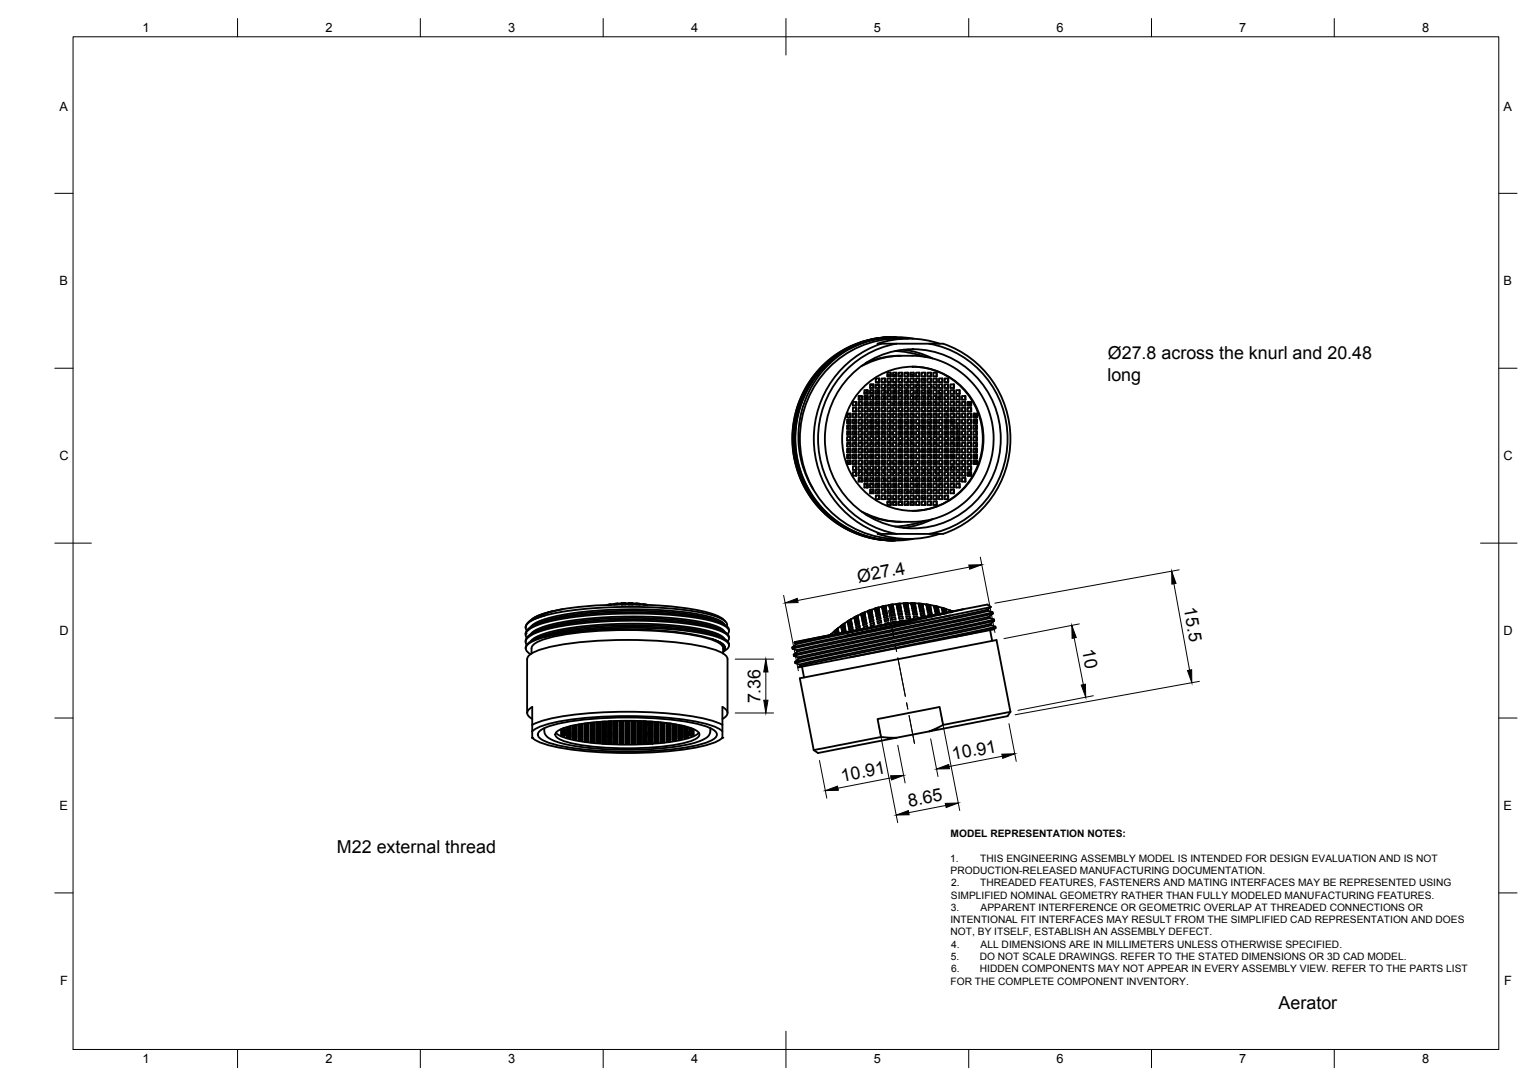
ISO-10303-21;
HEADER;
/* Generated by software containing ST-Developer
 * from STEP Tools, Inc. (www.steptools.com) 
 */

FILE_DESCRIPTION(
/* description */ ('STEP AP214'),
/* implementation_level */ '2;1');

FILE_NAME(
/* name */ 'Aerator.step',
/* time_stamp */ '2026-10-05T23:18:41-07:00',
/* author */ (''),
/* organization */ (''),
/* preprocessor_version */ 'ST-DEVELOPER v20.2',
/* originating_system */ 'Autodesk Translation Framework v15.15.0.0',
/* authorisation */ '');

FILE_SCHEMA (('AUTOMOTIVE_DESIGN { 1 0 10303 214 3 1 1 }'));
ENDSEC;

DATA;
#10=MECHANICAL_DESIGN_GEOMETRIC_PRESENTATION_REPRESENTATION('',(#110),#221662);
#71=MANIFOLD_SOLID_BREP('Body1',#79333);
#84=SHAPE_REPRESENTATION_RELATIONSHIP('SRR','None',#221719,#97);
#97=ADVANCED_BREP_SHAPE_REPRESENTATION('',(#71),#221659);
#110=STYLED_ITEM('',(#221783),#71);
#201=B_SPLINE_SURFACE_WITH_KNOTS('',3,3,((#184914,#184915,#184916,#184917,
#184918,#184919,#184920,#184921,#184922,#184923,#184924,#184925,#184926,
#184927,#184928,#184929,#184930,#184931,#184932,#184933,#184934,#184935,
#184936,#184937,#184938,#184939,#184940,#184941,#184942,#184943,#184944,
#184945,#184946,#184947,#184948),(#184949,#184950,#184951,#184952,#184953,
#184954,#184955,#184956,#184957,#184958,#184959,#184960,#184961,#184962,
#184963,#184964,#184965,#184966,#184967,#184968,#184969,#184970,#184971,
#184972,#184973,#184974,#184975,#184976,#184977,#184978,#184979,#184980,
#184981,#184982,#184983),(#184984,#184985,#184986,#184987,#184988,#184989,
#184990,#184991,#184992,#184993,#184994,#184995,#184996,#184997,#184998,
#184999,#185000,#185001,#185002,#185003,#185004,#185005,#185006,#185007,
#185008,#185009,#185010,#185011,#185012,#185013,#185014,#185015,#185016,
#185017,#185018),(#185019,#185020,#185021,#185022,#185023,#185024,#185025,
#185026,#185027,#185028,#185029,#185030,#185031,#185032,#185033,#185034,
#185035,#185036,#185037,#185038,#185039,#185040,#185041,#185042,#185043,
#185044,#185045,#185046,#185047,#185048,#185049,#185050,#185051,#185052,
#185053)),.UNSPECIFIED.,.F.,.F.,.F.,(4,4),(4,1,1,1,1,1,1,1,1,1,1,1,1,1,
1,1,1,1,1,1,1,1,1,1,1,1,1,1,1,1,1,1,4),(0.,1.),(0.,0.0312500000000065,0.0625000000000025,
0.0937500000000037,0.125000000000005,0.156250000000045,0.187500000000073,
0.218749999999969,0.249999999999997,0.281250000000024,0.312500000000052,
0.343750000000079,0.374999999999975,0.40625,0.43750000000003,0.468750000000058,
0.500000000000085,0.531249999999982,0.562500000000009,0.593750000000036,
0.625000000000064,0.656250000000091,0.687499999999988,0.718750000000015,
0.750000000000043,0.78125000000007,0.812500000000097,0.84375,0.875000000000021,
0.906250000000049,0.937500000000076,0.968750000000104,1.),.UNSPECIFIED.);
#202=B_SPLINE_SURFACE_WITH_KNOTS('',3,3,((#185513,#185514,#185515,#185516,
#185517,#185518,#185519,#185520,#185521,#185522,#185523,#185524,#185525,
#185526,#185527,#185528,#185529,#185530,#185531),(#185532,#185533,#185534,
#185535,#185536,#185537,#185538,#185539,#185540,#185541,#185542,#185543,
#185544,#185545,#185546,#185547,#185548,#185549,#185550),(#185551,#185552,
#185553,#185554,#185555,#185556,#185557,#185558,#185559,#185560,#185561,
#185562,#185563,#185564,#185565,#185566,#185567,#185568,#185569),(#185570,
#185571,#185572,#185573,#185574,#185575,#185576,#185577,#185578,#185579,
#185580,#185581,#185582,#185583,#185584,#185585,#185586,#185587,#185588)),
 .UNSPECIFIED.,.F.,.F.,.F.,(4,4),(4,1,1,1,1,1,1,1,1,1,1,1,1,1,1,1,4),(0.,
1.),(0.,0.0625000000000177,0.124999999999754,0.187499999999772,0.249999999999789,
0.312499999999525,0.374999999999543,0.437499999999561,0.499999999999297,
0.562499999999315,0.624999999999332,0.687499999999069,0.749999999999086,
0.812499999998822,0.87499999999884,0.937499999998858,1.),.UNSPECIFIED.);
#203=B_SPLINE_SURFACE_WITH_KNOTS('',3,3,((#185868,#185869,#185870,#185871,
#185872,#185873,#185874,#185875,#185876,#185877,#185878,#185879,#185880,
#185881,#185882,#185883,#185884,#185885,#185886,#185887,#185888,#185889,
#185890,#185891,#185892,#185893,#185894,#185895,#185896,#185897,#185898,
#185899,#185900,#185901,#185902),(#185903,#185904,#185905,#185906,#185907,
#185908,#185909,#185910,#185911,#185912,#185913,#185914,#185915,#185916,
#185917,#185918,#185919,#185920,#185921,#185922,#185923,#185924,#185925,
#185926,#185927,#185928,#185929,#185930,#185931,#185932,#185933,#185934,
#185935,#185936,#185937),(#185938,#185939,#185940,#185941,#185942,#185943,
#185944,#185945,#185946,#185947,#185948,#185949,#185950,#185951,#185952,
#185953,#185954,#185955,#185956,#185957,#185958,#185959,#185960,#185961,
#185962,#185963,#185964,#185965,#185966,#185967,#185968,#185969,#185970,
#185971,#185972),(#185973,#185974,#185975,#185976,#185977,#185978,#185979,
#185980,#185981,#185982,#185983,#185984,#185985,#185986,#185987,#185988,
#185989,#185990,#185991,#185992,#185993,#185994,#185995,#185996,#185997,
#185998,#185999,#186000,#186001,#186002,#186003,#186004,#186005,#186006,
#186007)),.UNSPECIFIED.,.F.,.F.,.F.,(4,4),(4,1,1,1,1,1,1,1,1,1,1,1,1,1,
1,1,1,1,1,1,1,1,1,1,1,1,1,1,1,1,1,1,4),(0.,1.),(0.,0.0312499999999954,0.0624999999999932,
0.0937499999999958,0.124999999999998,0.15625,0.187500000000028,0.218750000000055,
0.249999999999961,0.281249999999988,0.312500000000014,0.343750000000041,
0.375000000000068,0.406249999999974,0.4375,0.468750000000028,0.500000000000054,
0.531250000000081,0.562499999999987,0.593750000000014,0.625000000000041,
0.656250000000068,0.687499999999974,0.71875,0.750000000000027,0.781250000000054,
0.812500000000081,0.843749999999987,0.875000000000014,0.90625000000004,
0.937500000000067,0.968750000000094,1.),.UNSPECIFIED.);
#204=B_SPLINE_SURFACE_WITH_KNOTS('',3,3,((#186635,#186636,#186637,#186638,
#186639,#186640,#186641,#186642,#186643,#186644,#186645,#186646,#186647,
#186648,#186649,#186650,#186651,#186652,#186653,#186654,#186655,#186656,
#186657,#186658,#186659,#186660,#186661,#186662,#186663,#186664,#186665,
#186666,#186667,#186668,#186669,#186670,#186671,#186672,#186673,#186674,
#186675,#186676,#186677,#186678,#186679,#186680,#186681,#186682,#186683,
#186684,#186685,#186686,#186687,#186688,#186689,#186690,#186691,#186692,
#186693,#186694,#186695,#186696,#186697,#186698,#186699,#186700,#186701),
(#186702,#186703,#186704,#186705,#186706,#186707,#186708,#186709,#186710,
#186711,#186712,#186713,#186714,#186715,#186716,#186717,#186718,#186719,
#186720,#186721,#186722,#186723,#186724,#186725,#186726,#186727,#186728,
#186729,#186730,#186731,#186732,#186733,#186734,#186735,#186736,#186737,
#186738,#186739,#186740,#186741,#186742,#186743,#186744,#186745,#186746,
#186747,#186748,#186749,#186750,#186751,#186752,#186753,#186754,#186755,
#186756,#186757,#186758,#186759,#186760,#186761,#186762,#186763,#186764,
#186765,#186766,#186767,#186768),(#186769,#186770,#186771,#186772,#186773,
#186774,#186775,#186776,#186777,#186778,#186779,#186780,#186781,#186782,
#186783,#186784,#186785,#186786,#186787,#186788,#186789,#186790,#186791,
#186792,#186793,#186794,#186795,#186796,#186797,#186798,#186799,#186800,
#186801,#186802,#186803,#186804,#186805,#186806,#186807,#186808,#186809,
#186810,#186811,#186812,#186813,#186814,#186815,#186816,#186817,#186818,
#186819,#186820,#186821,#186822,#186823,#186824,#186825,#186826,#186827,
#186828,#186829,#186830,#186831,#186832,#186833,#186834,#186835),(#186836,
#186837,#186838,#186839,#186840,#186841,#186842,#186843,#186844,#186845,
#186846,#186847,#186848,#186849,#186850,#186851,#186852,#186853,#186854,
#186855,#186856,#186857,#186858,#186859,#186860,#186861,#186862,#186863,
#186864,#186865,#186866,#186867,#186868,#186869,#186870,#186871,#186872,
#186873,#186874,#186875,#186876,#186877,#186878,#186879,#186880,#186881,
#186882,#186883,#186884,#186885,#186886,#186887,#186888,#186889,#186890,
#186891,#186892,#186893,#186894,#186895,#186896,#186897,#186898,#186899,
#186900,#186901,#186902)),.UNSPECIFIED.,.F.,.F.,.F.,(4,4),(4,1,1,1,1,1,
1,1,1,1,1,1,1,1,1,1,1,1,1,1,1,1,1,1,1,1,1,1,1,1,1,1,1,1,1,1,1,1,1,1,1,1,
1,1,1,1,1,1,1,1,1,1,1,1,1,1,1,1,1,1,1,1,1,1,4),(0.,1.),(0.,0.0156250000000016,
0.031250000000001,0.0468750000000015,0.062500000000002,0.0781250000000025,
0.093750000000003,0.109375000000004,0.125000000000004,0.140625000000026,
0.156249999999973,0.171875000000027,0.187499999999974,0.203125000000028,
0.218749999999975,0.234375000000029,0.249999999999976,0.26562500000003,
0.281249999999977,0.296875000000031,0.312499999999978,0.328125000000032,
0.343749999999979,0.359375000000033,0.37499999999998,0.390625000000034,
0.406249999999981,0.421875000000035,0.437499999999982,0.453125000000036,
0.468749999999983,0.484375000000037,0.499999999999984,0.515625000000038,
0.531249999999985,0.546875000000039,0.562499999999986,0.57812500000004,
0.593749999999987,0.609375000000041,0.624999999999988,0.640625000000042,
0.656249999999989,0.671875000000043,0.68749999999999,0.703125000000044,
0.718749999999991,0.734375000000045,0.749999999999992,0.765625000000046,
0.78125,0.796875000000047,0.8125,0.828125000000048,0.84375,0.859374999999941,
0.875,0.890624999999943,0.90625,0.921874999999943,0.9375,0.953124999999945,
0.96875,0.984374999999945,1.),.UNSPECIFIED.);
#205=B_SPLINE_SURFACE_WITH_KNOTS('',3,3,((#186905,#186906,#186907,#186908,
#186909,#186910,#186911,#186912,#186913,#186914,#186915,#186916,#186917,
#186918,#186919,#186920,#186921,#186922,#186923),(#186924,#186925,#186926,
#186927,#186928,#186929,#186930,#186931,#186932,#186933,#186934,#186935,
#186936,#186937,#186938,#186939,#186940,#186941,#186942),(#186943,#186944,
#186945,#186946,#186947,#186948,#186949,#186950,#186951,#186952,#186953,
#186954,#186955,#186956,#186957,#186958,#186959,#186960,#186961),(#186962,
#186963,#186964,#186965,#186966,#186967,#186968,#186969,#186970,#186971,
#186972,#186973,#186974,#186975,#186976,#186977,#186978,#186979,#186980)),
 .UNSPECIFIED.,.F.,.F.,.F.,(4,4),(4,1,1,1,1,1,1,1,1,1,1,1,1,1,1,1,4),(0.,
1.),(0.,0.062499999999931,0.124999999999862,0.187500000000069,0.25,0.312499999999931,
0.374999999999862,0.437499999999793,0.499999999999724,0.562499999999931,
0.624999999999862,0.687499999999793,0.749999999999724,0.812499999999656,
0.874999999999587,0.937499999999793,1.),.UNSPECIFIED.);
#206=B_SPLINE_SURFACE_WITH_KNOTS('',3,3,((#186987,#186988,#186989,#186990,
#186991,#186992,#186993,#186994,#186995,#186996,#186997,#186998,#186999,
#187000,#187001,#187002,#187003,#187004,#187005),(#187006,#187007,#187008,
#187009,#187010,#187011,#187012,#187013,#187014,#187015,#187016,#187017,
#187018,#187019,#187020,#187021,#187022,#187023,#187024),(#187025,#187026,
#187027,#187028,#187029,#187030,#187031,#187032,#187033,#187034,#187035,
#187036,#187037,#187038,#187039,#187040,#187041,#187042,#187043),(#187044,
#187045,#187046,#187047,#187048,#187049,#187050,#187051,#187052,#187053,
#187054,#187055,#187056,#187057,#187058,#187059,#187060,#187061,#187062)),
 .UNSPECIFIED.,.F.,.F.,.F.,(4,4),(4,1,1,1,1,1,1,1,1,1,1,1,1,1,1,1,4),(0.,
1.),(0.,0.0625000000000641,0.125000000000129,0.18749999999985,0.249999999999914,
0.312499999999979,0.3749999999997,0.437499999999764,0.499999999999828,0.562499999999549,
0.624999999999614,0.687499999999335,0.749999999999399,0.812499999999464,
0.874999999999185,0.937499999999249,1.),.UNSPECIFIED.);
#319=FACE_BOUND('',#24953,.T.);
#320=FACE_BOUND('',#24954,.T.);
#321=FACE_BOUND('',#24955,.T.);
#322=FACE_BOUND('',#24959,.T.);
#323=FACE_BOUND('',#24960,.T.);
#324=FACE_BOUND('',#24961,.T.);
#325=FACE_BOUND('',#24984,.T.);
#326=FACE_BOUND('',#24986,.T.);
#327=FACE_BOUND('',#24992,.T.);
#328=FACE_BOUND('',#24994,.T.);
#329=FACE_BOUND('',#24996,.T.);
#330=FACE_BOUND('',#26056,.T.);
#331=FACE_BOUND('',#27802,.T.);
#332=FACE_BOUND('',#27804,.T.);
#333=FACE_BOUND('',#27805,.T.);
#334=FACE_BOUND('',#27806,.T.);
#335=FACE_BOUND('',#27807,.T.);
#336=FACE_BOUND('',#27808,.T.);
#337=FACE_BOUND('',#27809,.T.);
#338=FACE_BOUND('',#27810,.T.);
#339=FACE_BOUND('',#27811,.T.);
#340=FACE_BOUND('',#27812,.T.);
#341=FACE_BOUND('',#27813,.T.);
#342=FACE_BOUND('',#27814,.T.);
#343=FACE_BOUND('',#27815,.T.);
#344=FACE_BOUND('',#27816,.T.);
#345=FACE_BOUND('',#27817,.T.);
#346=FACE_BOUND('',#27818,.T.);
#347=FACE_BOUND('',#27819,.T.);
#348=FACE_BOUND('',#27820,.T.);
#349=FACE_BOUND('',#27821,.T.);
#350=FACE_BOUND('',#27822,.T.);
#351=FACE_BOUND('',#27823,.T.);
#352=FACE_BOUND('',#27824,.T.);
#353=FACE_BOUND('',#27825,.T.);
#354=FACE_BOUND('',#27826,.T.);
#355=FACE_BOUND('',#27827,.T.);
#356=FACE_BOUND('',#27828,.T.);
#357=FACE_BOUND('',#27829,.T.);
#358=FACE_BOUND('',#27830,.T.);
#359=FACE_BOUND('',#27831,.T.);
#360=FACE_BOUND('',#27832,.T.);
#361=FACE_BOUND('',#27833,.T.);
#362=FACE_BOUND('',#27834,.T.);
#363=FACE_BOUND('',#27835,.T.);
#364=FACE_BOUND('',#27836,.T.);
#365=FACE_BOUND('',#27837,.T.);
#366=FACE_BOUND('',#27838,.T.);
#367=FACE_BOUND('',#27839,.T.);
#368=FACE_BOUND('',#27840,.T.);
#369=FACE_BOUND('',#27841,.T.);
#370=FACE_BOUND('',#27842,.T.);
#371=FACE_BOUND('',#27843,.T.);
#372=FACE_BOUND('',#27844,.T.);
#373=FACE_BOUND('',#27845,.T.);
#374=FACE_BOUND('',#27846,.T.);
#375=FACE_BOUND('',#27847,.T.);
#376=FACE_BOUND('',#27848,.T.);
#377=FACE_BOUND('',#27849,.T.);
#378=FACE_BOUND('',#27850,.T.);
#379=FACE_BOUND('',#27851,.T.);
#380=FACE_BOUND('',#27852,.T.);
#381=FACE_BOUND('',#27853,.T.);
#382=FACE_BOUND('',#27854,.T.);
#383=FACE_BOUND('',#27855,.T.);
#384=FACE_BOUND('',#27856,.T.);
#385=FACE_BOUND('',#27857,.T.);
#386=FACE_BOUND('',#27858,.T.);
#387=FACE_BOUND('',#27859,.T.);
#388=FACE_BOUND('',#27860,.T.);
#389=FACE_BOUND('',#27861,.T.);
#390=FACE_BOUND('',#27862,.T.);
#391=FACE_BOUND('',#27863,.T.);
#392=FACE_BOUND('',#27864,.T.);
#393=FACE_BOUND('',#27865,.T.);
#394=FACE_BOUND('',#27866,.T.);
#395=FACE_BOUND('',#27867,.T.);
#396=FACE_BOUND('',#27868,.T.);
#397=FACE_BOUND('',#27869,.T.);
#398=FACE_BOUND('',#27870,.T.);
#399=FACE_BOUND('',#27871,.T.);
#400=FACE_BOUND('',#27872,.T.);
#401=FACE_BOUND('',#27873,.T.);
#402=FACE_BOUND('',#27874,.T.);
#403=FACE_BOUND('',#27875,.T.);
#404=FACE_BOUND('',#27876,.T.);
#405=FACE_BOUND('',#27877,.T.);
#406=FACE_BOUND('',#27878,.T.);
#407=FACE_BOUND('',#27879,.T.);
#408=FACE_BOUND('',#27880,.T.);
#409=FACE_BOUND('',#27881,.T.);
#410=FACE_BOUND('',#27882,.T.);
#411=FACE_BOUND('',#27883,.T.);
#412=FACE_BOUND('',#27884,.T.);
#413=FACE_BOUND('',#27885,.T.);
#414=FACE_BOUND('',#27886,.T.);
#415=FACE_BOUND('',#27887,.T.);
#416=FACE_BOUND('',#27888,.T.);
#417=FACE_BOUND('',#27889,.T.);
#418=FACE_BOUND('',#27890,.T.);
#419=FACE_BOUND('',#27891,.T.);
#420=FACE_BOUND('',#27892,.T.);
#421=FACE_BOUND('',#27893,.T.);
#422=FACE_BOUND('',#27894,.T.);
#423=FACE_BOUND('',#27895,.T.);
#424=FACE_BOUND('',#27896,.T.);
#425=FACE_BOUND('',#27897,.T.);
#426=FACE_BOUND('',#27898,.T.);
#427=FACE_BOUND('',#27899,.T.);
#428=FACE_BOUND('',#27900,.T.);
#429=FACE_BOUND('',#27901,.T.);
#430=FACE_BOUND('',#27902,.T.);
#431=FACE_BOUND('',#27903,.T.);
#432=FACE_BOUND('',#27904,.T.);
#433=FACE_BOUND('',#27905,.T.);
#434=FACE_BOUND('',#27906,.T.);
#435=FACE_BOUND('',#27907,.T.);
#436=FACE_BOUND('',#27908,.T.);
#437=FACE_BOUND('',#27909,.T.);
#438=FACE_BOUND('',#27910,.T.);
#439=FACE_BOUND('',#27911,.T.);
#440=FACE_BOUND('',#27912,.T.);
#441=FACE_BOUND('',#27913,.T.);
#442=FACE_BOUND('',#27914,.T.);
#443=FACE_BOUND('',#27915,.T.);
#444=FACE_BOUND('',#27916,.T.);
#445=FACE_BOUND('',#27917,.T.);
#446=FACE_BOUND('',#27918,.T.);
#447=FACE_BOUND('',#27919,.T.);
#448=FACE_BOUND('',#27920,.T.);
#449=FACE_BOUND('',#27921,.T.);
#450=FACE_BOUND('',#27922,.T.);
#451=FACE_BOUND('',#27923,.T.);
#452=FACE_BOUND('',#27924,.T.);
#453=FACE_BOUND('',#27925,.T.);
#454=FACE_BOUND('',#27926,.T.);
#455=FACE_BOUND('',#27927,.T.);
#456=FACE_BOUND('',#27928,.T.);
#457=FACE_BOUND('',#27929,.T.);
#458=FACE_BOUND('',#27930,.T.);
#459=FACE_BOUND('',#27931,.T.);
#460=FACE_BOUND('',#27932,.T.);
#461=FACE_BOUND('',#27933,.T.);
#462=FACE_BOUND('',#27934,.T.);
#463=FACE_BOUND('',#27935,.T.);
#464=FACE_BOUND('',#27936,.T.);
#465=FACE_BOUND('',#27937,.T.);
#466=FACE_BOUND('',#27938,.T.);
#467=FACE_BOUND('',#27939,.T.);
#468=FACE_BOUND('',#27940,.T.);
#469=FACE_BOUND('',#27941,.T.);
#470=FACE_BOUND('',#27942,.T.);
#471=FACE_BOUND('',#27943,.T.);
#472=FACE_BOUND('',#27944,.T.);
#473=FACE_BOUND('',#27945,.T.);
#474=FACE_BOUND('',#27946,.T.);
#475=FACE_BOUND('',#27947,.T.);
#476=FACE_BOUND('',#27948,.T.);
#477=FACE_BOUND('',#27949,.T.);
#478=FACE_BOUND('',#27950,.T.);
#479=FACE_BOUND('',#27951,.T.);
#480=FACE_BOUND('',#27952,.T.);
#481=FACE_BOUND('',#27953,.T.);
#482=FACE_BOUND('',#27954,.T.);
#483=FACE_BOUND('',#27955,.T.);
#484=FACE_BOUND('',#27956,.T.);
#485=FACE_BOUND('',#27957,.T.);
#486=FACE_BOUND('',#27958,.T.);
#487=FACE_BOUND('',#27959,.T.);
#488=FACE_BOUND('',#27960,.T.);
#489=FACE_BOUND('',#27961,.T.);
#490=FACE_BOUND('',#27962,.T.);
#491=FACE_BOUND('',#27963,.T.);
#492=FACE_BOUND('',#27964,.T.);
#493=FACE_BOUND('',#27965,.T.);
#494=FACE_BOUND('',#27966,.T.);
#495=FACE_BOUND('',#27967,.T.);
#496=FACE_BOUND('',#27968,.T.);
#497=FACE_BOUND('',#27969,.T.);
#498=FACE_BOUND('',#27970,.T.);
#499=FACE_BOUND('',#27971,.T.);
#500=FACE_BOUND('',#27972,.T.);
#501=FACE_BOUND('',#27973,.T.);
#502=FACE_BOUND('',#27974,.T.);
#503=FACE_BOUND('',#27975,.T.);
#504=FACE_BOUND('',#27976,.T.);
#505=FACE_BOUND('',#27977,.T.);
#506=FACE_BOUND('',#27978,.T.);
#507=FACE_BOUND('',#27979,.T.);
#508=FACE_BOUND('',#27980,.T.);
#509=FACE_BOUND('',#27981,.T.);
#510=FACE_BOUND('',#27982,.T.);
#511=FACE_BOUND('',#27983,.T.);
#512=FACE_BOUND('',#27984,.T.);
#513=FACE_BOUND('',#27985,.T.);
#514=FACE_BOUND('',#27986,.T.);
#515=FACE_BOUND('',#27987,.T.);
#516=FACE_BOUND('',#27988,.T.);
#517=FACE_BOUND('',#27989,.T.);
#518=FACE_BOUND('',#27990,.T.);
#519=FACE_BOUND('',#27991,.T.);
#520=FACE_BOUND('',#27992,.T.);
#521=FACE_BOUND('',#27993,.T.);
#522=FACE_BOUND('',#27994,.T.);
#523=FACE_BOUND('',#27995,.T.);
#524=FACE_BOUND('',#27996,.T.);
#525=FACE_BOUND('',#27997,.T.);
#526=FACE_BOUND('',#27998,.T.);
#527=FACE_BOUND('',#27999,.T.);
#528=FACE_BOUND('',#28000,.T.);
#529=FACE_BOUND('',#28001,.T.);
#530=FACE_BOUND('',#28002,.T.);
#531=FACE_BOUND('',#28003,.T.);
#532=FACE_BOUND('',#28004,.T.);
#533=FACE_BOUND('',#28005,.T.);
#534=FACE_BOUND('',#28006,.T.);
#535=FACE_BOUND('',#28007,.T.);
#536=FACE_BOUND('',#28008,.T.);
#537=FACE_BOUND('',#28009,.T.);
#538=FACE_BOUND('',#28010,.T.);
#539=FACE_BOUND('',#28011,.T.);
#540=FACE_BOUND('',#28012,.T.);
#541=FACE_BOUND('',#28013,.T.);
#542=FACE_BOUND('',#28014,.T.);
#543=FACE_BOUND('',#28015,.T.);
#544=FACE_BOUND('',#28016,.T.);
#545=FACE_BOUND('',#28017,.T.);
#546=FACE_BOUND('',#28018,.T.);
#547=FACE_BOUND('',#28019,.T.);
#548=FACE_BOUND('',#28020,.T.);
#549=FACE_BOUND('',#28021,.T.);
#550=FACE_BOUND('',#28022,.T.);
#551=FACE_BOUND('',#28023,.T.);
#552=FACE_BOUND('',#28024,.T.);
#553=FACE_BOUND('',#28025,.T.);
#554=FACE_BOUND('',#28026,.T.);
#555=FACE_BOUND('',#28027,.T.);
#556=FACE_BOUND('',#28028,.T.);
#557=FACE_BOUND('',#28029,.T.);
#558=FACE_BOUND('',#28030,.T.);
#559=FACE_BOUND('',#28031,.T.);
#560=FACE_BOUND('',#28032,.T.);
#561=FACE_BOUND('',#28033,.T.);
#562=FACE_BOUND('',#28034,.T.);
#563=FACE_BOUND('',#28035,.T.);
#564=FACE_BOUND('',#28036,.T.);
#565=FACE_BOUND('',#28037,.T.);
#566=FACE_BOUND('',#28038,.T.);
#567=FACE_BOUND('',#28039,.T.);
#568=FACE_BOUND('',#28040,.T.);
#569=FACE_BOUND('',#28041,.T.);
#570=FACE_BOUND('',#28042,.T.);
#571=FACE_BOUND('',#28043,.T.);
#572=FACE_BOUND('',#28044,.T.);
#573=FACE_BOUND('',#28045,.T.);
#574=FACE_BOUND('',#28046,.T.);
#575=FACE_BOUND('',#28047,.T.);
#576=FACE_BOUND('',#28048,.T.);
#577=FACE_BOUND('',#28049,.T.);
#578=FACE_BOUND('',#28050,.T.);
#579=FACE_BOUND('',#28051,.T.);
#580=FACE_BOUND('',#28052,.T.);
#581=FACE_BOUND('',#28053,.T.);
#582=FACE_BOUND('',#28054,.T.);
#583=FACE_BOUND('',#28055,.T.);
#584=FACE_BOUND('',#28056,.T.);
#585=FACE_BOUND('',#28057,.T.);
#586=FACE_BOUND('',#28058,.T.);
#587=FACE_BOUND('',#28059,.T.);
#588=FACE_BOUND('',#28060,.T.);
#589=FACE_BOUND('',#28061,.T.);
#590=FACE_BOUND('',#28062,.T.);
#591=FACE_BOUND('',#28063,.T.);
#592=FACE_BOUND('',#28064,.T.);
#593=FACE_BOUND('',#28065,.T.);
#594=FACE_BOUND('',#28066,.T.);
#595=FACE_BOUND('',#28067,.T.);
#596=FACE_BOUND('',#28068,.T.);
#597=FACE_BOUND('',#28069,.T.);
#598=FACE_BOUND('',#28070,.T.);
#599=FACE_BOUND('',#28071,.T.);
#600=FACE_BOUND('',#28072,.T.);
#601=FACE_BOUND('',#28073,.T.);
#602=FACE_BOUND('',#28074,.T.);
#603=FACE_BOUND('',#28075,.T.);
#604=FACE_BOUND('',#28076,.T.);
#605=FACE_BOUND('',#28077,.T.);
#606=FACE_BOUND('',#28078,.T.);
#607=FACE_BOUND('',#28079,.T.);
#608=FACE_BOUND('',#28080,.T.);
#609=FACE_BOUND('',#28081,.T.);
#610=FACE_BOUND('',#28082,.T.);
#611=FACE_BOUND('',#28083,.T.);
#612=FACE_BOUND('',#28084,.T.);
#613=FACE_BOUND('',#28085,.T.);
#614=FACE_BOUND('',#28086,.T.);
#615=FACE_BOUND('',#28087,.T.);
#616=FACE_BOUND('',#28088,.T.);
#617=FACE_BOUND('',#28089,.T.);
#618=FACE_BOUND('',#28090,.T.);
#619=FACE_BOUND('',#28091,.T.);
#620=FACE_BOUND('',#28092,.T.);
#621=FACE_BOUND('',#28093,.T.);
#622=FACE_BOUND('',#28094,.T.);
#623=FACE_BOUND('',#28095,.T.);
#624=FACE_BOUND('',#28096,.T.);
#625=FACE_BOUND('',#28097,.T.);
#626=FACE_BOUND('',#28098,.T.);
#627=FACE_BOUND('',#28099,.T.);
#628=FACE_BOUND('',#28100,.T.);
#629=FACE_BOUND('',#28101,.T.);
#630=FACE_BOUND('',#28102,.T.);
#631=FACE_BOUND('',#28103,.T.);
#632=FACE_BOUND('',#28104,.T.);
#633=FACE_BOUND('',#28105,.T.);
#634=FACE_BOUND('',#28106,.T.);
#635=FACE_BOUND('',#28107,.T.);
#636=FACE_BOUND('',#28108,.T.);
#637=FACE_BOUND('',#28109,.T.);
#638=FACE_BOUND('',#28110,.T.);
#639=FACE_BOUND('',#28111,.T.);
#640=FACE_BOUND('',#28112,.T.);
#641=FACE_BOUND('',#28113,.T.);
#642=FACE_BOUND('',#28114,.T.);
#643=FACE_BOUND('',#28115,.T.);
#644=FACE_BOUND('',#28116,.T.);
#645=FACE_BOUND('',#28117,.T.);
#646=FACE_BOUND('',#28118,.T.);
#647=FACE_BOUND('',#28119,.T.);
#648=FACE_BOUND('',#28120,.T.);
#649=FACE_BOUND('',#28121,.T.);
#650=FACE_BOUND('',#28122,.T.);
#651=FACE_BOUND('',#28123,.T.);
#652=FACE_BOUND('',#28124,.T.);
#653=FACE_BOUND('',#28125,.T.);
#654=FACE_BOUND('',#28126,.T.);
#655=FACE_BOUND('',#28127,.T.);
#656=FACE_BOUND('',#28128,.T.);
#657=FACE_BOUND('',#28129,.T.);
#658=FACE_BOUND('',#28130,.T.);
#659=FACE_BOUND('',#28131,.T.);
#660=FACE_BOUND('',#28132,.T.);
#661=FACE_BOUND('',#28133,.T.);
#662=FACE_BOUND('',#28134,.T.);
#663=FACE_BOUND('',#28135,.T.);
#664=FACE_BOUND('',#28136,.T.);
#665=FACE_BOUND('',#28137,.T.);
#666=FACE_BOUND('',#28138,.T.);
#667=FACE_BOUND('',#28139,.T.);
#668=FACE_BOUND('',#28140,.T.);
#669=FACE_BOUND('',#28141,.T.);
#670=FACE_BOUND('',#28142,.T.);
#671=FACE_BOUND('',#28143,.T.);
#672=FACE_BOUND('',#28144,.T.);
#673=FACE_BOUND('',#28145,.T.);
#674=FACE_BOUND('',#28146,.T.);
#675=FACE_BOUND('',#28147,.T.);
#676=FACE_BOUND('',#28148,.T.);
#677=FACE_BOUND('',#28149,.T.);
#678=FACE_BOUND('',#28150,.T.);
#679=FACE_BOUND('',#28151,.T.);
#680=FACE_BOUND('',#28152,.T.);
#681=FACE_BOUND('',#28153,.T.);
#682=FACE_BOUND('',#28154,.T.);
#683=FACE_BOUND('',#28155,.T.);
#684=FACE_BOUND('',#28156,.T.);
#685=FACE_BOUND('',#28157,.T.);
#686=FACE_BOUND('',#28158,.T.);
#687=FACE_BOUND('',#28159,.T.);
#688=FACE_BOUND('',#28160,.T.);
#689=FACE_BOUND('',#28161,.T.);
#690=FACE_BOUND('',#28162,.T.);
#691=FACE_BOUND('',#28163,.T.);
#692=FACE_BOUND('',#28164,.T.);
#693=FACE_BOUND('',#28165,.T.);
#694=FACE_BOUND('',#28166,.T.);
#695=FACE_BOUND('',#28167,.T.);
#696=FACE_BOUND('',#28168,.T.);
#697=FACE_BOUND('',#28169,.T.);
#698=FACE_BOUND('',#28170,.T.);
#699=FACE_BOUND('',#28171,.T.);
#700=FACE_BOUND('',#28172,.T.);
#701=FACE_BOUND('',#28173,.T.);
#702=FACE_BOUND('',#28174,.T.);
#703=FACE_BOUND('',#28175,.T.);
#704=FACE_BOUND('',#28176,.T.);
#705=FACE_BOUND('',#28177,.T.);
#706=FACE_BOUND('',#28178,.T.);
#707=FACE_BOUND('',#28179,.T.);
#708=FACE_BOUND('',#28180,.T.);
#709=FACE_BOUND('',#28181,.T.);
#710=FACE_BOUND('',#28182,.T.);
#711=FACE_BOUND('',#28183,.T.);
#712=FACE_BOUND('',#28184,.T.);
#713=FACE_BOUND('',#28185,.T.);
#714=FACE_BOUND('',#28186,.T.);
#715=FACE_BOUND('',#28187,.T.);
#716=FACE_BOUND('',#28188,.T.);
#717=FACE_BOUND('',#28189,.T.);
#718=FACE_BOUND('',#28190,.T.);
#719=FACE_BOUND('',#28191,.T.);
#720=FACE_BOUND('',#28192,.T.);
#721=FACE_BOUND('',#28193,.T.);
#722=FACE_BOUND('',#28194,.T.);
#723=FACE_BOUND('',#28195,.T.);
#724=FACE_BOUND('',#28196,.T.);
#725=FACE_BOUND('',#28197,.T.);
#726=FACE_BOUND('',#28198,.T.);
#727=FACE_BOUND('',#28199,.T.);
#728=FACE_BOUND('',#28200,.T.);
#729=FACE_BOUND('',#28201,.T.);
#730=FACE_BOUND('',#28202,.T.);
#731=FACE_BOUND('',#28203,.T.);
#732=FACE_BOUND('',#28204,.T.);
#733=FACE_BOUND('',#28205,.T.);
#734=FACE_BOUND('',#28206,.T.);
#735=FACE_BOUND('',#28207,.T.);
#736=FACE_BOUND('',#28208,.T.);
#737=FACE_BOUND('',#28209,.T.);
#738=FACE_BOUND('',#28210,.T.);
#739=FACE_BOUND('',#28211,.T.);
#740=FACE_BOUND('',#28212,.T.);
#741=FACE_BOUND('',#28213,.T.);
#742=FACE_BOUND('',#28214,.T.);
#743=FACE_BOUND('',#28215,.T.);
#744=FACE_BOUND('',#28216,.T.);
#745=FACE_BOUND('',#28217,.T.);
#746=FACE_BOUND('',#28218,.T.);
#747=FACE_BOUND('',#28219,.T.);
#748=FACE_BOUND('',#28220,.T.);
#749=FACE_BOUND('',#28221,.T.);
#750=FACE_BOUND('',#28222,.T.);
#751=FACE_BOUND('',#28223,.T.);
#752=FACE_BOUND('',#28224,.T.);
#753=FACE_BOUND('',#28225,.T.);
#754=FACE_BOUND('',#28226,.T.);
#755=FACE_BOUND('',#28227,.T.);
#756=FACE_BOUND('',#28228,.T.);
#757=FACE_BOUND('',#28229,.T.);
#758=FACE_BOUND('',#28230,.T.);
#759=FACE_BOUND('',#28231,.T.);
#760=FACE_BOUND('',#28232,.T.);
#761=FACE_BOUND('',#28233,.T.);
#762=FACE_BOUND('',#28234,.T.);
#763=FACE_BOUND('',#28235,.T.);
#764=FACE_BOUND('',#28236,.T.);
#765=FACE_BOUND('',#28237,.T.);
#766=FACE_BOUND('',#28238,.T.);
#767=FACE_BOUND('',#28239,.T.);
#768=FACE_BOUND('',#28240,.T.);
#769=FACE_BOUND('',#28246,.T.);
#770=FACE_BOUND('',#28247,.T.);
#771=FACE_BOUND('',#28248,.T.);
#772=FACE_BOUND('',#28249,.T.);
#773=FACE_BOUND('',#28250,.T.);
#774=FACE_BOUND('',#28251,.T.);
#775=FACE_BOUND('',#28252,.T.);
#776=FACE_BOUND('',#28253,.T.);
#777=FACE_BOUND('',#28254,.T.);
#778=FACE_BOUND('',#28255,.T.);
#779=FACE_BOUND('',#28256,.T.);
#780=FACE_BOUND('',#28257,.T.);
#781=FACE_BOUND('',#28258,.T.);
#782=FACE_BOUND('',#28259,.T.);
#783=FACE_BOUND('',#28260,.T.);
#784=FACE_BOUND('',#28261,.T.);
#785=FACE_BOUND('',#28262,.T.);
#786=FACE_BOUND('',#28263,.T.);
#787=FACE_BOUND('',#28264,.T.);
#788=FACE_BOUND('',#28265,.T.);
#789=FACE_BOUND('',#28266,.T.);
#790=FACE_BOUND('',#28267,.T.);
#791=FACE_BOUND('',#28268,.T.);
#792=FACE_BOUND('',#28269,.T.);
#793=FACE_BOUND('',#28270,.T.);
#794=FACE_BOUND('',#28271,.T.);
#795=FACE_BOUND('',#28272,.T.);
#796=FACE_BOUND('',#28273,.T.);
#797=FACE_BOUND('',#28274,.T.);
#798=FACE_BOUND('',#28275,.T.);
#799=FACE_BOUND('',#28276,.T.);
#800=FACE_BOUND('',#28277,.T.);
#801=FACE_BOUND('',#28278,.T.);
#802=FACE_BOUND('',#28279,.T.);
#803=FACE_BOUND('',#28280,.T.);
#804=FACE_BOUND('',#28281,.T.);
#805=FACE_BOUND('',#28282,.T.);
#806=FACE_BOUND('',#28283,.T.);
#807=FACE_BOUND('',#28284,.T.);
#808=FACE_BOUND('',#28285,.T.);
#809=FACE_BOUND('',#28286,.T.);
#810=FACE_BOUND('',#28287,.T.);
#811=FACE_BOUND('',#28288,.T.);
#812=FACE_BOUND('',#28289,.T.);
#813=FACE_BOUND('',#28290,.T.);
#814=FACE_BOUND('',#28291,.T.);
#815=FACE_BOUND('',#28292,.T.);
#816=FACE_BOUND('',#28293,.T.);
#817=FACE_BOUND('',#28294,.T.);
#818=FACE_BOUND('',#28295,.T.);
#819=FACE_BOUND('',#28296,.T.);
#820=FACE_BOUND('',#28297,.T.);
#821=FACE_BOUND('',#28298,.T.);
#822=FACE_BOUND('',#28299,.T.);
#823=FACE_BOUND('',#28300,.T.);
#824=FACE_BOUND('',#28301,.T.);
#825=FACE_BOUND('',#28302,.T.);
#826=FACE_BOUND('',#28303,.T.);
#827=FACE_BOUND('',#28304,.T.);
#828=FACE_BOUND('',#28305,.T.);
#829=FACE_BOUND('',#28306,.T.);
#830=FACE_BOUND('',#28307,.T.);
#831=FACE_BOUND('',#28308,.T.);
#832=FACE_BOUND('',#28309,.T.);
#833=FACE_BOUND('',#28310,.T.);
#834=FACE_BOUND('',#28311,.T.);
#835=FACE_BOUND('',#28312,.T.);
#836=FACE_BOUND('',#28313,.T.);
#837=FACE_BOUND('',#28314,.T.);
#838=FACE_BOUND('',#28315,.T.);
#839=FACE_BOUND('',#28316,.T.);
#840=FACE_BOUND('',#28317,.T.);
#841=FACE_BOUND('',#28318,.T.);
#842=FACE_BOUND('',#28319,.T.);
#843=FACE_BOUND('',#28320,.T.);
#844=FACE_BOUND('',#28321,.T.);
#845=FACE_BOUND('',#28322,.T.);
#846=FACE_BOUND('',#28323,.T.);
#847=FACE_BOUND('',#28324,.T.);
#848=FACE_BOUND('',#28325,.T.);
#849=FACE_BOUND('',#28326,.T.);
#850=FACE_BOUND('',#28327,.T.);
#851=FACE_BOUND('',#28328,.T.);
#852=FACE_BOUND('',#28329,.T.);
#853=FACE_BOUND('',#28330,.T.);
#854=FACE_BOUND('',#28331,.T.);
#855=FACE_BOUND('',#28332,.T.);
#856=FACE_BOUND('',#28333,.T.);
#857=FACE_BOUND('',#28334,.T.);
#858=FACE_BOUND('',#28335,.T.);
#859=FACE_BOUND('',#28336,.T.);
#860=FACE_BOUND('',#28337,.T.);
#861=FACE_BOUND('',#28338,.T.);
#862=FACE_BOUND('',#28339,.T.);
#863=FACE_BOUND('',#28340,.T.);
#864=FACE_BOUND('',#28341,.T.);
#865=FACE_BOUND('',#28342,.T.);
#866=FACE_BOUND('',#28343,.T.);
#867=FACE_BOUND('',#28344,.T.);
#868=FACE_BOUND('',#28345,.T.);
#869=FACE_BOUND('',#28346,.T.);
#870=FACE_BOUND('',#28347,.T.);
#871=FACE_BOUND('',#28348,.T.);
#872=FACE_BOUND('',#28349,.T.);
#873=FACE_BOUND('',#28350,.T.);
#874=FACE_BOUND('',#28351,.T.);
#875=FACE_BOUND('',#28352,.T.);
#876=FACE_BOUND('',#28353,.T.);
#877=FACE_BOUND('',#28354,.T.);
#878=FACE_BOUND('',#28355,.T.);
#879=FACE_BOUND('',#28356,.T.);
#880=FACE_BOUND('',#28357,.T.);
#881=FACE_BOUND('',#28358,.T.);
#882=FACE_BOUND('',#28359,.T.);
#883=FACE_BOUND('',#28360,.T.);
#884=FACE_BOUND('',#28361,.T.);
#885=FACE_BOUND('',#28362,.T.);
#886=FACE_BOUND('',#28363,.T.);
#887=FACE_BOUND('',#28364,.T.);
#888=FACE_BOUND('',#28365,.T.);
#889=FACE_BOUND('',#28366,.T.);
#890=FACE_BOUND('',#28367,.T.);
#891=FACE_BOUND('',#28368,.T.);
#892=FACE_BOUND('',#28369,.T.);
#893=FACE_BOUND('',#28370,.T.);
#894=FACE_BOUND('',#28371,.T.);
#895=FACE_BOUND('',#28372,.T.);
#896=FACE_BOUND('',#28373,.T.);
#897=FACE_BOUND('',#28374,.T.);
#898=FACE_BOUND('',#28375,.T.);
#899=FACE_BOUND('',#28376,.T.);
#900=FACE_BOUND('',#28377,.T.);
#901=FACE_BOUND('',#28378,.T.);
#902=FACE_BOUND('',#28379,.T.);
#903=FACE_BOUND('',#28380,.T.);
#904=FACE_BOUND('',#28381,.T.);
#905=FACE_BOUND('',#28382,.T.);
#906=FACE_BOUND('',#28383,.T.);
#907=FACE_BOUND('',#28384,.T.);
#908=FACE_BOUND('',#28385,.T.);
#909=FACE_BOUND('',#28386,.T.);
#910=FACE_BOUND('',#28387,.T.);
#911=FACE_BOUND('',#28388,.T.);
#912=FACE_BOUND('',#28389,.T.);
#913=FACE_BOUND('',#28390,.T.);
#914=FACE_BOUND('',#28391,.T.);
#915=FACE_BOUND('',#28392,.T.);
#916=FACE_BOUND('',#28393,.T.);
#917=FACE_BOUND('',#28394,.T.);
#918=FACE_BOUND('',#28395,.T.);
#919=FACE_BOUND('',#28396,.T.);
#920=FACE_BOUND('',#28397,.T.);
#921=FACE_BOUND('',#28398,.T.);
#922=FACE_BOUND('',#28399,.T.);
#923=FACE_BOUND('',#28400,.T.);
#924=FACE_BOUND('',#28401,.T.);
#925=FACE_BOUND('',#28402,.T.);
#926=FACE_BOUND('',#28403,.T.);
#927=FACE_BOUND('',#28404,.T.);
#928=FACE_BOUND('',#28405,.T.);
#929=FACE_BOUND('',#28406,.T.);
#930=FACE_BOUND('',#28407,.T.);
#931=FACE_BOUND('',#28408,.T.);
#932=FACE_BOUND('',#28409,.T.);
#933=FACE_BOUND('',#28410,.T.);
#934=FACE_BOUND('',#28411,.T.);
#935=FACE_BOUND('',#28412,.T.);
#936=FACE_BOUND('',#28413,.T.);
#937=FACE_BOUND('',#28414,.T.);
#938=FACE_BOUND('',#28415,.T.);
#939=FACE_BOUND('',#28416,.T.);
#940=FACE_BOUND('',#28417,.T.);
#941=FACE_BOUND('',#28418,.T.);
#942=FACE_BOUND('',#28419,.T.);
#943=FACE_BOUND('',#28420,.T.);
#944=FACE_BOUND('',#28421,.T.);
#945=FACE_BOUND('',#28422,.T.);
#946=FACE_BOUND('',#28423,.T.);
#947=FACE_BOUND('',#28424,.T.);
#948=FACE_BOUND('',#28425,.T.);
#949=FACE_BOUND('',#28426,.T.);
#950=FACE_BOUND('',#28427,.T.);
#951=FACE_BOUND('',#28428,.T.);
#952=FACE_BOUND('',#28429,.T.);
#953=FACE_BOUND('',#28430,.T.);
#954=FACE_BOUND('',#28431,.T.);
#955=FACE_BOUND('',#28432,.T.);
#956=FACE_BOUND('',#28433,.T.);
#957=FACE_BOUND('',#28434,.T.);
#958=FACE_BOUND('',#28435,.T.);
#959=FACE_BOUND('',#28436,.T.);
#960=FACE_BOUND('',#28437,.T.);
#961=FACE_BOUND('',#28438,.T.);
#962=FACE_BOUND('',#28439,.T.);
#963=FACE_BOUND('',#28440,.T.);
#964=FACE_BOUND('',#28441,.T.);
#965=FACE_BOUND('',#28442,.T.);
#966=FACE_BOUND('',#28443,.T.);
#967=FACE_BOUND('',#28444,.T.);
#968=FACE_BOUND('',#28445,.T.);
#969=FACE_BOUND('',#28446,.T.);
#970=FACE_BOUND('',#28447,.T.);
#971=FACE_BOUND('',#28448,.T.);
#972=FACE_BOUND('',#28449,.T.);
#973=FACE_BOUND('',#28450,.T.);
#974=FACE_BOUND('',#28451,.T.);
#975=FACE_BOUND('',#28452,.T.);
#976=FACE_BOUND('',#28453,.T.);
#977=FACE_BOUND('',#28454,.T.);
#978=FACE_BOUND('',#28455,.T.);
#979=FACE_BOUND('',#28456,.T.);
#980=FACE_BOUND('',#28457,.T.);
#981=FACE_BOUND('',#28458,.T.);
#982=FACE_BOUND('',#28459,.T.);
#983=FACE_BOUND('',#28460,.T.);
#984=FACE_BOUND('',#28461,.T.);
#985=FACE_BOUND('',#28462,.T.);
#986=FACE_BOUND('',#28463,.T.);
#987=FACE_BOUND('',#28464,.T.);
#988=FACE_BOUND('',#28465,.T.);
#989=FACE_BOUND('',#28466,.T.);
#990=FACE_BOUND('',#28467,.T.);
#991=FACE_BOUND('',#28468,.T.);
#992=FACE_BOUND('',#28469,.T.);
#993=FACE_BOUND('',#28470,.T.);
#994=FACE_BOUND('',#28471,.T.);
#995=FACE_BOUND('',#28472,.T.);
#996=FACE_BOUND('',#28473,.T.);
#997=FACE_BOUND('',#28474,.T.);
#998=FACE_BOUND('',#28475,.T.);
#999=FACE_BOUND('',#28476,.T.);
#1000=FACE_BOUND('',#28477,.T.);
#1001=FACE_BOUND('',#28478,.T.);
#1002=FACE_BOUND('',#28479,.T.);
#1003=FACE_BOUND('',#28480,.T.);
#1004=FACE_BOUND('',#28481,.T.);
#1005=FACE_BOUND('',#28482,.T.);
#1006=FACE_BOUND('',#28483,.T.);
#1007=FACE_BOUND('',#28484,.T.);
#1008=FACE_BOUND('',#28485,.T.);
#1009=FACE_BOUND('',#28486,.T.);
#1010=FACE_BOUND('',#28487,.T.);
#1011=FACE_BOUND('',#28488,.T.);
#1012=FACE_BOUND('',#28489,.T.);
#1013=FACE_BOUND('',#28490,.T.);
#1014=FACE_BOUND('',#28491,.T.);
#1015=FACE_BOUND('',#28492,.T.);
#1016=FACE_BOUND('',#28493,.T.);
#1017=FACE_BOUND('',#28494,.T.);
#1018=FACE_BOUND('',#28495,.T.);
#1019=FACE_BOUND('',#28496,.T.);
#1020=FACE_BOUND('',#28497,.T.);
#1021=FACE_BOUND('',#28498,.T.);
#1022=FACE_BOUND('',#28499,.T.);
#1023=FACE_BOUND('',#28500,.T.);
#1024=FACE_BOUND('',#28501,.T.);
#1025=FACE_BOUND('',#28502,.T.);
#1026=FACE_BOUND('',#28503,.T.);
#1027=FACE_BOUND('',#28504,.T.);
#1028=FACE_BOUND('',#28505,.T.);
#1029=FACE_BOUND('',#28506,.T.);
#1030=FACE_BOUND('',#28507,.T.);
#1031=FACE_BOUND('',#28508,.T.);
#1032=FACE_BOUND('',#28509,.T.);
#1033=FACE_BOUND('',#28510,.T.);
#1034=FACE_BOUND('',#28511,.T.);
#1035=FACE_BOUND('',#28512,.T.);
#1036=FACE_BOUND('',#28513,.T.);
#1037=FACE_BOUND('',#28514,.T.);
#1038=FACE_BOUND('',#28515,.T.);
#1039=FACE_BOUND('',#28516,.T.);
#1040=FACE_BOUND('',#28517,.T.);
#1041=FACE_BOUND('',#28518,.T.);
#1042=FACE_BOUND('',#28519,.T.);
#1043=FACE_BOUND('',#28520,.T.);
#1044=FACE_BOUND('',#28521,.T.);
#1045=FACE_BOUND('',#28522,.T.);
#1046=FACE_BOUND('',#28523,.T.);
#1047=FACE_BOUND('',#28524,.T.);
#1048=FACE_BOUND('',#28525,.T.);
#1049=FACE_BOUND('',#28526,.T.);
#1050=FACE_BOUND('',#28527,.T.);
#1051=FACE_BOUND('',#28528,.T.);
#1052=FACE_BOUND('',#28529,.T.);
#1053=FACE_BOUND('',#28530,.T.);
#1054=FACE_BOUND('',#28531,.T.);
#1055=FACE_BOUND('',#28532,.T.);
#1056=FACE_BOUND('',#28533,.T.);
#1057=FACE_BOUND('',#28534,.T.);
#1058=FACE_BOUND('',#28535,.T.);
#1059=FACE_BOUND('',#28536,.T.);
#1060=FACE_BOUND('',#28537,.T.);
#1061=FACE_BOUND('',#28538,.T.);
#1062=FACE_BOUND('',#28539,.T.);
#1063=FACE_BOUND('',#28540,.T.);
#1064=FACE_BOUND('',#28541,.T.);
#1065=FACE_BOUND('',#28542,.T.);
#1066=FACE_BOUND('',#28543,.T.);
#1067=FACE_BOUND('',#28544,.T.);
#1068=FACE_BOUND('',#28545,.T.);
#1069=FACE_BOUND('',#28546,.T.);
#1070=FACE_BOUND('',#28547,.T.);
#1071=FACE_BOUND('',#28548,.T.);
#1072=FACE_BOUND('',#28549,.T.);
#1073=FACE_BOUND('',#28550,.T.);
#1074=FACE_BOUND('',#28551,.T.);
#1075=FACE_BOUND('',#28552,.T.);
#1076=FACE_BOUND('',#28553,.T.);
#1077=FACE_BOUND('',#28554,.T.);
#1078=FACE_BOUND('',#28555,.T.);
#1079=FACE_BOUND('',#28556,.T.);
#1080=FACE_BOUND('',#28557,.T.);
#1081=FACE_BOUND('',#28558,.T.);
#1082=FACE_BOUND('',#28559,.T.);
#1083=FACE_BOUND('',#28560,.T.);
#1084=FACE_BOUND('',#28561,.T.);
#1085=FACE_BOUND('',#28562,.T.);
#1086=FACE_BOUND('',#28563,.T.);
#1087=FACE_BOUND('',#28564,.T.);
#1088=FACE_BOUND('',#28565,.T.);
#1089=FACE_BOUND('',#28566,.T.);
#1090=FACE_BOUND('',#28567,.T.);
#1091=FACE_BOUND('',#28568,.T.);
#1092=FACE_BOUND('',#28569,.T.);
#1093=FACE_BOUND('',#28570,.T.);
#1094=FACE_BOUND('',#28571,.T.);
#1095=FACE_BOUND('',#28572,.T.);
#1096=FACE_BOUND('',#28573,.T.);
#1097=FACE_BOUND('',#28574,.T.);
#1098=FACE_BOUND('',#28575,.T.);
#1099=FACE_BOUND('',#28576,.T.);
#1100=FACE_BOUND('',#28577,.T.);
#1101=FACE_BOUND('',#28578,.T.);
#1102=FACE_BOUND('',#28579,.T.);
#1103=FACE_BOUND('',#28580,.T.);
#1104=FACE_BOUND('',#28581,.T.);
#1105=FACE_BOUND('',#28582,.T.);
#1106=FACE_BOUND('',#28583,.T.);
#1107=FACE_BOUND('',#28584,.T.);
#1108=FACE_BOUND('',#28585,.T.);
#1109=FACE_BOUND('',#28586,.T.);
#1110=FACE_BOUND('',#28587,.T.);
#1111=FACE_BOUND('',#28588,.T.);
#1112=FACE_BOUND('',#28589,.T.);
#1113=FACE_BOUND('',#28590,.T.);
#1114=FACE_BOUND('',#28591,.T.);
#1115=FACE_BOUND('',#28592,.T.);
#1116=FACE_BOUND('',#28593,.T.);
#1117=FACE_BOUND('',#28594,.T.);
#1118=FACE_BOUND('',#28595,.T.);
#1119=FACE_BOUND('',#28596,.T.);
#1120=FACE_BOUND('',#28597,.T.);
#1121=FACE_BOUND('',#28598,.T.);
#1122=FACE_BOUND('',#28599,.T.);
#1123=FACE_BOUND('',#28600,.T.);
#1124=FACE_BOUND('',#28601,.T.);
#1125=FACE_BOUND('',#28602,.T.);
#1126=FACE_BOUND('',#28603,.T.);
#1127=FACE_BOUND('',#28604,.T.);
#1128=FACE_BOUND('',#28605,.T.);
#1129=FACE_BOUND('',#28606,.T.);
#1130=FACE_BOUND('',#28607,.T.);
#1131=FACE_BOUND('',#28608,.T.);
#1132=FACE_BOUND('',#28609,.T.);
#1133=FACE_BOUND('',#28610,.T.);
#1134=FACE_BOUND('',#28611,.T.);
#1135=FACE_BOUND('',#28612,.T.);
#1136=FACE_BOUND('',#28613,.T.);
#1137=FACE_BOUND('',#28614,.T.);
#1138=FACE_BOUND('',#28615,.T.);
#1139=FACE_BOUND('',#28616,.T.);
#1140=FACE_BOUND('',#28617,.T.);
#1141=FACE_BOUND('',#28618,.T.);
#1142=FACE_BOUND('',#28619,.T.);
#1143=FACE_BOUND('',#28620,.T.);
#1144=FACE_BOUND('',#28621,.T.);
#1145=FACE_BOUND('',#28622,.T.);
#1146=FACE_BOUND('',#28623,.T.);
#1147=FACE_BOUND('',#28624,.T.);
#1148=FACE_BOUND('',#28625,.T.);
#1149=FACE_BOUND('',#28626,.T.);
#1150=FACE_BOUND('',#28627,.T.);
#1151=FACE_BOUND('',#28628,.T.);
#1152=FACE_BOUND('',#28629,.T.);
#1153=FACE_BOUND('',#28630,.T.);
#1154=FACE_BOUND('',#28631,.T.);
#1155=FACE_BOUND('',#28632,.T.);
#1156=FACE_BOUND('',#28633,.T.);
#1157=FACE_BOUND('',#28634,.T.);
#1158=FACE_BOUND('',#28635,.T.);
#1159=FACE_BOUND('',#28636,.T.);
#1160=FACE_BOUND('',#28637,.T.);
#1161=FACE_BOUND('',#28638,.T.);
#1162=FACE_BOUND('',#28639,.T.);
#1163=FACE_BOUND('',#28640,.T.);
#1164=FACE_BOUND('',#28641,.T.);
#1165=FACE_BOUND('',#28642,.T.);
#1166=FACE_BOUND('',#28643,.T.);
#1167=FACE_BOUND('',#28644,.T.);
#1168=FACE_BOUND('',#28645,.T.);
#1169=FACE_BOUND('',#28646,.T.);
#1170=FACE_BOUND('',#28647,.T.);
#1171=FACE_BOUND('',#28648,.T.);
#1172=FACE_BOUND('',#28649,.T.);
#1173=FACE_BOUND('',#28650,.T.);
#1174=FACE_BOUND('',#28651,.T.);
#1175=FACE_BOUND('',#28652,.T.);
#1176=FACE_BOUND('',#28653,.T.);
#1177=FACE_BOUND('',#28654,.T.);
#1178=FACE_BOUND('',#28655,.T.);
#1179=FACE_BOUND('',#28656,.T.);
#1180=FACE_BOUND('',#28657,.T.);
#1181=FACE_BOUND('',#28658,.T.);
#1182=FACE_BOUND('',#28659,.T.);
#1183=FACE_BOUND('',#28660,.T.);
#1184=FACE_BOUND('',#28661,.T.);
#1185=FACE_BOUND('',#28662,.T.);
#1186=FACE_BOUND('',#28663,.T.);
#1187=FACE_BOUND('',#28664,.T.);
#1188=FACE_BOUND('',#28665,.T.);
#1189=FACE_BOUND('',#28666,.T.);
#1190=FACE_BOUND('',#28667,.T.);
#1191=FACE_BOUND('',#28668,.T.);
#1192=FACE_BOUND('',#28669,.T.);
#1193=FACE_BOUND('',#28670,.T.);
#1194=FACE_BOUND('',#28671,.T.);
#1195=FACE_BOUND('',#28672,.T.);
#1196=FACE_BOUND('',#28673,.T.);
#1197=FACE_BOUND('',#28674,.T.);
#1198=FACE_BOUND('',#28675,.T.);
#1199=FACE_BOUND('',#28676,.T.);
#1200=FACE_BOUND('',#28677,.T.);
#1201=FACE_BOUND('',#28678,.T.);
#1202=FACE_BOUND('',#28679,.T.);
#1203=FACE_BOUND('',#28680,.T.);
#1204=FACE_BOUND('',#28681,.T.);
#1205=FACE_BOUND('',#28682,.T.);
#1206=FACE_BOUND('',#28684,.T.);
#1207=FACE_BOUND('',#28698,.T.);
#1208=FACE_BOUND('',#28700,.T.);
#1209=FACE_BOUND('',#28701,.T.);
#1210=FACE_BOUND('',#28702,.T.);
#1211=FACE_BOUND('',#28703,.T.);
#1212=FACE_BOUND('',#28704,.T.);
#1213=FACE_BOUND('',#28705,.T.);
#1214=FACE_BOUND('',#28706,.T.);
#1215=FACE_BOUND('',#28707,.T.);
#1216=FACE_BOUND('',#28708,.T.);
#1217=FACE_BOUND('',#28709,.T.);
#1218=FACE_BOUND('',#28710,.T.);
#1219=FACE_BOUND('',#28711,.T.);
#1220=FACE_BOUND('',#28712,.T.);
#1221=FACE_BOUND('',#28713,.T.);
#1222=FACE_BOUND('',#28714,.T.);
#1223=FACE_BOUND('',#28715,.T.);
#1224=FACE_BOUND('',#28716,.T.);
#1225=FACE_BOUND('',#28717,.T.);
#1226=FACE_BOUND('',#28718,.T.);
#1227=FACE_BOUND('',#28719,.T.);
#1228=FACE_BOUND('',#28720,.T.);
#1229=FACE_BOUND('',#28721,.T.);
#1230=FACE_BOUND('',#28722,.T.);
#1231=FACE_BOUND('',#28723,.T.);
#1232=FACE_BOUND('',#28724,.T.);
#1233=FACE_BOUND('',#28725,.T.);
#1234=FACE_BOUND('',#28726,.T.);
#1235=FACE_BOUND('',#28727,.T.);
#1236=FACE_BOUND('',#28728,.T.);
#1237=FACE_BOUND('',#28729,.T.);
#1238=FACE_BOUND('',#28730,.T.);
#1239=FACE_BOUND('',#28731,.T.);
#1240=FACE_BOUND('',#28732,.T.);
#1241=FACE_BOUND('',#28733,.T.);
#1242=FACE_BOUND('',#28734,.T.);
#1243=FACE_BOUND('',#28735,.T.);
#1244=FACE_BOUND('',#28736,.T.);
#1245=FACE_BOUND('',#28737,.T.);
#1246=FACE_BOUND('',#28738,.T.);
#1247=FACE_BOUND('',#28739,.T.);
#1248=FACE_BOUND('',#28740,.T.);
#1249=FACE_BOUND('',#28741,.T.);
#1250=FACE_BOUND('',#28742,.T.);
#1251=FACE_BOUND('',#28743,.T.);
#1252=FACE_BOUND('',#28744,.T.);
#1253=FACE_BOUND('',#28745,.T.);
#1254=FACE_BOUND('',#28746,.T.);
#1255=FACE_BOUND('',#28747,.T.);
#1256=FACE_BOUND('',#28748,.T.);
#1257=FACE_BOUND('',#28749,.T.);
#1258=FACE_BOUND('',#28750,.T.);
#1259=FACE_BOUND('',#28751,.T.);
#1260=FACE_BOUND('',#28752,.T.);
#1261=FACE_BOUND('',#28753,.T.);
#1262=FACE_BOUND('',#28754,.T.);
#1263=FACE_BOUND('',#28755,.T.);
#1264=FACE_BOUND('',#28756,.T.);
#1265=FACE_BOUND('',#28757,.T.);
#1266=FACE_BOUND('',#28758,.T.);
#1267=FACE_BOUND('',#28759,.T.);
#1268=FACE_BOUND('',#28760,.T.);
#1269=FACE_BOUND('',#28761,.T.);
#1270=FACE_BOUND('',#28762,.T.);
#1271=FACE_BOUND('',#28763,.T.);
#1272=FACE_BOUND('',#28764,.T.);
#1273=FACE_BOUND('',#28765,.T.);
#1274=FACE_BOUND('',#28766,.T.);
#1275=FACE_BOUND('',#28767,.T.);
#1276=FACE_BOUND('',#28768,.T.);
#1277=FACE_BOUND('',#28769,.T.);
#1278=FACE_BOUND('',#28770,.T.);
#1279=FACE_BOUND('',#28771,.T.);
#1280=FACE_BOUND('',#28772,.T.);
#1281=FACE_BOUND('',#28773,.T.);
#1282=FACE_BOUND('',#28774,.T.);
#1283=FACE_BOUND('',#28775,.T.);
#1284=FACE_BOUND('',#28776,.T.);
#1285=FACE_BOUND('',#28777,.T.);
#1286=FACE_BOUND('',#28778,.T.);
#1287=FACE_BOUND('',#28779,.T.);
#1288=FACE_BOUND('',#28780,.T.);
#1289=FACE_BOUND('',#28781,.T.);
#1290=FACE_BOUND('',#28782,.T.);
#1291=FACE_BOUND('',#28783,.T.);
#1292=FACE_BOUND('',#28784,.T.);
#1293=FACE_BOUND('',#28785,.T.);
#1294=FACE_BOUND('',#28786,.T.);
#1295=FACE_BOUND('',#28787,.T.);
#1296=FACE_BOUND('',#28788,.T.);
#1297=FACE_BOUND('',#28789,.T.);
#1298=FACE_BOUND('',#28790,.T.);
#1299=FACE_BOUND('',#28791,.T.);
#1300=FACE_BOUND('',#28792,.T.);
#1301=FACE_BOUND('',#28793,.T.);
#1302=FACE_BOUND('',#28794,.T.);
#1303=FACE_BOUND('',#28795,.T.);
#1304=FACE_BOUND('',#28796,.T.);
#1305=FACE_BOUND('',#28797,.T.);
#1306=FACE_BOUND('',#28798,.T.);
#1307=FACE_BOUND('',#28799,.T.);
#1308=FACE_BOUND('',#28800,.T.);
#1309=FACE_BOUND('',#28801,.T.);
#1310=FACE_BOUND('',#28802,.T.);
#1311=FACE_BOUND('',#28803,.T.);
#1312=FACE_BOUND('',#28804,.T.);
#1313=FACE_BOUND('',#28805,.T.);
#1314=FACE_BOUND('',#28806,.T.);
#1315=FACE_BOUND('',#28807,.T.);
#1316=FACE_BOUND('',#28808,.T.);
#1317=FACE_BOUND('',#28809,.T.);
#1318=FACE_BOUND('',#28810,.T.);
#1319=FACE_BOUND('',#28811,.T.);
#1320=FACE_BOUND('',#28812,.T.);
#1321=FACE_BOUND('',#28813,.T.);
#1322=FACE_BOUND('',#28814,.T.);
#1323=FACE_BOUND('',#28815,.T.);
#1324=FACE_BOUND('',#28816,.T.);
#1325=FACE_BOUND('',#28817,.T.);
#1326=FACE_BOUND('',#28818,.T.);
#1327=FACE_BOUND('',#28819,.T.);
#1328=FACE_BOUND('',#28820,.T.);
#1329=FACE_BOUND('',#28821,.T.);
#1330=FACE_BOUND('',#28822,.T.);
#1331=FACE_BOUND('',#28823,.T.);
#1332=FACE_BOUND('',#28824,.T.);
#1333=FACE_BOUND('',#28825,.T.);
#1334=FACE_BOUND('',#28826,.T.);
#1335=FACE_BOUND('',#28827,.T.);
#1336=FACE_BOUND('',#28828,.T.);
#1337=FACE_BOUND('',#28829,.T.);
#1338=FACE_BOUND('',#28830,.T.);
#1339=FACE_BOUND('',#28831,.T.);
#1340=FACE_BOUND('',#28832,.T.);
#1341=FACE_BOUND('',#28833,.T.);
#1342=FACE_BOUND('',#28834,.T.);
#1343=FACE_BOUND('',#28835,.T.);
#1344=FACE_BOUND('',#28836,.T.);
#1345=FACE_BOUND('',#28837,.T.);
#1346=FACE_BOUND('',#28838,.T.);
#1347=FACE_BOUND('',#28839,.T.);
#1348=FACE_BOUND('',#28840,.T.);
#1349=FACE_BOUND('',#28841,.T.);
#1350=FACE_BOUND('',#28842,.T.);
#1351=FACE_BOUND('',#28843,.T.);
#1352=FACE_BOUND('',#28844,.T.);
#1353=FACE_BOUND('',#28845,.T.);
#1354=FACE_BOUND('',#28846,.T.);
#1355=FACE_BOUND('',#28847,.T.);
#1356=FACE_BOUND('',#28848,.T.);
#1357=FACE_BOUND('',#28849,.T.);
#1358=FACE_BOUND('',#28850,.T.);
#1359=FACE_BOUND('',#28851,.T.);
#1360=FACE_BOUND('',#28852,.T.);
#1361=FACE_BOUND('',#28853,.T.);
#1362=FACE_BOUND('',#28854,.T.);
#1363=FACE_BOUND('',#28855,.T.);
#1364=FACE_BOUND('',#28856,.T.);
#1365=FACE_BOUND('',#28857,.T.);
#1366=FACE_BOUND('',#28858,.T.);
#1367=FACE_BOUND('',#28859,.T.);
#1368=FACE_BOUND('',#28860,.T.);
#1369=FACE_BOUND('',#28861,.T.);
#1370=FACE_BOUND('',#28862,.T.);
#1371=FACE_BOUND('',#28863,.T.);
#1372=FACE_BOUND('',#28864,.T.);
#1373=FACE_BOUND('',#28865,.T.);
#1374=FACE_BOUND('',#28866,.T.);
#1375=FACE_BOUND('',#28867,.T.);
#1376=FACE_BOUND('',#28868,.T.);
#1377=FACE_BOUND('',#28869,.T.);
#1378=FACE_BOUND('',#28870,.T.);
#1379=FACE_BOUND('',#28871,.T.);
#1380=FACE_BOUND('',#28872,.T.);
#1381=FACE_BOUND('',#28873,.T.);
#1382=FACE_BOUND('',#28874,.T.);
#1383=FACE_BOUND('',#28875,.T.);
#1384=FACE_BOUND('',#28876,.T.);
#1385=FACE_BOUND('',#28877,.T.);
#1386=FACE_BOUND('',#28878,.T.);
#1387=FACE_BOUND('',#28879,.T.);
#1388=FACE_BOUND('',#28880,.T.);
#1389=FACE_BOUND('',#28881,.T.);
#1390=FACE_BOUND('',#28882,.T.);
#1391=FACE_BOUND('',#28883,.T.);
#1392=FACE_BOUND('',#28884,.T.);
#1393=FACE_BOUND('',#28885,.T.);
#1394=FACE_BOUND('',#28886,.T.);
#1395=FACE_BOUND('',#28887,.T.);
#1396=FACE_BOUND('',#28888,.T.);
#1397=FACE_BOUND('',#28889,.T.);
#1398=FACE_BOUND('',#28890,.T.);
#1399=FACE_BOUND('',#28891,.T.);
#1400=FACE_BOUND('',#28892,.T.);
#1401=FACE_BOUND('',#28893,.T.);
#1402=FACE_BOUND('',#28894,.T.);
#1403=FACE_BOUND('',#28895,.T.);
#1404=FACE_BOUND('',#28896,.T.);
#1405=FACE_BOUND('',#28897,.T.);
#1406=FACE_BOUND('',#28898,.T.);
#1407=FACE_BOUND('',#28899,.T.);
#1408=FACE_BOUND('',#28900,.T.);
#1409=FACE_BOUND('',#28901,.T.);
#1410=FACE_BOUND('',#28902,.T.);
#1411=FACE_BOUND('',#28903,.T.);
#1412=FACE_BOUND('',#28904,.T.);
#1413=FACE_BOUND('',#28905,.T.);
#1414=FACE_BOUND('',#28906,.T.);
#1415=FACE_BOUND('',#28907,.T.);
#1416=FACE_BOUND('',#28908,.T.);
#1417=FACE_BOUND('',#28909,.T.);
#1418=FACE_BOUND('',#28910,.T.);
#1419=FACE_BOUND('',#28911,.T.);
#1420=FACE_BOUND('',#28912,.T.);
#1421=FACE_BOUND('',#28913,.T.);
#1422=FACE_BOUND('',#28914,.T.);
#1423=FACE_BOUND('',#28915,.T.);
#1424=FACE_BOUND('',#28916,.T.);
#1425=FACE_BOUND('',#28917,.T.);
#1426=FACE_BOUND('',#28918,.T.);
#1427=FACE_BOUND('',#28919,.T.);
#1428=FACE_BOUND('',#28920,.T.);
#1429=FACE_BOUND('',#28921,.T.);
#1430=FACE_BOUND('',#28922,.T.);
#1431=FACE_BOUND('',#28923,.T.);
#1432=FACE_BOUND('',#28924,.T.);
#1433=FACE_BOUND('',#28925,.T.);
#1434=FACE_BOUND('',#28926,.T.);
#1435=FACE_BOUND('',#28927,.T.);
#1436=FACE_BOUND('',#28928,.T.);
#1437=FACE_BOUND('',#28929,.T.);
#1438=FACE_BOUND('',#28930,.T.);
#1439=FACE_BOUND('',#28931,.T.);
#1440=FACE_BOUND('',#28932,.T.);
#1441=FACE_BOUND('',#28933,.T.);
#1442=FACE_BOUND('',#28934,.T.);
#1443=FACE_BOUND('',#28935,.T.);
#1444=FACE_BOUND('',#28936,.T.);
#1445=FACE_BOUND('',#28937,.T.);
#1446=FACE_BOUND('',#28938,.T.);
#1447=FACE_BOUND('',#28939,.T.);
#1448=FACE_BOUND('',#28940,.T.);
#1449=FACE_BOUND('',#28941,.T.);
#1450=FACE_BOUND('',#28942,.T.);
#1451=FACE_BOUND('',#28943,.T.);
#1452=FACE_BOUND('',#28944,.T.);
#1453=FACE_BOUND('',#28945,.T.);
#1454=FACE_BOUND('',#28946,.T.);
#1455=FACE_BOUND('',#28947,.T.);
#1456=FACE_BOUND('',#28948,.T.);
#1457=FACE_BOUND('',#28949,.T.);
#1458=FACE_BOUND('',#28950,.T.);
#1459=FACE_BOUND('',#28951,.T.);
#1460=FACE_BOUND('',#28952,.T.);
#1461=FACE_BOUND('',#28953,.T.);
#1462=FACE_BOUND('',#28954,.T.);
#1463=FACE_BOUND('',#28955,.T.);
#1464=FACE_BOUND('',#28961,.T.);
#1465=FACE_BOUND('',#28962,.T.);
#1466=FACE_BOUND('',#28963,.T.);
#1467=FACE_BOUND('',#28964,.T.);
#1468=FACE_BOUND('',#28965,.T.);
#1469=FACE_BOUND('',#28966,.T.);
#1470=FACE_BOUND('',#28967,.T.);
#1471=FACE_BOUND('',#28968,.T.);
#1472=FACE_BOUND('',#28969,.T.);
#1473=FACE_BOUND('',#28970,.T.);
#1474=FACE_BOUND('',#28971,.T.);
#1475=FACE_BOUND('',#28972,.T.);
#1476=FACE_BOUND('',#28973,.T.);
#1477=FACE_BOUND('',#28974,.T.);
#1478=FACE_BOUND('',#28975,.T.);
#1479=FACE_BOUND('',#28976,.T.);
#1480=FACE_BOUND('',#28977,.T.);
#1481=FACE_BOUND('',#28978,.T.);
#1482=FACE_BOUND('',#28979,.T.);
#1483=FACE_BOUND('',#28980,.T.);
#1484=FACE_BOUND('',#28981,.T.);
#1485=FACE_BOUND('',#28982,.T.);
#1486=FACE_BOUND('',#28983,.T.);
#1487=FACE_BOUND('',#28984,.T.);
#1488=FACE_BOUND('',#28985,.T.);
#1489=FACE_BOUND('',#28986,.T.);
#1490=FACE_BOUND('',#28987,.T.);
#1491=FACE_BOUND('',#28988,.T.);
#1492=FACE_BOUND('',#28989,.T.);
#1493=FACE_BOUND('',#28990,.T.);
#1494=FACE_BOUND('',#28991,.T.);
#1495=FACE_BOUND('',#28992,.T.);
#1496=FACE_BOUND('',#28993,.T.);
#1497=FACE_BOUND('',#28994,.T.);
#1498=FACE_BOUND('',#28995,.T.);
#1499=FACE_BOUND('',#28996,.T.);
#1500=FACE_BOUND('',#28997,.T.);
#1501=FACE_BOUND('',#28998,.T.);
#1502=FACE_BOUND('',#28999,.T.);
#1503=FACE_BOUND('',#29000,.T.);
#1504=FACE_BOUND('',#29001,.T.);
#1505=FACE_BOUND('',#29002,.T.);
#1506=FACE_BOUND('',#29003,.T.);
#1507=FACE_BOUND('',#29004,.T.);
#1508=FACE_BOUND('',#29005,.T.);
#1509=FACE_BOUND('',#29006,.T.);
#1510=FACE_BOUND('',#29007,.T.);
#1511=FACE_BOUND('',#29008,.T.);
#1512=FACE_BOUND('',#29009,.T.);
#1513=FACE_BOUND('',#29010,.T.);
#1514=FACE_BOUND('',#29011,.T.);
#1515=FACE_BOUND('',#29012,.T.);
#1516=FACE_BOUND('',#29013,.T.);
#1517=FACE_BOUND('',#29014,.T.);
#1518=FACE_BOUND('',#29015,.T.);
#1519=FACE_BOUND('',#29016,.T.);
#1520=FACE_BOUND('',#29017,.T.);
#1521=FACE_BOUND('',#29018,.T.);
#1522=FACE_BOUND('',#29019,.T.);
#1523=FACE_BOUND('',#29020,.T.);
#1524=FACE_BOUND('',#29021,.T.);
#1525=FACE_BOUND('',#29022,.T.);
#1526=FACE_BOUND('',#29023,.T.);
#1527=FACE_BOUND('',#29024,.T.);
#1528=FACE_BOUND('',#29025,.T.);
#1529=FACE_BOUND('',#29026,.T.);
#1530=FACE_BOUND('',#29027,.T.);
#1531=FACE_BOUND('',#29028,.T.);
#1532=FACE_BOUND('',#29029,.T.);
#1533=FACE_BOUND('',#29030,.T.);
#1534=FACE_BOUND('',#29031,.T.);
#1535=FACE_BOUND('',#29032,.T.);
#1536=FACE_BOUND('',#29033,.T.);
#1537=FACE_BOUND('',#29034,.T.);
#1538=FACE_BOUND('',#29035,.T.);
#1539=FACE_BOUND('',#29036,.T.);
#1540=FACE_BOUND('',#29037,.T.);
#1541=FACE_BOUND('',#29038,.T.);
#1542=FACE_BOUND('',#29039,.T.);
#1543=FACE_BOUND('',#29040,.T.);
#1544=FACE_BOUND('',#29041,.T.);
#1545=FACE_BOUND('',#29042,.T.);
#1546=FACE_BOUND('',#29043,.T.);
#1547=FACE_BOUND('',#29044,.T.);
#1548=FACE_BOUND('',#29045,.T.);
#1549=FACE_BOUND('',#29046,.T.);
#1550=FACE_BOUND('',#29047,.T.);
#1551=FACE_BOUND('',#29048,.T.);
#1552=FACE_BOUND('',#29049,.T.);
#1553=FACE_BOUND('',#29050,.T.);
#1554=FACE_BOUND('',#29051,.T.);
#1555=FACE_BOUND('',#29052,.T.);
#1556=FACE_BOUND('',#29053,.T.);
#1557=FACE_BOUND('',#29054,.T.);
#1558=FACE_BOUND('',#29055,.T.);
#1559=FACE_BOUND('',#29056,.T.);
#1560=FACE_BOUND('',#29057,.T.);
#1561=FACE_BOUND('',#29058,.T.);
#1562=FACE_BOUND('',#29059,.T.);
#1563=FACE_BOUND('',#29060,.T.);
#1564=FACE_BOUND('',#29061,.T.);
#1565=FACE_BOUND('',#29062,.T.);
#1566=FACE_BOUND('',#29063,.T.);
#1567=FACE_BOUND('',#29064,.T.);
#1568=FACE_BOUND('',#29065,.T.);
#1569=FACE_BOUND('',#29066,.T.);
#1570=FACE_BOUND('',#29067,.T.);
#1571=FACE_BOUND('',#29068,.T.);
#1572=FACE_BOUND('',#29069,.T.);
#1573=FACE_BOUND('',#29070,.T.);
#1574=FACE_BOUND('',#29071,.T.);
#1575=FACE_BOUND('',#29072,.T.);
#1576=FACE_BOUND('',#29073,.T.);
#1577=FACE_BOUND('',#29074,.T.);
#1578=FACE_BOUND('',#29075,.T.);
#1579=FACE_BOUND('',#29076,.T.);
#1580=FACE_BOUND('',#29077,.T.);
#1581=FACE_BOUND('',#29078,.T.);
#1582=FACE_BOUND('',#29079,.T.);
#1583=FACE_BOUND('',#29080,.T.);
#1584=FACE_BOUND('',#29081,.T.);
#1585=FACE_BOUND('',#29082,.T.);
#1586=FACE_BOUND('',#29083,.T.);
#1587=FACE_BOUND('',#29084,.T.);
#1588=FACE_BOUND('',#29085,.T.);
#1589=FACE_BOUND('',#29086,.T.);
#1590=FACE_BOUND('',#29087,.T.);
#1591=FACE_BOUND('',#29088,.T.);
#1592=FACE_BOUND('',#29089,.T.);
#1593=FACE_BOUND('',#29090,.T.);
#1594=FACE_BOUND('',#29091,.T.);
#1595=FACE_BOUND('',#29092,.T.);
#1596=FACE_BOUND('',#29093,.T.);
#1597=FACE_BOUND('',#29094,.T.);
#1598=FACE_BOUND('',#29095,.T.);
#1599=FACE_BOUND('',#29096,.T.);
#1600=FACE_BOUND('',#29097,.T.);
#1601=FACE_BOUND('',#29098,.T.);
#1602=FACE_BOUND('',#29099,.T.);
#1603=FACE_BOUND('',#29100,.T.);
#1604=FACE_BOUND('',#29101,.T.);
#1605=FACE_BOUND('',#29102,.T.);
#1606=FACE_BOUND('',#29103,.T.);
#1607=FACE_BOUND('',#29104,.T.);
#1608=FACE_BOUND('',#29105,.T.);
#1609=FACE_BOUND('',#29106,.T.);
#1610=FACE_BOUND('',#29107,.T.);
#1611=FACE_BOUND('',#29108,.T.);
#1612=FACE_BOUND('',#29109,.T.);
#1613=FACE_BOUND('',#29110,.T.);
#1614=FACE_BOUND('',#29111,.T.);
#1615=FACE_BOUND('',#29112,.T.);
#1616=FACE_BOUND('',#29113,.T.);
#1617=FACE_BOUND('',#29114,.T.);
#1618=FACE_BOUND('',#29115,.T.);
#1619=FACE_BOUND('',#29116,.T.);
#1620=FACE_BOUND('',#29117,.T.);
#1621=FACE_BOUND('',#29118,.T.);
#1622=FACE_BOUND('',#29119,.T.);
#1623=FACE_BOUND('',#29120,.T.);
#1624=FACE_BOUND('',#29121,.T.);
#1625=FACE_BOUND('',#29122,.T.);
#1626=FACE_BOUND('',#29123,.T.);
#1627=FACE_BOUND('',#29124,.T.);
#1628=FACE_BOUND('',#29125,.T.);
#1629=FACE_BOUND('',#29126,.T.);
#1630=FACE_BOUND('',#29127,.T.);
#1631=FACE_BOUND('',#29128,.T.);
#1632=FACE_BOUND('',#29129,.T.);
#1633=FACE_BOUND('',#29130,.T.);
#1634=FACE_BOUND('',#29131,.T.);
#1635=FACE_BOUND('',#29132,.T.);
#1636=FACE_BOUND('',#29133,.T.);
#1637=FACE_BOUND('',#29134,.T.);
#1638=FACE_BOUND('',#29135,.T.);
#1639=FACE_BOUND('',#29136,.T.);
#1640=FACE_BOUND('',#29137,.T.);
#1641=FACE_BOUND('',#29138,.T.);
#1642=FACE_BOUND('',#29139,.T.);
#1643=FACE_BOUND('',#29140,.T.);
#1644=FACE_BOUND('',#29141,.T.);
#1645=FACE_BOUND('',#29142,.T.);
#1646=FACE_BOUND('',#29143,.T.);
#1647=FACE_BOUND('',#29144,.T.);
#1648=FACE_BOUND('',#29145,.T.);
#1649=FACE_BOUND('',#29146,.T.);
#1650=FACE_BOUND('',#29147,.T.);
#1651=FACE_BOUND('',#29148,.T.);
#1652=FACE_BOUND('',#29149,.T.);
#1653=FACE_BOUND('',#29150,.T.);
#1654=FACE_BOUND('',#29151,.T.);
#1655=FACE_BOUND('',#29152,.T.);
#1656=FACE_BOUND('',#29153,.T.);
#1657=FACE_BOUND('',#29154,.T.);
#1658=FACE_BOUND('',#29155,.T.);
#1659=FACE_BOUND('',#29156,.T.);
#1660=FACE_BOUND('',#29157,.T.);
#1661=FACE_BOUND('',#29158,.T.);
#1662=FACE_BOUND('',#29159,.T.);
#1663=FACE_BOUND('',#29160,.T.);
#1664=FACE_BOUND('',#29161,.T.);
#1665=FACE_BOUND('',#29162,.T.);
#1666=FACE_BOUND('',#29163,.T.);
#1667=FACE_BOUND('',#29164,.T.);
#1668=FACE_BOUND('',#29165,.T.);
#1669=FACE_BOUND('',#29166,.T.);
#1670=FACE_BOUND('',#29167,.T.);
#1671=FACE_BOUND('',#29168,.T.);
#1672=FACE_BOUND('',#29169,.T.);
#1673=FACE_BOUND('',#29170,.T.);
#1674=FACE_BOUND('',#29171,.T.);
#1675=FACE_BOUND('',#29172,.T.);
#1676=FACE_BOUND('',#29173,.T.);
#1677=FACE_BOUND('',#29174,.T.);
#1678=FACE_BOUND('',#29175,.T.);
#1679=FACE_BOUND('',#29176,.T.);
#1680=FACE_BOUND('',#29177,.T.);
#1681=FACE_BOUND('',#29178,.T.);
#1682=FACE_BOUND('',#29179,.T.);
#1683=FACE_BOUND('',#29180,.T.);
#1684=FACE_BOUND('',#29181,.T.);
#1685=FACE_BOUND('',#29182,.T.);
#1686=FACE_BOUND('',#29183,.T.);
#1687=FACE_BOUND('',#29184,.T.);
#1688=FACE_BOUND('',#29185,.T.);
#1689=FACE_BOUND('',#29186,.T.);
#1690=FACE_BOUND('',#29187,.T.);
#1691=FACE_BOUND('',#29188,.T.);
#1692=FACE_BOUND('',#29189,.T.);
#1693=FACE_BOUND('',#29190,.T.);
#1694=FACE_BOUND('',#29191,.T.);
#1695=FACE_BOUND('',#29192,.T.);
#1696=FACE_BOUND('',#29193,.T.);
#1697=FACE_BOUND('',#29194,.T.);
#1698=FACE_BOUND('',#29195,.T.);
#1699=FACE_BOUND('',#29196,.T.);
#1700=FACE_BOUND('',#29197,.T.);
#1701=FACE_BOUND('',#29198,.T.);
#1702=FACE_BOUND('',#29199,.T.);
#1703=FACE_BOUND('',#29200,.T.);
#1704=FACE_BOUND('',#29201,.T.);
#1705=FACE_BOUND('',#29202,.T.);
#1706=FACE_BOUND('',#29203,.T.);
#1707=FACE_BOUND('',#29204,.T.);
#1708=FACE_BOUND('',#29205,.T.);
#1709=FACE_BOUND('',#29206,.T.);
#1710=FACE_BOUND('',#29207,.T.);
#1711=FACE_BOUND('',#29208,.T.);
#1712=FACE_BOUND('',#29209,.T.);
#1713=FACE_BOUND('',#29210,.T.);
#1714=FACE_BOUND('',#29211,.T.);
#1715=FACE_BOUND('',#29212,.T.);
#1716=FACE_BOUND('',#29213,.T.);
#1717=FACE_BOUND('',#29214,.T.);
#1718=FACE_BOUND('',#29215,.T.);
#1719=FACE_BOUND('',#29216,.T.);
#1720=FACE_BOUND('',#29218,.T.);
#1802=(
BOUNDED_CURVE()
B_SPLINE_CURVE(2,(#186587,#186588,#186589),.UNSPECIFIED.,.F.,.F.)
B_SPLINE_CURVE_WITH_KNOTS((3,3),(1.17484908943589,1.45283332058119),
 .UNSPECIFIED.)
CURVE()
GEOMETRIC_REPRESENTATION_ITEM()
RATIONAL_B_SPLINE_CURVE((1.26057059861676,1.27619589726591,1.28462728942758))
REPRESENTATION_ITEM('')
);
#1803=(
BOUNDED_CURVE()
B_SPLINE_CURVE(2,(#186592,#186593,#186594),.UNSPECIFIED.,.F.,.F.)
B_SPLINE_CURVE_WITH_KNOTS((3,3),(1.81320048054135,2.07306669608502),
 .UNSPECIFIED.)
CURVE()
GEOMETRIC_REPRESENTATION_ITEM()
RATIONAL_B_SPLINE_CURVE((1.22106645430084,1.21305223086313,1.19820004130138))
REPRESENTATION_ITEM('')
);
#1804=(
BOUNDED_CURVE()
B_SPLINE_CURVE(2,(#186598,#186599,#186600),.UNSPECIFIED.,.F.,.F.)
B_SPLINE_CURVE_WITH_KNOTS((3,3),(-1.45283332058118,-1.17484908943588),
 .UNSPECIFIED.)
CURVE()
GEOMETRIC_REPRESENTATION_ITEM()
RATIONAL_B_SPLINE_CURVE((1.28462728942758,1.27619589726592,1.26057059861677))
REPRESENTATION_ITEM('')
);
#1805=(
BOUNDED_CURVE()
B_SPLINE_CURVE(2,(#186604,#186605,#186606),.UNSPECIFIED.,.F.,.F.)
B_SPLINE_CURVE_WITH_KNOTS((3,3),(-2.07306669608501,-1.81320048054134),
 .UNSPECIFIED.)
CURVE()
GEOMETRIC_REPRESENTATION_ITEM()
RATIONAL_B_SPLINE_CURVE((1.19820004130138,1.21305223086313,1.22106645430084))
REPRESENTATION_ITEM('')
);
#1905=TOROIDAL_SURFACE('',#80993,10.88886271061,0.7);
#1906=TOROIDAL_SURFACE('',#80996,12.35,1.3);
#1907=TOROIDAL_SURFACE('',#81028,10.85,0.5);
#1908=TOROIDAL_SURFACE('',#81037,12.35,1.);
#1909=TOROIDAL_SURFACE('',#81040,10.88886271061,1.);
#1958=CONICAL_SURFACE('',#80989,11.64412671312,0.0349065849999998);
#1959=CONICAL_SURFACE('',#81044,11.94412676881,0.0349065849999998);
#1960=CONICAL_SURFACE('',#81062,13.65,0.7853981625);
#1961=CONICAL_SURFACE('',#81068,13.45,0.7853981625);
#1962=CONICAL_SURFACE('',#81070,13.45,0.7853981625);
#2277=CYLINDRICAL_SURFACE('',#80982,13.9);
#2278=CYLINDRICAL_SURFACE('',#80984,13.9);
#2279=CYLINDRICAL_SURFACE('',#80986,13.9);
#2280=CYLINDRICAL_SURFACE('',#80987,13.9);
#2281=CYLINDRICAL_SURFACE('',#80999,0.75);
#2282=CYLINDRICAL_SURFACE('',#81000,0.75);
#2283=CYLINDRICAL_SURFACE('',#81001,11.05);
#2284=CYLINDRICAL_SURFACE('',#81013,0.75);
#2285=CYLINDRICAL_SURFACE('',#81014,0.75);
#2286=CYLINDRICAL_SURFACE('',#81015,11.35);
#2287=CYLINDRICAL_SURFACE('',#81031,9.85);
#2288=CYLINDRICAL_SURFACE('',#81034,10.15);
#2289=CYLINDRICAL_SURFACE('',#81046,12.25);
#2290=CYLINDRICAL_SURFACE('',#81049,12.75);
#2291=CYLINDRICAL_SURFACE('',#81052,13.1);
#2292=CYLINDRICAL_SURFACE('',#81055,13.7);
#2293=CYLINDRICAL_SURFACE('',#81064,12.75);
#2294=CYLINDRICAL_SURFACE('',#81078,13.9);
#2295=CYLINDRICAL_SURFACE('',#85941,0.75);
#2296=CYLINDRICAL_SURFACE('',#85942,0.75);
#2297=CYLINDRICAL_SURFACE('',#85947,0.75);
#2298=CYLINDRICAL_SURFACE('',#85948,0.75);
#3226=LINE('',#183811,#10293);
#3227=LINE('',#183825,#10294);
#3228=LINE('',#183967,#10295);
#3229=LINE('',#184165,#10296);
#3230=LINE('',#184353,#10297);
#3231=LINE('',#184386,#10298);
#3232=LINE('',#184406,#10299);
#3233=LINE('',#184429,#10300);
#3234=LINE('',#184449,#10301);
#3235=LINE('',#184452,#10302);
#3236=LINE('',#184478,#10303);
#3237=LINE('',#184612,#10304);
#3238=LINE('',#184613,#10305);
#3239=LINE('',#184616,#10306);
#3240=LINE('',#184636,#10307);
#3241=LINE('',#184641,#10308);
#3242=LINE('',#184667,#10309);
#3243=LINE('',#184748,#10310);
#3244=LINE('',#184754,#10311);
#3245=LINE('',#184769,#10312);
#3246=LINE('',#184774,#10313);
#3247=LINE('',#184780,#10314);
#3248=LINE('',#184786,#10315);
#3249=LINE('',#184793,#10316);
#3250=LINE('',#184797,#10317);
#3251=LINE('',#184801,#10318);
#3252=LINE('',#184805,#10319);
#3253=LINE('',#184809,#10320);
#3254=LINE('',#184912,#10321);
#3255=LINE('',#185512,#10322);
#3256=LINE('',#185590,#10323);
#3257=LINE('',#186590,#10324);
#3258=LINE('',#186595,#10325);
#3259=LINE('',#186609,#10326);
#3260=LINE('',#186610,#10327);
#3261=LINE('',#186903,#10328);
#3262=LINE('',#187082,#10329);
#3263=LINE('',#187084,#10330);
#3264=LINE('',#187085,#10331);
#3265=LINE('',#187088,#10332);
#3266=LINE('',#187092,#10333);
#3267=LINE('',#187099,#10334);
#3268=LINE('',#187104,#10335);
#3269=LINE('',#187112,#10336);
#3270=LINE('',#187114,#10337);
#3271=LINE('',#187115,#10338);
#3272=LINE('',#187121,#10339);
#3273=LINE('',#187123,#10340);
#3274=LINE('',#187129,#10341);
#3275=LINE('',#187134,#10342);
#3276=LINE('',#187140,#10343);
#3277=LINE('',#187144,#10344);
#3278=LINE('',#187149,#10345);
#3279=LINE('',#187150,#10346);
#3280=LINE('',#187155,#10347);
#3281=LINE('',#187156,#10348);
#3282=LINE('',#187161,#10349);
#3283=LINE('',#187168,#10350);
#3284=LINE('',#187172,#10351);
#3285=LINE('',#187177,#10352);
#3286=LINE('',#187183,#10353);
#3287=LINE('',#187192,#10354);
#3288=LINE('',#187196,#10355);
#3289=LINE('',#187201,#10356);
#3290=LINE('',#187207,#10357);
#3291=LINE('',#187216,#10358);
#3292=LINE('',#187220,#10359);
#3293=LINE('',#187225,#10360);
#3294=LINE('',#187231,#10361);
#3295=LINE('',#187240,#10362);
#3296=LINE('',#187244,#10363);
#3297=LINE('',#187249,#10364);
#3298=LINE('',#187255,#10365);
#3299=LINE('',#187266,#10366);
#3300=LINE('',#187268,#10367);
#3301=LINE('',#187269,#10368);
#3302=LINE('',#187275,#10369);
#3303=LINE('',#187277,#10370);
#3304=LINE('',#187283,#10371);
#3305=LINE('',#187288,#10372);
#3306=LINE('',#187294,#10373);
#3307=LINE('',#187298,#10374);
#3308=LINE('',#187303,#10375);
#3309=LINE('',#187305,#10376);
#3310=LINE('',#187311,#10377);
#3311=LINE('',#187312,#10378);
#3312=LINE('',#187317,#10379);
#3313=LINE('',#187324,#10380);
#3314=LINE('',#187328,#10381);
#3315=LINE('',#187333,#10382);
#3316=LINE('',#187335,#10383);
#3317=LINE('',#187341,#10384);
#3318=LINE('',#187342,#10385);
#3319=LINE('',#187347,#10386);
#3320=LINE('',#187354,#10387);
#3321=LINE('',#187358,#10388);
#3322=LINE('',#187363,#10389);
#3323=LINE('',#187369,#10390);
#3324=LINE('',#187371,#10391);
#3325=LINE('',#187377,#10392);
#3326=LINE('',#187384,#10393);
#3327=LINE('',#187388,#10394);
#3328=LINE('',#187393,#10395);
#3329=LINE('',#187399,#10396);
#3330=LINE('',#187408,#10397);
#3331=LINE('',#187412,#10398);
#3332=LINE('',#187417,#10399);
#3333=LINE('',#187419,#10400);
#3334=LINE('',#187425,#10401);
#3335=LINE('',#187426,#10402);
#3336=LINE('',#187431,#10403);
#3337=LINE('',#187438,#10404);
#3338=LINE('',#187442,#10405);
#3339=LINE('',#187447,#10406);
#3340=LINE('',#187449,#10407);
#3341=LINE('',#187455,#10408);
#3342=LINE('',#187456,#10409);
#3343=LINE('',#187461,#10410);
#3344=LINE('',#187468,#10411);
#3345=LINE('',#187472,#10412);
#3346=LINE('',#187477,#10413);
#3347=LINE('',#187479,#10414);
#3348=LINE('',#187485,#10415);
#3349=LINE('',#187486,#10416);
#3350=LINE('',#187491,#10417);
#3351=LINE('',#187498,#10418);
#3352=LINE('',#187502,#10419);
#3353=LINE('',#187507,#10420);
#3354=LINE('',#187509,#10421);
#3355=LINE('',#187515,#10422);
#3356=LINE('',#187516,#10423);
#3357=LINE('',#187521,#10424);
#3358=LINE('',#187528,#10425);
#3359=LINE('',#187532,#10426);
#3360=LINE('',#187537,#10427);
#3361=LINE('',#187543,#10428);
#3362=LINE('',#187552,#10429);
#3363=LINE('',#187556,#10430);
#3364=LINE('',#187561,#10431);
#3365=LINE('',#187567,#10432);
#3366=LINE('',#187576,#10433);
#3367=LINE('',#187580,#10434);
#3368=LINE('',#187585,#10435);
#3369=LINE('',#187591,#10436);
#3370=LINE('',#187600,#10437);
#3371=LINE('',#187604,#10438);
#3372=LINE('',#187609,#10439);
#3373=LINE('',#187615,#10440);
#3374=LINE('',#187624,#10441);
#3375=LINE('',#187628,#10442);
#3376=LINE('',#187633,#10443);
#3377=LINE('',#187639,#10444);
#3378=LINE('',#187648,#10445);
#3379=LINE('',#187652,#10446);
#3380=LINE('',#187657,#10447);
#3381=LINE('',#187663,#10448);
#3382=LINE('',#187674,#10449);
#3383=LINE('',#187677,#10450);
#3384=LINE('',#187682,#10451);
#3385=LINE('',#187687,#10452);
#3386=LINE('',#187691,#10453);
#3387=LINE('',#187696,#10454);
#3388=LINE('',#187702,#10455);
#3389=LINE('',#187706,#10456);
#3390=LINE('',#187711,#10457);
#3391=LINE('',#187713,#10458);
#3392=LINE('',#187719,#10459);
#3393=LINE('',#187720,#10460);
#3394=LINE('',#187725,#10461);
#3395=LINE('',#187732,#10462);
#3396=LINE('',#187736,#10463);
#3397=LINE('',#187741,#10464);
#3398=LINE('',#187747,#10465);
#3399=LINE('',#187756,#10466);
#3400=LINE('',#187760,#10467);
#3401=LINE('',#187765,#10468);
#3402=LINE('',#187771,#10469);
#3403=LINE('',#187780,#10470);
#3404=LINE('',#187784,#10471);
#3405=LINE('',#187789,#10472);
#3406=LINE('',#187795,#10473);
#3407=LINE('',#187804,#10474);
#3408=LINE('',#187808,#10475);
#3409=LINE('',#187813,#10476);
#3410=LINE('',#187819,#10477);
#3411=LINE('',#187828,#10478);
#3412=LINE('',#187832,#10479);
#3413=LINE('',#187837,#10480);
#3414=LINE('',#187843,#10481);
#3415=LINE('',#187852,#10482);
#3416=LINE('',#187856,#10483);
#3417=LINE('',#187861,#10484);
#3418=LINE('',#187867,#10485);
#3419=LINE('',#187876,#10486);
#3420=LINE('',#187880,#10487);
#3421=LINE('',#187885,#10488);
#3422=LINE('',#187891,#10489);
#3423=LINE('',#187900,#10490);
#3424=LINE('',#187904,#10491);
#3425=LINE('',#187909,#10492);
#3426=LINE('',#187915,#10493);
#3427=LINE('',#187924,#10494);
#3428=LINE('',#187928,#10495);
#3429=LINE('',#187933,#10496);
#3430=LINE('',#187935,#10497);
#3431=LINE('',#187941,#10498);
#3432=LINE('',#187942,#10499);
#3433=LINE('',#187947,#10500);
#3434=LINE('',#187954,#10501);
#3435=LINE('',#187958,#10502);
#3436=LINE('',#187963,#10503);
#3437=LINE('',#187965,#10504);
#3438=LINE('',#187971,#10505);
#3439=LINE('',#187972,#10506);
#3440=LINE('',#187977,#10507);
#3441=LINE('',#187984,#10508);
#3442=LINE('',#187988,#10509);
#3443=LINE('',#187993,#10510);
#3444=LINE('',#187999,#10511);
#3445=LINE('',#188008,#10512);
#3446=LINE('',#188012,#10513);
#3447=LINE('',#188017,#10514);
#3448=LINE('',#188023,#10515);
#3449=LINE('',#188032,#10516);
#3450=LINE('',#188036,#10517);
#3451=LINE('',#188041,#10518);
#3452=LINE('',#188047,#10519);
#3453=LINE('',#188056,#10520);
#3454=LINE('',#188060,#10521);
#3455=LINE('',#188065,#10522);
#3456=LINE('',#188071,#10523);
#3457=LINE('',#188080,#10524);
#3458=LINE('',#188084,#10525);
#3459=LINE('',#188089,#10526);
#3460=LINE('',#188095,#10527);
#3461=LINE('',#188104,#10528);
#3462=LINE('',#188108,#10529);
#3463=LINE('',#188113,#10530);
#3464=LINE('',#188119,#10531);
#3465=LINE('',#188128,#10532);
#3466=LINE('',#188132,#10533);
#3467=LINE('',#188137,#10534);
#3468=LINE('',#188143,#10535);
#3469=LINE('',#188152,#10536);
#3470=LINE('',#188156,#10537);
#3471=LINE('',#188161,#10538);
#3472=LINE('',#188167,#10539);
#3473=LINE('',#188176,#10540);
#3474=LINE('',#188180,#10541);
#3475=LINE('',#188185,#10542);
#3476=LINE('',#188191,#10543);
#3477=LINE('',#188200,#10544);
#3478=LINE('',#188204,#10545);
#3479=LINE('',#188209,#10546);
#3480=LINE('',#188215,#10547);
#3481=LINE('',#188224,#10548);
#3482=LINE('',#188226,#10549);
#3483=LINE('',#188231,#10550);
#3484=LINE('',#188235,#10551);
#3485=LINE('',#188240,#10552);
#3486=LINE('',#188245,#10553);
#3487=LINE('',#188254,#10554);
#3488=LINE('',#188258,#10555);
#3489=LINE('',#188263,#10556);
#3490=LINE('',#188269,#10557);
#3491=LINE('',#188278,#10558);
#3492=LINE('',#188282,#10559);
#3493=LINE('',#188287,#10560);
#3494=LINE('',#188293,#10561);
#3495=LINE('',#188302,#10562);
#3496=LINE('',#188306,#10563);
#3497=LINE('',#188311,#10564);
#3498=LINE('',#188317,#10565);
#3499=LINE('',#188326,#10566);
#3500=LINE('',#188330,#10567);
#3501=LINE('',#188335,#10568);
#3502=LINE('',#188341,#10569);
#3503=LINE('',#188350,#10570);
#3504=LINE('',#188354,#10571);
#3505=LINE('',#188359,#10572);
#3506=LINE('',#188365,#10573);
#3507=LINE('',#188374,#10574);
#3508=LINE('',#188378,#10575);
#3509=LINE('',#188383,#10576);
#3510=LINE('',#188389,#10577);
#3511=LINE('',#188398,#10578);
#3512=LINE('',#188402,#10579);
#3513=LINE('',#188407,#10580);
#3514=LINE('',#188413,#10581);
#3515=LINE('',#188422,#10582);
#3516=LINE('',#188426,#10583);
#3517=LINE('',#188431,#10584);
#3518=LINE('',#188437,#10585);
#3519=LINE('',#188446,#10586);
#3520=LINE('',#188450,#10587);
#3521=LINE('',#188455,#10588);
#3522=LINE('',#188461,#10589);
#3523=LINE('',#188470,#10590);
#3524=LINE('',#188474,#10591);
#3525=LINE('',#188479,#10592);
#3526=LINE('',#188485,#10593);
#3527=LINE('',#188494,#10594);
#3528=LINE('',#188498,#10595);
#3529=LINE('',#188503,#10596);
#3530=LINE('',#188509,#10597);
#3531=LINE('',#188511,#10598);
#3532=LINE('',#188517,#10599);
#3533=LINE('',#188524,#10600);
#3534=LINE('',#188528,#10601);
#3535=LINE('',#188533,#10602);
#3536=LINE('',#188539,#10603);
#3537=LINE('',#188541,#10604);
#3538=LINE('',#188547,#10605);
#3539=LINE('',#188554,#10606);
#3540=LINE('',#188558,#10607);
#3541=LINE('',#188563,#10608);
#3542=LINE('',#188569,#10609);
#3543=LINE('',#188578,#10610);
#3544=LINE('',#188582,#10611);
#3545=LINE('',#188587,#10612);
#3546=LINE('',#188593,#10613);
#3547=LINE('',#188602,#10614);
#3548=LINE('',#188606,#10615);
#3549=LINE('',#188611,#10616);
#3550=LINE('',#188617,#10617);
#3551=LINE('',#188626,#10618);
#3552=LINE('',#188630,#10619);
#3553=LINE('',#188635,#10620);
#3554=LINE('',#188641,#10621);
#3555=LINE('',#188650,#10622);
#3556=LINE('',#188654,#10623);
#3557=LINE('',#188659,#10624);
#3558=LINE('',#188665,#10625);
#3559=LINE('',#188674,#10626);
#3560=LINE('',#188678,#10627);
#3561=LINE('',#188683,#10628);
#3562=LINE('',#188689,#10629);
#3563=LINE('',#188698,#10630);
#3564=LINE('',#188702,#10631);
#3565=LINE('',#188707,#10632);
#3566=LINE('',#188713,#10633);
#3567=LINE('',#188722,#10634);
#3568=LINE('',#188726,#10635);
#3569=LINE('',#188731,#10636);
#3570=LINE('',#188737,#10637);
#3571=LINE('',#188746,#10638);
#3572=LINE('',#188750,#10639);
#3573=LINE('',#188755,#10640);
#3574=LINE('',#188761,#10641);
#3575=LINE('',#188770,#10642);
#3576=LINE('',#188774,#10643);
#3577=LINE('',#188779,#10644);
#3578=LINE('',#188785,#10645);
#3579=LINE('',#188794,#10646);
#3580=LINE('',#188798,#10647);
#3581=LINE('',#188803,#10648);
#3582=LINE('',#188809,#10649);
#3583=LINE('',#188818,#10650);
#3584=LINE('',#188822,#10651);
#3585=LINE('',#188827,#10652);
#3586=LINE('',#188833,#10653);
#3587=LINE('',#188842,#10654);
#3588=LINE('',#188846,#10655);
#3589=LINE('',#188851,#10656);
#3590=LINE('',#188857,#10657);
#3591=LINE('',#188866,#10658);
#3592=LINE('',#188870,#10659);
#3593=LINE('',#188875,#10660);
#3594=LINE('',#188881,#10661);
#3595=LINE('',#188890,#10662);
#3596=LINE('',#188894,#10663);
#3597=LINE('',#188899,#10664);
#3598=LINE('',#188905,#10665);
#3599=LINE('',#188914,#10666);
#3600=LINE('',#188918,#10667);
#3601=LINE('',#188923,#10668);
#3602=LINE('',#188929,#10669);
#3603=LINE('',#188938,#10670);
#3604=LINE('',#188942,#10671);
#3605=LINE('',#188947,#10672);
#3606=LINE('',#188953,#10673);
#3607=LINE('',#188962,#10674);
#3608=LINE('',#188966,#10675);
#3609=LINE('',#188971,#10676);
#3610=LINE('',#188977,#10677);
#3611=LINE('',#188986,#10678);
#3612=LINE('',#188990,#10679);
#3613=LINE('',#188995,#10680);
#3614=LINE('',#189001,#10681);
#3615=LINE('',#189010,#10682);
#3616=LINE('',#189014,#10683);
#3617=LINE('',#189019,#10684);
#3618=LINE('',#189025,#10685);
#3619=LINE('',#189034,#10686);
#3620=LINE('',#189038,#10687);
#3621=LINE('',#189043,#10688);
#3622=LINE('',#189049,#10689);
#3623=LINE('',#189058,#10690);
#3624=LINE('',#189062,#10691);
#3625=LINE('',#189067,#10692);
#3626=LINE('',#189073,#10693);
#3627=LINE('',#189082,#10694);
#3628=LINE('',#189086,#10695);
#3629=LINE('',#189091,#10696);
#3630=LINE('',#189097,#10697);
#3631=LINE('',#189106,#10698);
#3632=LINE('',#189110,#10699);
#3633=LINE('',#189115,#10700);
#3634=LINE('',#189121,#10701);
#3635=LINE('',#189130,#10702);
#3636=LINE('',#189134,#10703);
#3637=LINE('',#189139,#10704);
#3638=LINE('',#189145,#10705);
#3639=LINE('',#189154,#10706);
#3640=LINE('',#189158,#10707);
#3641=LINE('',#189163,#10708);
#3642=LINE('',#189169,#10709);
#3643=LINE('',#189178,#10710);
#3644=LINE('',#189182,#10711);
#3645=LINE('',#189187,#10712);
#3646=LINE('',#189193,#10713);
#3647=LINE('',#189202,#10714);
#3648=LINE('',#189206,#10715);
#3649=LINE('',#189211,#10716);
#3650=LINE('',#189217,#10717);
#3651=LINE('',#189226,#10718);
#3652=LINE('',#189230,#10719);
#3653=LINE('',#189235,#10720);
#3654=LINE('',#189241,#10721);
#3655=LINE('',#189250,#10722);
#3656=LINE('',#189254,#10723);
#3657=LINE('',#189259,#10724);
#3658=LINE('',#189265,#10725);
#3659=LINE('',#189274,#10726);
#3660=LINE('',#189278,#10727);
#3661=LINE('',#189283,#10728);
#3662=LINE('',#189289,#10729);
#3663=LINE('',#189298,#10730);
#3664=LINE('',#189302,#10731);
#3665=LINE('',#189307,#10732);
#3666=LINE('',#189313,#10733);
#3667=LINE('',#189322,#10734);
#3668=LINE('',#189326,#10735);
#3669=LINE('',#189331,#10736);
#3670=LINE('',#189337,#10737);
#3671=LINE('',#189346,#10738);
#3672=LINE('',#189350,#10739);
#3673=LINE('',#189355,#10740);
#3674=LINE('',#189361,#10741);
#3675=LINE('',#189370,#10742);
#3676=LINE('',#189374,#10743);
#3677=LINE('',#189379,#10744);
#3678=LINE('',#189385,#10745);
#3679=LINE('',#189394,#10746);
#3680=LINE('',#189398,#10747);
#3681=LINE('',#189403,#10748);
#3682=LINE('',#189409,#10749);
#3683=LINE('',#189418,#10750);
#3684=LINE('',#189422,#10751);
#3685=LINE('',#189427,#10752);
#3686=LINE('',#189433,#10753);
#3687=LINE('',#189442,#10754);
#3688=LINE('',#189446,#10755);
#3689=LINE('',#189451,#10756);
#3690=LINE('',#189457,#10757);
#3691=LINE('',#189466,#10758);
#3692=LINE('',#189470,#10759);
#3693=LINE('',#189475,#10760);
#3694=LINE('',#189481,#10761);
#3695=LINE('',#189490,#10762);
#3696=LINE('',#189494,#10763);
#3697=LINE('',#189499,#10764);
#3698=LINE('',#189505,#10765);
#3699=LINE('',#189514,#10766);
#3700=LINE('',#189518,#10767);
#3701=LINE('',#189523,#10768);
#3702=LINE('',#189529,#10769);
#3703=LINE('',#189538,#10770);
#3704=LINE('',#189542,#10771);
#3705=LINE('',#189547,#10772);
#3706=LINE('',#189553,#10773);
#3707=LINE('',#189562,#10774);
#3708=LINE('',#189566,#10775);
#3709=LINE('',#189571,#10776);
#3710=LINE('',#189577,#10777);
#3711=LINE('',#189586,#10778);
#3712=LINE('',#189590,#10779);
#3713=LINE('',#189595,#10780);
#3714=LINE('',#189601,#10781);
#3715=LINE('',#189610,#10782);
#3716=LINE('',#189614,#10783);
#3717=LINE('',#189619,#10784);
#3718=LINE('',#189625,#10785);
#3719=LINE('',#189634,#10786);
#3720=LINE('',#189638,#10787);
#3721=LINE('',#189643,#10788);
#3722=LINE('',#189649,#10789);
#3723=LINE('',#189658,#10790);
#3724=LINE('',#189662,#10791);
#3725=LINE('',#189667,#10792);
#3726=LINE('',#189673,#10793);
#3727=LINE('',#189682,#10794);
#3728=LINE('',#189686,#10795);
#3729=LINE('',#189691,#10796);
#3730=LINE('',#189697,#10797);
#3731=LINE('',#189706,#10798);
#3732=LINE('',#189710,#10799);
#3733=LINE('',#189715,#10800);
#3734=LINE('',#189721,#10801);
#3735=LINE('',#189730,#10802);
#3736=LINE('',#189734,#10803);
#3737=LINE('',#189739,#10804);
#3738=LINE('',#189745,#10805);
#3739=LINE('',#189754,#10806);
#3740=LINE('',#189758,#10807);
#3741=LINE('',#189763,#10808);
#3742=LINE('',#189769,#10809);
#3743=LINE('',#189778,#10810);
#3744=LINE('',#189782,#10811);
#3745=LINE('',#189787,#10812);
#3746=LINE('',#189793,#10813);
#3747=LINE('',#189802,#10814);
#3748=LINE('',#189806,#10815);
#3749=LINE('',#189811,#10816);
#3750=LINE('',#189817,#10817);
#3751=LINE('',#189826,#10818);
#3752=LINE('',#189830,#10819);
#3753=LINE('',#189835,#10820);
#3754=LINE('',#189841,#10821);
#3755=LINE('',#189850,#10822);
#3756=LINE('',#189854,#10823);
#3757=LINE('',#189859,#10824);
#3758=LINE('',#189865,#10825);
#3759=LINE('',#189874,#10826);
#3760=LINE('',#189878,#10827);
#3761=LINE('',#189883,#10828);
#3762=LINE('',#189889,#10829);
#3763=LINE('',#189898,#10830);
#3764=LINE('',#189902,#10831);
#3765=LINE('',#189907,#10832);
#3766=LINE('',#189913,#10833);
#3767=LINE('',#189922,#10834);
#3768=LINE('',#189926,#10835);
#3769=LINE('',#189931,#10836);
#3770=LINE('',#189937,#10837);
#3771=LINE('',#189946,#10838);
#3772=LINE('',#189950,#10839);
#3773=LINE('',#189955,#10840);
#3774=LINE('',#189961,#10841);
#3775=LINE('',#189970,#10842);
#3776=LINE('',#189974,#10843);
#3777=LINE('',#189979,#10844);
#3778=LINE('',#189985,#10845);
#3779=LINE('',#189994,#10846);
#3780=LINE('',#189998,#10847);
#3781=LINE('',#190003,#10848);
#3782=LINE('',#190009,#10849);
#3783=LINE('',#190018,#10850);
#3784=LINE('',#190022,#10851);
#3785=LINE('',#190027,#10852);
#3786=LINE('',#190033,#10853);
#3787=LINE('',#190042,#10854);
#3788=LINE('',#190046,#10855);
#3789=LINE('',#190051,#10856);
#3790=LINE('',#190057,#10857);
#3791=LINE('',#190066,#10858);
#3792=LINE('',#190070,#10859);
#3793=LINE('',#190075,#10860);
#3794=LINE('',#190081,#10861);
#3795=LINE('',#190090,#10862);
#3796=LINE('',#190094,#10863);
#3797=LINE('',#190099,#10864);
#3798=LINE('',#190105,#10865);
#3799=LINE('',#190114,#10866);
#3800=LINE('',#190118,#10867);
#3801=LINE('',#190123,#10868);
#3802=LINE('',#190129,#10869);
#3803=LINE('',#190138,#10870);
#3804=LINE('',#190142,#10871);
#3805=LINE('',#190147,#10872);
#3806=LINE('',#190153,#10873);
#3807=LINE('',#190162,#10874);
#3808=LINE('',#190166,#10875);
#3809=LINE('',#190171,#10876);
#3810=LINE('',#190177,#10877);
#3811=LINE('',#190186,#10878);
#3812=LINE('',#190190,#10879);
#3813=LINE('',#190195,#10880);
#3814=LINE('',#190201,#10881);
#3815=LINE('',#190210,#10882);
#3816=LINE('',#190214,#10883);
#3817=LINE('',#190219,#10884);
#3818=LINE('',#190225,#10885);
#3819=LINE('',#190234,#10886);
#3820=LINE('',#190238,#10887);
#3821=LINE('',#190243,#10888);
#3822=LINE('',#190245,#10889);
#3823=LINE('',#190251,#10890);
#3824=LINE('',#190252,#10891);
#3825=LINE('',#190255,#10892);
#3826=LINE('',#190262,#10893);
#3827=LINE('',#190266,#10894);
#3828=LINE('',#190271,#10895);
#3829=LINE('',#190273,#10896);
#3830=LINE('',#190279,#10897);
#3831=LINE('',#190280,#10898);
#3832=LINE('',#190285,#10899);
#3833=LINE('',#190292,#10900);
#3834=LINE('',#190296,#10901);
#3835=LINE('',#190301,#10902);
#3836=LINE('',#190303,#10903);
#3837=LINE('',#190309,#10904);
#3838=LINE('',#190310,#10905);
#3839=LINE('',#190315,#10906);
#3840=LINE('',#190322,#10907);
#3841=LINE('',#190326,#10908);
#3842=LINE('',#190331,#10909);
#3843=LINE('',#190333,#10910);
#3844=LINE('',#190339,#10911);
#3845=LINE('',#190340,#10912);
#3846=LINE('',#190345,#10913);
#3847=LINE('',#190352,#10914);
#3848=LINE('',#190356,#10915);
#3849=LINE('',#190361,#10916);
#3850=LINE('',#190363,#10917);
#3851=LINE('',#190369,#10918);
#3852=LINE('',#190370,#10919);
#3853=LINE('',#190375,#10920);
#3854=LINE('',#190382,#10921);
#3855=LINE('',#190384,#10922);
#3856=LINE('',#190388,#10923);
#3857=LINE('',#190393,#10924);
#3858=LINE('',#190394,#10925);
#3859=LINE('',#190399,#10926);
#3860=LINE('',#190400,#10927);
#3861=LINE('',#190405,#10928);
#3862=LINE('',#190412,#10929);
#3863=LINE('',#190414,#10930);
#3864=LINE('',#190418,#10931);
#3865=LINE('',#190423,#10932);
#3866=LINE('',#190424,#10933);
#3867=LINE('',#190429,#10934);
#3868=LINE('',#190430,#10935);
#3869=LINE('',#190435,#10936);
#3870=LINE('',#190442,#10937);
#3871=LINE('',#190446,#10938);
#3872=LINE('',#190451,#10939);
#3873=LINE('',#190453,#10940);
#3874=LINE('',#190459,#10941);
#3875=LINE('',#190460,#10942);
#3876=LINE('',#190465,#10943);
#3877=LINE('',#190472,#10944);
#3878=LINE('',#190476,#10945);
#3879=LINE('',#190481,#10946);
#3880=LINE('',#190483,#10947);
#3881=LINE('',#190489,#10948);
#3882=LINE('',#190490,#10949);
#3883=LINE('',#190495,#10950);
#3884=LINE('',#190502,#10951);
#3885=LINE('',#190506,#10952);
#3886=LINE('',#190511,#10953);
#3887=LINE('',#190513,#10954);
#3888=LINE('',#190519,#10955);
#3889=LINE('',#190520,#10956);
#3890=LINE('',#190525,#10957);
#3891=LINE('',#190532,#10958);
#3892=LINE('',#190536,#10959);
#3893=LINE('',#190541,#10960);
#3894=LINE('',#190547,#10961);
#3895=LINE('',#190556,#10962);
#3896=LINE('',#190560,#10963);
#3897=LINE('',#190565,#10964);
#3898=LINE('',#190571,#10965);
#3899=LINE('',#190580,#10966);
#3900=LINE('',#190584,#10967);
#3901=LINE('',#190589,#10968);
#3902=LINE('',#190595,#10969);
#3903=LINE('',#190604,#10970);
#3904=LINE('',#190608,#10971);
#3905=LINE('',#190613,#10972);
#3906=LINE('',#190619,#10973);
#3907=LINE('',#190628,#10974);
#3908=LINE('',#190632,#10975);
#3909=LINE('',#190637,#10976);
#3910=LINE('',#190643,#10977);
#3911=LINE('',#190652,#10978);
#3912=LINE('',#190656,#10979);
#3913=LINE('',#190661,#10980);
#3914=LINE('',#190667,#10981);
#3915=LINE('',#190676,#10982);
#3916=LINE('',#190680,#10983);
#3917=LINE('',#190685,#10984);
#3918=LINE('',#190691,#10985);
#3919=LINE('',#190700,#10986);
#3920=LINE('',#190704,#10987);
#3921=LINE('',#190709,#10988);
#3922=LINE('',#190715,#10989);
#3923=LINE('',#190724,#10990);
#3924=LINE('',#190726,#10991);
#3925=LINE('',#190730,#10992);
#3926=LINE('',#190735,#10993);
#3927=LINE('',#190736,#10994);
#3928=LINE('',#190741,#10995);
#3929=LINE('',#190742,#10996);
#3930=LINE('',#190747,#10997);
#3931=LINE('',#190754,#10998);
#3932=LINE('',#190756,#10999);
#3933=LINE('',#190760,#11000);
#3934=LINE('',#190765,#11001);
#3935=LINE('',#190766,#11002);
#3936=LINE('',#190771,#11003);
#3937=LINE('',#190772,#11004);
#3938=LINE('',#190777,#11005);
#3939=LINE('',#190784,#11006);
#3940=LINE('',#190788,#11007);
#3941=LINE('',#190793,#11008);
#3942=LINE('',#190799,#11009);
#3943=LINE('',#190808,#11010);
#3944=LINE('',#190812,#11011);
#3945=LINE('',#190817,#11012);
#3946=LINE('',#190823,#11013);
#3947=LINE('',#190832,#11014);
#3948=LINE('',#190836,#11015);
#3949=LINE('',#190841,#11016);
#3950=LINE('',#190847,#11017);
#3951=LINE('',#190856,#11018);
#3952=LINE('',#190860,#11019);
#3953=LINE('',#190865,#11020);
#3954=LINE('',#190871,#11021);
#3955=LINE('',#190880,#11022);
#3956=LINE('',#190884,#11023);
#3957=LINE('',#190889,#11024);
#3958=LINE('',#190895,#11025);
#3959=LINE('',#190897,#11026);
#3960=LINE('',#190903,#11027);
#3961=LINE('',#190910,#11028);
#3962=LINE('',#190914,#11029);
#3963=LINE('',#190919,#11030);
#3964=LINE('',#190921,#11031);
#3965=LINE('',#190927,#11032);
#3966=LINE('',#190928,#11033);
#3967=LINE('',#190933,#11034);
#3968=LINE('',#190940,#11035);
#3969=LINE('',#190944,#11036);
#3970=LINE('',#190949,#11037);
#3971=LINE('',#190951,#11038);
#3972=LINE('',#190957,#11039);
#3973=LINE('',#190958,#11040);
#3974=LINE('',#190963,#11041);
#3975=LINE('',#190970,#11042);
#3976=LINE('',#190974,#11043);
#3977=LINE('',#190979,#11044);
#3978=LINE('',#190985,#11045);
#3979=LINE('',#190987,#11046);
#3980=LINE('',#190993,#11047);
#3981=LINE('',#191000,#11048);
#3982=LINE('',#191004,#11049);
#3983=LINE('',#191009,#11050);
#3984=LINE('',#191015,#11051);
#3985=LINE('',#191024,#11052);
#3986=LINE('',#191028,#11053);
#3987=LINE('',#191033,#11054);
#3988=LINE('',#191039,#11055);
#3989=LINE('',#191048,#11056);
#3990=LINE('',#191052,#11057);
#3991=LINE('',#191057,#11058);
#3992=LINE('',#191063,#11059);
#3993=LINE('',#191072,#11060);
#3994=LINE('',#191076,#11061);
#3995=LINE('',#191081,#11062);
#3996=LINE('',#191087,#11063);
#3997=LINE('',#191096,#11064);
#3998=LINE('',#191100,#11065);
#3999=LINE('',#191105,#11066);
#4000=LINE('',#191111,#11067);
#4001=LINE('',#191120,#11068);
#4002=LINE('',#191124,#11069);
#4003=LINE('',#191129,#11070);
#4004=LINE('',#191135,#11071);
#4005=LINE('',#191144,#11072);
#4006=LINE('',#191148,#11073);
#4007=LINE('',#191153,#11074);
#4008=LINE('',#191159,#11075);
#4009=LINE('',#191168,#11076);
#4010=LINE('',#191172,#11077);
#4011=LINE('',#191177,#11078);
#4012=LINE('',#191183,#11079);
#4013=LINE('',#191192,#11080);
#4014=LINE('',#191196,#11081);
#4015=LINE('',#191201,#11082);
#4016=LINE('',#191207,#11083);
#4017=LINE('',#191216,#11084);
#4018=LINE('',#191220,#11085);
#4019=LINE('',#191225,#11086);
#4020=LINE('',#191231,#11087);
#4021=LINE('',#191240,#11088);
#4022=LINE('',#191244,#11089);
#4023=LINE('',#191249,#11090);
#4024=LINE('',#191255,#11091);
#4025=LINE('',#191257,#11092);
#4026=LINE('',#191263,#11093);
#4027=LINE('',#191270,#11094);
#4028=LINE('',#191274,#11095);
#4029=LINE('',#191279,#11096);
#4030=LINE('',#191285,#11097);
#4031=LINE('',#191287,#11098);
#4032=LINE('',#191293,#11099);
#4033=LINE('',#191300,#11100);
#4034=LINE('',#191304,#11101);
#4035=LINE('',#191309,#11102);
#4036=LINE('',#191315,#11103);
#4037=LINE('',#191324,#11104);
#4038=LINE('',#191328,#11105);
#4039=LINE('',#191333,#11106);
#4040=LINE('',#191339,#11107);
#4041=LINE('',#191348,#11108);
#4042=LINE('',#191352,#11109);
#4043=LINE('',#191357,#11110);
#4044=LINE('',#191363,#11111);
#4045=LINE('',#191372,#11112);
#4046=LINE('',#191376,#11113);
#4047=LINE('',#191381,#11114);
#4048=LINE('',#191387,#11115);
#4049=LINE('',#191396,#11116);
#4050=LINE('',#191400,#11117);
#4051=LINE('',#191405,#11118);
#4052=LINE('',#191411,#11119);
#4053=LINE('',#191420,#11120);
#4054=LINE('',#191424,#11121);
#4055=LINE('',#191429,#11122);
#4056=LINE('',#191435,#11123);
#4057=LINE('',#191444,#11124);
#4058=LINE('',#191448,#11125);
#4059=LINE('',#191453,#11126);
#4060=LINE('',#191459,#11127);
#4061=LINE('',#191468,#11128);
#4062=LINE('',#191472,#11129);
#4063=LINE('',#191477,#11130);
#4064=LINE('',#191483,#11131);
#4065=LINE('',#191492,#11132);
#4066=LINE('',#191496,#11133);
#4067=LINE('',#191501,#11134);
#4068=LINE('',#191507,#11135);
#4069=LINE('',#191516,#11136);
#4070=LINE('',#191520,#11137);
#4071=LINE('',#191525,#11138);
#4072=LINE('',#191527,#11139);
#4073=LINE('',#191533,#11140);
#4074=LINE('',#191534,#11141);
#4075=LINE('',#191539,#11142);
#4076=LINE('',#191546,#11143);
#4077=LINE('',#191550,#11144);
#4078=LINE('',#191555,#11145);
#4079=LINE('',#191561,#11146);
#4080=LINE('',#191563,#11147);
#4081=LINE('',#191569,#11148);
#4082=LINE('',#191576,#11149);
#4083=LINE('',#191580,#11150);
#4084=LINE('',#191585,#11151);
#4085=LINE('',#191591,#11152);
#4086=LINE('',#191600,#11153);
#4087=LINE('',#191604,#11154);
#4088=LINE('',#191609,#11155);
#4089=LINE('',#191615,#11156);
#4090=LINE('',#191624,#11157);
#4091=LINE('',#191628,#11158);
#4092=LINE('',#191633,#11159);
#4093=LINE('',#191639,#11160);
#4094=LINE('',#191648,#11161);
#4095=LINE('',#191652,#11162);
#4096=LINE('',#191657,#11163);
#4097=LINE('',#191663,#11164);
#4098=LINE('',#191672,#11165);
#4099=LINE('',#191676,#11166);
#4100=LINE('',#191681,#11167);
#4101=LINE('',#191687,#11168);
#4102=LINE('',#191696,#11169);
#4103=LINE('',#191700,#11170);
#4104=LINE('',#191705,#11171);
#4105=LINE('',#191711,#11172);
#4106=LINE('',#191720,#11173);
#4107=LINE('',#191724,#11174);
#4108=LINE('',#191729,#11175);
#4109=LINE('',#191735,#11176);
#4110=LINE('',#191744,#11177);
#4111=LINE('',#191748,#11178);
#4112=LINE('',#191753,#11179);
#4113=LINE('',#191759,#11180);
#4114=LINE('',#191768,#11181);
#4115=LINE('',#191772,#11182);
#4116=LINE('',#191777,#11183);
#4117=LINE('',#191783,#11184);
#4118=LINE('',#191792,#11185);
#4119=LINE('',#191796,#11186);
#4120=LINE('',#191801,#11187);
#4121=LINE('',#191807,#11188);
#4122=LINE('',#191816,#11189);
#4123=LINE('',#191820,#11190);
#4124=LINE('',#191825,#11191);
#4125=LINE('',#191831,#11192);
#4126=LINE('',#191840,#11193);
#4127=LINE('',#191844,#11194);
#4128=LINE('',#191849,#11195);
#4129=LINE('',#191855,#11196);
#4130=LINE('',#191864,#11197);
#4131=LINE('',#191868,#11198);
#4132=LINE('',#191873,#11199);
#4133=LINE('',#191879,#11200);
#4134=LINE('',#191888,#11201);
#4135=LINE('',#191892,#11202);
#4136=LINE('',#191897,#11203);
#4137=LINE('',#191903,#11204);
#4138=LINE('',#191912,#11205);
#4139=LINE('',#191916,#11206);
#4140=LINE('',#191921,#11207);
#4141=LINE('',#191927,#11208);
#4142=LINE('',#191936,#11209);
#4143=LINE('',#191940,#11210);
#4144=LINE('',#191945,#11211);
#4145=LINE('',#191951,#11212);
#4146=LINE('',#191960,#11213);
#4147=LINE('',#191964,#11214);
#4148=LINE('',#191969,#11215);
#4149=LINE('',#191975,#11216);
#4150=LINE('',#191984,#11217);
#4151=LINE('',#191988,#11218);
#4152=LINE('',#191993,#11219);
#4153=LINE('',#191999,#11220);
#4154=LINE('',#192008,#11221);
#4155=LINE('',#192012,#11222);
#4156=LINE('',#192017,#11223);
#4157=LINE('',#192023,#11224);
#4158=LINE('',#192032,#11225);
#4159=LINE('',#192036,#11226);
#4160=LINE('',#192041,#11227);
#4161=LINE('',#192047,#11228);
#4162=LINE('',#192056,#11229);
#4163=LINE('',#192060,#11230);
#4164=LINE('',#192065,#11231);
#4165=LINE('',#192071,#11232);
#4166=LINE('',#192080,#11233);
#4167=LINE('',#192084,#11234);
#4168=LINE('',#192089,#11235);
#4169=LINE('',#192095,#11236);
#4170=LINE('',#192104,#11237);
#4171=LINE('',#192108,#11238);
#4172=LINE('',#192113,#11239);
#4173=LINE('',#192119,#11240);
#4174=LINE('',#192128,#11241);
#4175=LINE('',#192132,#11242);
#4176=LINE('',#192137,#11243);
#4177=LINE('',#192143,#11244);
#4178=LINE('',#192152,#11245);
#4179=LINE('',#192156,#11246);
#4180=LINE('',#192161,#11247);
#4181=LINE('',#192167,#11248);
#4182=LINE('',#192176,#11249);
#4183=LINE('',#192180,#11250);
#4184=LINE('',#192185,#11251);
#4185=LINE('',#192191,#11252);
#4186=LINE('',#192200,#11253);
#4187=LINE('',#192204,#11254);
#4188=LINE('',#192209,#11255);
#4189=LINE('',#192215,#11256);
#4190=LINE('',#192224,#11257);
#4191=LINE('',#192228,#11258);
#4192=LINE('',#192233,#11259);
#4193=LINE('',#192239,#11260);
#4194=LINE('',#192248,#11261);
#4195=LINE('',#192252,#11262);
#4196=LINE('',#192257,#11263);
#4197=LINE('',#192263,#11264);
#4198=LINE('',#192272,#11265);
#4199=LINE('',#192276,#11266);
#4200=LINE('',#192281,#11267);
#4201=LINE('',#192287,#11268);
#4202=LINE('',#192296,#11269);
#4203=LINE('',#192300,#11270);
#4204=LINE('',#192305,#11271);
#4205=LINE('',#192311,#11272);
#4206=LINE('',#192320,#11273);
#4207=LINE('',#192324,#11274);
#4208=LINE('',#192329,#11275);
#4209=LINE('',#192335,#11276);
#4210=LINE('',#192344,#11277);
#4211=LINE('',#192348,#11278);
#4212=LINE('',#192353,#11279);
#4213=LINE('',#192359,#11280);
#4214=LINE('',#192368,#11281);
#4215=LINE('',#192372,#11282);
#4216=LINE('',#192377,#11283);
#4217=LINE('',#192383,#11284);
#4218=LINE('',#192392,#11285);
#4219=LINE('',#192396,#11286);
#4220=LINE('',#192401,#11287);
#4221=LINE('',#192407,#11288);
#4222=LINE('',#192416,#11289);
#4223=LINE('',#192420,#11290);
#4224=LINE('',#192425,#11291);
#4225=LINE('',#192431,#11292);
#4226=LINE('',#192440,#11293);
#4227=LINE('',#192444,#11294);
#4228=LINE('',#192449,#11295);
#4229=LINE('',#192455,#11296);
#4230=LINE('',#192464,#11297);
#4231=LINE('',#192468,#11298);
#4232=LINE('',#192473,#11299);
#4233=LINE('',#192479,#11300);
#4234=LINE('',#192488,#11301);
#4235=LINE('',#192492,#11302);
#4236=LINE('',#192497,#11303);
#4237=LINE('',#192503,#11304);
#4238=LINE('',#192512,#11305);
#4239=LINE('',#192516,#11306);
#4240=LINE('',#192521,#11307);
#4241=LINE('',#192527,#11308);
#4242=LINE('',#192536,#11309);
#4243=LINE('',#192540,#11310);
#4244=LINE('',#192545,#11311);
#4245=LINE('',#192551,#11312);
#4246=LINE('',#192560,#11313);
#4247=LINE('',#192564,#11314);
#4248=LINE('',#192569,#11315);
#4249=LINE('',#192575,#11316);
#4250=LINE('',#192584,#11317);
#4251=LINE('',#192588,#11318);
#4252=LINE('',#192593,#11319);
#4253=LINE('',#192599,#11320);
#4254=LINE('',#192608,#11321);
#4255=LINE('',#192612,#11322);
#4256=LINE('',#192617,#11323);
#4257=LINE('',#192623,#11324);
#4258=LINE('',#192632,#11325);
#4259=LINE('',#192636,#11326);
#4260=LINE('',#192641,#11327);
#4261=LINE('',#192647,#11328);
#4262=LINE('',#192656,#11329);
#4263=LINE('',#192660,#11330);
#4264=LINE('',#192665,#11331);
#4265=LINE('',#192671,#11332);
#4266=LINE('',#192680,#11333);
#4267=LINE('',#192684,#11334);
#4268=LINE('',#192689,#11335);
#4269=LINE('',#192695,#11336);
#4270=LINE('',#192704,#11337);
#4271=LINE('',#192708,#11338);
#4272=LINE('',#192713,#11339);
#4273=LINE('',#192719,#11340);
#4274=LINE('',#192728,#11341);
#4275=LINE('',#192732,#11342);
#4276=LINE('',#192737,#11343);
#4277=LINE('',#192743,#11344);
#4278=LINE('',#192752,#11345);
#4279=LINE('',#192756,#11346);
#4280=LINE('',#192761,#11347);
#4281=LINE('',#192767,#11348);
#4282=LINE('',#192776,#11349);
#4283=LINE('',#192780,#11350);
#4284=LINE('',#192785,#11351);
#4285=LINE('',#192791,#11352);
#4286=LINE('',#192800,#11353);
#4287=LINE('',#192804,#11354);
#4288=LINE('',#192809,#11355);
#4289=LINE('',#192815,#11356);
#4290=LINE('',#192824,#11357);
#4291=LINE('',#192828,#11358);
#4292=LINE('',#192833,#11359);
#4293=LINE('',#192839,#11360);
#4294=LINE('',#192848,#11361);
#4295=LINE('',#192852,#11362);
#4296=LINE('',#192857,#11363);
#4297=LINE('',#192863,#11364);
#4298=LINE('',#192872,#11365);
#4299=LINE('',#192876,#11366);
#4300=LINE('',#192881,#11367);
#4301=LINE('',#192887,#11368);
#4302=LINE('',#192896,#11369);
#4303=LINE('',#192900,#11370);
#4304=LINE('',#192905,#11371);
#4305=LINE('',#192911,#11372);
#4306=LINE('',#192920,#11373);
#4307=LINE('',#192924,#11374);
#4308=LINE('',#192929,#11375);
#4309=LINE('',#192935,#11376);
#4310=LINE('',#192944,#11377);
#4311=LINE('',#192948,#11378);
#4312=LINE('',#192953,#11379);
#4313=LINE('',#192959,#11380);
#4314=LINE('',#192968,#11381);
#4315=LINE('',#192972,#11382);
#4316=LINE('',#192977,#11383);
#4317=LINE('',#192983,#11384);
#4318=LINE('',#192992,#11385);
#4319=LINE('',#192996,#11386);
#4320=LINE('',#193001,#11387);
#4321=LINE('',#193007,#11388);
#4322=LINE('',#193016,#11389);
#4323=LINE('',#193020,#11390);
#4324=LINE('',#193025,#11391);
#4325=LINE('',#193031,#11392);
#4326=LINE('',#193040,#11393);
#4327=LINE('',#193044,#11394);
#4328=LINE('',#193049,#11395);
#4329=LINE('',#193055,#11396);
#4330=LINE('',#193064,#11397);
#4331=LINE('',#193068,#11398);
#4332=LINE('',#193073,#11399);
#4333=LINE('',#193079,#11400);
#4334=LINE('',#193088,#11401);
#4335=LINE('',#193092,#11402);
#4336=LINE('',#193097,#11403);
#4337=LINE('',#193103,#11404);
#4338=LINE('',#193112,#11405);
#4339=LINE('',#193116,#11406);
#4340=LINE('',#193121,#11407);
#4341=LINE('',#193127,#11408);
#4342=LINE('',#193136,#11409);
#4343=LINE('',#193140,#11410);
#4344=LINE('',#193145,#11411);
#4345=LINE('',#193151,#11412);
#4346=LINE('',#193160,#11413);
#4347=LINE('',#193164,#11414);
#4348=LINE('',#193169,#11415);
#4349=LINE('',#193175,#11416);
#4350=LINE('',#193184,#11417);
#4351=LINE('',#193188,#11418);
#4352=LINE('',#193193,#11419);
#4353=LINE('',#193199,#11420);
#4354=LINE('',#193208,#11421);
#4355=LINE('',#193212,#11422);
#4356=LINE('',#193217,#11423);
#4357=LINE('',#193223,#11424);
#4358=LINE('',#193232,#11425);
#4359=LINE('',#193236,#11426);
#4360=LINE('',#193241,#11427);
#4361=LINE('',#193247,#11428);
#4362=LINE('',#193256,#11429);
#4363=LINE('',#193260,#11430);
#4364=LINE('',#193265,#11431);
#4365=LINE('',#193271,#11432);
#4366=LINE('',#193280,#11433);
#4367=LINE('',#193284,#11434);
#4368=LINE('',#193289,#11435);
#4369=LINE('',#193295,#11436);
#4370=LINE('',#193304,#11437);
#4371=LINE('',#193308,#11438);
#4372=LINE('',#193313,#11439);
#4373=LINE('',#193319,#11440);
#4374=LINE('',#193328,#11441);
#4375=LINE('',#193332,#11442);
#4376=LINE('',#193337,#11443);
#4377=LINE('',#193343,#11444);
#4378=LINE('',#193352,#11445);
#4379=LINE('',#193356,#11446);
#4380=LINE('',#193361,#11447);
#4381=LINE('',#193367,#11448);
#4382=LINE('',#193376,#11449);
#4383=LINE('',#193380,#11450);
#4384=LINE('',#193385,#11451);
#4385=LINE('',#193391,#11452);
#4386=LINE('',#193400,#11453);
#4387=LINE('',#193404,#11454);
#4388=LINE('',#193409,#11455);
#4389=LINE('',#193415,#11456);
#4390=LINE('',#193425,#11457);
#4391=LINE('',#193427,#11458);
#4392=LINE('',#193429,#11459);
#4393=LINE('',#193430,#11460);
#4394=LINE('',#193434,#11461);
#4395=LINE('',#193435,#11462);
#4396=LINE('',#193436,#11463);
#4397=LINE('',#193440,#11464);
#4398=LINE('',#193441,#11465);
#4399=LINE('',#193442,#11466);
#4400=LINE('',#193444,#11467);
#4401=LINE('',#193445,#11468);
#4402=LINE('',#193449,#11469);
#4403=LINE('',#193451,#11470);
#4404=LINE('',#193453,#11471);
#4405=LINE('',#193454,#11472);
#4406=LINE('',#193458,#11473);
#4407=LINE('',#193459,#11474);
#4408=LINE('',#193460,#11475);
#4409=LINE('',#193464,#11476);
#4410=LINE('',#193465,#11477);
#4411=LINE('',#193466,#11478);
#4412=LINE('',#193468,#11479);
#4413=LINE('',#193469,#11480);
#4414=LINE('',#193473,#11481);
#4415=LINE('',#193475,#11482);
#4416=LINE('',#193477,#11483);
#4417=LINE('',#193478,#11484);
#4418=LINE('',#193482,#11485);
#4419=LINE('',#193483,#11486);
#4420=LINE('',#193484,#11487);
#4421=LINE('',#193488,#11488);
#4422=LINE('',#193489,#11489);
#4423=LINE('',#193490,#11490);
#4424=LINE('',#193492,#11491);
#4425=LINE('',#193493,#11492);
#4426=LINE('',#193497,#11493);
#4427=LINE('',#193499,#11494);
#4428=LINE('',#193501,#11495);
#4429=LINE('',#193502,#11496);
#4430=LINE('',#193506,#11497);
#4431=LINE('',#193507,#11498);
#4432=LINE('',#193508,#11499);
#4433=LINE('',#193512,#11500);
#4434=LINE('',#193513,#11501);
#4435=LINE('',#193514,#11502);
#4436=LINE('',#193516,#11503);
#4437=LINE('',#193517,#11504);
#4438=LINE('',#193521,#11505);
#4439=LINE('',#193523,#11506);
#4440=LINE('',#193525,#11507);
#4441=LINE('',#193526,#11508);
#4442=LINE('',#193530,#11509);
#4443=LINE('',#193531,#11510);
#4444=LINE('',#193532,#11511);
#4445=LINE('',#193536,#11512);
#4446=LINE('',#193537,#11513);
#4447=LINE('',#193538,#11514);
#4448=LINE('',#193540,#11515);
#4449=LINE('',#193541,#11516);
#4450=LINE('',#193545,#11517);
#4451=LINE('',#193547,#11518);
#4452=LINE('',#193549,#11519);
#4453=LINE('',#193550,#11520);
#4454=LINE('',#193554,#11521);
#4455=LINE('',#193555,#11522);
#4456=LINE('',#193556,#11523);
#4457=LINE('',#193560,#11524);
#4458=LINE('',#193561,#11525);
#4459=LINE('',#193562,#11526);
#4460=LINE('',#193564,#11527);
#4461=LINE('',#193565,#11528);
#4462=LINE('',#193569,#11529);
#4463=LINE('',#193571,#11530);
#4464=LINE('',#193573,#11531);
#4465=LINE('',#193574,#11532);
#4466=LINE('',#193578,#11533);
#4467=LINE('',#193579,#11534);
#4468=LINE('',#193580,#11535);
#4469=LINE('',#193584,#11536);
#4470=LINE('',#193585,#11537);
#4471=LINE('',#193586,#11538);
#4472=LINE('',#193588,#11539);
#4473=LINE('',#193589,#11540);
#4474=LINE('',#193593,#11541);
#4475=LINE('',#193595,#11542);
#4476=LINE('',#193597,#11543);
#4477=LINE('',#193598,#11544);
#4478=LINE('',#193602,#11545);
#4479=LINE('',#193603,#11546);
#4480=LINE('',#193604,#11547);
#4481=LINE('',#193608,#11548);
#4482=LINE('',#193609,#11549);
#4483=LINE('',#193610,#11550);
#4484=LINE('',#193612,#11551);
#4485=LINE('',#193613,#11552);
#4486=LINE('',#193617,#11553);
#4487=LINE('',#193619,#11554);
#4488=LINE('',#193621,#11555);
#4489=LINE('',#193622,#11556);
#4490=LINE('',#193626,#11557);
#4491=LINE('',#193627,#11558);
#4492=LINE('',#193628,#11559);
#4493=LINE('',#193632,#11560);
#4494=LINE('',#193633,#11561);
#4495=LINE('',#193634,#11562);
#4496=LINE('',#193636,#11563);
#4497=LINE('',#193637,#11564);
#4498=LINE('',#193641,#11565);
#4499=LINE('',#193643,#11566);
#4500=LINE('',#193645,#11567);
#4501=LINE('',#193646,#11568);
#4502=LINE('',#193650,#11569);
#4503=LINE('',#193651,#11570);
#4504=LINE('',#193652,#11571);
#4505=LINE('',#193656,#11572);
#4506=LINE('',#193657,#11573);
#4507=LINE('',#193658,#11574);
#4508=LINE('',#193660,#11575);
#4509=LINE('',#193661,#11576);
#4510=LINE('',#193665,#11577);
#4511=LINE('',#193667,#11578);
#4512=LINE('',#193669,#11579);
#4513=LINE('',#193670,#11580);
#4514=LINE('',#193674,#11581);
#4515=LINE('',#193675,#11582);
#4516=LINE('',#193676,#11583);
#4517=LINE('',#193680,#11584);
#4518=LINE('',#193681,#11585);
#4519=LINE('',#193682,#11586);
#4520=LINE('',#193684,#11587);
#4521=LINE('',#193685,#11588);
#4522=LINE('',#193689,#11589);
#4523=LINE('',#193691,#11590);
#4524=LINE('',#193693,#11591);
#4525=LINE('',#193694,#11592);
#4526=LINE('',#193698,#11593);
#4527=LINE('',#193699,#11594);
#4528=LINE('',#193700,#11595);
#4529=LINE('',#193704,#11596);
#4530=LINE('',#193705,#11597);
#4531=LINE('',#193706,#11598);
#4532=LINE('',#193708,#11599);
#4533=LINE('',#193709,#11600);
#4534=LINE('',#193713,#11601);
#4535=LINE('',#193715,#11602);
#4536=LINE('',#193717,#11603);
#4537=LINE('',#193718,#11604);
#4538=LINE('',#193722,#11605);
#4539=LINE('',#193723,#11606);
#4540=LINE('',#193724,#11607);
#4541=LINE('',#193728,#11608);
#4542=LINE('',#193729,#11609);
#4543=LINE('',#193730,#11610);
#4544=LINE('',#193732,#11611);
#4545=LINE('',#193733,#11612);
#4546=LINE('',#193737,#11613);
#4547=LINE('',#193739,#11614);
#4548=LINE('',#193741,#11615);
#4549=LINE('',#193742,#11616);
#4550=LINE('',#193746,#11617);
#4551=LINE('',#193747,#11618);
#4552=LINE('',#193748,#11619);
#4553=LINE('',#193752,#11620);
#4554=LINE('',#193753,#11621);
#4555=LINE('',#193754,#11622);
#4556=LINE('',#193756,#11623);
#4557=LINE('',#193757,#11624);
#4558=LINE('',#193761,#11625);
#4559=LINE('',#193763,#11626);
#4560=LINE('',#193765,#11627);
#4561=LINE('',#193766,#11628);
#4562=LINE('',#193770,#11629);
#4563=LINE('',#193771,#11630);
#4564=LINE('',#193772,#11631);
#4565=LINE('',#193776,#11632);
#4566=LINE('',#193777,#11633);
#4567=LINE('',#193778,#11634);
#4568=LINE('',#193780,#11635);
#4569=LINE('',#193781,#11636);
#4570=LINE('',#193785,#11637);
#4571=LINE('',#193787,#11638);
#4572=LINE('',#193789,#11639);
#4573=LINE('',#193790,#11640);
#4574=LINE('',#193794,#11641);
#4575=LINE('',#193795,#11642);
#4576=LINE('',#193796,#11643);
#4577=LINE('',#193800,#11644);
#4578=LINE('',#193801,#11645);
#4579=LINE('',#193802,#11646);
#4580=LINE('',#193804,#11647);
#4581=LINE('',#193805,#11648);
#4582=LINE('',#193809,#11649);
#4583=LINE('',#193811,#11650);
#4584=LINE('',#193813,#11651);
#4585=LINE('',#193814,#11652);
#4586=LINE('',#193818,#11653);
#4587=LINE('',#193819,#11654);
#4588=LINE('',#193820,#11655);
#4589=LINE('',#193824,#11656);
#4590=LINE('',#193825,#11657);
#4591=LINE('',#193826,#11658);
#4592=LINE('',#193828,#11659);
#4593=LINE('',#193829,#11660);
#4594=LINE('',#193833,#11661);
#4595=LINE('',#193835,#11662);
#4596=LINE('',#193837,#11663);
#4597=LINE('',#193838,#11664);
#4598=LINE('',#193842,#11665);
#4599=LINE('',#193843,#11666);
#4600=LINE('',#193844,#11667);
#4601=LINE('',#193848,#11668);
#4602=LINE('',#193849,#11669);
#4603=LINE('',#193850,#11670);
#4604=LINE('',#193852,#11671);
#4605=LINE('',#193853,#11672);
#4606=LINE('',#193857,#11673);
#4607=LINE('',#193859,#11674);
#4608=LINE('',#193861,#11675);
#4609=LINE('',#193862,#11676);
#4610=LINE('',#193866,#11677);
#4611=LINE('',#193867,#11678);
#4612=LINE('',#193868,#11679);
#4613=LINE('',#193872,#11680);
#4614=LINE('',#193873,#11681);
#4615=LINE('',#193874,#11682);
#4616=LINE('',#193876,#11683);
#4617=LINE('',#193877,#11684);
#4618=LINE('',#193881,#11685);
#4619=LINE('',#193883,#11686);
#4620=LINE('',#193885,#11687);
#4621=LINE('',#193886,#11688);
#4622=LINE('',#193890,#11689);
#4623=LINE('',#193891,#11690);
#4624=LINE('',#193892,#11691);
#4625=LINE('',#193896,#11692);
#4626=LINE('',#193897,#11693);
#4627=LINE('',#193898,#11694);
#4628=LINE('',#193900,#11695);
#4629=LINE('',#193901,#11696);
#4630=LINE('',#193905,#11697);
#4631=LINE('',#193907,#11698);
#4632=LINE('',#193909,#11699);
#4633=LINE('',#193910,#11700);
#4634=LINE('',#193914,#11701);
#4635=LINE('',#193915,#11702);
#4636=LINE('',#193916,#11703);
#4637=LINE('',#193920,#11704);
#4638=LINE('',#193921,#11705);
#4639=LINE('',#193922,#11706);
#4640=LINE('',#193924,#11707);
#4641=LINE('',#193925,#11708);
#4642=LINE('',#193929,#11709);
#4643=LINE('',#193931,#11710);
#4644=LINE('',#193933,#11711);
#4645=LINE('',#193934,#11712);
#4646=LINE('',#193938,#11713);
#4647=LINE('',#193939,#11714);
#4648=LINE('',#193940,#11715);
#4649=LINE('',#193944,#11716);
#4650=LINE('',#193945,#11717);
#4651=LINE('',#193946,#11718);
#4652=LINE('',#193948,#11719);
#4653=LINE('',#193949,#11720);
#4654=LINE('',#193953,#11721);
#4655=LINE('',#193955,#11722);
#4656=LINE('',#193957,#11723);
#4657=LINE('',#193958,#11724);
#4658=LINE('',#193962,#11725);
#4659=LINE('',#193963,#11726);
#4660=LINE('',#193964,#11727);
#4661=LINE('',#193968,#11728);
#4662=LINE('',#193969,#11729);
#4663=LINE('',#193970,#11730);
#4664=LINE('',#193972,#11731);
#4665=LINE('',#193973,#11732);
#4666=LINE('',#193977,#11733);
#4667=LINE('',#193979,#11734);
#4668=LINE('',#193981,#11735);
#4669=LINE('',#193982,#11736);
#4670=LINE('',#193986,#11737);
#4671=LINE('',#193987,#11738);
#4672=LINE('',#193988,#11739);
#4673=LINE('',#193992,#11740);
#4674=LINE('',#193993,#11741);
#4675=LINE('',#193994,#11742);
#4676=LINE('',#193996,#11743);
#4677=LINE('',#193997,#11744);
#4678=LINE('',#194001,#11745);
#4679=LINE('',#194003,#11746);
#4680=LINE('',#194005,#11747);
#4681=LINE('',#194006,#11748);
#4682=LINE('',#194010,#11749);
#4683=LINE('',#194011,#11750);
#4684=LINE('',#194012,#11751);
#4685=LINE('',#194016,#11752);
#4686=LINE('',#194017,#11753);
#4687=LINE('',#194018,#11754);
#4688=LINE('',#194020,#11755);
#4689=LINE('',#194021,#11756);
#4690=LINE('',#194025,#11757);
#4691=LINE('',#194027,#11758);
#4692=LINE('',#194029,#11759);
#4693=LINE('',#194030,#11760);
#4694=LINE('',#194034,#11761);
#4695=LINE('',#194035,#11762);
#4696=LINE('',#194036,#11763);
#4697=LINE('',#194040,#11764);
#4698=LINE('',#194041,#11765);
#4699=LINE('',#194042,#11766);
#4700=LINE('',#194044,#11767);
#4701=LINE('',#194045,#11768);
#4702=LINE('',#194049,#11769);
#4703=LINE('',#194051,#11770);
#4704=LINE('',#194053,#11771);
#4705=LINE('',#194054,#11772);
#4706=LINE('',#194058,#11773);
#4707=LINE('',#194059,#11774);
#4708=LINE('',#194060,#11775);
#4709=LINE('',#194064,#11776);
#4710=LINE('',#194065,#11777);
#4711=LINE('',#194066,#11778);
#4712=LINE('',#194068,#11779);
#4713=LINE('',#194069,#11780);
#4714=LINE('',#194073,#11781);
#4715=LINE('',#194075,#11782);
#4716=LINE('',#194077,#11783);
#4717=LINE('',#194078,#11784);
#4718=LINE('',#194082,#11785);
#4719=LINE('',#194083,#11786);
#4720=LINE('',#194084,#11787);
#4721=LINE('',#194088,#11788);
#4722=LINE('',#194089,#11789);
#4723=LINE('',#194090,#11790);
#4724=LINE('',#194092,#11791);
#4725=LINE('',#194093,#11792);
#4726=LINE('',#194097,#11793);
#4727=LINE('',#194099,#11794);
#4728=LINE('',#194101,#11795);
#4729=LINE('',#194102,#11796);
#4730=LINE('',#194106,#11797);
#4731=LINE('',#194107,#11798);
#4732=LINE('',#194108,#11799);
#4733=LINE('',#194112,#11800);
#4734=LINE('',#194113,#11801);
#4735=LINE('',#194114,#11802);
#4736=LINE('',#194116,#11803);
#4737=LINE('',#194117,#11804);
#4738=LINE('',#194121,#11805);
#4739=LINE('',#194123,#11806);
#4740=LINE('',#194125,#11807);
#4741=LINE('',#194126,#11808);
#4742=LINE('',#194130,#11809);
#4743=LINE('',#194131,#11810);
#4744=LINE('',#194132,#11811);
#4745=LINE('',#194136,#11812);
#4746=LINE('',#194137,#11813);
#4747=LINE('',#194138,#11814);
#4748=LINE('',#194140,#11815);
#4749=LINE('',#194141,#11816);
#4750=LINE('',#194145,#11817);
#4751=LINE('',#194147,#11818);
#4752=LINE('',#194149,#11819);
#4753=LINE('',#194150,#11820);
#4754=LINE('',#194154,#11821);
#4755=LINE('',#194155,#11822);
#4756=LINE('',#194156,#11823);
#4757=LINE('',#194160,#11824);
#4758=LINE('',#194161,#11825);
#4759=LINE('',#194162,#11826);
#4760=LINE('',#194164,#11827);
#4761=LINE('',#194165,#11828);
#4762=LINE('',#194169,#11829);
#4763=LINE('',#194171,#11830);
#4764=LINE('',#194173,#11831);
#4765=LINE('',#194174,#11832);
#4766=LINE('',#194178,#11833);
#4767=LINE('',#194179,#11834);
#4768=LINE('',#194180,#11835);
#4769=LINE('',#194184,#11836);
#4770=LINE('',#194185,#11837);
#4771=LINE('',#194186,#11838);
#4772=LINE('',#194188,#11839);
#4773=LINE('',#194189,#11840);
#4774=LINE('',#194193,#11841);
#4775=LINE('',#194195,#11842);
#4776=LINE('',#194197,#11843);
#4777=LINE('',#194198,#11844);
#4778=LINE('',#194202,#11845);
#4779=LINE('',#194203,#11846);
#4780=LINE('',#194204,#11847);
#4781=LINE('',#194208,#11848);
#4782=LINE('',#194209,#11849);
#4783=LINE('',#194210,#11850);
#4784=LINE('',#194212,#11851);
#4785=LINE('',#194213,#11852);
#4786=LINE('',#194217,#11853);
#4787=LINE('',#194219,#11854);
#4788=LINE('',#194221,#11855);
#4789=LINE('',#194222,#11856);
#4790=LINE('',#194226,#11857);
#4791=LINE('',#194227,#11858);
#4792=LINE('',#194228,#11859);
#4793=LINE('',#194232,#11860);
#4794=LINE('',#194233,#11861);
#4795=LINE('',#194234,#11862);
#4796=LINE('',#194236,#11863);
#4797=LINE('',#194237,#11864);
#4798=LINE('',#194241,#11865);
#4799=LINE('',#194243,#11866);
#4800=LINE('',#194245,#11867);
#4801=LINE('',#194246,#11868);
#4802=LINE('',#194250,#11869);
#4803=LINE('',#194251,#11870);
#4804=LINE('',#194252,#11871);
#4805=LINE('',#194256,#11872);
#4806=LINE('',#194257,#11873);
#4807=LINE('',#194258,#11874);
#4808=LINE('',#194260,#11875);
#4809=LINE('',#194261,#11876);
#4810=LINE('',#194265,#11877);
#4811=LINE('',#194267,#11878);
#4812=LINE('',#194269,#11879);
#4813=LINE('',#194270,#11880);
#4814=LINE('',#194274,#11881);
#4815=LINE('',#194275,#11882);
#4816=LINE('',#194276,#11883);
#4817=LINE('',#194280,#11884);
#4818=LINE('',#194281,#11885);
#4819=LINE('',#194282,#11886);
#4820=LINE('',#194284,#11887);
#4821=LINE('',#194285,#11888);
#4822=LINE('',#194289,#11889);
#4823=LINE('',#194291,#11890);
#4824=LINE('',#194293,#11891);
#4825=LINE('',#194294,#11892);
#4826=LINE('',#194298,#11893);
#4827=LINE('',#194299,#11894);
#4828=LINE('',#194300,#11895);
#4829=LINE('',#194304,#11896);
#4830=LINE('',#194305,#11897);
#4831=LINE('',#194306,#11898);
#4832=LINE('',#194308,#11899);
#4833=LINE('',#194309,#11900);
#4834=LINE('',#194313,#11901);
#4835=LINE('',#194315,#11902);
#4836=LINE('',#194317,#11903);
#4837=LINE('',#194318,#11904);
#4838=LINE('',#194322,#11905);
#4839=LINE('',#194323,#11906);
#4840=LINE('',#194324,#11907);
#4841=LINE('',#194328,#11908);
#4842=LINE('',#194329,#11909);
#4843=LINE('',#194330,#11910);
#4844=LINE('',#194332,#11911);
#4845=LINE('',#194333,#11912);
#4846=LINE('',#194337,#11913);
#4847=LINE('',#194339,#11914);
#4848=LINE('',#194341,#11915);
#4849=LINE('',#194342,#11916);
#4850=LINE('',#194346,#11917);
#4851=LINE('',#194347,#11918);
#4852=LINE('',#194348,#11919);
#4853=LINE('',#194352,#11920);
#4854=LINE('',#194353,#11921);
#4855=LINE('',#194354,#11922);
#4856=LINE('',#194356,#11923);
#4857=LINE('',#194357,#11924);
#4858=LINE('',#194361,#11925);
#4859=LINE('',#194363,#11926);
#4860=LINE('',#194365,#11927);
#4861=LINE('',#194366,#11928);
#4862=LINE('',#194370,#11929);
#4863=LINE('',#194371,#11930);
#4864=LINE('',#194372,#11931);
#4865=LINE('',#194376,#11932);
#4866=LINE('',#194377,#11933);
#4867=LINE('',#194378,#11934);
#4868=LINE('',#194380,#11935);
#4869=LINE('',#194381,#11936);
#4870=LINE('',#194385,#11937);
#4871=LINE('',#194387,#11938);
#4872=LINE('',#194389,#11939);
#4873=LINE('',#194390,#11940);
#4874=LINE('',#194394,#11941);
#4875=LINE('',#194395,#11942);
#4876=LINE('',#194396,#11943);
#4877=LINE('',#194400,#11944);
#4878=LINE('',#194401,#11945);
#4879=LINE('',#194402,#11946);
#4880=LINE('',#194404,#11947);
#4881=LINE('',#194405,#11948);
#4882=LINE('',#194409,#11949);
#4883=LINE('',#194411,#11950);
#4884=LINE('',#194413,#11951);
#4885=LINE('',#194414,#11952);
#4886=LINE('',#194418,#11953);
#4887=LINE('',#194419,#11954);
#4888=LINE('',#194420,#11955);
#4889=LINE('',#194424,#11956);
#4890=LINE('',#194425,#11957);
#4891=LINE('',#194426,#11958);
#4892=LINE('',#194428,#11959);
#4893=LINE('',#194429,#11960);
#4894=LINE('',#194433,#11961);
#4895=LINE('',#194435,#11962);
#4896=LINE('',#194437,#11963);
#4897=LINE('',#194438,#11964);
#4898=LINE('',#194442,#11965);
#4899=LINE('',#194443,#11966);
#4900=LINE('',#194444,#11967);
#4901=LINE('',#194448,#11968);
#4902=LINE('',#194449,#11969);
#4903=LINE('',#194450,#11970);
#4904=LINE('',#194452,#11971);
#4905=LINE('',#194453,#11972);
#4906=LINE('',#194457,#11973);
#4907=LINE('',#194459,#11974);
#4908=LINE('',#194461,#11975);
#4909=LINE('',#194462,#11976);
#4910=LINE('',#194466,#11977);
#4911=LINE('',#194467,#11978);
#4912=LINE('',#194468,#11979);
#4913=LINE('',#194472,#11980);
#4914=LINE('',#194473,#11981);
#4915=LINE('',#194474,#11982);
#4916=LINE('',#194476,#11983);
#4917=LINE('',#194477,#11984);
#4918=LINE('',#194481,#11985);
#4919=LINE('',#194483,#11986);
#4920=LINE('',#194485,#11987);
#4921=LINE('',#194486,#11988);
#4922=LINE('',#194490,#11989);
#4923=LINE('',#194491,#11990);
#4924=LINE('',#194492,#11991);
#4925=LINE('',#194496,#11992);
#4926=LINE('',#194497,#11993);
#4927=LINE('',#194498,#11994);
#4928=LINE('',#194500,#11995);
#4929=LINE('',#194501,#11996);
#4930=LINE('',#194505,#11997);
#4931=LINE('',#194507,#11998);
#4932=LINE('',#194509,#11999);
#4933=LINE('',#194510,#12000);
#4934=LINE('',#194514,#12001);
#4935=LINE('',#194515,#12002);
#4936=LINE('',#194516,#12003);
#4937=LINE('',#194520,#12004);
#4938=LINE('',#194521,#12005);
#4939=LINE('',#194522,#12006);
#4940=LINE('',#194524,#12007);
#4941=LINE('',#194525,#12008);
#4942=LINE('',#194529,#12009);
#4943=LINE('',#194531,#12010);
#4944=LINE('',#194533,#12011);
#4945=LINE('',#194534,#12012);
#4946=LINE('',#194538,#12013);
#4947=LINE('',#194539,#12014);
#4948=LINE('',#194540,#12015);
#4949=LINE('',#194544,#12016);
#4950=LINE('',#194545,#12017);
#4951=LINE('',#194546,#12018);
#4952=LINE('',#194548,#12019);
#4953=LINE('',#194549,#12020);
#4954=LINE('',#194553,#12021);
#4955=LINE('',#194555,#12022);
#4956=LINE('',#194557,#12023);
#4957=LINE('',#194558,#12024);
#4958=LINE('',#194562,#12025);
#4959=LINE('',#194563,#12026);
#4960=LINE('',#194564,#12027);
#4961=LINE('',#194568,#12028);
#4962=LINE('',#194569,#12029);
#4963=LINE('',#194570,#12030);
#4964=LINE('',#194572,#12031);
#4965=LINE('',#194573,#12032);
#4966=LINE('',#194577,#12033);
#4967=LINE('',#194579,#12034);
#4968=LINE('',#194581,#12035);
#4969=LINE('',#194582,#12036);
#4970=LINE('',#194586,#12037);
#4971=LINE('',#194587,#12038);
#4972=LINE('',#194588,#12039);
#4973=LINE('',#194592,#12040);
#4974=LINE('',#194593,#12041);
#4975=LINE('',#194594,#12042);
#4976=LINE('',#194596,#12043);
#4977=LINE('',#194597,#12044);
#4978=LINE('',#194601,#12045);
#4979=LINE('',#194603,#12046);
#4980=LINE('',#194605,#12047);
#4981=LINE('',#194606,#12048);
#4982=LINE('',#194610,#12049);
#4983=LINE('',#194611,#12050);
#4984=LINE('',#194612,#12051);
#4985=LINE('',#194616,#12052);
#4986=LINE('',#194617,#12053);
#4987=LINE('',#194618,#12054);
#4988=LINE('',#194620,#12055);
#4989=LINE('',#194621,#12056);
#4990=LINE('',#194625,#12057);
#4991=LINE('',#194627,#12058);
#4992=LINE('',#194629,#12059);
#4993=LINE('',#194630,#12060);
#4994=LINE('',#194634,#12061);
#4995=LINE('',#194635,#12062);
#4996=LINE('',#194636,#12063);
#4997=LINE('',#194640,#12064);
#4998=LINE('',#194641,#12065);
#4999=LINE('',#194642,#12066);
#5000=LINE('',#194644,#12067);
#5001=LINE('',#194645,#12068);
#5002=LINE('',#194649,#12069);
#5003=LINE('',#194651,#12070);
#5004=LINE('',#194653,#12071);
#5005=LINE('',#194654,#12072);
#5006=LINE('',#194658,#12073);
#5007=LINE('',#194659,#12074);
#5008=LINE('',#194660,#12075);
#5009=LINE('',#194664,#12076);
#5010=LINE('',#194665,#12077);
#5011=LINE('',#194666,#12078);
#5012=LINE('',#194668,#12079);
#5013=LINE('',#194669,#12080);
#5014=LINE('',#194673,#12081);
#5015=LINE('',#194675,#12082);
#5016=LINE('',#194677,#12083);
#5017=LINE('',#194678,#12084);
#5018=LINE('',#194682,#12085);
#5019=LINE('',#194683,#12086);
#5020=LINE('',#194684,#12087);
#5021=LINE('',#194688,#12088);
#5022=LINE('',#194689,#12089);
#5023=LINE('',#194690,#12090);
#5024=LINE('',#194692,#12091);
#5025=LINE('',#194693,#12092);
#5026=LINE('',#194697,#12093);
#5027=LINE('',#194699,#12094);
#5028=LINE('',#194701,#12095);
#5029=LINE('',#194702,#12096);
#5030=LINE('',#194706,#12097);
#5031=LINE('',#194707,#12098);
#5032=LINE('',#194708,#12099);
#5033=LINE('',#194712,#12100);
#5034=LINE('',#194713,#12101);
#5035=LINE('',#194714,#12102);
#5036=LINE('',#194716,#12103);
#5037=LINE('',#194717,#12104);
#5038=LINE('',#194721,#12105);
#5039=LINE('',#194723,#12106);
#5040=LINE('',#194725,#12107);
#5041=LINE('',#194726,#12108);
#5042=LINE('',#194730,#12109);
#5043=LINE('',#194731,#12110);
#5044=LINE('',#194732,#12111);
#5045=LINE('',#194736,#12112);
#5046=LINE('',#194737,#12113);
#5047=LINE('',#194738,#12114);
#5048=LINE('',#194740,#12115);
#5049=LINE('',#194741,#12116);
#5050=LINE('',#194745,#12117);
#5051=LINE('',#194747,#12118);
#5052=LINE('',#194749,#12119);
#5053=LINE('',#194750,#12120);
#5054=LINE('',#194754,#12121);
#5055=LINE('',#194755,#12122);
#5056=LINE('',#194756,#12123);
#5057=LINE('',#194760,#12124);
#5058=LINE('',#194761,#12125);
#5059=LINE('',#194762,#12126);
#5060=LINE('',#194764,#12127);
#5061=LINE('',#194765,#12128);
#5062=LINE('',#194769,#12129);
#5063=LINE('',#194771,#12130);
#5064=LINE('',#194773,#12131);
#5065=LINE('',#194774,#12132);
#5066=LINE('',#194778,#12133);
#5067=LINE('',#194779,#12134);
#5068=LINE('',#194780,#12135);
#5069=LINE('',#194784,#12136);
#5070=LINE('',#194785,#12137);
#5071=LINE('',#194786,#12138);
#5072=LINE('',#194788,#12139);
#5073=LINE('',#194789,#12140);
#5074=LINE('',#194793,#12141);
#5075=LINE('',#194795,#12142);
#5076=LINE('',#194797,#12143);
#5077=LINE('',#194798,#12144);
#5078=LINE('',#194802,#12145);
#5079=LINE('',#194803,#12146);
#5080=LINE('',#194804,#12147);
#5081=LINE('',#194808,#12148);
#5082=LINE('',#194809,#12149);
#5083=LINE('',#194810,#12150);
#5084=LINE('',#194812,#12151);
#5085=LINE('',#194813,#12152);
#5086=LINE('',#194817,#12153);
#5087=LINE('',#194819,#12154);
#5088=LINE('',#194821,#12155);
#5089=LINE('',#194822,#12156);
#5090=LINE('',#194826,#12157);
#5091=LINE('',#194827,#12158);
#5092=LINE('',#194828,#12159);
#5093=LINE('',#194832,#12160);
#5094=LINE('',#194833,#12161);
#5095=LINE('',#194834,#12162);
#5096=LINE('',#194836,#12163);
#5097=LINE('',#194837,#12164);
#5098=LINE('',#194841,#12165);
#5099=LINE('',#194843,#12166);
#5100=LINE('',#194845,#12167);
#5101=LINE('',#194846,#12168);
#5102=LINE('',#194850,#12169);
#5103=LINE('',#194851,#12170);
#5104=LINE('',#194852,#12171);
#5105=LINE('',#194856,#12172);
#5106=LINE('',#194857,#12173);
#5107=LINE('',#194858,#12174);
#5108=LINE('',#194860,#12175);
#5109=LINE('',#194861,#12176);
#5110=LINE('',#194865,#12177);
#5111=LINE('',#194867,#12178);
#5112=LINE('',#194869,#12179);
#5113=LINE('',#194870,#12180);
#5114=LINE('',#194874,#12181);
#5115=LINE('',#194875,#12182);
#5116=LINE('',#194876,#12183);
#5117=LINE('',#194880,#12184);
#5118=LINE('',#194881,#12185);
#5119=LINE('',#194882,#12186);
#5120=LINE('',#194884,#12187);
#5121=LINE('',#194885,#12188);
#5122=LINE('',#194889,#12189);
#5123=LINE('',#194891,#12190);
#5124=LINE('',#194893,#12191);
#5125=LINE('',#194894,#12192);
#5126=LINE('',#194898,#12193);
#5127=LINE('',#194899,#12194);
#5128=LINE('',#194900,#12195);
#5129=LINE('',#194904,#12196);
#5130=LINE('',#194905,#12197);
#5131=LINE('',#194906,#12198);
#5132=LINE('',#194908,#12199);
#5133=LINE('',#194909,#12200);
#5134=LINE('',#194913,#12201);
#5135=LINE('',#194915,#12202);
#5136=LINE('',#194917,#12203);
#5137=LINE('',#194918,#12204);
#5138=LINE('',#194922,#12205);
#5139=LINE('',#194923,#12206);
#5140=LINE('',#194924,#12207);
#5141=LINE('',#194928,#12208);
#5142=LINE('',#194929,#12209);
#5143=LINE('',#194930,#12210);
#5144=LINE('',#194932,#12211);
#5145=LINE('',#194933,#12212);
#5146=LINE('',#194937,#12213);
#5147=LINE('',#194939,#12214);
#5148=LINE('',#194941,#12215);
#5149=LINE('',#194942,#12216);
#5150=LINE('',#194946,#12217);
#5151=LINE('',#194947,#12218);
#5152=LINE('',#194948,#12219);
#5153=LINE('',#194952,#12220);
#5154=LINE('',#194953,#12221);
#5155=LINE('',#194954,#12222);
#5156=LINE('',#194956,#12223);
#5157=LINE('',#194957,#12224);
#5158=LINE('',#194961,#12225);
#5159=LINE('',#194963,#12226);
#5160=LINE('',#194965,#12227);
#5161=LINE('',#194966,#12228);
#5162=LINE('',#194970,#12229);
#5163=LINE('',#194971,#12230);
#5164=LINE('',#194972,#12231);
#5165=LINE('',#194976,#12232);
#5166=LINE('',#194977,#12233);
#5167=LINE('',#194978,#12234);
#5168=LINE('',#194980,#12235);
#5169=LINE('',#194981,#12236);
#5170=LINE('',#194985,#12237);
#5171=LINE('',#194987,#12238);
#5172=LINE('',#194989,#12239);
#5173=LINE('',#194990,#12240);
#5174=LINE('',#194994,#12241);
#5175=LINE('',#194995,#12242);
#5176=LINE('',#194996,#12243);
#5177=LINE('',#195000,#12244);
#5178=LINE('',#195001,#12245);
#5179=LINE('',#195002,#12246);
#5180=LINE('',#195004,#12247);
#5181=LINE('',#195005,#12248);
#5182=LINE('',#195009,#12249);
#5183=LINE('',#195011,#12250);
#5184=LINE('',#195013,#12251);
#5185=LINE('',#195014,#12252);
#5186=LINE('',#195018,#12253);
#5187=LINE('',#195019,#12254);
#5188=LINE('',#195020,#12255);
#5189=LINE('',#195024,#12256);
#5190=LINE('',#195025,#12257);
#5191=LINE('',#195026,#12258);
#5192=LINE('',#195028,#12259);
#5193=LINE('',#195029,#12260);
#5194=LINE('',#195033,#12261);
#5195=LINE('',#195035,#12262);
#5196=LINE('',#195037,#12263);
#5197=LINE('',#195038,#12264);
#5198=LINE('',#195042,#12265);
#5199=LINE('',#195043,#12266);
#5200=LINE('',#195044,#12267);
#5201=LINE('',#195048,#12268);
#5202=LINE('',#195049,#12269);
#5203=LINE('',#195050,#12270);
#5204=LINE('',#195052,#12271);
#5205=LINE('',#195053,#12272);
#5206=LINE('',#195057,#12273);
#5207=LINE('',#195059,#12274);
#5208=LINE('',#195061,#12275);
#5209=LINE('',#195062,#12276);
#5210=LINE('',#195066,#12277);
#5211=LINE('',#195067,#12278);
#5212=LINE('',#195068,#12279);
#5213=LINE('',#195072,#12280);
#5214=LINE('',#195073,#12281);
#5215=LINE('',#195074,#12282);
#5216=LINE('',#195076,#12283);
#5217=LINE('',#195077,#12284);
#5218=LINE('',#195081,#12285);
#5219=LINE('',#195083,#12286);
#5220=LINE('',#195085,#12287);
#5221=LINE('',#195086,#12288);
#5222=LINE('',#195090,#12289);
#5223=LINE('',#195091,#12290);
#5224=LINE('',#195092,#12291);
#5225=LINE('',#195096,#12292);
#5226=LINE('',#195097,#12293);
#5227=LINE('',#195098,#12294);
#5228=LINE('',#195100,#12295);
#5229=LINE('',#195101,#12296);
#5230=LINE('',#195105,#12297);
#5231=LINE('',#195107,#12298);
#5232=LINE('',#195109,#12299);
#5233=LINE('',#195110,#12300);
#5234=LINE('',#195114,#12301);
#5235=LINE('',#195115,#12302);
#5236=LINE('',#195116,#12303);
#5237=LINE('',#195120,#12304);
#5238=LINE('',#195121,#12305);
#5239=LINE('',#195122,#12306);
#5240=LINE('',#195124,#12307);
#5241=LINE('',#195125,#12308);
#5242=LINE('',#195129,#12309);
#5243=LINE('',#195131,#12310);
#5244=LINE('',#195133,#12311);
#5245=LINE('',#195134,#12312);
#5246=LINE('',#195138,#12313);
#5247=LINE('',#195139,#12314);
#5248=LINE('',#195140,#12315);
#5249=LINE('',#195144,#12316);
#5250=LINE('',#195145,#12317);
#5251=LINE('',#195146,#12318);
#5252=LINE('',#195148,#12319);
#5253=LINE('',#195149,#12320);
#5254=LINE('',#195153,#12321);
#5255=LINE('',#195155,#12322);
#5256=LINE('',#195157,#12323);
#5257=LINE('',#195158,#12324);
#5258=LINE('',#195162,#12325);
#5259=LINE('',#195163,#12326);
#5260=LINE('',#195164,#12327);
#5261=LINE('',#195168,#12328);
#5262=LINE('',#195169,#12329);
#5263=LINE('',#195170,#12330);
#5264=LINE('',#195172,#12331);
#5265=LINE('',#195173,#12332);
#5266=LINE('',#195177,#12333);
#5267=LINE('',#195179,#12334);
#5268=LINE('',#195181,#12335);
#5269=LINE('',#195182,#12336);
#5270=LINE('',#195186,#12337);
#5271=LINE('',#195187,#12338);
#5272=LINE('',#195188,#12339);
#5273=LINE('',#195192,#12340);
#5274=LINE('',#195193,#12341);
#5275=LINE('',#195194,#12342);
#5276=LINE('',#195196,#12343);
#5277=LINE('',#195197,#12344);
#5278=LINE('',#195201,#12345);
#5279=LINE('',#195203,#12346);
#5280=LINE('',#195205,#12347);
#5281=LINE('',#195206,#12348);
#5282=LINE('',#195210,#12349);
#5283=LINE('',#195211,#12350);
#5284=LINE('',#195212,#12351);
#5285=LINE('',#195216,#12352);
#5286=LINE('',#195217,#12353);
#5287=LINE('',#195218,#12354);
#5288=LINE('',#195220,#12355);
#5289=LINE('',#195221,#12356);
#5290=LINE('',#195225,#12357);
#5291=LINE('',#195227,#12358);
#5292=LINE('',#195229,#12359);
#5293=LINE('',#195230,#12360);
#5294=LINE('',#195234,#12361);
#5295=LINE('',#195235,#12362);
#5296=LINE('',#195236,#12363);
#5297=LINE('',#195240,#12364);
#5298=LINE('',#195241,#12365);
#5299=LINE('',#195242,#12366);
#5300=LINE('',#195244,#12367);
#5301=LINE('',#195245,#12368);
#5302=LINE('',#195249,#12369);
#5303=LINE('',#195251,#12370);
#5304=LINE('',#195253,#12371);
#5305=LINE('',#195254,#12372);
#5306=LINE('',#195258,#12373);
#5307=LINE('',#195259,#12374);
#5308=LINE('',#195260,#12375);
#5309=LINE('',#195264,#12376);
#5310=LINE('',#195265,#12377);
#5311=LINE('',#195266,#12378);
#5312=LINE('',#195268,#12379);
#5313=LINE('',#195269,#12380);
#5314=LINE('',#195273,#12381);
#5315=LINE('',#195275,#12382);
#5316=LINE('',#195277,#12383);
#5317=LINE('',#195278,#12384);
#5318=LINE('',#195282,#12385);
#5319=LINE('',#195283,#12386);
#5320=LINE('',#195284,#12387);
#5321=LINE('',#195288,#12388);
#5322=LINE('',#195289,#12389);
#5323=LINE('',#195290,#12390);
#5324=LINE('',#195292,#12391);
#5325=LINE('',#195293,#12392);
#5326=LINE('',#195297,#12393);
#5327=LINE('',#195299,#12394);
#5328=LINE('',#195301,#12395);
#5329=LINE('',#195302,#12396);
#5330=LINE('',#195306,#12397);
#5331=LINE('',#195307,#12398);
#5332=LINE('',#195308,#12399);
#5333=LINE('',#195312,#12400);
#5334=LINE('',#195313,#12401);
#5335=LINE('',#195314,#12402);
#5336=LINE('',#195316,#12403);
#5337=LINE('',#195317,#12404);
#5338=LINE('',#195321,#12405);
#5339=LINE('',#195323,#12406);
#5340=LINE('',#195325,#12407);
#5341=LINE('',#195326,#12408);
#5342=LINE('',#195330,#12409);
#5343=LINE('',#195331,#12410);
#5344=LINE('',#195332,#12411);
#5345=LINE('',#195336,#12412);
#5346=LINE('',#195337,#12413);
#5347=LINE('',#195338,#12414);
#5348=LINE('',#195340,#12415);
#5349=LINE('',#195341,#12416);
#5350=LINE('',#195345,#12417);
#5351=LINE('',#195347,#12418);
#5352=LINE('',#195349,#12419);
#5353=LINE('',#195350,#12420);
#5354=LINE('',#195354,#12421);
#5355=LINE('',#195355,#12422);
#5356=LINE('',#195356,#12423);
#5357=LINE('',#195360,#12424);
#5358=LINE('',#195361,#12425);
#5359=LINE('',#195362,#12426);
#5360=LINE('',#195364,#12427);
#5361=LINE('',#195365,#12428);
#5362=LINE('',#195369,#12429);
#5363=LINE('',#195371,#12430);
#5364=LINE('',#195373,#12431);
#5365=LINE('',#195374,#12432);
#5366=LINE('',#195378,#12433);
#5367=LINE('',#195379,#12434);
#5368=LINE('',#195380,#12435);
#5369=LINE('',#195384,#12436);
#5370=LINE('',#195385,#12437);
#5371=LINE('',#195386,#12438);
#5372=LINE('',#195388,#12439);
#5373=LINE('',#195389,#12440);
#5374=LINE('',#195393,#12441);
#5375=LINE('',#195395,#12442);
#5376=LINE('',#195397,#12443);
#5377=LINE('',#195398,#12444);
#5378=LINE('',#195402,#12445);
#5379=LINE('',#195403,#12446);
#5380=LINE('',#195404,#12447);
#5381=LINE('',#195408,#12448);
#5382=LINE('',#195409,#12449);
#5383=LINE('',#195410,#12450);
#5384=LINE('',#195412,#12451);
#5385=LINE('',#195413,#12452);
#5386=LINE('',#195417,#12453);
#5387=LINE('',#195419,#12454);
#5388=LINE('',#195421,#12455);
#5389=LINE('',#195422,#12456);
#5390=LINE('',#195426,#12457);
#5391=LINE('',#195427,#12458);
#5392=LINE('',#195428,#12459);
#5393=LINE('',#195432,#12460);
#5394=LINE('',#195433,#12461);
#5395=LINE('',#195434,#12462);
#5396=LINE('',#195436,#12463);
#5397=LINE('',#195437,#12464);
#5398=LINE('',#195441,#12465);
#5399=LINE('',#195443,#12466);
#5400=LINE('',#195445,#12467);
#5401=LINE('',#195446,#12468);
#5402=LINE('',#195450,#12469);
#5403=LINE('',#195451,#12470);
#5404=LINE('',#195452,#12471);
#5405=LINE('',#195456,#12472);
#5406=LINE('',#195457,#12473);
#5407=LINE('',#195458,#12474);
#5408=LINE('',#195460,#12475);
#5409=LINE('',#195461,#12476);
#5410=LINE('',#195465,#12477);
#5411=LINE('',#195467,#12478);
#5412=LINE('',#195469,#12479);
#5413=LINE('',#195470,#12480);
#5414=LINE('',#195474,#12481);
#5415=LINE('',#195475,#12482);
#5416=LINE('',#195476,#12483);
#5417=LINE('',#195480,#12484);
#5418=LINE('',#195481,#12485);
#5419=LINE('',#195482,#12486);
#5420=LINE('',#195484,#12487);
#5421=LINE('',#195485,#12488);
#5422=LINE('',#195489,#12489);
#5423=LINE('',#195491,#12490);
#5424=LINE('',#195493,#12491);
#5425=LINE('',#195494,#12492);
#5426=LINE('',#195498,#12493);
#5427=LINE('',#195499,#12494);
#5428=LINE('',#195500,#12495);
#5429=LINE('',#195504,#12496);
#5430=LINE('',#195505,#12497);
#5431=LINE('',#195506,#12498);
#5432=LINE('',#195508,#12499);
#5433=LINE('',#195509,#12500);
#5434=LINE('',#195513,#12501);
#5435=LINE('',#195515,#12502);
#5436=LINE('',#195517,#12503);
#5437=LINE('',#195518,#12504);
#5438=LINE('',#195522,#12505);
#5439=LINE('',#195523,#12506);
#5440=LINE('',#195524,#12507);
#5441=LINE('',#195528,#12508);
#5442=LINE('',#195529,#12509);
#5443=LINE('',#195530,#12510);
#5444=LINE('',#195532,#12511);
#5445=LINE('',#195533,#12512);
#5446=LINE('',#195537,#12513);
#5447=LINE('',#195539,#12514);
#5448=LINE('',#195541,#12515);
#5449=LINE('',#195542,#12516);
#5450=LINE('',#195546,#12517);
#5451=LINE('',#195547,#12518);
#5452=LINE('',#195548,#12519);
#5453=LINE('',#195552,#12520);
#5454=LINE('',#195553,#12521);
#5455=LINE('',#195554,#12522);
#5456=LINE('',#195556,#12523);
#5457=LINE('',#195557,#12524);
#5458=LINE('',#195561,#12525);
#5459=LINE('',#195563,#12526);
#5460=LINE('',#195565,#12527);
#5461=LINE('',#195566,#12528);
#5462=LINE('',#195570,#12529);
#5463=LINE('',#195571,#12530);
#5464=LINE('',#195572,#12531);
#5465=LINE('',#195576,#12532);
#5466=LINE('',#195577,#12533);
#5467=LINE('',#195578,#12534);
#5468=LINE('',#195580,#12535);
#5469=LINE('',#195581,#12536);
#5470=LINE('',#195585,#12537);
#5471=LINE('',#195587,#12538);
#5472=LINE('',#195589,#12539);
#5473=LINE('',#195590,#12540);
#5474=LINE('',#195594,#12541);
#5475=LINE('',#195595,#12542);
#5476=LINE('',#195596,#12543);
#5477=LINE('',#195600,#12544);
#5478=LINE('',#195601,#12545);
#5479=LINE('',#195602,#12546);
#5480=LINE('',#195604,#12547);
#5481=LINE('',#195605,#12548);
#5482=LINE('',#195609,#12549);
#5483=LINE('',#195611,#12550);
#5484=LINE('',#195613,#12551);
#5485=LINE('',#195614,#12552);
#5486=LINE('',#195618,#12553);
#5487=LINE('',#195619,#12554);
#5488=LINE('',#195620,#12555);
#5489=LINE('',#195624,#12556);
#5490=LINE('',#195625,#12557);
#5491=LINE('',#195626,#12558);
#5492=LINE('',#195628,#12559);
#5493=LINE('',#195629,#12560);
#5494=LINE('',#195633,#12561);
#5495=LINE('',#195635,#12562);
#5496=LINE('',#195637,#12563);
#5497=LINE('',#195638,#12564);
#5498=LINE('',#195642,#12565);
#5499=LINE('',#195643,#12566);
#5500=LINE('',#195644,#12567);
#5501=LINE('',#195648,#12568);
#5502=LINE('',#195649,#12569);
#5503=LINE('',#195650,#12570);
#5504=LINE('',#195652,#12571);
#5505=LINE('',#195653,#12572);
#5506=LINE('',#195657,#12573);
#5507=LINE('',#195659,#12574);
#5508=LINE('',#195661,#12575);
#5509=LINE('',#195662,#12576);
#5510=LINE('',#195666,#12577);
#5511=LINE('',#195667,#12578);
#5512=LINE('',#195668,#12579);
#5513=LINE('',#195672,#12580);
#5514=LINE('',#195673,#12581);
#5515=LINE('',#195674,#12582);
#5516=LINE('',#195676,#12583);
#5517=LINE('',#195677,#12584);
#5518=LINE('',#195681,#12585);
#5519=LINE('',#195683,#12586);
#5520=LINE('',#195685,#12587);
#5521=LINE('',#195686,#12588);
#5522=LINE('',#195690,#12589);
#5523=LINE('',#195691,#12590);
#5524=LINE('',#195692,#12591);
#5525=LINE('',#195696,#12592);
#5526=LINE('',#195697,#12593);
#5527=LINE('',#195698,#12594);
#5528=LINE('',#195700,#12595);
#5529=LINE('',#195701,#12596);
#5530=LINE('',#195705,#12597);
#5531=LINE('',#195707,#12598);
#5532=LINE('',#195709,#12599);
#5533=LINE('',#195710,#12600);
#5534=LINE('',#195714,#12601);
#5535=LINE('',#195715,#12602);
#5536=LINE('',#195716,#12603);
#5537=LINE('',#195720,#12604);
#5538=LINE('',#195721,#12605);
#5539=LINE('',#195722,#12606);
#5540=LINE('',#195724,#12607);
#5541=LINE('',#195725,#12608);
#5542=LINE('',#195729,#12609);
#5543=LINE('',#195731,#12610);
#5544=LINE('',#195733,#12611);
#5545=LINE('',#195734,#12612);
#5546=LINE('',#195738,#12613);
#5547=LINE('',#195739,#12614);
#5548=LINE('',#195740,#12615);
#5549=LINE('',#195744,#12616);
#5550=LINE('',#195745,#12617);
#5551=LINE('',#195746,#12618);
#5552=LINE('',#195748,#12619);
#5553=LINE('',#195749,#12620);
#5554=LINE('',#195753,#12621);
#5555=LINE('',#195755,#12622);
#5556=LINE('',#195757,#12623);
#5557=LINE('',#195758,#12624);
#5558=LINE('',#195762,#12625);
#5559=LINE('',#195763,#12626);
#5560=LINE('',#195764,#12627);
#5561=LINE('',#195768,#12628);
#5562=LINE('',#195769,#12629);
#5563=LINE('',#195770,#12630);
#5564=LINE('',#195772,#12631);
#5565=LINE('',#195773,#12632);
#5566=LINE('',#195777,#12633);
#5567=LINE('',#195779,#12634);
#5568=LINE('',#195781,#12635);
#5569=LINE('',#195782,#12636);
#5570=LINE('',#195786,#12637);
#5571=LINE('',#195787,#12638);
#5572=LINE('',#195788,#12639);
#5573=LINE('',#195792,#12640);
#5574=LINE('',#195793,#12641);
#5575=LINE('',#195794,#12642);
#5576=LINE('',#195796,#12643);
#5577=LINE('',#195797,#12644);
#5578=LINE('',#195801,#12645);
#5579=LINE('',#195803,#12646);
#5580=LINE('',#195805,#12647);
#5581=LINE('',#195806,#12648);
#5582=LINE('',#195810,#12649);
#5583=LINE('',#195811,#12650);
#5584=LINE('',#195812,#12651);
#5585=LINE('',#195816,#12652);
#5586=LINE('',#195817,#12653);
#5587=LINE('',#195818,#12654);
#5588=LINE('',#195820,#12655);
#5589=LINE('',#195821,#12656);
#5590=LINE('',#195825,#12657);
#5591=LINE('',#195827,#12658);
#5592=LINE('',#195829,#12659);
#5593=LINE('',#195830,#12660);
#5594=LINE('',#195834,#12661);
#5595=LINE('',#195835,#12662);
#5596=LINE('',#195836,#12663);
#5597=LINE('',#195840,#12664);
#5598=LINE('',#195841,#12665);
#5599=LINE('',#195842,#12666);
#5600=LINE('',#195844,#12667);
#5601=LINE('',#195845,#12668);
#5602=LINE('',#195849,#12669);
#5603=LINE('',#195851,#12670);
#5604=LINE('',#195853,#12671);
#5605=LINE('',#195854,#12672);
#5606=LINE('',#195858,#12673);
#5607=LINE('',#195859,#12674);
#5608=LINE('',#195860,#12675);
#5609=LINE('',#195864,#12676);
#5610=LINE('',#195865,#12677);
#5611=LINE('',#195866,#12678);
#5612=LINE('',#195868,#12679);
#5613=LINE('',#195869,#12680);
#5614=LINE('',#195873,#12681);
#5615=LINE('',#195875,#12682);
#5616=LINE('',#195877,#12683);
#5617=LINE('',#195878,#12684);
#5618=LINE('',#195882,#12685);
#5619=LINE('',#195883,#12686);
#5620=LINE('',#195884,#12687);
#5621=LINE('',#195888,#12688);
#5622=LINE('',#195889,#12689);
#5623=LINE('',#195890,#12690);
#5624=LINE('',#195892,#12691);
#5625=LINE('',#195893,#12692);
#5626=LINE('',#195897,#12693);
#5627=LINE('',#195899,#12694);
#5628=LINE('',#195901,#12695);
#5629=LINE('',#195902,#12696);
#5630=LINE('',#195906,#12697);
#5631=LINE('',#195907,#12698);
#5632=LINE('',#195908,#12699);
#5633=LINE('',#195912,#12700);
#5634=LINE('',#195913,#12701);
#5635=LINE('',#195914,#12702);
#5636=LINE('',#195916,#12703);
#5637=LINE('',#195917,#12704);
#5638=LINE('',#195921,#12705);
#5639=LINE('',#195923,#12706);
#5640=LINE('',#195925,#12707);
#5641=LINE('',#195926,#12708);
#5642=LINE('',#195930,#12709);
#5643=LINE('',#195931,#12710);
#5644=LINE('',#195932,#12711);
#5645=LINE('',#195936,#12712);
#5646=LINE('',#195937,#12713);
#5647=LINE('',#195938,#12714);
#5648=LINE('',#195940,#12715);
#5649=LINE('',#195941,#12716);
#5650=LINE('',#195945,#12717);
#5651=LINE('',#195947,#12718);
#5652=LINE('',#195949,#12719);
#5653=LINE('',#195950,#12720);
#5654=LINE('',#195954,#12721);
#5655=LINE('',#195955,#12722);
#5656=LINE('',#195956,#12723);
#5657=LINE('',#195960,#12724);
#5658=LINE('',#195961,#12725);
#5659=LINE('',#195962,#12726);
#5660=LINE('',#195964,#12727);
#5661=LINE('',#195965,#12728);
#5662=LINE('',#195969,#12729);
#5663=LINE('',#195971,#12730);
#5664=LINE('',#195973,#12731);
#5665=LINE('',#195974,#12732);
#5666=LINE('',#195978,#12733);
#5667=LINE('',#195979,#12734);
#5668=LINE('',#195980,#12735);
#5669=LINE('',#195984,#12736);
#5670=LINE('',#195985,#12737);
#5671=LINE('',#195986,#12738);
#5672=LINE('',#195988,#12739);
#5673=LINE('',#195989,#12740);
#5674=LINE('',#195993,#12741);
#5675=LINE('',#195995,#12742);
#5676=LINE('',#195997,#12743);
#5677=LINE('',#195998,#12744);
#5678=LINE('',#196002,#12745);
#5679=LINE('',#196003,#12746);
#5680=LINE('',#196004,#12747);
#5681=LINE('',#196008,#12748);
#5682=LINE('',#196009,#12749);
#5683=LINE('',#196010,#12750);
#5684=LINE('',#196012,#12751);
#5685=LINE('',#196013,#12752);
#5686=LINE('',#196017,#12753);
#5687=LINE('',#196019,#12754);
#5688=LINE('',#196021,#12755);
#5689=LINE('',#196022,#12756);
#5690=LINE('',#196026,#12757);
#5691=LINE('',#196027,#12758);
#5692=LINE('',#196028,#12759);
#5693=LINE('',#196032,#12760);
#5694=LINE('',#196033,#12761);
#5695=LINE('',#196034,#12762);
#5696=LINE('',#196036,#12763);
#5697=LINE('',#196037,#12764);
#5698=LINE('',#196041,#12765);
#5699=LINE('',#196043,#12766);
#5700=LINE('',#196045,#12767);
#5701=LINE('',#196046,#12768);
#5702=LINE('',#196050,#12769);
#5703=LINE('',#196051,#12770);
#5704=LINE('',#196052,#12771);
#5705=LINE('',#196056,#12772);
#5706=LINE('',#196057,#12773);
#5707=LINE('',#196058,#12774);
#5708=LINE('',#196060,#12775);
#5709=LINE('',#196061,#12776);
#5710=LINE('',#196065,#12777);
#5711=LINE('',#196067,#12778);
#5712=LINE('',#196069,#12779);
#5713=LINE('',#196070,#12780);
#5714=LINE('',#196074,#12781);
#5715=LINE('',#196075,#12782);
#5716=LINE('',#196076,#12783);
#5717=LINE('',#196080,#12784);
#5718=LINE('',#196081,#12785);
#5719=LINE('',#196082,#12786);
#5720=LINE('',#196084,#12787);
#5721=LINE('',#196085,#12788);
#5722=LINE('',#196089,#12789);
#5723=LINE('',#196091,#12790);
#5724=LINE('',#196093,#12791);
#5725=LINE('',#196094,#12792);
#5726=LINE('',#196098,#12793);
#5727=LINE('',#196099,#12794);
#5728=LINE('',#196100,#12795);
#5729=LINE('',#196104,#12796);
#5730=LINE('',#196105,#12797);
#5731=LINE('',#196106,#12798);
#5732=LINE('',#196108,#12799);
#5733=LINE('',#196109,#12800);
#5734=LINE('',#196113,#12801);
#5735=LINE('',#196115,#12802);
#5736=LINE('',#196117,#12803);
#5737=LINE('',#196118,#12804);
#5738=LINE('',#196122,#12805);
#5739=LINE('',#196123,#12806);
#5740=LINE('',#196124,#12807);
#5741=LINE('',#196128,#12808);
#5742=LINE('',#196129,#12809);
#5743=LINE('',#196130,#12810);
#5744=LINE('',#196132,#12811);
#5745=LINE('',#196133,#12812);
#5746=LINE('',#196137,#12813);
#5747=LINE('',#196139,#12814);
#5748=LINE('',#196141,#12815);
#5749=LINE('',#196142,#12816);
#5750=LINE('',#196146,#12817);
#5751=LINE('',#196147,#12818);
#5752=LINE('',#196148,#12819);
#5753=LINE('',#196152,#12820);
#5754=LINE('',#196153,#12821);
#5755=LINE('',#196154,#12822);
#5756=LINE('',#196156,#12823);
#5757=LINE('',#196157,#12824);
#5758=LINE('',#196161,#12825);
#5759=LINE('',#196163,#12826);
#5760=LINE('',#196165,#12827);
#5761=LINE('',#196166,#12828);
#5762=LINE('',#196170,#12829);
#5763=LINE('',#196171,#12830);
#5764=LINE('',#196172,#12831);
#5765=LINE('',#196176,#12832);
#5766=LINE('',#196177,#12833);
#5767=LINE('',#196178,#12834);
#5768=LINE('',#196180,#12835);
#5769=LINE('',#196181,#12836);
#5770=LINE('',#196185,#12837);
#5771=LINE('',#196187,#12838);
#5772=LINE('',#196189,#12839);
#5773=LINE('',#196190,#12840);
#5774=LINE('',#196194,#12841);
#5775=LINE('',#196195,#12842);
#5776=LINE('',#196196,#12843);
#5777=LINE('',#196200,#12844);
#5778=LINE('',#196201,#12845);
#5779=LINE('',#196202,#12846);
#5780=LINE('',#196204,#12847);
#5781=LINE('',#196205,#12848);
#5782=LINE('',#196209,#12849);
#5783=LINE('',#196211,#12850);
#5784=LINE('',#196213,#12851);
#5785=LINE('',#196214,#12852);
#5786=LINE('',#196218,#12853);
#5787=LINE('',#196219,#12854);
#5788=LINE('',#196220,#12855);
#5789=LINE('',#196224,#12856);
#5790=LINE('',#196225,#12857);
#5791=LINE('',#196226,#12858);
#5792=LINE('',#196228,#12859);
#5793=LINE('',#196229,#12860);
#5794=LINE('',#196233,#12861);
#5795=LINE('',#196235,#12862);
#5796=LINE('',#196237,#12863);
#5797=LINE('',#196238,#12864);
#5798=LINE('',#196242,#12865);
#5799=LINE('',#196243,#12866);
#5800=LINE('',#196244,#12867);
#5801=LINE('',#196248,#12868);
#5802=LINE('',#196249,#12869);
#5803=LINE('',#196250,#12870);
#5804=LINE('',#196252,#12871);
#5805=LINE('',#196253,#12872);
#5806=LINE('',#196257,#12873);
#5807=LINE('',#196259,#12874);
#5808=LINE('',#196261,#12875);
#5809=LINE('',#196262,#12876);
#5810=LINE('',#196266,#12877);
#5811=LINE('',#196267,#12878);
#5812=LINE('',#196268,#12879);
#5813=LINE('',#196272,#12880);
#5814=LINE('',#196273,#12881);
#5815=LINE('',#196274,#12882);
#5816=LINE('',#196276,#12883);
#5817=LINE('',#196277,#12884);
#5818=LINE('',#196281,#12885);
#5819=LINE('',#196283,#12886);
#5820=LINE('',#196285,#12887);
#5821=LINE('',#196286,#12888);
#5822=LINE('',#196290,#12889);
#5823=LINE('',#196291,#12890);
#5824=LINE('',#196292,#12891);
#5825=LINE('',#196296,#12892);
#5826=LINE('',#196297,#12893);
#5827=LINE('',#196298,#12894);
#5828=LINE('',#196300,#12895);
#5829=LINE('',#196301,#12896);
#5830=LINE('',#196305,#12897);
#5831=LINE('',#196307,#12898);
#5832=LINE('',#196309,#12899);
#5833=LINE('',#196310,#12900);
#5834=LINE('',#196314,#12901);
#5835=LINE('',#196315,#12902);
#5836=LINE('',#196316,#12903);
#5837=LINE('',#196320,#12904);
#5838=LINE('',#196321,#12905);
#5839=LINE('',#196322,#12906);
#5840=LINE('',#196324,#12907);
#5841=LINE('',#196325,#12908);
#5842=LINE('',#196329,#12909);
#5843=LINE('',#196331,#12910);
#5844=LINE('',#196333,#12911);
#5845=LINE('',#196334,#12912);
#5846=LINE('',#196338,#12913);
#5847=LINE('',#196339,#12914);
#5848=LINE('',#196340,#12915);
#5849=LINE('',#196344,#12916);
#5850=LINE('',#196345,#12917);
#5851=LINE('',#196346,#12918);
#5852=LINE('',#196348,#12919);
#5853=LINE('',#196349,#12920);
#5854=LINE('',#196353,#12921);
#5855=LINE('',#196355,#12922);
#5856=LINE('',#196357,#12923);
#5857=LINE('',#196358,#12924);
#5858=LINE('',#196362,#12925);
#5859=LINE('',#196363,#12926);
#5860=LINE('',#196364,#12927);
#5861=LINE('',#196368,#12928);
#5862=LINE('',#196369,#12929);
#5863=LINE('',#196370,#12930);
#5864=LINE('',#196372,#12931);
#5865=LINE('',#196373,#12932);
#5866=LINE('',#196377,#12933);
#5867=LINE('',#196379,#12934);
#5868=LINE('',#196381,#12935);
#5869=LINE('',#196382,#12936);
#5870=LINE('',#196386,#12937);
#5871=LINE('',#196387,#12938);
#5872=LINE('',#196388,#12939);
#5873=LINE('',#196392,#12940);
#5874=LINE('',#196393,#12941);
#5875=LINE('',#196394,#12942);
#5876=LINE('',#196396,#12943);
#5877=LINE('',#196397,#12944);
#5878=LINE('',#196401,#12945);
#5879=LINE('',#196403,#12946);
#5880=LINE('',#196405,#12947);
#5881=LINE('',#196406,#12948);
#5882=LINE('',#196410,#12949);
#5883=LINE('',#196411,#12950);
#5884=LINE('',#196412,#12951);
#5885=LINE('',#196416,#12952);
#5886=LINE('',#196417,#12953);
#5887=LINE('',#196418,#12954);
#5888=LINE('',#196420,#12955);
#5889=LINE('',#196421,#12956);
#5890=LINE('',#196425,#12957);
#5891=LINE('',#196427,#12958);
#5892=LINE('',#196429,#12959);
#5893=LINE('',#196430,#12960);
#5894=LINE('',#196434,#12961);
#5895=LINE('',#196435,#12962);
#5896=LINE('',#196436,#12963);
#5897=LINE('',#196440,#12964);
#5898=LINE('',#196441,#12965);
#5899=LINE('',#196442,#12966);
#5900=LINE('',#196444,#12967);
#5901=LINE('',#196445,#12968);
#5902=LINE('',#196449,#12969);
#5903=LINE('',#196451,#12970);
#5904=LINE('',#196453,#12971);
#5905=LINE('',#196454,#12972);
#5906=LINE('',#196458,#12973);
#5907=LINE('',#196459,#12974);
#5908=LINE('',#196460,#12975);
#5909=LINE('',#196464,#12976);
#5910=LINE('',#196465,#12977);
#5911=LINE('',#196466,#12978);
#5912=LINE('',#196468,#12979);
#5913=LINE('',#196469,#12980);
#5914=LINE('',#196473,#12981);
#5915=LINE('',#196475,#12982);
#5916=LINE('',#196477,#12983);
#5917=LINE('',#196478,#12984);
#5918=LINE('',#196482,#12985);
#5919=LINE('',#196483,#12986);
#5920=LINE('',#196484,#12987);
#5921=LINE('',#196488,#12988);
#5922=LINE('',#196489,#12989);
#5923=LINE('',#196490,#12990);
#5924=LINE('',#196492,#12991);
#5925=LINE('',#196493,#12992);
#5926=LINE('',#196497,#12993);
#5927=LINE('',#196499,#12994);
#5928=LINE('',#196501,#12995);
#5929=LINE('',#196502,#12996);
#5930=LINE('',#196506,#12997);
#5931=LINE('',#196507,#12998);
#5932=LINE('',#196508,#12999);
#5933=LINE('',#196512,#13000);
#5934=LINE('',#196513,#13001);
#5935=LINE('',#196514,#13002);
#5936=LINE('',#196516,#13003);
#5937=LINE('',#196517,#13004);
#5938=LINE('',#196521,#13005);
#5939=LINE('',#196523,#13006);
#5940=LINE('',#196525,#13007);
#5941=LINE('',#196526,#13008);
#5942=LINE('',#196530,#13009);
#5943=LINE('',#196531,#13010);
#5944=LINE('',#196532,#13011);
#5945=LINE('',#196536,#13012);
#5946=LINE('',#196537,#13013);
#5947=LINE('',#196538,#13014);
#5948=LINE('',#196540,#13015);
#5949=LINE('',#196541,#13016);
#5950=LINE('',#196545,#13017);
#5951=LINE('',#196547,#13018);
#5952=LINE('',#196549,#13019);
#5953=LINE('',#196550,#13020);
#5954=LINE('',#196554,#13021);
#5955=LINE('',#196555,#13022);
#5956=LINE('',#196556,#13023);
#5957=LINE('',#196560,#13024);
#5958=LINE('',#196561,#13025);
#5959=LINE('',#196562,#13026);
#5960=LINE('',#196564,#13027);
#5961=LINE('',#196565,#13028);
#5962=LINE('',#196569,#13029);
#5963=LINE('',#196571,#13030);
#5964=LINE('',#196573,#13031);
#5965=LINE('',#196574,#13032);
#5966=LINE('',#196578,#13033);
#5967=LINE('',#196579,#13034);
#5968=LINE('',#196580,#13035);
#5969=LINE('',#196584,#13036);
#5970=LINE('',#196585,#13037);
#5971=LINE('',#196586,#13038);
#5972=LINE('',#196588,#13039);
#5973=LINE('',#196589,#13040);
#5974=LINE('',#196593,#13041);
#5975=LINE('',#196595,#13042);
#5976=LINE('',#196597,#13043);
#5977=LINE('',#196598,#13044);
#5978=LINE('',#196602,#13045);
#5979=LINE('',#196603,#13046);
#5980=LINE('',#196604,#13047);
#5981=LINE('',#196608,#13048);
#5982=LINE('',#196609,#13049);
#5983=LINE('',#196610,#13050);
#5984=LINE('',#196612,#13051);
#5985=LINE('',#196613,#13052);
#5986=LINE('',#196617,#13053);
#5987=LINE('',#196619,#13054);
#5988=LINE('',#196621,#13055);
#5989=LINE('',#196622,#13056);
#5990=LINE('',#196626,#13057);
#5991=LINE('',#196627,#13058);
#5992=LINE('',#196628,#13059);
#5993=LINE('',#196632,#13060);
#5994=LINE('',#196633,#13061);
#5995=LINE('',#196634,#13062);
#5996=LINE('',#196636,#13063);
#5997=LINE('',#196637,#13064);
#5998=LINE('',#196641,#13065);
#5999=LINE('',#196643,#13066);
#6000=LINE('',#196645,#13067);
#6001=LINE('',#196646,#13068);
#6002=LINE('',#196650,#13069);
#6003=LINE('',#196651,#13070);
#6004=LINE('',#196652,#13071);
#6005=LINE('',#196656,#13072);
#6006=LINE('',#196657,#13073);
#6007=LINE('',#196658,#13074);
#6008=LINE('',#196660,#13075);
#6009=LINE('',#196661,#13076);
#6010=LINE('',#196665,#13077);
#6011=LINE('',#196667,#13078);
#6012=LINE('',#196669,#13079);
#6013=LINE('',#196670,#13080);
#6014=LINE('',#196674,#13081);
#6015=LINE('',#196675,#13082);
#6016=LINE('',#196676,#13083);
#6017=LINE('',#196680,#13084);
#6018=LINE('',#196681,#13085);
#6019=LINE('',#196682,#13086);
#6020=LINE('',#196684,#13087);
#6021=LINE('',#196685,#13088);
#6022=LINE('',#196689,#13089);
#6023=LINE('',#196691,#13090);
#6024=LINE('',#196693,#13091);
#6025=LINE('',#196694,#13092);
#6026=LINE('',#196698,#13093);
#6027=LINE('',#196699,#13094);
#6028=LINE('',#196700,#13095);
#6029=LINE('',#196704,#13096);
#6030=LINE('',#196705,#13097);
#6031=LINE('',#196706,#13098);
#6032=LINE('',#196708,#13099);
#6033=LINE('',#196709,#13100);
#6034=LINE('',#196713,#13101);
#6035=LINE('',#196715,#13102);
#6036=LINE('',#196717,#13103);
#6037=LINE('',#196718,#13104);
#6038=LINE('',#196722,#13105);
#6039=LINE('',#196723,#13106);
#6040=LINE('',#196724,#13107);
#6041=LINE('',#196728,#13108);
#6042=LINE('',#196729,#13109);
#6043=LINE('',#196730,#13110);
#6044=LINE('',#196732,#13111);
#6045=LINE('',#196733,#13112);
#6046=LINE('',#196737,#13113);
#6047=LINE('',#196739,#13114);
#6048=LINE('',#196741,#13115);
#6049=LINE('',#196742,#13116);
#6050=LINE('',#196746,#13117);
#6051=LINE('',#196747,#13118);
#6052=LINE('',#196748,#13119);
#6053=LINE('',#196752,#13120);
#6054=LINE('',#196753,#13121);
#6055=LINE('',#196754,#13122);
#6056=LINE('',#196756,#13123);
#6057=LINE('',#196757,#13124);
#6058=LINE('',#196761,#13125);
#6059=LINE('',#196763,#13126);
#6060=LINE('',#196765,#13127);
#6061=LINE('',#196766,#13128);
#6062=LINE('',#196770,#13129);
#6063=LINE('',#196771,#13130);
#6064=LINE('',#196772,#13131);
#6065=LINE('',#196776,#13132);
#6066=LINE('',#196777,#13133);
#6067=LINE('',#196778,#13134);
#6068=LINE('',#196780,#13135);
#6069=LINE('',#196781,#13136);
#6070=LINE('',#196785,#13137);
#6071=LINE('',#196787,#13138);
#6072=LINE('',#196789,#13139);
#6073=LINE('',#196790,#13140);
#6074=LINE('',#196794,#13141);
#6075=LINE('',#196795,#13142);
#6076=LINE('',#196796,#13143);
#6077=LINE('',#196800,#13144);
#6078=LINE('',#196801,#13145);
#6079=LINE('',#196802,#13146);
#6080=LINE('',#196804,#13147);
#6081=LINE('',#196805,#13148);
#6082=LINE('',#196809,#13149);
#6083=LINE('',#196811,#13150);
#6084=LINE('',#196813,#13151);
#6085=LINE('',#196814,#13152);
#6086=LINE('',#196818,#13153);
#6087=LINE('',#196819,#13154);
#6088=LINE('',#196820,#13155);
#6089=LINE('',#196824,#13156);
#6090=LINE('',#196825,#13157);
#6091=LINE('',#196826,#13158);
#6092=LINE('',#196828,#13159);
#6093=LINE('',#196829,#13160);
#6094=LINE('',#196833,#13161);
#6095=LINE('',#196835,#13162);
#6096=LINE('',#196837,#13163);
#6097=LINE('',#196838,#13164);
#6098=LINE('',#196842,#13165);
#6099=LINE('',#196843,#13166);
#6100=LINE('',#196844,#13167);
#6101=LINE('',#196848,#13168);
#6102=LINE('',#196849,#13169);
#6103=LINE('',#196850,#13170);
#6104=LINE('',#196852,#13171);
#6105=LINE('',#196853,#13172);
#6106=LINE('',#196857,#13173);
#6107=LINE('',#196859,#13174);
#6108=LINE('',#196861,#13175);
#6109=LINE('',#196862,#13176);
#6110=LINE('',#196866,#13177);
#6111=LINE('',#196867,#13178);
#6112=LINE('',#196868,#13179);
#6113=LINE('',#196872,#13180);
#6114=LINE('',#196873,#13181);
#6115=LINE('',#196874,#13182);
#6116=LINE('',#196876,#13183);
#6117=LINE('',#196877,#13184);
#6118=LINE('',#196881,#13185);
#6119=LINE('',#196883,#13186);
#6120=LINE('',#196885,#13187);
#6121=LINE('',#196886,#13188);
#6122=LINE('',#196890,#13189);
#6123=LINE('',#196891,#13190);
#6124=LINE('',#196892,#13191);
#6125=LINE('',#196896,#13192);
#6126=LINE('',#196897,#13193);
#6127=LINE('',#196898,#13194);
#6128=LINE('',#196900,#13195);
#6129=LINE('',#196901,#13196);
#6130=LINE('',#196905,#13197);
#6131=LINE('',#196907,#13198);
#6132=LINE('',#196909,#13199);
#6133=LINE('',#196910,#13200);
#6134=LINE('',#196914,#13201);
#6135=LINE('',#196915,#13202);
#6136=LINE('',#196916,#13203);
#6137=LINE('',#196920,#13204);
#6138=LINE('',#196921,#13205);
#6139=LINE('',#196922,#13206);
#6140=LINE('',#196924,#13207);
#6141=LINE('',#196925,#13208);
#6142=LINE('',#196929,#13209);
#6143=LINE('',#196931,#13210);
#6144=LINE('',#196933,#13211);
#6145=LINE('',#196934,#13212);
#6146=LINE('',#196938,#13213);
#6147=LINE('',#196939,#13214);
#6148=LINE('',#196940,#13215);
#6149=LINE('',#196944,#13216);
#6150=LINE('',#196945,#13217);
#6151=LINE('',#196946,#13218);
#6152=LINE('',#196948,#13219);
#6153=LINE('',#196949,#13220);
#6154=LINE('',#196953,#13221);
#6155=LINE('',#196955,#13222);
#6156=LINE('',#196957,#13223);
#6157=LINE('',#196958,#13224);
#6158=LINE('',#196962,#13225);
#6159=LINE('',#196963,#13226);
#6160=LINE('',#196964,#13227);
#6161=LINE('',#196968,#13228);
#6162=LINE('',#196969,#13229);
#6163=LINE('',#196970,#13230);
#6164=LINE('',#196972,#13231);
#6165=LINE('',#196973,#13232);
#6166=LINE('',#196977,#13233);
#6167=LINE('',#196979,#13234);
#6168=LINE('',#196981,#13235);
#6169=LINE('',#196982,#13236);
#6170=LINE('',#196986,#13237);
#6171=LINE('',#196987,#13238);
#6172=LINE('',#196988,#13239);
#6173=LINE('',#196992,#13240);
#6174=LINE('',#196993,#13241);
#6175=LINE('',#196994,#13242);
#6176=LINE('',#196996,#13243);
#6177=LINE('',#196997,#13244);
#6178=LINE('',#197001,#13245);
#6179=LINE('',#197003,#13246);
#6180=LINE('',#197005,#13247);
#6181=LINE('',#197006,#13248);
#6182=LINE('',#197010,#13249);
#6183=LINE('',#197011,#13250);
#6184=LINE('',#197012,#13251);
#6185=LINE('',#197016,#13252);
#6186=LINE('',#197017,#13253);
#6187=LINE('',#197018,#13254);
#6188=LINE('',#197020,#13255);
#6189=LINE('',#197021,#13256);
#6190=LINE('',#197025,#13257);
#6191=LINE('',#197027,#13258);
#6192=LINE('',#197029,#13259);
#6193=LINE('',#197030,#13260);
#6194=LINE('',#197034,#13261);
#6195=LINE('',#197035,#13262);
#6196=LINE('',#197036,#13263);
#6197=LINE('',#197040,#13264);
#6198=LINE('',#197041,#13265);
#6199=LINE('',#197042,#13266);
#6200=LINE('',#197044,#13267);
#6201=LINE('',#197045,#13268);
#6202=LINE('',#197049,#13269);
#6203=LINE('',#197051,#13270);
#6204=LINE('',#197053,#13271);
#6205=LINE('',#197054,#13272);
#6206=LINE('',#197058,#13273);
#6207=LINE('',#197059,#13274);
#6208=LINE('',#197060,#13275);
#6209=LINE('',#197064,#13276);
#6210=LINE('',#197065,#13277);
#6211=LINE('',#197066,#13278);
#6212=LINE('',#197068,#13279);
#6213=LINE('',#197069,#13280);
#6214=LINE('',#197073,#13281);
#6215=LINE('',#197075,#13282);
#6216=LINE('',#197077,#13283);
#6217=LINE('',#197078,#13284);
#6218=LINE('',#197082,#13285);
#6219=LINE('',#197083,#13286);
#6220=LINE('',#197084,#13287);
#6221=LINE('',#197088,#13288);
#6222=LINE('',#197089,#13289);
#6223=LINE('',#197090,#13290);
#6224=LINE('',#197092,#13291);
#6225=LINE('',#197093,#13292);
#6226=LINE('',#197097,#13293);
#6227=LINE('',#197099,#13294);
#6228=LINE('',#197101,#13295);
#6229=LINE('',#197102,#13296);
#6230=LINE('',#197106,#13297);
#6231=LINE('',#197107,#13298);
#6232=LINE('',#197108,#13299);
#6233=LINE('',#197112,#13300);
#6234=LINE('',#197113,#13301);
#6235=LINE('',#197114,#13302);
#6236=LINE('',#197116,#13303);
#6237=LINE('',#197117,#13304);
#6238=LINE('',#197121,#13305);
#6239=LINE('',#197123,#13306);
#6240=LINE('',#197125,#13307);
#6241=LINE('',#197126,#13308);
#6242=LINE('',#197130,#13309);
#6243=LINE('',#197131,#13310);
#6244=LINE('',#197132,#13311);
#6245=LINE('',#197136,#13312);
#6246=LINE('',#197137,#13313);
#6247=LINE('',#197138,#13314);
#6248=LINE('',#197140,#13315);
#6249=LINE('',#197141,#13316);
#6250=LINE('',#197145,#13317);
#6251=LINE('',#197147,#13318);
#6252=LINE('',#197149,#13319);
#6253=LINE('',#197150,#13320);
#6254=LINE('',#197154,#13321);
#6255=LINE('',#197155,#13322);
#6256=LINE('',#197156,#13323);
#6257=LINE('',#197160,#13324);
#6258=LINE('',#197161,#13325);
#6259=LINE('',#197162,#13326);
#6260=LINE('',#197164,#13327);
#6261=LINE('',#197165,#13328);
#6262=LINE('',#197169,#13329);
#6263=LINE('',#197171,#13330);
#6264=LINE('',#197173,#13331);
#6265=LINE('',#197174,#13332);
#6266=LINE('',#197178,#13333);
#6267=LINE('',#197179,#13334);
#6268=LINE('',#197180,#13335);
#6269=LINE('',#197184,#13336);
#6270=LINE('',#197185,#13337);
#6271=LINE('',#197186,#13338);
#6272=LINE('',#197188,#13339);
#6273=LINE('',#197189,#13340);
#6274=LINE('',#197193,#13341);
#6275=LINE('',#197195,#13342);
#6276=LINE('',#197197,#13343);
#6277=LINE('',#197198,#13344);
#6278=LINE('',#197202,#13345);
#6279=LINE('',#197203,#13346);
#6280=LINE('',#197204,#13347);
#6281=LINE('',#197208,#13348);
#6282=LINE('',#197209,#13349);
#6283=LINE('',#197210,#13350);
#6284=LINE('',#197212,#13351);
#6285=LINE('',#197213,#13352);
#6286=LINE('',#197217,#13353);
#6287=LINE('',#197219,#13354);
#6288=LINE('',#197221,#13355);
#6289=LINE('',#197222,#13356);
#6290=LINE('',#197226,#13357);
#6291=LINE('',#197227,#13358);
#6292=LINE('',#197228,#13359);
#6293=LINE('',#197232,#13360);
#6294=LINE('',#197233,#13361);
#6295=LINE('',#197234,#13362);
#6296=LINE('',#197236,#13363);
#6297=LINE('',#197237,#13364);
#6298=LINE('',#197241,#13365);
#6299=LINE('',#197243,#13366);
#6300=LINE('',#197245,#13367);
#6301=LINE('',#197246,#13368);
#6302=LINE('',#197250,#13369);
#6303=LINE('',#197251,#13370);
#6304=LINE('',#197252,#13371);
#6305=LINE('',#197256,#13372);
#6306=LINE('',#197257,#13373);
#6307=LINE('',#197258,#13374);
#6308=LINE('',#197260,#13375);
#6309=LINE('',#197261,#13376);
#6310=LINE('',#197265,#13377);
#6311=LINE('',#197267,#13378);
#6312=LINE('',#197269,#13379);
#6313=LINE('',#197270,#13380);
#6314=LINE('',#197274,#13381);
#6315=LINE('',#197275,#13382);
#6316=LINE('',#197276,#13383);
#6317=LINE('',#197280,#13384);
#6318=LINE('',#197281,#13385);
#6319=LINE('',#197282,#13386);
#6320=LINE('',#197284,#13387);
#6321=LINE('',#197285,#13388);
#6322=LINE('',#197289,#13389);
#6323=LINE('',#197291,#13390);
#6324=LINE('',#197293,#13391);
#6325=LINE('',#197294,#13392);
#6326=LINE('',#197298,#13393);
#6327=LINE('',#197299,#13394);
#6328=LINE('',#197300,#13395);
#6329=LINE('',#197304,#13396);
#6330=LINE('',#197305,#13397);
#6331=LINE('',#197306,#13398);
#6332=LINE('',#197308,#13399);
#6333=LINE('',#197309,#13400);
#6334=LINE('',#197313,#13401);
#6335=LINE('',#197315,#13402);
#6336=LINE('',#197317,#13403);
#6337=LINE('',#197318,#13404);
#6338=LINE('',#197322,#13405);
#6339=LINE('',#197323,#13406);
#6340=LINE('',#197324,#13407);
#6341=LINE('',#197328,#13408);
#6342=LINE('',#197329,#13409);
#6343=LINE('',#197330,#13410);
#6344=LINE('',#197332,#13411);
#6345=LINE('',#197333,#13412);
#6346=LINE('',#197337,#13413);
#6347=LINE('',#197339,#13414);
#6348=LINE('',#197341,#13415);
#6349=LINE('',#197342,#13416);
#6350=LINE('',#197346,#13417);
#6351=LINE('',#197347,#13418);
#6352=LINE('',#197348,#13419);
#6353=LINE('',#197352,#13420);
#6354=LINE('',#197353,#13421);
#6355=LINE('',#197354,#13422);
#6356=LINE('',#197356,#13423);
#6357=LINE('',#197357,#13424);
#6358=LINE('',#197361,#13425);
#6359=LINE('',#197363,#13426);
#6360=LINE('',#197365,#13427);
#6361=LINE('',#197366,#13428);
#6362=LINE('',#197370,#13429);
#6363=LINE('',#197371,#13430);
#6364=LINE('',#197372,#13431);
#6365=LINE('',#197376,#13432);
#6366=LINE('',#197377,#13433);
#6367=LINE('',#197378,#13434);
#6368=LINE('',#197380,#13435);
#6369=LINE('',#197381,#13436);
#6370=LINE('',#197385,#13437);
#6371=LINE('',#197387,#13438);
#6372=LINE('',#197389,#13439);
#6373=LINE('',#197390,#13440);
#6374=LINE('',#197394,#13441);
#6375=LINE('',#197395,#13442);
#6376=LINE('',#197396,#13443);
#6377=LINE('',#197400,#13444);
#6378=LINE('',#197401,#13445);
#6379=LINE('',#197402,#13446);
#6380=LINE('',#197404,#13447);
#6381=LINE('',#197405,#13448);
#6382=LINE('',#197409,#13449);
#6383=LINE('',#197411,#13450);
#6384=LINE('',#197413,#13451);
#6385=LINE('',#197414,#13452);
#6386=LINE('',#197418,#13453);
#6387=LINE('',#197419,#13454);
#6388=LINE('',#197420,#13455);
#6389=LINE('',#197424,#13456);
#6390=LINE('',#197425,#13457);
#6391=LINE('',#197426,#13458);
#6392=LINE('',#197428,#13459);
#6393=LINE('',#197429,#13460);
#6394=LINE('',#197433,#13461);
#6395=LINE('',#197435,#13462);
#6396=LINE('',#197437,#13463);
#6397=LINE('',#197438,#13464);
#6398=LINE('',#197442,#13465);
#6399=LINE('',#197443,#13466);
#6400=LINE('',#197444,#13467);
#6401=LINE('',#197448,#13468);
#6402=LINE('',#197449,#13469);
#6403=LINE('',#197450,#13470);
#6404=LINE('',#197452,#13471);
#6405=LINE('',#197453,#13472);
#6406=LINE('',#197457,#13473);
#6407=LINE('',#197459,#13474);
#6408=LINE('',#197461,#13475);
#6409=LINE('',#197462,#13476);
#6410=LINE('',#197466,#13477);
#6411=LINE('',#197467,#13478);
#6412=LINE('',#197468,#13479);
#6413=LINE('',#197472,#13480);
#6414=LINE('',#197473,#13481);
#6415=LINE('',#197474,#13482);
#6416=LINE('',#197476,#13483);
#6417=LINE('',#197477,#13484);
#6418=LINE('',#197481,#13485);
#6419=LINE('',#197483,#13486);
#6420=LINE('',#197485,#13487);
#6421=LINE('',#197486,#13488);
#6422=LINE('',#197490,#13489);
#6423=LINE('',#197491,#13490);
#6424=LINE('',#197492,#13491);
#6425=LINE('',#197496,#13492);
#6426=LINE('',#197497,#13493);
#6427=LINE('',#197498,#13494);
#6428=LINE('',#197500,#13495);
#6429=LINE('',#197501,#13496);
#6430=LINE('',#197505,#13497);
#6431=LINE('',#197507,#13498);
#6432=LINE('',#197509,#13499);
#6433=LINE('',#197510,#13500);
#6434=LINE('',#197514,#13501);
#6435=LINE('',#197515,#13502);
#6436=LINE('',#197516,#13503);
#6437=LINE('',#197520,#13504);
#6438=LINE('',#197521,#13505);
#6439=LINE('',#197522,#13506);
#6440=LINE('',#197524,#13507);
#6441=LINE('',#197525,#13508);
#6442=LINE('',#197529,#13509);
#6443=LINE('',#197531,#13510);
#6444=LINE('',#197533,#13511);
#6445=LINE('',#197534,#13512);
#6446=LINE('',#197538,#13513);
#6447=LINE('',#197539,#13514);
#6448=LINE('',#197540,#13515);
#6449=LINE('',#197544,#13516);
#6450=LINE('',#197545,#13517);
#6451=LINE('',#197546,#13518);
#6452=LINE('',#197548,#13519);
#6453=LINE('',#197549,#13520);
#6454=LINE('',#197553,#13521);
#6455=LINE('',#197555,#13522);
#6456=LINE('',#197557,#13523);
#6457=LINE('',#197558,#13524);
#6458=LINE('',#197562,#13525);
#6459=LINE('',#197563,#13526);
#6460=LINE('',#197564,#13527);
#6461=LINE('',#197568,#13528);
#6462=LINE('',#197569,#13529);
#6463=LINE('',#197570,#13530);
#6464=LINE('',#197572,#13531);
#6465=LINE('',#197573,#13532);
#6466=LINE('',#197577,#13533);
#6467=LINE('',#197579,#13534);
#6468=LINE('',#197581,#13535);
#6469=LINE('',#197582,#13536);
#6470=LINE('',#197586,#13537);
#6471=LINE('',#197587,#13538);
#6472=LINE('',#197588,#13539);
#6473=LINE('',#197592,#13540);
#6474=LINE('',#197593,#13541);
#6475=LINE('',#197594,#13542);
#6476=LINE('',#197596,#13543);
#6477=LINE('',#197597,#13544);
#6478=LINE('',#197601,#13545);
#6479=LINE('',#197603,#13546);
#6480=LINE('',#197605,#13547);
#6481=LINE('',#197606,#13548);
#6482=LINE('',#197610,#13549);
#6483=LINE('',#197611,#13550);
#6484=LINE('',#197612,#13551);
#6485=LINE('',#197616,#13552);
#6486=LINE('',#197617,#13553);
#6487=LINE('',#197618,#13554);
#6488=LINE('',#197620,#13555);
#6489=LINE('',#197621,#13556);
#6490=LINE('',#197625,#13557);
#6491=LINE('',#197627,#13558);
#6492=LINE('',#197629,#13559);
#6493=LINE('',#197630,#13560);
#6494=LINE('',#197634,#13561);
#6495=LINE('',#197635,#13562);
#6496=LINE('',#197636,#13563);
#6497=LINE('',#197640,#13564);
#6498=LINE('',#197641,#13565);
#6499=LINE('',#197642,#13566);
#6500=LINE('',#197644,#13567);
#6501=LINE('',#197645,#13568);
#6502=LINE('',#197649,#13569);
#6503=LINE('',#197651,#13570);
#6504=LINE('',#197653,#13571);
#6505=LINE('',#197654,#13572);
#6506=LINE('',#197658,#13573);
#6507=LINE('',#197659,#13574);
#6508=LINE('',#197660,#13575);
#6509=LINE('',#197664,#13576);
#6510=LINE('',#197665,#13577);
#6511=LINE('',#197666,#13578);
#6512=LINE('',#197668,#13579);
#6513=LINE('',#197669,#13580);
#6514=LINE('',#197673,#13581);
#6515=LINE('',#197675,#13582);
#6516=LINE('',#197677,#13583);
#6517=LINE('',#197678,#13584);
#6518=LINE('',#197682,#13585);
#6519=LINE('',#197683,#13586);
#6520=LINE('',#197684,#13587);
#6521=LINE('',#197688,#13588);
#6522=LINE('',#197689,#13589);
#6523=LINE('',#197690,#13590);
#6524=LINE('',#197692,#13591);
#6525=LINE('',#197693,#13592);
#6526=LINE('',#197697,#13593);
#6527=LINE('',#197699,#13594);
#6528=LINE('',#197701,#13595);
#6529=LINE('',#197702,#13596);
#6530=LINE('',#197706,#13597);
#6531=LINE('',#197707,#13598);
#6532=LINE('',#197708,#13599);
#6533=LINE('',#197712,#13600);
#6534=LINE('',#197713,#13601);
#6535=LINE('',#197714,#13602);
#6536=LINE('',#197716,#13603);
#6537=LINE('',#197717,#13604);
#6538=LINE('',#197721,#13605);
#6539=LINE('',#197723,#13606);
#6540=LINE('',#197725,#13607);
#6541=LINE('',#197726,#13608);
#6542=LINE('',#197730,#13609);
#6543=LINE('',#197731,#13610);
#6544=LINE('',#197732,#13611);
#6545=LINE('',#197736,#13612);
#6546=LINE('',#197737,#13613);
#6547=LINE('',#197738,#13614);
#6548=LINE('',#197740,#13615);
#6549=LINE('',#197741,#13616);
#6550=LINE('',#197745,#13617);
#6551=LINE('',#197747,#13618);
#6552=LINE('',#197749,#13619);
#6553=LINE('',#197750,#13620);
#6554=LINE('',#197754,#13621);
#6555=LINE('',#197755,#13622);
#6556=LINE('',#197756,#13623);
#6557=LINE('',#197760,#13624);
#6558=LINE('',#197761,#13625);
#6559=LINE('',#197762,#13626);
#6560=LINE('',#197764,#13627);
#6561=LINE('',#197765,#13628);
#6562=LINE('',#197769,#13629);
#6563=LINE('',#197771,#13630);
#6564=LINE('',#197773,#13631);
#6565=LINE('',#197774,#13632);
#6566=LINE('',#197778,#13633);
#6567=LINE('',#197779,#13634);
#6568=LINE('',#197780,#13635);
#6569=LINE('',#197784,#13636);
#6570=LINE('',#197785,#13637);
#6571=LINE('',#197786,#13638);
#6572=LINE('',#197788,#13639);
#6573=LINE('',#197789,#13640);
#6574=LINE('',#197793,#13641);
#6575=LINE('',#197795,#13642);
#6576=LINE('',#197797,#13643);
#6577=LINE('',#197798,#13644);
#6578=LINE('',#197802,#13645);
#6579=LINE('',#197803,#13646);
#6580=LINE('',#197804,#13647);
#6581=LINE('',#197808,#13648);
#6582=LINE('',#197809,#13649);
#6583=LINE('',#197810,#13650);
#6584=LINE('',#197812,#13651);
#6585=LINE('',#197813,#13652);
#6586=LINE('',#197817,#13653);
#6587=LINE('',#197819,#13654);
#6588=LINE('',#197821,#13655);
#6589=LINE('',#197822,#13656);
#6590=LINE('',#197826,#13657);
#6591=LINE('',#197827,#13658);
#6592=LINE('',#197828,#13659);
#6593=LINE('',#197832,#13660);
#6594=LINE('',#197833,#13661);
#6595=LINE('',#197834,#13662);
#6596=LINE('',#197836,#13663);
#6597=LINE('',#197837,#13664);
#6598=LINE('',#197841,#13665);
#6599=LINE('',#197843,#13666);
#6600=LINE('',#197845,#13667);
#6601=LINE('',#197846,#13668);
#6602=LINE('',#197850,#13669);
#6603=LINE('',#197851,#13670);
#6604=LINE('',#197852,#13671);
#6605=LINE('',#197856,#13672);
#6606=LINE('',#197857,#13673);
#6607=LINE('',#197858,#13674);
#6608=LINE('',#197860,#13675);
#6609=LINE('',#197861,#13676);
#6610=LINE('',#197865,#13677);
#6611=LINE('',#197867,#13678);
#6612=LINE('',#197869,#13679);
#6613=LINE('',#197870,#13680);
#6614=LINE('',#197874,#13681);
#6615=LINE('',#197875,#13682);
#6616=LINE('',#197876,#13683);
#6617=LINE('',#197880,#13684);
#6618=LINE('',#197881,#13685);
#6619=LINE('',#197882,#13686);
#6620=LINE('',#197884,#13687);
#6621=LINE('',#197885,#13688);
#6622=LINE('',#197889,#13689);
#6623=LINE('',#197891,#13690);
#6624=LINE('',#197893,#13691);
#6625=LINE('',#197894,#13692);
#6626=LINE('',#197898,#13693);
#6627=LINE('',#197899,#13694);
#6628=LINE('',#197900,#13695);
#6629=LINE('',#197904,#13696);
#6630=LINE('',#197905,#13697);
#6631=LINE('',#197906,#13698);
#6632=LINE('',#197908,#13699);
#6633=LINE('',#197909,#13700);
#6634=LINE('',#197913,#13701);
#6635=LINE('',#197915,#13702);
#6636=LINE('',#197917,#13703);
#6637=LINE('',#197918,#13704);
#6638=LINE('',#197922,#13705);
#6639=LINE('',#197923,#13706);
#6640=LINE('',#197924,#13707);
#6641=LINE('',#197928,#13708);
#6642=LINE('',#197929,#13709);
#6643=LINE('',#197930,#13710);
#6644=LINE('',#197932,#13711);
#6645=LINE('',#197933,#13712);
#6646=LINE('',#197937,#13713);
#6647=LINE('',#197939,#13714);
#6648=LINE('',#197941,#13715);
#6649=LINE('',#197942,#13716);
#6650=LINE('',#197946,#13717);
#6651=LINE('',#197947,#13718);
#6652=LINE('',#197948,#13719);
#6653=LINE('',#197952,#13720);
#6654=LINE('',#197953,#13721);
#6655=LINE('',#197954,#13722);
#6656=LINE('',#197956,#13723);
#6657=LINE('',#197957,#13724);
#6658=LINE('',#197961,#13725);
#6659=LINE('',#197963,#13726);
#6660=LINE('',#197965,#13727);
#6661=LINE('',#197966,#13728);
#6662=LINE('',#197970,#13729);
#6663=LINE('',#197971,#13730);
#6664=LINE('',#197972,#13731);
#6665=LINE('',#197976,#13732);
#6666=LINE('',#197977,#13733);
#6667=LINE('',#197978,#13734);
#6668=LINE('',#197980,#13735);
#6669=LINE('',#197981,#13736);
#6670=LINE('',#197985,#13737);
#6671=LINE('',#197987,#13738);
#6672=LINE('',#197989,#13739);
#6673=LINE('',#197990,#13740);
#6674=LINE('',#197994,#13741);
#6675=LINE('',#197995,#13742);
#6676=LINE('',#197996,#13743);
#6677=LINE('',#198000,#13744);
#6678=LINE('',#198001,#13745);
#6679=LINE('',#198002,#13746);
#6680=LINE('',#198004,#13747);
#6681=LINE('',#198005,#13748);
#6682=LINE('',#198009,#13749);
#6683=LINE('',#198011,#13750);
#6684=LINE('',#198013,#13751);
#6685=LINE('',#198014,#13752);
#6686=LINE('',#198018,#13753);
#6687=LINE('',#198019,#13754);
#6688=LINE('',#198020,#13755);
#6689=LINE('',#198024,#13756);
#6690=LINE('',#198025,#13757);
#6691=LINE('',#198026,#13758);
#6692=LINE('',#198028,#13759);
#6693=LINE('',#198029,#13760);
#6694=LINE('',#198033,#13761);
#6695=LINE('',#198035,#13762);
#6696=LINE('',#198037,#13763);
#6697=LINE('',#198038,#13764);
#6698=LINE('',#198042,#13765);
#6699=LINE('',#198043,#13766);
#6700=LINE('',#198044,#13767);
#6701=LINE('',#198048,#13768);
#6702=LINE('',#198049,#13769);
#6703=LINE('',#198050,#13770);
#6704=LINE('',#198052,#13771);
#6705=LINE('',#198053,#13772);
#6706=LINE('',#198057,#13773);
#6707=LINE('',#198059,#13774);
#6708=LINE('',#198061,#13775);
#6709=LINE('',#198062,#13776);
#6710=LINE('',#198066,#13777);
#6711=LINE('',#198067,#13778);
#6712=LINE('',#198068,#13779);
#6713=LINE('',#198072,#13780);
#6714=LINE('',#198073,#13781);
#6715=LINE('',#198074,#13782);
#6716=LINE('',#198076,#13783);
#6717=LINE('',#198077,#13784);
#6718=LINE('',#198081,#13785);
#6719=LINE('',#198083,#13786);
#6720=LINE('',#198085,#13787);
#6721=LINE('',#198086,#13788);
#6722=LINE('',#198090,#13789);
#6723=LINE('',#198091,#13790);
#6724=LINE('',#198092,#13791);
#6725=LINE('',#198096,#13792);
#6726=LINE('',#198097,#13793);
#6727=LINE('',#198098,#13794);
#6728=LINE('',#198100,#13795);
#6729=LINE('',#198101,#13796);
#6730=LINE('',#198105,#13797);
#6731=LINE('',#198107,#13798);
#6732=LINE('',#198109,#13799);
#6733=LINE('',#198110,#13800);
#6734=LINE('',#198114,#13801);
#6735=LINE('',#198115,#13802);
#6736=LINE('',#198116,#13803);
#6737=LINE('',#198120,#13804);
#6738=LINE('',#198121,#13805);
#6739=LINE('',#198122,#13806);
#6740=LINE('',#198124,#13807);
#6741=LINE('',#198125,#13808);
#6742=LINE('',#198129,#13809);
#6743=LINE('',#198131,#13810);
#6744=LINE('',#198133,#13811);
#6745=LINE('',#198134,#13812);
#6746=LINE('',#198138,#13813);
#6747=LINE('',#198139,#13814);
#6748=LINE('',#198140,#13815);
#6749=LINE('',#198144,#13816);
#6750=LINE('',#198145,#13817);
#6751=LINE('',#198146,#13818);
#6752=LINE('',#198148,#13819);
#6753=LINE('',#198149,#13820);
#6754=LINE('',#198153,#13821);
#6755=LINE('',#198155,#13822);
#6756=LINE('',#198157,#13823);
#6757=LINE('',#198158,#13824);
#6758=LINE('',#198162,#13825);
#6759=LINE('',#198163,#13826);
#6760=LINE('',#198164,#13827);
#6761=LINE('',#198168,#13828);
#6762=LINE('',#198169,#13829);
#6763=LINE('',#198170,#13830);
#6764=LINE('',#198172,#13831);
#6765=LINE('',#198173,#13832);
#6766=LINE('',#198177,#13833);
#6767=LINE('',#198179,#13834);
#6768=LINE('',#198181,#13835);
#6769=LINE('',#198182,#13836);
#6770=LINE('',#198186,#13837);
#6771=LINE('',#198187,#13838);
#6772=LINE('',#198188,#13839);
#6773=LINE('',#198192,#13840);
#6774=LINE('',#198193,#13841);
#6775=LINE('',#198194,#13842);
#6776=LINE('',#198196,#13843);
#6777=LINE('',#198197,#13844);
#6778=LINE('',#198201,#13845);
#6779=LINE('',#198203,#13846);
#6780=LINE('',#198205,#13847);
#6781=LINE('',#198206,#13848);
#6782=LINE('',#198210,#13849);
#6783=LINE('',#198211,#13850);
#6784=LINE('',#198212,#13851);
#6785=LINE('',#198216,#13852);
#6786=LINE('',#198217,#13853);
#6787=LINE('',#198218,#13854);
#6788=LINE('',#198220,#13855);
#6789=LINE('',#198221,#13856);
#6790=LINE('',#198225,#13857);
#6791=LINE('',#198227,#13858);
#6792=LINE('',#198229,#13859);
#6793=LINE('',#198230,#13860);
#6794=LINE('',#198234,#13861);
#6795=LINE('',#198235,#13862);
#6796=LINE('',#198236,#13863);
#6797=LINE('',#198240,#13864);
#6798=LINE('',#198241,#13865);
#6799=LINE('',#198242,#13866);
#6800=LINE('',#198244,#13867);
#6801=LINE('',#198245,#13868);
#6802=LINE('',#198249,#13869);
#6803=LINE('',#198251,#13870);
#6804=LINE('',#198253,#13871);
#6805=LINE('',#198254,#13872);
#6806=LINE('',#198258,#13873);
#6807=LINE('',#198259,#13874);
#6808=LINE('',#198260,#13875);
#6809=LINE('',#198264,#13876);
#6810=LINE('',#198265,#13877);
#6811=LINE('',#198266,#13878);
#6812=LINE('',#198268,#13879);
#6813=LINE('',#198269,#13880);
#6814=LINE('',#198273,#13881);
#6815=LINE('',#198275,#13882);
#6816=LINE('',#198277,#13883);
#6817=LINE('',#198278,#13884);
#6818=LINE('',#198282,#13885);
#6819=LINE('',#198283,#13886);
#6820=LINE('',#198284,#13887);
#6821=LINE('',#198288,#13888);
#6822=LINE('',#198289,#13889);
#6823=LINE('',#198290,#13890);
#6824=LINE('',#198292,#13891);
#6825=LINE('',#198293,#13892);
#6826=LINE('',#198297,#13893);
#6827=LINE('',#198299,#13894);
#6828=LINE('',#198301,#13895);
#6829=LINE('',#198302,#13896);
#6830=LINE('',#198306,#13897);
#6831=LINE('',#198307,#13898);
#6832=LINE('',#198308,#13899);
#6833=LINE('',#198312,#13900);
#6834=LINE('',#198313,#13901);
#6835=LINE('',#198314,#13902);
#6836=LINE('',#198316,#13903);
#6837=LINE('',#198317,#13904);
#6838=LINE('',#198321,#13905);
#6839=LINE('',#198323,#13906);
#6840=LINE('',#198325,#13907);
#6841=LINE('',#198326,#13908);
#6842=LINE('',#198330,#13909);
#6843=LINE('',#198331,#13910);
#6844=LINE('',#198332,#13911);
#6845=LINE('',#198336,#13912);
#6846=LINE('',#198337,#13913);
#6847=LINE('',#198338,#13914);
#6848=LINE('',#198340,#13915);
#6849=LINE('',#198341,#13916);
#6850=LINE('',#198345,#13917);
#6851=LINE('',#198347,#13918);
#6852=LINE('',#198349,#13919);
#6853=LINE('',#198350,#13920);
#6854=LINE('',#198354,#13921);
#6855=LINE('',#198355,#13922);
#6856=LINE('',#198356,#13923);
#6857=LINE('',#198360,#13924);
#6858=LINE('',#198361,#13925);
#6859=LINE('',#198362,#13926);
#6860=LINE('',#198364,#13927);
#6861=LINE('',#198365,#13928);
#6862=LINE('',#198369,#13929);
#6863=LINE('',#198371,#13930);
#6864=LINE('',#198373,#13931);
#6865=LINE('',#198374,#13932);
#6866=LINE('',#198378,#13933);
#6867=LINE('',#198379,#13934);
#6868=LINE('',#198380,#13935);
#6869=LINE('',#198384,#13936);
#6870=LINE('',#198385,#13937);
#6871=LINE('',#198386,#13938);
#6872=LINE('',#198388,#13939);
#6873=LINE('',#198389,#13940);
#6874=LINE('',#198393,#13941);
#6875=LINE('',#198395,#13942);
#6876=LINE('',#198397,#13943);
#6877=LINE('',#198398,#13944);
#6878=LINE('',#198402,#13945);
#6879=LINE('',#198403,#13946);
#6880=LINE('',#198404,#13947);
#6881=LINE('',#198408,#13948);
#6882=LINE('',#198409,#13949);
#6883=LINE('',#198410,#13950);
#6884=LINE('',#198412,#13951);
#6885=LINE('',#198413,#13952);
#6886=LINE('',#198417,#13953);
#6887=LINE('',#198419,#13954);
#6888=LINE('',#198421,#13955);
#6889=LINE('',#198422,#13956);
#6890=LINE('',#198426,#13957);
#6891=LINE('',#198427,#13958);
#6892=LINE('',#198428,#13959);
#6893=LINE('',#198432,#13960);
#6894=LINE('',#198433,#13961);
#6895=LINE('',#198434,#13962);
#6896=LINE('',#198436,#13963);
#6897=LINE('',#198437,#13964);
#6898=LINE('',#198441,#13965);
#6899=LINE('',#198443,#13966);
#6900=LINE('',#198445,#13967);
#6901=LINE('',#198446,#13968);
#6902=LINE('',#198450,#13969);
#6903=LINE('',#198451,#13970);
#6904=LINE('',#198452,#13971);
#6905=LINE('',#198456,#13972);
#6906=LINE('',#198457,#13973);
#6907=LINE('',#198458,#13974);
#6908=LINE('',#198460,#13975);
#6909=LINE('',#198461,#13976);
#6910=LINE('',#198465,#13977);
#6911=LINE('',#198467,#13978);
#6912=LINE('',#198469,#13979);
#6913=LINE('',#198470,#13980);
#6914=LINE('',#198474,#13981);
#6915=LINE('',#198475,#13982);
#6916=LINE('',#198476,#13983);
#6917=LINE('',#198480,#13984);
#6918=LINE('',#198481,#13985);
#6919=LINE('',#198482,#13986);
#6920=LINE('',#198484,#13987);
#6921=LINE('',#198485,#13988);
#6922=LINE('',#198489,#13989);
#6923=LINE('',#198491,#13990);
#6924=LINE('',#198493,#13991);
#6925=LINE('',#198494,#13992);
#6926=LINE('',#198498,#13993);
#6927=LINE('',#198499,#13994);
#6928=LINE('',#198500,#13995);
#6929=LINE('',#198504,#13996);
#6930=LINE('',#198505,#13997);
#6931=LINE('',#198506,#13998);
#6932=LINE('',#198508,#13999);
#6933=LINE('',#198509,#14000);
#6934=LINE('',#198513,#14001);
#6935=LINE('',#198515,#14002);
#6936=LINE('',#198517,#14003);
#6937=LINE('',#198518,#14004);
#6938=LINE('',#198522,#14005);
#6939=LINE('',#198523,#14006);
#6940=LINE('',#198524,#14007);
#6941=LINE('',#198528,#14008);
#6942=LINE('',#198529,#14009);
#6943=LINE('',#198530,#14010);
#6944=LINE('',#198532,#14011);
#6945=LINE('',#198533,#14012);
#6946=LINE('',#198537,#14013);
#6947=LINE('',#198539,#14014);
#6948=LINE('',#198541,#14015);
#6949=LINE('',#198542,#14016);
#6950=LINE('',#198546,#14017);
#6951=LINE('',#198547,#14018);
#6952=LINE('',#198548,#14019);
#6953=LINE('',#198552,#14020);
#6954=LINE('',#198553,#14021);
#6955=LINE('',#198554,#14022);
#6956=LINE('',#198556,#14023);
#6957=LINE('',#198557,#14024);
#6958=LINE('',#198561,#14025);
#6959=LINE('',#198563,#14026);
#6960=LINE('',#198565,#14027);
#6961=LINE('',#198566,#14028);
#6962=LINE('',#198570,#14029);
#6963=LINE('',#198571,#14030);
#6964=LINE('',#198572,#14031);
#6965=LINE('',#198576,#14032);
#6966=LINE('',#198577,#14033);
#6967=LINE('',#198578,#14034);
#6968=LINE('',#198580,#14035);
#6969=LINE('',#198581,#14036);
#6970=LINE('',#198585,#14037);
#6971=LINE('',#198587,#14038);
#6972=LINE('',#198589,#14039);
#6973=LINE('',#198590,#14040);
#6974=LINE('',#198594,#14041);
#6975=LINE('',#198595,#14042);
#6976=LINE('',#198596,#14043);
#6977=LINE('',#198600,#14044);
#6978=LINE('',#198601,#14045);
#6979=LINE('',#198602,#14046);
#6980=LINE('',#198604,#14047);
#6981=LINE('',#198605,#14048);
#6982=LINE('',#198609,#14049);
#6983=LINE('',#198611,#14050);
#6984=LINE('',#198613,#14051);
#6985=LINE('',#198614,#14052);
#6986=LINE('',#198618,#14053);
#6987=LINE('',#198619,#14054);
#6988=LINE('',#198620,#14055);
#6989=LINE('',#198624,#14056);
#6990=LINE('',#198625,#14057);
#6991=LINE('',#198626,#14058);
#6992=LINE('',#198628,#14059);
#6993=LINE('',#198629,#14060);
#6994=LINE('',#198633,#14061);
#6995=LINE('',#198635,#14062);
#6996=LINE('',#198637,#14063);
#6997=LINE('',#198638,#14064);
#6998=LINE('',#198642,#14065);
#6999=LINE('',#198643,#14066);
#7000=LINE('',#198644,#14067);
#7001=LINE('',#198648,#14068);
#7002=LINE('',#198649,#14069);
#7003=LINE('',#198650,#14070);
#7004=LINE('',#198652,#14071);
#7005=LINE('',#198653,#14072);
#7006=LINE('',#198657,#14073);
#7007=LINE('',#198659,#14074);
#7008=LINE('',#198661,#14075);
#7009=LINE('',#198662,#14076);
#7010=LINE('',#198666,#14077);
#7011=LINE('',#198667,#14078);
#7012=LINE('',#198668,#14079);
#7013=LINE('',#198672,#14080);
#7014=LINE('',#198673,#14081);
#7015=LINE('',#198674,#14082);
#7016=LINE('',#198676,#14083);
#7017=LINE('',#198677,#14084);
#7018=LINE('',#198681,#14085);
#7019=LINE('',#198683,#14086);
#7020=LINE('',#198685,#14087);
#7021=LINE('',#198686,#14088);
#7022=LINE('',#198690,#14089);
#7023=LINE('',#198691,#14090);
#7024=LINE('',#198692,#14091);
#7025=LINE('',#198696,#14092);
#7026=LINE('',#198697,#14093);
#7027=LINE('',#198698,#14094);
#7028=LINE('',#198700,#14095);
#7029=LINE('',#198701,#14096);
#7030=LINE('',#198705,#14097);
#7031=LINE('',#198707,#14098);
#7032=LINE('',#198709,#14099);
#7033=LINE('',#198710,#14100);
#7034=LINE('',#198714,#14101);
#7035=LINE('',#198715,#14102);
#7036=LINE('',#198716,#14103);
#7037=LINE('',#198720,#14104);
#7038=LINE('',#198721,#14105);
#7039=LINE('',#198722,#14106);
#7040=LINE('',#198724,#14107);
#7041=LINE('',#198725,#14108);
#7042=LINE('',#198729,#14109);
#7043=LINE('',#198731,#14110);
#7044=LINE('',#198733,#14111);
#7045=LINE('',#198734,#14112);
#7046=LINE('',#198738,#14113);
#7047=LINE('',#198739,#14114);
#7048=LINE('',#198740,#14115);
#7049=LINE('',#198744,#14116);
#7050=LINE('',#198745,#14117);
#7051=LINE('',#198746,#14118);
#7052=LINE('',#198748,#14119);
#7053=LINE('',#198749,#14120);
#7054=LINE('',#198753,#14121);
#7055=LINE('',#198755,#14122);
#7056=LINE('',#198757,#14123);
#7057=LINE('',#198758,#14124);
#7058=LINE('',#198762,#14125);
#7059=LINE('',#198763,#14126);
#7060=LINE('',#198764,#14127);
#7061=LINE('',#198768,#14128);
#7062=LINE('',#198769,#14129);
#7063=LINE('',#198770,#14130);
#7064=LINE('',#198772,#14131);
#7065=LINE('',#198773,#14132);
#7066=LINE('',#198777,#14133);
#7067=LINE('',#198779,#14134);
#7068=LINE('',#198781,#14135);
#7069=LINE('',#198782,#14136);
#7070=LINE('',#198786,#14137);
#7071=LINE('',#198787,#14138);
#7072=LINE('',#198788,#14139);
#7073=LINE('',#198792,#14140);
#7074=LINE('',#198793,#14141);
#7075=LINE('',#198794,#14142);
#7076=LINE('',#198796,#14143);
#7077=LINE('',#198797,#14144);
#7078=LINE('',#198801,#14145);
#7079=LINE('',#198803,#14146);
#7080=LINE('',#198805,#14147);
#7081=LINE('',#198806,#14148);
#7082=LINE('',#198810,#14149);
#7083=LINE('',#198811,#14150);
#7084=LINE('',#198812,#14151);
#7085=LINE('',#198816,#14152);
#7086=LINE('',#198817,#14153);
#7087=LINE('',#198818,#14154);
#7088=LINE('',#198820,#14155);
#7089=LINE('',#198821,#14156);
#7090=LINE('',#198825,#14157);
#7091=LINE('',#198827,#14158);
#7092=LINE('',#198829,#14159);
#7093=LINE('',#198830,#14160);
#7094=LINE('',#198834,#14161);
#7095=LINE('',#198835,#14162);
#7096=LINE('',#198836,#14163);
#7097=LINE('',#198840,#14164);
#7098=LINE('',#198841,#14165);
#7099=LINE('',#198842,#14166);
#7100=LINE('',#198844,#14167);
#7101=LINE('',#198845,#14168);
#7102=LINE('',#198849,#14169);
#7103=LINE('',#198851,#14170);
#7104=LINE('',#198853,#14171);
#7105=LINE('',#198854,#14172);
#7106=LINE('',#198858,#14173);
#7107=LINE('',#198859,#14174);
#7108=LINE('',#198860,#14175);
#7109=LINE('',#198864,#14176);
#7110=LINE('',#198865,#14177);
#7111=LINE('',#198866,#14178);
#7112=LINE('',#198868,#14179);
#7113=LINE('',#198869,#14180);
#7114=LINE('',#198873,#14181);
#7115=LINE('',#198875,#14182);
#7116=LINE('',#198877,#14183);
#7117=LINE('',#198878,#14184);
#7118=LINE('',#198882,#14185);
#7119=LINE('',#198883,#14186);
#7120=LINE('',#198884,#14187);
#7121=LINE('',#198888,#14188);
#7122=LINE('',#198889,#14189);
#7123=LINE('',#198890,#14190);
#7124=LINE('',#198892,#14191);
#7125=LINE('',#198893,#14192);
#7126=LINE('',#198897,#14193);
#7127=LINE('',#198899,#14194);
#7128=LINE('',#198901,#14195);
#7129=LINE('',#198902,#14196);
#7130=LINE('',#198906,#14197);
#7131=LINE('',#198907,#14198);
#7132=LINE('',#198908,#14199);
#7133=LINE('',#198912,#14200);
#7134=LINE('',#198913,#14201);
#7135=LINE('',#198914,#14202);
#7136=LINE('',#198916,#14203);
#7137=LINE('',#198917,#14204);
#7138=LINE('',#198921,#14205);
#7139=LINE('',#198923,#14206);
#7140=LINE('',#198925,#14207);
#7141=LINE('',#198926,#14208);
#7142=LINE('',#198930,#14209);
#7143=LINE('',#198931,#14210);
#7144=LINE('',#198932,#14211);
#7145=LINE('',#198936,#14212);
#7146=LINE('',#198937,#14213);
#7147=LINE('',#198938,#14214);
#7148=LINE('',#198940,#14215);
#7149=LINE('',#198941,#14216);
#7150=LINE('',#198945,#14217);
#7151=LINE('',#198947,#14218);
#7152=LINE('',#198949,#14219);
#7153=LINE('',#198950,#14220);
#7154=LINE('',#198954,#14221);
#7155=LINE('',#198955,#14222);
#7156=LINE('',#198956,#14223);
#7157=LINE('',#198960,#14224);
#7158=LINE('',#198961,#14225);
#7159=LINE('',#198962,#14226);
#7160=LINE('',#198964,#14227);
#7161=LINE('',#198965,#14228);
#7162=LINE('',#198969,#14229);
#7163=LINE('',#198971,#14230);
#7164=LINE('',#198973,#14231);
#7165=LINE('',#198974,#14232);
#7166=LINE('',#198978,#14233);
#7167=LINE('',#198979,#14234);
#7168=LINE('',#198980,#14235);
#7169=LINE('',#198984,#14236);
#7170=LINE('',#198985,#14237);
#7171=LINE('',#198986,#14238);
#7172=LINE('',#198988,#14239);
#7173=LINE('',#198989,#14240);
#7174=LINE('',#198993,#14241);
#7175=LINE('',#198995,#14242);
#7176=LINE('',#198997,#14243);
#7177=LINE('',#198998,#14244);
#7178=LINE('',#199002,#14245);
#7179=LINE('',#199003,#14246);
#7180=LINE('',#199004,#14247);
#7181=LINE('',#199008,#14248);
#7182=LINE('',#199009,#14249);
#7183=LINE('',#199010,#14250);
#7184=LINE('',#199012,#14251);
#7185=LINE('',#199013,#14252);
#7186=LINE('',#199017,#14253);
#7187=LINE('',#199019,#14254);
#7188=LINE('',#199021,#14255);
#7189=LINE('',#199022,#14256);
#7190=LINE('',#199026,#14257);
#7191=LINE('',#199027,#14258);
#7192=LINE('',#199028,#14259);
#7193=LINE('',#199032,#14260);
#7194=LINE('',#199033,#14261);
#7195=LINE('',#199034,#14262);
#7196=LINE('',#199036,#14263);
#7197=LINE('',#199037,#14264);
#7198=LINE('',#199041,#14265);
#7199=LINE('',#199043,#14266);
#7200=LINE('',#199045,#14267);
#7201=LINE('',#199046,#14268);
#7202=LINE('',#199050,#14269);
#7203=LINE('',#199051,#14270);
#7204=LINE('',#199052,#14271);
#7205=LINE('',#199056,#14272);
#7206=LINE('',#199057,#14273);
#7207=LINE('',#199058,#14274);
#7208=LINE('',#199060,#14275);
#7209=LINE('',#199061,#14276);
#7210=LINE('',#199065,#14277);
#7211=LINE('',#199067,#14278);
#7212=LINE('',#199069,#14279);
#7213=LINE('',#199070,#14280);
#7214=LINE('',#199074,#14281);
#7215=LINE('',#199075,#14282);
#7216=LINE('',#199076,#14283);
#7217=LINE('',#199080,#14284);
#7218=LINE('',#199081,#14285);
#7219=LINE('',#199082,#14286);
#7220=LINE('',#199084,#14287);
#7221=LINE('',#199085,#14288);
#7222=LINE('',#199089,#14289);
#7223=LINE('',#199091,#14290);
#7224=LINE('',#199093,#14291);
#7225=LINE('',#199094,#14292);
#7226=LINE('',#199098,#14293);
#7227=LINE('',#199099,#14294);
#7228=LINE('',#199100,#14295);
#7229=LINE('',#199104,#14296);
#7230=LINE('',#199105,#14297);
#7231=LINE('',#199106,#14298);
#7232=LINE('',#199108,#14299);
#7233=LINE('',#199109,#14300);
#7234=LINE('',#199113,#14301);
#7235=LINE('',#199115,#14302);
#7236=LINE('',#199117,#14303);
#7237=LINE('',#199118,#14304);
#7238=LINE('',#199122,#14305);
#7239=LINE('',#199123,#14306);
#7240=LINE('',#199124,#14307);
#7241=LINE('',#199128,#14308);
#7242=LINE('',#199129,#14309);
#7243=LINE('',#199130,#14310);
#7244=LINE('',#199132,#14311);
#7245=LINE('',#199133,#14312);
#7246=LINE('',#199137,#14313);
#7247=LINE('',#199139,#14314);
#7248=LINE('',#199141,#14315);
#7249=LINE('',#199142,#14316);
#7250=LINE('',#199146,#14317);
#7251=LINE('',#199147,#14318);
#7252=LINE('',#199148,#14319);
#7253=LINE('',#199152,#14320);
#7254=LINE('',#199153,#14321);
#7255=LINE('',#199154,#14322);
#7256=LINE('',#199156,#14323);
#7257=LINE('',#199157,#14324);
#7258=LINE('',#199161,#14325);
#7259=LINE('',#199163,#14326);
#7260=LINE('',#199165,#14327);
#7261=LINE('',#199166,#14328);
#7262=LINE('',#199170,#14329);
#7263=LINE('',#199171,#14330);
#7264=LINE('',#199172,#14331);
#7265=LINE('',#199176,#14332);
#7266=LINE('',#199177,#14333);
#7267=LINE('',#199178,#14334);
#7268=LINE('',#199180,#14335);
#7269=LINE('',#199181,#14336);
#7270=LINE('',#199185,#14337);
#7271=LINE('',#199187,#14338);
#7272=LINE('',#199189,#14339);
#7273=LINE('',#199190,#14340);
#7274=LINE('',#199194,#14341);
#7275=LINE('',#199195,#14342);
#7276=LINE('',#199196,#14343);
#7277=LINE('',#199200,#14344);
#7278=LINE('',#199201,#14345);
#7279=LINE('',#199202,#14346);
#7280=LINE('',#199204,#14347);
#7281=LINE('',#199205,#14348);
#7282=LINE('',#199209,#14349);
#7283=LINE('',#199211,#14350);
#7284=LINE('',#199213,#14351);
#7285=LINE('',#199214,#14352);
#7286=LINE('',#199218,#14353);
#7287=LINE('',#199219,#14354);
#7288=LINE('',#199220,#14355);
#7289=LINE('',#199224,#14356);
#7290=LINE('',#199225,#14357);
#7291=LINE('',#199226,#14358);
#7292=LINE('',#199228,#14359);
#7293=LINE('',#199229,#14360);
#7294=LINE('',#199233,#14361);
#7295=LINE('',#199235,#14362);
#7296=LINE('',#199237,#14363);
#7297=LINE('',#199238,#14364);
#7298=LINE('',#199242,#14365);
#7299=LINE('',#199243,#14366);
#7300=LINE('',#199244,#14367);
#7301=LINE('',#199248,#14368);
#7302=LINE('',#199249,#14369);
#7303=LINE('',#199250,#14370);
#7304=LINE('',#199252,#14371);
#7305=LINE('',#199253,#14372);
#7306=LINE('',#199257,#14373);
#7307=LINE('',#199259,#14374);
#7308=LINE('',#199261,#14375);
#7309=LINE('',#199262,#14376);
#7310=LINE('',#199266,#14377);
#7311=LINE('',#199267,#14378);
#7312=LINE('',#199268,#14379);
#7313=LINE('',#199272,#14380);
#7314=LINE('',#199273,#14381);
#7315=LINE('',#199274,#14382);
#7316=LINE('',#199276,#14383);
#7317=LINE('',#199277,#14384);
#7318=LINE('',#199281,#14385);
#7319=LINE('',#199283,#14386);
#7320=LINE('',#199285,#14387);
#7321=LINE('',#199286,#14388);
#7322=LINE('',#199290,#14389);
#7323=LINE('',#199291,#14390);
#7324=LINE('',#199292,#14391);
#7325=LINE('',#199296,#14392);
#7326=LINE('',#199297,#14393);
#7327=LINE('',#199298,#14394);
#7328=LINE('',#199300,#14395);
#7329=LINE('',#199301,#14396);
#7330=LINE('',#199305,#14397);
#7331=LINE('',#199307,#14398);
#7332=LINE('',#199309,#14399);
#7333=LINE('',#199310,#14400);
#7334=LINE('',#199314,#14401);
#7335=LINE('',#199315,#14402);
#7336=LINE('',#199316,#14403);
#7337=LINE('',#199320,#14404);
#7338=LINE('',#199321,#14405);
#7339=LINE('',#199322,#14406);
#7340=LINE('',#199324,#14407);
#7341=LINE('',#199325,#14408);
#7342=LINE('',#199329,#14409);
#7343=LINE('',#199331,#14410);
#7344=LINE('',#199333,#14411);
#7345=LINE('',#199334,#14412);
#7346=LINE('',#199338,#14413);
#7347=LINE('',#199339,#14414);
#7348=LINE('',#199340,#14415);
#7349=LINE('',#199344,#14416);
#7350=LINE('',#199345,#14417);
#7351=LINE('',#199346,#14418);
#7352=LINE('',#199348,#14419);
#7353=LINE('',#199349,#14420);
#7354=LINE('',#199353,#14421);
#7355=LINE('',#199355,#14422);
#7356=LINE('',#199357,#14423);
#7357=LINE('',#199358,#14424);
#7358=LINE('',#199362,#14425);
#7359=LINE('',#199363,#14426);
#7360=LINE('',#199364,#14427);
#7361=LINE('',#199368,#14428);
#7362=LINE('',#199369,#14429);
#7363=LINE('',#199370,#14430);
#7364=LINE('',#199372,#14431);
#7365=LINE('',#199373,#14432);
#7366=LINE('',#199377,#14433);
#7367=LINE('',#199379,#14434);
#7368=LINE('',#199381,#14435);
#7369=LINE('',#199382,#14436);
#7370=LINE('',#199386,#14437);
#7371=LINE('',#199387,#14438);
#7372=LINE('',#199388,#14439);
#7373=LINE('',#199392,#14440);
#7374=LINE('',#199393,#14441);
#7375=LINE('',#199394,#14442);
#7376=LINE('',#199396,#14443);
#7377=LINE('',#199397,#14444);
#7378=LINE('',#199401,#14445);
#7379=LINE('',#199403,#14446);
#7380=LINE('',#199405,#14447);
#7381=LINE('',#199406,#14448);
#7382=LINE('',#199410,#14449);
#7383=LINE('',#199411,#14450);
#7384=LINE('',#199412,#14451);
#7385=LINE('',#199416,#14452);
#7386=LINE('',#199417,#14453);
#7387=LINE('',#199418,#14454);
#7388=LINE('',#199420,#14455);
#7389=LINE('',#199421,#14456);
#7390=LINE('',#199425,#14457);
#7391=LINE('',#199427,#14458);
#7392=LINE('',#199429,#14459);
#7393=LINE('',#199430,#14460);
#7394=LINE('',#199434,#14461);
#7395=LINE('',#199435,#14462);
#7396=LINE('',#199436,#14463);
#7397=LINE('',#199440,#14464);
#7398=LINE('',#199441,#14465);
#7399=LINE('',#199442,#14466);
#7400=LINE('',#199444,#14467);
#7401=LINE('',#199445,#14468);
#7402=LINE('',#199449,#14469);
#7403=LINE('',#199451,#14470);
#7404=LINE('',#199453,#14471);
#7405=LINE('',#199454,#14472);
#7406=LINE('',#199458,#14473);
#7407=LINE('',#199459,#14474);
#7408=LINE('',#199460,#14475);
#7409=LINE('',#199464,#14476);
#7410=LINE('',#199465,#14477);
#7411=LINE('',#199466,#14478);
#7412=LINE('',#199468,#14479);
#7413=LINE('',#199469,#14480);
#7414=LINE('',#199473,#14481);
#7415=LINE('',#199475,#14482);
#7416=LINE('',#199477,#14483);
#7417=LINE('',#199478,#14484);
#7418=LINE('',#199482,#14485);
#7419=LINE('',#199483,#14486);
#7420=LINE('',#199484,#14487);
#7421=LINE('',#199488,#14488);
#7422=LINE('',#199489,#14489);
#7423=LINE('',#199490,#14490);
#7424=LINE('',#199492,#14491);
#7425=LINE('',#199493,#14492);
#7426=LINE('',#199497,#14493);
#7427=LINE('',#199499,#14494);
#7428=LINE('',#199501,#14495);
#7429=LINE('',#199502,#14496);
#7430=LINE('',#199506,#14497);
#7431=LINE('',#199507,#14498);
#7432=LINE('',#199508,#14499);
#7433=LINE('',#199512,#14500);
#7434=LINE('',#199513,#14501);
#7435=LINE('',#199514,#14502);
#7436=LINE('',#199516,#14503);
#7437=LINE('',#199517,#14504);
#7438=LINE('',#199521,#14505);
#7439=LINE('',#199523,#14506);
#7440=LINE('',#199525,#14507);
#7441=LINE('',#199526,#14508);
#7442=LINE('',#199530,#14509);
#7443=LINE('',#199531,#14510);
#7444=LINE('',#199532,#14511);
#7445=LINE('',#199536,#14512);
#7446=LINE('',#199537,#14513);
#7447=LINE('',#199538,#14514);
#7448=LINE('',#199540,#14515);
#7449=LINE('',#199541,#14516);
#7450=LINE('',#199545,#14517);
#7451=LINE('',#199547,#14518);
#7452=LINE('',#199549,#14519);
#7453=LINE('',#199550,#14520);
#7454=LINE('',#199554,#14521);
#7455=LINE('',#199555,#14522);
#7456=LINE('',#199556,#14523);
#7457=LINE('',#199560,#14524);
#7458=LINE('',#199561,#14525);
#7459=LINE('',#199562,#14526);
#7460=LINE('',#199564,#14527);
#7461=LINE('',#199565,#14528);
#7462=LINE('',#199569,#14529);
#7463=LINE('',#199571,#14530);
#7464=LINE('',#199573,#14531);
#7465=LINE('',#199574,#14532);
#7466=LINE('',#199578,#14533);
#7467=LINE('',#199579,#14534);
#7468=LINE('',#199580,#14535);
#7469=LINE('',#199584,#14536);
#7470=LINE('',#199585,#14537);
#7471=LINE('',#199586,#14538);
#7472=LINE('',#199588,#14539);
#7473=LINE('',#199589,#14540);
#7474=LINE('',#199593,#14541);
#7475=LINE('',#199595,#14542);
#7476=LINE('',#199597,#14543);
#7477=LINE('',#199598,#14544);
#7478=LINE('',#199602,#14545);
#7479=LINE('',#199603,#14546);
#7480=LINE('',#199604,#14547);
#7481=LINE('',#199608,#14548);
#7482=LINE('',#199609,#14549);
#7483=LINE('',#199610,#14550);
#7484=LINE('',#199612,#14551);
#7485=LINE('',#199613,#14552);
#7486=LINE('',#199617,#14553);
#7487=LINE('',#199619,#14554);
#7488=LINE('',#199621,#14555);
#7489=LINE('',#199622,#14556);
#7490=LINE('',#199626,#14557);
#7491=LINE('',#199627,#14558);
#7492=LINE('',#199628,#14559);
#7493=LINE('',#199632,#14560);
#7494=LINE('',#199633,#14561);
#7495=LINE('',#199634,#14562);
#7496=LINE('',#199636,#14563);
#7497=LINE('',#199637,#14564);
#7498=LINE('',#199641,#14565);
#7499=LINE('',#199643,#14566);
#7500=LINE('',#199645,#14567);
#7501=LINE('',#199646,#14568);
#7502=LINE('',#199650,#14569);
#7503=LINE('',#199651,#14570);
#7504=LINE('',#199652,#14571);
#7505=LINE('',#199656,#14572);
#7506=LINE('',#199657,#14573);
#7507=LINE('',#199658,#14574);
#7508=LINE('',#199660,#14575);
#7509=LINE('',#199661,#14576);
#7510=LINE('',#199665,#14577);
#7511=LINE('',#199667,#14578);
#7512=LINE('',#199669,#14579);
#7513=LINE('',#199670,#14580);
#7514=LINE('',#199674,#14581);
#7515=LINE('',#199675,#14582);
#7516=LINE('',#199676,#14583);
#7517=LINE('',#199680,#14584);
#7518=LINE('',#199681,#14585);
#7519=LINE('',#199682,#14586);
#7520=LINE('',#199684,#14587);
#7521=LINE('',#199685,#14588);
#7522=LINE('',#199689,#14589);
#7523=LINE('',#199691,#14590);
#7524=LINE('',#199693,#14591);
#7525=LINE('',#199694,#14592);
#7526=LINE('',#199698,#14593);
#7527=LINE('',#199699,#14594);
#7528=LINE('',#199700,#14595);
#7529=LINE('',#199704,#14596);
#7530=LINE('',#199705,#14597);
#7531=LINE('',#199706,#14598);
#7532=LINE('',#199708,#14599);
#7533=LINE('',#199709,#14600);
#7534=LINE('',#199713,#14601);
#7535=LINE('',#199715,#14602);
#7536=LINE('',#199717,#14603);
#7537=LINE('',#199718,#14604);
#7538=LINE('',#199722,#14605);
#7539=LINE('',#199723,#14606);
#7540=LINE('',#199724,#14607);
#7541=LINE('',#199728,#14608);
#7542=LINE('',#199729,#14609);
#7543=LINE('',#199730,#14610);
#7544=LINE('',#199732,#14611);
#7545=LINE('',#199733,#14612);
#7546=LINE('',#199737,#14613);
#7547=LINE('',#199739,#14614);
#7548=LINE('',#199741,#14615);
#7549=LINE('',#199742,#14616);
#7550=LINE('',#199746,#14617);
#7551=LINE('',#199747,#14618);
#7552=LINE('',#199748,#14619);
#7553=LINE('',#199752,#14620);
#7554=LINE('',#199753,#14621);
#7555=LINE('',#199754,#14622);
#7556=LINE('',#199756,#14623);
#7557=LINE('',#199757,#14624);
#7558=LINE('',#199761,#14625);
#7559=LINE('',#199763,#14626);
#7560=LINE('',#199765,#14627);
#7561=LINE('',#199766,#14628);
#7562=LINE('',#199770,#14629);
#7563=LINE('',#199771,#14630);
#7564=LINE('',#199772,#14631);
#7565=LINE('',#199776,#14632);
#7566=LINE('',#199777,#14633);
#7567=LINE('',#199778,#14634);
#7568=LINE('',#199780,#14635);
#7569=LINE('',#199781,#14636);
#7570=LINE('',#199785,#14637);
#7571=LINE('',#199787,#14638);
#7572=LINE('',#199789,#14639);
#7573=LINE('',#199790,#14640);
#7574=LINE('',#199794,#14641);
#7575=LINE('',#199795,#14642);
#7576=LINE('',#199796,#14643);
#7577=LINE('',#199800,#14644);
#7578=LINE('',#199801,#14645);
#7579=LINE('',#199802,#14646);
#7580=LINE('',#199804,#14647);
#7581=LINE('',#199805,#14648);
#7582=LINE('',#199809,#14649);
#7583=LINE('',#199811,#14650);
#7584=LINE('',#199813,#14651);
#7585=LINE('',#199814,#14652);
#7586=LINE('',#199818,#14653);
#7587=LINE('',#199819,#14654);
#7588=LINE('',#199820,#14655);
#7589=LINE('',#199824,#14656);
#7590=LINE('',#199825,#14657);
#7591=LINE('',#199826,#14658);
#7592=LINE('',#199828,#14659);
#7593=LINE('',#199829,#14660);
#7594=LINE('',#199833,#14661);
#7595=LINE('',#199835,#14662);
#7596=LINE('',#199837,#14663);
#7597=LINE('',#199838,#14664);
#7598=LINE('',#199842,#14665);
#7599=LINE('',#199843,#14666);
#7600=LINE('',#199844,#14667);
#7601=LINE('',#199848,#14668);
#7602=LINE('',#199849,#14669);
#7603=LINE('',#199850,#14670);
#7604=LINE('',#199852,#14671);
#7605=LINE('',#199853,#14672);
#7606=LINE('',#199857,#14673);
#7607=LINE('',#199859,#14674);
#7608=LINE('',#199861,#14675);
#7609=LINE('',#199862,#14676);
#7610=LINE('',#199866,#14677);
#7611=LINE('',#199867,#14678);
#7612=LINE('',#199868,#14679);
#7613=LINE('',#199872,#14680);
#7614=LINE('',#199873,#14681);
#7615=LINE('',#199874,#14682);
#7616=LINE('',#199876,#14683);
#7617=LINE('',#199877,#14684);
#7618=LINE('',#199881,#14685);
#7619=LINE('',#199883,#14686);
#7620=LINE('',#199885,#14687);
#7621=LINE('',#199886,#14688);
#7622=LINE('',#199890,#14689);
#7623=LINE('',#199891,#14690);
#7624=LINE('',#199892,#14691);
#7625=LINE('',#199896,#14692);
#7626=LINE('',#199897,#14693);
#7627=LINE('',#199898,#14694);
#7628=LINE('',#199900,#14695);
#7629=LINE('',#199901,#14696);
#7630=LINE('',#199905,#14697);
#7631=LINE('',#199907,#14698);
#7632=LINE('',#199909,#14699);
#7633=LINE('',#199910,#14700);
#7634=LINE('',#199914,#14701);
#7635=LINE('',#199915,#14702);
#7636=LINE('',#199916,#14703);
#7637=LINE('',#199920,#14704);
#7638=LINE('',#199921,#14705);
#7639=LINE('',#199922,#14706);
#7640=LINE('',#199924,#14707);
#7641=LINE('',#199925,#14708);
#7642=LINE('',#199929,#14709);
#7643=LINE('',#199931,#14710);
#7644=LINE('',#199933,#14711);
#7645=LINE('',#199934,#14712);
#7646=LINE('',#199938,#14713);
#7647=LINE('',#199939,#14714);
#7648=LINE('',#199940,#14715);
#7649=LINE('',#199944,#14716);
#7650=LINE('',#199945,#14717);
#7651=LINE('',#199946,#14718);
#7652=LINE('',#199948,#14719);
#7653=LINE('',#199949,#14720);
#7654=LINE('',#199953,#14721);
#7655=LINE('',#199955,#14722);
#7656=LINE('',#199957,#14723);
#7657=LINE('',#199958,#14724);
#7658=LINE('',#199962,#14725);
#7659=LINE('',#199963,#14726);
#7660=LINE('',#199964,#14727);
#7661=LINE('',#199968,#14728);
#7662=LINE('',#199969,#14729);
#7663=LINE('',#199970,#14730);
#7664=LINE('',#199972,#14731);
#7665=LINE('',#199973,#14732);
#7666=LINE('',#199977,#14733);
#7667=LINE('',#199979,#14734);
#7668=LINE('',#199981,#14735);
#7669=LINE('',#199982,#14736);
#7670=LINE('',#199986,#14737);
#7671=LINE('',#199987,#14738);
#7672=LINE('',#199988,#14739);
#7673=LINE('',#199992,#14740);
#7674=LINE('',#199993,#14741);
#7675=LINE('',#199994,#14742);
#7676=LINE('',#199996,#14743);
#7677=LINE('',#199997,#14744);
#7678=LINE('',#200001,#14745);
#7679=LINE('',#200003,#14746);
#7680=LINE('',#200005,#14747);
#7681=LINE('',#200006,#14748);
#7682=LINE('',#200010,#14749);
#7683=LINE('',#200011,#14750);
#7684=LINE('',#200012,#14751);
#7685=LINE('',#200016,#14752);
#7686=LINE('',#200017,#14753);
#7687=LINE('',#200018,#14754);
#7688=LINE('',#200020,#14755);
#7689=LINE('',#200021,#14756);
#7690=LINE('',#200025,#14757);
#7691=LINE('',#200027,#14758);
#7692=LINE('',#200029,#14759);
#7693=LINE('',#200030,#14760);
#7694=LINE('',#200034,#14761);
#7695=LINE('',#200035,#14762);
#7696=LINE('',#200036,#14763);
#7697=LINE('',#200040,#14764);
#7698=LINE('',#200041,#14765);
#7699=LINE('',#200042,#14766);
#7700=LINE('',#200044,#14767);
#7701=LINE('',#200045,#14768);
#7702=LINE('',#200049,#14769);
#7703=LINE('',#200051,#14770);
#7704=LINE('',#200053,#14771);
#7705=LINE('',#200054,#14772);
#7706=LINE('',#200058,#14773);
#7707=LINE('',#200059,#14774);
#7708=LINE('',#200060,#14775);
#7709=LINE('',#200064,#14776);
#7710=LINE('',#200065,#14777);
#7711=LINE('',#200066,#14778);
#7712=LINE('',#200068,#14779);
#7713=LINE('',#200069,#14780);
#7714=LINE('',#200073,#14781);
#7715=LINE('',#200075,#14782);
#7716=LINE('',#200077,#14783);
#7717=LINE('',#200078,#14784);
#7718=LINE('',#200082,#14785);
#7719=LINE('',#200083,#14786);
#7720=LINE('',#200084,#14787);
#7721=LINE('',#200088,#14788);
#7722=LINE('',#200089,#14789);
#7723=LINE('',#200090,#14790);
#7724=LINE('',#200092,#14791);
#7725=LINE('',#200093,#14792);
#7726=LINE('',#200097,#14793);
#7727=LINE('',#200099,#14794);
#7728=LINE('',#200101,#14795);
#7729=LINE('',#200102,#14796);
#7730=LINE('',#200106,#14797);
#7731=LINE('',#200107,#14798);
#7732=LINE('',#200108,#14799);
#7733=LINE('',#200112,#14800);
#7734=LINE('',#200113,#14801);
#7735=LINE('',#200114,#14802);
#7736=LINE('',#200116,#14803);
#7737=LINE('',#200117,#14804);
#7738=LINE('',#200121,#14805);
#7739=LINE('',#200123,#14806);
#7740=LINE('',#200125,#14807);
#7741=LINE('',#200126,#14808);
#7742=LINE('',#200130,#14809);
#7743=LINE('',#200131,#14810);
#7744=LINE('',#200132,#14811);
#7745=LINE('',#200136,#14812);
#7746=LINE('',#200137,#14813);
#7747=LINE('',#200138,#14814);
#7748=LINE('',#200140,#14815);
#7749=LINE('',#200141,#14816);
#7750=LINE('',#200145,#14817);
#7751=LINE('',#200147,#14818);
#7752=LINE('',#200149,#14819);
#7753=LINE('',#200150,#14820);
#7754=LINE('',#200154,#14821);
#7755=LINE('',#200155,#14822);
#7756=LINE('',#200156,#14823);
#7757=LINE('',#200160,#14824);
#7758=LINE('',#200161,#14825);
#7759=LINE('',#200162,#14826);
#7760=LINE('',#200164,#14827);
#7761=LINE('',#200165,#14828);
#7762=LINE('',#200169,#14829);
#7763=LINE('',#200171,#14830);
#7764=LINE('',#200173,#14831);
#7765=LINE('',#200174,#14832);
#7766=LINE('',#200178,#14833);
#7767=LINE('',#200179,#14834);
#7768=LINE('',#200180,#14835);
#7769=LINE('',#200184,#14836);
#7770=LINE('',#200185,#14837);
#7771=LINE('',#200186,#14838);
#7772=LINE('',#200188,#14839);
#7773=LINE('',#200189,#14840);
#7774=LINE('',#200193,#14841);
#7775=LINE('',#200195,#14842);
#7776=LINE('',#200197,#14843);
#7777=LINE('',#200198,#14844);
#7778=LINE('',#200202,#14845);
#7779=LINE('',#200203,#14846);
#7780=LINE('',#200204,#14847);
#7781=LINE('',#200208,#14848);
#7782=LINE('',#200209,#14849);
#7783=LINE('',#200210,#14850);
#7784=LINE('',#200212,#14851);
#7785=LINE('',#200213,#14852);
#7786=LINE('',#200217,#14853);
#7787=LINE('',#200219,#14854);
#7788=LINE('',#200221,#14855);
#7789=LINE('',#200222,#14856);
#7790=LINE('',#200226,#14857);
#7791=LINE('',#200227,#14858);
#7792=LINE('',#200228,#14859);
#7793=LINE('',#200232,#14860);
#7794=LINE('',#200233,#14861);
#7795=LINE('',#200234,#14862);
#7796=LINE('',#200236,#14863);
#7797=LINE('',#200237,#14864);
#7798=LINE('',#200241,#14865);
#7799=LINE('',#200243,#14866);
#7800=LINE('',#200245,#14867);
#7801=LINE('',#200246,#14868);
#7802=LINE('',#200250,#14869);
#7803=LINE('',#200251,#14870);
#7804=LINE('',#200252,#14871);
#7805=LINE('',#200256,#14872);
#7806=LINE('',#200257,#14873);
#7807=LINE('',#200258,#14874);
#7808=LINE('',#200260,#14875);
#7809=LINE('',#200261,#14876);
#7810=LINE('',#200265,#14877);
#7811=LINE('',#200267,#14878);
#7812=LINE('',#200269,#14879);
#7813=LINE('',#200270,#14880);
#7814=LINE('',#200274,#14881);
#7815=LINE('',#200275,#14882);
#7816=LINE('',#200276,#14883);
#7817=LINE('',#200280,#14884);
#7818=LINE('',#200281,#14885);
#7819=LINE('',#200282,#14886);
#7820=LINE('',#200284,#14887);
#7821=LINE('',#200285,#14888);
#7822=LINE('',#200289,#14889);
#7823=LINE('',#200291,#14890);
#7824=LINE('',#200293,#14891);
#7825=LINE('',#200294,#14892);
#7826=LINE('',#200298,#14893);
#7827=LINE('',#200299,#14894);
#7828=LINE('',#200300,#14895);
#7829=LINE('',#200304,#14896);
#7830=LINE('',#200305,#14897);
#7831=LINE('',#200306,#14898);
#7832=LINE('',#200308,#14899);
#7833=LINE('',#200309,#14900);
#7834=LINE('',#200313,#14901);
#7835=LINE('',#200315,#14902);
#7836=LINE('',#200317,#14903);
#7837=LINE('',#200318,#14904);
#7838=LINE('',#200322,#14905);
#7839=LINE('',#200323,#14906);
#7840=LINE('',#200324,#14907);
#7841=LINE('',#200328,#14908);
#7842=LINE('',#200329,#14909);
#7843=LINE('',#200330,#14910);
#7844=LINE('',#200332,#14911);
#7845=LINE('',#200333,#14912);
#7846=LINE('',#200337,#14913);
#7847=LINE('',#200339,#14914);
#7848=LINE('',#200341,#14915);
#7849=LINE('',#200342,#14916);
#7850=LINE('',#200346,#14917);
#7851=LINE('',#200347,#14918);
#7852=LINE('',#200348,#14919);
#7853=LINE('',#200352,#14920);
#7854=LINE('',#200353,#14921);
#7855=LINE('',#200354,#14922);
#7856=LINE('',#200356,#14923);
#7857=LINE('',#200357,#14924);
#7858=LINE('',#200361,#14925);
#7859=LINE('',#200363,#14926);
#7860=LINE('',#200365,#14927);
#7861=LINE('',#200366,#14928);
#7862=LINE('',#200370,#14929);
#7863=LINE('',#200371,#14930);
#7864=LINE('',#200372,#14931);
#7865=LINE('',#200376,#14932);
#7866=LINE('',#200377,#14933);
#7867=LINE('',#200378,#14934);
#7868=LINE('',#200380,#14935);
#7869=LINE('',#200381,#14936);
#7870=LINE('',#200385,#14937);
#7871=LINE('',#200387,#14938);
#7872=LINE('',#200389,#14939);
#7873=LINE('',#200390,#14940);
#7874=LINE('',#200394,#14941);
#7875=LINE('',#200395,#14942);
#7876=LINE('',#200396,#14943);
#7877=LINE('',#200400,#14944);
#7878=LINE('',#200401,#14945);
#7879=LINE('',#200402,#14946);
#7880=LINE('',#200404,#14947);
#7881=LINE('',#200405,#14948);
#7882=LINE('',#200409,#14949);
#7883=LINE('',#200411,#14950);
#7884=LINE('',#200413,#14951);
#7885=LINE('',#200414,#14952);
#7886=LINE('',#200418,#14953);
#7887=LINE('',#200419,#14954);
#7888=LINE('',#200420,#14955);
#7889=LINE('',#200424,#14956);
#7890=LINE('',#200425,#14957);
#7891=LINE('',#200426,#14958);
#7892=LINE('',#200428,#14959);
#7893=LINE('',#200429,#14960);
#7894=LINE('',#200433,#14961);
#7895=LINE('',#200435,#14962);
#7896=LINE('',#200437,#14963);
#7897=LINE('',#200438,#14964);
#7898=LINE('',#200442,#14965);
#7899=LINE('',#200443,#14966);
#7900=LINE('',#200444,#14967);
#7901=LINE('',#200448,#14968);
#7902=LINE('',#200449,#14969);
#7903=LINE('',#200450,#14970);
#7904=LINE('',#200452,#14971);
#7905=LINE('',#200453,#14972);
#7906=LINE('',#200457,#14973);
#7907=LINE('',#200459,#14974);
#7908=LINE('',#200461,#14975);
#7909=LINE('',#200462,#14976);
#7910=LINE('',#200466,#14977);
#7911=LINE('',#200467,#14978);
#7912=LINE('',#200468,#14979);
#7913=LINE('',#200472,#14980);
#7914=LINE('',#200473,#14981);
#7915=LINE('',#200474,#14982);
#7916=LINE('',#200476,#14983);
#7917=LINE('',#200477,#14984);
#7918=LINE('',#200481,#14985);
#7919=LINE('',#200483,#14986);
#7920=LINE('',#200485,#14987);
#7921=LINE('',#200486,#14988);
#7922=LINE('',#200490,#14989);
#7923=LINE('',#200491,#14990);
#7924=LINE('',#200492,#14991);
#7925=LINE('',#200496,#14992);
#7926=LINE('',#200497,#14993);
#7927=LINE('',#200498,#14994);
#7928=LINE('',#200500,#14995);
#7929=LINE('',#200501,#14996);
#7930=LINE('',#200505,#14997);
#7931=LINE('',#200507,#14998);
#7932=LINE('',#200509,#14999);
#7933=LINE('',#200510,#15000);
#7934=LINE('',#200514,#15001);
#7935=LINE('',#200515,#15002);
#7936=LINE('',#200516,#15003);
#7937=LINE('',#200520,#15004);
#7938=LINE('',#200521,#15005);
#7939=LINE('',#200522,#15006);
#7940=LINE('',#200524,#15007);
#7941=LINE('',#200525,#15008);
#7942=LINE('',#200529,#15009);
#7943=LINE('',#200531,#15010);
#7944=LINE('',#200533,#15011);
#7945=LINE('',#200534,#15012);
#7946=LINE('',#200538,#15013);
#7947=LINE('',#200539,#15014);
#7948=LINE('',#200540,#15015);
#7949=LINE('',#200544,#15016);
#7950=LINE('',#200545,#15017);
#7951=LINE('',#200546,#15018);
#7952=LINE('',#200548,#15019);
#7953=LINE('',#200549,#15020);
#7954=LINE('',#200553,#15021);
#7955=LINE('',#200555,#15022);
#7956=LINE('',#200557,#15023);
#7957=LINE('',#200558,#15024);
#7958=LINE('',#200562,#15025);
#7959=LINE('',#200563,#15026);
#7960=LINE('',#200564,#15027);
#7961=LINE('',#200568,#15028);
#7962=LINE('',#200569,#15029);
#7963=LINE('',#200570,#15030);
#7964=LINE('',#200572,#15031);
#7965=LINE('',#200573,#15032);
#7966=LINE('',#200577,#15033);
#7967=LINE('',#200579,#15034);
#7968=LINE('',#200581,#15035);
#7969=LINE('',#200582,#15036);
#7970=LINE('',#200586,#15037);
#7971=LINE('',#200587,#15038);
#7972=LINE('',#200588,#15039);
#7973=LINE('',#200592,#15040);
#7974=LINE('',#200593,#15041);
#7975=LINE('',#200594,#15042);
#7976=LINE('',#200596,#15043);
#7977=LINE('',#200597,#15044);
#7978=LINE('',#200601,#15045);
#7979=LINE('',#200603,#15046);
#7980=LINE('',#200605,#15047);
#7981=LINE('',#200606,#15048);
#7982=LINE('',#200610,#15049);
#7983=LINE('',#200611,#15050);
#7984=LINE('',#200612,#15051);
#7985=LINE('',#200616,#15052);
#7986=LINE('',#200617,#15053);
#7987=LINE('',#200618,#15054);
#7988=LINE('',#200620,#15055);
#7989=LINE('',#200621,#15056);
#7990=LINE('',#200625,#15057);
#7991=LINE('',#200627,#15058);
#7992=LINE('',#200629,#15059);
#7993=LINE('',#200630,#15060);
#7994=LINE('',#200634,#15061);
#7995=LINE('',#200635,#15062);
#7996=LINE('',#200636,#15063);
#7997=LINE('',#200640,#15064);
#7998=LINE('',#200641,#15065);
#7999=LINE('',#200642,#15066);
#8000=LINE('',#200644,#15067);
#8001=LINE('',#200645,#15068);
#8002=LINE('',#200649,#15069);
#8003=LINE('',#200651,#15070);
#8004=LINE('',#200653,#15071);
#8005=LINE('',#200654,#15072);
#8006=LINE('',#200658,#15073);
#8007=LINE('',#200659,#15074);
#8008=LINE('',#200660,#15075);
#8009=LINE('',#200664,#15076);
#8010=LINE('',#200665,#15077);
#8011=LINE('',#200666,#15078);
#8012=LINE('',#200668,#15079);
#8013=LINE('',#200669,#15080);
#8014=LINE('',#200673,#15081);
#8015=LINE('',#200675,#15082);
#8016=LINE('',#200677,#15083);
#8017=LINE('',#200678,#15084);
#8018=LINE('',#200682,#15085);
#8019=LINE('',#200683,#15086);
#8020=LINE('',#200684,#15087);
#8021=LINE('',#200688,#15088);
#8022=LINE('',#200689,#15089);
#8023=LINE('',#200690,#15090);
#8024=LINE('',#200692,#15091);
#8025=LINE('',#200693,#15092);
#8026=LINE('',#200697,#15093);
#8027=LINE('',#200699,#15094);
#8028=LINE('',#200701,#15095);
#8029=LINE('',#200702,#15096);
#8030=LINE('',#200706,#15097);
#8031=LINE('',#200707,#15098);
#8032=LINE('',#200708,#15099);
#8033=LINE('',#200712,#15100);
#8034=LINE('',#200713,#15101);
#8035=LINE('',#200714,#15102);
#8036=LINE('',#200716,#15103);
#8037=LINE('',#200717,#15104);
#8038=LINE('',#200721,#15105);
#8039=LINE('',#200723,#15106);
#8040=LINE('',#200725,#15107);
#8041=LINE('',#200726,#15108);
#8042=LINE('',#200730,#15109);
#8043=LINE('',#200731,#15110);
#8044=LINE('',#200732,#15111);
#8045=LINE('',#200736,#15112);
#8046=LINE('',#200737,#15113);
#8047=LINE('',#200738,#15114);
#8048=LINE('',#200740,#15115);
#8049=LINE('',#200741,#15116);
#8050=LINE('',#200745,#15117);
#8051=LINE('',#200747,#15118);
#8052=LINE('',#200749,#15119);
#8053=LINE('',#200750,#15120);
#8054=LINE('',#200754,#15121);
#8055=LINE('',#200755,#15122);
#8056=LINE('',#200756,#15123);
#8057=LINE('',#200760,#15124);
#8058=LINE('',#200761,#15125);
#8059=LINE('',#200762,#15126);
#8060=LINE('',#200764,#15127);
#8061=LINE('',#200765,#15128);
#8062=LINE('',#200769,#15129);
#8063=LINE('',#200771,#15130);
#8064=LINE('',#200773,#15131);
#8065=LINE('',#200774,#15132);
#8066=LINE('',#200778,#15133);
#8067=LINE('',#200779,#15134);
#8068=LINE('',#200780,#15135);
#8069=LINE('',#200784,#15136);
#8070=LINE('',#200785,#15137);
#8071=LINE('',#200786,#15138);
#8072=LINE('',#200788,#15139);
#8073=LINE('',#200789,#15140);
#8074=LINE('',#200793,#15141);
#8075=LINE('',#200795,#15142);
#8076=LINE('',#200797,#15143);
#8077=LINE('',#200798,#15144);
#8078=LINE('',#200802,#15145);
#8079=LINE('',#200803,#15146);
#8080=LINE('',#200804,#15147);
#8081=LINE('',#200808,#15148);
#8082=LINE('',#200809,#15149);
#8083=LINE('',#200810,#15150);
#8084=LINE('',#200812,#15151);
#8085=LINE('',#200813,#15152);
#8086=LINE('',#200817,#15153);
#8087=LINE('',#200819,#15154);
#8088=LINE('',#200821,#15155);
#8089=LINE('',#200822,#15156);
#8090=LINE('',#200826,#15157);
#8091=LINE('',#200827,#15158);
#8092=LINE('',#200828,#15159);
#8093=LINE('',#200832,#15160);
#8094=LINE('',#200833,#15161);
#8095=LINE('',#200834,#15162);
#8096=LINE('',#200836,#15163);
#8097=LINE('',#200837,#15164);
#8098=LINE('',#200841,#15165);
#8099=LINE('',#200843,#15166);
#8100=LINE('',#200845,#15167);
#8101=LINE('',#200846,#15168);
#8102=LINE('',#200850,#15169);
#8103=LINE('',#200851,#15170);
#8104=LINE('',#200852,#15171);
#8105=LINE('',#200856,#15172);
#8106=LINE('',#200857,#15173);
#8107=LINE('',#200858,#15174);
#8108=LINE('',#200860,#15175);
#8109=LINE('',#200861,#15176);
#8110=LINE('',#200865,#15177);
#8111=LINE('',#200867,#15178);
#8112=LINE('',#200869,#15179);
#8113=LINE('',#200870,#15180);
#8114=LINE('',#200874,#15181);
#8115=LINE('',#200875,#15182);
#8116=LINE('',#200876,#15183);
#8117=LINE('',#200880,#15184);
#8118=LINE('',#200881,#15185);
#8119=LINE('',#200882,#15186);
#8120=LINE('',#200884,#15187);
#8121=LINE('',#200885,#15188);
#8122=LINE('',#200889,#15189);
#8123=LINE('',#200891,#15190);
#8124=LINE('',#200893,#15191);
#8125=LINE('',#200894,#15192);
#8126=LINE('',#200898,#15193);
#8127=LINE('',#200899,#15194);
#8128=LINE('',#200900,#15195);
#8129=LINE('',#200904,#15196);
#8130=LINE('',#200905,#15197);
#8131=LINE('',#200906,#15198);
#8132=LINE('',#200908,#15199);
#8133=LINE('',#200909,#15200);
#8134=LINE('',#200913,#15201);
#8135=LINE('',#200915,#15202);
#8136=LINE('',#200917,#15203);
#8137=LINE('',#200918,#15204);
#8138=LINE('',#200922,#15205);
#8139=LINE('',#200923,#15206);
#8140=LINE('',#200924,#15207);
#8141=LINE('',#200928,#15208);
#8142=LINE('',#200929,#15209);
#8143=LINE('',#200930,#15210);
#8144=LINE('',#200932,#15211);
#8145=LINE('',#200933,#15212);
#8146=LINE('',#200937,#15213);
#8147=LINE('',#200939,#15214);
#8148=LINE('',#200941,#15215);
#8149=LINE('',#200942,#15216);
#8150=LINE('',#200946,#15217);
#8151=LINE('',#200947,#15218);
#8152=LINE('',#200948,#15219);
#8153=LINE('',#200952,#15220);
#8154=LINE('',#200953,#15221);
#8155=LINE('',#200954,#15222);
#8156=LINE('',#200956,#15223);
#8157=LINE('',#200957,#15224);
#8158=LINE('',#200961,#15225);
#8159=LINE('',#200963,#15226);
#8160=LINE('',#200965,#15227);
#8161=LINE('',#200966,#15228);
#8162=LINE('',#200970,#15229);
#8163=LINE('',#200971,#15230);
#8164=LINE('',#200972,#15231);
#8165=LINE('',#200976,#15232);
#8166=LINE('',#200977,#15233);
#8167=LINE('',#200978,#15234);
#8168=LINE('',#200980,#15235);
#8169=LINE('',#200981,#15236);
#8170=LINE('',#200985,#15237);
#8171=LINE('',#200987,#15238);
#8172=LINE('',#200989,#15239);
#8173=LINE('',#200990,#15240);
#8174=LINE('',#200994,#15241);
#8175=LINE('',#200995,#15242);
#8176=LINE('',#200996,#15243);
#8177=LINE('',#201000,#15244);
#8178=LINE('',#201001,#15245);
#8179=LINE('',#201002,#15246);
#8180=LINE('',#201004,#15247);
#8181=LINE('',#201005,#15248);
#8182=LINE('',#201009,#15249);
#8183=LINE('',#201011,#15250);
#8184=LINE('',#201013,#15251);
#8185=LINE('',#201014,#15252);
#8186=LINE('',#201018,#15253);
#8187=LINE('',#201019,#15254);
#8188=LINE('',#201020,#15255);
#8189=LINE('',#201024,#15256);
#8190=LINE('',#201025,#15257);
#8191=LINE('',#201026,#15258);
#8192=LINE('',#201028,#15259);
#8193=LINE('',#201029,#15260);
#8194=LINE('',#201033,#15261);
#8195=LINE('',#201035,#15262);
#8196=LINE('',#201037,#15263);
#8197=LINE('',#201038,#15264);
#8198=LINE('',#201042,#15265);
#8199=LINE('',#201043,#15266);
#8200=LINE('',#201044,#15267);
#8201=LINE('',#201048,#15268);
#8202=LINE('',#201049,#15269);
#8203=LINE('',#201050,#15270);
#8204=LINE('',#201052,#15271);
#8205=LINE('',#201053,#15272);
#8206=LINE('',#201057,#15273);
#8207=LINE('',#201059,#15274);
#8208=LINE('',#201061,#15275);
#8209=LINE('',#201062,#15276);
#8210=LINE('',#201066,#15277);
#8211=LINE('',#201067,#15278);
#8212=LINE('',#201068,#15279);
#8213=LINE('',#201072,#15280);
#8214=LINE('',#201073,#15281);
#8215=LINE('',#201074,#15282);
#8216=LINE('',#201076,#15283);
#8217=LINE('',#201077,#15284);
#8218=LINE('',#201081,#15285);
#8219=LINE('',#201083,#15286);
#8220=LINE('',#201085,#15287);
#8221=LINE('',#201086,#15288);
#8222=LINE('',#201090,#15289);
#8223=LINE('',#201091,#15290);
#8224=LINE('',#201092,#15291);
#8225=LINE('',#201096,#15292);
#8226=LINE('',#201097,#15293);
#8227=LINE('',#201098,#15294);
#8228=LINE('',#201100,#15295);
#8229=LINE('',#201101,#15296);
#8230=LINE('',#201105,#15297);
#8231=LINE('',#201107,#15298);
#8232=LINE('',#201109,#15299);
#8233=LINE('',#201110,#15300);
#8234=LINE('',#201114,#15301);
#8235=LINE('',#201115,#15302);
#8236=LINE('',#201116,#15303);
#8237=LINE('',#201120,#15304);
#8238=LINE('',#201121,#15305);
#8239=LINE('',#201122,#15306);
#8240=LINE('',#201124,#15307);
#8241=LINE('',#201125,#15308);
#8242=LINE('',#201129,#15309);
#8243=LINE('',#201131,#15310);
#8244=LINE('',#201133,#15311);
#8245=LINE('',#201134,#15312);
#8246=LINE('',#201138,#15313);
#8247=LINE('',#201139,#15314);
#8248=LINE('',#201140,#15315);
#8249=LINE('',#201144,#15316);
#8250=LINE('',#201145,#15317);
#8251=LINE('',#201146,#15318);
#8252=LINE('',#201148,#15319);
#8253=LINE('',#201149,#15320);
#8254=LINE('',#201153,#15321);
#8255=LINE('',#201155,#15322);
#8256=LINE('',#201157,#15323);
#8257=LINE('',#201158,#15324);
#8258=LINE('',#201162,#15325);
#8259=LINE('',#201163,#15326);
#8260=LINE('',#201164,#15327);
#8261=LINE('',#201168,#15328);
#8262=LINE('',#201169,#15329);
#8263=LINE('',#201170,#15330);
#8264=LINE('',#201172,#15331);
#8265=LINE('',#201173,#15332);
#8266=LINE('',#201177,#15333);
#8267=LINE('',#201179,#15334);
#8268=LINE('',#201181,#15335);
#8269=LINE('',#201182,#15336);
#8270=LINE('',#201186,#15337);
#8271=LINE('',#201187,#15338);
#8272=LINE('',#201188,#15339);
#8273=LINE('',#201192,#15340);
#8274=LINE('',#201193,#15341);
#8275=LINE('',#201194,#15342);
#8276=LINE('',#201196,#15343);
#8277=LINE('',#201197,#15344);
#8278=LINE('',#201201,#15345);
#8279=LINE('',#201203,#15346);
#8280=LINE('',#201205,#15347);
#8281=LINE('',#201206,#15348);
#8282=LINE('',#201210,#15349);
#8283=LINE('',#201211,#15350);
#8284=LINE('',#201212,#15351);
#8285=LINE('',#201216,#15352);
#8286=LINE('',#201217,#15353);
#8287=LINE('',#201218,#15354);
#8288=LINE('',#201220,#15355);
#8289=LINE('',#201221,#15356);
#8290=LINE('',#201225,#15357);
#8291=LINE('',#201227,#15358);
#8292=LINE('',#201229,#15359);
#8293=LINE('',#201230,#15360);
#8294=LINE('',#201234,#15361);
#8295=LINE('',#201235,#15362);
#8296=LINE('',#201236,#15363);
#8297=LINE('',#201240,#15364);
#8298=LINE('',#201241,#15365);
#8299=LINE('',#201242,#15366);
#8300=LINE('',#201244,#15367);
#8301=LINE('',#201245,#15368);
#8302=LINE('',#201249,#15369);
#8303=LINE('',#201251,#15370);
#8304=LINE('',#201253,#15371);
#8305=LINE('',#201254,#15372);
#8306=LINE('',#201258,#15373);
#8307=LINE('',#201259,#15374);
#8308=LINE('',#201260,#15375);
#8309=LINE('',#201264,#15376);
#8310=LINE('',#201265,#15377);
#8311=LINE('',#201266,#15378);
#8312=LINE('',#201268,#15379);
#8313=LINE('',#201269,#15380);
#8314=LINE('',#201273,#15381);
#8315=LINE('',#201275,#15382);
#8316=LINE('',#201277,#15383);
#8317=LINE('',#201278,#15384);
#8318=LINE('',#201282,#15385);
#8319=LINE('',#201283,#15386);
#8320=LINE('',#201284,#15387);
#8321=LINE('',#201288,#15388);
#8322=LINE('',#201289,#15389);
#8323=LINE('',#201290,#15390);
#8324=LINE('',#201292,#15391);
#8325=LINE('',#201293,#15392);
#8326=LINE('',#201297,#15393);
#8327=LINE('',#201299,#15394);
#8328=LINE('',#201301,#15395);
#8329=LINE('',#201302,#15396);
#8330=LINE('',#201306,#15397);
#8331=LINE('',#201307,#15398);
#8332=LINE('',#201308,#15399);
#8333=LINE('',#201312,#15400);
#8334=LINE('',#201313,#15401);
#8335=LINE('',#201314,#15402);
#8336=LINE('',#201316,#15403);
#8337=LINE('',#201317,#15404);
#8338=LINE('',#201321,#15405);
#8339=LINE('',#201323,#15406);
#8340=LINE('',#201325,#15407);
#8341=LINE('',#201326,#15408);
#8342=LINE('',#201330,#15409);
#8343=LINE('',#201331,#15410);
#8344=LINE('',#201332,#15411);
#8345=LINE('',#201336,#15412);
#8346=LINE('',#201337,#15413);
#8347=LINE('',#201338,#15414);
#8348=LINE('',#201340,#15415);
#8349=LINE('',#201341,#15416);
#8350=LINE('',#201345,#15417);
#8351=LINE('',#201347,#15418);
#8352=LINE('',#201349,#15419);
#8353=LINE('',#201350,#15420);
#8354=LINE('',#201354,#15421);
#8355=LINE('',#201355,#15422);
#8356=LINE('',#201356,#15423);
#8357=LINE('',#201360,#15424);
#8358=LINE('',#201361,#15425);
#8359=LINE('',#201362,#15426);
#8360=LINE('',#201364,#15427);
#8361=LINE('',#201365,#15428);
#8362=LINE('',#201369,#15429);
#8363=LINE('',#201371,#15430);
#8364=LINE('',#201373,#15431);
#8365=LINE('',#201374,#15432);
#8366=LINE('',#201378,#15433);
#8367=LINE('',#201379,#15434);
#8368=LINE('',#201380,#15435);
#8369=LINE('',#201384,#15436);
#8370=LINE('',#201385,#15437);
#8371=LINE('',#201386,#15438);
#8372=LINE('',#201388,#15439);
#8373=LINE('',#201389,#15440);
#8374=LINE('',#201393,#15441);
#8375=LINE('',#201395,#15442);
#8376=LINE('',#201397,#15443);
#8377=LINE('',#201398,#15444);
#8378=LINE('',#201402,#15445);
#8379=LINE('',#201403,#15446);
#8380=LINE('',#201404,#15447);
#8381=LINE('',#201408,#15448);
#8382=LINE('',#201409,#15449);
#8383=LINE('',#201410,#15450);
#8384=LINE('',#201412,#15451);
#8385=LINE('',#201413,#15452);
#8386=LINE('',#201417,#15453);
#8387=LINE('',#201419,#15454);
#8388=LINE('',#201421,#15455);
#8389=LINE('',#201422,#15456);
#8390=LINE('',#201426,#15457);
#8391=LINE('',#201427,#15458);
#8392=LINE('',#201428,#15459);
#8393=LINE('',#201432,#15460);
#8394=LINE('',#201433,#15461);
#8395=LINE('',#201434,#15462);
#8396=LINE('',#201436,#15463);
#8397=LINE('',#201437,#15464);
#8398=LINE('',#201441,#15465);
#8399=LINE('',#201443,#15466);
#8400=LINE('',#201445,#15467);
#8401=LINE('',#201446,#15468);
#8402=LINE('',#201450,#15469);
#8403=LINE('',#201451,#15470);
#8404=LINE('',#201452,#15471);
#8405=LINE('',#201456,#15472);
#8406=LINE('',#201457,#15473);
#8407=LINE('',#201458,#15474);
#8408=LINE('',#201460,#15475);
#8409=LINE('',#201461,#15476);
#8410=LINE('',#201465,#15477);
#8411=LINE('',#201467,#15478);
#8412=LINE('',#201469,#15479);
#8413=LINE('',#201470,#15480);
#8414=LINE('',#201474,#15481);
#8415=LINE('',#201475,#15482);
#8416=LINE('',#201476,#15483);
#8417=LINE('',#201480,#15484);
#8418=LINE('',#201481,#15485);
#8419=LINE('',#201482,#15486);
#8420=LINE('',#201484,#15487);
#8421=LINE('',#201485,#15488);
#8422=LINE('',#201489,#15489);
#8423=LINE('',#201491,#15490);
#8424=LINE('',#201493,#15491);
#8425=LINE('',#201494,#15492);
#8426=LINE('',#201498,#15493);
#8427=LINE('',#201499,#15494);
#8428=LINE('',#201500,#15495);
#8429=LINE('',#201504,#15496);
#8430=LINE('',#201505,#15497);
#8431=LINE('',#201506,#15498);
#8432=LINE('',#201508,#15499);
#8433=LINE('',#201509,#15500);
#8434=LINE('',#201513,#15501);
#8435=LINE('',#201515,#15502);
#8436=LINE('',#201517,#15503);
#8437=LINE('',#201518,#15504);
#8438=LINE('',#201522,#15505);
#8439=LINE('',#201523,#15506);
#8440=LINE('',#201524,#15507);
#8441=LINE('',#201528,#15508);
#8442=LINE('',#201529,#15509);
#8443=LINE('',#201530,#15510);
#8444=LINE('',#201532,#15511);
#8445=LINE('',#201533,#15512);
#8446=LINE('',#201537,#15513);
#8447=LINE('',#201539,#15514);
#8448=LINE('',#201541,#15515);
#8449=LINE('',#201542,#15516);
#8450=LINE('',#201546,#15517);
#8451=LINE('',#201547,#15518);
#8452=LINE('',#201548,#15519);
#8453=LINE('',#201552,#15520);
#8454=LINE('',#201553,#15521);
#8455=LINE('',#201554,#15522);
#8456=LINE('',#201556,#15523);
#8457=LINE('',#201557,#15524);
#8458=LINE('',#201561,#15525);
#8459=LINE('',#201563,#15526);
#8460=LINE('',#201565,#15527);
#8461=LINE('',#201566,#15528);
#8462=LINE('',#201570,#15529);
#8463=LINE('',#201571,#15530);
#8464=LINE('',#201572,#15531);
#8465=LINE('',#201576,#15532);
#8466=LINE('',#201577,#15533);
#8467=LINE('',#201578,#15534);
#8468=LINE('',#201580,#15535);
#8469=LINE('',#201581,#15536);
#8470=LINE('',#201585,#15537);
#8471=LINE('',#201587,#15538);
#8472=LINE('',#201589,#15539);
#8473=LINE('',#201590,#15540);
#8474=LINE('',#201594,#15541);
#8475=LINE('',#201595,#15542);
#8476=LINE('',#201596,#15543);
#8477=LINE('',#201600,#15544);
#8478=LINE('',#201601,#15545);
#8479=LINE('',#201602,#15546);
#8480=LINE('',#201604,#15547);
#8481=LINE('',#201605,#15548);
#8482=LINE('',#201609,#15549);
#8483=LINE('',#201611,#15550);
#8484=LINE('',#201613,#15551);
#8485=LINE('',#201614,#15552);
#8486=LINE('',#201618,#15553);
#8487=LINE('',#201619,#15554);
#8488=LINE('',#201620,#15555);
#8489=LINE('',#201624,#15556);
#8490=LINE('',#201625,#15557);
#8491=LINE('',#201626,#15558);
#8492=LINE('',#201628,#15559);
#8493=LINE('',#201629,#15560);
#8494=LINE('',#201633,#15561);
#8495=LINE('',#201635,#15562);
#8496=LINE('',#201637,#15563);
#8497=LINE('',#201638,#15564);
#8498=LINE('',#201642,#15565);
#8499=LINE('',#201643,#15566);
#8500=LINE('',#201644,#15567);
#8501=LINE('',#201648,#15568);
#8502=LINE('',#201649,#15569);
#8503=LINE('',#201650,#15570);
#8504=LINE('',#201652,#15571);
#8505=LINE('',#201653,#15572);
#8506=LINE('',#201657,#15573);
#8507=LINE('',#201659,#15574);
#8508=LINE('',#201661,#15575);
#8509=LINE('',#201662,#15576);
#8510=LINE('',#201666,#15577);
#8511=LINE('',#201667,#15578);
#8512=LINE('',#201668,#15579);
#8513=LINE('',#201672,#15580);
#8514=LINE('',#201673,#15581);
#8515=LINE('',#201674,#15582);
#8516=LINE('',#201676,#15583);
#8517=LINE('',#201677,#15584);
#8518=LINE('',#201681,#15585);
#8519=LINE('',#201683,#15586);
#8520=LINE('',#201685,#15587);
#8521=LINE('',#201686,#15588);
#8522=LINE('',#201690,#15589);
#8523=LINE('',#201691,#15590);
#8524=LINE('',#201692,#15591);
#8525=LINE('',#201696,#15592);
#8526=LINE('',#201697,#15593);
#8527=LINE('',#201698,#15594);
#8528=LINE('',#201700,#15595);
#8529=LINE('',#201701,#15596);
#8530=LINE('',#201705,#15597);
#8531=LINE('',#201707,#15598);
#8532=LINE('',#201709,#15599);
#8533=LINE('',#201710,#15600);
#8534=LINE('',#201714,#15601);
#8535=LINE('',#201715,#15602);
#8536=LINE('',#201716,#15603);
#8537=LINE('',#201720,#15604);
#8538=LINE('',#201721,#15605);
#8539=LINE('',#201722,#15606);
#8540=LINE('',#201724,#15607);
#8541=LINE('',#201725,#15608);
#8542=LINE('',#201729,#15609);
#8543=LINE('',#201731,#15610);
#8544=LINE('',#201733,#15611);
#8545=LINE('',#201734,#15612);
#8546=LINE('',#201738,#15613);
#8547=LINE('',#201739,#15614);
#8548=LINE('',#201740,#15615);
#8549=LINE('',#201744,#15616);
#8550=LINE('',#201745,#15617);
#8551=LINE('',#201746,#15618);
#8552=LINE('',#201748,#15619);
#8553=LINE('',#201749,#15620);
#8554=LINE('',#201753,#15621);
#8555=LINE('',#201755,#15622);
#8556=LINE('',#201757,#15623);
#8557=LINE('',#201758,#15624);
#8558=LINE('',#201762,#15625);
#8559=LINE('',#201763,#15626);
#8560=LINE('',#201764,#15627);
#8561=LINE('',#201768,#15628);
#8562=LINE('',#201769,#15629);
#8563=LINE('',#201770,#15630);
#8564=LINE('',#201772,#15631);
#8565=LINE('',#201773,#15632);
#8566=LINE('',#201777,#15633);
#8567=LINE('',#201779,#15634);
#8568=LINE('',#201781,#15635);
#8569=LINE('',#201782,#15636);
#8570=LINE('',#201786,#15637);
#8571=LINE('',#201787,#15638);
#8572=LINE('',#201788,#15639);
#8573=LINE('',#201792,#15640);
#8574=LINE('',#201793,#15641);
#8575=LINE('',#201794,#15642);
#8576=LINE('',#201796,#15643);
#8577=LINE('',#201797,#15644);
#8578=LINE('',#201801,#15645);
#8579=LINE('',#201803,#15646);
#8580=LINE('',#201805,#15647);
#8581=LINE('',#201806,#15648);
#8582=LINE('',#201810,#15649);
#8583=LINE('',#201811,#15650);
#8584=LINE('',#201812,#15651);
#8585=LINE('',#201816,#15652);
#8586=LINE('',#201817,#15653);
#8587=LINE('',#201818,#15654);
#8588=LINE('',#201820,#15655);
#8589=LINE('',#201821,#15656);
#8590=LINE('',#201825,#15657);
#8591=LINE('',#201827,#15658);
#8592=LINE('',#201829,#15659);
#8593=LINE('',#201830,#15660);
#8594=LINE('',#201834,#15661);
#8595=LINE('',#201835,#15662);
#8596=LINE('',#201836,#15663);
#8597=LINE('',#201840,#15664);
#8598=LINE('',#201841,#15665);
#8599=LINE('',#201842,#15666);
#8600=LINE('',#201844,#15667);
#8601=LINE('',#201845,#15668);
#8602=LINE('',#201849,#15669);
#8603=LINE('',#201851,#15670);
#8604=LINE('',#201853,#15671);
#8605=LINE('',#201854,#15672);
#8606=LINE('',#201858,#15673);
#8607=LINE('',#201859,#15674);
#8608=LINE('',#201860,#15675);
#8609=LINE('',#201864,#15676);
#8610=LINE('',#201865,#15677);
#8611=LINE('',#201866,#15678);
#8612=LINE('',#201868,#15679);
#8613=LINE('',#201869,#15680);
#8614=LINE('',#201873,#15681);
#8615=LINE('',#201875,#15682);
#8616=LINE('',#201877,#15683);
#8617=LINE('',#201878,#15684);
#8618=LINE('',#201882,#15685);
#8619=LINE('',#201883,#15686);
#8620=LINE('',#201884,#15687);
#8621=LINE('',#201888,#15688);
#8622=LINE('',#201889,#15689);
#8623=LINE('',#201890,#15690);
#8624=LINE('',#201892,#15691);
#8625=LINE('',#201893,#15692);
#8626=LINE('',#201897,#15693);
#8627=LINE('',#201899,#15694);
#8628=LINE('',#201901,#15695);
#8629=LINE('',#201902,#15696);
#8630=LINE('',#201906,#15697);
#8631=LINE('',#201907,#15698);
#8632=LINE('',#201908,#15699);
#8633=LINE('',#201912,#15700);
#8634=LINE('',#201913,#15701);
#8635=LINE('',#201914,#15702);
#8636=LINE('',#201916,#15703);
#8637=LINE('',#201917,#15704);
#8638=LINE('',#201921,#15705);
#8639=LINE('',#201923,#15706);
#8640=LINE('',#201925,#15707);
#8641=LINE('',#201926,#15708);
#8642=LINE('',#201930,#15709);
#8643=LINE('',#201931,#15710);
#8644=LINE('',#201932,#15711);
#8645=LINE('',#201936,#15712);
#8646=LINE('',#201937,#15713);
#8647=LINE('',#201938,#15714);
#8648=LINE('',#201940,#15715);
#8649=LINE('',#201941,#15716);
#8650=LINE('',#201945,#15717);
#8651=LINE('',#201947,#15718);
#8652=LINE('',#201949,#15719);
#8653=LINE('',#201950,#15720);
#8654=LINE('',#201954,#15721);
#8655=LINE('',#201955,#15722);
#8656=LINE('',#201956,#15723);
#8657=LINE('',#201960,#15724);
#8658=LINE('',#201961,#15725);
#8659=LINE('',#201962,#15726);
#8660=LINE('',#201964,#15727);
#8661=LINE('',#201965,#15728);
#8662=LINE('',#201969,#15729);
#8663=LINE('',#201971,#15730);
#8664=LINE('',#201973,#15731);
#8665=LINE('',#201974,#15732);
#8666=LINE('',#201978,#15733);
#8667=LINE('',#201979,#15734);
#8668=LINE('',#201980,#15735);
#8669=LINE('',#201984,#15736);
#8670=LINE('',#201985,#15737);
#8671=LINE('',#201986,#15738);
#8672=LINE('',#201988,#15739);
#8673=LINE('',#201989,#15740);
#8674=LINE('',#201993,#15741);
#8675=LINE('',#201995,#15742);
#8676=LINE('',#201997,#15743);
#8677=LINE('',#201998,#15744);
#8678=LINE('',#202002,#15745);
#8679=LINE('',#202003,#15746);
#8680=LINE('',#202004,#15747);
#8681=LINE('',#202008,#15748);
#8682=LINE('',#202009,#15749);
#8683=LINE('',#202010,#15750);
#8684=LINE('',#202012,#15751);
#8685=LINE('',#202013,#15752);
#8686=LINE('',#202017,#15753);
#8687=LINE('',#202019,#15754);
#8688=LINE('',#202021,#15755);
#8689=LINE('',#202022,#15756);
#8690=LINE('',#202026,#15757);
#8691=LINE('',#202027,#15758);
#8692=LINE('',#202028,#15759);
#8693=LINE('',#202032,#15760);
#8694=LINE('',#202033,#15761);
#8695=LINE('',#202034,#15762);
#8696=LINE('',#202036,#15763);
#8697=LINE('',#202037,#15764);
#8698=LINE('',#202041,#15765);
#8699=LINE('',#202043,#15766);
#8700=LINE('',#202045,#15767);
#8701=LINE('',#202046,#15768);
#8702=LINE('',#202050,#15769);
#8703=LINE('',#202051,#15770);
#8704=LINE('',#202052,#15771);
#8705=LINE('',#202056,#15772);
#8706=LINE('',#202057,#15773);
#8707=LINE('',#202058,#15774);
#8708=LINE('',#202060,#15775);
#8709=LINE('',#202061,#15776);
#8710=LINE('',#202065,#15777);
#8711=LINE('',#202067,#15778);
#8712=LINE('',#202069,#15779);
#8713=LINE('',#202070,#15780);
#8714=LINE('',#202074,#15781);
#8715=LINE('',#202075,#15782);
#8716=LINE('',#202076,#15783);
#8717=LINE('',#202080,#15784);
#8718=LINE('',#202081,#15785);
#8719=LINE('',#202082,#15786);
#8720=LINE('',#202084,#15787);
#8721=LINE('',#202085,#15788);
#8722=LINE('',#202089,#15789);
#8723=LINE('',#202091,#15790);
#8724=LINE('',#202093,#15791);
#8725=LINE('',#202094,#15792);
#8726=LINE('',#202098,#15793);
#8727=LINE('',#202099,#15794);
#8728=LINE('',#202100,#15795);
#8729=LINE('',#202104,#15796);
#8730=LINE('',#202105,#15797);
#8731=LINE('',#202106,#15798);
#8732=LINE('',#202108,#15799);
#8733=LINE('',#202109,#15800);
#8734=LINE('',#202113,#15801);
#8735=LINE('',#202115,#15802);
#8736=LINE('',#202117,#15803);
#8737=LINE('',#202118,#15804);
#8738=LINE('',#202122,#15805);
#8739=LINE('',#202123,#15806);
#8740=LINE('',#202124,#15807);
#8741=LINE('',#202128,#15808);
#8742=LINE('',#202129,#15809);
#8743=LINE('',#202130,#15810);
#8744=LINE('',#202132,#15811);
#8745=LINE('',#202133,#15812);
#8746=LINE('',#202137,#15813);
#8747=LINE('',#202139,#15814);
#8748=LINE('',#202141,#15815);
#8749=LINE('',#202142,#15816);
#8750=LINE('',#202146,#15817);
#8751=LINE('',#202147,#15818);
#8752=LINE('',#202148,#15819);
#8753=LINE('',#202152,#15820);
#8754=LINE('',#202153,#15821);
#8755=LINE('',#202154,#15822);
#8756=LINE('',#202156,#15823);
#8757=LINE('',#202157,#15824);
#8758=LINE('',#202161,#15825);
#8759=LINE('',#202163,#15826);
#8760=LINE('',#202165,#15827);
#8761=LINE('',#202166,#15828);
#8762=LINE('',#202170,#15829);
#8763=LINE('',#202171,#15830);
#8764=LINE('',#202172,#15831);
#8765=LINE('',#202176,#15832);
#8766=LINE('',#202177,#15833);
#8767=LINE('',#202178,#15834);
#8768=LINE('',#202180,#15835);
#8769=LINE('',#202181,#15836);
#8770=LINE('',#202185,#15837);
#8771=LINE('',#202187,#15838);
#8772=LINE('',#202189,#15839);
#8773=LINE('',#202190,#15840);
#8774=LINE('',#202194,#15841);
#8775=LINE('',#202195,#15842);
#8776=LINE('',#202196,#15843);
#8777=LINE('',#202200,#15844);
#8778=LINE('',#202201,#15845);
#8779=LINE('',#202202,#15846);
#8780=LINE('',#202204,#15847);
#8781=LINE('',#202205,#15848);
#8782=LINE('',#202209,#15849);
#8783=LINE('',#202211,#15850);
#8784=LINE('',#202213,#15851);
#8785=LINE('',#202214,#15852);
#8786=LINE('',#202218,#15853);
#8787=LINE('',#202219,#15854);
#8788=LINE('',#202220,#15855);
#8789=LINE('',#202224,#15856);
#8790=LINE('',#202225,#15857);
#8791=LINE('',#202226,#15858);
#8792=LINE('',#202228,#15859);
#8793=LINE('',#202229,#15860);
#8794=LINE('',#202233,#15861);
#8795=LINE('',#202235,#15862);
#8796=LINE('',#202237,#15863);
#8797=LINE('',#202238,#15864);
#8798=LINE('',#202242,#15865);
#8799=LINE('',#202243,#15866);
#8800=LINE('',#202244,#15867);
#8801=LINE('',#202248,#15868);
#8802=LINE('',#202249,#15869);
#8803=LINE('',#202250,#15870);
#8804=LINE('',#202252,#15871);
#8805=LINE('',#202253,#15872);
#8806=LINE('',#202257,#15873);
#8807=LINE('',#202259,#15874);
#8808=LINE('',#202261,#15875);
#8809=LINE('',#202262,#15876);
#8810=LINE('',#202266,#15877);
#8811=LINE('',#202267,#15878);
#8812=LINE('',#202268,#15879);
#8813=LINE('',#202272,#15880);
#8814=LINE('',#202273,#15881);
#8815=LINE('',#202274,#15882);
#8816=LINE('',#202276,#15883);
#8817=LINE('',#202277,#15884);
#8818=LINE('',#202281,#15885);
#8819=LINE('',#202283,#15886);
#8820=LINE('',#202285,#15887);
#8821=LINE('',#202286,#15888);
#8822=LINE('',#202290,#15889);
#8823=LINE('',#202291,#15890);
#8824=LINE('',#202292,#15891);
#8825=LINE('',#202296,#15892);
#8826=LINE('',#202297,#15893);
#8827=LINE('',#202298,#15894);
#8828=LINE('',#202300,#15895);
#8829=LINE('',#202301,#15896);
#8830=LINE('',#202305,#15897);
#8831=LINE('',#202307,#15898);
#8832=LINE('',#202309,#15899);
#8833=LINE('',#202310,#15900);
#8834=LINE('',#202314,#15901);
#8835=LINE('',#202315,#15902);
#8836=LINE('',#202316,#15903);
#8837=LINE('',#202320,#15904);
#8838=LINE('',#202321,#15905);
#8839=LINE('',#202322,#15906);
#8840=LINE('',#202324,#15907);
#8841=LINE('',#202325,#15908);
#8842=LINE('',#202329,#15909);
#8843=LINE('',#202331,#15910);
#8844=LINE('',#202333,#15911);
#8845=LINE('',#202334,#15912);
#8846=LINE('',#202338,#15913);
#8847=LINE('',#202339,#15914);
#8848=LINE('',#202340,#15915);
#8849=LINE('',#202344,#15916);
#8850=LINE('',#202345,#15917);
#8851=LINE('',#202346,#15918);
#8852=LINE('',#202348,#15919);
#8853=LINE('',#202349,#15920);
#8854=LINE('',#202353,#15921);
#8855=LINE('',#202355,#15922);
#8856=LINE('',#202357,#15923);
#8857=LINE('',#202358,#15924);
#8858=LINE('',#202362,#15925);
#8859=LINE('',#202363,#15926);
#8860=LINE('',#202364,#15927);
#8861=LINE('',#202368,#15928);
#8862=LINE('',#202369,#15929);
#8863=LINE('',#202370,#15930);
#8864=LINE('',#202372,#15931);
#8865=LINE('',#202373,#15932);
#8866=LINE('',#202377,#15933);
#8867=LINE('',#202379,#15934);
#8868=LINE('',#202381,#15935);
#8869=LINE('',#202382,#15936);
#8870=LINE('',#202386,#15937);
#8871=LINE('',#202387,#15938);
#8872=LINE('',#202388,#15939);
#8873=LINE('',#202392,#15940);
#8874=LINE('',#202393,#15941);
#8875=LINE('',#202394,#15942);
#8876=LINE('',#202396,#15943);
#8877=LINE('',#202397,#15944);
#8878=LINE('',#202401,#15945);
#8879=LINE('',#202403,#15946);
#8880=LINE('',#202405,#15947);
#8881=LINE('',#202406,#15948);
#8882=LINE('',#202410,#15949);
#8883=LINE('',#202411,#15950);
#8884=LINE('',#202412,#15951);
#8885=LINE('',#202416,#15952);
#8886=LINE('',#202417,#15953);
#8887=LINE('',#202418,#15954);
#8888=LINE('',#202420,#15955);
#8889=LINE('',#202421,#15956);
#8890=LINE('',#202425,#15957);
#8891=LINE('',#202427,#15958);
#8892=LINE('',#202429,#15959);
#8893=LINE('',#202430,#15960);
#8894=LINE('',#202434,#15961);
#8895=LINE('',#202435,#15962);
#8896=LINE('',#202436,#15963);
#8897=LINE('',#202440,#15964);
#8898=LINE('',#202441,#15965);
#8899=LINE('',#202442,#15966);
#8900=LINE('',#202444,#15967);
#8901=LINE('',#202445,#15968);
#8902=LINE('',#202449,#15969);
#8903=LINE('',#202451,#15970);
#8904=LINE('',#202453,#15971);
#8905=LINE('',#202454,#15972);
#8906=LINE('',#202458,#15973);
#8907=LINE('',#202459,#15974);
#8908=LINE('',#202460,#15975);
#8909=LINE('',#202464,#15976);
#8910=LINE('',#202465,#15977);
#8911=LINE('',#202466,#15978);
#8912=LINE('',#202468,#15979);
#8913=LINE('',#202469,#15980);
#8914=LINE('',#202473,#15981);
#8915=LINE('',#202475,#15982);
#8916=LINE('',#202477,#15983);
#8917=LINE('',#202478,#15984);
#8918=LINE('',#202482,#15985);
#8919=LINE('',#202483,#15986);
#8920=LINE('',#202484,#15987);
#8921=LINE('',#202488,#15988);
#8922=LINE('',#202489,#15989);
#8923=LINE('',#202490,#15990);
#8924=LINE('',#202492,#15991);
#8925=LINE('',#202493,#15992);
#8926=LINE('',#202497,#15993);
#8927=LINE('',#202499,#15994);
#8928=LINE('',#202501,#15995);
#8929=LINE('',#202502,#15996);
#8930=LINE('',#202506,#15997);
#8931=LINE('',#202507,#15998);
#8932=LINE('',#202508,#15999);
#8933=LINE('',#202512,#16000);
#8934=LINE('',#202513,#16001);
#8935=LINE('',#202514,#16002);
#8936=LINE('',#202516,#16003);
#8937=LINE('',#202517,#16004);
#8938=LINE('',#202521,#16005);
#8939=LINE('',#202523,#16006);
#8940=LINE('',#202525,#16007);
#8941=LINE('',#202526,#16008);
#8942=LINE('',#202530,#16009);
#8943=LINE('',#202531,#16010);
#8944=LINE('',#202532,#16011);
#8945=LINE('',#202536,#16012);
#8946=LINE('',#202537,#16013);
#8947=LINE('',#202538,#16014);
#8948=LINE('',#202540,#16015);
#8949=LINE('',#202541,#16016);
#8950=LINE('',#202545,#16017);
#8951=LINE('',#202547,#16018);
#8952=LINE('',#202549,#16019);
#8953=LINE('',#202550,#16020);
#8954=LINE('',#202554,#16021);
#8955=LINE('',#202555,#16022);
#8956=LINE('',#202556,#16023);
#8957=LINE('',#202560,#16024);
#8958=LINE('',#202561,#16025);
#8959=LINE('',#202562,#16026);
#8960=LINE('',#202564,#16027);
#8961=LINE('',#202565,#16028);
#8962=LINE('',#202569,#16029);
#8963=LINE('',#202571,#16030);
#8964=LINE('',#202573,#16031);
#8965=LINE('',#202574,#16032);
#8966=LINE('',#202578,#16033);
#8967=LINE('',#202579,#16034);
#8968=LINE('',#202580,#16035);
#8969=LINE('',#202584,#16036);
#8970=LINE('',#202585,#16037);
#8971=LINE('',#202586,#16038);
#8972=LINE('',#202588,#16039);
#8973=LINE('',#202589,#16040);
#8974=LINE('',#202593,#16041);
#8975=LINE('',#202595,#16042);
#8976=LINE('',#202597,#16043);
#8977=LINE('',#202598,#16044);
#8978=LINE('',#202602,#16045);
#8979=LINE('',#202603,#16046);
#8980=LINE('',#202604,#16047);
#8981=LINE('',#202608,#16048);
#8982=LINE('',#202609,#16049);
#8983=LINE('',#202610,#16050);
#8984=LINE('',#202612,#16051);
#8985=LINE('',#202613,#16052);
#8986=LINE('',#202617,#16053);
#8987=LINE('',#202619,#16054);
#8988=LINE('',#202621,#16055);
#8989=LINE('',#202622,#16056);
#8990=LINE('',#202626,#16057);
#8991=LINE('',#202627,#16058);
#8992=LINE('',#202628,#16059);
#8993=LINE('',#202632,#16060);
#8994=LINE('',#202633,#16061);
#8995=LINE('',#202634,#16062);
#8996=LINE('',#202636,#16063);
#8997=LINE('',#202637,#16064);
#8998=LINE('',#202641,#16065);
#8999=LINE('',#202643,#16066);
#9000=LINE('',#202645,#16067);
#9001=LINE('',#202646,#16068);
#9002=LINE('',#202650,#16069);
#9003=LINE('',#202651,#16070);
#9004=LINE('',#202652,#16071);
#9005=LINE('',#202656,#16072);
#9006=LINE('',#202657,#16073);
#9007=LINE('',#202658,#16074);
#9008=LINE('',#202660,#16075);
#9009=LINE('',#202661,#16076);
#9010=LINE('',#202665,#16077);
#9011=LINE('',#202667,#16078);
#9012=LINE('',#202669,#16079);
#9013=LINE('',#202670,#16080);
#9014=LINE('',#202674,#16081);
#9015=LINE('',#202675,#16082);
#9016=LINE('',#202676,#16083);
#9017=LINE('',#202680,#16084);
#9018=LINE('',#202681,#16085);
#9019=LINE('',#202682,#16086);
#9020=LINE('',#202684,#16087);
#9021=LINE('',#202685,#16088);
#9022=LINE('',#202689,#16089);
#9023=LINE('',#202691,#16090);
#9024=LINE('',#202693,#16091);
#9025=LINE('',#202694,#16092);
#9026=LINE('',#202698,#16093);
#9027=LINE('',#202699,#16094);
#9028=LINE('',#202700,#16095);
#9029=LINE('',#202704,#16096);
#9030=LINE('',#202705,#16097);
#9031=LINE('',#202706,#16098);
#9032=LINE('',#202708,#16099);
#9033=LINE('',#202709,#16100);
#9034=LINE('',#202713,#16101);
#9035=LINE('',#202715,#16102);
#9036=LINE('',#202717,#16103);
#9037=LINE('',#202718,#16104);
#9038=LINE('',#202722,#16105);
#9039=LINE('',#202723,#16106);
#9040=LINE('',#202724,#16107);
#9041=LINE('',#202728,#16108);
#9042=LINE('',#202729,#16109);
#9043=LINE('',#202730,#16110);
#9044=LINE('',#202732,#16111);
#9045=LINE('',#202733,#16112);
#9046=LINE('',#202737,#16113);
#9047=LINE('',#202739,#16114);
#9048=LINE('',#202741,#16115);
#9049=LINE('',#202742,#16116);
#9050=LINE('',#202746,#16117);
#9051=LINE('',#202747,#16118);
#9052=LINE('',#202748,#16119);
#9053=LINE('',#202752,#16120);
#9054=LINE('',#202753,#16121);
#9055=LINE('',#202754,#16122);
#9056=LINE('',#202756,#16123);
#9057=LINE('',#202757,#16124);
#9058=LINE('',#202761,#16125);
#9059=LINE('',#202763,#16126);
#9060=LINE('',#202765,#16127);
#9061=LINE('',#202766,#16128);
#9062=LINE('',#202770,#16129);
#9063=LINE('',#202771,#16130);
#9064=LINE('',#202772,#16131);
#9065=LINE('',#202776,#16132);
#9066=LINE('',#202777,#16133);
#9067=LINE('',#202778,#16134);
#9068=LINE('',#202780,#16135);
#9069=LINE('',#202781,#16136);
#9070=LINE('',#202785,#16137);
#9071=LINE('',#202787,#16138);
#9072=LINE('',#202789,#16139);
#9073=LINE('',#202790,#16140);
#9074=LINE('',#202794,#16141);
#9075=LINE('',#202795,#16142);
#9076=LINE('',#202796,#16143);
#9077=LINE('',#202800,#16144);
#9078=LINE('',#202801,#16145);
#9079=LINE('',#202802,#16146);
#9080=LINE('',#202804,#16147);
#9081=LINE('',#202805,#16148);
#9082=LINE('',#202809,#16149);
#9083=LINE('',#202811,#16150);
#9084=LINE('',#202813,#16151);
#9085=LINE('',#202814,#16152);
#9086=LINE('',#202818,#16153);
#9087=LINE('',#202819,#16154);
#9088=LINE('',#202820,#16155);
#9089=LINE('',#202824,#16156);
#9090=LINE('',#202825,#16157);
#9091=LINE('',#202826,#16158);
#9092=LINE('',#202828,#16159);
#9093=LINE('',#202829,#16160);
#9094=LINE('',#202833,#16161);
#9095=LINE('',#202835,#16162);
#9096=LINE('',#202837,#16163);
#9097=LINE('',#202838,#16164);
#9098=LINE('',#202842,#16165);
#9099=LINE('',#202843,#16166);
#9100=LINE('',#202844,#16167);
#9101=LINE('',#202848,#16168);
#9102=LINE('',#202849,#16169);
#9103=LINE('',#202850,#16170);
#9104=LINE('',#202852,#16171);
#9105=LINE('',#202853,#16172);
#9106=LINE('',#202857,#16173);
#9107=LINE('',#202859,#16174);
#9108=LINE('',#202861,#16175);
#9109=LINE('',#202862,#16176);
#9110=LINE('',#202866,#16177);
#9111=LINE('',#202867,#16178);
#9112=LINE('',#202868,#16179);
#9113=LINE('',#202872,#16180);
#9114=LINE('',#202873,#16181);
#9115=LINE('',#202874,#16182);
#9116=LINE('',#202876,#16183);
#9117=LINE('',#202877,#16184);
#9118=LINE('',#202881,#16185);
#9119=LINE('',#202883,#16186);
#9120=LINE('',#202885,#16187);
#9121=LINE('',#202886,#16188);
#9122=LINE('',#202890,#16189);
#9123=LINE('',#202891,#16190);
#9124=LINE('',#202892,#16191);
#9125=LINE('',#202896,#16192);
#9126=LINE('',#202897,#16193);
#9127=LINE('',#202898,#16194);
#9128=LINE('',#202900,#16195);
#9129=LINE('',#202901,#16196);
#9130=LINE('',#202905,#16197);
#9131=LINE('',#202907,#16198);
#9132=LINE('',#202909,#16199);
#9133=LINE('',#202910,#16200);
#9134=LINE('',#202914,#16201);
#9135=LINE('',#202915,#16202);
#9136=LINE('',#202916,#16203);
#9137=LINE('',#202920,#16204);
#9138=LINE('',#202921,#16205);
#9139=LINE('',#202922,#16206);
#9140=LINE('',#202924,#16207);
#9141=LINE('',#202925,#16208);
#9142=LINE('',#202929,#16209);
#9143=LINE('',#202931,#16210);
#9144=LINE('',#202933,#16211);
#9145=LINE('',#202934,#16212);
#9146=LINE('',#202938,#16213);
#9147=LINE('',#202939,#16214);
#9148=LINE('',#202940,#16215);
#9149=LINE('',#202944,#16216);
#9150=LINE('',#202945,#16217);
#9151=LINE('',#202946,#16218);
#9152=LINE('',#202948,#16219);
#9153=LINE('',#202949,#16220);
#9154=LINE('',#202953,#16221);
#9155=LINE('',#202955,#16222);
#9156=LINE('',#202957,#16223);
#9157=LINE('',#202958,#16224);
#9158=LINE('',#202962,#16225);
#9159=LINE('',#202963,#16226);
#9160=LINE('',#202964,#16227);
#9161=LINE('',#202968,#16228);
#9162=LINE('',#202969,#16229);
#9163=LINE('',#202970,#16230);
#9164=LINE('',#202972,#16231);
#9165=LINE('',#202973,#16232);
#9166=LINE('',#202977,#16233);
#9167=LINE('',#202979,#16234);
#9168=LINE('',#202981,#16235);
#9169=LINE('',#202982,#16236);
#9170=LINE('',#202986,#16237);
#9171=LINE('',#202987,#16238);
#9172=LINE('',#202988,#16239);
#9173=LINE('',#202992,#16240);
#9174=LINE('',#202993,#16241);
#9175=LINE('',#202994,#16242);
#9176=LINE('',#202996,#16243);
#9177=LINE('',#202997,#16244);
#9178=LINE('',#203001,#16245);
#9179=LINE('',#203003,#16246);
#9180=LINE('',#203005,#16247);
#9181=LINE('',#203006,#16248);
#9182=LINE('',#203010,#16249);
#9183=LINE('',#203011,#16250);
#9184=LINE('',#203012,#16251);
#9185=LINE('',#203016,#16252);
#9186=LINE('',#203017,#16253);
#9187=LINE('',#203018,#16254);
#9188=LINE('',#203020,#16255);
#9189=LINE('',#203021,#16256);
#9190=LINE('',#203025,#16257);
#9191=LINE('',#203027,#16258);
#9192=LINE('',#203029,#16259);
#9193=LINE('',#203030,#16260);
#9194=LINE('',#203034,#16261);
#9195=LINE('',#203035,#16262);
#9196=LINE('',#203036,#16263);
#9197=LINE('',#203040,#16264);
#9198=LINE('',#203041,#16265);
#9199=LINE('',#203042,#16266);
#9200=LINE('',#203044,#16267);
#9201=LINE('',#203045,#16268);
#9202=LINE('',#203049,#16269);
#9203=LINE('',#203051,#16270);
#9204=LINE('',#203053,#16271);
#9205=LINE('',#203054,#16272);
#9206=LINE('',#203058,#16273);
#9207=LINE('',#203059,#16274);
#9208=LINE('',#203060,#16275);
#9209=LINE('',#203064,#16276);
#9210=LINE('',#203065,#16277);
#9211=LINE('',#203066,#16278);
#9212=LINE('',#203068,#16279);
#9213=LINE('',#203069,#16280);
#9214=LINE('',#203073,#16281);
#9215=LINE('',#203075,#16282);
#9216=LINE('',#203077,#16283);
#9217=LINE('',#203078,#16284);
#9218=LINE('',#203082,#16285);
#9219=LINE('',#203083,#16286);
#9220=LINE('',#203084,#16287);
#9221=LINE('',#203088,#16288);
#9222=LINE('',#203089,#16289);
#9223=LINE('',#203090,#16290);
#9224=LINE('',#203092,#16291);
#9225=LINE('',#203093,#16292);
#9226=LINE('',#203097,#16293);
#9227=LINE('',#203099,#16294);
#9228=LINE('',#203101,#16295);
#9229=LINE('',#203102,#16296);
#9230=LINE('',#203106,#16297);
#9231=LINE('',#203107,#16298);
#9232=LINE('',#203108,#16299);
#9233=LINE('',#203112,#16300);
#9234=LINE('',#203113,#16301);
#9235=LINE('',#203114,#16302);
#9236=LINE('',#203116,#16303);
#9237=LINE('',#203117,#16304);
#9238=LINE('',#203121,#16305);
#9239=LINE('',#203123,#16306);
#9240=LINE('',#203125,#16307);
#9241=LINE('',#203126,#16308);
#9242=LINE('',#203130,#16309);
#9243=LINE('',#203131,#16310);
#9244=LINE('',#203132,#16311);
#9245=LINE('',#203136,#16312);
#9246=LINE('',#203137,#16313);
#9247=LINE('',#203138,#16314);
#9248=LINE('',#203140,#16315);
#9249=LINE('',#203141,#16316);
#9250=LINE('',#203145,#16317);
#9251=LINE('',#203147,#16318);
#9252=LINE('',#203149,#16319);
#9253=LINE('',#203150,#16320);
#9254=LINE('',#203154,#16321);
#9255=LINE('',#203155,#16322);
#9256=LINE('',#203156,#16323);
#9257=LINE('',#203160,#16324);
#9258=LINE('',#203161,#16325);
#9259=LINE('',#203162,#16326);
#9260=LINE('',#203164,#16327);
#9261=LINE('',#203165,#16328);
#9262=LINE('',#203169,#16329);
#9263=LINE('',#203171,#16330);
#9264=LINE('',#203173,#16331);
#9265=LINE('',#203174,#16332);
#9266=LINE('',#203178,#16333);
#9267=LINE('',#203179,#16334);
#9268=LINE('',#203180,#16335);
#9269=LINE('',#203184,#16336);
#9270=LINE('',#203185,#16337);
#9271=LINE('',#203186,#16338);
#9272=LINE('',#203188,#16339);
#9273=LINE('',#203189,#16340);
#9274=LINE('',#203193,#16341);
#9275=LINE('',#203195,#16342);
#9276=LINE('',#203197,#16343);
#9277=LINE('',#203198,#16344);
#9278=LINE('',#203202,#16345);
#9279=LINE('',#203203,#16346);
#9280=LINE('',#203204,#16347);
#9281=LINE('',#203208,#16348);
#9282=LINE('',#203209,#16349);
#9283=LINE('',#203210,#16350);
#9284=LINE('',#203212,#16351);
#9285=LINE('',#203213,#16352);
#9286=LINE('',#203217,#16353);
#9287=LINE('',#203219,#16354);
#9288=LINE('',#203221,#16355);
#9289=LINE('',#203222,#16356);
#9290=LINE('',#203226,#16357);
#9291=LINE('',#203227,#16358);
#9292=LINE('',#203228,#16359);
#9293=LINE('',#203232,#16360);
#9294=LINE('',#203233,#16361);
#9295=LINE('',#203234,#16362);
#9296=LINE('',#203236,#16363);
#9297=LINE('',#203237,#16364);
#9298=LINE('',#203241,#16365);
#9299=LINE('',#203243,#16366);
#9300=LINE('',#203245,#16367);
#9301=LINE('',#203246,#16368);
#9302=LINE('',#203250,#16369);
#9303=LINE('',#203251,#16370);
#9304=LINE('',#203252,#16371);
#9305=LINE('',#203256,#16372);
#9306=LINE('',#203257,#16373);
#9307=LINE('',#203258,#16374);
#9308=LINE('',#203260,#16375);
#9309=LINE('',#203261,#16376);
#9310=LINE('',#203265,#16377);
#9311=LINE('',#203267,#16378);
#9312=LINE('',#203269,#16379);
#9313=LINE('',#203270,#16380);
#9314=LINE('',#203274,#16381);
#9315=LINE('',#203275,#16382);
#9316=LINE('',#203276,#16383);
#9317=LINE('',#203280,#16384);
#9318=LINE('',#203281,#16385);
#9319=LINE('',#203282,#16386);
#9320=LINE('',#203284,#16387);
#9321=LINE('',#203285,#16388);
#9322=LINE('',#203289,#16389);
#9323=LINE('',#203291,#16390);
#9324=LINE('',#203293,#16391);
#9325=LINE('',#203294,#16392);
#9326=LINE('',#203298,#16393);
#9327=LINE('',#203299,#16394);
#9328=LINE('',#203300,#16395);
#9329=LINE('',#203304,#16396);
#9330=LINE('',#203305,#16397);
#9331=LINE('',#203306,#16398);
#9332=LINE('',#203308,#16399);
#9333=LINE('',#203309,#16400);
#9334=LINE('',#203313,#16401);
#9335=LINE('',#203315,#16402);
#9336=LINE('',#203317,#16403);
#9337=LINE('',#203318,#16404);
#9338=LINE('',#203322,#16405);
#9339=LINE('',#203323,#16406);
#9340=LINE('',#203324,#16407);
#9341=LINE('',#203328,#16408);
#9342=LINE('',#203329,#16409);
#9343=LINE('',#203330,#16410);
#9344=LINE('',#203332,#16411);
#9345=LINE('',#203333,#16412);
#9346=LINE('',#203337,#16413);
#9347=LINE('',#203339,#16414);
#9348=LINE('',#203341,#16415);
#9349=LINE('',#203342,#16416);
#9350=LINE('',#203346,#16417);
#9351=LINE('',#203347,#16418);
#9352=LINE('',#203348,#16419);
#9353=LINE('',#203352,#16420);
#9354=LINE('',#203353,#16421);
#9355=LINE('',#203354,#16422);
#9356=LINE('',#203356,#16423);
#9357=LINE('',#203357,#16424);
#9358=LINE('',#203361,#16425);
#9359=LINE('',#203363,#16426);
#9360=LINE('',#203365,#16427);
#9361=LINE('',#203366,#16428);
#9362=LINE('',#203370,#16429);
#9363=LINE('',#203371,#16430);
#9364=LINE('',#203372,#16431);
#9365=LINE('',#203376,#16432);
#9366=LINE('',#203377,#16433);
#9367=LINE('',#203378,#16434);
#9368=LINE('',#203380,#16435);
#9369=LINE('',#203381,#16436);
#9370=LINE('',#203385,#16437);
#9371=LINE('',#203387,#16438);
#9372=LINE('',#203389,#16439);
#9373=LINE('',#203390,#16440);
#9374=LINE('',#203394,#16441);
#9375=LINE('',#203395,#16442);
#9376=LINE('',#203396,#16443);
#9377=LINE('',#203400,#16444);
#9378=LINE('',#203401,#16445);
#9379=LINE('',#203402,#16446);
#9380=LINE('',#203404,#16447);
#9381=LINE('',#203405,#16448);
#9382=LINE('',#203409,#16449);
#9383=LINE('',#203411,#16450);
#9384=LINE('',#203413,#16451);
#9385=LINE('',#203414,#16452);
#9386=LINE('',#203418,#16453);
#9387=LINE('',#203419,#16454);
#9388=LINE('',#203420,#16455);
#9389=LINE('',#203424,#16456);
#9390=LINE('',#203425,#16457);
#9391=LINE('',#203426,#16458);
#9392=LINE('',#203428,#16459);
#9393=LINE('',#203429,#16460);
#9394=LINE('',#203433,#16461);
#9395=LINE('',#203435,#16462);
#9396=LINE('',#203437,#16463);
#9397=LINE('',#203438,#16464);
#9398=LINE('',#203442,#16465);
#9399=LINE('',#203443,#16466);
#9400=LINE('',#203444,#16467);
#9401=LINE('',#203448,#16468);
#9402=LINE('',#203449,#16469);
#9403=LINE('',#203450,#16470);
#9404=LINE('',#203452,#16471);
#9405=LINE('',#203453,#16472);
#9406=LINE('',#203457,#16473);
#9407=LINE('',#203459,#16474);
#9408=LINE('',#203461,#16475);
#9409=LINE('',#203462,#16476);
#9410=LINE('',#203466,#16477);
#9411=LINE('',#203467,#16478);
#9412=LINE('',#203468,#16479);
#9413=LINE('',#203472,#16480);
#9414=LINE('',#203473,#16481);
#9415=LINE('',#203474,#16482);
#9416=LINE('',#203476,#16483);
#9417=LINE('',#203477,#16484);
#9418=LINE('',#203481,#16485);
#9419=LINE('',#203483,#16486);
#9420=LINE('',#203485,#16487);
#9421=LINE('',#203486,#16488);
#9422=LINE('',#203490,#16489);
#9423=LINE('',#203491,#16490);
#9424=LINE('',#203492,#16491);
#9425=LINE('',#203496,#16492);
#9426=LINE('',#203497,#16493);
#9427=LINE('',#203498,#16494);
#9428=LINE('',#203500,#16495);
#9429=LINE('',#203501,#16496);
#9430=LINE('',#203505,#16497);
#9431=LINE('',#203507,#16498);
#9432=LINE('',#203509,#16499);
#9433=LINE('',#203510,#16500);
#9434=LINE('',#203514,#16501);
#9435=LINE('',#203515,#16502);
#9436=LINE('',#203516,#16503);
#9437=LINE('',#203520,#16504);
#9438=LINE('',#203521,#16505);
#9439=LINE('',#203522,#16506);
#9440=LINE('',#203524,#16507);
#9441=LINE('',#203525,#16508);
#9442=LINE('',#203529,#16509);
#9443=LINE('',#203531,#16510);
#9444=LINE('',#203533,#16511);
#9445=LINE('',#203534,#16512);
#9446=LINE('',#203538,#16513);
#9447=LINE('',#203539,#16514);
#9448=LINE('',#203540,#16515);
#9449=LINE('',#203544,#16516);
#9450=LINE('',#203545,#16517);
#9451=LINE('',#203546,#16518);
#9452=LINE('',#203548,#16519);
#9453=LINE('',#203549,#16520);
#9454=LINE('',#203553,#16521);
#9455=LINE('',#203555,#16522);
#9456=LINE('',#203557,#16523);
#9457=LINE('',#203558,#16524);
#9458=LINE('',#203562,#16525);
#9459=LINE('',#203563,#16526);
#9460=LINE('',#203564,#16527);
#9461=LINE('',#203568,#16528);
#9462=LINE('',#203569,#16529);
#9463=LINE('',#203570,#16530);
#9464=LINE('',#203572,#16531);
#9465=LINE('',#203573,#16532);
#9466=LINE('',#203577,#16533);
#9467=LINE('',#203579,#16534);
#9468=LINE('',#203581,#16535);
#9469=LINE('',#203582,#16536);
#9470=LINE('',#203586,#16537);
#9471=LINE('',#203587,#16538);
#9472=LINE('',#203588,#16539);
#9473=LINE('',#203592,#16540);
#9474=LINE('',#203593,#16541);
#9475=LINE('',#203594,#16542);
#9476=LINE('',#203596,#16543);
#9477=LINE('',#203597,#16544);
#9478=LINE('',#203601,#16545);
#9479=LINE('',#203603,#16546);
#9480=LINE('',#203605,#16547);
#9481=LINE('',#203606,#16548);
#9482=LINE('',#203610,#16549);
#9483=LINE('',#203611,#16550);
#9484=LINE('',#203612,#16551);
#9485=LINE('',#203616,#16552);
#9486=LINE('',#203617,#16553);
#9487=LINE('',#203618,#16554);
#9488=LINE('',#203620,#16555);
#9489=LINE('',#203621,#16556);
#9490=LINE('',#203625,#16557);
#9491=LINE('',#203627,#16558);
#9492=LINE('',#203629,#16559);
#9493=LINE('',#203630,#16560);
#9494=LINE('',#203634,#16561);
#9495=LINE('',#203635,#16562);
#9496=LINE('',#203636,#16563);
#9497=LINE('',#203640,#16564);
#9498=LINE('',#203641,#16565);
#9499=LINE('',#203642,#16566);
#9500=LINE('',#203644,#16567);
#9501=LINE('',#203645,#16568);
#9502=LINE('',#203649,#16569);
#9503=LINE('',#203651,#16570);
#9504=LINE('',#203653,#16571);
#9505=LINE('',#203654,#16572);
#9506=LINE('',#203658,#16573);
#9507=LINE('',#203659,#16574);
#9508=LINE('',#203660,#16575);
#9509=LINE('',#203664,#16576);
#9510=LINE('',#203665,#16577);
#9511=LINE('',#203666,#16578);
#9512=LINE('',#203668,#16579);
#9513=LINE('',#203669,#16580);
#9514=LINE('',#203673,#16581);
#9515=LINE('',#203675,#16582);
#9516=LINE('',#203677,#16583);
#9517=LINE('',#203678,#16584);
#9518=LINE('',#203682,#16585);
#9519=LINE('',#203683,#16586);
#9520=LINE('',#203684,#16587);
#9521=LINE('',#203688,#16588);
#9522=LINE('',#203689,#16589);
#9523=LINE('',#203690,#16590);
#9524=LINE('',#203692,#16591);
#9525=LINE('',#203693,#16592);
#9526=LINE('',#203697,#16593);
#9527=LINE('',#203699,#16594);
#9528=LINE('',#203701,#16595);
#9529=LINE('',#203702,#16596);
#9530=LINE('',#203706,#16597);
#9531=LINE('',#203707,#16598);
#9532=LINE('',#203708,#16599);
#9533=LINE('',#203712,#16600);
#9534=LINE('',#203713,#16601);
#9535=LINE('',#203714,#16602);
#9536=LINE('',#203716,#16603);
#9537=LINE('',#203717,#16604);
#9538=LINE('',#203721,#16605);
#9539=LINE('',#203723,#16606);
#9540=LINE('',#203725,#16607);
#9541=LINE('',#203726,#16608);
#9542=LINE('',#203730,#16609);
#9543=LINE('',#203731,#16610);
#9544=LINE('',#203732,#16611);
#9545=LINE('',#203736,#16612);
#9546=LINE('',#203737,#16613);
#9547=LINE('',#203738,#16614);
#9548=LINE('',#203740,#16615);
#9549=LINE('',#203741,#16616);
#9550=LINE('',#203745,#16617);
#9551=LINE('',#203747,#16618);
#9552=LINE('',#203749,#16619);
#9553=LINE('',#203750,#16620);
#9554=LINE('',#203754,#16621);
#9555=LINE('',#203755,#16622);
#9556=LINE('',#203756,#16623);
#9557=LINE('',#203760,#16624);
#9558=LINE('',#203761,#16625);
#9559=LINE('',#203762,#16626);
#9560=LINE('',#203764,#16627);
#9561=LINE('',#203765,#16628);
#9562=LINE('',#203769,#16629);
#9563=LINE('',#203771,#16630);
#9564=LINE('',#203773,#16631);
#9565=LINE('',#203774,#16632);
#9566=LINE('',#203778,#16633);
#9567=LINE('',#203779,#16634);
#9568=LINE('',#203780,#16635);
#9569=LINE('',#203784,#16636);
#9570=LINE('',#203785,#16637);
#9571=LINE('',#203786,#16638);
#9572=LINE('',#203788,#16639);
#9573=LINE('',#203789,#16640);
#9574=LINE('',#203793,#16641);
#9575=LINE('',#203795,#16642);
#9576=LINE('',#203797,#16643);
#9577=LINE('',#203798,#16644);
#9578=LINE('',#203802,#16645);
#9579=LINE('',#203803,#16646);
#9580=LINE('',#203804,#16647);
#9581=LINE('',#203808,#16648);
#9582=LINE('',#203809,#16649);
#9583=LINE('',#203810,#16650);
#9584=LINE('',#203812,#16651);
#9585=LINE('',#203813,#16652);
#9586=LINE('',#203817,#16653);
#9587=LINE('',#203819,#16654);
#9588=LINE('',#203821,#16655);
#9589=LINE('',#203822,#16656);
#9590=LINE('',#203826,#16657);
#9591=LINE('',#203827,#16658);
#9592=LINE('',#203828,#16659);
#9593=LINE('',#203832,#16660);
#9594=LINE('',#203833,#16661);
#9595=LINE('',#203834,#16662);
#9596=LINE('',#203836,#16663);
#9597=LINE('',#203837,#16664);
#9598=LINE('',#203841,#16665);
#9599=LINE('',#203843,#16666);
#9600=LINE('',#203845,#16667);
#9601=LINE('',#203846,#16668);
#9602=LINE('',#203850,#16669);
#9603=LINE('',#203851,#16670);
#9604=LINE('',#203852,#16671);
#9605=LINE('',#203856,#16672);
#9606=LINE('',#203857,#16673);
#9607=LINE('',#203858,#16674);
#9608=LINE('',#203860,#16675);
#9609=LINE('',#203861,#16676);
#9610=LINE('',#203865,#16677);
#9611=LINE('',#203867,#16678);
#9612=LINE('',#203869,#16679);
#9613=LINE('',#203870,#16680);
#9614=LINE('',#203874,#16681);
#9615=LINE('',#203875,#16682);
#9616=LINE('',#203876,#16683);
#9617=LINE('',#203880,#16684);
#9618=LINE('',#203881,#16685);
#9619=LINE('',#203882,#16686);
#9620=LINE('',#203884,#16687);
#9621=LINE('',#203885,#16688);
#9622=LINE('',#203890,#16689);
#9623=LINE('',#203892,#16690);
#9624=LINE('',#203894,#16691);
#9625=LINE('',#203895,#16692);
#9626=LINE('',#203898,#16693);
#9627=LINE('',#203900,#16694);
#9628=LINE('',#203901,#16695);
#9629=LINE('',#203904,#16696);
#9630=LINE('',#203905,#16697);
#9631=LINE('',#203908,#16698);
#9632=LINE('',#203909,#16699);
#9633=LINE('',#203911,#16700);
#9634=LINE('',#203915,#16701);
#9635=LINE('',#203917,#16702);
#9636=LINE('',#203919,#16703);
#9637=LINE('',#203921,#16704);
#9638=LINE('',#203925,#16705);
#9639=LINE('',#203927,#16706);
#9640=LINE('',#203929,#16707);
#9641=LINE('',#203931,#16708);
#9642=LINE('',#203948,#16709);
#9643=LINE('',#203950,#16710);
#9644=LINE('',#203954,#16711);
#9645=LINE('',#203958,#16712);
#10293=VECTOR('',#89691,13.9);
#10294=VECTOR('',#89696,13.9);
#10295=VECTOR('',#89701,13.9);
#10296=VECTOR('',#89704,13.9);
#10297=VECTOR('',#89711,11.64412671312);
#10298=VECTOR('',#89730,1000.);
#10299=VECTOR('',#89731,1000.);
#10300=VECTOR('',#89734,1000.);
#10301=VECTOR('',#89735,1000.);
#10302=VECTOR('',#89738,11.05);
#10303=VECTOR('',#89743,11.05);
#10304=VECTOR('',#89764,1000.);
#10305=VECTOR('',#89765,1000.);
#10306=VECTOR('',#89768,1000.);
#10307=VECTOR('',#89769,1000.);
#10308=VECTOR('',#89774,11.35);
#10309=VECTOR('',#89779,11.35);
#10310=VECTOR('',#89808,9.85);
#10311=VECTOR('',#89815,10.15);
#10312=VECTOR('',#89836,11.94412676881);
#10313=VECTOR('',#89841,12.25);
#10314=VECTOR('',#89848,12.75);
#10315=VECTOR('',#89855,13.1);
#10316=VECTOR('',#89862,1000.);
#10317=VECTOR('',#89865,1000.);
#10318=VECTOR('',#89868,1000.);
#10319=VECTOR('',#89871,13.7);
#10320=VECTOR('',#89876,1000.);
#10321=VECTOR('',#89885,12.75);
#10322=VECTOR('',#89888,10.);
#10323=VECTOR('',#89889,10.);
#10324=VECTOR('',#89892,1000.);
#10325=VECTOR('',#89893,1000.);
#10326=VECTOR('',#89904,1000.);
#10327=VECTOR('',#89905,1000.);
#10328=VECTOR('',#89916,10.);
#10329=VECTOR('',#89929,1000.);
#10330=VECTOR('',#89930,1000.);
#10331=VECTOR('',#89931,1000.);
#10332=VECTOR('',#89934,1000.);
#10333=VECTOR('',#89937,1000.);
#10334=VECTOR('',#89946,1000.);
#10335=VECTOR('',#89953,1000.);
#10336=VECTOR('',#89962,1000.);
#10337=VECTOR('',#89963,1000.);
#10338=VECTOR('',#89964,1000.);
#10339=VECTOR('',#89969,1000.);
#10340=VECTOR('',#89972,1000.);
#10341=VECTOR('',#89979,1000.);
#10342=VECTOR('',#89986,1000.);
#10343=VECTOR('',#89993,1000.);
#10344=VECTOR('',#89996,1000.);
#10345=VECTOR('',#90001,1000.);
#10346=VECTOR('',#90002,1000.);
#10347=VECTOR('',#90007,1000.);
#10348=VECTOR('',#90008,1000.);
#10349=VECTOR('',#90015,1000.);
#10350=VECTOR('',#90024,1000.);
#10351=VECTOR('',#90027,1000.);
#10352=VECTOR('',#90032,1000.);
#10353=VECTOR('',#90039,1000.);
#10354=VECTOR('',#90052,1000.);
#10355=VECTOR('',#90055,1000.);
#10356=VECTOR('',#90060,1000.);
#10357=VECTOR('',#90067,1000.);
#10358=VECTOR('',#90080,1000.);
#10359=VECTOR('',#90083,1000.);
#10360=VECTOR('',#90088,1000.);
#10361=VECTOR('',#90095,1000.);
#10362=VECTOR('',#90108,1000.);
#10363=VECTOR('',#90111,1000.);
#10364=VECTOR('',#90116,1000.);
#10365=VECTOR('',#90123,1000.);
#10366=VECTOR('',#90138,1000.);
#10367=VECTOR('',#90139,1000.);
#10368=VECTOR('',#90140,1000.);
#10369=VECTOR('',#90145,1000.);
#10370=VECTOR('',#90148,1000.);
#10371=VECTOR('',#90155,1000.);
#10372=VECTOR('',#90162,1000.);
#10373=VECTOR('',#90169,1000.);
#10374=VECTOR('',#90172,1000.);
#10375=VECTOR('',#90177,1000.);
#10376=VECTOR('',#90178,1000.);
#10377=VECTOR('',#90185,1000.);
#10378=VECTOR('',#90186,1000.);
#10379=VECTOR('',#90193,1000.);
#10380=VECTOR('',#90202,1000.);
#10381=VECTOR('',#90205,1000.);
#10382=VECTOR('',#90210,1000.);
#10383=VECTOR('',#90211,1000.);
#10384=VECTOR('',#90218,1000.);
#10385=VECTOR('',#90219,1000.);
#10386=VECTOR('',#90226,1000.);
#10387=VECTOR('',#90235,1000.);
#10388=VECTOR('',#90238,1000.);
#10389=VECTOR('',#90243,1000.);
#10390=VECTOR('',#90250,1000.);
#10391=VECTOR('',#90251,1000.);
#10392=VECTOR('',#90260,1000.);
#10393=VECTOR('',#90269,1000.);
#10394=VECTOR('',#90272,1000.);
#10395=VECTOR('',#90277,1000.);
#10396=VECTOR('',#90284,1000.);
#10397=VECTOR('',#90297,1000.);
#10398=VECTOR('',#90300,1000.);
#10399=VECTOR('',#90305,1000.);
#10400=VECTOR('',#90306,1000.);
#10401=VECTOR('',#90313,1000.);
#10402=VECTOR('',#90314,1000.);
#10403=VECTOR('',#90321,1000.);
#10404=VECTOR('',#90330,1000.);
#10405=VECTOR('',#90333,1000.);
#10406=VECTOR('',#90338,1000.);
#10407=VECTOR('',#90339,1000.);
#10408=VECTOR('',#90346,1000.);
#10409=VECTOR('',#90347,1000.);
#10410=VECTOR('',#90354,1000.);
#10411=VECTOR('',#90363,1000.);
#10412=VECTOR('',#90366,1000.);
#10413=VECTOR('',#90371,1000.);
#10414=VECTOR('',#90372,1000.);
#10415=VECTOR('',#90379,1000.);
#10416=VECTOR('',#90380,1000.);
#10417=VECTOR('',#90387,1000.);
#10418=VECTOR('',#90396,1000.);
#10419=VECTOR('',#90399,1000.);
#10420=VECTOR('',#90404,1000.);
#10421=VECTOR('',#90405,1000.);
#10422=VECTOR('',#90412,1000.);
#10423=VECTOR('',#90413,1000.);
#10424=VECTOR('',#90420,1000.);
#10425=VECTOR('',#90429,1000.);
#10426=VECTOR('',#90432,1000.);
#10427=VECTOR('',#90437,1000.);
#10428=VECTOR('',#90444,1000.);
#10429=VECTOR('',#90457,1000.);
#10430=VECTOR('',#90460,1000.);
#10431=VECTOR('',#90465,1000.);
#10432=VECTOR('',#90472,1000.);
#10433=VECTOR('',#90485,1000.);
#10434=VECTOR('',#90488,1000.);
#10435=VECTOR('',#90493,1000.);
#10436=VECTOR('',#90500,1000.);
#10437=VECTOR('',#90513,1000.);
#10438=VECTOR('',#90516,1000.);
#10439=VECTOR('',#90521,1000.);
#10440=VECTOR('',#90528,1000.);
#10441=VECTOR('',#90541,1000.);
#10442=VECTOR('',#90544,1000.);
#10443=VECTOR('',#90549,1000.);
#10444=VECTOR('',#90556,1000.);
#10445=VECTOR('',#90569,1000.);
#10446=VECTOR('',#90572,1000.);
#10447=VECTOR('',#90577,1000.);
#10448=VECTOR('',#90584,1000.);
#10449=VECTOR('',#90599,1000.);
#10450=VECTOR('',#90602,1000.);
#10451=VECTOR('',#90607,1000.);
#10452=VECTOR('',#90612,1000.);
#10453=VECTOR('',#90617,1000.);
#10454=VECTOR('',#90624,1000.);
#10455=VECTOR('',#90631,1000.);
#10456=VECTOR('',#90634,1000.);
#10457=VECTOR('',#90639,1000.);
#10458=VECTOR('',#90640,1000.);
#10459=VECTOR('',#90647,1000.);
#10460=VECTOR('',#90648,1000.);
#10461=VECTOR('',#90655,1000.);
#10462=VECTOR('',#90664,1000.);
#10463=VECTOR('',#90667,1000.);
#10464=VECTOR('',#90672,1000.);
#10465=VECTOR('',#90679,1000.);
#10466=VECTOR('',#90692,1000.);
#10467=VECTOR('',#90695,1000.);
#10468=VECTOR('',#90700,1000.);
#10469=VECTOR('',#90707,1000.);
#10470=VECTOR('',#90720,1000.);
#10471=VECTOR('',#90723,1000.);
#10472=VECTOR('',#90728,1000.);
#10473=VECTOR('',#90735,1000.);
#10474=VECTOR('',#90748,1000.);
#10475=VECTOR('',#90751,1000.);
#10476=VECTOR('',#90756,1000.);
#10477=VECTOR('',#90763,1000.);
#10478=VECTOR('',#90776,1000.);
#10479=VECTOR('',#90779,1000.);
#10480=VECTOR('',#90784,1000.);
#10481=VECTOR('',#90791,1000.);
#10482=VECTOR('',#90804,1000.);
#10483=VECTOR('',#90807,1000.);
#10484=VECTOR('',#90812,1000.);
#10485=VECTOR('',#90819,1000.);
#10486=VECTOR('',#90832,1000.);
#10487=VECTOR('',#90835,1000.);
#10488=VECTOR('',#90840,1000.);
#10489=VECTOR('',#90847,1000.);
#10490=VECTOR('',#90860,1000.);
#10491=VECTOR('',#90863,1000.);
#10492=VECTOR('',#90868,1000.);
#10493=VECTOR('',#90875,1000.);
#10494=VECTOR('',#90888,1000.);
#10495=VECTOR('',#90891,1000.);
#10496=VECTOR('',#90896,1000.);
#10497=VECTOR('',#90897,1000.);
#10498=VECTOR('',#90904,1000.);
#10499=VECTOR('',#90905,1000.);
#10500=VECTOR('',#90912,1000.);
#10501=VECTOR('',#90921,1000.);
#10502=VECTOR('',#90924,1000.);
#10503=VECTOR('',#90929,1000.);
#10504=VECTOR('',#90930,1000.);
#10505=VECTOR('',#90937,1000.);
#10506=VECTOR('',#90938,1000.);
#10507=VECTOR('',#90945,1000.);
#10508=VECTOR('',#90954,1000.);
#10509=VECTOR('',#90957,1000.);
#10510=VECTOR('',#90962,1000.);
#10511=VECTOR('',#90969,1000.);
#10512=VECTOR('',#90982,1000.);
#10513=VECTOR('',#90985,1000.);
#10514=VECTOR('',#90990,1000.);
#10515=VECTOR('',#90997,1000.);
#10516=VECTOR('',#91010,1000.);
#10517=VECTOR('',#91013,1000.);
#10518=VECTOR('',#91018,1000.);
#10519=VECTOR('',#91025,1000.);
#10520=VECTOR('',#91038,1000.);
#10521=VECTOR('',#91041,1000.);
#10522=VECTOR('',#91046,1000.);
#10523=VECTOR('',#91053,1000.);
#10524=VECTOR('',#91066,1000.);
#10525=VECTOR('',#91069,1000.);
#10526=VECTOR('',#91074,1000.);
#10527=VECTOR('',#91081,1000.);
#10528=VECTOR('',#91094,1000.);
#10529=VECTOR('',#91097,1000.);
#10530=VECTOR('',#91102,1000.);
#10531=VECTOR('',#91109,1000.);
#10532=VECTOR('',#91122,1000.);
#10533=VECTOR('',#91125,1000.);
#10534=VECTOR('',#91130,1000.);
#10535=VECTOR('',#91137,1000.);
#10536=VECTOR('',#91150,1000.);
#10537=VECTOR('',#91153,1000.);
#10538=VECTOR('',#91158,1000.);
#10539=VECTOR('',#91165,1000.);
#10540=VECTOR('',#91178,1000.);
#10541=VECTOR('',#91181,1000.);
#10542=VECTOR('',#91186,1000.);
#10543=VECTOR('',#91193,1000.);
#10544=VECTOR('',#91206,1000.);
#10545=VECTOR('',#91209,1000.);
#10546=VECTOR('',#91214,1000.);
#10547=VECTOR('',#91221,1000.);
#10548=VECTOR('',#91234,1000.);
#10549=VECTOR('',#91235,1000.);
#10550=VECTOR('',#91240,1000.);
#10551=VECTOR('',#91243,1000.);
#10552=VECTOR('',#91248,1000.);
#10553=VECTOR('',#91255,1000.);
#10554=VECTOR('',#91268,1000.);
#10555=VECTOR('',#91271,1000.);
#10556=VECTOR('',#91276,1000.);
#10557=VECTOR('',#91283,1000.);
#10558=VECTOR('',#91296,1000.);
#10559=VECTOR('',#91299,1000.);
#10560=VECTOR('',#91304,1000.);
#10561=VECTOR('',#91311,1000.);
#10562=VECTOR('',#91324,1000.);
#10563=VECTOR('',#91327,1000.);
#10564=VECTOR('',#91332,1000.);
#10565=VECTOR('',#91339,1000.);
#10566=VECTOR('',#91352,1000.);
#10567=VECTOR('',#91355,1000.);
#10568=VECTOR('',#91360,1000.);
#10569=VECTOR('',#91367,1000.);
#10570=VECTOR('',#91380,1000.);
#10571=VECTOR('',#91383,1000.);
#10572=VECTOR('',#91388,1000.);
#10573=VECTOR('',#91395,1000.);
#10574=VECTOR('',#91408,1000.);
#10575=VECTOR('',#91411,1000.);
#10576=VECTOR('',#91416,1000.);
#10577=VECTOR('',#91423,1000.);
#10578=VECTOR('',#91436,1000.);
#10579=VECTOR('',#91439,1000.);
#10580=VECTOR('',#91444,1000.);
#10581=VECTOR('',#91451,1000.);
#10582=VECTOR('',#91464,1000.);
#10583=VECTOR('',#91467,1000.);
#10584=VECTOR('',#91472,1000.);
#10585=VECTOR('',#91479,1000.);
#10586=VECTOR('',#91492,1000.);
#10587=VECTOR('',#91495,1000.);
#10588=VECTOR('',#91500,1000.);
#10589=VECTOR('',#91507,1000.);
#10590=VECTOR('',#91520,1000.);
#10591=VECTOR('',#91523,1000.);
#10592=VECTOR('',#91528,1000.);
#10593=VECTOR('',#91535,1000.);
#10594=VECTOR('',#91548,1000.);
#10595=VECTOR('',#91551,1000.);
#10596=VECTOR('',#91556,1000.);
#10597=VECTOR('',#91563,1000.);
#10598=VECTOR('',#91564,1000.);
#10599=VECTOR('',#91573,1000.);
#10600=VECTOR('',#91582,1000.);
#10601=VECTOR('',#91585,1000.);
#10602=VECTOR('',#91590,1000.);
#10603=VECTOR('',#91597,1000.);
#10604=VECTOR('',#91598,1000.);
#10605=VECTOR('',#91607,1000.);
#10606=VECTOR('',#91616,1000.);
#10607=VECTOR('',#91619,1000.);
#10608=VECTOR('',#91624,1000.);
#10609=VECTOR('',#91631,1000.);
#10610=VECTOR('',#91644,1000.);
#10611=VECTOR('',#91647,1000.);
#10612=VECTOR('',#91652,1000.);
#10613=VECTOR('',#91659,1000.);
#10614=VECTOR('',#91672,1000.);
#10615=VECTOR('',#91675,1000.);
#10616=VECTOR('',#91680,1000.);
#10617=VECTOR('',#91687,1000.);
#10618=VECTOR('',#91700,1000.);
#10619=VECTOR('',#91703,1000.);
#10620=VECTOR('',#91708,1000.);
#10621=VECTOR('',#91715,1000.);
#10622=VECTOR('',#91728,1000.);
#10623=VECTOR('',#91731,1000.);
#10624=VECTOR('',#91736,1000.);
#10625=VECTOR('',#91743,1000.);
#10626=VECTOR('',#91756,1000.);
#10627=VECTOR('',#91759,1000.);
#10628=VECTOR('',#91764,1000.);
#10629=VECTOR('',#91771,1000.);
#10630=VECTOR('',#91784,1000.);
#10631=VECTOR('',#91787,1000.);
#10632=VECTOR('',#91792,1000.);
#10633=VECTOR('',#91799,1000.);
#10634=VECTOR('',#91812,1000.);
#10635=VECTOR('',#91815,1000.);
#10636=VECTOR('',#91820,1000.);
#10637=VECTOR('',#91827,1000.);
#10638=VECTOR('',#91840,1000.);
#10639=VECTOR('',#91843,1000.);
#10640=VECTOR('',#91848,1000.);
#10641=VECTOR('',#91855,1000.);
#10642=VECTOR('',#91868,1000.);
#10643=VECTOR('',#91871,1000.);
#10644=VECTOR('',#91876,1000.);
#10645=VECTOR('',#91883,1000.);
#10646=VECTOR('',#91896,1000.);
#10647=VECTOR('',#91899,1000.);
#10648=VECTOR('',#91904,1000.);
#10649=VECTOR('',#91911,1000.);
#10650=VECTOR('',#91924,1000.);
#10651=VECTOR('',#91927,1000.);
#10652=VECTOR('',#91932,1000.);
#10653=VECTOR('',#91939,1000.);
#10654=VECTOR('',#91952,1000.);
#10655=VECTOR('',#91955,1000.);
#10656=VECTOR('',#91960,1000.);
#10657=VECTOR('',#91967,1000.);
#10658=VECTOR('',#91980,1000.);
#10659=VECTOR('',#91983,1000.);
#10660=VECTOR('',#91988,1000.);
#10661=VECTOR('',#91995,1000.);
#10662=VECTOR('',#92008,1000.);
#10663=VECTOR('',#92011,1000.);
#10664=VECTOR('',#92016,1000.);
#10665=VECTOR('',#92023,1000.);
#10666=VECTOR('',#92036,1000.);
#10667=VECTOR('',#92039,1000.);
#10668=VECTOR('',#92044,1000.);
#10669=VECTOR('',#92051,1000.);
#10670=VECTOR('',#92064,1000.);
#10671=VECTOR('',#92067,1000.);
#10672=VECTOR('',#92072,1000.);
#10673=VECTOR('',#92079,1000.);
#10674=VECTOR('',#92092,1000.);
#10675=VECTOR('',#92095,1000.);
#10676=VECTOR('',#92100,1000.);
#10677=VECTOR('',#92107,1000.);
#10678=VECTOR('',#92120,1000.);
#10679=VECTOR('',#92123,1000.);
#10680=VECTOR('',#92128,1000.);
#10681=VECTOR('',#92135,1000.);
#10682=VECTOR('',#92148,1000.);
#10683=VECTOR('',#92151,1000.);
#10684=VECTOR('',#92156,1000.);
#10685=VECTOR('',#92163,1000.);
#10686=VECTOR('',#92176,1000.);
#10687=VECTOR('',#92179,1000.);
#10688=VECTOR('',#92184,1000.);
#10689=VECTOR('',#92191,1000.);
#10690=VECTOR('',#92204,1000.);
#10691=VECTOR('',#92207,1000.);
#10692=VECTOR('',#92212,1000.);
#10693=VECTOR('',#92219,1000.);
#10694=VECTOR('',#92232,1000.);
#10695=VECTOR('',#92235,1000.);
#10696=VECTOR('',#92240,1000.);
#10697=VECTOR('',#92247,1000.);
#10698=VECTOR('',#92260,1000.);
#10699=VECTOR('',#92263,1000.);
#10700=VECTOR('',#92268,1000.);
#10701=VECTOR('',#92275,1000.);
#10702=VECTOR('',#92288,1000.);
#10703=VECTOR('',#92291,1000.);
#10704=VECTOR('',#92296,1000.);
#10705=VECTOR('',#92303,1000.);
#10706=VECTOR('',#92316,1000.);
#10707=VECTOR('',#92319,1000.);
#10708=VECTOR('',#92324,1000.);
#10709=VECTOR('',#92331,1000.);
#10710=VECTOR('',#92344,1000.);
#10711=VECTOR('',#92347,1000.);
#10712=VECTOR('',#92352,1000.);
#10713=VECTOR('',#92359,1000.);
#10714=VECTOR('',#92372,1000.);
#10715=VECTOR('',#92375,1000.);
#10716=VECTOR('',#92380,1000.);
#10717=VECTOR('',#92387,1000.);
#10718=VECTOR('',#92400,1000.);
#10719=VECTOR('',#92403,1000.);
#10720=VECTOR('',#92408,1000.);
#10721=VECTOR('',#92415,1000.);
#10722=VECTOR('',#92428,1000.);
#10723=VECTOR('',#92431,1000.);
#10724=VECTOR('',#92436,1000.);
#10725=VECTOR('',#92443,1000.);
#10726=VECTOR('',#92456,1000.);
#10727=VECTOR('',#92459,1000.);
#10728=VECTOR('',#92464,1000.);
#10729=VECTOR('',#92471,1000.);
#10730=VECTOR('',#92484,1000.);
#10731=VECTOR('',#92487,1000.);
#10732=VECTOR('',#92492,1000.);
#10733=VECTOR('',#92499,1000.);
#10734=VECTOR('',#92512,1000.);
#10735=VECTOR('',#92515,1000.);
#10736=VECTOR('',#92520,1000.);
#10737=VECTOR('',#92527,1000.);
#10738=VECTOR('',#92540,1000.);
#10739=VECTOR('',#92543,1000.);
#10740=VECTOR('',#92548,1000.);
#10741=VECTOR('',#92555,1000.);
#10742=VECTOR('',#92568,1000.);
#10743=VECTOR('',#92571,1000.);
#10744=VECTOR('',#92576,1000.);
#10745=VECTOR('',#92583,1000.);
#10746=VECTOR('',#92596,1000.);
#10747=VECTOR('',#92599,1000.);
#10748=VECTOR('',#92604,1000.);
#10749=VECTOR('',#92611,1000.);
#10750=VECTOR('',#92624,1000.);
#10751=VECTOR('',#92627,1000.);
#10752=VECTOR('',#92632,1000.);
#10753=VECTOR('',#92639,1000.);
#10754=VECTOR('',#92652,1000.);
#10755=VECTOR('',#92655,1000.);
#10756=VECTOR('',#92660,1000.);
#10757=VECTOR('',#92667,1000.);
#10758=VECTOR('',#92680,1000.);
#10759=VECTOR('',#92683,1000.);
#10760=VECTOR('',#92688,1000.);
#10761=VECTOR('',#92695,1000.);
#10762=VECTOR('',#92708,1000.);
#10763=VECTOR('',#92711,1000.);
#10764=VECTOR('',#92716,1000.);
#10765=VECTOR('',#92723,1000.);
#10766=VECTOR('',#92736,1000.);
#10767=VECTOR('',#92739,1000.);
#10768=VECTOR('',#92744,1000.);
#10769=VECTOR('',#92751,1000.);
#10770=VECTOR('',#92764,1000.);
#10771=VECTOR('',#92767,1000.);
#10772=VECTOR('',#92772,1000.);
#10773=VECTOR('',#92779,1000.);
#10774=VECTOR('',#92792,1000.);
#10775=VECTOR('',#92795,1000.);
#10776=VECTOR('',#92800,1000.);
#10777=VECTOR('',#92807,1000.);
#10778=VECTOR('',#92820,1000.);
#10779=VECTOR('',#92823,1000.);
#10780=VECTOR('',#92828,1000.);
#10781=VECTOR('',#92835,1000.);
#10782=VECTOR('',#92848,1000.);
#10783=VECTOR('',#92851,1000.);
#10784=VECTOR('',#92856,1000.);
#10785=VECTOR('',#92863,1000.);
#10786=VECTOR('',#92876,1000.);
#10787=VECTOR('',#92879,1000.);
#10788=VECTOR('',#92884,1000.);
#10789=VECTOR('',#92891,1000.);
#10790=VECTOR('',#92904,1000.);
#10791=VECTOR('',#92907,1000.);
#10792=VECTOR('',#92912,1000.);
#10793=VECTOR('',#92919,1000.);
#10794=VECTOR('',#92932,1000.);
#10795=VECTOR('',#92935,1000.);
#10796=VECTOR('',#92940,1000.);
#10797=VECTOR('',#92947,1000.);
#10798=VECTOR('',#92960,1000.);
#10799=VECTOR('',#92963,1000.);
#10800=VECTOR('',#92968,1000.);
#10801=VECTOR('',#92975,1000.);
#10802=VECTOR('',#92988,1000.);
#10803=VECTOR('',#92991,1000.);
#10804=VECTOR('',#92996,1000.);
#10805=VECTOR('',#93003,1000.);
#10806=VECTOR('',#93016,1000.);
#10807=VECTOR('',#93019,1000.);
#10808=VECTOR('',#93024,1000.);
#10809=VECTOR('',#93031,1000.);
#10810=VECTOR('',#93044,1000.);
#10811=VECTOR('',#93047,1000.);
#10812=VECTOR('',#93052,1000.);
#10813=VECTOR('',#93059,1000.);
#10814=VECTOR('',#93072,1000.);
#10815=VECTOR('',#93075,1000.);
#10816=VECTOR('',#93080,1000.);
#10817=VECTOR('',#93087,1000.);
#10818=VECTOR('',#93100,1000.);
#10819=VECTOR('',#93103,1000.);
#10820=VECTOR('',#93108,1000.);
#10821=VECTOR('',#93115,1000.);
#10822=VECTOR('',#93128,1000.);
#10823=VECTOR('',#93131,1000.);
#10824=VECTOR('',#93136,1000.);
#10825=VECTOR('',#93143,1000.);
#10826=VECTOR('',#93156,1000.);
#10827=VECTOR('',#93159,1000.);
#10828=VECTOR('',#93164,1000.);
#10829=VECTOR('',#93171,1000.);
#10830=VECTOR('',#93184,1000.);
#10831=VECTOR('',#93187,1000.);
#10832=VECTOR('',#93192,1000.);
#10833=VECTOR('',#93199,1000.);
#10834=VECTOR('',#93212,1000.);
#10835=VECTOR('',#93215,1000.);
#10836=VECTOR('',#93220,1000.);
#10837=VECTOR('',#93227,1000.);
#10838=VECTOR('',#93240,1000.);
#10839=VECTOR('',#93243,1000.);
#10840=VECTOR('',#93248,1000.);
#10841=VECTOR('',#93255,1000.);
#10842=VECTOR('',#93268,1000.);
#10843=VECTOR('',#93271,1000.);
#10844=VECTOR('',#93276,1000.);
#10845=VECTOR('',#93283,1000.);
#10846=VECTOR('',#93296,1000.);
#10847=VECTOR('',#93299,1000.);
#10848=VECTOR('',#93304,1000.);
#10849=VECTOR('',#93311,1000.);
#10850=VECTOR('',#93324,1000.);
#10851=VECTOR('',#93327,1000.);
#10852=VECTOR('',#93332,1000.);
#10853=VECTOR('',#93339,1000.);
#10854=VECTOR('',#93352,1000.);
#10855=VECTOR('',#93355,1000.);
#10856=VECTOR('',#93360,1000.);
#10857=VECTOR('',#93367,1000.);
#10858=VECTOR('',#93380,1000.);
#10859=VECTOR('',#93383,1000.);
#10860=VECTOR('',#93388,1000.);
#10861=VECTOR('',#93395,1000.);
#10862=VECTOR('',#93408,1000.);
#10863=VECTOR('',#93411,1000.);
#10864=VECTOR('',#93416,1000.);
#10865=VECTOR('',#93423,1000.);
#10866=VECTOR('',#93436,1000.);
#10867=VECTOR('',#93439,1000.);
#10868=VECTOR('',#93444,1000.);
#10869=VECTOR('',#93451,1000.);
#10870=VECTOR('',#93464,1000.);
#10871=VECTOR('',#93467,1000.);
#10872=VECTOR('',#93472,1000.);
#10873=VECTOR('',#93479,1000.);
#10874=VECTOR('',#93492,1000.);
#10875=VECTOR('',#93495,1000.);
#10876=VECTOR('',#93500,1000.);
#10877=VECTOR('',#93507,1000.);
#10878=VECTOR('',#93520,1000.);
#10879=VECTOR('',#93523,1000.);
#10880=VECTOR('',#93528,1000.);
#10881=VECTOR('',#93535,1000.);
#10882=VECTOR('',#93548,1000.);
#10883=VECTOR('',#93551,1000.);
#10884=VECTOR('',#93556,1000.);
#10885=VECTOR('',#93563,1000.);
#10886=VECTOR('',#93576,1000.);
#10887=VECTOR('',#93579,1000.);
#10888=VECTOR('',#93584,1000.);
#10889=VECTOR('',#93585,1000.);
#10890=VECTOR('',#93592,1000.);
#10891=VECTOR('',#93593,1000.);
#10892=VECTOR('',#93598,1000.);
#10893=VECTOR('',#93607,1000.);
#10894=VECTOR('',#93610,1000.);
#10895=VECTOR('',#93615,1000.);
#10896=VECTOR('',#93616,1000.);
#10897=VECTOR('',#93623,1000.);
#10898=VECTOR('',#93624,1000.);
#10899=VECTOR('',#93631,1000.);
#10900=VECTOR('',#93640,1000.);
#10901=VECTOR('',#93643,1000.);
#10902=VECTOR('',#93648,1000.);
#10903=VECTOR('',#93649,1000.);
#10904=VECTOR('',#93656,1000.);
#10905=VECTOR('',#93657,1000.);
#10906=VECTOR('',#93664,1000.);
#10907=VECTOR('',#93673,1000.);
#10908=VECTOR('',#93676,1000.);
#10909=VECTOR('',#93681,1000.);
#10910=VECTOR('',#93682,1000.);
#10911=VECTOR('',#93689,1000.);
#10912=VECTOR('',#93690,1000.);
#10913=VECTOR('',#93697,1000.);
#10914=VECTOR('',#93706,1000.);
#10915=VECTOR('',#93709,1000.);
#10916=VECTOR('',#93714,1000.);
#10917=VECTOR('',#93715,1000.);
#10918=VECTOR('',#93722,1000.);
#10919=VECTOR('',#93723,1000.);
#10920=VECTOR('',#93730,1000.);
#10921=VECTOR('',#93739,1000.);
#10922=VECTOR('',#93740,1000.);
#10923=VECTOR('',#93743,1000.);
#10924=VECTOR('',#93748,1000.);
#10925=VECTOR('',#93749,1000.);
#10926=VECTOR('',#93754,1000.);
#10927=VECTOR('',#93755,1000.);
#10928=VECTOR('',#93762,1000.);
#10929=VECTOR('',#93771,1000.);
#10930=VECTOR('',#93772,1000.);
#10931=VECTOR('',#93775,1000.);
#10932=VECTOR('',#93780,1000.);
#10933=VECTOR('',#93781,1000.);
#10934=VECTOR('',#93786,1000.);
#10935=VECTOR('',#93787,1000.);
#10936=VECTOR('',#93794,1000.);
#10937=VECTOR('',#93803,1000.);
#10938=VECTOR('',#93806,1000.);
#10939=VECTOR('',#93811,1000.);
#10940=VECTOR('',#93812,1000.);
#10941=VECTOR('',#93819,1000.);
#10942=VECTOR('',#93820,1000.);
#10943=VECTOR('',#93827,1000.);
#10944=VECTOR('',#93836,1000.);
#10945=VECTOR('',#93839,1000.);
#10946=VECTOR('',#93844,1000.);
#10947=VECTOR('',#93845,1000.);
#10948=VECTOR('',#93852,1000.);
#10949=VECTOR('',#93853,1000.);
#10950=VECTOR('',#93860,1000.);
#10951=VECTOR('',#93869,1000.);
#10952=VECTOR('',#93872,1000.);
#10953=VECTOR('',#93877,1000.);
#10954=VECTOR('',#93878,1000.);
#10955=VECTOR('',#93885,1000.);
#10956=VECTOR('',#93886,1000.);
#10957=VECTOR('',#93893,1000.);
#10958=VECTOR('',#93902,1000.);
#10959=VECTOR('',#93905,1000.);
#10960=VECTOR('',#93910,1000.);
#10961=VECTOR('',#93917,1000.);
#10962=VECTOR('',#93930,1000.);
#10963=VECTOR('',#93933,1000.);
#10964=VECTOR('',#93938,1000.);
#10965=VECTOR('',#93945,1000.);
#10966=VECTOR('',#93958,1000.);
#10967=VECTOR('',#93961,1000.);
#10968=VECTOR('',#93966,1000.);
#10969=VECTOR('',#93973,1000.);
#10970=VECTOR('',#93986,1000.);
#10971=VECTOR('',#93989,1000.);
#10972=VECTOR('',#93994,1000.);
#10973=VECTOR('',#94001,1000.);
#10974=VECTOR('',#94014,1000.);
#10975=VECTOR('',#94017,1000.);
#10976=VECTOR('',#94022,1000.);
#10977=VECTOR('',#94029,1000.);
#10978=VECTOR('',#94042,1000.);
#10979=VECTOR('',#94045,1000.);
#10980=VECTOR('',#94050,1000.);
#10981=VECTOR('',#94057,1000.);
#10982=VECTOR('',#94070,1000.);
#10983=VECTOR('',#94073,1000.);
#10984=VECTOR('',#94078,1000.);
#10985=VECTOR('',#94085,1000.);
#10986=VECTOR('',#94098,1000.);
#10987=VECTOR('',#94101,1000.);
#10988=VECTOR('',#94106,1000.);
#10989=VECTOR('',#94113,1000.);
#10990=VECTOR('',#94126,1000.);
#10991=VECTOR('',#94127,1000.);
#10992=VECTOR('',#94130,1000.);
#10993=VECTOR('',#94135,1000.);
#10994=VECTOR('',#94136,1000.);
#10995=VECTOR('',#94141,1000.);
#10996=VECTOR('',#94142,1000.);
#10997=VECTOR('',#94149,1000.);
#10998=VECTOR('',#94158,1000.);
#10999=VECTOR('',#94159,1000.);
#11000=VECTOR('',#94162,1000.);
#11001=VECTOR('',#94167,1000.);
#11002=VECTOR('',#94168,1000.);
#11003=VECTOR('',#94173,1000.);
#11004=VECTOR('',#94174,1000.);
#11005=VECTOR('',#94181,1000.);
#11006=VECTOR('',#94190,1000.);
#11007=VECTOR('',#94193,1000.);
#11008=VECTOR('',#94198,1000.);
#11009=VECTOR('',#94205,1000.);
#11010=VECTOR('',#94218,1000.);
#11011=VECTOR('',#94221,1000.);
#11012=VECTOR('',#94226,1000.);
#11013=VECTOR('',#94233,1000.);
#11014=VECTOR('',#94246,1000.);
#11015=VECTOR('',#94249,1000.);
#11016=VECTOR('',#94254,1000.);
#11017=VECTOR('',#94261,1000.);
#11018=VECTOR('',#94274,1000.);
#11019=VECTOR('',#94277,1000.);
#11020=VECTOR('',#94282,1000.);
#11021=VECTOR('',#94289,1000.);
#11022=VECTOR('',#94302,1000.);
#11023=VECTOR('',#94305,1000.);
#11024=VECTOR('',#94310,1000.);
#11025=VECTOR('',#94317,1000.);
#11026=VECTOR('',#94318,1000.);
#11027=VECTOR('',#94327,1000.);
#11028=VECTOR('',#94336,1000.);
#11029=VECTOR('',#94339,1000.);
#11030=VECTOR('',#94344,1000.);
#11031=VECTOR('',#94345,1000.);
#11032=VECTOR('',#94352,1000.);
#11033=VECTOR('',#94353,1000.);
#11034=VECTOR('',#94360,1000.);
#11035=VECTOR('',#94369,1000.);
#11036=VECTOR('',#94372,1000.);
#11037=VECTOR('',#94377,1000.);
#11038=VECTOR('',#94378,1000.);
#11039=VECTOR('',#94385,1000.);
#11040=VECTOR('',#94386,1000.);
#11041=VECTOR('',#94393,1000.);
#11042=VECTOR('',#94402,1000.);
#11043=VECTOR('',#94405,1000.);
#11044=VECTOR('',#94410,1000.);
#11045=VECTOR('',#94417,1000.);
#11046=VECTOR('',#94418,1000.);
#11047=VECTOR('',#94427,1000.);
#11048=VECTOR('',#94436,1000.);
#11049=VECTOR('',#94439,1000.);
#11050=VECTOR('',#94444,1000.);
#11051=VECTOR('',#94451,1000.);
#11052=VECTOR('',#94464,1000.);
#11053=VECTOR('',#94467,1000.);
#11054=VECTOR('',#94472,1000.);
#11055=VECTOR('',#94479,1000.);
#11056=VECTOR('',#94492,1000.);
#11057=VECTOR('',#94495,1000.);
#11058=VECTOR('',#94500,1000.);
#11059=VECTOR('',#94507,1000.);
#11060=VECTOR('',#94520,1000.);
#11061=VECTOR('',#94523,1000.);
#11062=VECTOR('',#94528,1000.);
#11063=VECTOR('',#94535,1000.);
#11064=VECTOR('',#94548,1000.);
#11065=VECTOR('',#94551,1000.);
#11066=VECTOR('',#94556,1000.);
#11067=VECTOR('',#94563,1000.);
#11068=VECTOR('',#94576,1000.);
#11069=VECTOR('',#94579,1000.);
#11070=VECTOR('',#94584,1000.);
#11071=VECTOR('',#94591,1000.);
#11072=VECTOR('',#94604,1000.);
#11073=VECTOR('',#94607,1000.);
#11074=VECTOR('',#94612,1000.);
#11075=VECTOR('',#94619,1000.);
#11076=VECTOR('',#94632,1000.);
#11077=VECTOR('',#94635,1000.);
#11078=VECTOR('',#94640,1000.);
#11079=VECTOR('',#94647,1000.);
#11080=VECTOR('',#94660,1000.);
#11081=VECTOR('',#94663,1000.);
#11082=VECTOR('',#94668,1000.);
#11083=VECTOR('',#94675,1000.);
#11084=VECTOR('',#94688,1000.);
#11085=VECTOR('',#94691,1000.);
#11086=VECTOR('',#94696,1000.);
#11087=VECTOR('',#94703,1000.);
#11088=VECTOR('',#94716,1000.);
#11089=VECTOR('',#94719,1000.);
#11090=VECTOR('',#94724,1000.);
#11091=VECTOR('',#94731,1000.);
#11092=VECTOR('',#94732,1000.);
#11093=VECTOR('',#94741,1000.);
#11094=VECTOR('',#94750,1000.);
#11095=VECTOR('',#94753,1000.);
#11096=VECTOR('',#94758,1000.);
#11097=VECTOR('',#94765,1000.);
#11098=VECTOR('',#94766,1000.);
#11099=VECTOR('',#94775,1000.);
#11100=VECTOR('',#94784,1000.);
#11101=VECTOR('',#94787,1000.);
#11102=VECTOR('',#94792,1000.);
#11103=VECTOR('',#94799,1000.);
#11104=VECTOR('',#94812,1000.);
#11105=VECTOR('',#94815,1000.);
#11106=VECTOR('',#94820,1000.);
#11107=VECTOR('',#94827,1000.);
#11108=VECTOR('',#94840,1000.);
#11109=VECTOR('',#94843,1000.);
#11110=VECTOR('',#94848,1000.);
#11111=VECTOR('',#94855,1000.);
#11112=VECTOR('',#94868,1000.);
#11113=VECTOR('',#94871,1000.);
#11114=VECTOR('',#94876,1000.);
#11115=VECTOR('',#94883,1000.);
#11116=VECTOR('',#94896,1000.);
#11117=VECTOR('',#94899,1000.);
#11118=VECTOR('',#94904,1000.);
#11119=VECTOR('',#94911,1000.);
#11120=VECTOR('',#94924,1000.);
#11121=VECTOR('',#94927,1000.);
#11122=VECTOR('',#94932,1000.);
#11123=VECTOR('',#94939,1000.);
#11124=VECTOR('',#94952,1000.);
#11125=VECTOR('',#94955,1000.);
#11126=VECTOR('',#94960,1000.);
#11127=VECTOR('',#94967,1000.);
#11128=VECTOR('',#94980,1000.);
#11129=VECTOR('',#94983,1000.);
#11130=VECTOR('',#94988,1000.);
#11131=VECTOR('',#94995,1000.);
#11132=VECTOR('',#95008,1000.);
#11133=VECTOR('',#95011,1000.);
#11134=VECTOR('',#95016,1000.);
#11135=VECTOR('',#95023,1000.);
#11136=VECTOR('',#95036,1000.);
#11137=VECTOR('',#95039,1000.);
#11138=VECTOR('',#95044,1000.);
#11139=VECTOR('',#95045,1000.);
#11140=VECTOR('',#95052,1000.);
#11141=VECTOR('',#95053,1000.);
#11142=VECTOR('',#95060,1000.);
#11143=VECTOR('',#95069,1000.);
#11144=VECTOR('',#95072,1000.);
#11145=VECTOR('',#95077,1000.);
#11146=VECTOR('',#95084,1000.);
#11147=VECTOR('',#95085,1000.);
#11148=VECTOR('',#95094,1000.);
#11149=VECTOR('',#95103,1000.);
#11150=VECTOR('',#95106,1000.);
#11151=VECTOR('',#95111,1000.);
#11152=VECTOR('',#95118,1000.);
#11153=VECTOR('',#95131,1000.);
#11154=VECTOR('',#95134,1000.);
#11155=VECTOR('',#95139,1000.);
#11156=VECTOR('',#95146,1000.);
#11157=VECTOR('',#95159,1000.);
#11158=VECTOR('',#95162,1000.);
#11159=VECTOR('',#95167,1000.);
#11160=VECTOR('',#95174,1000.);
#11161=VECTOR('',#95187,1000.);
#11162=VECTOR('',#95190,1000.);
#11163=VECTOR('',#95195,1000.);
#11164=VECTOR('',#95202,1000.);
#11165=VECTOR('',#95215,1000.);
#11166=VECTOR('',#95218,1000.);
#11167=VECTOR('',#95223,1000.);
#11168=VECTOR('',#95230,1000.);
#11169=VECTOR('',#95243,1000.);
#11170=VECTOR('',#95246,1000.);
#11171=VECTOR('',#95251,1000.);
#11172=VECTOR('',#95258,1000.);
#11173=VECTOR('',#95271,1000.);
#11174=VECTOR('',#95274,1000.);
#11175=VECTOR('',#95279,1000.);
#11176=VECTOR('',#95286,1000.);
#11177=VECTOR('',#95299,1000.);
#11178=VECTOR('',#95302,1000.);
#11179=VECTOR('',#95307,1000.);
#11180=VECTOR('',#95314,1000.);
#11181=VECTOR('',#95327,1000.);
#11182=VECTOR('',#95330,1000.);
#11183=VECTOR('',#95335,1000.);
#11184=VECTOR('',#95342,1000.);
#11185=VECTOR('',#95355,1000.);
#11186=VECTOR('',#95358,1000.);
#11187=VECTOR('',#95363,1000.);
#11188=VECTOR('',#95370,1000.);
#11189=VECTOR('',#95383,1000.);
#11190=VECTOR('',#95386,1000.);
#11191=VECTOR('',#95391,1000.);
#11192=VECTOR('',#95398,1000.);
#11193=VECTOR('',#95411,1000.);
#11194=VECTOR('',#95414,1000.);
#11195=VECTOR('',#95419,1000.);
#11196=VECTOR('',#95426,1000.);
#11197=VECTOR('',#95439,1000.);
#11198=VECTOR('',#95442,1000.);
#11199=VECTOR('',#95447,1000.);
#11200=VECTOR('',#95454,1000.);
#11201=VECTOR('',#95467,1000.);
#11202=VECTOR('',#95470,1000.);
#11203=VECTOR('',#95475,1000.);
#11204=VECTOR('',#95482,1000.);
#11205=VECTOR('',#95495,1000.);
#11206=VECTOR('',#95498,1000.);
#11207=VECTOR('',#95503,1000.);
#11208=VECTOR('',#95510,1000.);
#11209=VECTOR('',#95523,1000.);
#11210=VECTOR('',#95526,1000.);
#11211=VECTOR('',#95531,1000.);
#11212=VECTOR('',#95538,1000.);
#11213=VECTOR('',#95551,1000.);
#11214=VECTOR('',#95554,1000.);
#11215=VECTOR('',#95559,1000.);
#11216=VECTOR('',#95566,1000.);
#11217=VECTOR('',#95579,1000.);
#11218=VECTOR('',#95582,1000.);
#11219=VECTOR('',#95587,1000.);
#11220=VECTOR('',#95594,1000.);
#11221=VECTOR('',#95607,1000.);
#11222=VECTOR('',#95610,1000.);
#11223=VECTOR('',#95615,1000.);
#11224=VECTOR('',#95622,1000.);
#11225=VECTOR('',#95635,1000.);
#11226=VECTOR('',#95638,1000.);
#11227=VECTOR('',#95643,1000.);
#11228=VECTOR('',#95650,1000.);
#11229=VECTOR('',#95663,1000.);
#11230=VECTOR('',#95666,1000.);
#11231=VECTOR('',#95671,1000.);
#11232=VECTOR('',#95678,1000.);
#11233=VECTOR('',#95691,1000.);
#11234=VECTOR('',#95694,1000.);
#11235=VECTOR('',#95699,1000.);
#11236=VECTOR('',#95706,1000.);
#11237=VECTOR('',#95719,1000.);
#11238=VECTOR('',#95722,1000.);
#11239=VECTOR('',#95727,1000.);
#11240=VECTOR('',#95734,1000.);
#11241=VECTOR('',#95747,1000.);
#11242=VECTOR('',#95750,1000.);
#11243=VECTOR('',#95755,1000.);
#11244=VECTOR('',#95762,1000.);
#11245=VECTOR('',#95775,1000.);
#11246=VECTOR('',#95778,1000.);
#11247=VECTOR('',#95783,1000.);
#11248=VECTOR('',#95790,1000.);
#11249=VECTOR('',#95803,1000.);
#11250=VECTOR('',#95806,1000.);
#11251=VECTOR('',#95811,1000.);
#11252=VECTOR('',#95818,1000.);
#11253=VECTOR('',#95831,1000.);
#11254=VECTOR('',#95834,1000.);
#11255=VECTOR('',#95839,1000.);
#11256=VECTOR('',#95846,1000.);
#11257=VECTOR('',#95859,1000.);
#11258=VECTOR('',#95862,1000.);
#11259=VECTOR('',#95867,1000.);
#11260=VECTOR('',#95874,1000.);
#11261=VECTOR('',#95887,1000.);
#11262=VECTOR('',#95890,1000.);
#11263=VECTOR('',#95895,1000.);
#11264=VECTOR('',#95902,1000.);
#11265=VECTOR('',#95915,1000.);
#11266=VECTOR('',#95918,1000.);
#11267=VECTOR('',#95923,1000.);
#11268=VECTOR('',#95930,1000.);
#11269=VECTOR('',#95943,1000.);
#11270=VECTOR('',#95946,1000.);
#11271=VECTOR('',#95951,1000.);
#11272=VECTOR('',#95958,1000.);
#11273=VECTOR('',#95971,1000.);
#11274=VECTOR('',#95974,1000.);
#11275=VECTOR('',#95979,1000.);
#11276=VECTOR('',#95986,1000.);
#11277=VECTOR('',#95999,1000.);
#11278=VECTOR('',#96002,1000.);
#11279=VECTOR('',#96007,1000.);
#11280=VECTOR('',#96014,1000.);
#11281=VECTOR('',#96027,1000.);
#11282=VECTOR('',#96030,1000.);
#11283=VECTOR('',#96035,1000.);
#11284=VECTOR('',#96042,1000.);
#11285=VECTOR('',#96055,1000.);
#11286=VECTOR('',#96058,1000.);
#11287=VECTOR('',#96063,1000.);
#11288=VECTOR('',#96070,1000.);
#11289=VECTOR('',#96083,1000.);
#11290=VECTOR('',#96086,1000.);
#11291=VECTOR('',#96091,1000.);
#11292=VECTOR('',#96098,1000.);
#11293=VECTOR('',#96111,1000.);
#11294=VECTOR('',#96114,1000.);
#11295=VECTOR('',#96119,1000.);
#11296=VECTOR('',#96126,1000.);
#11297=VECTOR('',#96139,1000.);
#11298=VECTOR('',#96142,1000.);
#11299=VECTOR('',#96147,1000.);
#11300=VECTOR('',#96154,1000.);
#11301=VECTOR('',#96167,1000.);
#11302=VECTOR('',#96170,1000.);
#11303=VECTOR('',#96175,1000.);
#11304=VECTOR('',#96182,1000.);
#11305=VECTOR('',#96195,1000.);
#11306=VECTOR('',#96198,1000.);
#11307=VECTOR('',#96203,1000.);
#11308=VECTOR('',#96210,1000.);
#11309=VECTOR('',#96223,1000.);
#11310=VECTOR('',#96226,1000.);
#11311=VECTOR('',#96231,1000.);
#11312=VECTOR('',#96238,1000.);
#11313=VECTOR('',#96251,1000.);
#11314=VECTOR('',#96254,1000.);
#11315=VECTOR('',#96259,1000.);
#11316=VECTOR('',#96266,1000.);
#11317=VECTOR('',#96279,1000.);
#11318=VECTOR('',#96282,1000.);
#11319=VECTOR('',#96287,1000.);
#11320=VECTOR('',#96294,1000.);
#11321=VECTOR('',#96307,1000.);
#11322=VECTOR('',#96310,1000.);
#11323=VECTOR('',#96315,1000.);
#11324=VECTOR('',#96322,1000.);
#11325=VECTOR('',#96335,1000.);
#11326=VECTOR('',#96338,1000.);
#11327=VECTOR('',#96343,1000.);
#11328=VECTOR('',#96350,1000.);
#11329=VECTOR('',#96363,1000.);
#11330=VECTOR('',#96366,1000.);
#11331=VECTOR('',#96371,1000.);
#11332=VECTOR('',#96378,1000.);
#11333=VECTOR('',#96391,1000.);
#11334=VECTOR('',#96394,1000.);
#11335=VECTOR('',#96399,1000.);
#11336=VECTOR('',#96406,1000.);
#11337=VECTOR('',#96419,1000.);
#11338=VECTOR('',#96422,1000.);
#11339=VECTOR('',#96427,1000.);
#11340=VECTOR('',#96434,1000.);
#11341=VECTOR('',#96447,1000.);
#11342=VECTOR('',#96450,1000.);
#11343=VECTOR('',#96455,1000.);
#11344=VECTOR('',#96462,1000.);
#11345=VECTOR('',#96475,1000.);
#11346=VECTOR('',#96478,1000.);
#11347=VECTOR('',#96483,1000.);
#11348=VECTOR('',#96490,1000.);
#11349=VECTOR('',#96503,1000.);
#11350=VECTOR('',#96506,1000.);
#11351=VECTOR('',#96511,1000.);
#11352=VECTOR('',#96518,1000.);
#11353=VECTOR('',#96531,1000.);
#11354=VECTOR('',#96534,1000.);
#11355=VECTOR('',#96539,1000.);
#11356=VECTOR('',#96546,1000.);
#11357=VECTOR('',#96559,1000.);
#11358=VECTOR('',#96562,1000.);
#11359=VECTOR('',#96567,1000.);
#11360=VECTOR('',#96574,1000.);
#11361=VECTOR('',#96587,1000.);
#11362=VECTOR('',#96590,1000.);
#11363=VECTOR('',#96595,1000.);
#11364=VECTOR('',#96602,1000.);
#11365=VECTOR('',#96615,1000.);
#11366=VECTOR('',#96618,1000.);
#11367=VECTOR('',#96623,1000.);
#11368=VECTOR('',#96630,1000.);
#11369=VECTOR('',#96643,1000.);
#11370=VECTOR('',#96646,1000.);
#11371=VECTOR('',#96651,1000.);
#11372=VECTOR('',#96658,1000.);
#11373=VECTOR('',#96671,1000.);
#11374=VECTOR('',#96674,1000.);
#11375=VECTOR('',#96679,1000.);
#11376=VECTOR('',#96686,1000.);
#11377=VECTOR('',#96699,1000.);
#11378=VECTOR('',#96702,1000.);
#11379=VECTOR('',#96707,1000.);
#11380=VECTOR('',#96714,1000.);
#11381=VECTOR('',#96727,1000.);
#11382=VECTOR('',#96730,1000.);
#11383=VECTOR('',#96735,1000.);
#11384=VECTOR('',#96742,1000.);
#11385=VECTOR('',#96755,1000.);
#11386=VECTOR('',#96758,1000.);
#11387=VECTOR('',#96763,1000.);
#11388=VECTOR('',#96770,1000.);
#11389=VECTOR('',#96783,1000.);
#11390=VECTOR('',#96786,1000.);
#11391=VECTOR('',#96791,1000.);
#11392=VECTOR('',#96798,1000.);
#11393=VECTOR('',#96811,1000.);
#11394=VECTOR('',#96814,1000.);
#11395=VECTOR('',#96819,1000.);
#11396=VECTOR('',#96826,1000.);
#11397=VECTOR('',#96839,1000.);
#11398=VECTOR('',#96842,1000.);
#11399=VECTOR('',#96847,1000.);
#11400=VECTOR('',#96854,1000.);
#11401=VECTOR('',#96867,1000.);
#11402=VECTOR('',#96870,1000.);
#11403=VECTOR('',#96875,1000.);
#11404=VECTOR('',#96882,1000.);
#11405=VECTOR('',#96895,1000.);
#11406=VECTOR('',#96898,1000.);
#11407=VECTOR('',#96903,1000.);
#11408=VECTOR('',#96910,1000.);
#11409=VECTOR('',#96923,1000.);
#11410=VECTOR('',#96926,1000.);
#11411=VECTOR('',#96931,1000.);
#11412=VECTOR('',#96938,1000.);
#11413=VECTOR('',#96951,1000.);
#11414=VECTOR('',#96954,1000.);
#11415=VECTOR('',#96959,1000.);
#11416=VECTOR('',#96966,1000.);
#11417=VECTOR('',#96979,1000.);
#11418=VECTOR('',#96982,1000.);
#11419=VECTOR('',#96987,1000.);
#11420=VECTOR('',#96994,1000.);
#11421=VECTOR('',#97007,1000.);
#11422=VECTOR('',#97010,1000.);
#11423=VECTOR('',#97015,1000.);
#11424=VECTOR('',#97022,1000.);
#11425=VECTOR('',#97035,1000.);
#11426=VECTOR('',#97038,1000.);
#11427=VECTOR('',#97043,1000.);
#11428=VECTOR('',#97050,1000.);
#11429=VECTOR('',#97063,1000.);
#11430=VECTOR('',#97066,1000.);
#11431=VECTOR('',#97071,1000.);
#11432=VECTOR('',#97078,1000.);
#11433=VECTOR('',#97091,1000.);
#11434=VECTOR('',#97094,1000.);
#11435=VECTOR('',#97099,1000.);
#11436=VECTOR('',#97106,1000.);
#11437=VECTOR('',#97119,1000.);
#11438=VECTOR('',#97122,1000.);
#11439=VECTOR('',#97127,1000.);
#11440=VECTOR('',#97134,1000.);
#11441=VECTOR('',#97147,1000.);
#11442=VECTOR('',#97150,1000.);
#11443=VECTOR('',#97155,1000.);
#11444=VECTOR('',#97162,1000.);
#11445=VECTOR('',#97175,1000.);
#11446=VECTOR('',#97178,1000.);
#11447=VECTOR('',#97183,1000.);
#11448=VECTOR('',#97190,1000.);
#11449=VECTOR('',#97203,1000.);
#11450=VECTOR('',#97206,1000.);
#11451=VECTOR('',#97211,1000.);
#11452=VECTOR('',#97218,1000.);
#11453=VECTOR('',#97231,1000.);
#11454=VECTOR('',#97234,1000.);
#11455=VECTOR('',#97239,1000.);
#11456=VECTOR('',#97246,1000.);
#11457=VECTOR('',#97261,1000.);
#11458=VECTOR('',#97262,1000.);
#11459=VECTOR('',#97263,1000.);
#11460=VECTOR('',#97264,1000.);
#11461=VECTOR('',#97267,1000.);
#11462=VECTOR('',#97268,1000.);
#11463=VECTOR('',#97269,1000.);
#11464=VECTOR('',#97272,1000.);
#11465=VECTOR('',#97273,1000.);
#11466=VECTOR('',#97274,1000.);
#11467=VECTOR('',#97277,1000.);
#11468=VECTOR('',#97278,1000.);
#11469=VECTOR('',#97281,1000.);
#11470=VECTOR('',#97282,1000.);
#11471=VECTOR('',#97283,1000.);
#11472=VECTOR('',#97284,1000.);
#11473=VECTOR('',#97287,1000.);
#11474=VECTOR('',#97288,1000.);
#11475=VECTOR('',#97289,1000.);
#11476=VECTOR('',#97292,1000.);
#11477=VECTOR('',#97293,1000.);
#11478=VECTOR('',#97294,1000.);
#11479=VECTOR('',#97297,1000.);
#11480=VECTOR('',#97298,1000.);
#11481=VECTOR('',#97301,1000.);
#11482=VECTOR('',#97302,1000.);
#11483=VECTOR('',#97303,1000.);
#11484=VECTOR('',#97304,1000.);
#11485=VECTOR('',#97307,1000.);
#11486=VECTOR('',#97308,1000.);
#11487=VECTOR('',#97309,1000.);
#11488=VECTOR('',#97312,1000.);
#11489=VECTOR('',#97313,1000.);
#11490=VECTOR('',#97314,1000.);
#11491=VECTOR('',#97317,1000.);
#11492=VECTOR('',#97318,1000.);
#11493=VECTOR('',#97321,1000.);
#11494=VECTOR('',#97322,1000.);
#11495=VECTOR('',#97323,1000.);
#11496=VECTOR('',#97324,1000.);
#11497=VECTOR('',#97327,1000.);
#11498=VECTOR('',#97328,1000.);
#11499=VECTOR('',#97329,1000.);
#11500=VECTOR('',#97332,1000.);
#11501=VECTOR('',#97333,1000.);
#11502=VECTOR('',#97334,1000.);
#11503=VECTOR('',#97337,1000.);
#11504=VECTOR('',#97338,1000.);
#11505=VECTOR('',#97341,1000.);
#11506=VECTOR('',#97342,1000.);
#11507=VECTOR('',#97343,1000.);
#11508=VECTOR('',#97344,1000.);
#11509=VECTOR('',#97347,1000.);
#11510=VECTOR('',#97348,1000.);
#11511=VECTOR('',#97349,1000.);
#11512=VECTOR('',#97352,1000.);
#11513=VECTOR('',#97353,1000.);
#11514=VECTOR('',#97354,1000.);
#11515=VECTOR('',#97357,1000.);
#11516=VECTOR('',#97358,1000.);
#11517=VECTOR('',#97361,1000.);
#11518=VECTOR('',#97362,1000.);
#11519=VECTOR('',#97363,1000.);
#11520=VECTOR('',#97364,1000.);
#11521=VECTOR('',#97367,1000.);
#11522=VECTOR('',#97368,1000.);
#11523=VECTOR('',#97369,1000.);
#11524=VECTOR('',#97372,1000.);
#11525=VECTOR('',#97373,1000.);
#11526=VECTOR('',#97374,1000.);
#11527=VECTOR('',#97377,1000.);
#11528=VECTOR('',#97378,1000.);
#11529=VECTOR('',#97381,1000.);
#11530=VECTOR('',#97382,1000.);
#11531=VECTOR('',#97383,1000.);
#11532=VECTOR('',#97384,1000.);
#11533=VECTOR('',#97387,1000.);
#11534=VECTOR('',#97388,1000.);
#11535=VECTOR('',#97389,1000.);
#11536=VECTOR('',#97392,1000.);
#11537=VECTOR('',#97393,1000.);
#11538=VECTOR('',#97394,1000.);
#11539=VECTOR('',#97397,1000.);
#11540=VECTOR('',#97398,1000.);
#11541=VECTOR('',#97401,1000.);
#11542=VECTOR('',#97402,1000.);
#11543=VECTOR('',#97403,1000.);
#11544=VECTOR('',#97404,1000.);
#11545=VECTOR('',#97407,1000.);
#11546=VECTOR('',#97408,1000.);
#11547=VECTOR('',#97409,1000.);
#11548=VECTOR('',#97412,1000.);
#11549=VECTOR('',#97413,1000.);
#11550=VECTOR('',#97414,1000.);
#11551=VECTOR('',#97417,1000.);
#11552=VECTOR('',#97418,1000.);
#11553=VECTOR('',#97421,1000.);
#11554=VECTOR('',#97422,1000.);
#11555=VECTOR('',#97423,1000.);
#11556=VECTOR('',#97424,1000.);
#11557=VECTOR('',#97427,1000.);
#11558=VECTOR('',#97428,1000.);
#11559=VECTOR('',#97429,1000.);
#11560=VECTOR('',#97432,1000.);
#11561=VECTOR('',#97433,1000.);
#11562=VECTOR('',#97434,1000.);
#11563=VECTOR('',#97437,1000.);
#11564=VECTOR('',#97438,1000.);
#11565=VECTOR('',#97441,1000.);
#11566=VECTOR('',#97442,1000.);
#11567=VECTOR('',#97443,1000.);
#11568=VECTOR('',#97444,1000.);
#11569=VECTOR('',#97447,1000.);
#11570=VECTOR('',#97448,1000.);
#11571=VECTOR('',#97449,1000.);
#11572=VECTOR('',#97452,1000.);
#11573=VECTOR('',#97453,1000.);
#11574=VECTOR('',#97454,1000.);
#11575=VECTOR('',#97457,1000.);
#11576=VECTOR('',#97458,1000.);
#11577=VECTOR('',#97461,1000.);
#11578=VECTOR('',#97462,1000.);
#11579=VECTOR('',#97463,1000.);
#11580=VECTOR('',#97464,1000.);
#11581=VECTOR('',#97467,1000.);
#11582=VECTOR('',#97468,1000.);
#11583=VECTOR('',#97469,1000.);
#11584=VECTOR('',#97472,1000.);
#11585=VECTOR('',#97473,1000.);
#11586=VECTOR('',#97474,1000.);
#11587=VECTOR('',#97477,1000.);
#11588=VECTOR('',#97478,1000.);
#11589=VECTOR('',#97481,1000.);
#11590=VECTOR('',#97482,1000.);
#11591=VECTOR('',#97483,1000.);
#11592=VECTOR('',#97484,1000.);
#11593=VECTOR('',#97487,1000.);
#11594=VECTOR('',#97488,1000.);
#11595=VECTOR('',#97489,1000.);
#11596=VECTOR('',#97492,1000.);
#11597=VECTOR('',#97493,1000.);
#11598=VECTOR('',#97494,1000.);
#11599=VECTOR('',#97497,1000.);
#11600=VECTOR('',#97498,1000.);
#11601=VECTOR('',#97501,1000.);
#11602=VECTOR('',#97502,1000.);
#11603=VECTOR('',#97503,1000.);
#11604=VECTOR('',#97504,1000.);
#11605=VECTOR('',#97507,1000.);
#11606=VECTOR('',#97508,1000.);
#11607=VECTOR('',#97509,1000.);
#11608=VECTOR('',#97512,1000.);
#11609=VECTOR('',#97513,1000.);
#11610=VECTOR('',#97514,1000.);
#11611=VECTOR('',#97517,1000.);
#11612=VECTOR('',#97518,1000.);
#11613=VECTOR('',#97521,1000.);
#11614=VECTOR('',#97522,1000.);
#11615=VECTOR('',#97523,1000.);
#11616=VECTOR('',#97524,1000.);
#11617=VECTOR('',#97527,1000.);
#11618=VECTOR('',#97528,1000.);
#11619=VECTOR('',#97529,1000.);
#11620=VECTOR('',#97532,1000.);
#11621=VECTOR('',#97533,1000.);
#11622=VECTOR('',#97534,1000.);
#11623=VECTOR('',#97537,1000.);
#11624=VECTOR('',#97538,1000.);
#11625=VECTOR('',#97541,1000.);
#11626=VECTOR('',#97542,1000.);
#11627=VECTOR('',#97543,1000.);
#11628=VECTOR('',#97544,1000.);
#11629=VECTOR('',#97547,1000.);
#11630=VECTOR('',#97548,1000.);
#11631=VECTOR('',#97549,1000.);
#11632=VECTOR('',#97552,1000.);
#11633=VECTOR('',#97553,1000.);
#11634=VECTOR('',#97554,1000.);
#11635=VECTOR('',#97557,1000.);
#11636=VECTOR('',#97558,1000.);
#11637=VECTOR('',#97561,1000.);
#11638=VECTOR('',#97562,1000.);
#11639=VECTOR('',#97563,1000.);
#11640=VECTOR('',#97564,1000.);
#11641=VECTOR('',#97567,1000.);
#11642=VECTOR('',#97568,1000.);
#11643=VECTOR('',#97569,1000.);
#11644=VECTOR('',#97572,1000.);
#11645=VECTOR('',#97573,1000.);
#11646=VECTOR('',#97574,1000.);
#11647=VECTOR('',#97577,1000.);
#11648=VECTOR('',#97578,1000.);
#11649=VECTOR('',#97581,1000.);
#11650=VECTOR('',#97582,1000.);
#11651=VECTOR('',#97583,1000.);
#11652=VECTOR('',#97584,1000.);
#11653=VECTOR('',#97587,1000.);
#11654=VECTOR('',#97588,1000.);
#11655=VECTOR('',#97589,1000.);
#11656=VECTOR('',#97592,1000.);
#11657=VECTOR('',#97593,1000.);
#11658=VECTOR('',#97594,1000.);
#11659=VECTOR('',#97597,1000.);
#11660=VECTOR('',#97598,1000.);
#11661=VECTOR('',#97601,1000.);
#11662=VECTOR('',#97602,1000.);
#11663=VECTOR('',#97603,1000.);
#11664=VECTOR('',#97604,1000.);
#11665=VECTOR('',#97607,1000.);
#11666=VECTOR('',#97608,1000.);
#11667=VECTOR('',#97609,1000.);
#11668=VECTOR('',#97612,1000.);
#11669=VECTOR('',#97613,1000.);
#11670=VECTOR('',#97614,1000.);
#11671=VECTOR('',#97617,1000.);
#11672=VECTOR('',#97618,1000.);
#11673=VECTOR('',#97621,1000.);
#11674=VECTOR('',#97622,1000.);
#11675=VECTOR('',#97623,1000.);
#11676=VECTOR('',#97624,1000.);
#11677=VECTOR('',#97627,1000.);
#11678=VECTOR('',#97628,1000.);
#11679=VECTOR('',#97629,1000.);
#11680=VECTOR('',#97632,1000.);
#11681=VECTOR('',#97633,1000.);
#11682=VECTOR('',#97634,1000.);
#11683=VECTOR('',#97637,1000.);
#11684=VECTOR('',#97638,1000.);
#11685=VECTOR('',#97641,1000.);
#11686=VECTOR('',#97642,1000.);
#11687=VECTOR('',#97643,1000.);
#11688=VECTOR('',#97644,1000.);
#11689=VECTOR('',#97647,1000.);
#11690=VECTOR('',#97648,1000.);
#11691=VECTOR('',#97649,1000.);
#11692=VECTOR('',#97652,1000.);
#11693=VECTOR('',#97653,1000.);
#11694=VECTOR('',#97654,1000.);
#11695=VECTOR('',#97657,1000.);
#11696=VECTOR('',#97658,1000.);
#11697=VECTOR('',#97661,1000.);
#11698=VECTOR('',#97662,1000.);
#11699=VECTOR('',#97663,1000.);
#11700=VECTOR('',#97664,1000.);
#11701=VECTOR('',#97667,1000.);
#11702=VECTOR('',#97668,1000.);
#11703=VECTOR('',#97669,1000.);
#11704=VECTOR('',#97672,1000.);
#11705=VECTOR('',#97673,1000.);
#11706=VECTOR('',#97674,1000.);
#11707=VECTOR('',#97677,1000.);
#11708=VECTOR('',#97678,1000.);
#11709=VECTOR('',#97681,1000.);
#11710=VECTOR('',#97682,1000.);
#11711=VECTOR('',#97683,1000.);
#11712=VECTOR('',#97684,1000.);
#11713=VECTOR('',#97687,1000.);
#11714=VECTOR('',#97688,1000.);
#11715=VECTOR('',#97689,1000.);
#11716=VECTOR('',#97692,1000.);
#11717=VECTOR('',#97693,1000.);
#11718=VECTOR('',#97694,1000.);
#11719=VECTOR('',#97697,1000.);
#11720=VECTOR('',#97698,1000.);
#11721=VECTOR('',#97701,1000.);
#11722=VECTOR('',#97702,1000.);
#11723=VECTOR('',#97703,1000.);
#11724=VECTOR('',#97704,1000.);
#11725=VECTOR('',#97707,1000.);
#11726=VECTOR('',#97708,1000.);
#11727=VECTOR('',#97709,1000.);
#11728=VECTOR('',#97712,1000.);
#11729=VECTOR('',#97713,1000.);
#11730=VECTOR('',#97714,1000.);
#11731=VECTOR('',#97717,1000.);
#11732=VECTOR('',#97718,1000.);
#11733=VECTOR('',#97721,1000.);
#11734=VECTOR('',#97722,1000.);
#11735=VECTOR('',#97723,1000.);
#11736=VECTOR('',#97724,1000.);
#11737=VECTOR('',#97727,1000.);
#11738=VECTOR('',#97728,1000.);
#11739=VECTOR('',#97729,1000.);
#11740=VECTOR('',#97732,1000.);
#11741=VECTOR('',#97733,1000.);
#11742=VECTOR('',#97734,1000.);
#11743=VECTOR('',#97737,1000.);
#11744=VECTOR('',#97738,1000.);
#11745=VECTOR('',#97741,1000.);
#11746=VECTOR('',#97742,1000.);
#11747=VECTOR('',#97743,1000.);
#11748=VECTOR('',#97744,1000.);
#11749=VECTOR('',#97747,1000.);
#11750=VECTOR('',#97748,1000.);
#11751=VECTOR('',#97749,1000.);
#11752=VECTOR('',#97752,1000.);
#11753=VECTOR('',#97753,1000.);
#11754=VECTOR('',#97754,1000.);
#11755=VECTOR('',#97757,1000.);
#11756=VECTOR('',#97758,1000.);
#11757=VECTOR('',#97761,1000.);
#11758=VECTOR('',#97762,1000.);
#11759=VECTOR('',#97763,1000.);
#11760=VECTOR('',#97764,1000.);
#11761=VECTOR('',#97767,1000.);
#11762=VECTOR('',#97768,1000.);
#11763=VECTOR('',#97769,1000.);
#11764=VECTOR('',#97772,1000.);
#11765=VECTOR('',#97773,1000.);
#11766=VECTOR('',#97774,1000.);
#11767=VECTOR('',#97777,1000.);
#11768=VECTOR('',#97778,1000.);
#11769=VECTOR('',#97781,1000.);
#11770=VECTOR('',#97782,1000.);
#11771=VECTOR('',#97783,1000.);
#11772=VECTOR('',#97784,1000.);
#11773=VECTOR('',#97787,1000.);
#11774=VECTOR('',#97788,1000.);
#11775=VECTOR('',#97789,1000.);
#11776=VECTOR('',#97792,1000.);
#11777=VECTOR('',#97793,1000.);
#11778=VECTOR('',#97794,1000.);
#11779=VECTOR('',#97797,1000.);
#11780=VECTOR('',#97798,1000.);
#11781=VECTOR('',#97801,1000.);
#11782=VECTOR('',#97802,1000.);
#11783=VECTOR('',#97803,1000.);
#11784=VECTOR('',#97804,1000.);
#11785=VECTOR('',#97807,1000.);
#11786=VECTOR('',#97808,1000.);
#11787=VECTOR('',#97809,1000.);
#11788=VECTOR('',#97812,1000.);
#11789=VECTOR('',#97813,1000.);
#11790=VECTOR('',#97814,1000.);
#11791=VECTOR('',#97817,1000.);
#11792=VECTOR('',#97818,1000.);
#11793=VECTOR('',#97821,1000.);
#11794=VECTOR('',#97822,1000.);
#11795=VECTOR('',#97823,1000.);
#11796=VECTOR('',#97824,1000.);
#11797=VECTOR('',#97827,1000.);
#11798=VECTOR('',#97828,1000.);
#11799=VECTOR('',#97829,1000.);
#11800=VECTOR('',#97832,1000.);
#11801=VECTOR('',#97833,1000.);
#11802=VECTOR('',#97834,1000.);
#11803=VECTOR('',#97837,1000.);
#11804=VECTOR('',#97838,1000.);
#11805=VECTOR('',#97841,1000.);
#11806=VECTOR('',#97842,1000.);
#11807=VECTOR('',#97843,1000.);
#11808=VECTOR('',#97844,1000.);
#11809=VECTOR('',#97847,1000.);
#11810=VECTOR('',#97848,1000.);
#11811=VECTOR('',#97849,1000.);
#11812=VECTOR('',#97852,1000.);
#11813=VECTOR('',#97853,1000.);
#11814=VECTOR('',#97854,1000.);
#11815=VECTOR('',#97857,1000.);
#11816=VECTOR('',#97858,1000.);
#11817=VECTOR('',#97861,1000.);
#11818=VECTOR('',#97862,1000.);
#11819=VECTOR('',#97863,1000.);
#11820=VECTOR('',#97864,1000.);
#11821=VECTOR('',#97867,1000.);
#11822=VECTOR('',#97868,1000.);
#11823=VECTOR('',#97869,1000.);
#11824=VECTOR('',#97872,1000.);
#11825=VECTOR('',#97873,1000.);
#11826=VECTOR('',#97874,1000.);
#11827=VECTOR('',#97877,1000.);
#11828=VECTOR('',#97878,1000.);
#11829=VECTOR('',#97881,1000.);
#11830=VECTOR('',#97882,1000.);
#11831=VECTOR('',#97883,1000.);
#11832=VECTOR('',#97884,1000.);
#11833=VECTOR('',#97887,1000.);
#11834=VECTOR('',#97888,1000.);
#11835=VECTOR('',#97889,1000.);
#11836=VECTOR('',#97892,1000.);
#11837=VECTOR('',#97893,1000.);
#11838=VECTOR('',#97894,1000.);
#11839=VECTOR('',#97897,1000.);
#11840=VECTOR('',#97898,1000.);
#11841=VECTOR('',#97901,1000.);
#11842=VECTOR('',#97902,1000.);
#11843=VECTOR('',#97903,1000.);
#11844=VECTOR('',#97904,1000.);
#11845=VECTOR('',#97907,1000.);
#11846=VECTOR('',#97908,1000.);
#11847=VECTOR('',#97909,1000.);
#11848=VECTOR('',#97912,1000.);
#11849=VECTOR('',#97913,1000.);
#11850=VECTOR('',#97914,1000.);
#11851=VECTOR('',#97917,1000.);
#11852=VECTOR('',#97918,1000.);
#11853=VECTOR('',#97921,1000.);
#11854=VECTOR('',#97922,1000.);
#11855=VECTOR('',#97923,1000.);
#11856=VECTOR('',#97924,1000.);
#11857=VECTOR('',#97927,1000.);
#11858=VECTOR('',#97928,1000.);
#11859=VECTOR('',#97929,1000.);
#11860=VECTOR('',#97932,1000.);
#11861=VECTOR('',#97933,1000.);
#11862=VECTOR('',#97934,1000.);
#11863=VECTOR('',#97937,1000.);
#11864=VECTOR('',#97938,1000.);
#11865=VECTOR('',#97941,1000.);
#11866=VECTOR('',#97942,1000.);
#11867=VECTOR('',#97943,1000.);
#11868=VECTOR('',#97944,1000.);
#11869=VECTOR('',#97947,1000.);
#11870=VECTOR('',#97948,1000.);
#11871=VECTOR('',#97949,1000.);
#11872=VECTOR('',#97952,1000.);
#11873=VECTOR('',#97953,1000.);
#11874=VECTOR('',#97954,1000.);
#11875=VECTOR('',#97957,1000.);
#11876=VECTOR('',#97958,1000.);
#11877=VECTOR('',#97961,1000.);
#11878=VECTOR('',#97962,1000.);
#11879=VECTOR('',#97963,1000.);
#11880=VECTOR('',#97964,1000.);
#11881=VECTOR('',#97967,1000.);
#11882=VECTOR('',#97968,1000.);
#11883=VECTOR('',#97969,1000.);
#11884=VECTOR('',#97972,1000.);
#11885=VECTOR('',#97973,1000.);
#11886=VECTOR('',#97974,1000.);
#11887=VECTOR('',#97977,1000.);
#11888=VECTOR('',#97978,1000.);
#11889=VECTOR('',#97981,1000.);
#11890=VECTOR('',#97982,1000.);
#11891=VECTOR('',#97983,1000.);
#11892=VECTOR('',#97984,1000.);
#11893=VECTOR('',#97987,1000.);
#11894=VECTOR('',#97988,1000.);
#11895=VECTOR('',#97989,1000.);
#11896=VECTOR('',#97992,1000.);
#11897=VECTOR('',#97993,1000.);
#11898=VECTOR('',#97994,1000.);
#11899=VECTOR('',#97997,1000.);
#11900=VECTOR('',#97998,1000.);
#11901=VECTOR('',#98001,1000.);
#11902=VECTOR('',#98002,1000.);
#11903=VECTOR('',#98003,1000.);
#11904=VECTOR('',#98004,1000.);
#11905=VECTOR('',#98007,1000.);
#11906=VECTOR('',#98008,1000.);
#11907=VECTOR('',#98009,1000.);
#11908=VECTOR('',#98012,1000.);
#11909=VECTOR('',#98013,1000.);
#11910=VECTOR('',#98014,1000.);
#11911=VECTOR('',#98017,1000.);
#11912=VECTOR('',#98018,1000.);
#11913=VECTOR('',#98021,1000.);
#11914=VECTOR('',#98022,1000.);
#11915=VECTOR('',#98023,1000.);
#11916=VECTOR('',#98024,1000.);
#11917=VECTOR('',#98027,1000.);
#11918=VECTOR('',#98028,1000.);
#11919=VECTOR('',#98029,1000.);
#11920=VECTOR('',#98032,1000.);
#11921=VECTOR('',#98033,1000.);
#11922=VECTOR('',#98034,1000.);
#11923=VECTOR('',#98037,1000.);
#11924=VECTOR('',#98038,1000.);
#11925=VECTOR('',#98041,1000.);
#11926=VECTOR('',#98042,1000.);
#11927=VECTOR('',#98043,1000.);
#11928=VECTOR('',#98044,1000.);
#11929=VECTOR('',#98047,1000.);
#11930=VECTOR('',#98048,1000.);
#11931=VECTOR('',#98049,1000.);
#11932=VECTOR('',#98052,1000.);
#11933=VECTOR('',#98053,1000.);
#11934=VECTOR('',#98054,1000.);
#11935=VECTOR('',#98057,1000.);
#11936=VECTOR('',#98058,1000.);
#11937=VECTOR('',#98061,1000.);
#11938=VECTOR('',#98062,1000.);
#11939=VECTOR('',#98063,1000.);
#11940=VECTOR('',#98064,1000.);
#11941=VECTOR('',#98067,1000.);
#11942=VECTOR('',#98068,1000.);
#11943=VECTOR('',#98069,1000.);
#11944=VECTOR('',#98072,1000.);
#11945=VECTOR('',#98073,1000.);
#11946=VECTOR('',#98074,1000.);
#11947=VECTOR('',#98077,1000.);
#11948=VECTOR('',#98078,1000.);
#11949=VECTOR('',#98081,1000.);
#11950=VECTOR('',#98082,1000.);
#11951=VECTOR('',#98083,1000.);
#11952=VECTOR('',#98084,1000.);
#11953=VECTOR('',#98087,1000.);
#11954=VECTOR('',#98088,1000.);
#11955=VECTOR('',#98089,1000.);
#11956=VECTOR('',#98092,1000.);
#11957=VECTOR('',#98093,1000.);
#11958=VECTOR('',#98094,1000.);
#11959=VECTOR('',#98097,1000.);
#11960=VECTOR('',#98098,1000.);
#11961=VECTOR('',#98101,1000.);
#11962=VECTOR('',#98102,1000.);
#11963=VECTOR('',#98103,1000.);
#11964=VECTOR('',#98104,1000.);
#11965=VECTOR('',#98107,1000.);
#11966=VECTOR('',#98108,1000.);
#11967=VECTOR('',#98109,1000.);
#11968=VECTOR('',#98112,1000.);
#11969=VECTOR('',#98113,1000.);
#11970=VECTOR('',#98114,1000.);
#11971=VECTOR('',#98117,1000.);
#11972=VECTOR('',#98118,1000.);
#11973=VECTOR('',#98121,1000.);
#11974=VECTOR('',#98122,1000.);
#11975=VECTOR('',#98123,1000.);
#11976=VECTOR('',#98124,1000.);
#11977=VECTOR('',#98127,1000.);
#11978=VECTOR('',#98128,1000.);
#11979=VECTOR('',#98129,1000.);
#11980=VECTOR('',#98132,1000.);
#11981=VECTOR('',#98133,1000.);
#11982=VECTOR('',#98134,1000.);
#11983=VECTOR('',#98137,1000.);
#11984=VECTOR('',#98138,1000.);
#11985=VECTOR('',#98141,1000.);
#11986=VECTOR('',#98142,1000.);
#11987=VECTOR('',#98143,1000.);
#11988=VECTOR('',#98144,1000.);
#11989=VECTOR('',#98147,1000.);
#11990=VECTOR('',#98148,1000.);
#11991=VECTOR('',#98149,1000.);
#11992=VECTOR('',#98152,1000.);
#11993=VECTOR('',#98153,1000.);
#11994=VECTOR('',#98154,1000.);
#11995=VECTOR('',#98157,1000.);
#11996=VECTOR('',#98158,1000.);
#11997=VECTOR('',#98161,1000.);
#11998=VECTOR('',#98162,1000.);
#11999=VECTOR('',#98163,1000.);
#12000=VECTOR('',#98164,1000.);
#12001=VECTOR('',#98167,1000.);
#12002=VECTOR('',#98168,1000.);
#12003=VECTOR('',#98169,1000.);
#12004=VECTOR('',#98172,1000.);
#12005=VECTOR('',#98173,1000.);
#12006=VECTOR('',#98174,1000.);
#12007=VECTOR('',#98177,1000.);
#12008=VECTOR('',#98178,1000.);
#12009=VECTOR('',#98181,1000.);
#12010=VECTOR('',#98182,1000.);
#12011=VECTOR('',#98183,1000.);
#12012=VECTOR('',#98184,1000.);
#12013=VECTOR('',#98187,1000.);
#12014=VECTOR('',#98188,1000.);
#12015=VECTOR('',#98189,1000.);
#12016=VECTOR('',#98192,1000.);
#12017=VECTOR('',#98193,1000.);
#12018=VECTOR('',#98194,1000.);
#12019=VECTOR('',#98197,1000.);
#12020=VECTOR('',#98198,1000.);
#12021=VECTOR('',#98201,1000.);
#12022=VECTOR('',#98202,1000.);
#12023=VECTOR('',#98203,1000.);
#12024=VECTOR('',#98204,1000.);
#12025=VECTOR('',#98207,1000.);
#12026=VECTOR('',#98208,1000.);
#12027=VECTOR('',#98209,1000.);
#12028=VECTOR('',#98212,1000.);
#12029=VECTOR('',#98213,1000.);
#12030=VECTOR('',#98214,1000.);
#12031=VECTOR('',#98217,1000.);
#12032=VECTOR('',#98218,1000.);
#12033=VECTOR('',#98221,1000.);
#12034=VECTOR('',#98222,1000.);
#12035=VECTOR('',#98223,1000.);
#12036=VECTOR('',#98224,1000.);
#12037=VECTOR('',#98227,1000.);
#12038=VECTOR('',#98228,1000.);
#12039=VECTOR('',#98229,1000.);
#12040=VECTOR('',#98232,1000.);
#12041=VECTOR('',#98233,1000.);
#12042=VECTOR('',#98234,1000.);
#12043=VECTOR('',#98237,1000.);
#12044=VECTOR('',#98238,1000.);
#12045=VECTOR('',#98241,1000.);
#12046=VECTOR('',#98242,1000.);
#12047=VECTOR('',#98243,1000.);
#12048=VECTOR('',#98244,1000.);
#12049=VECTOR('',#98247,1000.);
#12050=VECTOR('',#98248,1000.);
#12051=VECTOR('',#98249,1000.);
#12052=VECTOR('',#98252,1000.);
#12053=VECTOR('',#98253,1000.);
#12054=VECTOR('',#98254,1000.);
#12055=VECTOR('',#98257,1000.);
#12056=VECTOR('',#98258,1000.);
#12057=VECTOR('',#98261,1000.);
#12058=VECTOR('',#98262,1000.);
#12059=VECTOR('',#98263,1000.);
#12060=VECTOR('',#98264,1000.);
#12061=VECTOR('',#98267,1000.);
#12062=VECTOR('',#98268,1000.);
#12063=VECTOR('',#98269,1000.);
#12064=VECTOR('',#98272,1000.);
#12065=VECTOR('',#98273,1000.);
#12066=VECTOR('',#98274,1000.);
#12067=VECTOR('',#98277,1000.);
#12068=VECTOR('',#98278,1000.);
#12069=VECTOR('',#98281,1000.);
#12070=VECTOR('',#98282,1000.);
#12071=VECTOR('',#98283,1000.);
#12072=VECTOR('',#98284,1000.);
#12073=VECTOR('',#98287,1000.);
#12074=VECTOR('',#98288,1000.);
#12075=VECTOR('',#98289,1000.);
#12076=VECTOR('',#98292,1000.);
#12077=VECTOR('',#98293,1000.);
#12078=VECTOR('',#98294,1000.);
#12079=VECTOR('',#98297,1000.);
#12080=VECTOR('',#98298,1000.);
#12081=VECTOR('',#98301,1000.);
#12082=VECTOR('',#98302,1000.);
#12083=VECTOR('',#98303,1000.);
#12084=VECTOR('',#98304,1000.);
#12085=VECTOR('',#98307,1000.);
#12086=VECTOR('',#98308,1000.);
#12087=VECTOR('',#98309,1000.);
#12088=VECTOR('',#98312,1000.);
#12089=VECTOR('',#98313,1000.);
#12090=VECTOR('',#98314,1000.);
#12091=VECTOR('',#98317,1000.);
#12092=VECTOR('',#98318,1000.);
#12093=VECTOR('',#98321,1000.);
#12094=VECTOR('',#98322,1000.);
#12095=VECTOR('',#98323,1000.);
#12096=VECTOR('',#98324,1000.);
#12097=VECTOR('',#98327,1000.);
#12098=VECTOR('',#98328,1000.);
#12099=VECTOR('',#98329,1000.);
#12100=VECTOR('',#98332,1000.);
#12101=VECTOR('',#98333,1000.);
#12102=VECTOR('',#98334,1000.);
#12103=VECTOR('',#98337,1000.);
#12104=VECTOR('',#98338,1000.);
#12105=VECTOR('',#98341,1000.);
#12106=VECTOR('',#98342,1000.);
#12107=VECTOR('',#98343,1000.);
#12108=VECTOR('',#98344,1000.);
#12109=VECTOR('',#98347,1000.);
#12110=VECTOR('',#98348,1000.);
#12111=VECTOR('',#98349,1000.);
#12112=VECTOR('',#98352,1000.);
#12113=VECTOR('',#98353,1000.);
#12114=VECTOR('',#98354,1000.);
#12115=VECTOR('',#98357,1000.);
#12116=VECTOR('',#98358,1000.);
#12117=VECTOR('',#98361,1000.);
#12118=VECTOR('',#98362,1000.);
#12119=VECTOR('',#98363,1000.);
#12120=VECTOR('',#98364,1000.);
#12121=VECTOR('',#98367,1000.);
#12122=VECTOR('',#98368,1000.);
#12123=VECTOR('',#98369,1000.);
#12124=VECTOR('',#98372,1000.);
#12125=VECTOR('',#98373,1000.);
#12126=VECTOR('',#98374,1000.);
#12127=VECTOR('',#98377,1000.);
#12128=VECTOR('',#98378,1000.);
#12129=VECTOR('',#98381,1000.);
#12130=VECTOR('',#98382,1000.);
#12131=VECTOR('',#98383,1000.);
#12132=VECTOR('',#98384,1000.);
#12133=VECTOR('',#98387,1000.);
#12134=VECTOR('',#98388,1000.);
#12135=VECTOR('',#98389,1000.);
#12136=VECTOR('',#98392,1000.);
#12137=VECTOR('',#98393,1000.);
#12138=VECTOR('',#98394,1000.);
#12139=VECTOR('',#98397,1000.);
#12140=VECTOR('',#98398,1000.);
#12141=VECTOR('',#98401,1000.);
#12142=VECTOR('',#98402,1000.);
#12143=VECTOR('',#98403,1000.);
#12144=VECTOR('',#98404,1000.);
#12145=VECTOR('',#98407,1000.);
#12146=VECTOR('',#98408,1000.);
#12147=VECTOR('',#98409,1000.);
#12148=VECTOR('',#98412,1000.);
#12149=VECTOR('',#98413,1000.);
#12150=VECTOR('',#98414,1000.);
#12151=VECTOR('',#98417,1000.);
#12152=VECTOR('',#98418,1000.);
#12153=VECTOR('',#98421,1000.);
#12154=VECTOR('',#98422,1000.);
#12155=VECTOR('',#98423,1000.);
#12156=VECTOR('',#98424,1000.);
#12157=VECTOR('',#98427,1000.);
#12158=VECTOR('',#98428,1000.);
#12159=VECTOR('',#98429,1000.);
#12160=VECTOR('',#98432,1000.);
#12161=VECTOR('',#98433,1000.);
#12162=VECTOR('',#98434,1000.);
#12163=VECTOR('',#98437,1000.);
#12164=VECTOR('',#98438,1000.);
#12165=VECTOR('',#98441,1000.);
#12166=VECTOR('',#98442,1000.);
#12167=VECTOR('',#98443,1000.);
#12168=VECTOR('',#98444,1000.);
#12169=VECTOR('',#98447,1000.);
#12170=VECTOR('',#98448,1000.);
#12171=VECTOR('',#98449,1000.);
#12172=VECTOR('',#98452,1000.);
#12173=VECTOR('',#98453,1000.);
#12174=VECTOR('',#98454,1000.);
#12175=VECTOR('',#98457,1000.);
#12176=VECTOR('',#98458,1000.);
#12177=VECTOR('',#98461,1000.);
#12178=VECTOR('',#98462,1000.);
#12179=VECTOR('',#98463,1000.);
#12180=VECTOR('',#98464,1000.);
#12181=VECTOR('',#98467,1000.);
#12182=VECTOR('',#98468,1000.);
#12183=VECTOR('',#98469,1000.);
#12184=VECTOR('',#98472,1000.);
#12185=VECTOR('',#98473,1000.);
#12186=VECTOR('',#98474,1000.);
#12187=VECTOR('',#98477,1000.);
#12188=VECTOR('',#98478,1000.);
#12189=VECTOR('',#98481,1000.);
#12190=VECTOR('',#98482,1000.);
#12191=VECTOR('',#98483,1000.);
#12192=VECTOR('',#98484,1000.);
#12193=VECTOR('',#98487,1000.);
#12194=VECTOR('',#98488,1000.);
#12195=VECTOR('',#98489,1000.);
#12196=VECTOR('',#98492,1000.);
#12197=VECTOR('',#98493,1000.);
#12198=VECTOR('',#98494,1000.);
#12199=VECTOR('',#98497,1000.);
#12200=VECTOR('',#98498,1000.);
#12201=VECTOR('',#98501,1000.);
#12202=VECTOR('',#98502,1000.);
#12203=VECTOR('',#98503,1000.);
#12204=VECTOR('',#98504,1000.);
#12205=VECTOR('',#98507,1000.);
#12206=VECTOR('',#98508,1000.);
#12207=VECTOR('',#98509,1000.);
#12208=VECTOR('',#98512,1000.);
#12209=VECTOR('',#98513,1000.);
#12210=VECTOR('',#98514,1000.);
#12211=VECTOR('',#98517,1000.);
#12212=VECTOR('',#98518,1000.);
#12213=VECTOR('',#98521,1000.);
#12214=VECTOR('',#98522,1000.);
#12215=VECTOR('',#98523,1000.);
#12216=VECTOR('',#98524,1000.);
#12217=VECTOR('',#98527,1000.);
#12218=VECTOR('',#98528,1000.);
#12219=VECTOR('',#98529,1000.);
#12220=VECTOR('',#98532,1000.);
#12221=VECTOR('',#98533,1000.);
#12222=VECTOR('',#98534,1000.);
#12223=VECTOR('',#98537,1000.);
#12224=VECTOR('',#98538,1000.);
#12225=VECTOR('',#98541,1000.);
#12226=VECTOR('',#98542,1000.);
#12227=VECTOR('',#98543,1000.);
#12228=VECTOR('',#98544,1000.);
#12229=VECTOR('',#98547,1000.);
#12230=VECTOR('',#98548,1000.);
#12231=VECTOR('',#98549,1000.);
#12232=VECTOR('',#98552,1000.);
#12233=VECTOR('',#98553,1000.);
#12234=VECTOR('',#98554,1000.);
#12235=VECTOR('',#98557,1000.);
#12236=VECTOR('',#98558,1000.);
#12237=VECTOR('',#98561,1000.);
#12238=VECTOR('',#98562,1000.);
#12239=VECTOR('',#98563,1000.);
#12240=VECTOR('',#98564,1000.);
#12241=VECTOR('',#98567,1000.);
#12242=VECTOR('',#98568,1000.);
#12243=VECTOR('',#98569,1000.);
#12244=VECTOR('',#98572,1000.);
#12245=VECTOR('',#98573,1000.);
#12246=VECTOR('',#98574,1000.);
#12247=VECTOR('',#98577,1000.);
#12248=VECTOR('',#98578,1000.);
#12249=VECTOR('',#98581,1000.);
#12250=VECTOR('',#98582,1000.);
#12251=VECTOR('',#98583,1000.);
#12252=VECTOR('',#98584,1000.);
#12253=VECTOR('',#98587,1000.);
#12254=VECTOR('',#98588,1000.);
#12255=VECTOR('',#98589,1000.);
#12256=VECTOR('',#98592,1000.);
#12257=VECTOR('',#98593,1000.);
#12258=VECTOR('',#98594,1000.);
#12259=VECTOR('',#98597,1000.);
#12260=VECTOR('',#98598,1000.);
#12261=VECTOR('',#98601,1000.);
#12262=VECTOR('',#98602,1000.);
#12263=VECTOR('',#98603,1000.);
#12264=VECTOR('',#98604,1000.);
#12265=VECTOR('',#98607,1000.);
#12266=VECTOR('',#98608,1000.);
#12267=VECTOR('',#98609,1000.);
#12268=VECTOR('',#98612,1000.);
#12269=VECTOR('',#98613,1000.);
#12270=VECTOR('',#98614,1000.);
#12271=VECTOR('',#98617,1000.);
#12272=VECTOR('',#98618,1000.);
#12273=VECTOR('',#98621,1000.);
#12274=VECTOR('',#98622,1000.);
#12275=VECTOR('',#98623,1000.);
#12276=VECTOR('',#98624,1000.);
#12277=VECTOR('',#98627,1000.);
#12278=VECTOR('',#98628,1000.);
#12279=VECTOR('',#98629,1000.);
#12280=VECTOR('',#98632,1000.);
#12281=VECTOR('',#98633,1000.);
#12282=VECTOR('',#98634,1000.);
#12283=VECTOR('',#98637,1000.);
#12284=VECTOR('',#98638,1000.);
#12285=VECTOR('',#98641,1000.);
#12286=VECTOR('',#98642,1000.);
#12287=VECTOR('',#98643,1000.);
#12288=VECTOR('',#98644,1000.);
#12289=VECTOR('',#98647,1000.);
#12290=VECTOR('',#98648,1000.);
#12291=VECTOR('',#98649,1000.);
#12292=VECTOR('',#98652,1000.);
#12293=VECTOR('',#98653,1000.);
#12294=VECTOR('',#98654,1000.);
#12295=VECTOR('',#98657,1000.);
#12296=VECTOR('',#98658,1000.);
#12297=VECTOR('',#98661,1000.);
#12298=VECTOR('',#98662,1000.);
#12299=VECTOR('',#98663,1000.);
#12300=VECTOR('',#98664,1000.);
#12301=VECTOR('',#98667,1000.);
#12302=VECTOR('',#98668,1000.);
#12303=VECTOR('',#98669,1000.);
#12304=VECTOR('',#98672,1000.);
#12305=VECTOR('',#98673,1000.);
#12306=VECTOR('',#98674,1000.);
#12307=VECTOR('',#98677,1000.);
#12308=VECTOR('',#98678,1000.);
#12309=VECTOR('',#98681,1000.);
#12310=VECTOR('',#98682,1000.);
#12311=VECTOR('',#98683,1000.);
#12312=VECTOR('',#98684,1000.);
#12313=VECTOR('',#98687,1000.);
#12314=VECTOR('',#98688,1000.);
#12315=VECTOR('',#98689,1000.);
#12316=VECTOR('',#98692,1000.);
#12317=VECTOR('',#98693,1000.);
#12318=VECTOR('',#98694,1000.);
#12319=VECTOR('',#98697,1000.);
#12320=VECTOR('',#98698,1000.);
#12321=VECTOR('',#98701,1000.);
#12322=VECTOR('',#98702,1000.);
#12323=VECTOR('',#98703,1000.);
#12324=VECTOR('',#98704,1000.);
#12325=VECTOR('',#98707,1000.);
#12326=VECTOR('',#98708,1000.);
#12327=VECTOR('',#98709,1000.);
#12328=VECTOR('',#98712,1000.);
#12329=VECTOR('',#98713,1000.);
#12330=VECTOR('',#98714,1000.);
#12331=VECTOR('',#98717,1000.);
#12332=VECTOR('',#98718,1000.);
#12333=VECTOR('',#98721,1000.);
#12334=VECTOR('',#98722,1000.);
#12335=VECTOR('',#98723,1000.);
#12336=VECTOR('',#98724,1000.);
#12337=VECTOR('',#98727,1000.);
#12338=VECTOR('',#98728,1000.);
#12339=VECTOR('',#98729,1000.);
#12340=VECTOR('',#98732,1000.);
#12341=VECTOR('',#98733,1000.);
#12342=VECTOR('',#98734,1000.);
#12343=VECTOR('',#98737,1000.);
#12344=VECTOR('',#98738,1000.);
#12345=VECTOR('',#98741,1000.);
#12346=VECTOR('',#98742,1000.);
#12347=VECTOR('',#98743,1000.);
#12348=VECTOR('',#98744,1000.);
#12349=VECTOR('',#98747,1000.);
#12350=VECTOR('',#98748,1000.);
#12351=VECTOR('',#98749,1000.);
#12352=VECTOR('',#98752,1000.);
#12353=VECTOR('',#98753,1000.);
#12354=VECTOR('',#98754,1000.);
#12355=VECTOR('',#98757,1000.);
#12356=VECTOR('',#98758,1000.);
#12357=VECTOR('',#98761,1000.);
#12358=VECTOR('',#98762,1000.);
#12359=VECTOR('',#98763,1000.);
#12360=VECTOR('',#98764,1000.);
#12361=VECTOR('',#98767,1000.);
#12362=VECTOR('',#98768,1000.);
#12363=VECTOR('',#98769,1000.);
#12364=VECTOR('',#98772,1000.);
#12365=VECTOR('',#98773,1000.);
#12366=VECTOR('',#98774,1000.);
#12367=VECTOR('',#98777,1000.);
#12368=VECTOR('',#98778,1000.);
#12369=VECTOR('',#98781,1000.);
#12370=VECTOR('',#98782,1000.);
#12371=VECTOR('',#98783,1000.);
#12372=VECTOR('',#98784,1000.);
#12373=VECTOR('',#98787,1000.);
#12374=VECTOR('',#98788,1000.);
#12375=VECTOR('',#98789,1000.);
#12376=VECTOR('',#98792,1000.);
#12377=VECTOR('',#98793,1000.);
#12378=VECTOR('',#98794,1000.);
#12379=VECTOR('',#98797,1000.);
#12380=VECTOR('',#98798,1000.);
#12381=VECTOR('',#98801,1000.);
#12382=VECTOR('',#98802,1000.);
#12383=VECTOR('',#98803,1000.);
#12384=VECTOR('',#98804,1000.);
#12385=VECTOR('',#98807,1000.);
#12386=VECTOR('',#98808,1000.);
#12387=VECTOR('',#98809,1000.);
#12388=VECTOR('',#98812,1000.);
#12389=VECTOR('',#98813,1000.);
#12390=VECTOR('',#98814,1000.);
#12391=VECTOR('',#98817,1000.);
#12392=VECTOR('',#98818,1000.);
#12393=VECTOR('',#98821,1000.);
#12394=VECTOR('',#98822,1000.);
#12395=VECTOR('',#98823,1000.);
#12396=VECTOR('',#98824,1000.);
#12397=VECTOR('',#98827,1000.);
#12398=VECTOR('',#98828,1000.);
#12399=VECTOR('',#98829,1000.);
#12400=VECTOR('',#98832,1000.);
#12401=VECTOR('',#98833,1000.);
#12402=VECTOR('',#98834,1000.);
#12403=VECTOR('',#98837,1000.);
#12404=VECTOR('',#98838,1000.);
#12405=VECTOR('',#98841,1000.);
#12406=VECTOR('',#98842,1000.);
#12407=VECTOR('',#98843,1000.);
#12408=VECTOR('',#98844,1000.);
#12409=VECTOR('',#98847,1000.);
#12410=VECTOR('',#98848,1000.);
#12411=VECTOR('',#98849,1000.);
#12412=VECTOR('',#98852,1000.);
#12413=VECTOR('',#98853,1000.);
#12414=VECTOR('',#98854,1000.);
#12415=VECTOR('',#98857,1000.);
#12416=VECTOR('',#98858,1000.);
#12417=VECTOR('',#98861,1000.);
#12418=VECTOR('',#98862,1000.);
#12419=VECTOR('',#98863,1000.);
#12420=VECTOR('',#98864,1000.);
#12421=VECTOR('',#98867,1000.);
#12422=VECTOR('',#98868,1000.);
#12423=VECTOR('',#98869,1000.);
#12424=VECTOR('',#98872,1000.);
#12425=VECTOR('',#98873,1000.);
#12426=VECTOR('',#98874,1000.);
#12427=VECTOR('',#98877,1000.);
#12428=VECTOR('',#98878,1000.);
#12429=VECTOR('',#98881,1000.);
#12430=VECTOR('',#98882,1000.);
#12431=VECTOR('',#98883,1000.);
#12432=VECTOR('',#98884,1000.);
#12433=VECTOR('',#98887,1000.);
#12434=VECTOR('',#98888,1000.);
#12435=VECTOR('',#98889,1000.);
#12436=VECTOR('',#98892,1000.);
#12437=VECTOR('',#98893,1000.);
#12438=VECTOR('',#98894,1000.);
#12439=VECTOR('',#98897,1000.);
#12440=VECTOR('',#98898,1000.);
#12441=VECTOR('',#98901,1000.);
#12442=VECTOR('',#98902,1000.);
#12443=VECTOR('',#98903,1000.);
#12444=VECTOR('',#98904,1000.);
#12445=VECTOR('',#98907,1000.);
#12446=VECTOR('',#98908,1000.);
#12447=VECTOR('',#98909,1000.);
#12448=VECTOR('',#98912,1000.);
#12449=VECTOR('',#98913,1000.);
#12450=VECTOR('',#98914,1000.);
#12451=VECTOR('',#98917,1000.);
#12452=VECTOR('',#98918,1000.);
#12453=VECTOR('',#98921,1000.);
#12454=VECTOR('',#98922,1000.);
#12455=VECTOR('',#98923,1000.);
#12456=VECTOR('',#98924,1000.);
#12457=VECTOR('',#98927,1000.);
#12458=VECTOR('',#98928,1000.);
#12459=VECTOR('',#98929,1000.);
#12460=VECTOR('',#98932,1000.);
#12461=VECTOR('',#98933,1000.);
#12462=VECTOR('',#98934,1000.);
#12463=VECTOR('',#98937,1000.);
#12464=VECTOR('',#98938,1000.);
#12465=VECTOR('',#98941,1000.);
#12466=VECTOR('',#98942,1000.);
#12467=VECTOR('',#98943,1000.);
#12468=VECTOR('',#98944,1000.);
#12469=VECTOR('',#98947,1000.);
#12470=VECTOR('',#98948,1000.);
#12471=VECTOR('',#98949,1000.);
#12472=VECTOR('',#98952,1000.);
#12473=VECTOR('',#98953,1000.);
#12474=VECTOR('',#98954,1000.);
#12475=VECTOR('',#98957,1000.);
#12476=VECTOR('',#98958,1000.);
#12477=VECTOR('',#98961,1000.);
#12478=VECTOR('',#98962,1000.);
#12479=VECTOR('',#98963,1000.);
#12480=VECTOR('',#98964,1000.);
#12481=VECTOR('',#98967,1000.);
#12482=VECTOR('',#98968,1000.);
#12483=VECTOR('',#98969,1000.);
#12484=VECTOR('',#98972,1000.);
#12485=VECTOR('',#98973,1000.);
#12486=VECTOR('',#98974,1000.);
#12487=VECTOR('',#98977,1000.);
#12488=VECTOR('',#98978,1000.);
#12489=VECTOR('',#98981,1000.);
#12490=VECTOR('',#98982,1000.);
#12491=VECTOR('',#98983,1000.);
#12492=VECTOR('',#98984,1000.);
#12493=VECTOR('',#98987,1000.);
#12494=VECTOR('',#98988,1000.);
#12495=VECTOR('',#98989,1000.);
#12496=VECTOR('',#98992,1000.);
#12497=VECTOR('',#98993,1000.);
#12498=VECTOR('',#98994,1000.);
#12499=VECTOR('',#98997,1000.);
#12500=VECTOR('',#98998,1000.);
#12501=VECTOR('',#99001,1000.);
#12502=VECTOR('',#99002,1000.);
#12503=VECTOR('',#99003,1000.);
#12504=VECTOR('',#99004,1000.);
#12505=VECTOR('',#99007,1000.);
#12506=VECTOR('',#99008,1000.);
#12507=VECTOR('',#99009,1000.);
#12508=VECTOR('',#99012,1000.);
#12509=VECTOR('',#99013,1000.);
#12510=VECTOR('',#99014,1000.);
#12511=VECTOR('',#99017,1000.);
#12512=VECTOR('',#99018,1000.);
#12513=VECTOR('',#99021,1000.);
#12514=VECTOR('',#99022,1000.);
#12515=VECTOR('',#99023,1000.);
#12516=VECTOR('',#99024,1000.);
#12517=VECTOR('',#99027,1000.);
#12518=VECTOR('',#99028,1000.);
#12519=VECTOR('',#99029,1000.);
#12520=VECTOR('',#99032,1000.);
#12521=VECTOR('',#99033,1000.);
#12522=VECTOR('',#99034,1000.);
#12523=VECTOR('',#99037,1000.);
#12524=VECTOR('',#99038,1000.);
#12525=VECTOR('',#99041,1000.);
#12526=VECTOR('',#99042,1000.);
#12527=VECTOR('',#99043,1000.);
#12528=VECTOR('',#99044,1000.);
#12529=VECTOR('',#99047,1000.);
#12530=VECTOR('',#99048,1000.);
#12531=VECTOR('',#99049,1000.);
#12532=VECTOR('',#99052,1000.);
#12533=VECTOR('',#99053,1000.);
#12534=VECTOR('',#99054,1000.);
#12535=VECTOR('',#99057,1000.);
#12536=VECTOR('',#99058,1000.);
#12537=VECTOR('',#99061,1000.);
#12538=VECTOR('',#99062,1000.);
#12539=VECTOR('',#99063,1000.);
#12540=VECTOR('',#99064,1000.);
#12541=VECTOR('',#99067,1000.);
#12542=VECTOR('',#99068,1000.);
#12543=VECTOR('',#99069,1000.);
#12544=VECTOR('',#99072,1000.);
#12545=VECTOR('',#99073,1000.);
#12546=VECTOR('',#99074,1000.);
#12547=VECTOR('',#99077,1000.);
#12548=VECTOR('',#99078,1000.);
#12549=VECTOR('',#99081,1000.);
#12550=VECTOR('',#99082,1000.);
#12551=VECTOR('',#99083,1000.);
#12552=VECTOR('',#99084,1000.);
#12553=VECTOR('',#99087,1000.);
#12554=VECTOR('',#99088,1000.);
#12555=VECTOR('',#99089,1000.);
#12556=VECTOR('',#99092,1000.);
#12557=VECTOR('',#99093,1000.);
#12558=VECTOR('',#99094,1000.);
#12559=VECTOR('',#99097,1000.);
#12560=VECTOR('',#99098,1000.);
#12561=VECTOR('',#99101,1000.);
#12562=VECTOR('',#99102,1000.);
#12563=VECTOR('',#99103,1000.);
#12564=VECTOR('',#99104,1000.);
#12565=VECTOR('',#99107,1000.);
#12566=VECTOR('',#99108,1000.);
#12567=VECTOR('',#99109,1000.);
#12568=VECTOR('',#99112,1000.);
#12569=VECTOR('',#99113,1000.);
#12570=VECTOR('',#99114,1000.);
#12571=VECTOR('',#99117,1000.);
#12572=VECTOR('',#99118,1000.);
#12573=VECTOR('',#99121,1000.);
#12574=VECTOR('',#99122,1000.);
#12575=VECTOR('',#99123,1000.);
#12576=VECTOR('',#99124,1000.);
#12577=VECTOR('',#99127,1000.);
#12578=VECTOR('',#99128,1000.);
#12579=VECTOR('',#99129,1000.);
#12580=VECTOR('',#99132,1000.);
#12581=VECTOR('',#99133,1000.);
#12582=VECTOR('',#99134,1000.);
#12583=VECTOR('',#99137,1000.);
#12584=VECTOR('',#99138,1000.);
#12585=VECTOR('',#99141,1000.);
#12586=VECTOR('',#99142,1000.);
#12587=VECTOR('',#99143,1000.);
#12588=VECTOR('',#99144,1000.);
#12589=VECTOR('',#99147,1000.);
#12590=VECTOR('',#99148,1000.);
#12591=VECTOR('',#99149,1000.);
#12592=VECTOR('',#99152,1000.);
#12593=VECTOR('',#99153,1000.);
#12594=VECTOR('',#99154,1000.);
#12595=VECTOR('',#99157,1000.);
#12596=VECTOR('',#99158,1000.);
#12597=VECTOR('',#99161,1000.);
#12598=VECTOR('',#99162,1000.);
#12599=VECTOR('',#99163,1000.);
#12600=VECTOR('',#99164,1000.);
#12601=VECTOR('',#99167,1000.);
#12602=VECTOR('',#99168,1000.);
#12603=VECTOR('',#99169,1000.);
#12604=VECTOR('',#99172,1000.);
#12605=VECTOR('',#99173,1000.);
#12606=VECTOR('',#99174,1000.);
#12607=VECTOR('',#99177,1000.);
#12608=VECTOR('',#99178,1000.);
#12609=VECTOR('',#99181,1000.);
#12610=VECTOR('',#99182,1000.);
#12611=VECTOR('',#99183,1000.);
#12612=VECTOR('',#99184,1000.);
#12613=VECTOR('',#99187,1000.);
#12614=VECTOR('',#99188,1000.);
#12615=VECTOR('',#99189,1000.);
#12616=VECTOR('',#99192,1000.);
#12617=VECTOR('',#99193,1000.);
#12618=VECTOR('',#99194,1000.);
#12619=VECTOR('',#99197,1000.);
#12620=VECTOR('',#99198,1000.);
#12621=VECTOR('',#99201,1000.);
#12622=VECTOR('',#99202,1000.);
#12623=VECTOR('',#99203,1000.);
#12624=VECTOR('',#99204,1000.);
#12625=VECTOR('',#99207,1000.);
#12626=VECTOR('',#99208,1000.);
#12627=VECTOR('',#99209,1000.);
#12628=VECTOR('',#99212,1000.);
#12629=VECTOR('',#99213,1000.);
#12630=VECTOR('',#99214,1000.);
#12631=VECTOR('',#99217,1000.);
#12632=VECTOR('',#99218,1000.);
#12633=VECTOR('',#99221,1000.);
#12634=VECTOR('',#99222,1000.);
#12635=VECTOR('',#99223,1000.);
#12636=VECTOR('',#99224,1000.);
#12637=VECTOR('',#99227,1000.);
#12638=VECTOR('',#99228,1000.);
#12639=VECTOR('',#99229,1000.);
#12640=VECTOR('',#99232,1000.);
#12641=VECTOR('',#99233,1000.);
#12642=VECTOR('',#99234,1000.);
#12643=VECTOR('',#99237,1000.);
#12644=VECTOR('',#99238,1000.);
#12645=VECTOR('',#99241,1000.);
#12646=VECTOR('',#99242,1000.);
#12647=VECTOR('',#99243,1000.);
#12648=VECTOR('',#99244,1000.);
#12649=VECTOR('',#99247,1000.);
#12650=VECTOR('',#99248,1000.);
#12651=VECTOR('',#99249,1000.);
#12652=VECTOR('',#99252,1000.);
#12653=VECTOR('',#99253,1000.);
#12654=VECTOR('',#99254,1000.);
#12655=VECTOR('',#99257,1000.);
#12656=VECTOR('',#99258,1000.);
#12657=VECTOR('',#99261,1000.);
#12658=VECTOR('',#99262,1000.);
#12659=VECTOR('',#99263,1000.);
#12660=VECTOR('',#99264,1000.);
#12661=VECTOR('',#99267,1000.);
#12662=VECTOR('',#99268,1000.);
#12663=VECTOR('',#99269,1000.);
#12664=VECTOR('',#99272,1000.);
#12665=VECTOR('',#99273,1000.);
#12666=VECTOR('',#99274,1000.);
#12667=VECTOR('',#99277,1000.);
#12668=VECTOR('',#99278,1000.);
#12669=VECTOR('',#99281,1000.);
#12670=VECTOR('',#99282,1000.);
#12671=VECTOR('',#99283,1000.);
#12672=VECTOR('',#99284,1000.);
#12673=VECTOR('',#99287,1000.);
#12674=VECTOR('',#99288,1000.);
#12675=VECTOR('',#99289,1000.);
#12676=VECTOR('',#99292,1000.);
#12677=VECTOR('',#99293,1000.);
#12678=VECTOR('',#99294,1000.);
#12679=VECTOR('',#99297,1000.);
#12680=VECTOR('',#99298,1000.);
#12681=VECTOR('',#99301,1000.);
#12682=VECTOR('',#99302,1000.);
#12683=VECTOR('',#99303,1000.);
#12684=VECTOR('',#99304,1000.);
#12685=VECTOR('',#99307,1000.);
#12686=VECTOR('',#99308,1000.);
#12687=VECTOR('',#99309,1000.);
#12688=VECTOR('',#99312,1000.);
#12689=VECTOR('',#99313,1000.);
#12690=VECTOR('',#99314,1000.);
#12691=VECTOR('',#99317,1000.);
#12692=VECTOR('',#99318,1000.);
#12693=VECTOR('',#99321,1000.);
#12694=VECTOR('',#99322,1000.);
#12695=VECTOR('',#99323,1000.);
#12696=VECTOR('',#99324,1000.);
#12697=VECTOR('',#99327,1000.);
#12698=VECTOR('',#99328,1000.);
#12699=VECTOR('',#99329,1000.);
#12700=VECTOR('',#99332,1000.);
#12701=VECTOR('',#99333,1000.);
#12702=VECTOR('',#99334,1000.);
#12703=VECTOR('',#99337,1000.);
#12704=VECTOR('',#99338,1000.);
#12705=VECTOR('',#99341,1000.);
#12706=VECTOR('',#99342,1000.);
#12707=VECTOR('',#99343,1000.);
#12708=VECTOR('',#99344,1000.);
#12709=VECTOR('',#99347,1000.);
#12710=VECTOR('',#99348,1000.);
#12711=VECTOR('',#99349,1000.);
#12712=VECTOR('',#99352,1000.);
#12713=VECTOR('',#99353,1000.);
#12714=VECTOR('',#99354,1000.);
#12715=VECTOR('',#99357,1000.);
#12716=VECTOR('',#99358,1000.);
#12717=VECTOR('',#99361,1000.);
#12718=VECTOR('',#99362,1000.);
#12719=VECTOR('',#99363,1000.);
#12720=VECTOR('',#99364,1000.);
#12721=VECTOR('',#99367,1000.);
#12722=VECTOR('',#99368,1000.);
#12723=VECTOR('',#99369,1000.);
#12724=VECTOR('',#99372,1000.);
#12725=VECTOR('',#99373,1000.);
#12726=VECTOR('',#99374,1000.);
#12727=VECTOR('',#99377,1000.);
#12728=VECTOR('',#99378,1000.);
#12729=VECTOR('',#99381,1000.);
#12730=VECTOR('',#99382,1000.);
#12731=VECTOR('',#99383,1000.);
#12732=VECTOR('',#99384,1000.);
#12733=VECTOR('',#99387,1000.);
#12734=VECTOR('',#99388,1000.);
#12735=VECTOR('',#99389,1000.);
#12736=VECTOR('',#99392,1000.);
#12737=VECTOR('',#99393,1000.);
#12738=VECTOR('',#99394,1000.);
#12739=VECTOR('',#99397,1000.);
#12740=VECTOR('',#99398,1000.);
#12741=VECTOR('',#99401,1000.);
#12742=VECTOR('',#99402,1000.);
#12743=VECTOR('',#99403,1000.);
#12744=VECTOR('',#99404,1000.);
#12745=VECTOR('',#99407,1000.);
#12746=VECTOR('',#99408,1000.);
#12747=VECTOR('',#99409,1000.);
#12748=VECTOR('',#99412,1000.);
#12749=VECTOR('',#99413,1000.);
#12750=VECTOR('',#99414,1000.);
#12751=VECTOR('',#99417,1000.);
#12752=VECTOR('',#99418,1000.);
#12753=VECTOR('',#99421,1000.);
#12754=VECTOR('',#99422,1000.);
#12755=VECTOR('',#99423,1000.);
#12756=VECTOR('',#99424,1000.);
#12757=VECTOR('',#99427,1000.);
#12758=VECTOR('',#99428,1000.);
#12759=VECTOR('',#99429,1000.);
#12760=VECTOR('',#99432,1000.);
#12761=VECTOR('',#99433,1000.);
#12762=VECTOR('',#99434,1000.);
#12763=VECTOR('',#99437,1000.);
#12764=VECTOR('',#99438,1000.);
#12765=VECTOR('',#99441,1000.);
#12766=VECTOR('',#99442,1000.);
#12767=VECTOR('',#99443,1000.);
#12768=VECTOR('',#99444,1000.);
#12769=VECTOR('',#99447,1000.);
#12770=VECTOR('',#99448,1000.);
#12771=VECTOR('',#99449,1000.);
#12772=VECTOR('',#99452,1000.);
#12773=VECTOR('',#99453,1000.);
#12774=VECTOR('',#99454,1000.);
#12775=VECTOR('',#99457,1000.);
#12776=VECTOR('',#99458,1000.);
#12777=VECTOR('',#99461,1000.);
#12778=VECTOR('',#99462,1000.);
#12779=VECTOR('',#99463,1000.);
#12780=VECTOR('',#99464,1000.);
#12781=VECTOR('',#99467,1000.);
#12782=VECTOR('',#99468,1000.);
#12783=VECTOR('',#99469,1000.);
#12784=VECTOR('',#99472,1000.);
#12785=VECTOR('',#99473,1000.);
#12786=VECTOR('',#99474,1000.);
#12787=VECTOR('',#99477,1000.);
#12788=VECTOR('',#99478,1000.);
#12789=VECTOR('',#99481,1000.);
#12790=VECTOR('',#99482,1000.);
#12791=VECTOR('',#99483,1000.);
#12792=VECTOR('',#99484,1000.);
#12793=VECTOR('',#99487,1000.);
#12794=VECTOR('',#99488,1000.);
#12795=VECTOR('',#99489,1000.);
#12796=VECTOR('',#99492,1000.);
#12797=VECTOR('',#99493,1000.);
#12798=VECTOR('',#99494,1000.);
#12799=VECTOR('',#99497,1000.);
#12800=VECTOR('',#99498,1000.);
#12801=VECTOR('',#99501,1000.);
#12802=VECTOR('',#99502,1000.);
#12803=VECTOR('',#99503,1000.);
#12804=VECTOR('',#99504,1000.);
#12805=VECTOR('',#99507,1000.);
#12806=VECTOR('',#99508,1000.);
#12807=VECTOR('',#99509,1000.);
#12808=VECTOR('',#99512,1000.);
#12809=VECTOR('',#99513,1000.);
#12810=VECTOR('',#99514,1000.);
#12811=VECTOR('',#99517,1000.);
#12812=VECTOR('',#99518,1000.);
#12813=VECTOR('',#99521,1000.);
#12814=VECTOR('',#99522,1000.);
#12815=VECTOR('',#99523,1000.);
#12816=VECTOR('',#99524,1000.);
#12817=VECTOR('',#99527,1000.);
#12818=VECTOR('',#99528,1000.);
#12819=VECTOR('',#99529,1000.);
#12820=VECTOR('',#99532,1000.);
#12821=VECTOR('',#99533,1000.);
#12822=VECTOR('',#99534,1000.);
#12823=VECTOR('',#99537,1000.);
#12824=VECTOR('',#99538,1000.);
#12825=VECTOR('',#99541,1000.);
#12826=VECTOR('',#99542,1000.);
#12827=VECTOR('',#99543,1000.);
#12828=VECTOR('',#99544,1000.);
#12829=VECTOR('',#99547,1000.);
#12830=VECTOR('',#99548,1000.);
#12831=VECTOR('',#99549,1000.);
#12832=VECTOR('',#99552,1000.);
#12833=VECTOR('',#99553,1000.);
#12834=VECTOR('',#99554,1000.);
#12835=VECTOR('',#99557,1000.);
#12836=VECTOR('',#99558,1000.);
#12837=VECTOR('',#99561,1000.);
#12838=VECTOR('',#99562,1000.);
#12839=VECTOR('',#99563,1000.);
#12840=VECTOR('',#99564,1000.);
#12841=VECTOR('',#99567,1000.);
#12842=VECTOR('',#99568,1000.);
#12843=VECTOR('',#99569,1000.);
#12844=VECTOR('',#99572,1000.);
#12845=VECTOR('',#99573,1000.);
#12846=VECTOR('',#99574,1000.);
#12847=VECTOR('',#99577,1000.);
#12848=VECTOR('',#99578,1000.);
#12849=VECTOR('',#99581,1000.);
#12850=VECTOR('',#99582,1000.);
#12851=VECTOR('',#99583,1000.);
#12852=VECTOR('',#99584,1000.);
#12853=VECTOR('',#99587,1000.);
#12854=VECTOR('',#99588,1000.);
#12855=VECTOR('',#99589,1000.);
#12856=VECTOR('',#99592,1000.);
#12857=VECTOR('',#99593,1000.);
#12858=VECTOR('',#99594,1000.);
#12859=VECTOR('',#99597,1000.);
#12860=VECTOR('',#99598,1000.);
#12861=VECTOR('',#99601,1000.);
#12862=VECTOR('',#99602,1000.);
#12863=VECTOR('',#99603,1000.);
#12864=VECTOR('',#99604,1000.);
#12865=VECTOR('',#99607,1000.);
#12866=VECTOR('',#99608,1000.);
#12867=VECTOR('',#99609,1000.);
#12868=VECTOR('',#99612,1000.);
#12869=VECTOR('',#99613,1000.);
#12870=VECTOR('',#99614,1000.);
#12871=VECTOR('',#99617,1000.);
#12872=VECTOR('',#99618,1000.);
#12873=VECTOR('',#99621,1000.);
#12874=VECTOR('',#99622,1000.);
#12875=VECTOR('',#99623,1000.);
#12876=VECTOR('',#99624,1000.);
#12877=VECTOR('',#99627,1000.);
#12878=VECTOR('',#99628,1000.);
#12879=VECTOR('',#99629,1000.);
#12880=VECTOR('',#99632,1000.);
#12881=VECTOR('',#99633,1000.);
#12882=VECTOR('',#99634,1000.);
#12883=VECTOR('',#99637,1000.);
#12884=VECTOR('',#99638,1000.);
#12885=VECTOR('',#99641,1000.);
#12886=VECTOR('',#99642,1000.);
#12887=VECTOR('',#99643,1000.);
#12888=VECTOR('',#99644,1000.);
#12889=VECTOR('',#99647,1000.);
#12890=VECTOR('',#99648,1000.);
#12891=VECTOR('',#99649,1000.);
#12892=VECTOR('',#99652,1000.);
#12893=VECTOR('',#99653,1000.);
#12894=VECTOR('',#99654,1000.);
#12895=VECTOR('',#99657,1000.);
#12896=VECTOR('',#99658,1000.);
#12897=VECTOR('',#99661,1000.);
#12898=VECTOR('',#99662,1000.);
#12899=VECTOR('',#99663,1000.);
#12900=VECTOR('',#99664,1000.);
#12901=VECTOR('',#99667,1000.);
#12902=VECTOR('',#99668,1000.);
#12903=VECTOR('',#99669,1000.);
#12904=VECTOR('',#99672,1000.);
#12905=VECTOR('',#99673,1000.);
#12906=VECTOR('',#99674,1000.);
#12907=VECTOR('',#99677,1000.);
#12908=VECTOR('',#99678,1000.);
#12909=VECTOR('',#99681,1000.);
#12910=VECTOR('',#99682,1000.);
#12911=VECTOR('',#99683,1000.);
#12912=VECTOR('',#99684,1000.);
#12913=VECTOR('',#99687,1000.);
#12914=VECTOR('',#99688,1000.);
#12915=VECTOR('',#99689,1000.);
#12916=VECTOR('',#99692,1000.);
#12917=VECTOR('',#99693,1000.);
#12918=VECTOR('',#99694,1000.);
#12919=VECTOR('',#99697,1000.);
#12920=VECTOR('',#99698,1000.);
#12921=VECTOR('',#99701,1000.);
#12922=VECTOR('',#99702,1000.);
#12923=VECTOR('',#99703,1000.);
#12924=VECTOR('',#99704,1000.);
#12925=VECTOR('',#99707,1000.);
#12926=VECTOR('',#99708,1000.);
#12927=VECTOR('',#99709,1000.);
#12928=VECTOR('',#99712,1000.);
#12929=VECTOR('',#99713,1000.);
#12930=VECTOR('',#99714,1000.);
#12931=VECTOR('',#99717,1000.);
#12932=VECTOR('',#99718,1000.);
#12933=VECTOR('',#99721,1000.);
#12934=VECTOR('',#99722,1000.);
#12935=VECTOR('',#99723,1000.);
#12936=VECTOR('',#99724,1000.);
#12937=VECTOR('',#99727,1000.);
#12938=VECTOR('',#99728,1000.);
#12939=VECTOR('',#99729,1000.);
#12940=VECTOR('',#99732,1000.);
#12941=VECTOR('',#99733,1000.);
#12942=VECTOR('',#99734,1000.);
#12943=VECTOR('',#99737,1000.);
#12944=VECTOR('',#99738,1000.);
#12945=VECTOR('',#99741,1000.);
#12946=VECTOR('',#99742,1000.);
#12947=VECTOR('',#99743,1000.);
#12948=VECTOR('',#99744,1000.);
#12949=VECTOR('',#99747,1000.);
#12950=VECTOR('',#99748,1000.);
#12951=VECTOR('',#99749,1000.);
#12952=VECTOR('',#99752,1000.);
#12953=VECTOR('',#99753,1000.);
#12954=VECTOR('',#99754,1000.);
#12955=VECTOR('',#99757,1000.);
#12956=VECTOR('',#99758,1000.);
#12957=VECTOR('',#99761,1000.);
#12958=VECTOR('',#99762,1000.);
#12959=VECTOR('',#99763,1000.);
#12960=VECTOR('',#99764,1000.);
#12961=VECTOR('',#99767,1000.);
#12962=VECTOR('',#99768,1000.);
#12963=VECTOR('',#99769,1000.);
#12964=VECTOR('',#99772,1000.);
#12965=VECTOR('',#99773,1000.);
#12966=VECTOR('',#99774,1000.);
#12967=VECTOR('',#99777,1000.);
#12968=VECTOR('',#99778,1000.);
#12969=VECTOR('',#99781,1000.);
#12970=VECTOR('',#99782,1000.);
#12971=VECTOR('',#99783,1000.);
#12972=VECTOR('',#99784,1000.);
#12973=VECTOR('',#99787,1000.);
#12974=VECTOR('',#99788,1000.);
#12975=VECTOR('',#99789,1000.);
#12976=VECTOR('',#99792,1000.);
#12977=VECTOR('',#99793,1000.);
#12978=VECTOR('',#99794,1000.);
#12979=VECTOR('',#99797,1000.);
#12980=VECTOR('',#99798,1000.);
#12981=VECTOR('',#99801,1000.);
#12982=VECTOR('',#99802,1000.);
#12983=VECTOR('',#99803,1000.);
#12984=VECTOR('',#99804,1000.);
#12985=VECTOR('',#99807,1000.);
#12986=VECTOR('',#99808,1000.);
#12987=VECTOR('',#99809,1000.);
#12988=VECTOR('',#99812,1000.);
#12989=VECTOR('',#99813,1000.);
#12990=VECTOR('',#99814,1000.);
#12991=VECTOR('',#99817,1000.);
#12992=VECTOR('',#99818,1000.);
#12993=VECTOR('',#99821,1000.);
#12994=VECTOR('',#99822,1000.);
#12995=VECTOR('',#99823,1000.);
#12996=VECTOR('',#99824,1000.);
#12997=VECTOR('',#99827,1000.);
#12998=VECTOR('',#99828,1000.);
#12999=VECTOR('',#99829,1000.);
#13000=VECTOR('',#99832,1000.);
#13001=VECTOR('',#99833,1000.);
#13002=VECTOR('',#99834,1000.);
#13003=VECTOR('',#99837,1000.);
#13004=VECTOR('',#99838,1000.);
#13005=VECTOR('',#99841,1000.);
#13006=VECTOR('',#99842,1000.);
#13007=VECTOR('',#99843,1000.);
#13008=VECTOR('',#99844,1000.);
#13009=VECTOR('',#99847,1000.);
#13010=VECTOR('',#99848,1000.);
#13011=VECTOR('',#99849,1000.);
#13012=VECTOR('',#99852,1000.);
#13013=VECTOR('',#99853,1000.);
#13014=VECTOR('',#99854,1000.);
#13015=VECTOR('',#99857,1000.);
#13016=VECTOR('',#99858,1000.);
#13017=VECTOR('',#99861,1000.);
#13018=VECTOR('',#99862,1000.);
#13019=VECTOR('',#99863,1000.);
#13020=VECTOR('',#99864,1000.);
#13021=VECTOR('',#99867,1000.);
#13022=VECTOR('',#99868,1000.);
#13023=VECTOR('',#99869,1000.);
#13024=VECTOR('',#99872,1000.);
#13025=VECTOR('',#99873,1000.);
#13026=VECTOR('',#99874,1000.);
#13027=VECTOR('',#99877,1000.);
#13028=VECTOR('',#99878,1000.);
#13029=VECTOR('',#99881,1000.);
#13030=VECTOR('',#99882,1000.);
#13031=VECTOR('',#99883,1000.);
#13032=VECTOR('',#99884,1000.);
#13033=VECTOR('',#99887,1000.);
#13034=VECTOR('',#99888,1000.);
#13035=VECTOR('',#99889,1000.);
#13036=VECTOR('',#99892,1000.);
#13037=VECTOR('',#99893,1000.);
#13038=VECTOR('',#99894,1000.);
#13039=VECTOR('',#99897,1000.);
#13040=VECTOR('',#99898,1000.);
#13041=VECTOR('',#99901,1000.);
#13042=VECTOR('',#99902,1000.);
#13043=VECTOR('',#99903,1000.);
#13044=VECTOR('',#99904,1000.);
#13045=VECTOR('',#99907,1000.);
#13046=VECTOR('',#99908,1000.);
#13047=VECTOR('',#99909,1000.);
#13048=VECTOR('',#99912,1000.);
#13049=VECTOR('',#99913,1000.);
#13050=VECTOR('',#99914,1000.);
#13051=VECTOR('',#99917,1000.);
#13052=VECTOR('',#99918,1000.);
#13053=VECTOR('',#99921,1000.);
#13054=VECTOR('',#99922,1000.);
#13055=VECTOR('',#99923,1000.);
#13056=VECTOR('',#99924,1000.);
#13057=VECTOR('',#99927,1000.);
#13058=VECTOR('',#99928,1000.);
#13059=VECTOR('',#99929,1000.);
#13060=VECTOR('',#99932,1000.);
#13061=VECTOR('',#99933,1000.);
#13062=VECTOR('',#99934,1000.);
#13063=VECTOR('',#99937,1000.);
#13064=VECTOR('',#99938,1000.);
#13065=VECTOR('',#99941,1000.);
#13066=VECTOR('',#99942,1000.);
#13067=VECTOR('',#99943,1000.);
#13068=VECTOR('',#99944,1000.);
#13069=VECTOR('',#99947,1000.);
#13070=VECTOR('',#99948,1000.);
#13071=VECTOR('',#99949,1000.);
#13072=VECTOR('',#99952,1000.);
#13073=VECTOR('',#99953,1000.);
#13074=VECTOR('',#99954,1000.);
#13075=VECTOR('',#99957,1000.);
#13076=VECTOR('',#99958,1000.);
#13077=VECTOR('',#99961,1000.);
#13078=VECTOR('',#99962,1000.);
#13079=VECTOR('',#99963,1000.);
#13080=VECTOR('',#99964,1000.);
#13081=VECTOR('',#99967,1000.);
#13082=VECTOR('',#99968,1000.);
#13083=VECTOR('',#99969,1000.);
#13084=VECTOR('',#99972,1000.);
#13085=VECTOR('',#99973,1000.);
#13086=VECTOR('',#99974,1000.);
#13087=VECTOR('',#99977,1000.);
#13088=VECTOR('',#99978,1000.);
#13089=VECTOR('',#99981,1000.);
#13090=VECTOR('',#99982,1000.);
#13091=VECTOR('',#99983,1000.);
#13092=VECTOR('',#99984,1000.);
#13093=VECTOR('',#99987,1000.);
#13094=VECTOR('',#99988,1000.);
#13095=VECTOR('',#99989,1000.);
#13096=VECTOR('',#99992,1000.);
#13097=VECTOR('',#99993,1000.);
#13098=VECTOR('',#99994,1000.);
#13099=VECTOR('',#99997,1000.);
#13100=VECTOR('',#99998,1000.);
#13101=VECTOR('',#100001,1000.);
#13102=VECTOR('',#100002,1000.);
#13103=VECTOR('',#100003,1000.);
#13104=VECTOR('',#100004,1000.);
#13105=VECTOR('',#100007,1000.);
#13106=VECTOR('',#100008,1000.);
#13107=VECTOR('',#100009,1000.);
#13108=VECTOR('',#100012,1000.);
#13109=VECTOR('',#100013,1000.);
#13110=VECTOR('',#100014,1000.);
#13111=VECTOR('',#100017,1000.);
#13112=VECTOR('',#100018,1000.);
#13113=VECTOR('',#100021,1000.);
#13114=VECTOR('',#100022,1000.);
#13115=VECTOR('',#100023,1000.);
#13116=VECTOR('',#100024,1000.);
#13117=VECTOR('',#100027,1000.);
#13118=VECTOR('',#100028,1000.);
#13119=VECTOR('',#100029,1000.);
#13120=VECTOR('',#100032,1000.);
#13121=VECTOR('',#100033,1000.);
#13122=VECTOR('',#100034,1000.);
#13123=VECTOR('',#100037,1000.);
#13124=VECTOR('',#100038,1000.);
#13125=VECTOR('',#100041,1000.);
#13126=VECTOR('',#100042,1000.);
#13127=VECTOR('',#100043,1000.);
#13128=VECTOR('',#100044,1000.);
#13129=VECTOR('',#100047,1000.);
#13130=VECTOR('',#100048,1000.);
#13131=VECTOR('',#100049,1000.);
#13132=VECTOR('',#100052,1000.);
#13133=VECTOR('',#100053,1000.);
#13134=VECTOR('',#100054,1000.);
#13135=VECTOR('',#100057,1000.);
#13136=VECTOR('',#100058,1000.);
#13137=VECTOR('',#100061,1000.);
#13138=VECTOR('',#100062,1000.);
#13139=VECTOR('',#100063,1000.);
#13140=VECTOR('',#100064,1000.);
#13141=VECTOR('',#100067,1000.);
#13142=VECTOR('',#100068,1000.);
#13143=VECTOR('',#100069,1000.);
#13144=VECTOR('',#100072,1000.);
#13145=VECTOR('',#100073,1000.);
#13146=VECTOR('',#100074,1000.);
#13147=VECTOR('',#100077,1000.);
#13148=VECTOR('',#100078,1000.);
#13149=VECTOR('',#100081,1000.);
#13150=VECTOR('',#100082,1000.);
#13151=VECTOR('',#100083,1000.);
#13152=VECTOR('',#100084,1000.);
#13153=VECTOR('',#100087,1000.);
#13154=VECTOR('',#100088,1000.);
#13155=VECTOR('',#100089,1000.);
#13156=VECTOR('',#100092,1000.);
#13157=VECTOR('',#100093,1000.);
#13158=VECTOR('',#100094,1000.);
#13159=VECTOR('',#100097,1000.);
#13160=VECTOR('',#100098,1000.);
#13161=VECTOR('',#100101,1000.);
#13162=VECTOR('',#100102,1000.);
#13163=VECTOR('',#100103,1000.);
#13164=VECTOR('',#100104,1000.);
#13165=VECTOR('',#100107,1000.);
#13166=VECTOR('',#100108,1000.);
#13167=VECTOR('',#100109,1000.);
#13168=VECTOR('',#100112,1000.);
#13169=VECTOR('',#100113,1000.);
#13170=VECTOR('',#100114,1000.);
#13171=VECTOR('',#100117,1000.);
#13172=VECTOR('',#100118,1000.);
#13173=VECTOR('',#100121,1000.);
#13174=VECTOR('',#100122,1000.);
#13175=VECTOR('',#100123,1000.);
#13176=VECTOR('',#100124,1000.);
#13177=VECTOR('',#100127,1000.);
#13178=VECTOR('',#100128,1000.);
#13179=VECTOR('',#100129,1000.);
#13180=VECTOR('',#100132,1000.);
#13181=VECTOR('',#100133,1000.);
#13182=VECTOR('',#100134,1000.);
#13183=VECTOR('',#100137,1000.);
#13184=VECTOR('',#100138,1000.);
#13185=VECTOR('',#100141,1000.);
#13186=VECTOR('',#100142,1000.);
#13187=VECTOR('',#100143,1000.);
#13188=VECTOR('',#100144,1000.);
#13189=VECTOR('',#100147,1000.);
#13190=VECTOR('',#100148,1000.);
#13191=VECTOR('',#100149,1000.);
#13192=VECTOR('',#100152,1000.);
#13193=VECTOR('',#100153,1000.);
#13194=VECTOR('',#100154,1000.);
#13195=VECTOR('',#100157,1000.);
#13196=VECTOR('',#100158,1000.);
#13197=VECTOR('',#100161,1000.);
#13198=VECTOR('',#100162,1000.);
#13199=VECTOR('',#100163,1000.);
#13200=VECTOR('',#100164,1000.);
#13201=VECTOR('',#100167,1000.);
#13202=VECTOR('',#100168,1000.);
#13203=VECTOR('',#100169,1000.);
#13204=VECTOR('',#100172,1000.);
#13205=VECTOR('',#100173,1000.);
#13206=VECTOR('',#100174,1000.);
#13207=VECTOR('',#100177,1000.);
#13208=VECTOR('',#100178,1000.);
#13209=VECTOR('',#100181,1000.);
#13210=VECTOR('',#100182,1000.);
#13211=VECTOR('',#100183,1000.);
#13212=VECTOR('',#100184,1000.);
#13213=VECTOR('',#100187,1000.);
#13214=VECTOR('',#100188,1000.);
#13215=VECTOR('',#100189,1000.);
#13216=VECTOR('',#100192,1000.);
#13217=VECTOR('',#100193,1000.);
#13218=VECTOR('',#100194,1000.);
#13219=VECTOR('',#100197,1000.);
#13220=VECTOR('',#100198,1000.);
#13221=VECTOR('',#100201,1000.);
#13222=VECTOR('',#100202,1000.);
#13223=VECTOR('',#100203,1000.);
#13224=VECTOR('',#100204,1000.);
#13225=VECTOR('',#100207,1000.);
#13226=VECTOR('',#100208,1000.);
#13227=VECTOR('',#100209,1000.);
#13228=VECTOR('',#100212,1000.);
#13229=VECTOR('',#100213,1000.);
#13230=VECTOR('',#100214,1000.);
#13231=VECTOR('',#100217,1000.);
#13232=VECTOR('',#100218,1000.);
#13233=VECTOR('',#100221,1000.);
#13234=VECTOR('',#100222,1000.);
#13235=VECTOR('',#100223,1000.);
#13236=VECTOR('',#100224,1000.);
#13237=VECTOR('',#100227,1000.);
#13238=VECTOR('',#100228,1000.);
#13239=VECTOR('',#100229,1000.);
#13240=VECTOR('',#100232,1000.);
#13241=VECTOR('',#100233,1000.);
#13242=VECTOR('',#100234,1000.);
#13243=VECTOR('',#100237,1000.);
#13244=VECTOR('',#100238,1000.);
#13245=VECTOR('',#100241,1000.);
#13246=VECTOR('',#100242,1000.);
#13247=VECTOR('',#100243,1000.);
#13248=VECTOR('',#100244,1000.);
#13249=VECTOR('',#100247,1000.);
#13250=VECTOR('',#100248,1000.);
#13251=VECTOR('',#100249,1000.);
#13252=VECTOR('',#100252,1000.);
#13253=VECTOR('',#100253,1000.);
#13254=VECTOR('',#100254,1000.);
#13255=VECTOR('',#100257,1000.);
#13256=VECTOR('',#100258,1000.);
#13257=VECTOR('',#100261,1000.);
#13258=VECTOR('',#100262,1000.);
#13259=VECTOR('',#100263,1000.);
#13260=VECTOR('',#100264,1000.);
#13261=VECTOR('',#100267,1000.);
#13262=VECTOR('',#100268,1000.);
#13263=VECTOR('',#100269,1000.);
#13264=VECTOR('',#100272,1000.);
#13265=VECTOR('',#100273,1000.);
#13266=VECTOR('',#100274,1000.);
#13267=VECTOR('',#100277,1000.);
#13268=VECTOR('',#100278,1000.);
#13269=VECTOR('',#100281,1000.);
#13270=VECTOR('',#100282,1000.);
#13271=VECTOR('',#100283,1000.);
#13272=VECTOR('',#100284,1000.);
#13273=VECTOR('',#100287,1000.);
#13274=VECTOR('',#100288,1000.);
#13275=VECTOR('',#100289,1000.);
#13276=VECTOR('',#100292,1000.);
#13277=VECTOR('',#100293,1000.);
#13278=VECTOR('',#100294,1000.);
#13279=VECTOR('',#100297,1000.);
#13280=VECTOR('',#100298,1000.);
#13281=VECTOR('',#100301,1000.);
#13282=VECTOR('',#100302,1000.);
#13283=VECTOR('',#100303,1000.);
#13284=VECTOR('',#100304,1000.);
#13285=VECTOR('',#100307,1000.);
#13286=VECTOR('',#100308,1000.);
#13287=VECTOR('',#100309,1000.);
#13288=VECTOR('',#100312,1000.);
#13289=VECTOR('',#100313,1000.);
#13290=VECTOR('',#100314,1000.);
#13291=VECTOR('',#100317,1000.);
#13292=VECTOR('',#100318,1000.);
#13293=VECTOR('',#100321,1000.);
#13294=VECTOR('',#100322,1000.);
#13295=VECTOR('',#100323,1000.);
#13296=VECTOR('',#100324,1000.);
#13297=VECTOR('',#100327,1000.);
#13298=VECTOR('',#100328,1000.);
#13299=VECTOR('',#100329,1000.);
#13300=VECTOR('',#100332,1000.);
#13301=VECTOR('',#100333,1000.);
#13302=VECTOR('',#100334,1000.);
#13303=VECTOR('',#100337,1000.);
#13304=VECTOR('',#100338,1000.);
#13305=VECTOR('',#100341,1000.);
#13306=VECTOR('',#100342,1000.);
#13307=VECTOR('',#100343,1000.);
#13308=VECTOR('',#100344,1000.);
#13309=VECTOR('',#100347,1000.);
#13310=VECTOR('',#100348,1000.);
#13311=VECTOR('',#100349,1000.);
#13312=VECTOR('',#100352,1000.);
#13313=VECTOR('',#100353,1000.);
#13314=VECTOR('',#100354,1000.);
#13315=VECTOR('',#100357,1000.);
#13316=VECTOR('',#100358,1000.);
#13317=VECTOR('',#100361,1000.);
#13318=VECTOR('',#100362,1000.);
#13319=VECTOR('',#100363,1000.);
#13320=VECTOR('',#100364,1000.);
#13321=VECTOR('',#100367,1000.);
#13322=VECTOR('',#100368,1000.);
#13323=VECTOR('',#100369,1000.);
#13324=VECTOR('',#100372,1000.);
#13325=VECTOR('',#100373,1000.);
#13326=VECTOR('',#100374,1000.);
#13327=VECTOR('',#100377,1000.);
#13328=VECTOR('',#100378,1000.);
#13329=VECTOR('',#100381,1000.);
#13330=VECTOR('',#100382,1000.);
#13331=VECTOR('',#100383,1000.);
#13332=VECTOR('',#100384,1000.);
#13333=VECTOR('',#100387,1000.);
#13334=VECTOR('',#100388,1000.);
#13335=VECTOR('',#100389,1000.);
#13336=VECTOR('',#100392,1000.);
#13337=VECTOR('',#100393,1000.);
#13338=VECTOR('',#100394,1000.);
#13339=VECTOR('',#100397,1000.);
#13340=VECTOR('',#100398,1000.);
#13341=VECTOR('',#100401,1000.);
#13342=VECTOR('',#100402,1000.);
#13343=VECTOR('',#100403,1000.);
#13344=VECTOR('',#100404,1000.);
#13345=VECTOR('',#100407,1000.);
#13346=VECTOR('',#100408,1000.);
#13347=VECTOR('',#100409,1000.);
#13348=VECTOR('',#100412,1000.);
#13349=VECTOR('',#100413,1000.);
#13350=VECTOR('',#100414,1000.);
#13351=VECTOR('',#100417,1000.);
#13352=VECTOR('',#100418,1000.);
#13353=VECTOR('',#100421,1000.);
#13354=VECTOR('',#100422,1000.);
#13355=VECTOR('',#100423,1000.);
#13356=VECTOR('',#100424,1000.);
#13357=VECTOR('',#100427,1000.);
#13358=VECTOR('',#100428,1000.);
#13359=VECTOR('',#100429,1000.);
#13360=VECTOR('',#100432,1000.);
#13361=VECTOR('',#100433,1000.);
#13362=VECTOR('',#100434,1000.);
#13363=VECTOR('',#100437,1000.);
#13364=VECTOR('',#100438,1000.);
#13365=VECTOR('',#100441,1000.);
#13366=VECTOR('',#100442,1000.);
#13367=VECTOR('',#100443,1000.);
#13368=VECTOR('',#100444,1000.);
#13369=VECTOR('',#100447,1000.);
#13370=VECTOR('',#100448,1000.);
#13371=VECTOR('',#100449,1000.);
#13372=VECTOR('',#100452,1000.);
#13373=VECTOR('',#100453,1000.);
#13374=VECTOR('',#100454,1000.);
#13375=VECTOR('',#100457,1000.);
#13376=VECTOR('',#100458,1000.);
#13377=VECTOR('',#100461,1000.);
#13378=VECTOR('',#100462,1000.);
#13379=VECTOR('',#100463,1000.);
#13380=VECTOR('',#100464,1000.);
#13381=VECTOR('',#100467,1000.);
#13382=VECTOR('',#100468,1000.);
#13383=VECTOR('',#100469,1000.);
#13384=VECTOR('',#100472,1000.);
#13385=VECTOR('',#100473,1000.);
#13386=VECTOR('',#100474,1000.);
#13387=VECTOR('',#100477,1000.);
#13388=VECTOR('',#100478,1000.);
#13389=VECTOR('',#100481,1000.);
#13390=VECTOR('',#100482,1000.);
#13391=VECTOR('',#100483,1000.);
#13392=VECTOR('',#100484,1000.);
#13393=VECTOR('',#100487,1000.);
#13394=VECTOR('',#100488,1000.);
#13395=VECTOR('',#100489,1000.);
#13396=VECTOR('',#100492,1000.);
#13397=VECTOR('',#100493,1000.);
#13398=VECTOR('',#100494,1000.);
#13399=VECTOR('',#100497,1000.);
#13400=VECTOR('',#100498,1000.);
#13401=VECTOR('',#100501,1000.);
#13402=VECTOR('',#100502,1000.);
#13403=VECTOR('',#100503,1000.);
#13404=VECTOR('',#100504,1000.);
#13405=VECTOR('',#100507,1000.);
#13406=VECTOR('',#100508,1000.);
#13407=VECTOR('',#100509,1000.);
#13408=VECTOR('',#100512,1000.);
#13409=VECTOR('',#100513,1000.);
#13410=VECTOR('',#100514,1000.);
#13411=VECTOR('',#100517,1000.);
#13412=VECTOR('',#100518,1000.);
#13413=VECTOR('',#100521,1000.);
#13414=VECTOR('',#100522,1000.);
#13415=VECTOR('',#100523,1000.);
#13416=VECTOR('',#100524,1000.);
#13417=VECTOR('',#100527,1000.);
#13418=VECTOR('',#100528,1000.);
#13419=VECTOR('',#100529,1000.);
#13420=VECTOR('',#100532,1000.);
#13421=VECTOR('',#100533,1000.);
#13422=VECTOR('',#100534,1000.);
#13423=VECTOR('',#100537,1000.);
#13424=VECTOR('',#100538,1000.);
#13425=VECTOR('',#100541,1000.);
#13426=VECTOR('',#100542,1000.);
#13427=VECTOR('',#100543,1000.);
#13428=VECTOR('',#100544,1000.);
#13429=VECTOR('',#100547,1000.);
#13430=VECTOR('',#100548,1000.);
#13431=VECTOR('',#100549,1000.);
#13432=VECTOR('',#100552,1000.);
#13433=VECTOR('',#100553,1000.);
#13434=VECTOR('',#100554,1000.);
#13435=VECTOR('',#100557,1000.);
#13436=VECTOR('',#100558,1000.);
#13437=VECTOR('',#100561,1000.);
#13438=VECTOR('',#100562,1000.);
#13439=VECTOR('',#100563,1000.);
#13440=VECTOR('',#100564,1000.);
#13441=VECTOR('',#100567,1000.);
#13442=VECTOR('',#100568,1000.);
#13443=VECTOR('',#100569,1000.);
#13444=VECTOR('',#100572,1000.);
#13445=VECTOR('',#100573,1000.);
#13446=VECTOR('',#100574,1000.);
#13447=VECTOR('',#100577,1000.);
#13448=VECTOR('',#100578,1000.);
#13449=VECTOR('',#100581,1000.);
#13450=VECTOR('',#100582,1000.);
#13451=VECTOR('',#100583,1000.);
#13452=VECTOR('',#100584,1000.);
#13453=VECTOR('',#100587,1000.);
#13454=VECTOR('',#100588,1000.);
#13455=VECTOR('',#100589,1000.);
#13456=VECTOR('',#100592,1000.);
#13457=VECTOR('',#100593,1000.);
#13458=VECTOR('',#100594,1000.);
#13459=VECTOR('',#100597,1000.);
#13460=VECTOR('',#100598,1000.);
#13461=VECTOR('',#100601,1000.);
#13462=VECTOR('',#100602,1000.);
#13463=VECTOR('',#100603,1000.);
#13464=VECTOR('',#100604,1000.);
#13465=VECTOR('',#100607,1000.);
#13466=VECTOR('',#100608,1000.);
#13467=VECTOR('',#100609,1000.);
#13468=VECTOR('',#100612,1000.);
#13469=VECTOR('',#100613,1000.);
#13470=VECTOR('',#100614,1000.);
#13471=VECTOR('',#100617,1000.);
#13472=VECTOR('',#100618,1000.);
#13473=VECTOR('',#100621,1000.);
#13474=VECTOR('',#100622,1000.);
#13475=VECTOR('',#100623,1000.);
#13476=VECTOR('',#100624,1000.);
#13477=VECTOR('',#100627,1000.);
#13478=VECTOR('',#100628,1000.);
#13479=VECTOR('',#100629,1000.);
#13480=VECTOR('',#100632,1000.);
#13481=VECTOR('',#100633,1000.);
#13482=VECTOR('',#100634,1000.);
#13483=VECTOR('',#100637,1000.);
#13484=VECTOR('',#100638,1000.);
#13485=VECTOR('',#100641,1000.);
#13486=VECTOR('',#100642,1000.);
#13487=VECTOR('',#100643,1000.);
#13488=VECTOR('',#100644,1000.);
#13489=VECTOR('',#100647,1000.);
#13490=VECTOR('',#100648,1000.);
#13491=VECTOR('',#100649,1000.);
#13492=VECTOR('',#100652,1000.);
#13493=VECTOR('',#100653,1000.);
#13494=VECTOR('',#100654,1000.);
#13495=VECTOR('',#100657,1000.);
#13496=VECTOR('',#100658,1000.);
#13497=VECTOR('',#100661,1000.);
#13498=VECTOR('',#100662,1000.);
#13499=VECTOR('',#100663,1000.);
#13500=VECTOR('',#100664,1000.);
#13501=VECTOR('',#100667,1000.);
#13502=VECTOR('',#100668,1000.);
#13503=VECTOR('',#100669,1000.);
#13504=VECTOR('',#100672,1000.);
#13505=VECTOR('',#100673,1000.);
#13506=VECTOR('',#100674,1000.);
#13507=VECTOR('',#100677,1000.);
#13508=VECTOR('',#100678,1000.);
#13509=VECTOR('',#100681,1000.);
#13510=VECTOR('',#100682,1000.);
#13511=VECTOR('',#100683,1000.);
#13512=VECTOR('',#100684,1000.);
#13513=VECTOR('',#100687,1000.);
#13514=VECTOR('',#100688,1000.);
#13515=VECTOR('',#100689,1000.);
#13516=VECTOR('',#100692,1000.);
#13517=VECTOR('',#100693,1000.);
#13518=VECTOR('',#100694,1000.);
#13519=VECTOR('',#100697,1000.);
#13520=VECTOR('',#100698,1000.);
#13521=VECTOR('',#100701,1000.);
#13522=VECTOR('',#100702,1000.);
#13523=VECTOR('',#100703,1000.);
#13524=VECTOR('',#100704,1000.);
#13525=VECTOR('',#100707,1000.);
#13526=VECTOR('',#100708,1000.);
#13527=VECTOR('',#100709,1000.);
#13528=VECTOR('',#100712,1000.);
#13529=VECTOR('',#100713,1000.);
#13530=VECTOR('',#100714,1000.);
#13531=VECTOR('',#100717,1000.);
#13532=VECTOR('',#100718,1000.);
#13533=VECTOR('',#100721,1000.);
#13534=VECTOR('',#100722,1000.);
#13535=VECTOR('',#100723,1000.);
#13536=VECTOR('',#100724,1000.);
#13537=VECTOR('',#100727,1000.);
#13538=VECTOR('',#100728,1000.);
#13539=VECTOR('',#100729,1000.);
#13540=VECTOR('',#100732,1000.);
#13541=VECTOR('',#100733,1000.);
#13542=VECTOR('',#100734,1000.);
#13543=VECTOR('',#100737,1000.);
#13544=VECTOR('',#100738,1000.);
#13545=VECTOR('',#100741,1000.);
#13546=VECTOR('',#100742,1000.);
#13547=VECTOR('',#100743,1000.);
#13548=VECTOR('',#100744,1000.);
#13549=VECTOR('',#100747,1000.);
#13550=VECTOR('',#100748,1000.);
#13551=VECTOR('',#100749,1000.);
#13552=VECTOR('',#100752,1000.);
#13553=VECTOR('',#100753,1000.);
#13554=VECTOR('',#100754,1000.);
#13555=VECTOR('',#100757,1000.);
#13556=VECTOR('',#100758,1000.);
#13557=VECTOR('',#100761,1000.);
#13558=VECTOR('',#100762,1000.);
#13559=VECTOR('',#100763,1000.);
#13560=VECTOR('',#100764,1000.);
#13561=VECTOR('',#100767,1000.);
#13562=VECTOR('',#100768,1000.);
#13563=VECTOR('',#100769,1000.);
#13564=VECTOR('',#100772,1000.);
#13565=VECTOR('',#100773,1000.);
#13566=VECTOR('',#100774,1000.);
#13567=VECTOR('',#100777,1000.);
#13568=VECTOR('',#100778,1000.);
#13569=VECTOR('',#100781,1000.);
#13570=VECTOR('',#100782,1000.);
#13571=VECTOR('',#100783,1000.);
#13572=VECTOR('',#100784,1000.);
#13573=VECTOR('',#100787,1000.);
#13574=VECTOR('',#100788,1000.);
#13575=VECTOR('',#100789,1000.);
#13576=VECTOR('',#100792,1000.);
#13577=VECTOR('',#100793,1000.);
#13578=VECTOR('',#100794,1000.);
#13579=VECTOR('',#100797,1000.);
#13580=VECTOR('',#100798,1000.);
#13581=VECTOR('',#100801,1000.);
#13582=VECTOR('',#100802,1000.);
#13583=VECTOR('',#100803,1000.);
#13584=VECTOR('',#100804,1000.);
#13585=VECTOR('',#100807,1000.);
#13586=VECTOR('',#100808,1000.);
#13587=VECTOR('',#100809,1000.);
#13588=VECTOR('',#100812,1000.);
#13589=VECTOR('',#100813,1000.);
#13590=VECTOR('',#100814,1000.);
#13591=VECTOR('',#100817,1000.);
#13592=VECTOR('',#100818,1000.);
#13593=VECTOR('',#100821,1000.);
#13594=VECTOR('',#100822,1000.);
#13595=VECTOR('',#100823,1000.);
#13596=VECTOR('',#100824,1000.);
#13597=VECTOR('',#100827,1000.);
#13598=VECTOR('',#100828,1000.);
#13599=VECTOR('',#100829,1000.);
#13600=VECTOR('',#100832,1000.);
#13601=VECTOR('',#100833,1000.);
#13602=VECTOR('',#100834,1000.);
#13603=VECTOR('',#100837,1000.);
#13604=VECTOR('',#100838,1000.);
#13605=VECTOR('',#100841,1000.);
#13606=VECTOR('',#100842,1000.);
#13607=VECTOR('',#100843,1000.);
#13608=VECTOR('',#100844,1000.);
#13609=VECTOR('',#100847,1000.);
#13610=VECTOR('',#100848,1000.);
#13611=VECTOR('',#100849,1000.);
#13612=VECTOR('',#100852,1000.);
#13613=VECTOR('',#100853,1000.);
#13614=VECTOR('',#100854,1000.);
#13615=VECTOR('',#100857,1000.);
#13616=VECTOR('',#100858,1000.);
#13617=VECTOR('',#100861,1000.);
#13618=VECTOR('',#100862,1000.);
#13619=VECTOR('',#100863,1000.);
#13620=VECTOR('',#100864,1000.);
#13621=VECTOR('',#100867,1000.);
#13622=VECTOR('',#100868,1000.);
#13623=VECTOR('',#100869,1000.);
#13624=VECTOR('',#100872,1000.);
#13625=VECTOR('',#100873,1000.);
#13626=VECTOR('',#100874,1000.);
#13627=VECTOR('',#100877,1000.);
#13628=VECTOR('',#100878,1000.);
#13629=VECTOR('',#100881,1000.);
#13630=VECTOR('',#100882,1000.);
#13631=VECTOR('',#100883,1000.);
#13632=VECTOR('',#100884,1000.);
#13633=VECTOR('',#100887,1000.);
#13634=VECTOR('',#100888,1000.);
#13635=VECTOR('',#100889,1000.);
#13636=VECTOR('',#100892,1000.);
#13637=VECTOR('',#100893,1000.);
#13638=VECTOR('',#100894,1000.);
#13639=VECTOR('',#100897,1000.);
#13640=VECTOR('',#100898,1000.);
#13641=VECTOR('',#100901,1000.);
#13642=VECTOR('',#100902,1000.);
#13643=VECTOR('',#100903,1000.);
#13644=VECTOR('',#100904,1000.);
#13645=VECTOR('',#100907,1000.);
#13646=VECTOR('',#100908,1000.);
#13647=VECTOR('',#100909,1000.);
#13648=VECTOR('',#100912,1000.);
#13649=VECTOR('',#100913,1000.);
#13650=VECTOR('',#100914,1000.);
#13651=VECTOR('',#100917,1000.);
#13652=VECTOR('',#100918,1000.);
#13653=VECTOR('',#100921,1000.);
#13654=VECTOR('',#100922,1000.);
#13655=VECTOR('',#100923,1000.);
#13656=VECTOR('',#100924,1000.);
#13657=VECTOR('',#100927,1000.);
#13658=VECTOR('',#100928,1000.);
#13659=VECTOR('',#100929,1000.);
#13660=VECTOR('',#100932,1000.);
#13661=VECTOR('',#100933,1000.);
#13662=VECTOR('',#100934,1000.);
#13663=VECTOR('',#100937,1000.);
#13664=VECTOR('',#100938,1000.);
#13665=VECTOR('',#100941,1000.);
#13666=VECTOR('',#100942,1000.);
#13667=VECTOR('',#100943,1000.);
#13668=VECTOR('',#100944,1000.);
#13669=VECTOR('',#100947,1000.);
#13670=VECTOR('',#100948,1000.);
#13671=VECTOR('',#100949,1000.);
#13672=VECTOR('',#100952,1000.);
#13673=VECTOR('',#100953,1000.);
#13674=VECTOR('',#100954,1000.);
#13675=VECTOR('',#100957,1000.);
#13676=VECTOR('',#100958,1000.);
#13677=VECTOR('',#100961,1000.);
#13678=VECTOR('',#100962,1000.);
#13679=VECTOR('',#100963,1000.);
#13680=VECTOR('',#100964,1000.);
#13681=VECTOR('',#100967,1000.);
#13682=VECTOR('',#100968,1000.);
#13683=VECTOR('',#100969,1000.);
#13684=VECTOR('',#100972,1000.);
#13685=VECTOR('',#100973,1000.);
#13686=VECTOR('',#100974,1000.);
#13687=VECTOR('',#100977,1000.);
#13688=VECTOR('',#100978,1000.);
#13689=VECTOR('',#100981,1000.);
#13690=VECTOR('',#100982,1000.);
#13691=VECTOR('',#100983,1000.);
#13692=VECTOR('',#100984,1000.);
#13693=VECTOR('',#100987,1000.);
#13694=VECTOR('',#100988,1000.);
#13695=VECTOR('',#100989,1000.);
#13696=VECTOR('',#100992,1000.);
#13697=VECTOR('',#100993,1000.);
#13698=VECTOR('',#100994,1000.);
#13699=VECTOR('',#100997,1000.);
#13700=VECTOR('',#100998,1000.);
#13701=VECTOR('',#101001,1000.);
#13702=VECTOR('',#101002,1000.);
#13703=VECTOR('',#101003,1000.);
#13704=VECTOR('',#101004,1000.);
#13705=VECTOR('',#101007,1000.);
#13706=VECTOR('',#101008,1000.);
#13707=VECTOR('',#101009,1000.);
#13708=VECTOR('',#101012,1000.);
#13709=VECTOR('',#101013,1000.);
#13710=VECTOR('',#101014,1000.);
#13711=VECTOR('',#101017,1000.);
#13712=VECTOR('',#101018,1000.);
#13713=VECTOR('',#101021,1000.);
#13714=VECTOR('',#101022,1000.);
#13715=VECTOR('',#101023,1000.);
#13716=VECTOR('',#101024,1000.);
#13717=VECTOR('',#101027,1000.);
#13718=VECTOR('',#101028,1000.);
#13719=VECTOR('',#101029,1000.);
#13720=VECTOR('',#101032,1000.);
#13721=VECTOR('',#101033,1000.);
#13722=VECTOR('',#101034,1000.);
#13723=VECTOR('',#101037,1000.);
#13724=VECTOR('',#101038,1000.);
#13725=VECTOR('',#101041,1000.);
#13726=VECTOR('',#101042,1000.);
#13727=VECTOR('',#101043,1000.);
#13728=VECTOR('',#101044,1000.);
#13729=VECTOR('',#101047,1000.);
#13730=VECTOR('',#101048,1000.);
#13731=VECTOR('',#101049,1000.);
#13732=VECTOR('',#101052,1000.);
#13733=VECTOR('',#101053,1000.);
#13734=VECTOR('',#101054,1000.);
#13735=VECTOR('',#101057,1000.);
#13736=VECTOR('',#101058,1000.);
#13737=VECTOR('',#101061,1000.);
#13738=VECTOR('',#101062,1000.);
#13739=VECTOR('',#101063,1000.);
#13740=VECTOR('',#101064,1000.);
#13741=VECTOR('',#101067,1000.);
#13742=VECTOR('',#101068,1000.);
#13743=VECTOR('',#101069,1000.);
#13744=VECTOR('',#101072,1000.);
#13745=VECTOR('',#101073,1000.);
#13746=VECTOR('',#101074,1000.);
#13747=VECTOR('',#101077,1000.);
#13748=VECTOR('',#101078,1000.);
#13749=VECTOR('',#101081,1000.);
#13750=VECTOR('',#101082,1000.);
#13751=VECTOR('',#101083,1000.);
#13752=VECTOR('',#101084,1000.);
#13753=VECTOR('',#101087,1000.);
#13754=VECTOR('',#101088,1000.);
#13755=VECTOR('',#101089,1000.);
#13756=VECTOR('',#101092,1000.);
#13757=VECTOR('',#101093,1000.);
#13758=VECTOR('',#101094,1000.);
#13759=VECTOR('',#101097,1000.);
#13760=VECTOR('',#101098,1000.);
#13761=VECTOR('',#101101,1000.);
#13762=VECTOR('',#101102,1000.);
#13763=VECTOR('',#101103,1000.);
#13764=VECTOR('',#101104,1000.);
#13765=VECTOR('',#101107,1000.);
#13766=VECTOR('',#101108,1000.);
#13767=VECTOR('',#101109,1000.);
#13768=VECTOR('',#101112,1000.);
#13769=VECTOR('',#101113,1000.);
#13770=VECTOR('',#101114,1000.);
#13771=VECTOR('',#101117,1000.);
#13772=VECTOR('',#101118,1000.);
#13773=VECTOR('',#101121,1000.);
#13774=VECTOR('',#101122,1000.);
#13775=VECTOR('',#101123,1000.);
#13776=VECTOR('',#101124,1000.);
#13777=VECTOR('',#101127,1000.);
#13778=VECTOR('',#101128,1000.);
#13779=VECTOR('',#101129,1000.);
#13780=VECTOR('',#101132,1000.);
#13781=VECTOR('',#101133,1000.);
#13782=VECTOR('',#101134,1000.);
#13783=VECTOR('',#101137,1000.);
#13784=VECTOR('',#101138,1000.);
#13785=VECTOR('',#101141,1000.);
#13786=VECTOR('',#101142,1000.);
#13787=VECTOR('',#101143,1000.);
#13788=VECTOR('',#101144,1000.);
#13789=VECTOR('',#101147,1000.);
#13790=VECTOR('',#101148,1000.);
#13791=VECTOR('',#101149,1000.);
#13792=VECTOR('',#101152,1000.);
#13793=VECTOR('',#101153,1000.);
#13794=VECTOR('',#101154,1000.);
#13795=VECTOR('',#101157,1000.);
#13796=VECTOR('',#101158,1000.);
#13797=VECTOR('',#101161,1000.);
#13798=VECTOR('',#101162,1000.);
#13799=VECTOR('',#101163,1000.);
#13800=VECTOR('',#101164,1000.);
#13801=VECTOR('',#101167,1000.);
#13802=VECTOR('',#101168,1000.);
#13803=VECTOR('',#101169,1000.);
#13804=VECTOR('',#101172,1000.);
#13805=VECTOR('',#101173,1000.);
#13806=VECTOR('',#101174,1000.);
#13807=VECTOR('',#101177,1000.);
#13808=VECTOR('',#101178,1000.);
#13809=VECTOR('',#101181,1000.);
#13810=VECTOR('',#101182,1000.);
#13811=VECTOR('',#101183,1000.);
#13812=VECTOR('',#101184,1000.);
#13813=VECTOR('',#101187,1000.);
#13814=VECTOR('',#101188,1000.);
#13815=VECTOR('',#101189,1000.);
#13816=VECTOR('',#101192,1000.);
#13817=VECTOR('',#101193,1000.);
#13818=VECTOR('',#101194,1000.);
#13819=VECTOR('',#101197,1000.);
#13820=VECTOR('',#101198,1000.);
#13821=VECTOR('',#101201,1000.);
#13822=VECTOR('',#101202,1000.);
#13823=VECTOR('',#101203,1000.);
#13824=VECTOR('',#101204,1000.);
#13825=VECTOR('',#101207,1000.);
#13826=VECTOR('',#101208,1000.);
#13827=VECTOR('',#101209,1000.);
#13828=VECTOR('',#101212,1000.);
#13829=VECTOR('',#101213,1000.);
#13830=VECTOR('',#101214,1000.);
#13831=VECTOR('',#101217,1000.);
#13832=VECTOR('',#101218,1000.);
#13833=VECTOR('',#101221,1000.);
#13834=VECTOR('',#101222,1000.);
#13835=VECTOR('',#101223,1000.);
#13836=VECTOR('',#101224,1000.);
#13837=VECTOR('',#101227,1000.);
#13838=VECTOR('',#101228,1000.);
#13839=VECTOR('',#101229,1000.);
#13840=VECTOR('',#101232,1000.);
#13841=VECTOR('',#101233,1000.);
#13842=VECTOR('',#101234,1000.);
#13843=VECTOR('',#101237,1000.);
#13844=VECTOR('',#101238,1000.);
#13845=VECTOR('',#101241,1000.);
#13846=VECTOR('',#101242,1000.);
#13847=VECTOR('',#101243,1000.);
#13848=VECTOR('',#101244,1000.);
#13849=VECTOR('',#101247,1000.);
#13850=VECTOR('',#101248,1000.);
#13851=VECTOR('',#101249,1000.);
#13852=VECTOR('',#101252,1000.);
#13853=VECTOR('',#101253,1000.);
#13854=VECTOR('',#101254,1000.);
#13855=VECTOR('',#101257,1000.);
#13856=VECTOR('',#101258,1000.);
#13857=VECTOR('',#101261,1000.);
#13858=VECTOR('',#101262,1000.);
#13859=VECTOR('',#101263,1000.);
#13860=VECTOR('',#101264,1000.);
#13861=VECTOR('',#101267,1000.);
#13862=VECTOR('',#101268,1000.);
#13863=VECTOR('',#101269,1000.);
#13864=VECTOR('',#101272,1000.);
#13865=VECTOR('',#101273,1000.);
#13866=VECTOR('',#101274,1000.);
#13867=VECTOR('',#101277,1000.);
#13868=VECTOR('',#101278,1000.);
#13869=VECTOR('',#101281,1000.);
#13870=VECTOR('',#101282,1000.);
#13871=VECTOR('',#101283,1000.);
#13872=VECTOR('',#101284,1000.);
#13873=VECTOR('',#101287,1000.);
#13874=VECTOR('',#101288,1000.);
#13875=VECTOR('',#101289,1000.);
#13876=VECTOR('',#101292,1000.);
#13877=VECTOR('',#101293,1000.);
#13878=VECTOR('',#101294,1000.);
#13879=VECTOR('',#101297,1000.);
#13880=VECTOR('',#101298,1000.);
#13881=VECTOR('',#101301,1000.);
#13882=VECTOR('',#101302,1000.);
#13883=VECTOR('',#101303,1000.);
#13884=VECTOR('',#101304,1000.);
#13885=VECTOR('',#101307,1000.);
#13886=VECTOR('',#101308,1000.);
#13887=VECTOR('',#101309,1000.);
#13888=VECTOR('',#101312,1000.);
#13889=VECTOR('',#101313,1000.);
#13890=VECTOR('',#101314,1000.);
#13891=VECTOR('',#101317,1000.);
#13892=VECTOR('',#101318,1000.);
#13893=VECTOR('',#101321,1000.);
#13894=VECTOR('',#101322,1000.);
#13895=VECTOR('',#101323,1000.);
#13896=VECTOR('',#101324,1000.);
#13897=VECTOR('',#101327,1000.);
#13898=VECTOR('',#101328,1000.);
#13899=VECTOR('',#101329,1000.);
#13900=VECTOR('',#101332,1000.);
#13901=VECTOR('',#101333,1000.);
#13902=VECTOR('',#101334,1000.);
#13903=VECTOR('',#101337,1000.);
#13904=VECTOR('',#101338,1000.);
#13905=VECTOR('',#101341,1000.);
#13906=VECTOR('',#101342,1000.);
#13907=VECTOR('',#101343,1000.);
#13908=VECTOR('',#101344,1000.);
#13909=VECTOR('',#101347,1000.);
#13910=VECTOR('',#101348,1000.);
#13911=VECTOR('',#101349,1000.);
#13912=VECTOR('',#101352,1000.);
#13913=VECTOR('',#101353,1000.);
#13914=VECTOR('',#101354,1000.);
#13915=VECTOR('',#101357,1000.);
#13916=VECTOR('',#101358,1000.);
#13917=VECTOR('',#101361,1000.);
#13918=VECTOR('',#101362,1000.);
#13919=VECTOR('',#101363,1000.);
#13920=VECTOR('',#101364,1000.);
#13921=VECTOR('',#101367,1000.);
#13922=VECTOR('',#101368,1000.);
#13923=VECTOR('',#101369,1000.);
#13924=VECTOR('',#101372,1000.);
#13925=VECTOR('',#101373,1000.);
#13926=VECTOR('',#101374,1000.);
#13927=VECTOR('',#101377,1000.);
#13928=VECTOR('',#101378,1000.);
#13929=VECTOR('',#101381,1000.);
#13930=VECTOR('',#101382,1000.);
#13931=VECTOR('',#101383,1000.);
#13932=VECTOR('',#101384,1000.);
#13933=VECTOR('',#101387,1000.);
#13934=VECTOR('',#101388,1000.);
#13935=VECTOR('',#101389,1000.);
#13936=VECTOR('',#101392,1000.);
#13937=VECTOR('',#101393,1000.);
#13938=VECTOR('',#101394,1000.);
#13939=VECTOR('',#101397,1000.);
#13940=VECTOR('',#101398,1000.);
#13941=VECTOR('',#101401,1000.);
#13942=VECTOR('',#101402,1000.);
#13943=VECTOR('',#101403,1000.);
#13944=VECTOR('',#101404,1000.);
#13945=VECTOR('',#101407,1000.);
#13946=VECTOR('',#101408,1000.);
#13947=VECTOR('',#101409,1000.);
#13948=VECTOR('',#101412,1000.);
#13949=VECTOR('',#101413,1000.);
#13950=VECTOR('',#101414,1000.);
#13951=VECTOR('',#101417,1000.);
#13952=VECTOR('',#101418,1000.);
#13953=VECTOR('',#101421,1000.);
#13954=VECTOR('',#101422,1000.);
#13955=VECTOR('',#101423,1000.);
#13956=VECTOR('',#101424,1000.);
#13957=VECTOR('',#101427,1000.);
#13958=VECTOR('',#101428,1000.);
#13959=VECTOR('',#101429,1000.);
#13960=VECTOR('',#101432,1000.);
#13961=VECTOR('',#101433,1000.);
#13962=VECTOR('',#101434,1000.);
#13963=VECTOR('',#101437,1000.);
#13964=VECTOR('',#101438,1000.);
#13965=VECTOR('',#101441,1000.);
#13966=VECTOR('',#101442,1000.);
#13967=VECTOR('',#101443,1000.);
#13968=VECTOR('',#101444,1000.);
#13969=VECTOR('',#101447,1000.);
#13970=VECTOR('',#101448,1000.);
#13971=VECTOR('',#101449,1000.);
#13972=VECTOR('',#101452,1000.);
#13973=VECTOR('',#101453,1000.);
#13974=VECTOR('',#101454,1000.);
#13975=VECTOR('',#101457,1000.);
#13976=VECTOR('',#101458,1000.);
#13977=VECTOR('',#101461,1000.);
#13978=VECTOR('',#101462,1000.);
#13979=VECTOR('',#101463,1000.);
#13980=VECTOR('',#101464,1000.);
#13981=VECTOR('',#101467,1000.);
#13982=VECTOR('',#101468,1000.);
#13983=VECTOR('',#101469,1000.);
#13984=VECTOR('',#101472,1000.);
#13985=VECTOR('',#101473,1000.);
#13986=VECTOR('',#101474,1000.);
#13987=VECTOR('',#101477,1000.);
#13988=VECTOR('',#101478,1000.);
#13989=VECTOR('',#101481,1000.);
#13990=VECTOR('',#101482,1000.);
#13991=VECTOR('',#101483,1000.);
#13992=VECTOR('',#101484,1000.);
#13993=VECTOR('',#101487,1000.);
#13994=VECTOR('',#101488,1000.);
#13995=VECTOR('',#101489,1000.);
#13996=VECTOR('',#101492,1000.);
#13997=VECTOR('',#101493,1000.);
#13998=VECTOR('',#101494,1000.);
#13999=VECTOR('',#101497,1000.);
#14000=VECTOR('',#101498,1000.);
#14001=VECTOR('',#101501,1000.);
#14002=VECTOR('',#101502,1000.);
#14003=VECTOR('',#101503,1000.);
#14004=VECTOR('',#101504,1000.);
#14005=VECTOR('',#101507,1000.);
#14006=VECTOR('',#101508,1000.);
#14007=VECTOR('',#101509,1000.);
#14008=VECTOR('',#101512,1000.);
#14009=VECTOR('',#101513,1000.);
#14010=VECTOR('',#101514,1000.);
#14011=VECTOR('',#101517,1000.);
#14012=VECTOR('',#101518,1000.);
#14013=VECTOR('',#101521,1000.);
#14014=VECTOR('',#101522,1000.);
#14015=VECTOR('',#101523,1000.);
#14016=VECTOR('',#101524,1000.);
#14017=VECTOR('',#101527,1000.);
#14018=VECTOR('',#101528,1000.);
#14019=VECTOR('',#101529,1000.);
#14020=VECTOR('',#101532,1000.);
#14021=VECTOR('',#101533,1000.);
#14022=VECTOR('',#101534,1000.);
#14023=VECTOR('',#101537,1000.);
#14024=VECTOR('',#101538,1000.);
#14025=VECTOR('',#101541,1000.);
#14026=VECTOR('',#101542,1000.);
#14027=VECTOR('',#101543,1000.);
#14028=VECTOR('',#101544,1000.);
#14029=VECTOR('',#101547,1000.);
#14030=VECTOR('',#101548,1000.);
#14031=VECTOR('',#101549,1000.);
#14032=VECTOR('',#101552,1000.);
#14033=VECTOR('',#101553,1000.);
#14034=VECTOR('',#101554,1000.);
#14035=VECTOR('',#101557,1000.);
#14036=VECTOR('',#101558,1000.);
#14037=VECTOR('',#101561,1000.);
#14038=VECTOR('',#101562,1000.);
#14039=VECTOR('',#101563,1000.);
#14040=VECTOR('',#101564,1000.);
#14041=VECTOR('',#101567,1000.);
#14042=VECTOR('',#101568,1000.);
#14043=VECTOR('',#101569,1000.);
#14044=VECTOR('',#101572,1000.);
#14045=VECTOR('',#101573,1000.);
#14046=VECTOR('',#101574,1000.);
#14047=VECTOR('',#101577,1000.);
#14048=VECTOR('',#101578,1000.);
#14049=VECTOR('',#101581,1000.);
#14050=VECTOR('',#101582,1000.);
#14051=VECTOR('',#101583,1000.);
#14052=VECTOR('',#101584,1000.);
#14053=VECTOR('',#101587,1000.);
#14054=VECTOR('',#101588,1000.);
#14055=VECTOR('',#101589,1000.);
#14056=VECTOR('',#101592,1000.);
#14057=VECTOR('',#101593,1000.);
#14058=VECTOR('',#101594,1000.);
#14059=VECTOR('',#101597,1000.);
#14060=VECTOR('',#101598,1000.);
#14061=VECTOR('',#101601,1000.);
#14062=VECTOR('',#101602,1000.);
#14063=VECTOR('',#101603,1000.);
#14064=VECTOR('',#101604,1000.);
#14065=VECTOR('',#101607,1000.);
#14066=VECTOR('',#101608,1000.);
#14067=VECTOR('',#101609,1000.);
#14068=VECTOR('',#101612,1000.);
#14069=VECTOR('',#101613,1000.);
#14070=VECTOR('',#101614,1000.);
#14071=VECTOR('',#101617,1000.);
#14072=VECTOR('',#101618,1000.);
#14073=VECTOR('',#101621,1000.);
#14074=VECTOR('',#101622,1000.);
#14075=VECTOR('',#101623,1000.);
#14076=VECTOR('',#101624,1000.);
#14077=VECTOR('',#101627,1000.);
#14078=VECTOR('',#101628,1000.);
#14079=VECTOR('',#101629,1000.);
#14080=VECTOR('',#101632,1000.);
#14081=VECTOR('',#101633,1000.);
#14082=VECTOR('',#101634,1000.);
#14083=VECTOR('',#101637,1000.);
#14084=VECTOR('',#101638,1000.);
#14085=VECTOR('',#101641,1000.);
#14086=VECTOR('',#101642,1000.);
#14087=VECTOR('',#101643,1000.);
#14088=VECTOR('',#101644,1000.);
#14089=VECTOR('',#101647,1000.);
#14090=VECTOR('',#101648,1000.);
#14091=VECTOR('',#101649,1000.);
#14092=VECTOR('',#101652,1000.);
#14093=VECTOR('',#101653,1000.);
#14094=VECTOR('',#101654,1000.);
#14095=VECTOR('',#101657,1000.);
#14096=VECTOR('',#101658,1000.);
#14097=VECTOR('',#101661,1000.);
#14098=VECTOR('',#101662,1000.);
#14099=VECTOR('',#101663,1000.);
#14100=VECTOR('',#101664,1000.);
#14101=VECTOR('',#101667,1000.);
#14102=VECTOR('',#101668,1000.);
#14103=VECTOR('',#101669,1000.);
#14104=VECTOR('',#101672,1000.);
#14105=VECTOR('',#101673,1000.);
#14106=VECTOR('',#101674,1000.);
#14107=VECTOR('',#101677,1000.);
#14108=VECTOR('',#101678,1000.);
#14109=VECTOR('',#101681,1000.);
#14110=VECTOR('',#101682,1000.);
#14111=VECTOR('',#101683,1000.);
#14112=VECTOR('',#101684,1000.);
#14113=VECTOR('',#101687,1000.);
#14114=VECTOR('',#101688,1000.);
#14115=VECTOR('',#101689,1000.);
#14116=VECTOR('',#101692,1000.);
#14117=VECTOR('',#101693,1000.);
#14118=VECTOR('',#101694,1000.);
#14119=VECTOR('',#101697,1000.);
#14120=VECTOR('',#101698,1000.);
#14121=VECTOR('',#101701,1000.);
#14122=VECTOR('',#101702,1000.);
#14123=VECTOR('',#101703,1000.);
#14124=VECTOR('',#101704,1000.);
#14125=VECTOR('',#101707,1000.);
#14126=VECTOR('',#101708,1000.);
#14127=VECTOR('',#101709,1000.);
#14128=VECTOR('',#101712,1000.);
#14129=VECTOR('',#101713,1000.);
#14130=VECTOR('',#101714,1000.);
#14131=VECTOR('',#101717,1000.);
#14132=VECTOR('',#101718,1000.);
#14133=VECTOR('',#101721,1000.);
#14134=VECTOR('',#101722,1000.);
#14135=VECTOR('',#101723,1000.);
#14136=VECTOR('',#101724,1000.);
#14137=VECTOR('',#101727,1000.);
#14138=VECTOR('',#101728,1000.);
#14139=VECTOR('',#101729,1000.);
#14140=VECTOR('',#101732,1000.);
#14141=VECTOR('',#101733,1000.);
#14142=VECTOR('',#101734,1000.);
#14143=VECTOR('',#101737,1000.);
#14144=VECTOR('',#101738,1000.);
#14145=VECTOR('',#101741,1000.);
#14146=VECTOR('',#101742,1000.);
#14147=VECTOR('',#101743,1000.);
#14148=VECTOR('',#101744,1000.);
#14149=VECTOR('',#101747,1000.);
#14150=VECTOR('',#101748,1000.);
#14151=VECTOR('',#101749,1000.);
#14152=VECTOR('',#101752,1000.);
#14153=VECTOR('',#101753,1000.);
#14154=VECTOR('',#101754,1000.);
#14155=VECTOR('',#101757,1000.);
#14156=VECTOR('',#101758,1000.);
#14157=VECTOR('',#101761,1000.);
#14158=VECTOR('',#101762,1000.);
#14159=VECTOR('',#101763,1000.);
#14160=VECTOR('',#101764,1000.);
#14161=VECTOR('',#101767,1000.);
#14162=VECTOR('',#101768,1000.);
#14163=VECTOR('',#101769,1000.);
#14164=VECTOR('',#101772,1000.);
#14165=VECTOR('',#101773,1000.);
#14166=VECTOR('',#101774,1000.);
#14167=VECTOR('',#101777,1000.);
#14168=VECTOR('',#101778,1000.);
#14169=VECTOR('',#101781,1000.);
#14170=VECTOR('',#101782,1000.);
#14171=VECTOR('',#101783,1000.);
#14172=VECTOR('',#101784,1000.);
#14173=VECTOR('',#101787,1000.);
#14174=VECTOR('',#101788,1000.);
#14175=VECTOR('',#101789,1000.);
#14176=VECTOR('',#101792,1000.);
#14177=VECTOR('',#101793,1000.);
#14178=VECTOR('',#101794,1000.);
#14179=VECTOR('',#101797,1000.);
#14180=VECTOR('',#101798,1000.);
#14181=VECTOR('',#101801,1000.);
#14182=VECTOR('',#101802,1000.);
#14183=VECTOR('',#101803,1000.);
#14184=VECTOR('',#101804,1000.);
#14185=VECTOR('',#101807,1000.);
#14186=VECTOR('',#101808,1000.);
#14187=VECTOR('',#101809,1000.);
#14188=VECTOR('',#101812,1000.);
#14189=VECTOR('',#101813,1000.);
#14190=VECTOR('',#101814,1000.);
#14191=VECTOR('',#101817,1000.);
#14192=VECTOR('',#101818,1000.);
#14193=VECTOR('',#101821,1000.);
#14194=VECTOR('',#101822,1000.);
#14195=VECTOR('',#101823,1000.);
#14196=VECTOR('',#101824,1000.);
#14197=VECTOR('',#101827,1000.);
#14198=VECTOR('',#101828,1000.);
#14199=VECTOR('',#101829,1000.);
#14200=VECTOR('',#101832,1000.);
#14201=VECTOR('',#101833,1000.);
#14202=VECTOR('',#101834,1000.);
#14203=VECTOR('',#101837,1000.);
#14204=VECTOR('',#101838,1000.);
#14205=VECTOR('',#101841,1000.);
#14206=VECTOR('',#101842,1000.);
#14207=VECTOR('',#101843,1000.);
#14208=VECTOR('',#101844,1000.);
#14209=VECTOR('',#101847,1000.);
#14210=VECTOR('',#101848,1000.);
#14211=VECTOR('',#101849,1000.);
#14212=VECTOR('',#101852,1000.);
#14213=VECTOR('',#101853,1000.);
#14214=VECTOR('',#101854,1000.);
#14215=VECTOR('',#101857,1000.);
#14216=VECTOR('',#101858,1000.);
#14217=VECTOR('',#101861,1000.);
#14218=VECTOR('',#101862,1000.);
#14219=VECTOR('',#101863,1000.);
#14220=VECTOR('',#101864,1000.);
#14221=VECTOR('',#101867,1000.);
#14222=VECTOR('',#101868,1000.);
#14223=VECTOR('',#101869,1000.);
#14224=VECTOR('',#101872,1000.);
#14225=VECTOR('',#101873,1000.);
#14226=VECTOR('',#101874,1000.);
#14227=VECTOR('',#101877,1000.);
#14228=VECTOR('',#101878,1000.);
#14229=VECTOR('',#101881,1000.);
#14230=VECTOR('',#101882,1000.);
#14231=VECTOR('',#101883,1000.);
#14232=VECTOR('',#101884,1000.);
#14233=VECTOR('',#101887,1000.);
#14234=VECTOR('',#101888,1000.);
#14235=VECTOR('',#101889,1000.);
#14236=VECTOR('',#101892,1000.);
#14237=VECTOR('',#101893,1000.);
#14238=VECTOR('',#101894,1000.);
#14239=VECTOR('',#101897,1000.);
#14240=VECTOR('',#101898,1000.);
#14241=VECTOR('',#101901,1000.);
#14242=VECTOR('',#101902,1000.);
#14243=VECTOR('',#101903,1000.);
#14244=VECTOR('',#101904,1000.);
#14245=VECTOR('',#101907,1000.);
#14246=VECTOR('',#101908,1000.);
#14247=VECTOR('',#101909,1000.);
#14248=VECTOR('',#101912,1000.);
#14249=VECTOR('',#101913,1000.);
#14250=VECTOR('',#101914,1000.);
#14251=VECTOR('',#101917,1000.);
#14252=VECTOR('',#101918,1000.);
#14253=VECTOR('',#101921,1000.);
#14254=VECTOR('',#101922,1000.);
#14255=VECTOR('',#101923,1000.);
#14256=VECTOR('',#101924,1000.);
#14257=VECTOR('',#101927,1000.);
#14258=VECTOR('',#101928,1000.);
#14259=VECTOR('',#101929,1000.);
#14260=VECTOR('',#101932,1000.);
#14261=VECTOR('',#101933,1000.);
#14262=VECTOR('',#101934,1000.);
#14263=VECTOR('',#101937,1000.);
#14264=VECTOR('',#101938,1000.);
#14265=VECTOR('',#101941,1000.);
#14266=VECTOR('',#101942,1000.);
#14267=VECTOR('',#101943,1000.);
#14268=VECTOR('',#101944,1000.);
#14269=VECTOR('',#101947,1000.);
#14270=VECTOR('',#101948,1000.);
#14271=VECTOR('',#101949,1000.);
#14272=VECTOR('',#101952,1000.);
#14273=VECTOR('',#101953,1000.);
#14274=VECTOR('',#101954,1000.);
#14275=VECTOR('',#101957,1000.);
#14276=VECTOR('',#101958,1000.);
#14277=VECTOR('',#101961,1000.);
#14278=VECTOR('',#101962,1000.);
#14279=VECTOR('',#101963,1000.);
#14280=VECTOR('',#101964,1000.);
#14281=VECTOR('',#101967,1000.);
#14282=VECTOR('',#101968,1000.);
#14283=VECTOR('',#101969,1000.);
#14284=VECTOR('',#101972,1000.);
#14285=VECTOR('',#101973,1000.);
#14286=VECTOR('',#101974,1000.);
#14287=VECTOR('',#101977,1000.);
#14288=VECTOR('',#101978,1000.);
#14289=VECTOR('',#101981,1000.);
#14290=VECTOR('',#101982,1000.);
#14291=VECTOR('',#101983,1000.);
#14292=VECTOR('',#101984,1000.);
#14293=VECTOR('',#101987,1000.);
#14294=VECTOR('',#101988,1000.);
#14295=VECTOR('',#101989,1000.);
#14296=VECTOR('',#101992,1000.);
#14297=VECTOR('',#101993,1000.);
#14298=VECTOR('',#101994,1000.);
#14299=VECTOR('',#101997,1000.);
#14300=VECTOR('',#101998,1000.);
#14301=VECTOR('',#102001,1000.);
#14302=VECTOR('',#102002,1000.);
#14303=VECTOR('',#102003,1000.);
#14304=VECTOR('',#102004,1000.);
#14305=VECTOR('',#102007,1000.);
#14306=VECTOR('',#102008,1000.);
#14307=VECTOR('',#102009,1000.);
#14308=VECTOR('',#102012,1000.);
#14309=VECTOR('',#102013,1000.);
#14310=VECTOR('',#102014,1000.);
#14311=VECTOR('',#102017,1000.);
#14312=VECTOR('',#102018,1000.);
#14313=VECTOR('',#102021,1000.);
#14314=VECTOR('',#102022,1000.);
#14315=VECTOR('',#102023,1000.);
#14316=VECTOR('',#102024,1000.);
#14317=VECTOR('',#102027,1000.);
#14318=VECTOR('',#102028,1000.);
#14319=VECTOR('',#102029,1000.);
#14320=VECTOR('',#102032,1000.);
#14321=VECTOR('',#102033,1000.);
#14322=VECTOR('',#102034,1000.);
#14323=VECTOR('',#102037,1000.);
#14324=VECTOR('',#102038,1000.);
#14325=VECTOR('',#102041,1000.);
#14326=VECTOR('',#102042,1000.);
#14327=VECTOR('',#102043,1000.);
#14328=VECTOR('',#102044,1000.);
#14329=VECTOR('',#102047,1000.);
#14330=VECTOR('',#102048,1000.);
#14331=VECTOR('',#102049,1000.);
#14332=VECTOR('',#102052,1000.);
#14333=VECTOR('',#102053,1000.);
#14334=VECTOR('',#102054,1000.);
#14335=VECTOR('',#102057,1000.);
#14336=VECTOR('',#102058,1000.);
#14337=VECTOR('',#102061,1000.);
#14338=VECTOR('',#102062,1000.);
#14339=VECTOR('',#102063,1000.);
#14340=VECTOR('',#102064,1000.);
#14341=VECTOR('',#102067,1000.);
#14342=VECTOR('',#102068,1000.);
#14343=VECTOR('',#102069,1000.);
#14344=VECTOR('',#102072,1000.);
#14345=VECTOR('',#102073,1000.);
#14346=VECTOR('',#102074,1000.);
#14347=VECTOR('',#102077,1000.);
#14348=VECTOR('',#102078,1000.);
#14349=VECTOR('',#102081,1000.);
#14350=VECTOR('',#102082,1000.);
#14351=VECTOR('',#102083,1000.);
#14352=VECTOR('',#102084,1000.);
#14353=VECTOR('',#102087,1000.);
#14354=VECTOR('',#102088,1000.);
#14355=VECTOR('',#102089,1000.);
#14356=VECTOR('',#102092,1000.);
#14357=VECTOR('',#102093,1000.);
#14358=VECTOR('',#102094,1000.);
#14359=VECTOR('',#102097,1000.);
#14360=VECTOR('',#102098,1000.);
#14361=VECTOR('',#102101,1000.);
#14362=VECTOR('',#102102,1000.);
#14363=VECTOR('',#102103,1000.);
#14364=VECTOR('',#102104,1000.);
#14365=VECTOR('',#102107,1000.);
#14366=VECTOR('',#102108,1000.);
#14367=VECTOR('',#102109,1000.);
#14368=VECTOR('',#102112,1000.);
#14369=VECTOR('',#102113,1000.);
#14370=VECTOR('',#102114,1000.);
#14371=VECTOR('',#102117,1000.);
#14372=VECTOR('',#102118,1000.);
#14373=VECTOR('',#102121,1000.);
#14374=VECTOR('',#102122,1000.);
#14375=VECTOR('',#102123,1000.);
#14376=VECTOR('',#102124,1000.);
#14377=VECTOR('',#102127,1000.);
#14378=VECTOR('',#102128,1000.);
#14379=VECTOR('',#102129,1000.);
#14380=VECTOR('',#102132,1000.);
#14381=VECTOR('',#102133,1000.);
#14382=VECTOR('',#102134,1000.);
#14383=VECTOR('',#102137,1000.);
#14384=VECTOR('',#102138,1000.);
#14385=VECTOR('',#102141,1000.);
#14386=VECTOR('',#102142,1000.);
#14387=VECTOR('',#102143,1000.);
#14388=VECTOR('',#102144,1000.);
#14389=VECTOR('',#102147,1000.);
#14390=VECTOR('',#102148,1000.);
#14391=VECTOR('',#102149,1000.);
#14392=VECTOR('',#102152,1000.);
#14393=VECTOR('',#102153,1000.);
#14394=VECTOR('',#102154,1000.);
#14395=VECTOR('',#102157,1000.);
#14396=VECTOR('',#102158,1000.);
#14397=VECTOR('',#102161,1000.);
#14398=VECTOR('',#102162,1000.);
#14399=VECTOR('',#102163,1000.);
#14400=VECTOR('',#102164,1000.);
#14401=VECTOR('',#102167,1000.);
#14402=VECTOR('',#102168,1000.);
#14403=VECTOR('',#102169,1000.);
#14404=VECTOR('',#102172,1000.);
#14405=VECTOR('',#102173,1000.);
#14406=VECTOR('',#102174,1000.);
#14407=VECTOR('',#102177,1000.);
#14408=VECTOR('',#102178,1000.);
#14409=VECTOR('',#102181,1000.);
#14410=VECTOR('',#102182,1000.);
#14411=VECTOR('',#102183,1000.);
#14412=VECTOR('',#102184,1000.);
#14413=VECTOR('',#102187,1000.);
#14414=VECTOR('',#102188,1000.);
#14415=VECTOR('',#102189,1000.);
#14416=VECTOR('',#102192,1000.);
#14417=VECTOR('',#102193,1000.);
#14418=VECTOR('',#102194,1000.);
#14419=VECTOR('',#102197,1000.);
#14420=VECTOR('',#102198,1000.);
#14421=VECTOR('',#102201,1000.);
#14422=VECTOR('',#102202,1000.);
#14423=VECTOR('',#102203,1000.);
#14424=VECTOR('',#102204,1000.);
#14425=VECTOR('',#102207,1000.);
#14426=VECTOR('',#102208,1000.);
#14427=VECTOR('',#102209,1000.);
#14428=VECTOR('',#102212,1000.);
#14429=VECTOR('',#102213,1000.);
#14430=VECTOR('',#102214,1000.);
#14431=VECTOR('',#102217,1000.);
#14432=VECTOR('',#102218,1000.);
#14433=VECTOR('',#102221,1000.);
#14434=VECTOR('',#102222,1000.);
#14435=VECTOR('',#102223,1000.);
#14436=VECTOR('',#102224,1000.);
#14437=VECTOR('',#102227,1000.);
#14438=VECTOR('',#102228,1000.);
#14439=VECTOR('',#102229,1000.);
#14440=VECTOR('',#102232,1000.);
#14441=VECTOR('',#102233,1000.);
#14442=VECTOR('',#102234,1000.);
#14443=VECTOR('',#102237,1000.);
#14444=VECTOR('',#102238,1000.);
#14445=VECTOR('',#102241,1000.);
#14446=VECTOR('',#102242,1000.);
#14447=VECTOR('',#102243,1000.);
#14448=VECTOR('',#102244,1000.);
#14449=VECTOR('',#102247,1000.);
#14450=VECTOR('',#102248,1000.);
#14451=VECTOR('',#102249,1000.);
#14452=VECTOR('',#102252,1000.);
#14453=VECTOR('',#102253,1000.);
#14454=VECTOR('',#102254,1000.);
#14455=VECTOR('',#102257,1000.);
#14456=VECTOR('',#102258,1000.);
#14457=VECTOR('',#102261,1000.);
#14458=VECTOR('',#102262,1000.);
#14459=VECTOR('',#102263,1000.);
#14460=VECTOR('',#102264,1000.);
#14461=VECTOR('',#102267,1000.);
#14462=VECTOR('',#102268,1000.);
#14463=VECTOR('',#102269,1000.);
#14464=VECTOR('',#102272,1000.);
#14465=VECTOR('',#102273,1000.);
#14466=VECTOR('',#102274,1000.);
#14467=VECTOR('',#102277,1000.);
#14468=VECTOR('',#102278,1000.);
#14469=VECTOR('',#102281,1000.);
#14470=VECTOR('',#102282,1000.);
#14471=VECTOR('',#102283,1000.);
#14472=VECTOR('',#102284,1000.);
#14473=VECTOR('',#102287,1000.);
#14474=VECTOR('',#102288,1000.);
#14475=VECTOR('',#102289,1000.);
#14476=VECTOR('',#102292,1000.);
#14477=VECTOR('',#102293,1000.);
#14478=VECTOR('',#102294,1000.);
#14479=VECTOR('',#102297,1000.);
#14480=VECTOR('',#102298,1000.);
#14481=VECTOR('',#102301,1000.);
#14482=VECTOR('',#102302,1000.);
#14483=VECTOR('',#102303,1000.);
#14484=VECTOR('',#102304,1000.);
#14485=VECTOR('',#102307,1000.);
#14486=VECTOR('',#102308,1000.);
#14487=VECTOR('',#102309,1000.);
#14488=VECTOR('',#102312,1000.);
#14489=VECTOR('',#102313,1000.);
#14490=VECTOR('',#102314,1000.);
#14491=VECTOR('',#102317,1000.);
#14492=VECTOR('',#102318,1000.);
#14493=VECTOR('',#102321,1000.);
#14494=VECTOR('',#102322,1000.);
#14495=VECTOR('',#102323,1000.);
#14496=VECTOR('',#102324,1000.);
#14497=VECTOR('',#102327,1000.);
#14498=VECTOR('',#102328,1000.);
#14499=VECTOR('',#102329,1000.);
#14500=VECTOR('',#102332,1000.);
#14501=VECTOR('',#102333,1000.);
#14502=VECTOR('',#102334,1000.);
#14503=VECTOR('',#102337,1000.);
#14504=VECTOR('',#102338,1000.);
#14505=VECTOR('',#102341,1000.);
#14506=VECTOR('',#102342,1000.);
#14507=VECTOR('',#102343,1000.);
#14508=VECTOR('',#102344,1000.);
#14509=VECTOR('',#102347,1000.);
#14510=VECTOR('',#102348,1000.);
#14511=VECTOR('',#102349,1000.);
#14512=VECTOR('',#102352,1000.);
#14513=VECTOR('',#102353,1000.);
#14514=VECTOR('',#102354,1000.);
#14515=VECTOR('',#102357,1000.);
#14516=VECTOR('',#102358,1000.);
#14517=VECTOR('',#102361,1000.);
#14518=VECTOR('',#102362,1000.);
#14519=VECTOR('',#102363,1000.);
#14520=VECTOR('',#102364,1000.);
#14521=VECTOR('',#102367,1000.);
#14522=VECTOR('',#102368,1000.);
#14523=VECTOR('',#102369,1000.);
#14524=VECTOR('',#102372,1000.);
#14525=VECTOR('',#102373,1000.);
#14526=VECTOR('',#102374,1000.);
#14527=VECTOR('',#102377,1000.);
#14528=VECTOR('',#102378,1000.);
#14529=VECTOR('',#102381,1000.);
#14530=VECTOR('',#102382,1000.);
#14531=VECTOR('',#102383,1000.);
#14532=VECTOR('',#102384,1000.);
#14533=VECTOR('',#102387,1000.);
#14534=VECTOR('',#102388,1000.);
#14535=VECTOR('',#102389,1000.);
#14536=VECTOR('',#102392,1000.);
#14537=VECTOR('',#102393,1000.);
#14538=VECTOR('',#102394,1000.);
#14539=VECTOR('',#102397,1000.);
#14540=VECTOR('',#102398,1000.);
#14541=VECTOR('',#102401,1000.);
#14542=VECTOR('',#102402,1000.);
#14543=VECTOR('',#102403,1000.);
#14544=VECTOR('',#102404,1000.);
#14545=VECTOR('',#102407,1000.);
#14546=VECTOR('',#102408,1000.);
#14547=VECTOR('',#102409,1000.);
#14548=VECTOR('',#102412,1000.);
#14549=VECTOR('',#102413,1000.);
#14550=VECTOR('',#102414,1000.);
#14551=VECTOR('',#102417,1000.);
#14552=VECTOR('',#102418,1000.);
#14553=VECTOR('',#102421,1000.);
#14554=VECTOR('',#102422,1000.);
#14555=VECTOR('',#102423,1000.);
#14556=VECTOR('',#102424,1000.);
#14557=VECTOR('',#102427,1000.);
#14558=VECTOR('',#102428,1000.);
#14559=VECTOR('',#102429,1000.);
#14560=VECTOR('',#102432,1000.);
#14561=VECTOR('',#102433,1000.);
#14562=VECTOR('',#102434,1000.);
#14563=VECTOR('',#102437,1000.);
#14564=VECTOR('',#102438,1000.);
#14565=VECTOR('',#102441,1000.);
#14566=VECTOR('',#102442,1000.);
#14567=VECTOR('',#102443,1000.);
#14568=VECTOR('',#102444,1000.);
#14569=VECTOR('',#102447,1000.);
#14570=VECTOR('',#102448,1000.);
#14571=VECTOR('',#102449,1000.);
#14572=VECTOR('',#102452,1000.);
#14573=VECTOR('',#102453,1000.);
#14574=VECTOR('',#102454,1000.);
#14575=VECTOR('',#102457,1000.);
#14576=VECTOR('',#102458,1000.);
#14577=VECTOR('',#102461,1000.);
#14578=VECTOR('',#102462,1000.);
#14579=VECTOR('',#102463,1000.);
#14580=VECTOR('',#102464,1000.);
#14581=VECTOR('',#102467,1000.);
#14582=VECTOR('',#102468,1000.);
#14583=VECTOR('',#102469,1000.);
#14584=VECTOR('',#102472,1000.);
#14585=VECTOR('',#102473,1000.);
#14586=VECTOR('',#102474,1000.);
#14587=VECTOR('',#102477,1000.);
#14588=VECTOR('',#102478,1000.);
#14589=VECTOR('',#102481,1000.);
#14590=VECTOR('',#102482,1000.);
#14591=VECTOR('',#102483,1000.);
#14592=VECTOR('',#102484,1000.);
#14593=VECTOR('',#102487,1000.);
#14594=VECTOR('',#102488,1000.);
#14595=VECTOR('',#102489,1000.);
#14596=VECTOR('',#102492,1000.);
#14597=VECTOR('',#102493,1000.);
#14598=VECTOR('',#102494,1000.);
#14599=VECTOR('',#102497,1000.);
#14600=VECTOR('',#102498,1000.);
#14601=VECTOR('',#102501,1000.);
#14602=VECTOR('',#102502,1000.);
#14603=VECTOR('',#102503,1000.);
#14604=VECTOR('',#102504,1000.);
#14605=VECTOR('',#102507,1000.);
#14606=VECTOR('',#102508,1000.);
#14607=VECTOR('',#102509,1000.);
#14608=VECTOR('',#102512,1000.);
#14609=VECTOR('',#102513,1000.);
#14610=VECTOR('',#102514,1000.);
#14611=VECTOR('',#102517,1000.);
#14612=VECTOR('',#102518,1000.);
#14613=VECTOR('',#102521,1000.);
#14614=VECTOR('',#102522,1000.);
#14615=VECTOR('',#102523,1000.);
#14616=VECTOR('',#102524,1000.);
#14617=VECTOR('',#102527,1000.);
#14618=VECTOR('',#102528,1000.);
#14619=VECTOR('',#102529,1000.);
#14620=VECTOR('',#102532,1000.);
#14621=VECTOR('',#102533,1000.);
#14622=VECTOR('',#102534,1000.);
#14623=VECTOR('',#102537,1000.);
#14624=VECTOR('',#102538,1000.);
#14625=VECTOR('',#102541,1000.);
#14626=VECTOR('',#102542,1000.);
#14627=VECTOR('',#102543,1000.);
#14628=VECTOR('',#102544,1000.);
#14629=VECTOR('',#102547,1000.);
#14630=VECTOR('',#102548,1000.);
#14631=VECTOR('',#102549,1000.);
#14632=VECTOR('',#102552,1000.);
#14633=VECTOR('',#102553,1000.);
#14634=VECTOR('',#102554,1000.);
#14635=VECTOR('',#102557,1000.);
#14636=VECTOR('',#102558,1000.);
#14637=VECTOR('',#102561,1000.);
#14638=VECTOR('',#102562,1000.);
#14639=VECTOR('',#102563,1000.);
#14640=VECTOR('',#102564,1000.);
#14641=VECTOR('',#102567,1000.);
#14642=VECTOR('',#102568,1000.);
#14643=VECTOR('',#102569,1000.);
#14644=VECTOR('',#102572,1000.);
#14645=VECTOR('',#102573,1000.);
#14646=VECTOR('',#102574,1000.);
#14647=VECTOR('',#102577,1000.);
#14648=VECTOR('',#102578,1000.);
#14649=VECTOR('',#102581,1000.);
#14650=VECTOR('',#102582,1000.);
#14651=VECTOR('',#102583,1000.);
#14652=VECTOR('',#102584,1000.);
#14653=VECTOR('',#102587,1000.);
#14654=VECTOR('',#102588,1000.);
#14655=VECTOR('',#102589,1000.);
#14656=VECTOR('',#102592,1000.);
#14657=VECTOR('',#102593,1000.);
#14658=VECTOR('',#102594,1000.);
#14659=VECTOR('',#102597,1000.);
#14660=VECTOR('',#102598,1000.);
#14661=VECTOR('',#102601,1000.);
#14662=VECTOR('',#102602,1000.);
#14663=VECTOR('',#102603,1000.);
#14664=VECTOR('',#102604,1000.);
#14665=VECTOR('',#102607,1000.);
#14666=VECTOR('',#102608,1000.);
#14667=VECTOR('',#102609,1000.);
#14668=VECTOR('',#102612,1000.);
#14669=VECTOR('',#102613,1000.);
#14670=VECTOR('',#102614,1000.);
#14671=VECTOR('',#102617,1000.);
#14672=VECTOR('',#102618,1000.);
#14673=VECTOR('',#102621,1000.);
#14674=VECTOR('',#102622,1000.);
#14675=VECTOR('',#102623,1000.);
#14676=VECTOR('',#102624,1000.);
#14677=VECTOR('',#102627,1000.);
#14678=VECTOR('',#102628,1000.);
#14679=VECTOR('',#102629,1000.);
#14680=VECTOR('',#102632,1000.);
#14681=VECTOR('',#102633,1000.);
#14682=VECTOR('',#102634,1000.);
#14683=VECTOR('',#102637,1000.);
#14684=VECTOR('',#102638,1000.);
#14685=VECTOR('',#102641,1000.);
#14686=VECTOR('',#102642,1000.);
#14687=VECTOR('',#102643,1000.);
#14688=VECTOR('',#102644,1000.);
#14689=VECTOR('',#102647,1000.);
#14690=VECTOR('',#102648,1000.);
#14691=VECTOR('',#102649,1000.);
#14692=VECTOR('',#102652,1000.);
#14693=VECTOR('',#102653,1000.);
#14694=VECTOR('',#102654,1000.);
#14695=VECTOR('',#102657,1000.);
#14696=VECTOR('',#102658,1000.);
#14697=VECTOR('',#102661,1000.);
#14698=VECTOR('',#102662,1000.);
#14699=VECTOR('',#102663,1000.);
#14700=VECTOR('',#102664,1000.);
#14701=VECTOR('',#102667,1000.);
#14702=VECTOR('',#102668,1000.);
#14703=VECTOR('',#102669,1000.);
#14704=VECTOR('',#102672,1000.);
#14705=VECTOR('',#102673,1000.);
#14706=VECTOR('',#102674,1000.);
#14707=VECTOR('',#102677,1000.);
#14708=VECTOR('',#102678,1000.);
#14709=VECTOR('',#102681,1000.);
#14710=VECTOR('',#102682,1000.);
#14711=VECTOR('',#102683,1000.);
#14712=VECTOR('',#102684,1000.);
#14713=VECTOR('',#102687,1000.);
#14714=VECTOR('',#102688,1000.);
#14715=VECTOR('',#102689,1000.);
#14716=VECTOR('',#102692,1000.);
#14717=VECTOR('',#102693,1000.);
#14718=VECTOR('',#102694,1000.);
#14719=VECTOR('',#102697,1000.);
#14720=VECTOR('',#102698,1000.);
#14721=VECTOR('',#102701,1000.);
#14722=VECTOR('',#102702,1000.);
#14723=VECTOR('',#102703,1000.);
#14724=VECTOR('',#102704,1000.);
#14725=VECTOR('',#102707,1000.);
#14726=VECTOR('',#102708,1000.);
#14727=VECTOR('',#102709,1000.);
#14728=VECTOR('',#102712,1000.);
#14729=VECTOR('',#102713,1000.);
#14730=VECTOR('',#102714,1000.);
#14731=VECTOR('',#102717,1000.);
#14732=VECTOR('',#102718,1000.);
#14733=VECTOR('',#102721,1000.);
#14734=VECTOR('',#102722,1000.);
#14735=VECTOR('',#102723,1000.);
#14736=VECTOR('',#102724,1000.);
#14737=VECTOR('',#102727,1000.);
#14738=VECTOR('',#102728,1000.);
#14739=VECTOR('',#102729,1000.);
#14740=VECTOR('',#102732,1000.);
#14741=VECTOR('',#102733,1000.);
#14742=VECTOR('',#102734,1000.);
#14743=VECTOR('',#102737,1000.);
#14744=VECTOR('',#102738,1000.);
#14745=VECTOR('',#102741,1000.);
#14746=VECTOR('',#102742,1000.);
#14747=VECTOR('',#102743,1000.);
#14748=VECTOR('',#102744,1000.);
#14749=VECTOR('',#102747,1000.);
#14750=VECTOR('',#102748,1000.);
#14751=VECTOR('',#102749,1000.);
#14752=VECTOR('',#102752,1000.);
#14753=VECTOR('',#102753,1000.);
#14754=VECTOR('',#102754,1000.);
#14755=VECTOR('',#102757,1000.);
#14756=VECTOR('',#102758,1000.);
#14757=VECTOR('',#102761,1000.);
#14758=VECTOR('',#102762,1000.);
#14759=VECTOR('',#102763,1000.);
#14760=VECTOR('',#102764,1000.);
#14761=VECTOR('',#102767,1000.);
#14762=VECTOR('',#102768,1000.);
#14763=VECTOR('',#102769,1000.);
#14764=VECTOR('',#102772,1000.);
#14765=VECTOR('',#102773,1000.);
#14766=VECTOR('',#102774,1000.);
#14767=VECTOR('',#102777,1000.);
#14768=VECTOR('',#102778,1000.);
#14769=VECTOR('',#102781,1000.);
#14770=VECTOR('',#102782,1000.);
#14771=VECTOR('',#102783,1000.);
#14772=VECTOR('',#102784,1000.);
#14773=VECTOR('',#102787,1000.);
#14774=VECTOR('',#102788,1000.);
#14775=VECTOR('',#102789,1000.);
#14776=VECTOR('',#102792,1000.);
#14777=VECTOR('',#102793,1000.);
#14778=VECTOR('',#102794,1000.);
#14779=VECTOR('',#102797,1000.);
#14780=VECTOR('',#102798,1000.);
#14781=VECTOR('',#102801,1000.);
#14782=VECTOR('',#102802,1000.);
#14783=VECTOR('',#102803,1000.);
#14784=VECTOR('',#102804,1000.);
#14785=VECTOR('',#102807,1000.);
#14786=VECTOR('',#102808,1000.);
#14787=VECTOR('',#102809,1000.);
#14788=VECTOR('',#102812,1000.);
#14789=VECTOR('',#102813,1000.);
#14790=VECTOR('',#102814,1000.);
#14791=VECTOR('',#102817,1000.);
#14792=VECTOR('',#102818,1000.);
#14793=VECTOR('',#102821,1000.);
#14794=VECTOR('',#102822,1000.);
#14795=VECTOR('',#102823,1000.);
#14796=VECTOR('',#102824,1000.);
#14797=VECTOR('',#102827,1000.);
#14798=VECTOR('',#102828,1000.);
#14799=VECTOR('',#102829,1000.);
#14800=VECTOR('',#102832,1000.);
#14801=VECTOR('',#102833,1000.);
#14802=VECTOR('',#102834,1000.);
#14803=VECTOR('',#102837,1000.);
#14804=VECTOR('',#102838,1000.);
#14805=VECTOR('',#102841,1000.);
#14806=VECTOR('',#102842,1000.);
#14807=VECTOR('',#102843,1000.);
#14808=VECTOR('',#102844,1000.);
#14809=VECTOR('',#102847,1000.);
#14810=VECTOR('',#102848,1000.);
#14811=VECTOR('',#102849,1000.);
#14812=VECTOR('',#102852,1000.);
#14813=VECTOR('',#102853,1000.);
#14814=VECTOR('',#102854,1000.);
#14815=VECTOR('',#102857,1000.);
#14816=VECTOR('',#102858,1000.);
#14817=VECTOR('',#102861,1000.);
#14818=VECTOR('',#102862,1000.);
#14819=VECTOR('',#102863,1000.);
#14820=VECTOR('',#102864,1000.);
#14821=VECTOR('',#102867,1000.);
#14822=VECTOR('',#102868,1000.);
#14823=VECTOR('',#102869,1000.);
#14824=VECTOR('',#102872,1000.);
#14825=VECTOR('',#102873,1000.);
#14826=VECTOR('',#102874,1000.);
#14827=VECTOR('',#102877,1000.);
#14828=VECTOR('',#102878,1000.);
#14829=VECTOR('',#102881,1000.);
#14830=VECTOR('',#102882,1000.);
#14831=VECTOR('',#102883,1000.);
#14832=VECTOR('',#102884,1000.);
#14833=VECTOR('',#102887,1000.);
#14834=VECTOR('',#102888,1000.);
#14835=VECTOR('',#102889,1000.);
#14836=VECTOR('',#102892,1000.);
#14837=VECTOR('',#102893,1000.);
#14838=VECTOR('',#102894,1000.);
#14839=VECTOR('',#102897,1000.);
#14840=VECTOR('',#102898,1000.);
#14841=VECTOR('',#102901,1000.);
#14842=VECTOR('',#102902,1000.);
#14843=VECTOR('',#102903,1000.);
#14844=VECTOR('',#102904,1000.);
#14845=VECTOR('',#102907,1000.);
#14846=VECTOR('',#102908,1000.);
#14847=VECTOR('',#102909,1000.);
#14848=VECTOR('',#102912,1000.);
#14849=VECTOR('',#102913,1000.);
#14850=VECTOR('',#102914,1000.);
#14851=VECTOR('',#102917,1000.);
#14852=VECTOR('',#102918,1000.);
#14853=VECTOR('',#102921,1000.);
#14854=VECTOR('',#102922,1000.);
#14855=VECTOR('',#102923,1000.);
#14856=VECTOR('',#102924,1000.);
#14857=VECTOR('',#102927,1000.);
#14858=VECTOR('',#102928,1000.);
#14859=VECTOR('',#102929,1000.);
#14860=VECTOR('',#102932,1000.);
#14861=VECTOR('',#102933,1000.);
#14862=VECTOR('',#102934,1000.);
#14863=VECTOR('',#102937,1000.);
#14864=VECTOR('',#102938,1000.);
#14865=VECTOR('',#102941,1000.);
#14866=VECTOR('',#102942,1000.);
#14867=VECTOR('',#102943,1000.);
#14868=VECTOR('',#102944,1000.);
#14869=VECTOR('',#102947,1000.);
#14870=VECTOR('',#102948,1000.);
#14871=VECTOR('',#102949,1000.);
#14872=VECTOR('',#102952,1000.);
#14873=VECTOR('',#102953,1000.);
#14874=VECTOR('',#102954,1000.);
#14875=VECTOR('',#102957,1000.);
#14876=VECTOR('',#102958,1000.);
#14877=VECTOR('',#102961,1000.);
#14878=VECTOR('',#102962,1000.);
#14879=VECTOR('',#102963,1000.);
#14880=VECTOR('',#102964,1000.);
#14881=VECTOR('',#102967,1000.);
#14882=VECTOR('',#102968,1000.);
#14883=VECTOR('',#102969,1000.);
#14884=VECTOR('',#102972,1000.);
#14885=VECTOR('',#102973,1000.);
#14886=VECTOR('',#102974,1000.);
#14887=VECTOR('',#102977,1000.);
#14888=VECTOR('',#102978,1000.);
#14889=VECTOR('',#102981,1000.);
#14890=VECTOR('',#102982,1000.);
#14891=VECTOR('',#102983,1000.);
#14892=VECTOR('',#102984,1000.);
#14893=VECTOR('',#102987,1000.);
#14894=VECTOR('',#102988,1000.);
#14895=VECTOR('',#102989,1000.);
#14896=VECTOR('',#102992,1000.);
#14897=VECTOR('',#102993,1000.);
#14898=VECTOR('',#102994,1000.);
#14899=VECTOR('',#102997,1000.);
#14900=VECTOR('',#102998,1000.);
#14901=VECTOR('',#103001,1000.);
#14902=VECTOR('',#103002,1000.);
#14903=VECTOR('',#103003,1000.);
#14904=VECTOR('',#103004,1000.);
#14905=VECTOR('',#103007,1000.);
#14906=VECTOR('',#103008,1000.);
#14907=VECTOR('',#103009,1000.);
#14908=VECTOR('',#103012,1000.);
#14909=VECTOR('',#103013,1000.);
#14910=VECTOR('',#103014,1000.);
#14911=VECTOR('',#103017,1000.);
#14912=VECTOR('',#103018,1000.);
#14913=VECTOR('',#103021,1000.);
#14914=VECTOR('',#103022,1000.);
#14915=VECTOR('',#103023,1000.);
#14916=VECTOR('',#103024,1000.);
#14917=VECTOR('',#103027,1000.);
#14918=VECTOR('',#103028,1000.);
#14919=VECTOR('',#103029,1000.);
#14920=VECTOR('',#103032,1000.);
#14921=VECTOR('',#103033,1000.);
#14922=VECTOR('',#103034,1000.);
#14923=VECTOR('',#103037,1000.);
#14924=VECTOR('',#103038,1000.);
#14925=VECTOR('',#103041,1000.);
#14926=VECTOR('',#103042,1000.);
#14927=VECTOR('',#103043,1000.);
#14928=VECTOR('',#103044,1000.);
#14929=VECTOR('',#103047,1000.);
#14930=VECTOR('',#103048,1000.);
#14931=VECTOR('',#103049,1000.);
#14932=VECTOR('',#103052,1000.);
#14933=VECTOR('',#103053,1000.);
#14934=VECTOR('',#103054,1000.);
#14935=VECTOR('',#103057,1000.);
#14936=VECTOR('',#103058,1000.);
#14937=VECTOR('',#103061,1000.);
#14938=VECTOR('',#103062,1000.);
#14939=VECTOR('',#103063,1000.);
#14940=VECTOR('',#103064,1000.);
#14941=VECTOR('',#103067,1000.);
#14942=VECTOR('',#103068,1000.);
#14943=VECTOR('',#103069,1000.);
#14944=VECTOR('',#103072,1000.);
#14945=VECTOR('',#103073,1000.);
#14946=VECTOR('',#103074,1000.);
#14947=VECTOR('',#103077,1000.);
#14948=VECTOR('',#103078,1000.);
#14949=VECTOR('',#103081,1000.);
#14950=VECTOR('',#103082,1000.);
#14951=VECTOR('',#103083,1000.);
#14952=VECTOR('',#103084,1000.);
#14953=VECTOR('',#103087,1000.);
#14954=VECTOR('',#103088,1000.);
#14955=VECTOR('',#103089,1000.);
#14956=VECTOR('',#103092,1000.);
#14957=VECTOR('',#103093,1000.);
#14958=VECTOR('',#103094,1000.);
#14959=VECTOR('',#103097,1000.);
#14960=VECTOR('',#103098,1000.);
#14961=VECTOR('',#103101,1000.);
#14962=VECTOR('',#103102,1000.);
#14963=VECTOR('',#103103,1000.);
#14964=VECTOR('',#103104,1000.);
#14965=VECTOR('',#103107,1000.);
#14966=VECTOR('',#103108,1000.);
#14967=VECTOR('',#103109,1000.);
#14968=VECTOR('',#103112,1000.);
#14969=VECTOR('',#103113,1000.);
#14970=VECTOR('',#103114,1000.);
#14971=VECTOR('',#103117,1000.);
#14972=VECTOR('',#103118,1000.);
#14973=VECTOR('',#103121,1000.);
#14974=VECTOR('',#103122,1000.);
#14975=VECTOR('',#103123,1000.);
#14976=VECTOR('',#103124,1000.);
#14977=VECTOR('',#103127,1000.);
#14978=VECTOR('',#103128,1000.);
#14979=VECTOR('',#103129,1000.);
#14980=VECTOR('',#103132,1000.);
#14981=VECTOR('',#103133,1000.);
#14982=VECTOR('',#103134,1000.);
#14983=VECTOR('',#103137,1000.);
#14984=VECTOR('',#103138,1000.);
#14985=VECTOR('',#103141,1000.);
#14986=VECTOR('',#103142,1000.);
#14987=VECTOR('',#103143,1000.);
#14988=VECTOR('',#103144,1000.);
#14989=VECTOR('',#103147,1000.);
#14990=VECTOR('',#103148,1000.);
#14991=VECTOR('',#103149,1000.);
#14992=VECTOR('',#103152,1000.);
#14993=VECTOR('',#103153,1000.);
#14994=VECTOR('',#103154,1000.);
#14995=VECTOR('',#103157,1000.);
#14996=VECTOR('',#103158,1000.);
#14997=VECTOR('',#103161,1000.);
#14998=VECTOR('',#103162,1000.);
#14999=VECTOR('',#103163,1000.);
#15000=VECTOR('',#103164,1000.);
#15001=VECTOR('',#103167,1000.);
#15002=VECTOR('',#103168,1000.);
#15003=VECTOR('',#103169,1000.);
#15004=VECTOR('',#103172,1000.);
#15005=VECTOR('',#103173,1000.);
#15006=VECTOR('',#103174,1000.);
#15007=VECTOR('',#103177,1000.);
#15008=VECTOR('',#103178,1000.);
#15009=VECTOR('',#103181,1000.);
#15010=VECTOR('',#103182,1000.);
#15011=VECTOR('',#103183,1000.);
#15012=VECTOR('',#103184,1000.);
#15013=VECTOR('',#103187,1000.);
#15014=VECTOR('',#103188,1000.);
#15015=VECTOR('',#103189,1000.);
#15016=VECTOR('',#103192,1000.);
#15017=VECTOR('',#103193,1000.);
#15018=VECTOR('',#103194,1000.);
#15019=VECTOR('',#103197,1000.);
#15020=VECTOR('',#103198,1000.);
#15021=VECTOR('',#103201,1000.);
#15022=VECTOR('',#103202,1000.);
#15023=VECTOR('',#103203,1000.);
#15024=VECTOR('',#103204,1000.);
#15025=VECTOR('',#103207,1000.);
#15026=VECTOR('',#103208,1000.);
#15027=VECTOR('',#103209,1000.);
#15028=VECTOR('',#103212,1000.);
#15029=VECTOR('',#103213,1000.);
#15030=VECTOR('',#103214,1000.);
#15031=VECTOR('',#103217,1000.);
#15032=VECTOR('',#103218,1000.);
#15033=VECTOR('',#103221,1000.);
#15034=VECTOR('',#103222,1000.);
#15035=VECTOR('',#103223,1000.);
#15036=VECTOR('',#103224,1000.);
#15037=VECTOR('',#103227,1000.);
#15038=VECTOR('',#103228,1000.);
#15039=VECTOR('',#103229,1000.);
#15040=VECTOR('',#103232,1000.);
#15041=VECTOR('',#103233,1000.);
#15042=VECTOR('',#103234,1000.);
#15043=VECTOR('',#103237,1000.);
#15044=VECTOR('',#103238,1000.);
#15045=VECTOR('',#103241,1000.);
#15046=VECTOR('',#103242,1000.);
#15047=VECTOR('',#103243,1000.);
#15048=VECTOR('',#103244,1000.);
#15049=VECTOR('',#103247,1000.);
#15050=VECTOR('',#103248,1000.);
#15051=VECTOR('',#103249,1000.);
#15052=VECTOR('',#103252,1000.);
#15053=VECTOR('',#103253,1000.);
#15054=VECTOR('',#103254,1000.);
#15055=VECTOR('',#103257,1000.);
#15056=VECTOR('',#103258,1000.);
#15057=VECTOR('',#103261,1000.);
#15058=VECTOR('',#103262,1000.);
#15059=VECTOR('',#103263,1000.);
#15060=VECTOR('',#103264,1000.);
#15061=VECTOR('',#103267,1000.);
#15062=VECTOR('',#103268,1000.);
#15063=VECTOR('',#103269,1000.);
#15064=VECTOR('',#103272,1000.);
#15065=VECTOR('',#103273,1000.);
#15066=VECTOR('',#103274,1000.);
#15067=VECTOR('',#103277,1000.);
#15068=VECTOR('',#103278,1000.);
#15069=VECTOR('',#103281,1000.);
#15070=VECTOR('',#103282,1000.);
#15071=VECTOR('',#103283,1000.);
#15072=VECTOR('',#103284,1000.);
#15073=VECTOR('',#103287,1000.);
#15074=VECTOR('',#103288,1000.);
#15075=VECTOR('',#103289,1000.);
#15076=VECTOR('',#103292,1000.);
#15077=VECTOR('',#103293,1000.);
#15078=VECTOR('',#103294,1000.);
#15079=VECTOR('',#103297,1000.);
#15080=VECTOR('',#103298,1000.);
#15081=VECTOR('',#103301,1000.);
#15082=VECTOR('',#103302,1000.);
#15083=VECTOR('',#103303,1000.);
#15084=VECTOR('',#103304,1000.);
#15085=VECTOR('',#103307,1000.);
#15086=VECTOR('',#103308,1000.);
#15087=VECTOR('',#103309,1000.);
#15088=VECTOR('',#103312,1000.);
#15089=VECTOR('',#103313,1000.);
#15090=VECTOR('',#103314,1000.);
#15091=VECTOR('',#103317,1000.);
#15092=VECTOR('',#103318,1000.);
#15093=VECTOR('',#103321,1000.);
#15094=VECTOR('',#103322,1000.);
#15095=VECTOR('',#103323,1000.);
#15096=VECTOR('',#103324,1000.);
#15097=VECTOR('',#103327,1000.);
#15098=VECTOR('',#103328,1000.);
#15099=VECTOR('',#103329,1000.);
#15100=VECTOR('',#103332,1000.);
#15101=VECTOR('',#103333,1000.);
#15102=VECTOR('',#103334,1000.);
#15103=VECTOR('',#103337,1000.);
#15104=VECTOR('',#103338,1000.);
#15105=VECTOR('',#103341,1000.);
#15106=VECTOR('',#103342,1000.);
#15107=VECTOR('',#103343,1000.);
#15108=VECTOR('',#103344,1000.);
#15109=VECTOR('',#103347,1000.);
#15110=VECTOR('',#103348,1000.);
#15111=VECTOR('',#103349,1000.);
#15112=VECTOR('',#103352,1000.);
#15113=VECTOR('',#103353,1000.);
#15114=VECTOR('',#103354,1000.);
#15115=VECTOR('',#103357,1000.);
#15116=VECTOR('',#103358,1000.);
#15117=VECTOR('',#103361,1000.);
#15118=VECTOR('',#103362,1000.);
#15119=VECTOR('',#103363,1000.);
#15120=VECTOR('',#103364,1000.);
#15121=VECTOR('',#103367,1000.);
#15122=VECTOR('',#103368,1000.);
#15123=VECTOR('',#103369,1000.);
#15124=VECTOR('',#103372,1000.);
#15125=VECTOR('',#103373,1000.);
#15126=VECTOR('',#103374,1000.);
#15127=VECTOR('',#103377,1000.);
#15128=VECTOR('',#103378,1000.);
#15129=VECTOR('',#103381,1000.);
#15130=VECTOR('',#103382,1000.);
#15131=VECTOR('',#103383,1000.);
#15132=VECTOR('',#103384,1000.);
#15133=VECTOR('',#103387,1000.);
#15134=VECTOR('',#103388,1000.);
#15135=VECTOR('',#103389,1000.);
#15136=VECTOR('',#103392,1000.);
#15137=VECTOR('',#103393,1000.);
#15138=VECTOR('',#103394,1000.);
#15139=VECTOR('',#103397,1000.);
#15140=VECTOR('',#103398,1000.);
#15141=VECTOR('',#103401,1000.);
#15142=VECTOR('',#103402,1000.);
#15143=VECTOR('',#103403,1000.);
#15144=VECTOR('',#103404,1000.);
#15145=VECTOR('',#103407,1000.);
#15146=VECTOR('',#103408,1000.);
#15147=VECTOR('',#103409,1000.);
#15148=VECTOR('',#103412,1000.);
#15149=VECTOR('',#103413,1000.);
#15150=VECTOR('',#103414,1000.);
#15151=VECTOR('',#103417,1000.);
#15152=VECTOR('',#103418,1000.);
#15153=VECTOR('',#103421,1000.);
#15154=VECTOR('',#103422,1000.);
#15155=VECTOR('',#103423,1000.);
#15156=VECTOR('',#103424,1000.);
#15157=VECTOR('',#103427,1000.);
#15158=VECTOR('',#103428,1000.);
#15159=VECTOR('',#103429,1000.);
#15160=VECTOR('',#103432,1000.);
#15161=VECTOR('',#103433,1000.);
#15162=VECTOR('',#103434,1000.);
#15163=VECTOR('',#103437,1000.);
#15164=VECTOR('',#103438,1000.);
#15165=VECTOR('',#103441,1000.);
#15166=VECTOR('',#103442,1000.);
#15167=VECTOR('',#103443,1000.);
#15168=VECTOR('',#103444,1000.);
#15169=VECTOR('',#103447,1000.);
#15170=VECTOR('',#103448,1000.);
#15171=VECTOR('',#103449,1000.);
#15172=VECTOR('',#103452,1000.);
#15173=VECTOR('',#103453,1000.);
#15174=VECTOR('',#103454,1000.);
#15175=VECTOR('',#103457,1000.);
#15176=VECTOR('',#103458,1000.);
#15177=VECTOR('',#103461,1000.);
#15178=VECTOR('',#103462,1000.);
#15179=VECTOR('',#103463,1000.);
#15180=VECTOR('',#103464,1000.);
#15181=VECTOR('',#103467,1000.);
#15182=VECTOR('',#103468,1000.);
#15183=VECTOR('',#103469,1000.);
#15184=VECTOR('',#103472,1000.);
#15185=VECTOR('',#103473,1000.);
#15186=VECTOR('',#103474,1000.);
#15187=VECTOR('',#103477,1000.);
#15188=VECTOR('',#103478,1000.);
#15189=VECTOR('',#103481,1000.);
#15190=VECTOR('',#103482,1000.);
#15191=VECTOR('',#103483,1000.);
#15192=VECTOR('',#103484,1000.);
#15193=VECTOR('',#103487,1000.);
#15194=VECTOR('',#103488,1000.);
#15195=VECTOR('',#103489,1000.);
#15196=VECTOR('',#103492,1000.);
#15197=VECTOR('',#103493,1000.);
#15198=VECTOR('',#103494,1000.);
#15199=VECTOR('',#103497,1000.);
#15200=VECTOR('',#103498,1000.);
#15201=VECTOR('',#103501,1000.);
#15202=VECTOR('',#103502,1000.);
#15203=VECTOR('',#103503,1000.);
#15204=VECTOR('',#103504,1000.);
#15205=VECTOR('',#103507,1000.);
#15206=VECTOR('',#103508,1000.);
#15207=VECTOR('',#103509,1000.);
#15208=VECTOR('',#103512,1000.);
#15209=VECTOR('',#103513,1000.);
#15210=VECTOR('',#103514,1000.);
#15211=VECTOR('',#103517,1000.);
#15212=VECTOR('',#103518,1000.);
#15213=VECTOR('',#103521,1000.);
#15214=VECTOR('',#103522,1000.);
#15215=VECTOR('',#103523,1000.);
#15216=VECTOR('',#103524,1000.);
#15217=VECTOR('',#103527,1000.);
#15218=VECTOR('',#103528,1000.);
#15219=VECTOR('',#103529,1000.);
#15220=VECTOR('',#103532,1000.);
#15221=VECTOR('',#103533,1000.);
#15222=VECTOR('',#103534,1000.);
#15223=VECTOR('',#103537,1000.);
#15224=VECTOR('',#103538,1000.);
#15225=VECTOR('',#103541,1000.);
#15226=VECTOR('',#103542,1000.);
#15227=VECTOR('',#103543,1000.);
#15228=VECTOR('',#103544,1000.);
#15229=VECTOR('',#103547,1000.);
#15230=VECTOR('',#103548,1000.);
#15231=VECTOR('',#103549,1000.);
#15232=VECTOR('',#103552,1000.);
#15233=VECTOR('',#103553,1000.);
#15234=VECTOR('',#103554,1000.);
#15235=VECTOR('',#103557,1000.);
#15236=VECTOR('',#103558,1000.);
#15237=VECTOR('',#103561,1000.);
#15238=VECTOR('',#103562,1000.);
#15239=VECTOR('',#103563,1000.);
#15240=VECTOR('',#103564,1000.);
#15241=VECTOR('',#103567,1000.);
#15242=VECTOR('',#103568,1000.);
#15243=VECTOR('',#103569,1000.);
#15244=VECTOR('',#103572,1000.);
#15245=VECTOR('',#103573,1000.);
#15246=VECTOR('',#103574,1000.);
#15247=VECTOR('',#103577,1000.);
#15248=VECTOR('',#103578,1000.);
#15249=VECTOR('',#103581,1000.);
#15250=VECTOR('',#103582,1000.);
#15251=VECTOR('',#103583,1000.);
#15252=VECTOR('',#103584,1000.);
#15253=VECTOR('',#103587,1000.);
#15254=VECTOR('',#103588,1000.);
#15255=VECTOR('',#103589,1000.);
#15256=VECTOR('',#103592,1000.);
#15257=VECTOR('',#103593,1000.);
#15258=VECTOR('',#103594,1000.);
#15259=VECTOR('',#103597,1000.);
#15260=VECTOR('',#103598,1000.);
#15261=VECTOR('',#103601,1000.);
#15262=VECTOR('',#103602,1000.);
#15263=VECTOR('',#103603,1000.);
#15264=VECTOR('',#103604,1000.);
#15265=VECTOR('',#103607,1000.);
#15266=VECTOR('',#103608,1000.);
#15267=VECTOR('',#103609,1000.);
#15268=VECTOR('',#103612,1000.);
#15269=VECTOR('',#103613,1000.);
#15270=VECTOR('',#103614,1000.);
#15271=VECTOR('',#103617,1000.);
#15272=VECTOR('',#103618,1000.);
#15273=VECTOR('',#103621,1000.);
#15274=VECTOR('',#103622,1000.);
#15275=VECTOR('',#103623,1000.);
#15276=VECTOR('',#103624,1000.);
#15277=VECTOR('',#103627,1000.);
#15278=VECTOR('',#103628,1000.);
#15279=VECTOR('',#103629,1000.);
#15280=VECTOR('',#103632,1000.);
#15281=VECTOR('',#103633,1000.);
#15282=VECTOR('',#103634,1000.);
#15283=VECTOR('',#103637,1000.);
#15284=VECTOR('',#103638,1000.);
#15285=VECTOR('',#103641,1000.);
#15286=VECTOR('',#103642,1000.);
#15287=VECTOR('',#103643,1000.);
#15288=VECTOR('',#103644,1000.);
#15289=VECTOR('',#103647,1000.);
#15290=VECTOR('',#103648,1000.);
#15291=VECTOR('',#103649,1000.);
#15292=VECTOR('',#103652,1000.);
#15293=VECTOR('',#103653,1000.);
#15294=VECTOR('',#103654,1000.);
#15295=VECTOR('',#103657,1000.);
#15296=VECTOR('',#103658,1000.);
#15297=VECTOR('',#103661,1000.);
#15298=VECTOR('',#103662,1000.);
#15299=VECTOR('',#103663,1000.);
#15300=VECTOR('',#103664,1000.);
#15301=VECTOR('',#103667,1000.);
#15302=VECTOR('',#103668,1000.);
#15303=VECTOR('',#103669,1000.);
#15304=VECTOR('',#103672,1000.);
#15305=VECTOR('',#103673,1000.);
#15306=VECTOR('',#103674,1000.);
#15307=VECTOR('',#103677,1000.);
#15308=VECTOR('',#103678,1000.);
#15309=VECTOR('',#103681,1000.);
#15310=VECTOR('',#103682,1000.);
#15311=VECTOR('',#103683,1000.);
#15312=VECTOR('',#103684,1000.);
#15313=VECTOR('',#103687,1000.);
#15314=VECTOR('',#103688,1000.);
#15315=VECTOR('',#103689,1000.);
#15316=VECTOR('',#103692,1000.);
#15317=VECTOR('',#103693,1000.);
#15318=VECTOR('',#103694,1000.);
#15319=VECTOR('',#103697,1000.);
#15320=VECTOR('',#103698,1000.);
#15321=VECTOR('',#103701,1000.);
#15322=VECTOR('',#103702,1000.);
#15323=VECTOR('',#103703,1000.);
#15324=VECTOR('',#103704,1000.);
#15325=VECTOR('',#103707,1000.);
#15326=VECTOR('',#103708,1000.);
#15327=VECTOR('',#103709,1000.);
#15328=VECTOR('',#103712,1000.);
#15329=VECTOR('',#103713,1000.);
#15330=VECTOR('',#103714,1000.);
#15331=VECTOR('',#103717,1000.);
#15332=VECTOR('',#103718,1000.);
#15333=VECTOR('',#103721,1000.);
#15334=VECTOR('',#103722,1000.);
#15335=VECTOR('',#103723,1000.);
#15336=VECTOR('',#103724,1000.);
#15337=VECTOR('',#103727,1000.);
#15338=VECTOR('',#103728,1000.);
#15339=VECTOR('',#103729,1000.);
#15340=VECTOR('',#103732,1000.);
#15341=VECTOR('',#103733,1000.);
#15342=VECTOR('',#103734,1000.);
#15343=VECTOR('',#103737,1000.);
#15344=VECTOR('',#103738,1000.);
#15345=VECTOR('',#103741,1000.);
#15346=VECTOR('',#103742,1000.);
#15347=VECTOR('',#103743,1000.);
#15348=VECTOR('',#103744,1000.);
#15349=VECTOR('',#103747,1000.);
#15350=VECTOR('',#103748,1000.);
#15351=VECTOR('',#103749,1000.);
#15352=VECTOR('',#103752,1000.);
#15353=VECTOR('',#103753,1000.);
#15354=VECTOR('',#103754,1000.);
#15355=VECTOR('',#103757,1000.);
#15356=VECTOR('',#103758,1000.);
#15357=VECTOR('',#103761,1000.);
#15358=VECTOR('',#103762,1000.);
#15359=VECTOR('',#103763,1000.);
#15360=VECTOR('',#103764,1000.);
#15361=VECTOR('',#103767,1000.);
#15362=VECTOR('',#103768,1000.);
#15363=VECTOR('',#103769,1000.);
#15364=VECTOR('',#103772,1000.);
#15365=VECTOR('',#103773,1000.);
#15366=VECTOR('',#103774,1000.);
#15367=VECTOR('',#103777,1000.);
#15368=VECTOR('',#103778,1000.);
#15369=VECTOR('',#103781,1000.);
#15370=VECTOR('',#103782,1000.);
#15371=VECTOR('',#103783,1000.);
#15372=VECTOR('',#103784,1000.);
#15373=VECTOR('',#103787,1000.);
#15374=VECTOR('',#103788,1000.);
#15375=VECTOR('',#103789,1000.);
#15376=VECTOR('',#103792,1000.);
#15377=VECTOR('',#103793,1000.);
#15378=VECTOR('',#103794,1000.);
#15379=VECTOR('',#103797,1000.);
#15380=VECTOR('',#103798,1000.);
#15381=VECTOR('',#103801,1000.);
#15382=VECTOR('',#103802,1000.);
#15383=VECTOR('',#103803,1000.);
#15384=VECTOR('',#103804,1000.);
#15385=VECTOR('',#103807,1000.);
#15386=VECTOR('',#103808,1000.);
#15387=VECTOR('',#103809,1000.);
#15388=VECTOR('',#103812,1000.);
#15389=VECTOR('',#103813,1000.);
#15390=VECTOR('',#103814,1000.);
#15391=VECTOR('',#103817,1000.);
#15392=VECTOR('',#103818,1000.);
#15393=VECTOR('',#103821,1000.);
#15394=VECTOR('',#103822,1000.);
#15395=VECTOR('',#103823,1000.);
#15396=VECTOR('',#103824,1000.);
#15397=VECTOR('',#103827,1000.);
#15398=VECTOR('',#103828,1000.);
#15399=VECTOR('',#103829,1000.);
#15400=VECTOR('',#103832,1000.);
#15401=VECTOR('',#103833,1000.);
#15402=VECTOR('',#103834,1000.);
#15403=VECTOR('',#103837,1000.);
#15404=VECTOR('',#103838,1000.);
#15405=VECTOR('',#103841,1000.);
#15406=VECTOR('',#103842,1000.);
#15407=VECTOR('',#103843,1000.);
#15408=VECTOR('',#103844,1000.);
#15409=VECTOR('',#103847,1000.);
#15410=VECTOR('',#103848,1000.);
#15411=VECTOR('',#103849,1000.);
#15412=VECTOR('',#103852,1000.);
#15413=VECTOR('',#103853,1000.);
#15414=VECTOR('',#103854,1000.);
#15415=VECTOR('',#103857,1000.);
#15416=VECTOR('',#103858,1000.);
#15417=VECTOR('',#103861,1000.);
#15418=VECTOR('',#103862,1000.);
#15419=VECTOR('',#103863,1000.);
#15420=VECTOR('',#103864,1000.);
#15421=VECTOR('',#103867,1000.);
#15422=VECTOR('',#103868,1000.);
#15423=VECTOR('',#103869,1000.);
#15424=VECTOR('',#103872,1000.);
#15425=VECTOR('',#103873,1000.);
#15426=VECTOR('',#103874,1000.);
#15427=VECTOR('',#103877,1000.);
#15428=VECTOR('',#103878,1000.);
#15429=VECTOR('',#103881,1000.);
#15430=VECTOR('',#103882,1000.);
#15431=VECTOR('',#103883,1000.);
#15432=VECTOR('',#103884,1000.);
#15433=VECTOR('',#103887,1000.);
#15434=VECTOR('',#103888,1000.);
#15435=VECTOR('',#103889,1000.);
#15436=VECTOR('',#103892,1000.);
#15437=VECTOR('',#103893,1000.);
#15438=VECTOR('',#103894,1000.);
#15439=VECTOR('',#103897,1000.);
#15440=VECTOR('',#103898,1000.);
#15441=VECTOR('',#103901,1000.);
#15442=VECTOR('',#103902,1000.);
#15443=VECTOR('',#103903,1000.);
#15444=VECTOR('',#103904,1000.);
#15445=VECTOR('',#103907,1000.);
#15446=VECTOR('',#103908,1000.);
#15447=VECTOR('',#103909,1000.);
#15448=VECTOR('',#103912,1000.);
#15449=VECTOR('',#103913,1000.);
#15450=VECTOR('',#103914,1000.);
#15451=VECTOR('',#103917,1000.);
#15452=VECTOR('',#103918,1000.);
#15453=VECTOR('',#103921,1000.);
#15454=VECTOR('',#103922,1000.);
#15455=VECTOR('',#103923,1000.);
#15456=VECTOR('',#103924,1000.);
#15457=VECTOR('',#103927,1000.);
#15458=VECTOR('',#103928,1000.);
#15459=VECTOR('',#103929,1000.);
#15460=VECTOR('',#103932,1000.);
#15461=VECTOR('',#103933,1000.);
#15462=VECTOR('',#103934,1000.);
#15463=VECTOR('',#103937,1000.);
#15464=VECTOR('',#103938,1000.);
#15465=VECTOR('',#103941,1000.);
#15466=VECTOR('',#103942,1000.);
#15467=VECTOR('',#103943,1000.);
#15468=VECTOR('',#103944,1000.);
#15469=VECTOR('',#103947,1000.);
#15470=VECTOR('',#103948,1000.);
#15471=VECTOR('',#103949,1000.);
#15472=VECTOR('',#103952,1000.);
#15473=VECTOR('',#103953,1000.);
#15474=VECTOR('',#103954,1000.);
#15475=VECTOR('',#103957,1000.);
#15476=VECTOR('',#103958,1000.);
#15477=VECTOR('',#103961,1000.);
#15478=VECTOR('',#103962,1000.);
#15479=VECTOR('',#103963,1000.);
#15480=VECTOR('',#103964,1000.);
#15481=VECTOR('',#103967,1000.);
#15482=VECTOR('',#103968,1000.);
#15483=VECTOR('',#103969,1000.);
#15484=VECTOR('',#103972,1000.);
#15485=VECTOR('',#103973,1000.);
#15486=VECTOR('',#103974,1000.);
#15487=VECTOR('',#103977,1000.);
#15488=VECTOR('',#103978,1000.);
#15489=VECTOR('',#103981,1000.);
#15490=VECTOR('',#103982,1000.);
#15491=VECTOR('',#103983,1000.);
#15492=VECTOR('',#103984,1000.);
#15493=VECTOR('',#103987,1000.);
#15494=VECTOR('',#103988,1000.);
#15495=VECTOR('',#103989,1000.);
#15496=VECTOR('',#103992,1000.);
#15497=VECTOR('',#103993,1000.);
#15498=VECTOR('',#103994,1000.);
#15499=VECTOR('',#103997,1000.);
#15500=VECTOR('',#103998,1000.);
#15501=VECTOR('',#104001,1000.);
#15502=VECTOR('',#104002,1000.);
#15503=VECTOR('',#104003,1000.);
#15504=VECTOR('',#104004,1000.);
#15505=VECTOR('',#104007,1000.);
#15506=VECTOR('',#104008,1000.);
#15507=VECTOR('',#104009,1000.);
#15508=VECTOR('',#104012,1000.);
#15509=VECTOR('',#104013,1000.);
#15510=VECTOR('',#104014,1000.);
#15511=VECTOR('',#104017,1000.);
#15512=VECTOR('',#104018,1000.);
#15513=VECTOR('',#104021,1000.);
#15514=VECTOR('',#104022,1000.);
#15515=VECTOR('',#104023,1000.);
#15516=VECTOR('',#104024,1000.);
#15517=VECTOR('',#104027,1000.);
#15518=VECTOR('',#104028,1000.);
#15519=VECTOR('',#104029,1000.);
#15520=VECTOR('',#104032,1000.);
#15521=VECTOR('',#104033,1000.);
#15522=VECTOR('',#104034,1000.);
#15523=VECTOR('',#104037,1000.);
#15524=VECTOR('',#104038,1000.);
#15525=VECTOR('',#104041,1000.);
#15526=VECTOR('',#104042,1000.);
#15527=VECTOR('',#104043,1000.);
#15528=VECTOR('',#104044,1000.);
#15529=VECTOR('',#104047,1000.);
#15530=VECTOR('',#104048,1000.);
#15531=VECTOR('',#104049,1000.);
#15532=VECTOR('',#104052,1000.);
#15533=VECTOR('',#104053,1000.);
#15534=VECTOR('',#104054,1000.);
#15535=VECTOR('',#104057,1000.);
#15536=VECTOR('',#104058,1000.);
#15537=VECTOR('',#104061,1000.);
#15538=VECTOR('',#104062,1000.);
#15539=VECTOR('',#104063,1000.);
#15540=VECTOR('',#104064,1000.);
#15541=VECTOR('',#104067,1000.);
#15542=VECTOR('',#104068,1000.);
#15543=VECTOR('',#104069,1000.);
#15544=VECTOR('',#104072,1000.);
#15545=VECTOR('',#104073,1000.);
#15546=VECTOR('',#104074,1000.);
#15547=VECTOR('',#104077,1000.);
#15548=VECTOR('',#104078,1000.);
#15549=VECTOR('',#104081,1000.);
#15550=VECTOR('',#104082,1000.);
#15551=VECTOR('',#104083,1000.);
#15552=VECTOR('',#104084,1000.);
#15553=VECTOR('',#104087,1000.);
#15554=VECTOR('',#104088,1000.);
#15555=VECTOR('',#104089,1000.);
#15556=VECTOR('',#104092,1000.);
#15557=VECTOR('',#104093,1000.);
#15558=VECTOR('',#104094,1000.);
#15559=VECTOR('',#104097,1000.);
#15560=VECTOR('',#104098,1000.);
#15561=VECTOR('',#104101,1000.);
#15562=VECTOR('',#104102,1000.);
#15563=VECTOR('',#104103,1000.);
#15564=VECTOR('',#104104,1000.);
#15565=VECTOR('',#104107,1000.);
#15566=VECTOR('',#104108,1000.);
#15567=VECTOR('',#104109,1000.);
#15568=VECTOR('',#104112,1000.);
#15569=VECTOR('',#104113,1000.);
#15570=VECTOR('',#104114,1000.);
#15571=VECTOR('',#104117,1000.);
#15572=VECTOR('',#104118,1000.);
#15573=VECTOR('',#104121,1000.);
#15574=VECTOR('',#104122,1000.);
#15575=VECTOR('',#104123,1000.);
#15576=VECTOR('',#104124,1000.);
#15577=VECTOR('',#104127,1000.);
#15578=VECTOR('',#104128,1000.);
#15579=VECTOR('',#104129,1000.);
#15580=VECTOR('',#104132,1000.);
#15581=VECTOR('',#104133,1000.);
#15582=VECTOR('',#104134,1000.);
#15583=VECTOR('',#104137,1000.);
#15584=VECTOR('',#104138,1000.);
#15585=VECTOR('',#104141,1000.);
#15586=VECTOR('',#104142,1000.);
#15587=VECTOR('',#104143,1000.);
#15588=VECTOR('',#104144,1000.);
#15589=VECTOR('',#104147,1000.);
#15590=VECTOR('',#104148,1000.);
#15591=VECTOR('',#104149,1000.);
#15592=VECTOR('',#104152,1000.);
#15593=VECTOR('',#104153,1000.);
#15594=VECTOR('',#104154,1000.);
#15595=VECTOR('',#104157,1000.);
#15596=VECTOR('',#104158,1000.);
#15597=VECTOR('',#104161,1000.);
#15598=VECTOR('',#104162,1000.);
#15599=VECTOR('',#104163,1000.);
#15600=VECTOR('',#104164,1000.);
#15601=VECTOR('',#104167,1000.);
#15602=VECTOR('',#104168,1000.);
#15603=VECTOR('',#104169,1000.);
#15604=VECTOR('',#104172,1000.);
#15605=VECTOR('',#104173,1000.);
#15606=VECTOR('',#104174,1000.);
#15607=VECTOR('',#104177,1000.);
#15608=VECTOR('',#104178,1000.);
#15609=VECTOR('',#104181,1000.);
#15610=VECTOR('',#104182,1000.);
#15611=VECTOR('',#104183,1000.);
#15612=VECTOR('',#104184,1000.);
#15613=VECTOR('',#104187,1000.);
#15614=VECTOR('',#104188,1000.);
#15615=VECTOR('',#104189,1000.);
#15616=VECTOR('',#104192,1000.);
#15617=VECTOR('',#104193,1000.);
#15618=VECTOR('',#104194,1000.);
#15619=VECTOR('',#104197,1000.);
#15620=VECTOR('',#104198,1000.);
#15621=VECTOR('',#104201,1000.);
#15622=VECTOR('',#104202,1000.);
#15623=VECTOR('',#104203,1000.);
#15624=VECTOR('',#104204,1000.);
#15625=VECTOR('',#104207,1000.);
#15626=VECTOR('',#104208,1000.);
#15627=VECTOR('',#104209,1000.);
#15628=VECTOR('',#104212,1000.);
#15629=VECTOR('',#104213,1000.);
#15630=VECTOR('',#104214,1000.);
#15631=VECTOR('',#104217,1000.);
#15632=VECTOR('',#104218,1000.);
#15633=VECTOR('',#104221,1000.);
#15634=VECTOR('',#104222,1000.);
#15635=VECTOR('',#104223,1000.);
#15636=VECTOR('',#104224,1000.);
#15637=VECTOR('',#104227,1000.);
#15638=VECTOR('',#104228,1000.);
#15639=VECTOR('',#104229,1000.);
#15640=VECTOR('',#104232,1000.);
#15641=VECTOR('',#104233,1000.);
#15642=VECTOR('',#104234,1000.);
#15643=VECTOR('',#104237,1000.);
#15644=VECTOR('',#104238,1000.);
#15645=VECTOR('',#104241,1000.);
#15646=VECTOR('',#104242,1000.);
#15647=VECTOR('',#104243,1000.);
#15648=VECTOR('',#104244,1000.);
#15649=VECTOR('',#104247,1000.);
#15650=VECTOR('',#104248,1000.);
#15651=VECTOR('',#104249,1000.);
#15652=VECTOR('',#104252,1000.);
#15653=VECTOR('',#104253,1000.);
#15654=VECTOR('',#104254,1000.);
#15655=VECTOR('',#104257,1000.);
#15656=VECTOR('',#104258,1000.);
#15657=VECTOR('',#104261,1000.);
#15658=VECTOR('',#104262,1000.);
#15659=VECTOR('',#104263,1000.);
#15660=VECTOR('',#104264,1000.);
#15661=VECTOR('',#104267,1000.);
#15662=VECTOR('',#104268,1000.);
#15663=VECTOR('',#104269,1000.);
#15664=VECTOR('',#104272,1000.);
#15665=VECTOR('',#104273,1000.);
#15666=VECTOR('',#104274,1000.);
#15667=VECTOR('',#104277,1000.);
#15668=VECTOR('',#104278,1000.);
#15669=VECTOR('',#104281,1000.);
#15670=VECTOR('',#104282,1000.);
#15671=VECTOR('',#104283,1000.);
#15672=VECTOR('',#104284,1000.);
#15673=VECTOR('',#104287,1000.);
#15674=VECTOR('',#104288,1000.);
#15675=VECTOR('',#104289,1000.);
#15676=VECTOR('',#104292,1000.);
#15677=VECTOR('',#104293,1000.);
#15678=VECTOR('',#104294,1000.);
#15679=VECTOR('',#104297,1000.);
#15680=VECTOR('',#104298,1000.);
#15681=VECTOR('',#104301,1000.);
#15682=VECTOR('',#104302,1000.);
#15683=VECTOR('',#104303,1000.);
#15684=VECTOR('',#104304,1000.);
#15685=VECTOR('',#104307,1000.);
#15686=VECTOR('',#104308,1000.);
#15687=VECTOR('',#104309,1000.);
#15688=VECTOR('',#104312,1000.);
#15689=VECTOR('',#104313,1000.);
#15690=VECTOR('',#104314,1000.);
#15691=VECTOR('',#104317,1000.);
#15692=VECTOR('',#104318,1000.);
#15693=VECTOR('',#104321,1000.);
#15694=VECTOR('',#104322,1000.);
#15695=VECTOR('',#104323,1000.);
#15696=VECTOR('',#104324,1000.);
#15697=VECTOR('',#104327,1000.);
#15698=VECTOR('',#104328,1000.);
#15699=VECTOR('',#104329,1000.);
#15700=VECTOR('',#104332,1000.);
#15701=VECTOR('',#104333,1000.);
#15702=VECTOR('',#104334,1000.);
#15703=VECTOR('',#104337,1000.);
#15704=VECTOR('',#104338,1000.);
#15705=VECTOR('',#104341,1000.);
#15706=VECTOR('',#104342,1000.);
#15707=VECTOR('',#104343,1000.);
#15708=VECTOR('',#104344,1000.);
#15709=VECTOR('',#104347,1000.);
#15710=VECTOR('',#104348,1000.);
#15711=VECTOR('',#104349,1000.);
#15712=VECTOR('',#104352,1000.);
#15713=VECTOR('',#104353,1000.);
#15714=VECTOR('',#104354,1000.);
#15715=VECTOR('',#104357,1000.);
#15716=VECTOR('',#104358,1000.);
#15717=VECTOR('',#104361,1000.);
#15718=VECTOR('',#104362,1000.);
#15719=VECTOR('',#104363,1000.);
#15720=VECTOR('',#104364,1000.);
#15721=VECTOR('',#104367,1000.);
#15722=VECTOR('',#104368,1000.);
#15723=VECTOR('',#104369,1000.);
#15724=VECTOR('',#104372,1000.);
#15725=VECTOR('',#104373,1000.);
#15726=VECTOR('',#104374,1000.);
#15727=VECTOR('',#104377,1000.);
#15728=VECTOR('',#104378,1000.);
#15729=VECTOR('',#104381,1000.);
#15730=VECTOR('',#104382,1000.);
#15731=VECTOR('',#104383,1000.);
#15732=VECTOR('',#104384,1000.);
#15733=VECTOR('',#104387,1000.);
#15734=VECTOR('',#104388,1000.);
#15735=VECTOR('',#104389,1000.);
#15736=VECTOR('',#104392,1000.);
#15737=VECTOR('',#104393,1000.);
#15738=VECTOR('',#104394,1000.);
#15739=VECTOR('',#104397,1000.);
#15740=VECTOR('',#104398,1000.);
#15741=VECTOR('',#104401,1000.);
#15742=VECTOR('',#104402,1000.);
#15743=VECTOR('',#104403,1000.);
#15744=VECTOR('',#104404,1000.);
#15745=VECTOR('',#104407,1000.);
#15746=VECTOR('',#104408,1000.);
#15747=VECTOR('',#104409,1000.);
#15748=VECTOR('',#104412,1000.);
#15749=VECTOR('',#104413,1000.);
#15750=VECTOR('',#104414,1000.);
#15751=VECTOR('',#104417,1000.);
#15752=VECTOR('',#104418,1000.);
#15753=VECTOR('',#104421,1000.);
#15754=VECTOR('',#104422,1000.);
#15755=VECTOR('',#104423,1000.);
#15756=VECTOR('',#104424,1000.);
#15757=VECTOR('',#104427,1000.);
#15758=VECTOR('',#104428,1000.);
#15759=VECTOR('',#104429,1000.);
#15760=VECTOR('',#104432,1000.);
#15761=VECTOR('',#104433,1000.);
#15762=VECTOR('',#104434,1000.);
#15763=VECTOR('',#104437,1000.);
#15764=VECTOR('',#104438,1000.);
#15765=VECTOR('',#104441,1000.);
#15766=VECTOR('',#104442,1000.);
#15767=VECTOR('',#104443,1000.);
#15768=VECTOR('',#104444,1000.);
#15769=VECTOR('',#104447,1000.);
#15770=VECTOR('',#104448,1000.);
#15771=VECTOR('',#104449,1000.);
#15772=VECTOR('',#104452,1000.);
#15773=VECTOR('',#104453,1000.);
#15774=VECTOR('',#104454,1000.);
#15775=VECTOR('',#104457,1000.);
#15776=VECTOR('',#104458,1000.);
#15777=VECTOR('',#104461,1000.);
#15778=VECTOR('',#104462,1000.);
#15779=VECTOR('',#104463,1000.);
#15780=VECTOR('',#104464,1000.);
#15781=VECTOR('',#104467,1000.);
#15782=VECTOR('',#104468,1000.);
#15783=VECTOR('',#104469,1000.);
#15784=VECTOR('',#104472,1000.);
#15785=VECTOR('',#104473,1000.);
#15786=VECTOR('',#104474,1000.);
#15787=VECTOR('',#104477,1000.);
#15788=VECTOR('',#104478,1000.);
#15789=VECTOR('',#104481,1000.);
#15790=VECTOR('',#104482,1000.);
#15791=VECTOR('',#104483,1000.);
#15792=VECTOR('',#104484,1000.);
#15793=VECTOR('',#104487,1000.);
#15794=VECTOR('',#104488,1000.);
#15795=VECTOR('',#104489,1000.);
#15796=VECTOR('',#104492,1000.);
#15797=VECTOR('',#104493,1000.);
#15798=VECTOR('',#104494,1000.);
#15799=VECTOR('',#104497,1000.);
#15800=VECTOR('',#104498,1000.);
#15801=VECTOR('',#104501,1000.);
#15802=VECTOR('',#104502,1000.);
#15803=VECTOR('',#104503,1000.);
#15804=VECTOR('',#104504,1000.);
#15805=VECTOR('',#104507,1000.);
#15806=VECTOR('',#104508,1000.);
#15807=VECTOR('',#104509,1000.);
#15808=VECTOR('',#104512,1000.);
#15809=VECTOR('',#104513,1000.);
#15810=VECTOR('',#104514,1000.);
#15811=VECTOR('',#104517,1000.);
#15812=VECTOR('',#104518,1000.);
#15813=VECTOR('',#104521,1000.);
#15814=VECTOR('',#104522,1000.);
#15815=VECTOR('',#104523,1000.);
#15816=VECTOR('',#104524,1000.);
#15817=VECTOR('',#104527,1000.);
#15818=VECTOR('',#104528,1000.);
#15819=VECTOR('',#104529,1000.);
#15820=VECTOR('',#104532,1000.);
#15821=VECTOR('',#104533,1000.);
#15822=VECTOR('',#104534,1000.);
#15823=VECTOR('',#104537,1000.);
#15824=VECTOR('',#104538,1000.);
#15825=VECTOR('',#104541,1000.);
#15826=VECTOR('',#104542,1000.);
#15827=VECTOR('',#104543,1000.);
#15828=VECTOR('',#104544,1000.);
#15829=VECTOR('',#104547,1000.);
#15830=VECTOR('',#104548,1000.);
#15831=VECTOR('',#104549,1000.);
#15832=VECTOR('',#104552,1000.);
#15833=VECTOR('',#104553,1000.);
#15834=VECTOR('',#104554,1000.);
#15835=VECTOR('',#104557,1000.);
#15836=VECTOR('',#104558,1000.);
#15837=VECTOR('',#104561,1000.);
#15838=VECTOR('',#104562,1000.);
#15839=VECTOR('',#104563,1000.);
#15840=VECTOR('',#104564,1000.);
#15841=VECTOR('',#104567,1000.);
#15842=VECTOR('',#104568,1000.);
#15843=VECTOR('',#104569,1000.);
#15844=VECTOR('',#104572,1000.);
#15845=VECTOR('',#104573,1000.);
#15846=VECTOR('',#104574,1000.);
#15847=VECTOR('',#104577,1000.);
#15848=VECTOR('',#104578,1000.);
#15849=VECTOR('',#104581,1000.);
#15850=VECTOR('',#104582,1000.);
#15851=VECTOR('',#104583,1000.);
#15852=VECTOR('',#104584,1000.);
#15853=VECTOR('',#104587,1000.);
#15854=VECTOR('',#104588,1000.);
#15855=VECTOR('',#104589,1000.);
#15856=VECTOR('',#104592,1000.);
#15857=VECTOR('',#104593,1000.);
#15858=VECTOR('',#104594,1000.);
#15859=VECTOR('',#104597,1000.);
#15860=VECTOR('',#104598,1000.);
#15861=VECTOR('',#104601,1000.);
#15862=VECTOR('',#104602,1000.);
#15863=VECTOR('',#104603,1000.);
#15864=VECTOR('',#104604,1000.);
#15865=VECTOR('',#104607,1000.);
#15866=VECTOR('',#104608,1000.);
#15867=VECTOR('',#104609,1000.);
#15868=VECTOR('',#104612,1000.);
#15869=VECTOR('',#104613,1000.);
#15870=VECTOR('',#104614,1000.);
#15871=VECTOR('',#104617,1000.);
#15872=VECTOR('',#104618,1000.);
#15873=VECTOR('',#104621,1000.);
#15874=VECTOR('',#104622,1000.);
#15875=VECTOR('',#104623,1000.);
#15876=VECTOR('',#104624,1000.);
#15877=VECTOR('',#104627,1000.);
#15878=VECTOR('',#104628,1000.);
#15879=VECTOR('',#104629,1000.);
#15880=VECTOR('',#104632,1000.);
#15881=VECTOR('',#104633,1000.);
#15882=VECTOR('',#104634,1000.);
#15883=VECTOR('',#104637,1000.);
#15884=VECTOR('',#104638,1000.);
#15885=VECTOR('',#104641,1000.);
#15886=VECTOR('',#104642,1000.);
#15887=VECTOR('',#104643,1000.);
#15888=VECTOR('',#104644,1000.);
#15889=VECTOR('',#104647,1000.);
#15890=VECTOR('',#104648,1000.);
#15891=VECTOR('',#104649,1000.);
#15892=VECTOR('',#104652,1000.);
#15893=VECTOR('',#104653,1000.);
#15894=VECTOR('',#104654,1000.);
#15895=VECTOR('',#104657,1000.);
#15896=VECTOR('',#104658,1000.);
#15897=VECTOR('',#104661,1000.);
#15898=VECTOR('',#104662,1000.);
#15899=VECTOR('',#104663,1000.);
#15900=VECTOR('',#104664,1000.);
#15901=VECTOR('',#104667,1000.);
#15902=VECTOR('',#104668,1000.);
#15903=VECTOR('',#104669,1000.);
#15904=VECTOR('',#104672,1000.);
#15905=VECTOR('',#104673,1000.);
#15906=VECTOR('',#104674,1000.);
#15907=VECTOR('',#104677,1000.);
#15908=VECTOR('',#104678,1000.);
#15909=VECTOR('',#104681,1000.);
#15910=VECTOR('',#104682,1000.);
#15911=VECTOR('',#104683,1000.);
#15912=VECTOR('',#104684,1000.);
#15913=VECTOR('',#104687,1000.);
#15914=VECTOR('',#104688,1000.);
#15915=VECTOR('',#104689,1000.);
#15916=VECTOR('',#104692,1000.);
#15917=VECTOR('',#104693,1000.);
#15918=VECTOR('',#104694,1000.);
#15919=VECTOR('',#104697,1000.);
#15920=VECTOR('',#104698,1000.);
#15921=VECTOR('',#104701,1000.);
#15922=VECTOR('',#104702,1000.);
#15923=VECTOR('',#104703,1000.);
#15924=VECTOR('',#104704,1000.);
#15925=VECTOR('',#104707,1000.);
#15926=VECTOR('',#104708,1000.);
#15927=VECTOR('',#104709,1000.);
#15928=VECTOR('',#104712,1000.);
#15929=VECTOR('',#104713,1000.);
#15930=VECTOR('',#104714,1000.);
#15931=VECTOR('',#104717,1000.);
#15932=VECTOR('',#104718,1000.);
#15933=VECTOR('',#104721,1000.);
#15934=VECTOR('',#104722,1000.);
#15935=VECTOR('',#104723,1000.);
#15936=VECTOR('',#104724,1000.);
#15937=VECTOR('',#104727,1000.);
#15938=VECTOR('',#104728,1000.);
#15939=VECTOR('',#104729,1000.);
#15940=VECTOR('',#104732,1000.);
#15941=VECTOR('',#104733,1000.);
#15942=VECTOR('',#104734,1000.);
#15943=VECTOR('',#104737,1000.);
#15944=VECTOR('',#104738,1000.);
#15945=VECTOR('',#104741,1000.);
#15946=VECTOR('',#104742,1000.);
#15947=VECTOR('',#104743,1000.);
#15948=VECTOR('',#104744,1000.);
#15949=VECTOR('',#104747,1000.);
#15950=VECTOR('',#104748,1000.);
#15951=VECTOR('',#104749,1000.);
#15952=VECTOR('',#104752,1000.);
#15953=VECTOR('',#104753,1000.);
#15954=VECTOR('',#104754,1000.);
#15955=VECTOR('',#104757,1000.);
#15956=VECTOR('',#104758,1000.);
#15957=VECTOR('',#104761,1000.);
#15958=VECTOR('',#104762,1000.);
#15959=VECTOR('',#104763,1000.);
#15960=VECTOR('',#104764,1000.);
#15961=VECTOR('',#104767,1000.);
#15962=VECTOR('',#104768,1000.);
#15963=VECTOR('',#104769,1000.);
#15964=VECTOR('',#104772,1000.);
#15965=VECTOR('',#104773,1000.);
#15966=VECTOR('',#104774,1000.);
#15967=VECTOR('',#104777,1000.);
#15968=VECTOR('',#104778,1000.);
#15969=VECTOR('',#104781,1000.);
#15970=VECTOR('',#104782,1000.);
#15971=VECTOR('',#104783,1000.);
#15972=VECTOR('',#104784,1000.);
#15973=VECTOR('',#104787,1000.);
#15974=VECTOR('',#104788,1000.);
#15975=VECTOR('',#104789,1000.);
#15976=VECTOR('',#104792,1000.);
#15977=VECTOR('',#104793,1000.);
#15978=VECTOR('',#104794,1000.);
#15979=VECTOR('',#104797,1000.);
#15980=VECTOR('',#104798,1000.);
#15981=VECTOR('',#104801,1000.);
#15982=VECTOR('',#104802,1000.);
#15983=VECTOR('',#104803,1000.);
#15984=VECTOR('',#104804,1000.);
#15985=VECTOR('',#104807,1000.);
#15986=VECTOR('',#104808,1000.);
#15987=VECTOR('',#104809,1000.);
#15988=VECTOR('',#104812,1000.);
#15989=VECTOR('',#104813,1000.);
#15990=VECTOR('',#104814,1000.);
#15991=VECTOR('',#104817,1000.);
#15992=VECTOR('',#104818,1000.);
#15993=VECTOR('',#104821,1000.);
#15994=VECTOR('',#104822,1000.);
#15995=VECTOR('',#104823,1000.);
#15996=VECTOR('',#104824,1000.);
#15997=VECTOR('',#104827,1000.);
#15998=VECTOR('',#104828,1000.);
#15999=VECTOR('',#104829,1000.);
#16000=VECTOR('',#104832,1000.);
#16001=VECTOR('',#104833,1000.);
#16002=VECTOR('',#104834,1000.);
#16003=VECTOR('',#104837,1000.);
#16004=VECTOR('',#104838,1000.);
#16005=VECTOR('',#104841,1000.);
#16006=VECTOR('',#104842,1000.);
#16007=VECTOR('',#104843,1000.);
#16008=VECTOR('',#104844,1000.);
#16009=VECTOR('',#104847,1000.);
#16010=VECTOR('',#104848,1000.);
#16011=VECTOR('',#104849,1000.);
#16012=VECTOR('',#104852,1000.);
#16013=VECTOR('',#104853,1000.);
#16014=VECTOR('',#104854,1000.);
#16015=VECTOR('',#104857,1000.);
#16016=VECTOR('',#104858,1000.);
#16017=VECTOR('',#104861,1000.);
#16018=VECTOR('',#104862,1000.);
#16019=VECTOR('',#104863,1000.);
#16020=VECTOR('',#104864,1000.);
#16021=VECTOR('',#104867,1000.);
#16022=VECTOR('',#104868,1000.);
#16023=VECTOR('',#104869,1000.);
#16024=VECTOR('',#104872,1000.);
#16025=VECTOR('',#104873,1000.);
#16026=VECTOR('',#104874,1000.);
#16027=VECTOR('',#104877,1000.);
#16028=VECTOR('',#104878,1000.);
#16029=VECTOR('',#104881,1000.);
#16030=VECTOR('',#104882,1000.);
#16031=VECTOR('',#104883,1000.);
#16032=VECTOR('',#104884,1000.);
#16033=VECTOR('',#104887,1000.);
#16034=VECTOR('',#104888,1000.);
#16035=VECTOR('',#104889,1000.);
#16036=VECTOR('',#104892,1000.);
#16037=VECTOR('',#104893,1000.);
#16038=VECTOR('',#104894,1000.);
#16039=VECTOR('',#104897,1000.);
#16040=VECTOR('',#104898,1000.);
#16041=VECTOR('',#104901,1000.);
#16042=VECTOR('',#104902,1000.);
#16043=VECTOR('',#104903,1000.);
#16044=VECTOR('',#104904,1000.);
#16045=VECTOR('',#104907,1000.);
#16046=VECTOR('',#104908,1000.);
#16047=VECTOR('',#104909,1000.);
#16048=VECTOR('',#104912,1000.);
#16049=VECTOR('',#104913,1000.);
#16050=VECTOR('',#104914,1000.);
#16051=VECTOR('',#104917,1000.);
#16052=VECTOR('',#104918,1000.);
#16053=VECTOR('',#104921,1000.);
#16054=VECTOR('',#104922,1000.);
#16055=VECTOR('',#104923,1000.);
#16056=VECTOR('',#104924,1000.);
#16057=VECTOR('',#104927,1000.);
#16058=VECTOR('',#104928,1000.);
#16059=VECTOR('',#104929,1000.);
#16060=VECTOR('',#104932,1000.);
#16061=VECTOR('',#104933,1000.);
#16062=VECTOR('',#104934,1000.);
#16063=VECTOR('',#104937,1000.);
#16064=VECTOR('',#104938,1000.);
#16065=VECTOR('',#104941,1000.);
#16066=VECTOR('',#104942,1000.);
#16067=VECTOR('',#104943,1000.);
#16068=VECTOR('',#104944,1000.);
#16069=VECTOR('',#104947,1000.);
#16070=VECTOR('',#104948,1000.);
#16071=VECTOR('',#104949,1000.);
#16072=VECTOR('',#104952,1000.);
#16073=VECTOR('',#104953,1000.);
#16074=VECTOR('',#104954,1000.);
#16075=VECTOR('',#104957,1000.);
#16076=VECTOR('',#104958,1000.);
#16077=VECTOR('',#104961,1000.);
#16078=VECTOR('',#104962,1000.);
#16079=VECTOR('',#104963,1000.);
#16080=VECTOR('',#104964,1000.);
#16081=VECTOR('',#104967,1000.);
#16082=VECTOR('',#104968,1000.);
#16083=VECTOR('',#104969,1000.);
#16084=VECTOR('',#104972,1000.);
#16085=VECTOR('',#104973,1000.);
#16086=VECTOR('',#104974,1000.);
#16087=VECTOR('',#104977,1000.);
#16088=VECTOR('',#104978,1000.);
#16089=VECTOR('',#104981,1000.);
#16090=VECTOR('',#104982,1000.);
#16091=VECTOR('',#104983,1000.);
#16092=VECTOR('',#104984,1000.);
#16093=VECTOR('',#104987,1000.);
#16094=VECTOR('',#104988,1000.);
#16095=VECTOR('',#104989,1000.);
#16096=VECTOR('',#104992,1000.);
#16097=VECTOR('',#104993,1000.);
#16098=VECTOR('',#104994,1000.);
#16099=VECTOR('',#104997,1000.);
#16100=VECTOR('',#104998,1000.);
#16101=VECTOR('',#105001,1000.);
#16102=VECTOR('',#105002,1000.);
#16103=VECTOR('',#105003,1000.);
#16104=VECTOR('',#105004,1000.);
#16105=VECTOR('',#105007,1000.);
#16106=VECTOR('',#105008,1000.);
#16107=VECTOR('',#105009,1000.);
#16108=VECTOR('',#105012,1000.);
#16109=VECTOR('',#105013,1000.);
#16110=VECTOR('',#105014,1000.);
#16111=VECTOR('',#105017,1000.);
#16112=VECTOR('',#105018,1000.);
#16113=VECTOR('',#105021,1000.);
#16114=VECTOR('',#105022,1000.);
#16115=VECTOR('',#105023,1000.);
#16116=VECTOR('',#105024,1000.);
#16117=VECTOR('',#105027,1000.);
#16118=VECTOR('',#105028,1000.);
#16119=VECTOR('',#105029,1000.);
#16120=VECTOR('',#105032,1000.);
#16121=VECTOR('',#105033,1000.);
#16122=VECTOR('',#105034,1000.);
#16123=VECTOR('',#105037,1000.);
#16124=VECTOR('',#105038,1000.);
#16125=VECTOR('',#105041,1000.);
#16126=VECTOR('',#105042,1000.);
#16127=VECTOR('',#105043,1000.);
#16128=VECTOR('',#105044,1000.);
#16129=VECTOR('',#105047,1000.);
#16130=VECTOR('',#105048,1000.);
#16131=VECTOR('',#105049,1000.);
#16132=VECTOR('',#105052,1000.);
#16133=VECTOR('',#105053,1000.);
#16134=VECTOR('',#105054,1000.);
#16135=VECTOR('',#105057,1000.);
#16136=VECTOR('',#105058,1000.);
#16137=VECTOR('',#105061,1000.);
#16138=VECTOR('',#105062,1000.);
#16139=VECTOR('',#105063,1000.);
#16140=VECTOR('',#105064,1000.);
#16141=VECTOR('',#105067,1000.);
#16142=VECTOR('',#105068,1000.);
#16143=VECTOR('',#105069,1000.);
#16144=VECTOR('',#105072,1000.);
#16145=VECTOR('',#105073,1000.);
#16146=VECTOR('',#105074,1000.);
#16147=VECTOR('',#105077,1000.);
#16148=VECTOR('',#105078,1000.);
#16149=VECTOR('',#105081,1000.);
#16150=VECTOR('',#105082,1000.);
#16151=VECTOR('',#105083,1000.);
#16152=VECTOR('',#105084,1000.);
#16153=VECTOR('',#105087,1000.);
#16154=VECTOR('',#105088,1000.);
#16155=VECTOR('',#105089,1000.);
#16156=VECTOR('',#105092,1000.);
#16157=VECTOR('',#105093,1000.);
#16158=VECTOR('',#105094,1000.);
#16159=VECTOR('',#105097,1000.);
#16160=VECTOR('',#105098,1000.);
#16161=VECTOR('',#105101,1000.);
#16162=VECTOR('',#105102,1000.);
#16163=VECTOR('',#105103,1000.);
#16164=VECTOR('',#105104,1000.);
#16165=VECTOR('',#105107,1000.);
#16166=VECTOR('',#105108,1000.);
#16167=VECTOR('',#105109,1000.);
#16168=VECTOR('',#105112,1000.);
#16169=VECTOR('',#105113,1000.);
#16170=VECTOR('',#105114,1000.);
#16171=VECTOR('',#105117,1000.);
#16172=VECTOR('',#105118,1000.);
#16173=VECTOR('',#105121,1000.);
#16174=VECTOR('',#105122,1000.);
#16175=VECTOR('',#105123,1000.);
#16176=VECTOR('',#105124,1000.);
#16177=VECTOR('',#105127,1000.);
#16178=VECTOR('',#105128,1000.);
#16179=VECTOR('',#105129,1000.);
#16180=VECTOR('',#105132,1000.);
#16181=VECTOR('',#105133,1000.);
#16182=VECTOR('',#105134,1000.);
#16183=VECTOR('',#105137,1000.);
#16184=VECTOR('',#105138,1000.);
#16185=VECTOR('',#105141,1000.);
#16186=VECTOR('',#105142,1000.);
#16187=VECTOR('',#105143,1000.);
#16188=VECTOR('',#105144,1000.);
#16189=VECTOR('',#105147,1000.);
#16190=VECTOR('',#105148,1000.);
#16191=VECTOR('',#105149,1000.);
#16192=VECTOR('',#105152,1000.);
#16193=VECTOR('',#105153,1000.);
#16194=VECTOR('',#105154,1000.);
#16195=VECTOR('',#105157,1000.);
#16196=VECTOR('',#105158,1000.);
#16197=VECTOR('',#105161,1000.);
#16198=VECTOR('',#105162,1000.);
#16199=VECTOR('',#105163,1000.);
#16200=VECTOR('',#105164,1000.);
#16201=VECTOR('',#105167,1000.);
#16202=VECTOR('',#105168,1000.);
#16203=VECTOR('',#105169,1000.);
#16204=VECTOR('',#105172,1000.);
#16205=VECTOR('',#105173,1000.);
#16206=VECTOR('',#105174,1000.);
#16207=VECTOR('',#105177,1000.);
#16208=VECTOR('',#105178,1000.);
#16209=VECTOR('',#105181,1000.);
#16210=VECTOR('',#105182,1000.);
#16211=VECTOR('',#105183,1000.);
#16212=VECTOR('',#105184,1000.);
#16213=VECTOR('',#105187,1000.);
#16214=VECTOR('',#105188,1000.);
#16215=VECTOR('',#105189,1000.);
#16216=VECTOR('',#105192,1000.);
#16217=VECTOR('',#105193,1000.);
#16218=VECTOR('',#105194,1000.);
#16219=VECTOR('',#105197,1000.);
#16220=VECTOR('',#105198,1000.);
#16221=VECTOR('',#105201,1000.);
#16222=VECTOR('',#105202,1000.);
#16223=VECTOR('',#105203,1000.);
#16224=VECTOR('',#105204,1000.);
#16225=VECTOR('',#105207,1000.);
#16226=VECTOR('',#105208,1000.);
#16227=VECTOR('',#105209,1000.);
#16228=VECTOR('',#105212,1000.);
#16229=VECTOR('',#105213,1000.);
#16230=VECTOR('',#105214,1000.);
#16231=VECTOR('',#105217,1000.);
#16232=VECTOR('',#105218,1000.);
#16233=VECTOR('',#105221,1000.);
#16234=VECTOR('',#105222,1000.);
#16235=VECTOR('',#105223,1000.);
#16236=VECTOR('',#105224,1000.);
#16237=VECTOR('',#105227,1000.);
#16238=VECTOR('',#105228,1000.);
#16239=VECTOR('',#105229,1000.);
#16240=VECTOR('',#105232,1000.);
#16241=VECTOR('',#105233,1000.);
#16242=VECTOR('',#105234,1000.);
#16243=VECTOR('',#105237,1000.);
#16244=VECTOR('',#105238,1000.);
#16245=VECTOR('',#105241,1000.);
#16246=VECTOR('',#105242,1000.);
#16247=VECTOR('',#105243,1000.);
#16248=VECTOR('',#105244,1000.);
#16249=VECTOR('',#105247,1000.);
#16250=VECTOR('',#105248,1000.);
#16251=VECTOR('',#105249,1000.);
#16252=VECTOR('',#105252,1000.);
#16253=VECTOR('',#105253,1000.);
#16254=VECTOR('',#105254,1000.);
#16255=VECTOR('',#105257,1000.);
#16256=VECTOR('',#105258,1000.);
#16257=VECTOR('',#105261,1000.);
#16258=VECTOR('',#105262,1000.);
#16259=VECTOR('',#105263,1000.);
#16260=VECTOR('',#105264,1000.);
#16261=VECTOR('',#105267,1000.);
#16262=VECTOR('',#105268,1000.);
#16263=VECTOR('',#105269,1000.);
#16264=VECTOR('',#105272,1000.);
#16265=VECTOR('',#105273,1000.);
#16266=VECTOR('',#105274,1000.);
#16267=VECTOR('',#105277,1000.);
#16268=VECTOR('',#105278,1000.);
#16269=VECTOR('',#105281,1000.);
#16270=VECTOR('',#105282,1000.);
#16271=VECTOR('',#105283,1000.);
#16272=VECTOR('',#105284,1000.);
#16273=VECTOR('',#105287,1000.);
#16274=VECTOR('',#105288,1000.);
#16275=VECTOR('',#105289,1000.);
#16276=VECTOR('',#105292,1000.);
#16277=VECTOR('',#105293,1000.);
#16278=VECTOR('',#105294,1000.);
#16279=VECTOR('',#105297,1000.);
#16280=VECTOR('',#105298,1000.);
#16281=VECTOR('',#105301,1000.);
#16282=VECTOR('',#105302,1000.);
#16283=VECTOR('',#105303,1000.);
#16284=VECTOR('',#105304,1000.);
#16285=VECTOR('',#105307,1000.);
#16286=VECTOR('',#105308,1000.);
#16287=VECTOR('',#105309,1000.);
#16288=VECTOR('',#105312,1000.);
#16289=VECTOR('',#105313,1000.);
#16290=VECTOR('',#105314,1000.);
#16291=VECTOR('',#105317,1000.);
#16292=VECTOR('',#105318,1000.);
#16293=VECTOR('',#105321,1000.);
#16294=VECTOR('',#105322,1000.);
#16295=VECTOR('',#105323,1000.);
#16296=VECTOR('',#105324,1000.);
#16297=VECTOR('',#105327,1000.);
#16298=VECTOR('',#105328,1000.);
#16299=VECTOR('',#105329,1000.);
#16300=VECTOR('',#105332,1000.);
#16301=VECTOR('',#105333,1000.);
#16302=VECTOR('',#105334,1000.);
#16303=VECTOR('',#105337,1000.);
#16304=VECTOR('',#105338,1000.);
#16305=VECTOR('',#105341,1000.);
#16306=VECTOR('',#105342,1000.);
#16307=VECTOR('',#105343,1000.);
#16308=VECTOR('',#105344,1000.);
#16309=VECTOR('',#105347,1000.);
#16310=VECTOR('',#105348,1000.);
#16311=VECTOR('',#105349,1000.);
#16312=VECTOR('',#105352,1000.);
#16313=VECTOR('',#105353,1000.);
#16314=VECTOR('',#105354,1000.);
#16315=VECTOR('',#105357,1000.);
#16316=VECTOR('',#105358,1000.);
#16317=VECTOR('',#105361,1000.);
#16318=VECTOR('',#105362,1000.);
#16319=VECTOR('',#105363,1000.);
#16320=VECTOR('',#105364,1000.);
#16321=VECTOR('',#105367,1000.);
#16322=VECTOR('',#105368,1000.);
#16323=VECTOR('',#105369,1000.);
#16324=VECTOR('',#105372,1000.);
#16325=VECTOR('',#105373,1000.);
#16326=VECTOR('',#105374,1000.);
#16327=VECTOR('',#105377,1000.);
#16328=VECTOR('',#105378,1000.);
#16329=VECTOR('',#105381,1000.);
#16330=VECTOR('',#105382,1000.);
#16331=VECTOR('',#105383,1000.);
#16332=VECTOR('',#105384,1000.);
#16333=VECTOR('',#105387,1000.);
#16334=VECTOR('',#105388,1000.);
#16335=VECTOR('',#105389,1000.);
#16336=VECTOR('',#105392,1000.);
#16337=VECTOR('',#105393,1000.);
#16338=VECTOR('',#105394,1000.);
#16339=VECTOR('',#105397,1000.);
#16340=VECTOR('',#105398,1000.);
#16341=VECTOR('',#105401,1000.);
#16342=VECTOR('',#105402,1000.);
#16343=VECTOR('',#105403,1000.);
#16344=VECTOR('',#105404,1000.);
#16345=VECTOR('',#105407,1000.);
#16346=VECTOR('',#105408,1000.);
#16347=VECTOR('',#105409,1000.);
#16348=VECTOR('',#105412,1000.);
#16349=VECTOR('',#105413,1000.);
#16350=VECTOR('',#105414,1000.);
#16351=VECTOR('',#105417,1000.);
#16352=VECTOR('',#105418,1000.);
#16353=VECTOR('',#105421,1000.);
#16354=VECTOR('',#105422,1000.);
#16355=VECTOR('',#105423,1000.);
#16356=VECTOR('',#105424,1000.);
#16357=VECTOR('',#105427,1000.);
#16358=VECTOR('',#105428,1000.);
#16359=VECTOR('',#105429,1000.);
#16360=VECTOR('',#105432,1000.);
#16361=VECTOR('',#105433,1000.);
#16362=VECTOR('',#105434,1000.);
#16363=VECTOR('',#105437,1000.);
#16364=VECTOR('',#105438,1000.);
#16365=VECTOR('',#105441,1000.);
#16366=VECTOR('',#105442,1000.);
#16367=VECTOR('',#105443,1000.);
#16368=VECTOR('',#105444,1000.);
#16369=VECTOR('',#105447,1000.);
#16370=VECTOR('',#105448,1000.);
#16371=VECTOR('',#105449,1000.);
#16372=VECTOR('',#105452,1000.);
#16373=VECTOR('',#105453,1000.);
#16374=VECTOR('',#105454,1000.);
#16375=VECTOR('',#105457,1000.);
#16376=VECTOR('',#105458,1000.);
#16377=VECTOR('',#105461,1000.);
#16378=VECTOR('',#105462,1000.);
#16379=VECTOR('',#105463,1000.);
#16380=VECTOR('',#105464,1000.);
#16381=VECTOR('',#105467,1000.);
#16382=VECTOR('',#105468,1000.);
#16383=VECTOR('',#105469,1000.);
#16384=VECTOR('',#105472,1000.);
#16385=VECTOR('',#105473,1000.);
#16386=VECTOR('',#105474,1000.);
#16387=VECTOR('',#105477,1000.);
#16388=VECTOR('',#105478,1000.);
#16389=VECTOR('',#105481,1000.);
#16390=VECTOR('',#105482,1000.);
#16391=VECTOR('',#105483,1000.);
#16392=VECTOR('',#105484,1000.);
#16393=VECTOR('',#105487,1000.);
#16394=VECTOR('',#105488,1000.);
#16395=VECTOR('',#105489,1000.);
#16396=VECTOR('',#105492,1000.);
#16397=VECTOR('',#105493,1000.);
#16398=VECTOR('',#105494,1000.);
#16399=VECTOR('',#105497,1000.);
#16400=VECTOR('',#105498,1000.);
#16401=VECTOR('',#105501,1000.);
#16402=VECTOR('',#105502,1000.);
#16403=VECTOR('',#105503,1000.);
#16404=VECTOR('',#105504,1000.);
#16405=VECTOR('',#105507,1000.);
#16406=VECTOR('',#105508,1000.);
#16407=VECTOR('',#105509,1000.);
#16408=VECTOR('',#105512,1000.);
#16409=VECTOR('',#105513,1000.);
#16410=VECTOR('',#105514,1000.);
#16411=VECTOR('',#105517,1000.);
#16412=VECTOR('',#105518,1000.);
#16413=VECTOR('',#105521,1000.);
#16414=VECTOR('',#105522,1000.);
#16415=VECTOR('',#105523,1000.);
#16416=VECTOR('',#105524,1000.);
#16417=VECTOR('',#105527,1000.);
#16418=VECTOR('',#105528,1000.);
#16419=VECTOR('',#105529,1000.);
#16420=VECTOR('',#105532,1000.);
#16421=VECTOR('',#105533,1000.);
#16422=VECTOR('',#105534,1000.);
#16423=VECTOR('',#105537,1000.);
#16424=VECTOR('',#105538,1000.);
#16425=VECTOR('',#105541,1000.);
#16426=VECTOR('',#105542,1000.);
#16427=VECTOR('',#105543,1000.);
#16428=VECTOR('',#105544,1000.);
#16429=VECTOR('',#105547,1000.);
#16430=VECTOR('',#105548,1000.);
#16431=VECTOR('',#105549,1000.);
#16432=VECTOR('',#105552,1000.);
#16433=VECTOR('',#105553,1000.);
#16434=VECTOR('',#105554,1000.);
#16435=VECTOR('',#105557,1000.);
#16436=VECTOR('',#105558,1000.);
#16437=VECTOR('',#105561,1000.);
#16438=VECTOR('',#105562,1000.);
#16439=VECTOR('',#105563,1000.);
#16440=VECTOR('',#105564,1000.);
#16441=VECTOR('',#105567,1000.);
#16442=VECTOR('',#105568,1000.);
#16443=VECTOR('',#105569,1000.);
#16444=VECTOR('',#105572,1000.);
#16445=VECTOR('',#105573,1000.);
#16446=VECTOR('',#105574,1000.);
#16447=VECTOR('',#105577,1000.);
#16448=VECTOR('',#105578,1000.);
#16449=VECTOR('',#105581,1000.);
#16450=VECTOR('',#105582,1000.);
#16451=VECTOR('',#105583,1000.);
#16452=VECTOR('',#105584,1000.);
#16453=VECTOR('',#105587,1000.);
#16454=VECTOR('',#105588,1000.);
#16455=VECTOR('',#105589,1000.);
#16456=VECTOR('',#105592,1000.);
#16457=VECTOR('',#105593,1000.);
#16458=VECTOR('',#105594,1000.);
#16459=VECTOR('',#105597,1000.);
#16460=VECTOR('',#105598,1000.);
#16461=VECTOR('',#105601,1000.);
#16462=VECTOR('',#105602,1000.);
#16463=VECTOR('',#105603,1000.);
#16464=VECTOR('',#105604,1000.);
#16465=VECTOR('',#105607,1000.);
#16466=VECTOR('',#105608,1000.);
#16467=VECTOR('',#105609,1000.);
#16468=VECTOR('',#105612,1000.);
#16469=VECTOR('',#105613,1000.);
#16470=VECTOR('',#105614,1000.);
#16471=VECTOR('',#105617,1000.);
#16472=VECTOR('',#105618,1000.);
#16473=VECTOR('',#105621,1000.);
#16474=VECTOR('',#105622,1000.);
#16475=VECTOR('',#105623,1000.);
#16476=VECTOR('',#105624,1000.);
#16477=VECTOR('',#105627,1000.);
#16478=VECTOR('',#105628,1000.);
#16479=VECTOR('',#105629,1000.);
#16480=VECTOR('',#105632,1000.);
#16481=VECTOR('',#105633,1000.);
#16482=VECTOR('',#105634,1000.);
#16483=VECTOR('',#105637,1000.);
#16484=VECTOR('',#105638,1000.);
#16485=VECTOR('',#105641,1000.);
#16486=VECTOR('',#105642,1000.);
#16487=VECTOR('',#105643,1000.);
#16488=VECTOR('',#105644,1000.);
#16489=VECTOR('',#105647,1000.);
#16490=VECTOR('',#105648,1000.);
#16491=VECTOR('',#105649,1000.);
#16492=VECTOR('',#105652,1000.);
#16493=VECTOR('',#105653,1000.);
#16494=VECTOR('',#105654,1000.);
#16495=VECTOR('',#105657,1000.);
#16496=VECTOR('',#105658,1000.);
#16497=VECTOR('',#105661,1000.);
#16498=VECTOR('',#105662,1000.);
#16499=VECTOR('',#105663,1000.);
#16500=VECTOR('',#105664,1000.);
#16501=VECTOR('',#105667,1000.);
#16502=VECTOR('',#105668,1000.);
#16503=VECTOR('',#105669,1000.);
#16504=VECTOR('',#105672,1000.);
#16505=VECTOR('',#105673,1000.);
#16506=VECTOR('',#105674,1000.);
#16507=VECTOR('',#105677,1000.);
#16508=VECTOR('',#105678,1000.);
#16509=VECTOR('',#105681,1000.);
#16510=VECTOR('',#105682,1000.);
#16511=VECTOR('',#105683,1000.);
#16512=VECTOR('',#105684,1000.);
#16513=VECTOR('',#105687,1000.);
#16514=VECTOR('',#105688,1000.);
#16515=VECTOR('',#105689,1000.);
#16516=VECTOR('',#105692,1000.);
#16517=VECTOR('',#105693,1000.);
#16518=VECTOR('',#105694,1000.);
#16519=VECTOR('',#105697,1000.);
#16520=VECTOR('',#105698,1000.);
#16521=VECTOR('',#105701,1000.);
#16522=VECTOR('',#105702,1000.);
#16523=VECTOR('',#105703,1000.);
#16524=VECTOR('',#105704,1000.);
#16525=VECTOR('',#105707,1000.);
#16526=VECTOR('',#105708,1000.);
#16527=VECTOR('',#105709,1000.);
#16528=VECTOR('',#105712,1000.);
#16529=VECTOR('',#105713,1000.);
#16530=VECTOR('',#105714,1000.);
#16531=VECTOR('',#105717,1000.);
#16532=VECTOR('',#105718,1000.);
#16533=VECTOR('',#105721,1000.);
#16534=VECTOR('',#105722,1000.);
#16535=VECTOR('',#105723,1000.);
#16536=VECTOR('',#105724,1000.);
#16537=VECTOR('',#105727,1000.);
#16538=VECTOR('',#105728,1000.);
#16539=VECTOR('',#105729,1000.);
#16540=VECTOR('',#105732,1000.);
#16541=VECTOR('',#105733,1000.);
#16542=VECTOR('',#105734,1000.);
#16543=VECTOR('',#105737,1000.);
#16544=VECTOR('',#105738,1000.);
#16545=VECTOR('',#105741,1000.);
#16546=VECTOR('',#105742,1000.);
#16547=VECTOR('',#105743,1000.);
#16548=VECTOR('',#105744,1000.);
#16549=VECTOR('',#105747,1000.);
#16550=VECTOR('',#105748,1000.);
#16551=VECTOR('',#105749,1000.);
#16552=VECTOR('',#105752,1000.);
#16553=VECTOR('',#105753,1000.);
#16554=VECTOR('',#105754,1000.);
#16555=VECTOR('',#105757,1000.);
#16556=VECTOR('',#105758,1000.);
#16557=VECTOR('',#105761,1000.);
#16558=VECTOR('',#105762,1000.);
#16559=VECTOR('',#105763,1000.);
#16560=VECTOR('',#105764,1000.);
#16561=VECTOR('',#105767,1000.);
#16562=VECTOR('',#105768,1000.);
#16563=VECTOR('',#105769,1000.);
#16564=VECTOR('',#105772,1000.);
#16565=VECTOR('',#105773,1000.);
#16566=VECTOR('',#105774,1000.);
#16567=VECTOR('',#105777,1000.);
#16568=VECTOR('',#105778,1000.);
#16569=VECTOR('',#105781,1000.);
#16570=VECTOR('',#105782,1000.);
#16571=VECTOR('',#105783,1000.);
#16572=VECTOR('',#105784,1000.);
#16573=VECTOR('',#105787,1000.);
#16574=VECTOR('',#105788,1000.);
#16575=VECTOR('',#105789,1000.);
#16576=VECTOR('',#105792,1000.);
#16577=VECTOR('',#105793,1000.);
#16578=VECTOR('',#105794,1000.);
#16579=VECTOR('',#105797,1000.);
#16580=VECTOR('',#105798,1000.);
#16581=VECTOR('',#105801,1000.);
#16582=VECTOR('',#105802,1000.);
#16583=VECTOR('',#105803,1000.);
#16584=VECTOR('',#105804,1000.);
#16585=VECTOR('',#105807,1000.);
#16586=VECTOR('',#105808,1000.);
#16587=VECTOR('',#105809,1000.);
#16588=VECTOR('',#105812,1000.);
#16589=VECTOR('',#105813,1000.);
#16590=VECTOR('',#105814,1000.);
#16591=VECTOR('',#105817,1000.);
#16592=VECTOR('',#105818,1000.);
#16593=VECTOR('',#105821,1000.);
#16594=VECTOR('',#105822,1000.);
#16595=VECTOR('',#105823,1000.);
#16596=VECTOR('',#105824,1000.);
#16597=VECTOR('',#105827,1000.);
#16598=VECTOR('',#105828,1000.);
#16599=VECTOR('',#105829,1000.);
#16600=VECTOR('',#105832,1000.);
#16601=VECTOR('',#105833,1000.);
#16602=VECTOR('',#105834,1000.);
#16603=VECTOR('',#105837,1000.);
#16604=VECTOR('',#105838,1000.);
#16605=VECTOR('',#105841,1000.);
#16606=VECTOR('',#105842,1000.);
#16607=VECTOR('',#105843,1000.);
#16608=VECTOR('',#105844,1000.);
#16609=VECTOR('',#105847,1000.);
#16610=VECTOR('',#105848,1000.);
#16611=VECTOR('',#105849,1000.);
#16612=VECTOR('',#105852,1000.);
#16613=VECTOR('',#105853,1000.);
#16614=VECTOR('',#105854,1000.);
#16615=VECTOR('',#105857,1000.);
#16616=VECTOR('',#105858,1000.);
#16617=VECTOR('',#105861,1000.);
#16618=VECTOR('',#105862,1000.);
#16619=VECTOR('',#105863,1000.);
#16620=VECTOR('',#105864,1000.);
#16621=VECTOR('',#105867,1000.);
#16622=VECTOR('',#105868,1000.);
#16623=VECTOR('',#105869,1000.);
#16624=VECTOR('',#105872,1000.);
#16625=VECTOR('',#105873,1000.);
#16626=VECTOR('',#105874,1000.);
#16627=VECTOR('',#105877,1000.);
#16628=VECTOR('',#105878,1000.);
#16629=VECTOR('',#105881,1000.);
#16630=VECTOR('',#105882,1000.);
#16631=VECTOR('',#105883,1000.);
#16632=VECTOR('',#105884,1000.);
#16633=VECTOR('',#105887,1000.);
#16634=VECTOR('',#105888,1000.);
#16635=VECTOR('',#105889,1000.);
#16636=VECTOR('',#105892,1000.);
#16637=VECTOR('',#105893,1000.);
#16638=VECTOR('',#105894,1000.);
#16639=VECTOR('',#105897,1000.);
#16640=VECTOR('',#105898,1000.);
#16641=VECTOR('',#105901,1000.);
#16642=VECTOR('',#105902,1000.);
#16643=VECTOR('',#105903,1000.);
#16644=VECTOR('',#105904,1000.);
#16645=VECTOR('',#105907,1000.);
#16646=VECTOR('',#105908,1000.);
#16647=VECTOR('',#105909,1000.);
#16648=VECTOR('',#105912,1000.);
#16649=VECTOR('',#105913,1000.);
#16650=VECTOR('',#105914,1000.);
#16651=VECTOR('',#105917,1000.);
#16652=VECTOR('',#105918,1000.);
#16653=VECTOR('',#105921,1000.);
#16654=VECTOR('',#105922,1000.);
#16655=VECTOR('',#105923,1000.);
#16656=VECTOR('',#105924,1000.);
#16657=VECTOR('',#105927,1000.);
#16658=VECTOR('',#105928,1000.);
#16659=VECTOR('',#105929,1000.);
#16660=VECTOR('',#105932,1000.);
#16661=VECTOR('',#105933,1000.);
#16662=VECTOR('',#105934,1000.);
#16663=VECTOR('',#105937,1000.);
#16664=VECTOR('',#105938,1000.);
#16665=VECTOR('',#105941,1000.);
#16666=VECTOR('',#105942,1000.);
#16667=VECTOR('',#105943,1000.);
#16668=VECTOR('',#105944,1000.);
#16669=VECTOR('',#105947,1000.);
#16670=VECTOR('',#105948,1000.);
#16671=VECTOR('',#105949,1000.);
#16672=VECTOR('',#105952,1000.);
#16673=VECTOR('',#105953,1000.);
#16674=VECTOR('',#105954,1000.);
#16675=VECTOR('',#105957,1000.);
#16676=VECTOR('',#105958,1000.);
#16677=VECTOR('',#105961,1000.);
#16678=VECTOR('',#105962,1000.);
#16679=VECTOR('',#105963,1000.);
#16680=VECTOR('',#105964,1000.);
#16681=VECTOR('',#105967,1000.);
#16682=VECTOR('',#105968,1000.);
#16683=VECTOR('',#105969,1000.);
#16684=VECTOR('',#105972,1000.);
#16685=VECTOR('',#105973,1000.);
#16686=VECTOR('',#105974,1000.);
#16687=VECTOR('',#105977,1000.);
#16688=VECTOR('',#105978,1000.);
#16689=VECTOR('',#105983,1000.);
#16690=VECTOR('',#105984,1000.);
#16691=VECTOR('',#105985,1000.);
#16692=VECTOR('',#105986,1000.);
#16693=VECTOR('',#105989,1000.);
#16694=VECTOR('',#105990,1000.);
#16695=VECTOR('',#105991,1000.);
#16696=VECTOR('',#105994,1000.);
#16697=VECTOR('',#105995,1000.);
#16698=VECTOR('',#105998,1000.);
#16699=VECTOR('',#105999,1000.);
#16700=VECTOR('',#106002,1000.);
#16701=VECTOR('',#106009,1000.);
#16702=VECTOR('',#106012,1000.);
#16703=VECTOR('',#106015,1000.);
#16704=VECTOR('',#106018,1000.);
#16705=VECTOR('',#106025,1000.);
#16706=VECTOR('',#106028,1000.);
#16707=VECTOR('',#106031,1000.);
#16708=VECTOR('',#106034,1000.);
#16709=VECTOR('',#106055,1000.);
#16710=VECTOR('',#106056,1000.);
#16711=VECTOR('',#106061,1000.);
#16712=VECTOR('',#106066,1000.);
#17023=PLANE('',#81067);
#17024=PLANE('',#81072);
#17025=PLANE('',#81073);
#17026=PLANE('',#81074);
#17027=PLANE('',#81075);
#17028=PLANE('',#81076);
#17029=PLANE('',#81079);
#17030=PLANE('',#81080);
#17031=PLANE('',#81081);
#17032=PLANE('',#81082);
#17033=PLANE('',#81084);
#17034=PLANE('',#81087);
#17035=PLANE('',#81090);
#17036=PLANE('',#81093);
#17037=PLANE('',#81095);
#17038=PLANE('',#81097);
#17039=PLANE('',#81100);
#17040=PLANE('',#81103);
#17041=PLANE('',#81106);
#17042=PLANE('',#81108);
#17043=PLANE('',#81111);
#17044=PLANE('',#81113);
#17045=PLANE('',#81115);
#17046=PLANE('',#81118);
#17047=PLANE('',#81120);
#17048=PLANE('',#81123);
#17049=PLANE('',#81126);
#17050=PLANE('',#81129);
#17051=PLANE('',#81132);
#17052=PLANE('',#81135);
#17053=PLANE('',#81138);
#17054=PLANE('',#81141);
#17055=PLANE('',#81144);
#17056=PLANE('',#81147);
#17057=PLANE('',#81150);
#17058=PLANE('',#81153);
#17059=PLANE('',#81156);
#17060=PLANE('',#81159);
#17061=PLANE('',#81162);
#17062=PLANE('',#81165);
#17063=PLANE('',#81168);
#17064=PLANE('',#81170);
#17065=PLANE('',#81173);
#17066=PLANE('',#81176);
#17067=PLANE('',#81179);
#17068=PLANE('',#81181);
#17069=PLANE('',#81184);
#17070=PLANE('',#81187);
#17071=PLANE('',#81189);
#17072=PLANE('',#81192);
#17073=PLANE('',#81194);
#17074=PLANE('',#81197);
#17075=PLANE('',#81200);
#17076=PLANE('',#81202);
#17077=PLANE('',#81205);
#17078=PLANE('',#81207);
#17079=PLANE('',#81210);
#17080=PLANE('',#81213);
#17081=PLANE('',#81216);
#17082=PLANE('',#81219);
#17083=PLANE('',#81221);
#17084=PLANE('',#81224);
#17085=PLANE('',#81227);
#17086=PLANE('',#81230);
#17087=PLANE('',#81233);
#17088=PLANE('',#81236);
#17089=PLANE('',#81239);
#17090=PLANE('',#81241);
#17091=PLANE('',#81244);
#17092=PLANE('',#81246);
#17093=PLANE('',#81249);
#17094=PLANE('',#81252);
#17095=PLANE('',#81254);
#17096=PLANE('',#81257);
#17097=PLANE('',#81259);
#17098=PLANE('',#81262);
#17099=PLANE('',#81265);
#17100=PLANE('',#81267);
#17101=PLANE('',#81270);
#17102=PLANE('',#81272);
#17103=PLANE('',#81275);
#17104=PLANE('',#81278);
#17105=PLANE('',#81280);
#17106=PLANE('',#81283);
#17107=PLANE('',#81285);
#17108=PLANE('',#81288);
#17109=PLANE('',#81291);
#17110=PLANE('',#81294);
#17111=PLANE('',#81297);
#17112=PLANE('',#81300);
#17113=PLANE('',#81303);
#17114=PLANE('',#81306);
#17115=PLANE('',#81309);
#17116=PLANE('',#81312);
#17117=PLANE('',#81315);
#17118=PLANE('',#81318);
#17119=PLANE('',#81321);
#17120=PLANE('',#81324);
#17121=PLANE('',#81327);
#17122=PLANE('',#81330);
#17123=PLANE('',#81333);
#17124=PLANE('',#81336);
#17125=PLANE('',#81339);
#17126=PLANE('',#81342);
#17127=PLANE('',#81345);
#17128=PLANE('',#81348);
#17129=PLANE('',#81351);
#17130=PLANE('',#81354);
#17131=PLANE('',#81357);
#17132=PLANE('',#81360);
#17133=PLANE('',#81363);
#17134=PLANE('',#81366);
#17135=PLANE('',#81369);
#17136=PLANE('',#81371);
#17137=PLANE('',#81374);
#17138=PLANE('',#81377);
#17139=PLANE('',#81379);
#17140=PLANE('',#81382);
#17141=PLANE('',#81384);
#17142=PLANE('',#81387);
#17143=PLANE('',#81390);
#17144=PLANE('',#81393);
#17145=PLANE('',#81396);
#17146=PLANE('',#81399);
#17147=PLANE('',#81402);
#17148=PLANE('',#81405);
#17149=PLANE('',#81408);
#17150=PLANE('',#81411);
#17151=PLANE('',#81414);
#17152=PLANE('',#81417);
#17153=PLANE('',#81420);
#17154=PLANE('',#81423);
#17155=PLANE('',#81426);
#17156=PLANE('',#81429);
#17157=PLANE('',#81432);
#17158=PLANE('',#81435);
#17159=PLANE('',#81438);
#17160=PLANE('',#81441);
#17161=PLANE('',#81444);
#17162=PLANE('',#81447);
#17163=PLANE('',#81450);
#17164=PLANE('',#81453);
#17165=PLANE('',#81456);
#17166=PLANE('',#81459);
#17167=PLANE('',#81462);
#17168=PLANE('',#81465);
#17169=PLANE('',#81468);
#17170=PLANE('',#81471);
#17171=PLANE('',#81474);
#17172=PLANE('',#81477);
#17173=PLANE('',#81480);
#17174=PLANE('',#81483);
#17175=PLANE('',#81486);
#17176=PLANE('',#81488);
#17177=PLANE('',#81491);
#17178=PLANE('',#81493);
#17179=PLANE('',#81496);
#17180=PLANE('',#81499);
#17181=PLANE('',#81501);
#17182=PLANE('',#81504);
#17183=PLANE('',#81506);
#17184=PLANE('',#81509);
#17185=PLANE('',#81512);
#17186=PLANE('',#81515);
#17187=PLANE('',#81518);
#17188=PLANE('',#81521);
#17189=PLANE('',#81524);
#17190=PLANE('',#81527);
#17191=PLANE('',#81530);
#17192=PLANE('',#81533);
#17193=PLANE('',#81536);
#17194=PLANE('',#81539);
#17195=PLANE('',#81542);
#17196=PLANE('',#81545);
#17197=PLANE('',#81548);
#17198=PLANE('',#81551);
#17199=PLANE('',#81554);
#17200=PLANE('',#81557);
#17201=PLANE('',#81560);
#17202=PLANE('',#81563);
#17203=PLANE('',#81566);
#17204=PLANE('',#81569);
#17205=PLANE('',#81572);
#17206=PLANE('',#81575);
#17207=PLANE('',#81578);
#17208=PLANE('',#81581);
#17209=PLANE('',#81584);
#17210=PLANE('',#81587);
#17211=PLANE('',#81590);
#17212=PLANE('',#81593);
#17213=PLANE('',#81596);
#17214=PLANE('',#81599);
#17215=PLANE('',#81602);
#17216=PLANE('',#81605);
#17217=PLANE('',#81608);
#17218=PLANE('',#81611);
#17219=PLANE('',#81614);
#17220=PLANE('',#81617);
#17221=PLANE('',#81620);
#17222=PLANE('',#81623);
#17223=PLANE('',#81626);
#17224=PLANE('',#81628);
#17225=PLANE('',#81631);
#17226=PLANE('',#81634);
#17227=PLANE('',#81637);
#17228=PLANE('',#81640);
#17229=PLANE('',#81643);
#17230=PLANE('',#81646);
#17231=PLANE('',#81649);
#17232=PLANE('',#81652);
#17233=PLANE('',#81655);
#17234=PLANE('',#81658);
#17235=PLANE('',#81661);
#17236=PLANE('',#81664);
#17237=PLANE('',#81667);
#17238=PLANE('',#81670);
#17239=PLANE('',#81673);
#17240=PLANE('',#81676);
#17241=PLANE('',#81679);
#17242=PLANE('',#81682);
#17243=PLANE('',#81685);
#17244=PLANE('',#81688);
#17245=PLANE('',#81691);
#17246=PLANE('',#81694);
#17247=PLANE('',#81697);
#17248=PLANE('',#81700);
#17249=PLANE('',#81703);
#17250=PLANE('',#81706);
#17251=PLANE('',#81709);
#17252=PLANE('',#81712);
#17253=PLANE('',#81715);
#17254=PLANE('',#81718);
#17255=PLANE('',#81721);
#17256=PLANE('',#81724);
#17257=PLANE('',#81727);
#17258=PLANE('',#81730);
#17259=PLANE('',#81733);
#17260=PLANE('',#81736);
#17261=PLANE('',#81739);
#17262=PLANE('',#81742);
#17263=PLANE('',#81745);
#17264=PLANE('',#81748);
#17265=PLANE('',#81751);
#17266=PLANE('',#81754);
#17267=PLANE('',#81757);
#17268=PLANE('',#81760);
#17269=PLANE('',#81763);
#17270=PLANE('',#81766);
#17271=PLANE('',#81769);
#17272=PLANE('',#81772);
#17273=PLANE('',#81774);
#17274=PLANE('',#81777);
#17275=PLANE('',#81780);
#17276=PLANE('',#81783);
#17277=PLANE('',#81786);
#17278=PLANE('',#81788);
#17279=PLANE('',#81791);
#17280=PLANE('',#81794);
#17281=PLANE('',#81797);
#17282=PLANE('',#81800);
#17283=PLANE('',#81803);
#17284=PLANE('',#81806);
#17285=PLANE('',#81809);
#17286=PLANE('',#81812);
#17287=PLANE('',#81815);
#17288=PLANE('',#81818);
#17289=PLANE('',#81821);
#17290=PLANE('',#81824);
#17291=PLANE('',#81827);
#17292=PLANE('',#81830);
#17293=PLANE('',#81833);
#17294=PLANE('',#81836);
#17295=PLANE('',#81839);
#17296=PLANE('',#81842);
#17297=PLANE('',#81845);
#17298=PLANE('',#81848);
#17299=PLANE('',#81851);
#17300=PLANE('',#81854);
#17301=PLANE('',#81857);
#17302=PLANE('',#81860);
#17303=PLANE('',#81863);
#17304=PLANE('',#81866);
#17305=PLANE('',#81869);
#17306=PLANE('',#81872);
#17307=PLANE('',#81875);
#17308=PLANE('',#81878);
#17309=PLANE('',#81881);
#17310=PLANE('',#81884);
#17311=PLANE('',#81887);
#17312=PLANE('',#81890);
#17313=PLANE('',#81893);
#17314=PLANE('',#81896);
#17315=PLANE('',#81899);
#17316=PLANE('',#81902);
#17317=PLANE('',#81905);
#17318=PLANE('',#81908);
#17319=PLANE('',#81911);
#17320=PLANE('',#81914);
#17321=PLANE('',#81917);
#17322=PLANE('',#81920);
#17323=PLANE('',#81923);
#17324=PLANE('',#81926);
#17325=PLANE('',#81929);
#17326=PLANE('',#81932);
#17327=PLANE('',#81935);
#17328=PLANE('',#81938);
#17329=PLANE('',#81941);
#17330=PLANE('',#81944);
#17331=PLANE('',#81947);
#17332=PLANE('',#81950);
#17333=PLANE('',#81953);
#17334=PLANE('',#81956);
#17335=PLANE('',#81959);
#17336=PLANE('',#81962);
#17337=PLANE('',#81965);
#17338=PLANE('',#81968);
#17339=PLANE('',#81971);
#17340=PLANE('',#81974);
#17341=PLANE('',#81977);
#17342=PLANE('',#81980);
#17343=PLANE('',#81983);
#17344=PLANE('',#81986);
#17345=PLANE('',#81989);
#17346=PLANE('',#81992);
#17347=PLANE('',#81995);
#17348=PLANE('',#81998);
#17349=PLANE('',#82001);
#17350=PLANE('',#82004);
#17351=PLANE('',#82007);
#17352=PLANE('',#82010);
#17353=PLANE('',#82013);
#17354=PLANE('',#82016);
#17355=PLANE('',#82019);
#17356=PLANE('',#82022);
#17357=PLANE('',#82025);
#17358=PLANE('',#82028);
#17359=PLANE('',#82031);
#17360=PLANE('',#82034);
#17361=PLANE('',#82037);
#17362=PLANE('',#82040);
#17363=PLANE('',#82043);
#17364=PLANE('',#82046);
#17365=PLANE('',#82049);
#17366=PLANE('',#82052);
#17367=PLANE('',#82055);
#17368=PLANE('',#82058);
#17369=PLANE('',#82061);
#17370=PLANE('',#82064);
#17371=PLANE('',#82067);
#17372=PLANE('',#82070);
#17373=PLANE('',#82073);
#17374=PLANE('',#82076);
#17375=PLANE('',#82079);
#17376=PLANE('',#82082);
#17377=PLANE('',#82085);
#17378=PLANE('',#82088);
#17379=PLANE('',#82091);
#17380=PLANE('',#82094);
#17381=PLANE('',#82097);
#17382=PLANE('',#82100);
#17383=PLANE('',#82103);
#17384=PLANE('',#82106);
#17385=PLANE('',#82109);
#17386=PLANE('',#82112);
#17387=PLANE('',#82115);
#17388=PLANE('',#82118);
#17389=PLANE('',#82121);
#17390=PLANE('',#82124);
#17391=PLANE('',#82127);
#17392=PLANE('',#82130);
#17393=PLANE('',#82133);
#17394=PLANE('',#82136);
#17395=PLANE('',#82139);
#17396=PLANE('',#82142);
#17397=PLANE('',#82145);
#17398=PLANE('',#82148);
#17399=PLANE('',#82151);
#17400=PLANE('',#82154);
#17401=PLANE('',#82157);
#17402=PLANE('',#82160);
#17403=PLANE('',#82163);
#17404=PLANE('',#82166);
#17405=PLANE('',#82169);
#17406=PLANE('',#82172);
#17407=PLANE('',#82175);
#17408=PLANE('',#82178);
#17409=PLANE('',#82181);
#17410=PLANE('',#82184);
#17411=PLANE('',#82187);
#17412=PLANE('',#82190);
#17413=PLANE('',#82193);
#17414=PLANE('',#82196);
#17415=PLANE('',#82199);
#17416=PLANE('',#82202);
#17417=PLANE('',#82205);
#17418=PLANE('',#82208);
#17419=PLANE('',#82211);
#17420=PLANE('',#82214);
#17421=PLANE('',#82217);
#17422=PLANE('',#82220);
#17423=PLANE('',#82223);
#17424=PLANE('',#82226);
#17425=PLANE('',#82229);
#17426=PLANE('',#82232);
#17427=PLANE('',#82235);
#17428=PLANE('',#82238);
#17429=PLANE('',#82241);
#17430=PLANE('',#82244);
#17431=PLANE('',#82247);
#17432=PLANE('',#82250);
#17433=PLANE('',#82253);
#17434=PLANE('',#82256);
#17435=PLANE('',#82259);
#17436=PLANE('',#82262);
#17437=PLANE('',#82265);
#17438=PLANE('',#82268);
#17439=PLANE('',#82271);
#17440=PLANE('',#82274);
#17441=PLANE('',#82277);
#17442=PLANE('',#82280);
#17443=PLANE('',#82283);
#17444=PLANE('',#82286);
#17445=PLANE('',#82289);
#17446=PLANE('',#82292);
#17447=PLANE('',#82295);
#17448=PLANE('',#82298);
#17449=PLANE('',#82301);
#17450=PLANE('',#82304);
#17451=PLANE('',#82307);
#17452=PLANE('',#82310);
#17453=PLANE('',#82313);
#17454=PLANE('',#82316);
#17455=PLANE('',#82319);
#17456=PLANE('',#82322);
#17457=PLANE('',#82325);
#17458=PLANE('',#82328);
#17459=PLANE('',#82331);
#17460=PLANE('',#82334);
#17461=PLANE('',#82337);
#17462=PLANE('',#82340);
#17463=PLANE('',#82343);
#17464=PLANE('',#82346);
#17465=PLANE('',#82349);
#17466=PLANE('',#82352);
#17467=PLANE('',#82355);
#17468=PLANE('',#82358);
#17469=PLANE('',#82361);
#17470=PLANE('',#82364);
#17471=PLANE('',#82367);
#17472=PLANE('',#82370);
#17473=PLANE('',#82373);
#17474=PLANE('',#82376);
#17475=PLANE('',#82379);
#17476=PLANE('',#82382);
#17477=PLANE('',#82385);
#17478=PLANE('',#82388);
#17479=PLANE('',#82391);
#17480=PLANE('',#82394);
#17481=PLANE('',#82397);
#17482=PLANE('',#82400);
#17483=PLANE('',#82403);
#17484=PLANE('',#82406);
#17485=PLANE('',#82409);
#17486=PLANE('',#82412);
#17487=PLANE('',#82415);
#17488=PLANE('',#82418);
#17489=PLANE('',#82421);
#17490=PLANE('',#82424);
#17491=PLANE('',#82427);
#17492=PLANE('',#82430);
#17493=PLANE('',#82433);
#17494=PLANE('',#82436);
#17495=PLANE('',#82439);
#17496=PLANE('',#82442);
#17497=PLANE('',#82445);
#17498=PLANE('',#82448);
#17499=PLANE('',#82451);
#17500=PLANE('',#82454);
#17501=PLANE('',#82457);
#17502=PLANE('',#82460);
#17503=PLANE('',#82463);
#17504=PLANE('',#82466);
#17505=PLANE('',#82469);
#17506=PLANE('',#82472);
#17507=PLANE('',#82475);
#17508=PLANE('',#82478);
#17509=PLANE('',#82481);
#17510=PLANE('',#82484);
#17511=PLANE('',#82487);
#17512=PLANE('',#82490);
#17513=PLANE('',#82493);
#17514=PLANE('',#82496);
#17515=PLANE('',#82499);
#17516=PLANE('',#82502);
#17517=PLANE('',#82505);
#17518=PLANE('',#82508);
#17519=PLANE('',#82511);
#17520=PLANE('',#82514);
#17521=PLANE('',#82517);
#17522=PLANE('',#82520);
#17523=PLANE('',#82523);
#17524=PLANE('',#82526);
#17525=PLANE('',#82529);
#17526=PLANE('',#82532);
#17527=PLANE('',#82535);
#17528=PLANE('',#82538);
#17529=PLANE('',#82541);
#17530=PLANE('',#82544);
#17531=PLANE('',#82547);
#17532=PLANE('',#82550);
#17533=PLANE('',#82553);
#17534=PLANE('',#82556);
#17535=PLANE('',#82559);
#17536=PLANE('',#82562);
#17537=PLANE('',#82565);
#17538=PLANE('',#82568);
#17539=PLANE('',#82571);
#17540=PLANE('',#82574);
#17541=PLANE('',#82577);
#17542=PLANE('',#82580);
#17543=PLANE('',#82583);
#17544=PLANE('',#82586);
#17545=PLANE('',#82589);
#17546=PLANE('',#82592);
#17547=PLANE('',#82595);
#17548=PLANE('',#82598);
#17549=PLANE('',#82601);
#17550=PLANE('',#82604);
#17551=PLANE('',#82607);
#17552=PLANE('',#82610);
#17553=PLANE('',#82613);
#17554=PLANE('',#82616);
#17555=PLANE('',#82619);
#17556=PLANE('',#82622);
#17557=PLANE('',#82625);
#17558=PLANE('',#82628);
#17559=PLANE('',#82631);
#17560=PLANE('',#82634);
#17561=PLANE('',#82636);
#17562=PLANE('',#82638);
#17563=PLANE('',#82640);
#17564=PLANE('',#82643);
#17565=PLANE('',#82646);
#17566=PLANE('',#82648);
#17567=PLANE('',#82651);
#17568=PLANE('',#82653);
#17569=PLANE('',#82656);
#17570=PLANE('',#82659);
#17571=PLANE('',#82661);
#17572=PLANE('',#82664);
#17573=PLANE('',#82666);
#17574=PLANE('',#82669);
#17575=PLANE('',#82672);
#17576=PLANE('',#82674);
#17577=PLANE('',#82677);
#17578=PLANE('',#82679);
#17579=PLANE('',#82682);
#17580=PLANE('',#82685);
#17581=PLANE('',#82687);
#17582=PLANE('',#82690);
#17583=PLANE('',#82692);
#17584=PLANE('',#82695);
#17585=PLANE('',#82697);
#17586=PLANE('',#82699);
#17587=PLANE('',#82702);
#17588=PLANE('',#82704);
#17589=PLANE('',#82707);
#17590=PLANE('',#82709);
#17591=PLANE('',#82711);
#17592=PLANE('',#82714);
#17593=PLANE('',#82716);
#17594=PLANE('',#82719);
#17595=PLANE('',#82722);
#17596=PLANE('',#82724);
#17597=PLANE('',#82727);
#17598=PLANE('',#82729);
#17599=PLANE('',#82732);
#17600=PLANE('',#82735);
#17601=PLANE('',#82737);
#17602=PLANE('',#82740);
#17603=PLANE('',#82742);
#17604=PLANE('',#82745);
#17605=PLANE('',#82748);
#17606=PLANE('',#82750);
#17607=PLANE('',#82753);
#17608=PLANE('',#82755);
#17609=PLANE('',#82758);
#17610=PLANE('',#82761);
#17611=PLANE('',#82764);
#17612=PLANE('',#82767);
#17613=PLANE('',#82770);
#17614=PLANE('',#82773);
#17615=PLANE('',#82776);
#17616=PLANE('',#82779);
#17617=PLANE('',#82782);
#17618=PLANE('',#82785);
#17619=PLANE('',#82788);
#17620=PLANE('',#82791);
#17621=PLANE('',#82794);
#17622=PLANE('',#82797);
#17623=PLANE('',#82800);
#17624=PLANE('',#82803);
#17625=PLANE('',#82806);
#17626=PLANE('',#82809);
#17627=PLANE('',#82812);
#17628=PLANE('',#82815);
#17629=PLANE('',#82818);
#17630=PLANE('',#82821);
#17631=PLANE('',#82824);
#17632=PLANE('',#82827);
#17633=PLANE('',#82830);
#17634=PLANE('',#82833);
#17635=PLANE('',#82836);
#17636=PLANE('',#82839);
#17637=PLANE('',#82842);
#17638=PLANE('',#82845);
#17639=PLANE('',#82848);
#17640=PLANE('',#82851);
#17641=PLANE('',#82854);
#17642=PLANE('',#82856);
#17643=PLANE('',#82858);
#17644=PLANE('',#82861);
#17645=PLANE('',#82863);
#17646=PLANE('',#82866);
#17647=PLANE('',#82868);
#17648=PLANE('',#82870);
#17649=PLANE('',#82873);
#17650=PLANE('',#82875);
#17651=PLANE('',#82878);
#17652=PLANE('',#82881);
#17653=PLANE('',#82884);
#17654=PLANE('',#82887);
#17655=PLANE('',#82890);
#17656=PLANE('',#82893);
#17657=PLANE('',#82896);
#17658=PLANE('',#82899);
#17659=PLANE('',#82902);
#17660=PLANE('',#82905);
#17661=PLANE('',#82908);
#17662=PLANE('',#82911);
#17663=PLANE('',#82914);
#17664=PLANE('',#82917);
#17665=PLANE('',#82920);
#17666=PLANE('',#82923);
#17667=PLANE('',#82926);
#17668=PLANE('',#82929);
#17669=PLANE('',#82932);
#17670=PLANE('',#82935);
#17671=PLANE('',#82937);
#17672=PLANE('',#82940);
#17673=PLANE('',#82943);
#17674=PLANE('',#82945);
#17675=PLANE('',#82948);
#17676=PLANE('',#82950);
#17677=PLANE('',#82953);
#17678=PLANE('',#82956);
#17679=PLANE('',#82958);
#17680=PLANE('',#82961);
#17681=PLANE('',#82963);
#17682=PLANE('',#82966);
#17683=PLANE('',#82969);
#17684=PLANE('',#82972);
#17685=PLANE('',#82975);
#17686=PLANE('',#82977);
#17687=PLANE('',#82980);
#17688=PLANE('',#82983);
#17689=PLANE('',#82986);
#17690=PLANE('',#82989);
#17691=PLANE('',#82992);
#17692=PLANE('',#82995);
#17693=PLANE('',#82998);
#17694=PLANE('',#83001);
#17695=PLANE('',#83004);
#17696=PLANE('',#83007);
#17697=PLANE('',#83010);
#17698=PLANE('',#83013);
#17699=PLANE('',#83016);
#17700=PLANE('',#83019);
#17701=PLANE('',#83022);
#17702=PLANE('',#83025);
#17703=PLANE('',#83028);
#17704=PLANE('',#83031);
#17705=PLANE('',#83034);
#17706=PLANE('',#83037);
#17707=PLANE('',#83040);
#17708=PLANE('',#83043);
#17709=PLANE('',#83046);
#17710=PLANE('',#83049);
#17711=PLANE('',#83052);
#17712=PLANE('',#83055);
#17713=PLANE('',#83058);
#17714=PLANE('',#83061);
#17715=PLANE('',#83064);
#17716=PLANE('',#83067);
#17717=PLANE('',#83070);
#17718=PLANE('',#83073);
#17719=PLANE('',#83076);
#17720=PLANE('',#83079);
#17721=PLANE('',#83082);
#17722=PLANE('',#83085);
#17723=PLANE('',#83088);
#17724=PLANE('',#83091);
#17725=PLANE('',#83094);
#17726=PLANE('',#83097);
#17727=PLANE('',#83100);
#17728=PLANE('',#83103);
#17729=PLANE('',#83106);
#17730=PLANE('',#83109);
#17731=PLANE('',#83111);
#17732=PLANE('',#83114);
#17733=PLANE('',#83117);
#17734=PLANE('',#83120);
#17735=PLANE('',#83123);
#17736=PLANE('',#83125);
#17737=PLANE('',#83128);
#17738=PLANE('',#83131);
#17739=PLANE('',#83134);
#17740=PLANE('',#83137);
#17741=PLANE('',#83140);
#17742=PLANE('',#83143);
#17743=PLANE('',#83146);
#17744=PLANE('',#83149);
#17745=PLANE('',#83152);
#17746=PLANE('',#83155);
#17747=PLANE('',#83158);
#17748=PLANE('',#83161);
#17749=PLANE('',#83164);
#17750=PLANE('',#83167);
#17751=PLANE('',#83170);
#17752=PLANE('',#83173);
#17753=PLANE('',#83176);
#17754=PLANE('',#83179);
#17755=PLANE('',#83182);
#17756=PLANE('',#83185);
#17757=PLANE('',#83188);
#17758=PLANE('',#83191);
#17759=PLANE('',#83194);
#17760=PLANE('',#83197);
#17761=PLANE('',#83200);
#17762=PLANE('',#83203);
#17763=PLANE('',#83206);
#17764=PLANE('',#83209);
#17765=PLANE('',#83212);
#17766=PLANE('',#83215);
#17767=PLANE('',#83218);
#17768=PLANE('',#83221);
#17769=PLANE('',#83224);
#17770=PLANE('',#83227);
#17771=PLANE('',#83230);
#17772=PLANE('',#83233);
#17773=PLANE('',#83236);
#17774=PLANE('',#83239);
#17775=PLANE('',#83241);
#17776=PLANE('',#83244);
#17777=PLANE('',#83246);
#17778=PLANE('',#83249);
#17779=PLANE('',#83252);
#17780=PLANE('',#83255);
#17781=PLANE('',#83258);
#17782=PLANE('',#83260);
#17783=PLANE('',#83263);
#17784=PLANE('',#83266);
#17785=PLANE('',#83269);
#17786=PLANE('',#83272);
#17787=PLANE('',#83275);
#17788=PLANE('',#83278);
#17789=PLANE('',#83281);
#17790=PLANE('',#83284);
#17791=PLANE('',#83287);
#17792=PLANE('',#83290);
#17793=PLANE('',#83293);
#17794=PLANE('',#83296);
#17795=PLANE('',#83299);
#17796=PLANE('',#83302);
#17797=PLANE('',#83305);
#17798=PLANE('',#83308);
#17799=PLANE('',#83311);
#17800=PLANE('',#83314);
#17801=PLANE('',#83317);
#17802=PLANE('',#83320);
#17803=PLANE('',#83323);
#17804=PLANE('',#83326);
#17805=PLANE('',#83329);
#17806=PLANE('',#83332);
#17807=PLANE('',#83335);
#17808=PLANE('',#83338);
#17809=PLANE('',#83341);
#17810=PLANE('',#83344);
#17811=PLANE('',#83347);
#17812=PLANE('',#83350);
#17813=PLANE('',#83353);
#17814=PLANE('',#83356);
#17815=PLANE('',#83359);
#17816=PLANE('',#83362);
#17817=PLANE('',#83365);
#17818=PLANE('',#83368);
#17819=PLANE('',#83371);
#17820=PLANE('',#83374);
#17821=PLANE('',#83377);
#17822=PLANE('',#83380);
#17823=PLANE('',#83383);
#17824=PLANE('',#83386);
#17825=PLANE('',#83389);
#17826=PLANE('',#83392);
#17827=PLANE('',#83395);
#17828=PLANE('',#83398);
#17829=PLANE('',#83401);
#17830=PLANE('',#83404);
#17831=PLANE('',#83407);
#17832=PLANE('',#83410);
#17833=PLANE('',#83413);
#17834=PLANE('',#83416);
#17835=PLANE('',#83419);
#17836=PLANE('',#83422);
#17837=PLANE('',#83425);
#17838=PLANE('',#83428);
#17839=PLANE('',#83431);
#17840=PLANE('',#83434);
#17841=PLANE('',#83437);
#17842=PLANE('',#83440);
#17843=PLANE('',#83443);
#17844=PLANE('',#83446);
#17845=PLANE('',#83449);
#17846=PLANE('',#83452);
#17847=PLANE('',#83455);
#17848=PLANE('',#83458);
#17849=PLANE('',#83461);
#17850=PLANE('',#83464);
#17851=PLANE('',#83467);
#17852=PLANE('',#83470);
#17853=PLANE('',#83473);
#17854=PLANE('',#83476);
#17855=PLANE('',#83479);
#17856=PLANE('',#83482);
#17857=PLANE('',#83485);
#17858=PLANE('',#83488);
#17859=PLANE('',#83491);
#17860=PLANE('',#83494);
#17861=PLANE('',#83497);
#17862=PLANE('',#83500);
#17863=PLANE('',#83503);
#17864=PLANE('',#83506);
#17865=PLANE('',#83509);
#17866=PLANE('',#83512);
#17867=PLANE('',#83515);
#17868=PLANE('',#83518);
#17869=PLANE('',#83521);
#17870=PLANE('',#83524);
#17871=PLANE('',#83527);
#17872=PLANE('',#83530);
#17873=PLANE('',#83533);
#17874=PLANE('',#83536);
#17875=PLANE('',#83539);
#17876=PLANE('',#83542);
#17877=PLANE('',#83545);
#17878=PLANE('',#83548);
#17879=PLANE('',#83551);
#17880=PLANE('',#83554);
#17881=PLANE('',#83557);
#17882=PLANE('',#83560);
#17883=PLANE('',#83563);
#17884=PLANE('',#83566);
#17885=PLANE('',#83569);
#17886=PLANE('',#83572);
#17887=PLANE('',#83575);
#17888=PLANE('',#83578);
#17889=PLANE('',#83581);
#17890=PLANE('',#83584);
#17891=PLANE('',#83587);
#17892=PLANE('',#83590);
#17893=PLANE('',#83593);
#17894=PLANE('',#83596);
#17895=PLANE('',#83599);
#17896=PLANE('',#83602);
#17897=PLANE('',#83605);
#17898=PLANE('',#83608);
#17899=PLANE('',#83611);
#17900=PLANE('',#83614);
#17901=PLANE('',#83617);
#17902=PLANE('',#83620);
#17903=PLANE('',#83623);
#17904=PLANE('',#83626);
#17905=PLANE('',#83629);
#17906=PLANE('',#83632);
#17907=PLANE('',#83635);
#17908=PLANE('',#83638);
#17909=PLANE('',#83641);
#17910=PLANE('',#83644);
#17911=PLANE('',#83647);
#17912=PLANE('',#83650);
#17913=PLANE('',#83653);
#17914=PLANE('',#83656);
#17915=PLANE('',#83659);
#17916=PLANE('',#83662);
#17917=PLANE('',#83665);
#17918=PLANE('',#83668);
#17919=PLANE('',#83671);
#17920=PLANE('',#83674);
#17921=PLANE('',#83677);
#17922=PLANE('',#83680);
#17923=PLANE('',#83683);
#17924=PLANE('',#83686);
#17925=PLANE('',#83689);
#17926=PLANE('',#83692);
#17927=PLANE('',#83695);
#17928=PLANE('',#83698);
#17929=PLANE('',#83701);
#17930=PLANE('',#83704);
#17931=PLANE('',#83707);
#17932=PLANE('',#83710);
#17933=PLANE('',#83713);
#17934=PLANE('',#83716);
#17935=PLANE('',#83719);
#17936=PLANE('',#83722);
#17937=PLANE('',#83725);
#17938=PLANE('',#83728);
#17939=PLANE('',#83731);
#17940=PLANE('',#83734);
#17941=PLANE('',#83737);
#17942=PLANE('',#83740);
#17943=PLANE('',#83743);
#17944=PLANE('',#83746);
#17945=PLANE('',#83749);
#17946=PLANE('',#83752);
#17947=PLANE('',#83755);
#17948=PLANE('',#83758);
#17949=PLANE('',#83761);
#17950=PLANE('',#83764);
#17951=PLANE('',#83767);
#17952=PLANE('',#83770);
#17953=PLANE('',#83773);
#17954=PLANE('',#83776);
#17955=PLANE('',#83779);
#17956=PLANE('',#83782);
#17957=PLANE('',#83785);
#17958=PLANE('',#83788);
#17959=PLANE('',#83791);
#17960=PLANE('',#83794);
#17961=PLANE('',#83797);
#17962=PLANE('',#83800);
#17963=PLANE('',#83803);
#17964=PLANE('',#83806);
#17965=PLANE('',#83809);
#17966=PLANE('',#83812);
#17967=PLANE('',#83815);
#17968=PLANE('',#83818);
#17969=PLANE('',#83821);
#17970=PLANE('',#83824);
#17971=PLANE('',#83827);
#17972=PLANE('',#83830);
#17973=PLANE('',#83833);
#17974=PLANE('',#83836);
#17975=PLANE('',#83839);
#17976=PLANE('',#83842);
#17977=PLANE('',#83845);
#17978=PLANE('',#83848);
#17979=PLANE('',#83851);
#17980=PLANE('',#83854);
#17981=PLANE('',#83857);
#17982=PLANE('',#83860);
#17983=PLANE('',#83863);
#17984=PLANE('',#83866);
#17985=PLANE('',#83869);
#17986=PLANE('',#83872);
#17987=PLANE('',#83875);
#17988=PLANE('',#83878);
#17989=PLANE('',#83881);
#17990=PLANE('',#83884);
#17991=PLANE('',#83887);
#17992=PLANE('',#83890);
#17993=PLANE('',#83893);
#17994=PLANE('',#83896);
#17995=PLANE('',#83899);
#17996=PLANE('',#83902);
#17997=PLANE('',#83905);
#17998=PLANE('',#83908);
#17999=PLANE('',#83911);
#18000=PLANE('',#83914);
#18001=PLANE('',#83917);
#18002=PLANE('',#83920);
#18003=PLANE('',#83923);
#18004=PLANE('',#83926);
#18005=PLANE('',#83929);
#18006=PLANE('',#83932);
#18007=PLANE('',#83935);
#18008=PLANE('',#83938);
#18009=PLANE('',#83941);
#18010=PLANE('',#83944);
#18011=PLANE('',#83947);
#18012=PLANE('',#83950);
#18013=PLANE('',#83953);
#18014=PLANE('',#83956);
#18015=PLANE('',#83959);
#18016=PLANE('',#83962);
#18017=PLANE('',#83965);
#18018=PLANE('',#83968);
#18019=PLANE('',#83971);
#18020=PLANE('',#83974);
#18021=PLANE('',#83977);
#18022=PLANE('',#83980);
#18023=PLANE('',#83983);
#18024=PLANE('',#83986);
#18025=PLANE('',#83989);
#18026=PLANE('',#83992);
#18027=PLANE('',#83995);
#18028=PLANE('',#83998);
#18029=PLANE('',#84001);
#18030=PLANE('',#84004);
#18031=PLANE('',#84007);
#18032=PLANE('',#84010);
#18033=PLANE('',#84013);
#18034=PLANE('',#84016);
#18035=PLANE('',#84019);
#18036=PLANE('',#84022);
#18037=PLANE('',#84025);
#18038=PLANE('',#84028);
#18039=PLANE('',#84031);
#18040=PLANE('',#84034);
#18041=PLANE('',#84037);
#18042=PLANE('',#84040);
#18043=PLANE('',#84043);
#18044=PLANE('',#84046);
#18045=PLANE('',#84049);
#18046=PLANE('',#84052);
#18047=PLANE('',#84055);
#18048=PLANE('',#84058);
#18049=PLANE('',#84061);
#18050=PLANE('',#84064);
#18051=PLANE('',#84067);
#18052=PLANE('',#84070);
#18053=PLANE('',#84073);
#18054=PLANE('',#84076);
#18055=PLANE('',#84079);
#18056=PLANE('',#84082);
#18057=PLANE('',#84085);
#18058=PLANE('',#84088);
#18059=PLANE('',#84091);
#18060=PLANE('',#84094);
#18061=PLANE('',#84097);
#18062=PLANE('',#84100);
#18063=PLANE('',#84103);
#18064=PLANE('',#84106);
#18065=PLANE('',#84109);
#18066=PLANE('',#84112);
#18067=PLANE('',#84115);
#18068=PLANE('',#84118);
#18069=PLANE('',#84121);
#18070=PLANE('',#84124);
#18071=PLANE('',#84127);
#18072=PLANE('',#84130);
#18073=PLANE('',#84133);
#18074=PLANE('',#84136);
#18075=PLANE('',#84139);
#18076=PLANE('',#84142);
#18077=PLANE('',#84145);
#18078=PLANE('',#84148);
#18079=PLANE('',#84151);
#18080=PLANE('',#84154);
#18081=PLANE('',#84157);
#18082=PLANE('',#84160);
#18083=PLANE('',#84163);
#18084=PLANE('',#84166);
#18085=PLANE('',#84169);
#18086=PLANE('',#84172);
#18087=PLANE('',#84175);
#18088=PLANE('',#84178);
#18089=PLANE('',#84181);
#18090=PLANE('',#84184);
#18091=PLANE('',#84185);
#18092=PLANE('',#84186);
#18093=PLANE('',#84187);
#18094=PLANE('',#84188);
#18095=PLANE('',#84189);
#18096=PLANE('',#84190);
#18097=PLANE('',#84191);
#18098=PLANE('',#84192);
#18099=PLANE('',#84193);
#18100=PLANE('',#84194);
#18101=PLANE('',#84195);
#18102=PLANE('',#84196);
#18103=PLANE('',#84197);
#18104=PLANE('',#84198);
#18105=PLANE('',#84199);
#18106=PLANE('',#84200);
#18107=PLANE('',#84201);
#18108=PLANE('',#84202);
#18109=PLANE('',#84203);
#18110=PLANE('',#84204);
#18111=PLANE('',#84205);
#18112=PLANE('',#84206);
#18113=PLANE('',#84207);
#18114=PLANE('',#84208);
#18115=PLANE('',#84209);
#18116=PLANE('',#84210);
#18117=PLANE('',#84211);
#18118=PLANE('',#84212);
#18119=PLANE('',#84213);
#18120=PLANE('',#84214);
#18121=PLANE('',#84215);
#18122=PLANE('',#84216);
#18123=PLANE('',#84217);
#18124=PLANE('',#84218);
#18125=PLANE('',#84219);
#18126=PLANE('',#84220);
#18127=PLANE('',#84221);
#18128=PLANE('',#84222);
#18129=PLANE('',#84223);
#18130=PLANE('',#84224);
#18131=PLANE('',#84225);
#18132=PLANE('',#84226);
#18133=PLANE('',#84227);
#18134=PLANE('',#84228);
#18135=PLANE('',#84229);
#18136=PLANE('',#84230);
#18137=PLANE('',#84231);
#18138=PLANE('',#84232);
#18139=PLANE('',#84233);
#18140=PLANE('',#84234);
#18141=PLANE('',#84235);
#18142=PLANE('',#84236);
#18143=PLANE('',#84237);
#18144=PLANE('',#84238);
#18145=PLANE('',#84239);
#18146=PLANE('',#84240);
#18147=PLANE('',#84241);
#18148=PLANE('',#84242);
#18149=PLANE('',#84243);
#18150=PLANE('',#84244);
#18151=PLANE('',#84245);
#18152=PLANE('',#84246);
#18153=PLANE('',#84247);
#18154=PLANE('',#84248);
#18155=PLANE('',#84249);
#18156=PLANE('',#84250);
#18157=PLANE('',#84251);
#18158=PLANE('',#84252);
#18159=PLANE('',#84253);
#18160=PLANE('',#84254);
#18161=PLANE('',#84255);
#18162=PLANE('',#84256);
#18163=PLANE('',#84257);
#18164=PLANE('',#84258);
#18165=PLANE('',#84259);
#18166=PLANE('',#84260);
#18167=PLANE('',#84261);
#18168=PLANE('',#84262);
#18169=PLANE('',#84263);
#18170=PLANE('',#84264);
#18171=PLANE('',#84265);
#18172=PLANE('',#84266);
#18173=PLANE('',#84267);
#18174=PLANE('',#84268);
#18175=PLANE('',#84269);
#18176=PLANE('',#84270);
#18177=PLANE('',#84271);
#18178=PLANE('',#84272);
#18179=PLANE('',#84273);
#18180=PLANE('',#84274);
#18181=PLANE('',#84275);
#18182=PLANE('',#84276);
#18183=PLANE('',#84277);
#18184=PLANE('',#84278);
#18185=PLANE('',#84279);
#18186=PLANE('',#84280);
#18187=PLANE('',#84281);
#18188=PLANE('',#84282);
#18189=PLANE('',#84283);
#18190=PLANE('',#84284);
#18191=PLANE('',#84285);
#18192=PLANE('',#84286);
#18193=PLANE('',#84287);
#18194=PLANE('',#84288);
#18195=PLANE('',#84289);
#18196=PLANE('',#84290);
#18197=PLANE('',#84291);
#18198=PLANE('',#84292);
#18199=PLANE('',#84293);
#18200=PLANE('',#84294);
#18201=PLANE('',#84295);
#18202=PLANE('',#84296);
#18203=PLANE('',#84297);
#18204=PLANE('',#84298);
#18205=PLANE('',#84299);
#18206=PLANE('',#84300);
#18207=PLANE('',#84301);
#18208=PLANE('',#84302);
#18209=PLANE('',#84303);
#18210=PLANE('',#84304);
#18211=PLANE('',#84305);
#18212=PLANE('',#84306);
#18213=PLANE('',#84307);
#18214=PLANE('',#84308);
#18215=PLANE('',#84309);
#18216=PLANE('',#84310);
#18217=PLANE('',#84311);
#18218=PLANE('',#84312);
#18219=PLANE('',#84313);
#18220=PLANE('',#84314);
#18221=PLANE('',#84315);
#18222=PLANE('',#84316);
#18223=PLANE('',#84317);
#18224=PLANE('',#84318);
#18225=PLANE('',#84319);
#18226=PLANE('',#84320);
#18227=PLANE('',#84321);
#18228=PLANE('',#84322);
#18229=PLANE('',#84323);
#18230=PLANE('',#84324);
#18231=PLANE('',#84325);
#18232=PLANE('',#84326);
#18233=PLANE('',#84327);
#18234=PLANE('',#84328);
#18235=PLANE('',#84329);
#18236=PLANE('',#84330);
#18237=PLANE('',#84331);
#18238=PLANE('',#84332);
#18239=PLANE('',#84333);
#18240=PLANE('',#84334);
#18241=PLANE('',#84335);
#18242=PLANE('',#84336);
#18243=PLANE('',#84337);
#18244=PLANE('',#84338);
#18245=PLANE('',#84339);
#18246=PLANE('',#84340);
#18247=PLANE('',#84341);
#18248=PLANE('',#84342);
#18249=PLANE('',#84343);
#18250=PLANE('',#84344);
#18251=PLANE('',#84345);
#18252=PLANE('',#84346);
#18253=PLANE('',#84347);
#18254=PLANE('',#84348);
#18255=PLANE('',#84349);
#18256=PLANE('',#84350);
#18257=PLANE('',#84351);
#18258=PLANE('',#84352);
#18259=PLANE('',#84353);
#18260=PLANE('',#84354);
#18261=PLANE('',#84355);
#18262=PLANE('',#84356);
#18263=PLANE('',#84357);
#18264=PLANE('',#84358);
#18265=PLANE('',#84359);
#18266=PLANE('',#84360);
#18267=PLANE('',#84361);
#18268=PLANE('',#84362);
#18269=PLANE('',#84363);
#18270=PLANE('',#84364);
#18271=PLANE('',#84365);
#18272=PLANE('',#84366);
#18273=PLANE('',#84367);
#18274=PLANE('',#84368);
#18275=PLANE('',#84369);
#18276=PLANE('',#84370);
#18277=PLANE('',#84371);
#18278=PLANE('',#84372);
#18279=PLANE('',#84373);
#18280=PLANE('',#84374);
#18281=PLANE('',#84375);
#18282=PLANE('',#84376);
#18283=PLANE('',#84377);
#18284=PLANE('',#84378);
#18285=PLANE('',#84379);
#18286=PLANE('',#84380);
#18287=PLANE('',#84381);
#18288=PLANE('',#84382);
#18289=PLANE('',#84383);
#18290=PLANE('',#84384);
#18291=PLANE('',#84385);
#18292=PLANE('',#84386);
#18293=PLANE('',#84387);
#18294=PLANE('',#84388);
#18295=PLANE('',#84389);
#18296=PLANE('',#84390);
#18297=PLANE('',#84391);
#18298=PLANE('',#84392);
#18299=PLANE('',#84393);
#18300=PLANE('',#84394);
#18301=PLANE('',#84395);
#18302=PLANE('',#84396);
#18303=PLANE('',#84397);
#18304=PLANE('',#84398);
#18305=PLANE('',#84399);
#18306=PLANE('',#84400);
#18307=PLANE('',#84401);
#18308=PLANE('',#84402);
#18309=PLANE('',#84403);
#18310=PLANE('',#84404);
#18311=PLANE('',#84405);
#18312=PLANE('',#84406);
#18313=PLANE('',#84407);
#18314=PLANE('',#84408);
#18315=PLANE('',#84409);
#18316=PLANE('',#84410);
#18317=PLANE('',#84411);
#18318=PLANE('',#84412);
#18319=PLANE('',#84413);
#18320=PLANE('',#84414);
#18321=PLANE('',#84415);
#18322=PLANE('',#84416);
#18323=PLANE('',#84417);
#18324=PLANE('',#84418);
#18325=PLANE('',#84419);
#18326=PLANE('',#84420);
#18327=PLANE('',#84421);
#18328=PLANE('',#84422);
#18329=PLANE('',#84423);
#18330=PLANE('',#84424);
#18331=PLANE('',#84425);
#18332=PLANE('',#84426);
#18333=PLANE('',#84427);
#18334=PLANE('',#84428);
#18335=PLANE('',#84429);
#18336=PLANE('',#84430);
#18337=PLANE('',#84431);
#18338=PLANE('',#84432);
#18339=PLANE('',#84433);
#18340=PLANE('',#84434);
#18341=PLANE('',#84435);
#18342=PLANE('',#84436);
#18343=PLANE('',#84437);
#18344=PLANE('',#84438);
#18345=PLANE('',#84439);
#18346=PLANE('',#84440);
#18347=PLANE('',#84441);
#18348=PLANE('',#84442);
#18349=PLANE('',#84443);
#18350=PLANE('',#84444);
#18351=PLANE('',#84445);
#18352=PLANE('',#84446);
#18353=PLANE('',#84447);
#18354=PLANE('',#84448);
#18355=PLANE('',#84449);
#18356=PLANE('',#84450);
#18357=PLANE('',#84451);
#18358=PLANE('',#84452);
#18359=PLANE('',#84453);
#18360=PLANE('',#84454);
#18361=PLANE('',#84455);
#18362=PLANE('',#84456);
#18363=PLANE('',#84457);
#18364=PLANE('',#84458);
#18365=PLANE('',#84459);
#18366=PLANE('',#84460);
#18367=PLANE('',#84461);
#18368=PLANE('',#84462);
#18369=PLANE('',#84463);
#18370=PLANE('',#84464);
#18371=PLANE('',#84465);
#18372=PLANE('',#84466);
#18373=PLANE('',#84467);
#18374=PLANE('',#84468);
#18375=PLANE('',#84469);
#18376=PLANE('',#84470);
#18377=PLANE('',#84471);
#18378=PLANE('',#84472);
#18379=PLANE('',#84473);
#18380=PLANE('',#84474);
#18381=PLANE('',#84475);
#18382=PLANE('',#84476);
#18383=PLANE('',#84477);
#18384=PLANE('',#84478);
#18385=PLANE('',#84479);
#18386=PLANE('',#84480);
#18387=PLANE('',#84481);
#18388=PLANE('',#84482);
#18389=PLANE('',#84483);
#18390=PLANE('',#84484);
#18391=PLANE('',#84485);
#18392=PLANE('',#84486);
#18393=PLANE('',#84487);
#18394=PLANE('',#84488);
#18395=PLANE('',#84489);
#18396=PLANE('',#84490);
#18397=PLANE('',#84491);
#18398=PLANE('',#84492);
#18399=PLANE('',#84493);
#18400=PLANE('',#84494);
#18401=PLANE('',#84495);
#18402=PLANE('',#84496);
#18403=PLANE('',#84497);
#18404=PLANE('',#84498);
#18405=PLANE('',#84499);
#18406=PLANE('',#84500);
#18407=PLANE('',#84501);
#18408=PLANE('',#84502);
#18409=PLANE('',#84503);
#18410=PLANE('',#84504);
#18411=PLANE('',#84505);
#18412=PLANE('',#84506);
#18413=PLANE('',#84507);
#18414=PLANE('',#84508);
#18415=PLANE('',#84509);
#18416=PLANE('',#84510);
#18417=PLANE('',#84511);
#18418=PLANE('',#84512);
#18419=PLANE('',#84513);
#18420=PLANE('',#84514);
#18421=PLANE('',#84515);
#18422=PLANE('',#84516);
#18423=PLANE('',#84517);
#18424=PLANE('',#84518);
#18425=PLANE('',#84519);
#18426=PLANE('',#84520);
#18427=PLANE('',#84521);
#18428=PLANE('',#84522);
#18429=PLANE('',#84523);
#18430=PLANE('',#84524);
#18431=PLANE('',#84525);
#18432=PLANE('',#84526);
#18433=PLANE('',#84527);
#18434=PLANE('',#84528);
#18435=PLANE('',#84529);
#18436=PLANE('',#84530);
#18437=PLANE('',#84531);
#18438=PLANE('',#84532);
#18439=PLANE('',#84533);
#18440=PLANE('',#84534);
#18441=PLANE('',#84535);
#18442=PLANE('',#84536);
#18443=PLANE('',#84537);
#18444=PLANE('',#84538);
#18445=PLANE('',#84539);
#18446=PLANE('',#84540);
#18447=PLANE('',#84541);
#18448=PLANE('',#84542);
#18449=PLANE('',#84543);
#18450=PLANE('',#84544);
#18451=PLANE('',#84545);
#18452=PLANE('',#84546);
#18453=PLANE('',#84547);
#18454=PLANE('',#84548);
#18455=PLANE('',#84549);
#18456=PLANE('',#84550);
#18457=PLANE('',#84551);
#18458=PLANE('',#84552);
#18459=PLANE('',#84553);
#18460=PLANE('',#84554);
#18461=PLANE('',#84555);
#18462=PLANE('',#84556);
#18463=PLANE('',#84557);
#18464=PLANE('',#84558);
#18465=PLANE('',#84559);
#18466=PLANE('',#84560);
#18467=PLANE('',#84561);
#18468=PLANE('',#84562);
#18469=PLANE('',#84563);
#18470=PLANE('',#84564);
#18471=PLANE('',#84565);
#18472=PLANE('',#84566);
#18473=PLANE('',#84567);
#18474=PLANE('',#84568);
#18475=PLANE('',#84569);
#18476=PLANE('',#84570);
#18477=PLANE('',#84571);
#18478=PLANE('',#84572);
#18479=PLANE('',#84573);
#18480=PLANE('',#84574);
#18481=PLANE('',#84575);
#18482=PLANE('',#84576);
#18483=PLANE('',#84577);
#18484=PLANE('',#84578);
#18485=PLANE('',#84579);
#18486=PLANE('',#84580);
#18487=PLANE('',#84581);
#18488=PLANE('',#84582);
#18489=PLANE('',#84583);
#18490=PLANE('',#84584);
#18491=PLANE('',#84585);
#18492=PLANE('',#84586);
#18493=PLANE('',#84587);
#18494=PLANE('',#84588);
#18495=PLANE('',#84589);
#18496=PLANE('',#84590);
#18497=PLANE('',#84591);
#18498=PLANE('',#84592);
#18499=PLANE('',#84593);
#18500=PLANE('',#84594);
#18501=PLANE('',#84595);
#18502=PLANE('',#84596);
#18503=PLANE('',#84597);
#18504=PLANE('',#84598);
#18505=PLANE('',#84599);
#18506=PLANE('',#84600);
#18507=PLANE('',#84601);
#18508=PLANE('',#84602);
#18509=PLANE('',#84603);
#18510=PLANE('',#84604);
#18511=PLANE('',#84605);
#18512=PLANE('',#84606);
#18513=PLANE('',#84607);
#18514=PLANE('',#84608);
#18515=PLANE('',#84609);
#18516=PLANE('',#84610);
#18517=PLANE('',#84611);
#18518=PLANE('',#84612);
#18519=PLANE('',#84613);
#18520=PLANE('',#84614);
#18521=PLANE('',#84615);
#18522=PLANE('',#84616);
#18523=PLANE('',#84617);
#18524=PLANE('',#84618);
#18525=PLANE('',#84619);
#18526=PLANE('',#84620);
#18527=PLANE('',#84621);
#18528=PLANE('',#84622);
#18529=PLANE('',#84623);
#18530=PLANE('',#84624);
#18531=PLANE('',#84625);
#18532=PLANE('',#84626);
#18533=PLANE('',#84627);
#18534=PLANE('',#84628);
#18535=PLANE('',#84629);
#18536=PLANE('',#84630);
#18537=PLANE('',#84631);
#18538=PLANE('',#84632);
#18539=PLANE('',#84633);
#18540=PLANE('',#84634);
#18541=PLANE('',#84635);
#18542=PLANE('',#84636);
#18543=PLANE('',#84637);
#18544=PLANE('',#84638);
#18545=PLANE('',#84639);
#18546=PLANE('',#84640);
#18547=PLANE('',#84641);
#18548=PLANE('',#84642);
#18549=PLANE('',#84643);
#18550=PLANE('',#84644);
#18551=PLANE('',#84645);
#18552=PLANE('',#84646);
#18553=PLANE('',#84647);
#18554=PLANE('',#84648);
#18555=PLANE('',#84649);
#18556=PLANE('',#84650);
#18557=PLANE('',#84651);
#18558=PLANE('',#84652);
#18559=PLANE('',#84653);
#18560=PLANE('',#84654);
#18561=PLANE('',#84655);
#18562=PLANE('',#84656);
#18563=PLANE('',#84657);
#18564=PLANE('',#84658);
#18565=PLANE('',#84659);
#18566=PLANE('',#84660);
#18567=PLANE('',#84661);
#18568=PLANE('',#84662);
#18569=PLANE('',#84663);
#18570=PLANE('',#84664);
#18571=PLANE('',#84665);
#18572=PLANE('',#84666);
#18573=PLANE('',#84667);
#18574=PLANE('',#84668);
#18575=PLANE('',#84669);
#18576=PLANE('',#84670);
#18577=PLANE('',#84671);
#18578=PLANE('',#84672);
#18579=PLANE('',#84673);
#18580=PLANE('',#84674);
#18581=PLANE('',#84675);
#18582=PLANE('',#84676);
#18583=PLANE('',#84677);
#18584=PLANE('',#84678);
#18585=PLANE('',#84679);
#18586=PLANE('',#84680);
#18587=PLANE('',#84681);
#18588=PLANE('',#84682);
#18589=PLANE('',#84683);
#18590=PLANE('',#84684);
#18591=PLANE('',#84685);
#18592=PLANE('',#84686);
#18593=PLANE('',#84687);
#18594=PLANE('',#84688);
#18595=PLANE('',#84689);
#18596=PLANE('',#84690);
#18597=PLANE('',#84691);
#18598=PLANE('',#84692);
#18599=PLANE('',#84693);
#18600=PLANE('',#84694);
#18601=PLANE('',#84695);
#18602=PLANE('',#84696);
#18603=PLANE('',#84697);
#18604=PLANE('',#84698);
#18605=PLANE('',#84699);
#18606=PLANE('',#84700);
#18607=PLANE('',#84701);
#18608=PLANE('',#84702);
#18609=PLANE('',#84703);
#18610=PLANE('',#84704);
#18611=PLANE('',#84705);
#18612=PLANE('',#84706);
#18613=PLANE('',#84707);
#18614=PLANE('',#84708);
#18615=PLANE('',#84709);
#18616=PLANE('',#84710);
#18617=PLANE('',#84711);
#18618=PLANE('',#84712);
#18619=PLANE('',#84713);
#18620=PLANE('',#84714);
#18621=PLANE('',#84715);
#18622=PLANE('',#84716);
#18623=PLANE('',#84717);
#18624=PLANE('',#84718);
#18625=PLANE('',#84719);
#18626=PLANE('',#84720);
#18627=PLANE('',#84721);
#18628=PLANE('',#84722);
#18629=PLANE('',#84723);
#18630=PLANE('',#84724);
#18631=PLANE('',#84725);
#18632=PLANE('',#84726);
#18633=PLANE('',#84727);
#18634=PLANE('',#84728);
#18635=PLANE('',#84729);
#18636=PLANE('',#84730);
#18637=PLANE('',#84731);
#18638=PLANE('',#84732);
#18639=PLANE('',#84733);
#18640=PLANE('',#84734);
#18641=PLANE('',#84735);
#18642=PLANE('',#84736);
#18643=PLANE('',#84737);
#18644=PLANE('',#84738);
#18645=PLANE('',#84739);
#18646=PLANE('',#84740);
#18647=PLANE('',#84741);
#18648=PLANE('',#84742);
#18649=PLANE('',#84743);
#18650=PLANE('',#84744);
#18651=PLANE('',#84745);
#18652=PLANE('',#84746);
#18653=PLANE('',#84747);
#18654=PLANE('',#84748);
#18655=PLANE('',#84749);
#18656=PLANE('',#84750);
#18657=PLANE('',#84751);
#18658=PLANE('',#84752);
#18659=PLANE('',#84753);
#18660=PLANE('',#84754);
#18661=PLANE('',#84755);
#18662=PLANE('',#84756);
#18663=PLANE('',#84757);
#18664=PLANE('',#84758);
#18665=PLANE('',#84759);
#18666=PLANE('',#84760);
#18667=PLANE('',#84761);
#18668=PLANE('',#84762);
#18669=PLANE('',#84763);
#18670=PLANE('',#84764);
#18671=PLANE('',#84765);
#18672=PLANE('',#84766);
#18673=PLANE('',#84767);
#18674=PLANE('',#84768);
#18675=PLANE('',#84769);
#18676=PLANE('',#84770);
#18677=PLANE('',#84771);
#18678=PLANE('',#84772);
#18679=PLANE('',#84773);
#18680=PLANE('',#84774);
#18681=PLANE('',#84775);
#18682=PLANE('',#84776);
#18683=PLANE('',#84777);
#18684=PLANE('',#84778);
#18685=PLANE('',#84779);
#18686=PLANE('',#84780);
#18687=PLANE('',#84781);
#18688=PLANE('',#84782);
#18689=PLANE('',#84783);
#18690=PLANE('',#84784);
#18691=PLANE('',#84785);
#18692=PLANE('',#84786);
#18693=PLANE('',#84787);
#18694=PLANE('',#84788);
#18695=PLANE('',#84789);
#18696=PLANE('',#84790);
#18697=PLANE('',#84791);
#18698=PLANE('',#84792);
#18699=PLANE('',#84793);
#18700=PLANE('',#84794);
#18701=PLANE('',#84795);
#18702=PLANE('',#84796);
#18703=PLANE('',#84797);
#18704=PLANE('',#84798);
#18705=PLANE('',#84799);
#18706=PLANE('',#84800);
#18707=PLANE('',#84801);
#18708=PLANE('',#84802);
#18709=PLANE('',#84803);
#18710=PLANE('',#84804);
#18711=PLANE('',#84805);
#18712=PLANE('',#84806);
#18713=PLANE('',#84807);
#18714=PLANE('',#84808);
#18715=PLANE('',#84809);
#18716=PLANE('',#84810);
#18717=PLANE('',#84811);
#18718=PLANE('',#84812);
#18719=PLANE('',#84813);
#18720=PLANE('',#84814);
#18721=PLANE('',#84815);
#18722=PLANE('',#84816);
#18723=PLANE('',#84817);
#18724=PLANE('',#84818);
#18725=PLANE('',#84819);
#18726=PLANE('',#84820);
#18727=PLANE('',#84821);
#18728=PLANE('',#84822);
#18729=PLANE('',#84823);
#18730=PLANE('',#84824);
#18731=PLANE('',#84825);
#18732=PLANE('',#84826);
#18733=PLANE('',#84827);
#18734=PLANE('',#84828);
#18735=PLANE('',#84829);
#18736=PLANE('',#84830);
#18737=PLANE('',#84831);
#18738=PLANE('',#84832);
#18739=PLANE('',#84833);
#18740=PLANE('',#84834);
#18741=PLANE('',#84835);
#18742=PLANE('',#84836);
#18743=PLANE('',#84837);
#18744=PLANE('',#84838);
#18745=PLANE('',#84839);
#18746=PLANE('',#84840);
#18747=PLANE('',#84841);
#18748=PLANE('',#84842);
#18749=PLANE('',#84843);
#18750=PLANE('',#84844);
#18751=PLANE('',#84845);
#18752=PLANE('',#84846);
#18753=PLANE('',#84847);
#18754=PLANE('',#84848);
#18755=PLANE('',#84849);
#18756=PLANE('',#84850);
#18757=PLANE('',#84851);
#18758=PLANE('',#84852);
#18759=PLANE('',#84853);
#18760=PLANE('',#84854);
#18761=PLANE('',#84855);
#18762=PLANE('',#84856);
#18763=PLANE('',#84857);
#18764=PLANE('',#84858);
#18765=PLANE('',#84859);
#18766=PLANE('',#84860);
#18767=PLANE('',#84861);
#18768=PLANE('',#84862);
#18769=PLANE('',#84863);
#18770=PLANE('',#84864);
#18771=PLANE('',#84865);
#18772=PLANE('',#84866);
#18773=PLANE('',#84867);
#18774=PLANE('',#84868);
#18775=PLANE('',#84869);
#18776=PLANE('',#84870);
#18777=PLANE('',#84871);
#18778=PLANE('',#84872);
#18779=PLANE('',#84873);
#18780=PLANE('',#84874);
#18781=PLANE('',#84875);
#18782=PLANE('',#84876);
#18783=PLANE('',#84877);
#18784=PLANE('',#84878);
#18785=PLANE('',#84879);
#18786=PLANE('',#84880);
#18787=PLANE('',#84881);
#18788=PLANE('',#84882);
#18789=PLANE('',#84883);
#18790=PLANE('',#84884);
#18791=PLANE('',#84885);
#18792=PLANE('',#84886);
#18793=PLANE('',#84887);
#18794=PLANE('',#84888);
#18795=PLANE('',#84889);
#18796=PLANE('',#84890);
#18797=PLANE('',#84891);
#18798=PLANE('',#84892);
#18799=PLANE('',#84893);
#18800=PLANE('',#84894);
#18801=PLANE('',#84895);
#18802=PLANE('',#84896);
#18803=PLANE('',#84897);
#18804=PLANE('',#84898);
#18805=PLANE('',#84899);
#18806=PLANE('',#84900);
#18807=PLANE('',#84901);
#18808=PLANE('',#84902);
#18809=PLANE('',#84903);
#18810=PLANE('',#84904);
#18811=PLANE('',#84905);
#18812=PLANE('',#84906);
#18813=PLANE('',#84907);
#18814=PLANE('',#84908);
#18815=PLANE('',#84909);
#18816=PLANE('',#84910);
#18817=PLANE('',#84911);
#18818=PLANE('',#84912);
#18819=PLANE('',#84913);
#18820=PLANE('',#84914);
#18821=PLANE('',#84915);
#18822=PLANE('',#84916);
#18823=PLANE('',#84917);
#18824=PLANE('',#84918);
#18825=PLANE('',#84919);
#18826=PLANE('',#84920);
#18827=PLANE('',#84921);
#18828=PLANE('',#84922);
#18829=PLANE('',#84923);
#18830=PLANE('',#84924);
#18831=PLANE('',#84925);
#18832=PLANE('',#84926);
#18833=PLANE('',#84927);
#18834=PLANE('',#84928);
#18835=PLANE('',#84929);
#18836=PLANE('',#84930);
#18837=PLANE('',#84931);
#18838=PLANE('',#84932);
#18839=PLANE('',#84933);
#18840=PLANE('',#84934);
#18841=PLANE('',#84935);
#18842=PLANE('',#84936);
#18843=PLANE('',#84937);
#18844=PLANE('',#84938);
#18845=PLANE('',#84939);
#18846=PLANE('',#84940);
#18847=PLANE('',#84941);
#18848=PLANE('',#84942);
#18849=PLANE('',#84943);
#18850=PLANE('',#84944);
#18851=PLANE('',#84945);
#18852=PLANE('',#84946);
#18853=PLANE('',#84947);
#18854=PLANE('',#84948);
#18855=PLANE('',#84949);
#18856=PLANE('',#84950);
#18857=PLANE('',#84951);
#18858=PLANE('',#84952);
#18859=PLANE('',#84953);
#18860=PLANE('',#84954);
#18861=PLANE('',#84955);
#18862=PLANE('',#84956);
#18863=PLANE('',#84957);
#18864=PLANE('',#84958);
#18865=PLANE('',#84959);
#18866=PLANE('',#84960);
#18867=PLANE('',#84961);
#18868=PLANE('',#84962);
#18869=PLANE('',#84963);
#18870=PLANE('',#84964);
#18871=PLANE('',#84965);
#18872=PLANE('',#84966);
#18873=PLANE('',#84967);
#18874=PLANE('',#84968);
#18875=PLANE('',#84969);
#18876=PLANE('',#84970);
#18877=PLANE('',#84971);
#18878=PLANE('',#84972);
#18879=PLANE('',#84973);
#18880=PLANE('',#84974);
#18881=PLANE('',#84975);
#18882=PLANE('',#84976);
#18883=PLANE('',#84977);
#18884=PLANE('',#84978);
#18885=PLANE('',#84979);
#18886=PLANE('',#84980);
#18887=PLANE('',#84981);
#18888=PLANE('',#84982);
#18889=PLANE('',#84983);
#18890=PLANE('',#84984);
#18891=PLANE('',#84985);
#18892=PLANE('',#84986);
#18893=PLANE('',#84987);
#18894=PLANE('',#84988);
#18895=PLANE('',#84989);
#18896=PLANE('',#84990);
#18897=PLANE('',#84991);
#18898=PLANE('',#84992);
#18899=PLANE('',#84993);
#18900=PLANE('',#84994);
#18901=PLANE('',#84995);
#18902=PLANE('',#84996);
#18903=PLANE('',#84997);
#18904=PLANE('',#84998);
#18905=PLANE('',#84999);
#18906=PLANE('',#85000);
#18907=PLANE('',#85001);
#18908=PLANE('',#85002);
#18909=PLANE('',#85003);
#18910=PLANE('',#85004);
#18911=PLANE('',#85005);
#18912=PLANE('',#85006);
#18913=PLANE('',#85007);
#18914=PLANE('',#85008);
#18915=PLANE('',#85009);
#18916=PLANE('',#85010);
#18917=PLANE('',#85011);
#18918=PLANE('',#85012);
#18919=PLANE('',#85013);
#18920=PLANE('',#85014);
#18921=PLANE('',#85015);
#18922=PLANE('',#85016);
#18923=PLANE('',#85017);
#18924=PLANE('',#85018);
#18925=PLANE('',#85019);
#18926=PLANE('',#85020);
#18927=PLANE('',#85021);
#18928=PLANE('',#85022);
#18929=PLANE('',#85023);
#18930=PLANE('',#85024);
#18931=PLANE('',#85025);
#18932=PLANE('',#85026);
#18933=PLANE('',#85027);
#18934=PLANE('',#85028);
#18935=PLANE('',#85029);
#18936=PLANE('',#85030);
#18937=PLANE('',#85031);
#18938=PLANE('',#85032);
#18939=PLANE('',#85033);
#18940=PLANE('',#85034);
#18941=PLANE('',#85035);
#18942=PLANE('',#85036);
#18943=PLANE('',#85037);
#18944=PLANE('',#85038);
#18945=PLANE('',#85039);
#18946=PLANE('',#85040);
#18947=PLANE('',#85041);
#18948=PLANE('',#85042);
#18949=PLANE('',#85043);
#18950=PLANE('',#85044);
#18951=PLANE('',#85045);
#18952=PLANE('',#85046);
#18953=PLANE('',#85047);
#18954=PLANE('',#85048);
#18955=PLANE('',#85049);
#18956=PLANE('',#85050);
#18957=PLANE('',#85051);
#18958=PLANE('',#85052);
#18959=PLANE('',#85053);
#18960=PLANE('',#85054);
#18961=PLANE('',#85055);
#18962=PLANE('',#85056);
#18963=PLANE('',#85057);
#18964=PLANE('',#85058);
#18965=PLANE('',#85059);
#18966=PLANE('',#85060);
#18967=PLANE('',#85061);
#18968=PLANE('',#85062);
#18969=PLANE('',#85063);
#18970=PLANE('',#85064);
#18971=PLANE('',#85065);
#18972=PLANE('',#85066);
#18973=PLANE('',#85067);
#18974=PLANE('',#85068);
#18975=PLANE('',#85069);
#18976=PLANE('',#85070);
#18977=PLANE('',#85071);
#18978=PLANE('',#85072);
#18979=PLANE('',#85073);
#18980=PLANE('',#85074);
#18981=PLANE('',#85075);
#18982=PLANE('',#85076);
#18983=PLANE('',#85077);
#18984=PLANE('',#85078);
#18985=PLANE('',#85079);
#18986=PLANE('',#85080);
#18987=PLANE('',#85081);
#18988=PLANE('',#85082);
#18989=PLANE('',#85083);
#18990=PLANE('',#85084);
#18991=PLANE('',#85085);
#18992=PLANE('',#85086);
#18993=PLANE('',#85087);
#18994=PLANE('',#85088);
#18995=PLANE('',#85089);
#18996=PLANE('',#85090);
#18997=PLANE('',#85091);
#18998=PLANE('',#85092);
#18999=PLANE('',#85093);
#19000=PLANE('',#85094);
#19001=PLANE('',#85095);
#19002=PLANE('',#85096);
#19003=PLANE('',#85097);
#19004=PLANE('',#85098);
#19005=PLANE('',#85099);
#19006=PLANE('',#85100);
#19007=PLANE('',#85101);
#19008=PLANE('',#85102);
#19009=PLANE('',#85103);
#19010=PLANE('',#85104);
#19011=PLANE('',#85105);
#19012=PLANE('',#85106);
#19013=PLANE('',#85107);
#19014=PLANE('',#85108);
#19015=PLANE('',#85109);
#19016=PLANE('',#85110);
#19017=PLANE('',#85111);
#19018=PLANE('',#85112);
#19019=PLANE('',#85113);
#19020=PLANE('',#85114);
#19021=PLANE('',#85115);
#19022=PLANE('',#85116);
#19023=PLANE('',#85117);
#19024=PLANE('',#85118);
#19025=PLANE('',#85119);
#19026=PLANE('',#85120);
#19027=PLANE('',#85121);
#19028=PLANE('',#85122);
#19029=PLANE('',#85123);
#19030=PLANE('',#85124);
#19031=PLANE('',#85125);
#19032=PLANE('',#85126);
#19033=PLANE('',#85127);
#19034=PLANE('',#85128);
#19035=PLANE('',#85129);
#19036=PLANE('',#85130);
#19037=PLANE('',#85131);
#19038=PLANE('',#85132);
#19039=PLANE('',#85133);
#19040=PLANE('',#85134);
#19041=PLANE('',#85135);
#19042=PLANE('',#85136);
#19043=PLANE('',#85137);
#19044=PLANE('',#85138);
#19045=PLANE('',#85139);
#19046=PLANE('',#85140);
#19047=PLANE('',#85141);
#19048=PLANE('',#85142);
#19049=PLANE('',#85143);
#19050=PLANE('',#85144);
#19051=PLANE('',#85145);
#19052=PLANE('',#85146);
#19053=PLANE('',#85147);
#19054=PLANE('',#85148);
#19055=PLANE('',#85149);
#19056=PLANE('',#85150);
#19057=PLANE('',#85151);
#19058=PLANE('',#85152);
#19059=PLANE('',#85153);
#19060=PLANE('',#85154);
#19061=PLANE('',#85155);
#19062=PLANE('',#85156);
#19063=PLANE('',#85157);
#19064=PLANE('',#85158);
#19065=PLANE('',#85159);
#19066=PLANE('',#85160);
#19067=PLANE('',#85161);
#19068=PLANE('',#85162);
#19069=PLANE('',#85163);
#19070=PLANE('',#85164);
#19071=PLANE('',#85165);
#19072=PLANE('',#85166);
#19073=PLANE('',#85167);
#19074=PLANE('',#85168);
#19075=PLANE('',#85169);
#19076=PLANE('',#85170);
#19077=PLANE('',#85171);
#19078=PLANE('',#85172);
#19079=PLANE('',#85173);
#19080=PLANE('',#85174);
#19081=PLANE('',#85175);
#19082=PLANE('',#85176);
#19083=PLANE('',#85177);
#19084=PLANE('',#85178);
#19085=PLANE('',#85179);
#19086=PLANE('',#85180);
#19087=PLANE('',#85181);
#19088=PLANE('',#85182);
#19089=PLANE('',#85183);
#19090=PLANE('',#85184);
#19091=PLANE('',#85185);
#19092=PLANE('',#85186);
#19093=PLANE('',#85187);
#19094=PLANE('',#85188);
#19095=PLANE('',#85189);
#19096=PLANE('',#85190);
#19097=PLANE('',#85191);
#19098=PLANE('',#85192);
#19099=PLANE('',#85193);
#19100=PLANE('',#85194);
#19101=PLANE('',#85195);
#19102=PLANE('',#85196);
#19103=PLANE('',#85197);
#19104=PLANE('',#85198);
#19105=PLANE('',#85199);
#19106=PLANE('',#85200);
#19107=PLANE('',#85201);
#19108=PLANE('',#85202);
#19109=PLANE('',#85203);
#19110=PLANE('',#85204);
#19111=PLANE('',#85205);
#19112=PLANE('',#85206);
#19113=PLANE('',#85207);
#19114=PLANE('',#85208);
#19115=PLANE('',#85209);
#19116=PLANE('',#85210);
#19117=PLANE('',#85211);
#19118=PLANE('',#85212);
#19119=PLANE('',#85213);
#19120=PLANE('',#85214);
#19121=PLANE('',#85215);
#19122=PLANE('',#85216);
#19123=PLANE('',#85217);
#19124=PLANE('',#85218);
#19125=PLANE('',#85219);
#19126=PLANE('',#85220);
#19127=PLANE('',#85221);
#19128=PLANE('',#85222);
#19129=PLANE('',#85223);
#19130=PLANE('',#85224);
#19131=PLANE('',#85225);
#19132=PLANE('',#85226);
#19133=PLANE('',#85227);
#19134=PLANE('',#85228);
#19135=PLANE('',#85229);
#19136=PLANE('',#85230);
#19137=PLANE('',#85231);
#19138=PLANE('',#85232);
#19139=PLANE('',#85233);
#19140=PLANE('',#85234);
#19141=PLANE('',#85235);
#19142=PLANE('',#85236);
#19143=PLANE('',#85237);
#19144=PLANE('',#85238);
#19145=PLANE('',#85239);
#19146=PLANE('',#85240);
#19147=PLANE('',#85241);
#19148=PLANE('',#85242);
#19149=PLANE('',#85243);
#19150=PLANE('',#85244);
#19151=PLANE('',#85245);
#19152=PLANE('',#85246);
#19153=PLANE('',#85247);
#19154=PLANE('',#85248);
#19155=PLANE('',#85249);
#19156=PLANE('',#85250);
#19157=PLANE('',#85251);
#19158=PLANE('',#85252);
#19159=PLANE('',#85253);
#19160=PLANE('',#85254);
#19161=PLANE('',#85255);
#19162=PLANE('',#85256);
#19163=PLANE('',#85257);
#19164=PLANE('',#85258);
#19165=PLANE('',#85259);
#19166=PLANE('',#85260);
#19167=PLANE('',#85261);
#19168=PLANE('',#85262);
#19169=PLANE('',#85263);
#19170=PLANE('',#85264);
#19171=PLANE('',#85265);
#19172=PLANE('',#85266);
#19173=PLANE('',#85267);
#19174=PLANE('',#85268);
#19175=PLANE('',#85269);
#19176=PLANE('',#85270);
#19177=PLANE('',#85271);
#19178=PLANE('',#85272);
#19179=PLANE('',#85273);
#19180=PLANE('',#85274);
#19181=PLANE('',#85275);
#19182=PLANE('',#85276);
#19183=PLANE('',#85277);
#19184=PLANE('',#85278);
#19185=PLANE('',#85279);
#19186=PLANE('',#85280);
#19187=PLANE('',#85281);
#19188=PLANE('',#85282);
#19189=PLANE('',#85283);
#19190=PLANE('',#85284);
#19191=PLANE('',#85285);
#19192=PLANE('',#85286);
#19193=PLANE('',#85287);
#19194=PLANE('',#85288);
#19195=PLANE('',#85289);
#19196=PLANE('',#85290);
#19197=PLANE('',#85291);
#19198=PLANE('',#85292);
#19199=PLANE('',#85293);
#19200=PLANE('',#85294);
#19201=PLANE('',#85295);
#19202=PLANE('',#85296);
#19203=PLANE('',#85297);
#19204=PLANE('',#85298);
#19205=PLANE('',#85299);
#19206=PLANE('',#85300);
#19207=PLANE('',#85301);
#19208=PLANE('',#85302);
#19209=PLANE('',#85303);
#19210=PLANE('',#85304);
#19211=PLANE('',#85305);
#19212=PLANE('',#85306);
#19213=PLANE('',#85307);
#19214=PLANE('',#85308);
#19215=PLANE('',#85309);
#19216=PLANE('',#85310);
#19217=PLANE('',#85311);
#19218=PLANE('',#85312);
#19219=PLANE('',#85313);
#19220=PLANE('',#85314);
#19221=PLANE('',#85315);
#19222=PLANE('',#85316);
#19223=PLANE('',#85317);
#19224=PLANE('',#85318);
#19225=PLANE('',#85319);
#19226=PLANE('',#85320);
#19227=PLANE('',#85321);
#19228=PLANE('',#85322);
#19229=PLANE('',#85323);
#19230=PLANE('',#85324);
#19231=PLANE('',#85325);
#19232=PLANE('',#85326);
#19233=PLANE('',#85327);
#19234=PLANE('',#85328);
#19235=PLANE('',#85329);
#19236=PLANE('',#85330);
#19237=PLANE('',#85331);
#19238=PLANE('',#85332);
#19239=PLANE('',#85333);
#19240=PLANE('',#85334);
#19241=PLANE('',#85335);
#19242=PLANE('',#85336);
#19243=PLANE('',#85337);
#19244=PLANE('',#85338);
#19245=PLANE('',#85339);
#19246=PLANE('',#85340);
#19247=PLANE('',#85341);
#19248=PLANE('',#85342);
#19249=PLANE('',#85343);
#19250=PLANE('',#85344);
#19251=PLANE('',#85345);
#19252=PLANE('',#85346);
#19253=PLANE('',#85347);
#19254=PLANE('',#85348);
#19255=PLANE('',#85349);
#19256=PLANE('',#85350);
#19257=PLANE('',#85351);
#19258=PLANE('',#85352);
#19259=PLANE('',#85353);
#19260=PLANE('',#85354);
#19261=PLANE('',#85355);
#19262=PLANE('',#85356);
#19263=PLANE('',#85357);
#19264=PLANE('',#85358);
#19265=PLANE('',#85359);
#19266=PLANE('',#85360);
#19267=PLANE('',#85361);
#19268=PLANE('',#85362);
#19269=PLANE('',#85363);
#19270=PLANE('',#85364);
#19271=PLANE('',#85365);
#19272=PLANE('',#85366);
#19273=PLANE('',#85367);
#19274=PLANE('',#85368);
#19275=PLANE('',#85369);
#19276=PLANE('',#85370);
#19277=PLANE('',#85371);
#19278=PLANE('',#85372);
#19279=PLANE('',#85373);
#19280=PLANE('',#85374);
#19281=PLANE('',#85375);
#19282=PLANE('',#85376);
#19283=PLANE('',#85377);
#19284=PLANE('',#85378);
#19285=PLANE('',#85379);
#19286=PLANE('',#85380);
#19287=PLANE('',#85381);
#19288=PLANE('',#85382);
#19289=PLANE('',#85383);
#19290=PLANE('',#85384);
#19291=PLANE('',#85385);
#19292=PLANE('',#85386);
#19293=PLANE('',#85387);
#19294=PLANE('',#85388);
#19295=PLANE('',#85389);
#19296=PLANE('',#85390);
#19297=PLANE('',#85391);
#19298=PLANE('',#85392);
#19299=PLANE('',#85393);
#19300=PLANE('',#85394);
#19301=PLANE('',#85395);
#19302=PLANE('',#85396);
#19303=PLANE('',#85397);
#19304=PLANE('',#85398);
#19305=PLANE('',#85399);
#19306=PLANE('',#85400);
#19307=PLANE('',#85401);
#19308=PLANE('',#85402);
#19309=PLANE('',#85403);
#19310=PLANE('',#85404);
#19311=PLANE('',#85405);
#19312=PLANE('',#85406);
#19313=PLANE('',#85407);
#19314=PLANE('',#85408);
#19315=PLANE('',#85409);
#19316=PLANE('',#85410);
#19317=PLANE('',#85411);
#19318=PLANE('',#85412);
#19319=PLANE('',#85413);
#19320=PLANE('',#85414);
#19321=PLANE('',#85415);
#19322=PLANE('',#85416);
#19323=PLANE('',#85417);
#19324=PLANE('',#85418);
#19325=PLANE('',#85419);
#19326=PLANE('',#85420);
#19327=PLANE('',#85421);
#19328=PLANE('',#85422);
#19329=PLANE('',#85423);
#19330=PLANE('',#85424);
#19331=PLANE('',#85425);
#19332=PLANE('',#85426);
#19333=PLANE('',#85427);
#19334=PLANE('',#85428);
#19335=PLANE('',#85429);
#19336=PLANE('',#85430);
#19337=PLANE('',#85431);
#19338=PLANE('',#85432);
#19339=PLANE('',#85433);
#19340=PLANE('',#85434);
#19341=PLANE('',#85435);
#19342=PLANE('',#85436);
#19343=PLANE('',#85437);
#19344=PLANE('',#85438);
#19345=PLANE('',#85439);
#19346=PLANE('',#85440);
#19347=PLANE('',#85441);
#19348=PLANE('',#85442);
#19349=PLANE('',#85443);
#19350=PLANE('',#85444);
#19351=PLANE('',#85445);
#19352=PLANE('',#85446);
#19353=PLANE('',#85447);
#19354=PLANE('',#85448);
#19355=PLANE('',#85449);
#19356=PLANE('',#85450);
#19357=PLANE('',#85451);
#19358=PLANE('',#85452);
#19359=PLANE('',#85453);
#19360=PLANE('',#85454);
#19361=PLANE('',#85455);
#19362=PLANE('',#85456);
#19363=PLANE('',#85457);
#19364=PLANE('',#85458);
#19365=PLANE('',#85459);
#19366=PLANE('',#85460);
#19367=PLANE('',#85461);
#19368=PLANE('',#85462);
#19369=PLANE('',#85463);
#19370=PLANE('',#85464);
#19371=PLANE('',#85465);
#19372=PLANE('',#85466);
#19373=PLANE('',#85467);
#19374=PLANE('',#85468);
#19375=PLANE('',#85469);
#19376=PLANE('',#85470);
#19377=PLANE('',#85471);
#19378=PLANE('',#85472);
#19379=PLANE('',#85473);
#19380=PLANE('',#85474);
#19381=PLANE('',#85475);
#19382=PLANE('',#85476);
#19383=PLANE('',#85477);
#19384=PLANE('',#85478);
#19385=PLANE('',#85479);
#19386=PLANE('',#85480);
#19387=PLANE('',#85481);
#19388=PLANE('',#85482);
#19389=PLANE('',#85483);
#19390=PLANE('',#85484);
#19391=PLANE('',#85485);
#19392=PLANE('',#85486);
#19393=PLANE('',#85487);
#19394=PLANE('',#85488);
#19395=PLANE('',#85489);
#19396=PLANE('',#85490);
#19397=PLANE('',#85491);
#19398=PLANE('',#85492);
#19399=PLANE('',#85493);
#19400=PLANE('',#85494);
#19401=PLANE('',#85495);
#19402=PLANE('',#85496);
#19403=PLANE('',#85497);
#19404=PLANE('',#85498);
#19405=PLANE('',#85499);
#19406=PLANE('',#85500);
#19407=PLANE('',#85501);
#19408=PLANE('',#85502);
#19409=PLANE('',#85503);
#19410=PLANE('',#85504);
#19411=PLANE('',#85505);
#19412=PLANE('',#85506);
#19413=PLANE('',#85507);
#19414=PLANE('',#85508);
#19415=PLANE('',#85509);
#19416=PLANE('',#85510);
#19417=PLANE('',#85511);
#19418=PLANE('',#85512);
#19419=PLANE('',#85513);
#19420=PLANE('',#85514);
#19421=PLANE('',#85515);
#19422=PLANE('',#85516);
#19423=PLANE('',#85517);
#19424=PLANE('',#85518);
#19425=PLANE('',#85519);
#19426=PLANE('',#85520);
#19427=PLANE('',#85521);
#19428=PLANE('',#85522);
#19429=PLANE('',#85523);
#19430=PLANE('',#85524);
#19431=PLANE('',#85525);
#19432=PLANE('',#85526);
#19433=PLANE('',#85527);
#19434=PLANE('',#85528);
#19435=PLANE('',#85529);
#19436=PLANE('',#85530);
#19437=PLANE('',#85531);
#19438=PLANE('',#85532);
#19439=PLANE('',#85533);
#19440=PLANE('',#85534);
#19441=PLANE('',#85535);
#19442=PLANE('',#85536);
#19443=PLANE('',#85537);
#19444=PLANE('',#85538);
#19445=PLANE('',#85539);
#19446=PLANE('',#85540);
#19447=PLANE('',#85541);
#19448=PLANE('',#85542);
#19449=PLANE('',#85543);
#19450=PLANE('',#85544);
#19451=PLANE('',#85545);
#19452=PLANE('',#85546);
#19453=PLANE('',#85547);
#19454=PLANE('',#85548);
#19455=PLANE('',#85549);
#19456=PLANE('',#85550);
#19457=PLANE('',#85551);
#19458=PLANE('',#85552);
#19459=PLANE('',#85553);
#19460=PLANE('',#85554);
#19461=PLANE('',#85555);
#19462=PLANE('',#85556);
#19463=PLANE('',#85557);
#19464=PLANE('',#85558);
#19465=PLANE('',#85559);
#19466=PLANE('',#85560);
#19467=PLANE('',#85561);
#19468=PLANE('',#85562);
#19469=PLANE('',#85563);
#19470=PLANE('',#85564);
#19471=PLANE('',#85565);
#19472=PLANE('',#85566);
#19473=PLANE('',#85567);
#19474=PLANE('',#85568);
#19475=PLANE('',#85569);
#19476=PLANE('',#85570);
#19477=PLANE('',#85571);
#19478=PLANE('',#85572);
#19479=PLANE('',#85573);
#19480=PLANE('',#85574);
#19481=PLANE('',#85575);
#19482=PLANE('',#85576);
#19483=PLANE('',#85577);
#19484=PLANE('',#85578);
#19485=PLANE('',#85579);
#19486=PLANE('',#85580);
#19487=PLANE('',#85581);
#19488=PLANE('',#85582);
#19489=PLANE('',#85583);
#19490=PLANE('',#85584);
#19491=PLANE('',#85585);
#19492=PLANE('',#85586);
#19493=PLANE('',#85587);
#19494=PLANE('',#85588);
#19495=PLANE('',#85589);
#19496=PLANE('',#85590);
#19497=PLANE('',#85591);
#19498=PLANE('',#85592);
#19499=PLANE('',#85593);
#19500=PLANE('',#85594);
#19501=PLANE('',#85595);
#19502=PLANE('',#85596);
#19503=PLANE('',#85597);
#19504=PLANE('',#85598);
#19505=PLANE('',#85599);
#19506=PLANE('',#85600);
#19507=PLANE('',#85601);
#19508=PLANE('',#85602);
#19509=PLANE('',#85603);
#19510=PLANE('',#85604);
#19511=PLANE('',#85605);
#19512=PLANE('',#85606);
#19513=PLANE('',#85607);
#19514=PLANE('',#85608);
#19515=PLANE('',#85609);
#19516=PLANE('',#85610);
#19517=PLANE('',#85611);
#19518=PLANE('',#85612);
#19519=PLANE('',#85613);
#19520=PLANE('',#85614);
#19521=PLANE('',#85615);
#19522=PLANE('',#85616);
#19523=PLANE('',#85617);
#19524=PLANE('',#85618);
#19525=PLANE('',#85619);
#19526=PLANE('',#85620);
#19527=PLANE('',#85621);
#19528=PLANE('',#85622);
#19529=PLANE('',#85623);
#19530=PLANE('',#85624);
#19531=PLANE('',#85625);
#19532=PLANE('',#85626);
#19533=PLANE('',#85627);
#19534=PLANE('',#85628);
#19535=PLANE('',#85629);
#19536=PLANE('',#85630);
#19537=PLANE('',#85631);
#19538=PLANE('',#85632);
#19539=PLANE('',#85633);
#19540=PLANE('',#85634);
#19541=PLANE('',#85635);
#19542=PLANE('',#85636);
#19543=PLANE('',#85637);
#19544=PLANE('',#85638);
#19545=PLANE('',#85639);
#19546=PLANE('',#85640);
#19547=PLANE('',#85641);
#19548=PLANE('',#85642);
#19549=PLANE('',#85643);
#19550=PLANE('',#85644);
#19551=PLANE('',#85645);
#19552=PLANE('',#85646);
#19553=PLANE('',#85647);
#19554=PLANE('',#85648);
#19555=PLANE('',#85649);
#19556=PLANE('',#85650);
#19557=PLANE('',#85651);
#19558=PLANE('',#85652);
#19559=PLANE('',#85653);
#19560=PLANE('',#85654);
#19561=PLANE('',#85655);
#19562=PLANE('',#85656);
#19563=PLANE('',#85657);
#19564=PLANE('',#85658);
#19565=PLANE('',#85659);
#19566=PLANE('',#85660);
#19567=PLANE('',#85661);
#19568=PLANE('',#85662);
#19569=PLANE('',#85663);
#19570=PLANE('',#85664);
#19571=PLANE('',#85665);
#19572=PLANE('',#85666);
#19573=PLANE('',#85667);
#19574=PLANE('',#85668);
#19575=PLANE('',#85669);
#19576=PLANE('',#85670);
#19577=PLANE('',#85671);
#19578=PLANE('',#85672);
#19579=PLANE('',#85673);
#19580=PLANE('',#85674);
#19581=PLANE('',#85675);
#19582=PLANE('',#85676);
#19583=PLANE('',#85677);
#19584=PLANE('',#85678);
#19585=PLANE('',#85679);
#19586=PLANE('',#85680);
#19587=PLANE('',#85681);
#19588=PLANE('',#85682);
#19589=PLANE('',#85683);
#19590=PLANE('',#85684);
#19591=PLANE('',#85685);
#19592=PLANE('',#85686);
#19593=PLANE('',#85687);
#19594=PLANE('',#85688);
#19595=PLANE('',#85689);
#19596=PLANE('',#85690);
#19597=PLANE('',#85691);
#19598=PLANE('',#85692);
#19599=PLANE('',#85693);
#19600=PLANE('',#85694);
#19601=PLANE('',#85695);
#19602=PLANE('',#85696);
#19603=PLANE('',#85697);
#19604=PLANE('',#85698);
#19605=PLANE('',#85699);
#19606=PLANE('',#85700);
#19607=PLANE('',#85701);
#19608=PLANE('',#85702);
#19609=PLANE('',#85703);
#19610=PLANE('',#85704);
#19611=PLANE('',#85705);
#19612=PLANE('',#85706);
#19613=PLANE('',#85707);
#19614=PLANE('',#85708);
#19615=PLANE('',#85709);
#19616=PLANE('',#85710);
#19617=PLANE('',#85711);
#19618=PLANE('',#85712);
#19619=PLANE('',#85713);
#19620=PLANE('',#85714);
#19621=PLANE('',#85715);
#19622=PLANE('',#85716);
#19623=PLANE('',#85717);
#19624=PLANE('',#85718);
#19625=PLANE('',#85719);
#19626=PLANE('',#85720);
#19627=PLANE('',#85721);
#19628=PLANE('',#85722);
#19629=PLANE('',#85723);
#19630=PLANE('',#85724);
#19631=PLANE('',#85725);
#19632=PLANE('',#85726);
#19633=PLANE('',#85727);
#19634=PLANE('',#85728);
#19635=PLANE('',#85729);
#19636=PLANE('',#85730);
#19637=PLANE('',#85731);
#19638=PLANE('',#85732);
#19639=PLANE('',#85733);
#19640=PLANE('',#85734);
#19641=PLANE('',#85735);
#19642=PLANE('',#85736);
#19643=PLANE('',#85737);
#19644=PLANE('',#85738);
#19645=PLANE('',#85739);
#19646=PLANE('',#85740);
#19647=PLANE('',#85741);
#19648=PLANE('',#85742);
#19649=PLANE('',#85743);
#19650=PLANE('',#85744);
#19651=PLANE('',#85745);
#19652=PLANE('',#85746);
#19653=PLANE('',#85747);
#19654=PLANE('',#85748);
#19655=PLANE('',#85749);
#19656=PLANE('',#85750);
#19657=PLANE('',#85751);
#19658=PLANE('',#85752);
#19659=PLANE('',#85753);
#19660=PLANE('',#85754);
#19661=PLANE('',#85755);
#19662=PLANE('',#85756);
#19663=PLANE('',#85757);
#19664=PLANE('',#85758);
#19665=PLANE('',#85759);
#19666=PLANE('',#85760);
#19667=PLANE('',#85761);
#19668=PLANE('',#85762);
#19669=PLANE('',#85763);
#19670=PLANE('',#85764);
#19671=PLANE('',#85765);
#19672=PLANE('',#85766);
#19673=PLANE('',#85767);
#19674=PLANE('',#85768);
#19675=PLANE('',#85769);
#19676=PLANE('',#85770);
#19677=PLANE('',#85771);
#19678=PLANE('',#85772);
#19679=PLANE('',#85773);
#19680=PLANE('',#85774);
#19681=PLANE('',#85775);
#19682=PLANE('',#85776);
#19683=PLANE('',#85777);
#19684=PLANE('',#85778);
#19685=PLANE('',#85779);
#19686=PLANE('',#85780);
#19687=PLANE('',#85781);
#19688=PLANE('',#85782);
#19689=PLANE('',#85783);
#19690=PLANE('',#85784);
#19691=PLANE('',#85785);
#19692=PLANE('',#85786);
#19693=PLANE('',#85787);
#19694=PLANE('',#85788);
#19695=PLANE('',#85789);
#19696=PLANE('',#85790);
#19697=PLANE('',#85791);
#19698=PLANE('',#85792);
#19699=PLANE('',#85793);
#19700=PLANE('',#85794);
#19701=PLANE('',#85795);
#19702=PLANE('',#85796);
#19703=PLANE('',#85797);
#19704=PLANE('',#85798);
#19705=PLANE('',#85799);
#19706=PLANE('',#85800);
#19707=PLANE('',#85801);
#19708=PLANE('',#85802);
#19709=PLANE('',#85803);
#19710=PLANE('',#85804);
#19711=PLANE('',#85805);
#19712=PLANE('',#85806);
#19713=PLANE('',#85807);
#19714=PLANE('',#85808);
#19715=PLANE('',#85809);
#19716=PLANE('',#85810);
#19717=PLANE('',#85811);
#19718=PLANE('',#85812);
#19719=PLANE('',#85813);
#19720=PLANE('',#85814);
#19721=PLANE('',#85815);
#19722=PLANE('',#85816);
#19723=PLANE('',#85817);
#19724=PLANE('',#85818);
#19725=PLANE('',#85819);
#19726=PLANE('',#85820);
#19727=PLANE('',#85821);
#19728=PLANE('',#85822);
#19729=PLANE('',#85823);
#19730=PLANE('',#85824);
#19731=PLANE('',#85825);
#19732=PLANE('',#85826);
#19733=PLANE('',#85827);
#19734=PLANE('',#85828);
#19735=PLANE('',#85829);
#19736=PLANE('',#85830);
#19737=PLANE('',#85831);
#19738=PLANE('',#85832);
#19739=PLANE('',#85833);
#19740=PLANE('',#85834);
#19741=PLANE('',#85835);
#19742=PLANE('',#85836);
#19743=PLANE('',#85837);
#19744=PLANE('',#85838);
#19745=PLANE('',#85839);
#19746=PLANE('',#85840);
#19747=PLANE('',#85841);
#19748=PLANE('',#85842);
#19749=PLANE('',#85843);
#19750=PLANE('',#85844);
#19751=PLANE('',#85845);
#19752=PLANE('',#85846);
#19753=PLANE('',#85847);
#19754=PLANE('',#85848);
#19755=PLANE('',#85849);
#19756=PLANE('',#85850);
#19757=PLANE('',#85851);
#19758=PLANE('',#85852);
#19759=PLANE('',#85853);
#19760=PLANE('',#85854);
#19761=PLANE('',#85855);
#19762=PLANE('',#85856);
#19763=PLANE('',#85857);
#19764=PLANE('',#85858);
#19765=PLANE('',#85859);
#19766=PLANE('',#85860);
#19767=PLANE('',#85861);
#19768=PLANE('',#85862);
#19769=PLANE('',#85863);
#19770=PLANE('',#85864);
#19771=PLANE('',#85865);
#19772=PLANE('',#85866);
#19773=PLANE('',#85867);
#19774=PLANE('',#85868);
#19775=PLANE('',#85869);
#19776=PLANE('',#85870);
#19777=PLANE('',#85871);
#19778=PLANE('',#85872);
#19779=PLANE('',#85873);
#19780=PLANE('',#85874);
#19781=PLANE('',#85875);
#19782=PLANE('',#85876);
#19783=PLANE('',#85877);
#19784=PLANE('',#85878);
#19785=PLANE('',#85879);
#19786=PLANE('',#85880);
#19787=PLANE('',#85881);
#19788=PLANE('',#85882);
#19789=PLANE('',#85883);
#19790=PLANE('',#85884);
#19791=PLANE('',#85885);
#19792=PLANE('',#85886);
#19793=PLANE('',#85887);
#19794=PLANE('',#85888);
#19795=PLANE('',#85889);
#19796=PLANE('',#85890);
#19797=PLANE('',#85891);
#19798=PLANE('',#85892);
#19799=PLANE('',#85893);
#19800=PLANE('',#85894);
#19801=PLANE('',#85895);
#19802=PLANE('',#85896);
#19803=PLANE('',#85897);
#19804=PLANE('',#85898);
#19805=PLANE('',#85899);
#19806=PLANE('',#85900);
#19807=PLANE('',#85901);
#19808=PLANE('',#85902);
#19809=PLANE('',#85903);
#19810=PLANE('',#85904);
#19811=PLANE('',#85905);
#19812=PLANE('',#85906);
#19813=PLANE('',#85907);
#19814=PLANE('',#85908);
#19815=PLANE('',#85909);
#19816=PLANE('',#85910);
#19817=PLANE('',#85911);
#19818=PLANE('',#85912);
#19819=PLANE('',#85913);
#19820=PLANE('',#85914);
#19821=PLANE('',#85915);
#19822=PLANE('',#85916);
#19823=PLANE('',#85917);
#19824=PLANE('',#85918);
#19825=PLANE('',#85919);
#19826=PLANE('',#85920);
#19827=PLANE('',#85921);
#19828=PLANE('',#85922);
#19829=PLANE('',#85923);
#19830=PLANE('',#85924);
#19831=PLANE('',#85925);
#19832=PLANE('',#85926);
#19833=PLANE('',#85927);
#19834=PLANE('',#85928);
#19835=PLANE('',#85929);
#19836=PLANE('',#85930);
#19837=PLANE('',#85931);
#19838=PLANE('',#85932);
#19839=PLANE('',#85933);
#19840=PLANE('',#85934);
#19841=PLANE('',#85935);
#19842=PLANE('',#85936);
#19843=PLANE('',#85937);
#19844=PLANE('',#85938);
#19845=PLANE('',#85939);
#19846=PLANE('',#85940);
#19847=PLANE('',#85943);
#19848=PLANE('',#85944);
#19849=PLANE('',#85945);
#19850=PLANE('',#85946);
#19851=PLANE('',#85949);
#19852=PLANE('',#85956);
#19853=PLANE('',#85958);
#19854=PLANE('',#85960);
#19855=PLANE('',#85962);
#19856=PLANE('',#85966);
#20854=FACE_OUTER_BOUND('',#24943,.T.);
#20855=FACE_OUTER_BOUND('',#24944,.T.);
#20856=FACE_OUTER_BOUND('',#24945,.T.);
#20857=FACE_OUTER_BOUND('',#24946,.T.);
#20858=FACE_OUTER_BOUND('',#24947,.T.);
#20859=FACE_OUTER_BOUND('',#24948,.T.);
#20860=FACE_OUTER_BOUND('',#24949,.T.);
#20861=FACE_OUTER_BOUND('',#24950,.T.);
#20862=FACE_OUTER_BOUND('',#24951,.T.);
#20863=FACE_OUTER_BOUND('',#24952,.T.);
#20864=FACE_OUTER_BOUND('',#24956,.T.);
#20865=FACE_OUTER_BOUND('',#24957,.T.);
#20866=FACE_OUTER_BOUND('',#24958,.T.);
#20867=FACE_OUTER_BOUND('',#24962,.T.);
#20868=FACE_OUTER_BOUND('',#24963,.T.);
#20869=FACE_OUTER_BOUND('',#24964,.T.);
#20870=FACE_OUTER_BOUND('',#24965,.T.);
#20871=FACE_OUTER_BOUND('',#24966,.T.);
#20872=FACE_OUTER_BOUND('',#24967,.T.);
#20873=FACE_OUTER_BOUND('',#24968,.T.);
#20874=FACE_OUTER_BOUND('',#24969,.T.);
#20875=FACE_OUTER_BOUND('',#24970,.T.);
#20876=FACE_OUTER_BOUND('',#24971,.T.);
#20877=FACE_OUTER_BOUND('',#24972,.T.);
#20878=FACE_OUTER_BOUND('',#24973,.T.);
#20879=FACE_OUTER_BOUND('',#24974,.T.);
#20880=FACE_OUTER_BOUND('',#24975,.T.);
#20881=FACE_OUTER_BOUND('',#24976,.T.);
#20882=FACE_OUTER_BOUND('',#24977,.T.);
#20883=FACE_OUTER_BOUND('',#24978,.T.);
#20884=FACE_OUTER_BOUND('',#24979,.T.);
#20885=FACE_OUTER_BOUND('',#24980,.T.);
#20886=FACE_OUTER_BOUND('',#24981,.T.);
#20887=FACE_OUTER_BOUND('',#24982,.T.);
#20888=FACE_OUTER_BOUND('',#24983,.T.);
#20889=FACE_OUTER_BOUND('',#24985,.T.);
#20890=FACE_OUTER_BOUND('',#24987,.T.);
#20891=FACE_OUTER_BOUND('',#24988,.T.);
#20892=FACE_OUTER_BOUND('',#24989,.T.);
#20893=FACE_OUTER_BOUND('',#24990,.T.);
#20894=FACE_OUTER_BOUND('',#24991,.T.);
#20895=FACE_OUTER_BOUND('',#24993,.T.);
#20896=FACE_OUTER_BOUND('',#24995,.T.);
#20897=FACE_OUTER_BOUND('',#24997,.T.);
#20898=FACE_OUTER_BOUND('',#24998,.T.);
#20899=FACE_OUTER_BOUND('',#24999,.T.);
#20900=FACE_OUTER_BOUND('',#25000,.T.);
#20901=FACE_OUTER_BOUND('',#25001,.T.);
#20902=FACE_OUTER_BOUND('',#25002,.T.);
#20903=FACE_OUTER_BOUND('',#25003,.T.);
#20904=FACE_OUTER_BOUND('',#25004,.T.);
#20905=FACE_OUTER_BOUND('',#25005,.T.);
#20906=FACE_OUTER_BOUND('',#25006,.T.);
#20907=FACE_OUTER_BOUND('',#25007,.T.);
#20908=FACE_OUTER_BOUND('',#25008,.T.);
#20909=FACE_OUTER_BOUND('',#25009,.T.);
#20910=FACE_OUTER_BOUND('',#25010,.T.);
#20911=FACE_OUTER_BOUND('',#25011,.T.);
#20912=FACE_OUTER_BOUND('',#25012,.T.);
#20913=FACE_OUTER_BOUND('',#25013,.T.);
#20914=FACE_OUTER_BOUND('',#25014,.T.);
#20915=FACE_OUTER_BOUND('',#25015,.T.);
#20916=FACE_OUTER_BOUND('',#25016,.T.);
#20917=FACE_OUTER_BOUND('',#25017,.T.);
#20918=FACE_OUTER_BOUND('',#25018,.T.);
#20919=FACE_OUTER_BOUND('',#25019,.T.);
#20920=FACE_OUTER_BOUND('',#25020,.T.);
#20921=FACE_OUTER_BOUND('',#25021,.T.);
#20922=FACE_OUTER_BOUND('',#25022,.T.);
#20923=FACE_OUTER_BOUND('',#25023,.T.);
#20924=FACE_OUTER_BOUND('',#25024,.T.);
#20925=FACE_OUTER_BOUND('',#25025,.T.);
#20926=FACE_OUTER_BOUND('',#25026,.T.);
#20927=FACE_OUTER_BOUND('',#25027,.T.);
#20928=FACE_OUTER_BOUND('',#25028,.T.);
#20929=FACE_OUTER_BOUND('',#25029,.T.);
#20930=FACE_OUTER_BOUND('',#25030,.T.);
#20931=FACE_OUTER_BOUND('',#25031,.T.);
#20932=FACE_OUTER_BOUND('',#25032,.T.);
#20933=FACE_OUTER_BOUND('',#25033,.T.);
#20934=FACE_OUTER_BOUND('',#25034,.T.);
#20935=FACE_OUTER_BOUND('',#25035,.T.);
#20936=FACE_OUTER_BOUND('',#25036,.T.);
#20937=FACE_OUTER_BOUND('',#25037,.T.);
#20938=FACE_OUTER_BOUND('',#25038,.T.);
#20939=FACE_OUTER_BOUND('',#25039,.T.);
#20940=FACE_OUTER_BOUND('',#25040,.T.);
#20941=FACE_OUTER_BOUND('',#25041,.T.);
#20942=FACE_OUTER_BOUND('',#25042,.T.);
#20943=FACE_OUTER_BOUND('',#25043,.T.);
#20944=FACE_OUTER_BOUND('',#25044,.T.);
#20945=FACE_OUTER_BOUND('',#25045,.T.);
#20946=FACE_OUTER_BOUND('',#25046,.T.);
#20947=FACE_OUTER_BOUND('',#25047,.T.);
#20948=FACE_OUTER_BOUND('',#25048,.T.);
#20949=FACE_OUTER_BOUND('',#25049,.T.);
#20950=FACE_OUTER_BOUND('',#25050,.T.);
#20951=FACE_OUTER_BOUND('',#25051,.T.);
#20952=FACE_OUTER_BOUND('',#25052,.T.);
#20953=FACE_OUTER_BOUND('',#25053,.T.);
#20954=FACE_OUTER_BOUND('',#25054,.T.);
#20955=FACE_OUTER_BOUND('',#25055,.T.);
#20956=FACE_OUTER_BOUND('',#25056,.T.);
#20957=FACE_OUTER_BOUND('',#25057,.T.);
#20958=FACE_OUTER_BOUND('',#25058,.T.);
#20959=FACE_OUTER_BOUND('',#25059,.T.);
#20960=FACE_OUTER_BOUND('',#25060,.T.);
#20961=FACE_OUTER_BOUND('',#25061,.T.);
#20962=FACE_OUTER_BOUND('',#25062,.T.);
#20963=FACE_OUTER_BOUND('',#25063,.T.);
#20964=FACE_OUTER_BOUND('',#25064,.T.);
#20965=FACE_OUTER_BOUND('',#25065,.T.);
#20966=FACE_OUTER_BOUND('',#25066,.T.);
#20967=FACE_OUTER_BOUND('',#25067,.T.);
#20968=FACE_OUTER_BOUND('',#25068,.T.);
#20969=FACE_OUTER_BOUND('',#25069,.T.);
#20970=FACE_OUTER_BOUND('',#25070,.T.);
#20971=FACE_OUTER_BOUND('',#25071,.T.);
#20972=FACE_OUTER_BOUND('',#25072,.T.);
#20973=FACE_OUTER_BOUND('',#25073,.T.);
#20974=FACE_OUTER_BOUND('',#25074,.T.);
#20975=FACE_OUTER_BOUND('',#25075,.T.);
#20976=FACE_OUTER_BOUND('',#25076,.T.);
#20977=FACE_OUTER_BOUND('',#25077,.T.);
#20978=FACE_OUTER_BOUND('',#25078,.T.);
#20979=FACE_OUTER_BOUND('',#25079,.T.);
#20980=FACE_OUTER_BOUND('',#25080,.T.);
#20981=FACE_OUTER_BOUND('',#25081,.T.);
#20982=FACE_OUTER_BOUND('',#25082,.T.);
#20983=FACE_OUTER_BOUND('',#25083,.T.);
#20984=FACE_OUTER_BOUND('',#25084,.T.);
#20985=FACE_OUTER_BOUND('',#25085,.T.);
#20986=FACE_OUTER_BOUND('',#25086,.T.);
#20987=FACE_OUTER_BOUND('',#25087,.T.);
#20988=FACE_OUTER_BOUND('',#25088,.T.);
#20989=FACE_OUTER_BOUND('',#25089,.T.);
#20990=FACE_OUTER_BOUND('',#25090,.T.);
#20991=FACE_OUTER_BOUND('',#25091,.T.);
#20992=FACE_OUTER_BOUND('',#25092,.T.);
#20993=FACE_OUTER_BOUND('',#25093,.T.);
#20994=FACE_OUTER_BOUND('',#25094,.T.);
#20995=FACE_OUTER_BOUND('',#25095,.T.);
#20996=FACE_OUTER_BOUND('',#25096,.T.);
#20997=FACE_OUTER_BOUND('',#25097,.T.);
#20998=FACE_OUTER_BOUND('',#25098,.T.);
#20999=FACE_OUTER_BOUND('',#25099,.T.);
#21000=FACE_OUTER_BOUND('',#25100,.T.);
#21001=FACE_OUTER_BOUND('',#25101,.T.);
#21002=FACE_OUTER_BOUND('',#25102,.T.);
#21003=FACE_OUTER_BOUND('',#25103,.T.);
#21004=FACE_OUTER_BOUND('',#25104,.T.);
#21005=FACE_OUTER_BOUND('',#25105,.T.);
#21006=FACE_OUTER_BOUND('',#25106,.T.);
#21007=FACE_OUTER_BOUND('',#25107,.T.);
#21008=FACE_OUTER_BOUND('',#25108,.T.);
#21009=FACE_OUTER_BOUND('',#25109,.T.);
#21010=FACE_OUTER_BOUND('',#25110,.T.);
#21011=FACE_OUTER_BOUND('',#25111,.T.);
#21012=FACE_OUTER_BOUND('',#25112,.T.);
#21013=FACE_OUTER_BOUND('',#25113,.T.);
#21014=FACE_OUTER_BOUND('',#25114,.T.);
#21015=FACE_OUTER_BOUND('',#25115,.T.);
#21016=FACE_OUTER_BOUND('',#25116,.T.);
#21017=FACE_OUTER_BOUND('',#25117,.T.);
#21018=FACE_OUTER_BOUND('',#25118,.T.);
#21019=FACE_OUTER_BOUND('',#25119,.T.);
#21020=FACE_OUTER_BOUND('',#25120,.T.);
#21021=FACE_OUTER_BOUND('',#25121,.T.);
#21022=FACE_OUTER_BOUND('',#25122,.T.);
#21023=FACE_OUTER_BOUND('',#25123,.T.);
#21024=FACE_OUTER_BOUND('',#25124,.T.);
#21025=FACE_OUTER_BOUND('',#25125,.T.);
#21026=FACE_OUTER_BOUND('',#25126,.T.);
#21027=FACE_OUTER_BOUND('',#25127,.T.);
#21028=FACE_OUTER_BOUND('',#25128,.T.);
#21029=FACE_OUTER_BOUND('',#25129,.T.);
#21030=FACE_OUTER_BOUND('',#25130,.T.);
#21031=FACE_OUTER_BOUND('',#25131,.T.);
#21032=FACE_OUTER_BOUND('',#25132,.T.);
#21033=FACE_OUTER_BOUND('',#25133,.T.);
#21034=FACE_OUTER_BOUND('',#25134,.T.);
#21035=FACE_OUTER_BOUND('',#25135,.T.);
#21036=FACE_OUTER_BOUND('',#25136,.T.);
#21037=FACE_OUTER_BOUND('',#25137,.T.);
#21038=FACE_OUTER_BOUND('',#25138,.T.);
#21039=FACE_OUTER_BOUND('',#25139,.T.);
#21040=FACE_OUTER_BOUND('',#25140,.T.);
#21041=FACE_OUTER_BOUND('',#25141,.T.);
#21042=FACE_OUTER_BOUND('',#25142,.T.);
#21043=FACE_OUTER_BOUND('',#25143,.T.);
#21044=FACE_OUTER_BOUND('',#25144,.T.);
#21045=FACE_OUTER_BOUND('',#25145,.T.);
#21046=FACE_OUTER_BOUND('',#25146,.T.);
#21047=FACE_OUTER_BOUND('',#25147,.T.);
#21048=FACE_OUTER_BOUND('',#25148,.T.);
#21049=FACE_OUTER_BOUND('',#25149,.T.);
#21050=FACE_OUTER_BOUND('',#25150,.T.);
#21051=FACE_OUTER_BOUND('',#25151,.T.);
#21052=FACE_OUTER_BOUND('',#25152,.T.);
#21053=FACE_OUTER_BOUND('',#25153,.T.);
#21054=FACE_OUTER_BOUND('',#25154,.T.);
#21055=FACE_OUTER_BOUND('',#25155,.T.);
#21056=FACE_OUTER_BOUND('',#25156,.T.);
#21057=FACE_OUTER_BOUND('',#25157,.T.);
#21058=FACE_OUTER_BOUND('',#25158,.T.);
#21059=FACE_OUTER_BOUND('',#25159,.T.);
#21060=FACE_OUTER_BOUND('',#25160,.T.);
#21061=FACE_OUTER_BOUND('',#25161,.T.);
#21062=FACE_OUTER_BOUND('',#25162,.T.);
#21063=FACE_OUTER_BOUND('',#25163,.T.);
#21064=FACE_OUTER_BOUND('',#25164,.T.);
#21065=FACE_OUTER_BOUND('',#25165,.T.);
#21066=FACE_OUTER_BOUND('',#25166,.T.);
#21067=FACE_OUTER_BOUND('',#25167,.T.);
#21068=FACE_OUTER_BOUND('',#25168,.T.);
#21069=FACE_OUTER_BOUND('',#25169,.T.);
#21070=FACE_OUTER_BOUND('',#25170,.T.);
#21071=FACE_OUTER_BOUND('',#25171,.T.);
#21072=FACE_OUTER_BOUND('',#25172,.T.);
#21073=FACE_OUTER_BOUND('',#25173,.T.);
#21074=FACE_OUTER_BOUND('',#25174,.T.);
#21075=FACE_OUTER_BOUND('',#25175,.T.);
#21076=FACE_OUTER_BOUND('',#25176,.T.);
#21077=FACE_OUTER_BOUND('',#25177,.T.);
#21078=FACE_OUTER_BOUND('',#25178,.T.);
#21079=FACE_OUTER_BOUND('',#25179,.T.);
#21080=FACE_OUTER_BOUND('',#25180,.T.);
#21081=FACE_OUTER_BOUND('',#25181,.T.);
#21082=FACE_OUTER_BOUND('',#25182,.T.);
#21083=FACE_OUTER_BOUND('',#25183,.T.);
#21084=FACE_OUTER_BOUND('',#25184,.T.);
#21085=FACE_OUTER_BOUND('',#25185,.T.);
#21086=FACE_OUTER_BOUND('',#25186,.T.);
#21087=FACE_OUTER_BOUND('',#25187,.T.);
#21088=FACE_OUTER_BOUND('',#25188,.T.);
#21089=FACE_OUTER_BOUND('',#25189,.T.);
#21090=FACE_OUTER_BOUND('',#25190,.T.);
#21091=FACE_OUTER_BOUND('',#25191,.T.);
#21092=FACE_OUTER_BOUND('',#25192,.T.);
#21093=FACE_OUTER_BOUND('',#25193,.T.);
#21094=FACE_OUTER_BOUND('',#25194,.T.);
#21095=FACE_OUTER_BOUND('',#25195,.T.);
#21096=FACE_OUTER_BOUND('',#25196,.T.);
#21097=FACE_OUTER_BOUND('',#25197,.T.);
#21098=FACE_OUTER_BOUND('',#25198,.T.);
#21099=FACE_OUTER_BOUND('',#25199,.T.);
#21100=FACE_OUTER_BOUND('',#25200,.T.);
#21101=FACE_OUTER_BOUND('',#25201,.T.);
#21102=FACE_OUTER_BOUND('',#25202,.T.);
#21103=FACE_OUTER_BOUND('',#25203,.T.);
#21104=FACE_OUTER_BOUND('',#25204,.T.);
#21105=FACE_OUTER_BOUND('',#25205,.T.);
#21106=FACE_OUTER_BOUND('',#25206,.T.);
#21107=FACE_OUTER_BOUND('',#25207,.T.);
#21108=FACE_OUTER_BOUND('',#25208,.T.);
#21109=FACE_OUTER_BOUND('',#25209,.T.);
#21110=FACE_OUTER_BOUND('',#25210,.T.);
#21111=FACE_OUTER_BOUND('',#25211,.T.);
#21112=FACE_OUTER_BOUND('',#25212,.T.);
#21113=FACE_OUTER_BOUND('',#25213,.T.);
#21114=FACE_OUTER_BOUND('',#25214,.T.);
#21115=FACE_OUTER_BOUND('',#25215,.T.);
#21116=FACE_OUTER_BOUND('',#25216,.T.);
#21117=FACE_OUTER_BOUND('',#25217,.T.);
#21118=FACE_OUTER_BOUND('',#25218,.T.);
#21119=FACE_OUTER_BOUND('',#25219,.T.);
#21120=FACE_OUTER_BOUND('',#25220,.T.);
#21121=FACE_OUTER_BOUND('',#25221,.T.);
#21122=FACE_OUTER_BOUND('',#25222,.T.);
#21123=FACE_OUTER_BOUND('',#25223,.T.);
#21124=FACE_OUTER_BOUND('',#25224,.T.);
#21125=FACE_OUTER_BOUND('',#25225,.T.);
#21126=FACE_OUTER_BOUND('',#25226,.T.);
#21127=FACE_OUTER_BOUND('',#25227,.T.);
#21128=FACE_OUTER_BOUND('',#25228,.T.);
#21129=FACE_OUTER_BOUND('',#25229,.T.);
#21130=FACE_OUTER_BOUND('',#25230,.T.);
#21131=FACE_OUTER_BOUND('',#25231,.T.);
#21132=FACE_OUTER_BOUND('',#25232,.T.);
#21133=FACE_OUTER_BOUND('',#25233,.T.);
#21134=FACE_OUTER_BOUND('',#25234,.T.);
#21135=FACE_OUTER_BOUND('',#25235,.T.);
#21136=FACE_OUTER_BOUND('',#25236,.T.);
#21137=FACE_OUTER_BOUND('',#25237,.T.);
#21138=FACE_OUTER_BOUND('',#25238,.T.);
#21139=FACE_OUTER_BOUND('',#25239,.T.);
#21140=FACE_OUTER_BOUND('',#25240,.T.);
#21141=FACE_OUTER_BOUND('',#25241,.T.);
#21142=FACE_OUTER_BOUND('',#25242,.T.);
#21143=FACE_OUTER_BOUND('',#25243,.T.);
#21144=FACE_OUTER_BOUND('',#25244,.T.);
#21145=FACE_OUTER_BOUND('',#25245,.T.);
#21146=FACE_OUTER_BOUND('',#25246,.T.);
#21147=FACE_OUTER_BOUND('',#25247,.T.);
#21148=FACE_OUTER_BOUND('',#25248,.T.);
#21149=FACE_OUTER_BOUND('',#25249,.T.);
#21150=FACE_OUTER_BOUND('',#25250,.T.);
#21151=FACE_OUTER_BOUND('',#25251,.T.);
#21152=FACE_OUTER_BOUND('',#25252,.T.);
#21153=FACE_OUTER_BOUND('',#25253,.T.);
#21154=FACE_OUTER_BOUND('',#25254,.T.);
#21155=FACE_OUTER_BOUND('',#25255,.T.);
#21156=FACE_OUTER_BOUND('',#25256,.T.);
#21157=FACE_OUTER_BOUND('',#25257,.T.);
#21158=FACE_OUTER_BOUND('',#25258,.T.);
#21159=FACE_OUTER_BOUND('',#25259,.T.);
#21160=FACE_OUTER_BOUND('',#25260,.T.);
#21161=FACE_OUTER_BOUND('',#25261,.T.);
#21162=FACE_OUTER_BOUND('',#25262,.T.);
#21163=FACE_OUTER_BOUND('',#25263,.T.);
#21164=FACE_OUTER_BOUND('',#25264,.T.);
#21165=FACE_OUTER_BOUND('',#25265,.T.);
#21166=FACE_OUTER_BOUND('',#25266,.T.);
#21167=FACE_OUTER_BOUND('',#25267,.T.);
#21168=FACE_OUTER_BOUND('',#25268,.T.);
#21169=FACE_OUTER_BOUND('',#25269,.T.);
#21170=FACE_OUTER_BOUND('',#25270,.T.);
#21171=FACE_OUTER_BOUND('',#25271,.T.);
#21172=FACE_OUTER_BOUND('',#25272,.T.);
#21173=FACE_OUTER_BOUND('',#25273,.T.);
#21174=FACE_OUTER_BOUND('',#25274,.T.);
#21175=FACE_OUTER_BOUND('',#25275,.T.);
#21176=FACE_OUTER_BOUND('',#25276,.T.);
#21177=FACE_OUTER_BOUND('',#25277,.T.);
#21178=FACE_OUTER_BOUND('',#25278,.T.);
#21179=FACE_OUTER_BOUND('',#25279,.T.);
#21180=FACE_OUTER_BOUND('',#25280,.T.);
#21181=FACE_OUTER_BOUND('',#25281,.T.);
#21182=FACE_OUTER_BOUND('',#25282,.T.);
#21183=FACE_OUTER_BOUND('',#25283,.T.);
#21184=FACE_OUTER_BOUND('',#25284,.T.);
#21185=FACE_OUTER_BOUND('',#25285,.T.);
#21186=FACE_OUTER_BOUND('',#25286,.T.);
#21187=FACE_OUTER_BOUND('',#25287,.T.);
#21188=FACE_OUTER_BOUND('',#25288,.T.);
#21189=FACE_OUTER_BOUND('',#25289,.T.);
#21190=FACE_OUTER_BOUND('',#25290,.T.);
#21191=FACE_OUTER_BOUND('',#25291,.T.);
#21192=FACE_OUTER_BOUND('',#25292,.T.);
#21193=FACE_OUTER_BOUND('',#25293,.T.);
#21194=FACE_OUTER_BOUND('',#25294,.T.);
#21195=FACE_OUTER_BOUND('',#25295,.T.);
#21196=FACE_OUTER_BOUND('',#25296,.T.);
#21197=FACE_OUTER_BOUND('',#25297,.T.);
#21198=FACE_OUTER_BOUND('',#25298,.T.);
#21199=FACE_OUTER_BOUND('',#25299,.T.);
#21200=FACE_OUTER_BOUND('',#25300,.T.);
#21201=FACE_OUTER_BOUND('',#25301,.T.);
#21202=FACE_OUTER_BOUND('',#25302,.T.);
#21203=FACE_OUTER_BOUND('',#25303,.T.);
#21204=FACE_OUTER_BOUND('',#25304,.T.);
#21205=FACE_OUTER_BOUND('',#25305,.T.);
#21206=FACE_OUTER_BOUND('',#25306,.T.);
#21207=FACE_OUTER_BOUND('',#25307,.T.);
#21208=FACE_OUTER_BOUND('',#25308,.T.);
#21209=FACE_OUTER_BOUND('',#25309,.T.);
#21210=FACE_OUTER_BOUND('',#25310,.T.);
#21211=FACE_OUTER_BOUND('',#25311,.T.);
#21212=FACE_OUTER_BOUND('',#25312,.T.);
#21213=FACE_OUTER_BOUND('',#25313,.T.);
#21214=FACE_OUTER_BOUND('',#25314,.T.);
#21215=FACE_OUTER_BOUND('',#25315,.T.);
#21216=FACE_OUTER_BOUND('',#25316,.T.);
#21217=FACE_OUTER_BOUND('',#25317,.T.);
#21218=FACE_OUTER_BOUND('',#25318,.T.);
#21219=FACE_OUTER_BOUND('',#25319,.T.);
#21220=FACE_OUTER_BOUND('',#25320,.T.);
#21221=FACE_OUTER_BOUND('',#25321,.T.);
#21222=FACE_OUTER_BOUND('',#25322,.T.);
#21223=FACE_OUTER_BOUND('',#25323,.T.);
#21224=FACE_OUTER_BOUND('',#25324,.T.);
#21225=FACE_OUTER_BOUND('',#25325,.T.);
#21226=FACE_OUTER_BOUND('',#25326,.T.);
#21227=FACE_OUTER_BOUND('',#25327,.T.);
#21228=FACE_OUTER_BOUND('',#25328,.T.);
#21229=FACE_OUTER_BOUND('',#25329,.T.);
#21230=FACE_OUTER_BOUND('',#25330,.T.);
#21231=FACE_OUTER_BOUND('',#25331,.T.);
#21232=FACE_OUTER_BOUND('',#25332,.T.);
#21233=FACE_OUTER_BOUND('',#25333,.T.);
#21234=FACE_OUTER_BOUND('',#25334,.T.);
#21235=FACE_OUTER_BOUND('',#25335,.T.);
#21236=FACE_OUTER_BOUND('',#25336,.T.);
#21237=FACE_OUTER_BOUND('',#25337,.T.);
#21238=FACE_OUTER_BOUND('',#25338,.T.);
#21239=FACE_OUTER_BOUND('',#25339,.T.);
#21240=FACE_OUTER_BOUND('',#25340,.T.);
#21241=FACE_OUTER_BOUND('',#25341,.T.);
#21242=FACE_OUTER_BOUND('',#25342,.T.);
#21243=FACE_OUTER_BOUND('',#25343,.T.);
#21244=FACE_OUTER_BOUND('',#25344,.T.);
#21245=FACE_OUTER_BOUND('',#25345,.T.);
#21246=FACE_OUTER_BOUND('',#25346,.T.);
#21247=FACE_OUTER_BOUND('',#25347,.T.);
#21248=FACE_OUTER_BOUND('',#25348,.T.);
#21249=FACE_OUTER_BOUND('',#25349,.T.);
#21250=FACE_OUTER_BOUND('',#25350,.T.);
#21251=FACE_OUTER_BOUND('',#25351,.T.);
#21252=FACE_OUTER_BOUND('',#25352,.T.);
#21253=FACE_OUTER_BOUND('',#25353,.T.);
#21254=FACE_OUTER_BOUND('',#25354,.T.);
#21255=FACE_OUTER_BOUND('',#25355,.T.);
#21256=FACE_OUTER_BOUND('',#25356,.T.);
#21257=FACE_OUTER_BOUND('',#25357,.T.);
#21258=FACE_OUTER_BOUND('',#25358,.T.);
#21259=FACE_OUTER_BOUND('',#25359,.T.);
#21260=FACE_OUTER_BOUND('',#25360,.T.);
#21261=FACE_OUTER_BOUND('',#25361,.T.);
#21262=FACE_OUTER_BOUND('',#25362,.T.);
#21263=FACE_OUTER_BOUND('',#25363,.T.);
#21264=FACE_OUTER_BOUND('',#25364,.T.);
#21265=FACE_OUTER_BOUND('',#25365,.T.);
#21266=FACE_OUTER_BOUND('',#25366,.T.);
#21267=FACE_OUTER_BOUND('',#25367,.T.);
#21268=FACE_OUTER_BOUND('',#25368,.T.);
#21269=FACE_OUTER_BOUND('',#25369,.T.);
#21270=FACE_OUTER_BOUND('',#25370,.T.);
#21271=FACE_OUTER_BOUND('',#25371,.T.);
#21272=FACE_OUTER_BOUND('',#25372,.T.);
#21273=FACE_OUTER_BOUND('',#25373,.T.);
#21274=FACE_OUTER_BOUND('',#25374,.T.);
#21275=FACE_OUTER_BOUND('',#25375,.T.);
#21276=FACE_OUTER_BOUND('',#25376,.T.);
#21277=FACE_OUTER_BOUND('',#25377,.T.);
#21278=FACE_OUTER_BOUND('',#25378,.T.);
#21279=FACE_OUTER_BOUND('',#25379,.T.);
#21280=FACE_OUTER_BOUND('',#25380,.T.);
#21281=FACE_OUTER_BOUND('',#25381,.T.);
#21282=FACE_OUTER_BOUND('',#25382,.T.);
#21283=FACE_OUTER_BOUND('',#25383,.T.);
#21284=FACE_OUTER_BOUND('',#25384,.T.);
#21285=FACE_OUTER_BOUND('',#25385,.T.);
#21286=FACE_OUTER_BOUND('',#25386,.T.);
#21287=FACE_OUTER_BOUND('',#25387,.T.);
#21288=FACE_OUTER_BOUND('',#25388,.T.);
#21289=FACE_OUTER_BOUND('',#25389,.T.);
#21290=FACE_OUTER_BOUND('',#25390,.T.);
#21291=FACE_OUTER_BOUND('',#25391,.T.);
#21292=FACE_OUTER_BOUND('',#25392,.T.);
#21293=FACE_OUTER_BOUND('',#25393,.T.);
#21294=FACE_OUTER_BOUND('',#25394,.T.);
#21295=FACE_OUTER_BOUND('',#25395,.T.);
#21296=FACE_OUTER_BOUND('',#25396,.T.);
#21297=FACE_OUTER_BOUND('',#25397,.T.);
#21298=FACE_OUTER_BOUND('',#25398,.T.);
#21299=FACE_OUTER_BOUND('',#25399,.T.);
#21300=FACE_OUTER_BOUND('',#25400,.T.);
#21301=FACE_OUTER_BOUND('',#25401,.T.);
#21302=FACE_OUTER_BOUND('',#25402,.T.);
#21303=FACE_OUTER_BOUND('',#25403,.T.);
#21304=FACE_OUTER_BOUND('',#25404,.T.);
#21305=FACE_OUTER_BOUND('',#25405,.T.);
#21306=FACE_OUTER_BOUND('',#25406,.T.);
#21307=FACE_OUTER_BOUND('',#25407,.T.);
#21308=FACE_OUTER_BOUND('',#25408,.T.);
#21309=FACE_OUTER_BOUND('',#25409,.T.);
#21310=FACE_OUTER_BOUND('',#25410,.T.);
#21311=FACE_OUTER_BOUND('',#25411,.T.);
#21312=FACE_OUTER_BOUND('',#25412,.T.);
#21313=FACE_OUTER_BOUND('',#25413,.T.);
#21314=FACE_OUTER_BOUND('',#25414,.T.);
#21315=FACE_OUTER_BOUND('',#25415,.T.);
#21316=FACE_OUTER_BOUND('',#25416,.T.);
#21317=FACE_OUTER_BOUND('',#25417,.T.);
#21318=FACE_OUTER_BOUND('',#25418,.T.);
#21319=FACE_OUTER_BOUND('',#25419,.T.);
#21320=FACE_OUTER_BOUND('',#25420,.T.);
#21321=FACE_OUTER_BOUND('',#25421,.T.);
#21322=FACE_OUTER_BOUND('',#25422,.T.);
#21323=FACE_OUTER_BOUND('',#25423,.T.);
#21324=FACE_OUTER_BOUND('',#25424,.T.);
#21325=FACE_OUTER_BOUND('',#25425,.T.);
#21326=FACE_OUTER_BOUND('',#25426,.T.);
#21327=FACE_OUTER_BOUND('',#25427,.T.);
#21328=FACE_OUTER_BOUND('',#25428,.T.);
#21329=FACE_OUTER_BOUND('',#25429,.T.);
#21330=FACE_OUTER_BOUND('',#25430,.T.);
#21331=FACE_OUTER_BOUND('',#25431,.T.);
#21332=FACE_OUTER_BOUND('',#25432,.T.);
#21333=FACE_OUTER_BOUND('',#25433,.T.);
#21334=FACE_OUTER_BOUND('',#25434,.T.);
#21335=FACE_OUTER_BOUND('',#25435,.T.);
#21336=FACE_OUTER_BOUND('',#25436,.T.);
#21337=FACE_OUTER_BOUND('',#25437,.T.);
#21338=FACE_OUTER_BOUND('',#25438,.T.);
#21339=FACE_OUTER_BOUND('',#25439,.T.);
#21340=FACE_OUTER_BOUND('',#25440,.T.);
#21341=FACE_OUTER_BOUND('',#25441,.T.);
#21342=FACE_OUTER_BOUND('',#25442,.T.);
#21343=FACE_OUTER_BOUND('',#25443,.T.);
#21344=FACE_OUTER_BOUND('',#25444,.T.);
#21345=FACE_OUTER_BOUND('',#25445,.T.);
#21346=FACE_OUTER_BOUND('',#25446,.T.);
#21347=FACE_OUTER_BOUND('',#25447,.T.);
#21348=FACE_OUTER_BOUND('',#25448,.T.);
#21349=FACE_OUTER_BOUND('',#25449,.T.);
#21350=FACE_OUTER_BOUND('',#25450,.T.);
#21351=FACE_OUTER_BOUND('',#25451,.T.);
#21352=FACE_OUTER_BOUND('',#25452,.T.);
#21353=FACE_OUTER_BOUND('',#25453,.T.);
#21354=FACE_OUTER_BOUND('',#25454,.T.);
#21355=FACE_OUTER_BOUND('',#25455,.T.);
#21356=FACE_OUTER_BOUND('',#25456,.T.);
#21357=FACE_OUTER_BOUND('',#25457,.T.);
#21358=FACE_OUTER_BOUND('',#25458,.T.);
#21359=FACE_OUTER_BOUND('',#25459,.T.);
#21360=FACE_OUTER_BOUND('',#25460,.T.);
#21361=FACE_OUTER_BOUND('',#25461,.T.);
#21362=FACE_OUTER_BOUND('',#25462,.T.);
#21363=FACE_OUTER_BOUND('',#25463,.T.);
#21364=FACE_OUTER_BOUND('',#25464,.T.);
#21365=FACE_OUTER_BOUND('',#25465,.T.);
#21366=FACE_OUTER_BOUND('',#25466,.T.);
#21367=FACE_OUTER_BOUND('',#25467,.T.);
#21368=FACE_OUTER_BOUND('',#25468,.T.);
#21369=FACE_OUTER_BOUND('',#25469,.T.);
#21370=FACE_OUTER_BOUND('',#25470,.T.);
#21371=FACE_OUTER_BOUND('',#25471,.T.);
#21372=FACE_OUTER_BOUND('',#25472,.T.);
#21373=FACE_OUTER_BOUND('',#25473,.T.);
#21374=FACE_OUTER_BOUND('',#25474,.T.);
#21375=FACE_OUTER_BOUND('',#25475,.T.);
#21376=FACE_OUTER_BOUND('',#25476,.T.);
#21377=FACE_OUTER_BOUND('',#25477,.T.);
#21378=FACE_OUTER_BOUND('',#25478,.T.);
#21379=FACE_OUTER_BOUND('',#25479,.T.);
#21380=FACE_OUTER_BOUND('',#25480,.T.);
#21381=FACE_OUTER_BOUND('',#25481,.T.);
#21382=FACE_OUTER_BOUND('',#25482,.T.);
#21383=FACE_OUTER_BOUND('',#25483,.T.);
#21384=FACE_OUTER_BOUND('',#25484,.T.);
#21385=FACE_OUTER_BOUND('',#25485,.T.);
#21386=FACE_OUTER_BOUND('',#25486,.T.);
#21387=FACE_OUTER_BOUND('',#25487,.T.);
#21388=FACE_OUTER_BOUND('',#25488,.T.);
#21389=FACE_OUTER_BOUND('',#25489,.T.);
#21390=FACE_OUTER_BOUND('',#25490,.T.);
#21391=FACE_OUTER_BOUND('',#25491,.T.);
#21392=FACE_OUTER_BOUND('',#25492,.T.);
#21393=FACE_OUTER_BOUND('',#25493,.T.);
#21394=FACE_OUTER_BOUND('',#25494,.T.);
#21395=FACE_OUTER_BOUND('',#25495,.T.);
#21396=FACE_OUTER_BOUND('',#25496,.T.);
#21397=FACE_OUTER_BOUND('',#25497,.T.);
#21398=FACE_OUTER_BOUND('',#25498,.T.);
#21399=FACE_OUTER_BOUND('',#25499,.T.);
#21400=FACE_OUTER_BOUND('',#25500,.T.);
#21401=FACE_OUTER_BOUND('',#25501,.T.);
#21402=FACE_OUTER_BOUND('',#25502,.T.);
#21403=FACE_OUTER_BOUND('',#25503,.T.);
#21404=FACE_OUTER_BOUND('',#25504,.T.);
#21405=FACE_OUTER_BOUND('',#25505,.T.);
#21406=FACE_OUTER_BOUND('',#25506,.T.);
#21407=FACE_OUTER_BOUND('',#25507,.T.);
#21408=FACE_OUTER_BOUND('',#25508,.T.);
#21409=FACE_OUTER_BOUND('',#25509,.T.);
#21410=FACE_OUTER_BOUND('',#25510,.T.);
#21411=FACE_OUTER_BOUND('',#25511,.T.);
#21412=FACE_OUTER_BOUND('',#25512,.T.);
#21413=FACE_OUTER_BOUND('',#25513,.T.);
#21414=FACE_OUTER_BOUND('',#25514,.T.);
#21415=FACE_OUTER_BOUND('',#25515,.T.);
#21416=FACE_OUTER_BOUND('',#25516,.T.);
#21417=FACE_OUTER_BOUND('',#25517,.T.);
#21418=FACE_OUTER_BOUND('',#25518,.T.);
#21419=FACE_OUTER_BOUND('',#25519,.T.);
#21420=FACE_OUTER_BOUND('',#25520,.T.);
#21421=FACE_OUTER_BOUND('',#25521,.T.);
#21422=FACE_OUTER_BOUND('',#25522,.T.);
#21423=FACE_OUTER_BOUND('',#25523,.T.);
#21424=FACE_OUTER_BOUND('',#25524,.T.);
#21425=FACE_OUTER_BOUND('',#25525,.T.);
#21426=FACE_OUTER_BOUND('',#25526,.T.);
#21427=FACE_OUTER_BOUND('',#25527,.T.);
#21428=FACE_OUTER_BOUND('',#25528,.T.);
#21429=FACE_OUTER_BOUND('',#25529,.T.);
#21430=FACE_OUTER_BOUND('',#25530,.T.);
#21431=FACE_OUTER_BOUND('',#25531,.T.);
#21432=FACE_OUTER_BOUND('',#25532,.T.);
#21433=FACE_OUTER_BOUND('',#25533,.T.);
#21434=FACE_OUTER_BOUND('',#25534,.T.);
#21435=FACE_OUTER_BOUND('',#25535,.T.);
#21436=FACE_OUTER_BOUND('',#25536,.T.);
#21437=FACE_OUTER_BOUND('',#25537,.T.);
#21438=FACE_OUTER_BOUND('',#25538,.T.);
#21439=FACE_OUTER_BOUND('',#25539,.T.);
#21440=FACE_OUTER_BOUND('',#25540,.T.);
#21441=FACE_OUTER_BOUND('',#25541,.T.);
#21442=FACE_OUTER_BOUND('',#25542,.T.);
#21443=FACE_OUTER_BOUND('',#25543,.T.);
#21444=FACE_OUTER_BOUND('',#25544,.T.);
#21445=FACE_OUTER_BOUND('',#25545,.T.);
#21446=FACE_OUTER_BOUND('',#25546,.T.);
#21447=FACE_OUTER_BOUND('',#25547,.T.);
#21448=FACE_OUTER_BOUND('',#25548,.T.);
#21449=FACE_OUTER_BOUND('',#25549,.T.);
#21450=FACE_OUTER_BOUND('',#25550,.T.);
#21451=FACE_OUTER_BOUND('',#25551,.T.);
#21452=FACE_OUTER_BOUND('',#25552,.T.);
#21453=FACE_OUTER_BOUND('',#25553,.T.);
#21454=FACE_OUTER_BOUND('',#25554,.T.);
#21455=FACE_OUTER_BOUND('',#25555,.T.);
#21456=FACE_OUTER_BOUND('',#25556,.T.);
#21457=FACE_OUTER_BOUND('',#25557,.T.);
#21458=FACE_OUTER_BOUND('',#25558,.T.);
#21459=FACE_OUTER_BOUND('',#25559,.T.);
#21460=FACE_OUTER_BOUND('',#25560,.T.);
#21461=FACE_OUTER_BOUND('',#25561,.T.);
#21462=FACE_OUTER_BOUND('',#25562,.T.);
#21463=FACE_OUTER_BOUND('',#25563,.T.);
#21464=FACE_OUTER_BOUND('',#25564,.T.);
#21465=FACE_OUTER_BOUND('',#25565,.T.);
#21466=FACE_OUTER_BOUND('',#25566,.T.);
#21467=FACE_OUTER_BOUND('',#25567,.T.);
#21468=FACE_OUTER_BOUND('',#25568,.T.);
#21469=FACE_OUTER_BOUND('',#25569,.T.);
#21470=FACE_OUTER_BOUND('',#25570,.T.);
#21471=FACE_OUTER_BOUND('',#25571,.T.);
#21472=FACE_OUTER_BOUND('',#25572,.T.);
#21473=FACE_OUTER_BOUND('',#25573,.T.);
#21474=FACE_OUTER_BOUND('',#25574,.T.);
#21475=FACE_OUTER_BOUND('',#25575,.T.);
#21476=FACE_OUTER_BOUND('',#25576,.T.);
#21477=FACE_OUTER_BOUND('',#25577,.T.);
#21478=FACE_OUTER_BOUND('',#25578,.T.);
#21479=FACE_OUTER_BOUND('',#25579,.T.);
#21480=FACE_OUTER_BOUND('',#25580,.T.);
#21481=FACE_OUTER_BOUND('',#25581,.T.);
#21482=FACE_OUTER_BOUND('',#25582,.T.);
#21483=FACE_OUTER_BOUND('',#25583,.T.);
#21484=FACE_OUTER_BOUND('',#25584,.T.);
#21485=FACE_OUTER_BOUND('',#25585,.T.);
#21486=FACE_OUTER_BOUND('',#25586,.T.);
#21487=FACE_OUTER_BOUND('',#25587,.T.);
#21488=FACE_OUTER_BOUND('',#25588,.T.);
#21489=FACE_OUTER_BOUND('',#25589,.T.);
#21490=FACE_OUTER_BOUND('',#25590,.T.);
#21491=FACE_OUTER_BOUND('',#25591,.T.);
#21492=FACE_OUTER_BOUND('',#25592,.T.);
#21493=FACE_OUTER_BOUND('',#25593,.T.);
#21494=FACE_OUTER_BOUND('',#25594,.T.);
#21495=FACE_OUTER_BOUND('',#25595,.T.);
#21496=FACE_OUTER_BOUND('',#25596,.T.);
#21497=FACE_OUTER_BOUND('',#25597,.T.);
#21498=FACE_OUTER_BOUND('',#25598,.T.);
#21499=FACE_OUTER_BOUND('',#25599,.T.);
#21500=FACE_OUTER_BOUND('',#25600,.T.);
#21501=FACE_OUTER_BOUND('',#25601,.T.);
#21502=FACE_OUTER_BOUND('',#25602,.T.);
#21503=FACE_OUTER_BOUND('',#25603,.T.);
#21504=FACE_OUTER_BOUND('',#25604,.T.);
#21505=FACE_OUTER_BOUND('',#25605,.T.);
#21506=FACE_OUTER_BOUND('',#25606,.T.);
#21507=FACE_OUTER_BOUND('',#25607,.T.);
#21508=FACE_OUTER_BOUND('',#25608,.T.);
#21509=FACE_OUTER_BOUND('',#25609,.T.);
#21510=FACE_OUTER_BOUND('',#25610,.T.);
#21511=FACE_OUTER_BOUND('',#25611,.T.);
#21512=FACE_OUTER_BOUND('',#25612,.T.);
#21513=FACE_OUTER_BOUND('',#25613,.T.);
#21514=FACE_OUTER_BOUND('',#25614,.T.);
#21515=FACE_OUTER_BOUND('',#25615,.T.);
#21516=FACE_OUTER_BOUND('',#25616,.T.);
#21517=FACE_OUTER_BOUND('',#25617,.T.);
#21518=FACE_OUTER_BOUND('',#25618,.T.);
#21519=FACE_OUTER_BOUND('',#25619,.T.);
#21520=FACE_OUTER_BOUND('',#25620,.T.);
#21521=FACE_OUTER_BOUND('',#25621,.T.);
#21522=FACE_OUTER_BOUND('',#25622,.T.);
#21523=FACE_OUTER_BOUND('',#25623,.T.);
#21524=FACE_OUTER_BOUND('',#25624,.T.);
#21525=FACE_OUTER_BOUND('',#25625,.T.);
#21526=FACE_OUTER_BOUND('',#25626,.T.);
#21527=FACE_OUTER_BOUND('',#25627,.T.);
#21528=FACE_OUTER_BOUND('',#25628,.T.);
#21529=FACE_OUTER_BOUND('',#25629,.T.);
#21530=FACE_OUTER_BOUND('',#25630,.T.);
#21531=FACE_OUTER_BOUND('',#25631,.T.);
#21532=FACE_OUTER_BOUND('',#25632,.T.);
#21533=FACE_OUTER_BOUND('',#25633,.T.);
#21534=FACE_OUTER_BOUND('',#25634,.T.);
#21535=FACE_OUTER_BOUND('',#25635,.T.);
#21536=FACE_OUTER_BOUND('',#25636,.T.);
#21537=FACE_OUTER_BOUND('',#25637,.T.);
#21538=FACE_OUTER_BOUND('',#25638,.T.);
#21539=FACE_OUTER_BOUND('',#25639,.T.);
#21540=FACE_OUTER_BOUND('',#25640,.T.);
#21541=FACE_OUTER_BOUND('',#25641,.T.);
#21542=FACE_OUTER_BOUND('',#25642,.T.);
#21543=FACE_OUTER_BOUND('',#25643,.T.);
#21544=FACE_OUTER_BOUND('',#25644,.T.);
#21545=FACE_OUTER_BOUND('',#25645,.T.);
#21546=FACE_OUTER_BOUND('',#25646,.T.);
#21547=FACE_OUTER_BOUND('',#25647,.T.);
#21548=FACE_OUTER_BOUND('',#25648,.T.);
#21549=FACE_OUTER_BOUND('',#25649,.T.);
#21550=FACE_OUTER_BOUND('',#25650,.T.);
#21551=FACE_OUTER_BOUND('',#25651,.T.);
#21552=FACE_OUTER_BOUND('',#25652,.T.);
#21553=FACE_OUTER_BOUND('',#25653,.T.);
#21554=FACE_OUTER_BOUND('',#25654,.T.);
#21555=FACE_OUTER_BOUND('',#25655,.T.);
#21556=FACE_OUTER_BOUND('',#25656,.T.);
#21557=FACE_OUTER_BOUND('',#25657,.T.);
#21558=FACE_OUTER_BOUND('',#25658,.T.);
#21559=FACE_OUTER_BOUND('',#25659,.T.);
#21560=FACE_OUTER_BOUND('',#25660,.T.);
#21561=FACE_OUTER_BOUND('',#25661,.T.);
#21562=FACE_OUTER_BOUND('',#25662,.T.);
#21563=FACE_OUTER_BOUND('',#25663,.T.);
#21564=FACE_OUTER_BOUND('',#25664,.T.);
#21565=FACE_OUTER_BOUND('',#25665,.T.);
#21566=FACE_OUTER_BOUND('',#25666,.T.);
#21567=FACE_OUTER_BOUND('',#25667,.T.);
#21568=FACE_OUTER_BOUND('',#25668,.T.);
#21569=FACE_OUTER_BOUND('',#25669,.T.);
#21570=FACE_OUTER_BOUND('',#25670,.T.);
#21571=FACE_OUTER_BOUND('',#25671,.T.);
#21572=FACE_OUTER_BOUND('',#25672,.T.);
#21573=FACE_OUTER_BOUND('',#25673,.T.);
#21574=FACE_OUTER_BOUND('',#25674,.T.);
#21575=FACE_OUTER_BOUND('',#25675,.T.);
#21576=FACE_OUTER_BOUND('',#25676,.T.);
#21577=FACE_OUTER_BOUND('',#25677,.T.);
#21578=FACE_OUTER_BOUND('',#25678,.T.);
#21579=FACE_OUTER_BOUND('',#25679,.T.);
#21580=FACE_OUTER_BOUND('',#25680,.T.);
#21581=FACE_OUTER_BOUND('',#25681,.T.);
#21582=FACE_OUTER_BOUND('',#25682,.T.);
#21583=FACE_OUTER_BOUND('',#25683,.T.);
#21584=FACE_OUTER_BOUND('',#25684,.T.);
#21585=FACE_OUTER_BOUND('',#25685,.T.);
#21586=FACE_OUTER_BOUND('',#25686,.T.);
#21587=FACE_OUTER_BOUND('',#25687,.T.);
#21588=FACE_OUTER_BOUND('',#25688,.T.);
#21589=FACE_OUTER_BOUND('',#25689,.T.);
#21590=FACE_OUTER_BOUND('',#25690,.T.);
#21591=FACE_OUTER_BOUND('',#25691,.T.);
#21592=FACE_OUTER_BOUND('',#25692,.T.);
#21593=FACE_OUTER_BOUND('',#25693,.T.);
#21594=FACE_OUTER_BOUND('',#25694,.T.);
#21595=FACE_OUTER_BOUND('',#25695,.T.);
#21596=FACE_OUTER_BOUND('',#25696,.T.);
#21597=FACE_OUTER_BOUND('',#25697,.T.);
#21598=FACE_OUTER_BOUND('',#25698,.T.);
#21599=FACE_OUTER_BOUND('',#25699,.T.);
#21600=FACE_OUTER_BOUND('',#25700,.T.);
#21601=FACE_OUTER_BOUND('',#25701,.T.);
#21602=FACE_OUTER_BOUND('',#25702,.T.);
#21603=FACE_OUTER_BOUND('',#25703,.T.);
#21604=FACE_OUTER_BOUND('',#25704,.T.);
#21605=FACE_OUTER_BOUND('',#25705,.T.);
#21606=FACE_OUTER_BOUND('',#25706,.T.);
#21607=FACE_OUTER_BOUND('',#25707,.T.);
#21608=FACE_OUTER_BOUND('',#25708,.T.);
#21609=FACE_OUTER_BOUND('',#25709,.T.);
#21610=FACE_OUTER_BOUND('',#25710,.T.);
#21611=FACE_OUTER_BOUND('',#25711,.T.);
#21612=FACE_OUTER_BOUND('',#25712,.T.);
#21613=FACE_OUTER_BOUND('',#25713,.T.);
#21614=FACE_OUTER_BOUND('',#25714,.T.);
#21615=FACE_OUTER_BOUND('',#25715,.T.);
#21616=FACE_OUTER_BOUND('',#25716,.T.);
#21617=FACE_OUTER_BOUND('',#25717,.T.);
#21618=FACE_OUTER_BOUND('',#25718,.T.);
#21619=FACE_OUTER_BOUND('',#25719,.T.);
#21620=FACE_OUTER_BOUND('',#25720,.T.);
#21621=FACE_OUTER_BOUND('',#25721,.T.);
#21622=FACE_OUTER_BOUND('',#25722,.T.);
#21623=FACE_OUTER_BOUND('',#25723,.T.);
#21624=FACE_OUTER_BOUND('',#25724,.T.);
#21625=FACE_OUTER_BOUND('',#25725,.T.);
#21626=FACE_OUTER_BOUND('',#25726,.T.);
#21627=FACE_OUTER_BOUND('',#25727,.T.);
#21628=FACE_OUTER_BOUND('',#25728,.T.);
#21629=FACE_OUTER_BOUND('',#25729,.T.);
#21630=FACE_OUTER_BOUND('',#25730,.T.);
#21631=FACE_OUTER_BOUND('',#25731,.T.);
#21632=FACE_OUTER_BOUND('',#25732,.T.);
#21633=FACE_OUTER_BOUND('',#25733,.T.);
#21634=FACE_OUTER_BOUND('',#25734,.T.);
#21635=FACE_OUTER_BOUND('',#25735,.T.);
#21636=FACE_OUTER_BOUND('',#25736,.T.);
#21637=FACE_OUTER_BOUND('',#25737,.T.);
#21638=FACE_OUTER_BOUND('',#25738,.T.);
#21639=FACE_OUTER_BOUND('',#25739,.T.);
#21640=FACE_OUTER_BOUND('',#25740,.T.);
#21641=FACE_OUTER_BOUND('',#25741,.T.);
#21642=FACE_OUTER_BOUND('',#25742,.T.);
#21643=FACE_OUTER_BOUND('',#25743,.T.);
#21644=FACE_OUTER_BOUND('',#25744,.T.);
#21645=FACE_OUTER_BOUND('',#25745,.T.);
#21646=FACE_OUTER_BOUND('',#25746,.T.);
#21647=FACE_OUTER_BOUND('',#25747,.T.);
#21648=FACE_OUTER_BOUND('',#25748,.T.);
#21649=FACE_OUTER_BOUND('',#25749,.T.);
#21650=FACE_OUTER_BOUND('',#25750,.T.);
#21651=FACE_OUTER_BOUND('',#25751,.T.);
#21652=FACE_OUTER_BOUND('',#25752,.T.);
#21653=FACE_OUTER_BOUND('',#25753,.T.);
#21654=FACE_OUTER_BOUND('',#25754,.T.);
#21655=FACE_OUTER_BOUND('',#25755,.T.);
#21656=FACE_OUTER_BOUND('',#25756,.T.);
#21657=FACE_OUTER_BOUND('',#25757,.T.);
#21658=FACE_OUTER_BOUND('',#25758,.T.);
#21659=FACE_OUTER_BOUND('',#25759,.T.);
#21660=FACE_OUTER_BOUND('',#25760,.T.);
#21661=FACE_OUTER_BOUND('',#25761,.T.);
#21662=FACE_OUTER_BOUND('',#25762,.T.);
#21663=FACE_OUTER_BOUND('',#25763,.T.);
#21664=FACE_OUTER_BOUND('',#25764,.T.);
#21665=FACE_OUTER_BOUND('',#25765,.T.);
#21666=FACE_OUTER_BOUND('',#25766,.T.);
#21667=FACE_OUTER_BOUND('',#25767,.T.);
#21668=FACE_OUTER_BOUND('',#25768,.T.);
#21669=FACE_OUTER_BOUND('',#25769,.T.);
#21670=FACE_OUTER_BOUND('',#25770,.T.);
#21671=FACE_OUTER_BOUND('',#25771,.T.);
#21672=FACE_OUTER_BOUND('',#25772,.T.);
#21673=FACE_OUTER_BOUND('',#25773,.T.);
#21674=FACE_OUTER_BOUND('',#25774,.T.);
#21675=FACE_OUTER_BOUND('',#25775,.T.);
#21676=FACE_OUTER_BOUND('',#25776,.T.);
#21677=FACE_OUTER_BOUND('',#25777,.T.);
#21678=FACE_OUTER_BOUND('',#25778,.T.);
#21679=FACE_OUTER_BOUND('',#25779,.T.);
#21680=FACE_OUTER_BOUND('',#25780,.T.);
#21681=FACE_OUTER_BOUND('',#25781,.T.);
#21682=FACE_OUTER_BOUND('',#25782,.T.);
#21683=FACE_OUTER_BOUND('',#25783,.T.);
#21684=FACE_OUTER_BOUND('',#25784,.T.);
#21685=FACE_OUTER_BOUND('',#25785,.T.);
#21686=FACE_OUTER_BOUND('',#25786,.T.);
#21687=FACE_OUTER_BOUND('',#25787,.T.);
#21688=FACE_OUTER_BOUND('',#25788,.T.);
#21689=FACE_OUTER_BOUND('',#25789,.T.);
#21690=FACE_OUTER_BOUND('',#25790,.T.);
#21691=FACE_OUTER_BOUND('',#25791,.T.);
#21692=FACE_OUTER_BOUND('',#25792,.T.);
#21693=FACE_OUTER_BOUND('',#25793,.T.);
#21694=FACE_OUTER_BOUND('',#25794,.T.);
#21695=FACE_OUTER_BOUND('',#25795,.T.);
#21696=FACE_OUTER_BOUND('',#25796,.T.);
#21697=FACE_OUTER_BOUND('',#25797,.T.);
#21698=FACE_OUTER_BOUND('',#25798,.T.);
#21699=FACE_OUTER_BOUND('',#25799,.T.);
#21700=FACE_OUTER_BOUND('',#25800,.T.);
#21701=FACE_OUTER_BOUND('',#25801,.T.);
#21702=FACE_OUTER_BOUND('',#25802,.T.);
#21703=FACE_OUTER_BOUND('',#25803,.T.);
#21704=FACE_OUTER_BOUND('',#25804,.T.);
#21705=FACE_OUTER_BOUND('',#25805,.T.);
#21706=FACE_OUTER_BOUND('',#25806,.T.);
#21707=FACE_OUTER_BOUND('',#25807,.T.);
#21708=FACE_OUTER_BOUND('',#25808,.T.);
#21709=FACE_OUTER_BOUND('',#25809,.T.);
#21710=FACE_OUTER_BOUND('',#25810,.T.);
#21711=FACE_OUTER_BOUND('',#25811,.T.);
#21712=FACE_OUTER_BOUND('',#25812,.T.);
#21713=FACE_OUTER_BOUND('',#25813,.T.);
#21714=FACE_OUTER_BOUND('',#25814,.T.);
#21715=FACE_OUTER_BOUND('',#25815,.T.);
#21716=FACE_OUTER_BOUND('',#25816,.T.);
#21717=FACE_OUTER_BOUND('',#25817,.T.);
#21718=FACE_OUTER_BOUND('',#25818,.T.);
#21719=FACE_OUTER_BOUND('',#25819,.T.);
#21720=FACE_OUTER_BOUND('',#25820,.T.);
#21721=FACE_OUTER_BOUND('',#25821,.T.);
#21722=FACE_OUTER_BOUND('',#25822,.T.);
#21723=FACE_OUTER_BOUND('',#25823,.T.);
#21724=FACE_OUTER_BOUND('',#25824,.T.);
#21725=FACE_OUTER_BOUND('',#25825,.T.);
#21726=FACE_OUTER_BOUND('',#25826,.T.);
#21727=FACE_OUTER_BOUND('',#25827,.T.);
#21728=FACE_OUTER_BOUND('',#25828,.T.);
#21729=FACE_OUTER_BOUND('',#25829,.T.);
#21730=FACE_OUTER_BOUND('',#25830,.T.);
#21731=FACE_OUTER_BOUND('',#25831,.T.);
#21732=FACE_OUTER_BOUND('',#25832,.T.);
#21733=FACE_OUTER_BOUND('',#25833,.T.);
#21734=FACE_OUTER_BOUND('',#25834,.T.);
#21735=FACE_OUTER_BOUND('',#25835,.T.);
#21736=FACE_OUTER_BOUND('',#25836,.T.);
#21737=FACE_OUTER_BOUND('',#25837,.T.);
#21738=FACE_OUTER_BOUND('',#25838,.T.);
#21739=FACE_OUTER_BOUND('',#25839,.T.);
#21740=FACE_OUTER_BOUND('',#25840,.T.);
#21741=FACE_OUTER_BOUND('',#25841,.T.);
#21742=FACE_OUTER_BOUND('',#25842,.T.);
#21743=FACE_OUTER_BOUND('',#25843,.T.);
#21744=FACE_OUTER_BOUND('',#25844,.T.);
#21745=FACE_OUTER_BOUND('',#25845,.T.);
#21746=FACE_OUTER_BOUND('',#25846,.T.);
#21747=FACE_OUTER_BOUND('',#25847,.T.);
#21748=FACE_OUTER_BOUND('',#25848,.T.);
#21749=FACE_OUTER_BOUND('',#25849,.T.);
#21750=FACE_OUTER_BOUND('',#25850,.T.);
#21751=FACE_OUTER_BOUND('',#25851,.T.);
#21752=FACE_OUTER_BOUND('',#25852,.T.);
#21753=FACE_OUTER_BOUND('',#25853,.T.);
#21754=FACE_OUTER_BOUND('',#25854,.T.);
#21755=FACE_OUTER_BOUND('',#25855,.T.);
#21756=FACE_OUTER_BOUND('',#25856,.T.);
#21757=FACE_OUTER_BOUND('',#25857,.T.);
#21758=FACE_OUTER_BOUND('',#25858,.T.);
#21759=FACE_OUTER_BOUND('',#25859,.T.);
#21760=FACE_OUTER_BOUND('',#25860,.T.);
#21761=FACE_OUTER_BOUND('',#25861,.T.);
#21762=FACE_OUTER_BOUND('',#25862,.T.);
#21763=FACE_OUTER_BOUND('',#25863,.T.);
#21764=FACE_OUTER_BOUND('',#25864,.T.);
#21765=FACE_OUTER_BOUND('',#25865,.T.);
#21766=FACE_OUTER_BOUND('',#25866,.T.);
#21767=FACE_OUTER_BOUND('',#25867,.T.);
#21768=FACE_OUTER_BOUND('',#25868,.T.);
#21769=FACE_OUTER_BOUND('',#25869,.T.);
#21770=FACE_OUTER_BOUND('',#25870,.T.);
#21771=FACE_OUTER_BOUND('',#25871,.T.);
#21772=FACE_OUTER_BOUND('',#25872,.T.);
#21773=FACE_OUTER_BOUND('',#25873,.T.);
#21774=FACE_OUTER_BOUND('',#25874,.T.);
#21775=FACE_OUTER_BOUND('',#25875,.T.);
#21776=FACE_OUTER_BOUND('',#25876,.T.);
#21777=FACE_OUTER_BOUND('',#25877,.T.);
#21778=FACE_OUTER_BOUND('',#25878,.T.);
#21779=FACE_OUTER_BOUND('',#25879,.T.);
#21780=FACE_OUTER_BOUND('',#25880,.T.);
#21781=FACE_OUTER_BOUND('',#25881,.T.);
#21782=FACE_OUTER_BOUND('',#25882,.T.);
#21783=FACE_OUTER_BOUND('',#25883,.T.);
#21784=FACE_OUTER_BOUND('',#25884,.T.);
#21785=FACE_OUTER_BOUND('',#25885,.T.);
#21786=FACE_OUTER_BOUND('',#25886,.T.);
#21787=FACE_OUTER_BOUND('',#25887,.T.);
#21788=FACE_OUTER_BOUND('',#25888,.T.);
#21789=FACE_OUTER_BOUND('',#25889,.T.);
#21790=FACE_OUTER_BOUND('',#25890,.T.);
#21791=FACE_OUTER_BOUND('',#25891,.T.);
#21792=FACE_OUTER_BOUND('',#25892,.T.);
#21793=FACE_OUTER_BOUND('',#25893,.T.);
#21794=FACE_OUTER_BOUND('',#25894,.T.);
#21795=FACE_OUTER_BOUND('',#25895,.T.);
#21796=FACE_OUTER_BOUND('',#25896,.T.);
#21797=FACE_OUTER_BOUND('',#25897,.T.);
#21798=FACE_OUTER_BOUND('',#25898,.T.);
#21799=FACE_OUTER_BOUND('',#25899,.T.);
#21800=FACE_OUTER_BOUND('',#25900,.T.);
#21801=FACE_OUTER_BOUND('',#25901,.T.);
#21802=FACE_OUTER_BOUND('',#25902,.T.);
#21803=FACE_OUTER_BOUND('',#25903,.T.);
#21804=FACE_OUTER_BOUND('',#25904,.T.);
#21805=FACE_OUTER_BOUND('',#25905,.T.);
#21806=FACE_OUTER_BOUND('',#25906,.T.);
#21807=FACE_OUTER_BOUND('',#25907,.T.);
#21808=FACE_OUTER_BOUND('',#25908,.T.);
#21809=FACE_OUTER_BOUND('',#25909,.T.);
#21810=FACE_OUTER_BOUND('',#25910,.T.);
#21811=FACE_OUTER_BOUND('',#25911,.T.);
#21812=FACE_OUTER_BOUND('',#25912,.T.);
#21813=FACE_OUTER_BOUND('',#25913,.T.);
#21814=FACE_OUTER_BOUND('',#25914,.T.);
#21815=FACE_OUTER_BOUND('',#25915,.T.);
#21816=FACE_OUTER_BOUND('',#25916,.T.);
#21817=FACE_OUTER_BOUND('',#25917,.T.);
#21818=FACE_OUTER_BOUND('',#25918,.T.);
#21819=FACE_OUTER_BOUND('',#25919,.T.);
#21820=FACE_OUTER_BOUND('',#25920,.T.);
#21821=FACE_OUTER_BOUND('',#25921,.T.);
#21822=FACE_OUTER_BOUND('',#25922,.T.);
#21823=FACE_OUTER_BOUND('',#25923,.T.);
#21824=FACE_OUTER_BOUND('',#25924,.T.);
#21825=FACE_OUTER_BOUND('',#25925,.T.);
#21826=FACE_OUTER_BOUND('',#25926,.T.);
#21827=FACE_OUTER_BOUND('',#25927,.T.);
#21828=FACE_OUTER_BOUND('',#25928,.T.);
#21829=FACE_OUTER_BOUND('',#25929,.T.);
#21830=FACE_OUTER_BOUND('',#25930,.T.);
#21831=FACE_OUTER_BOUND('',#25931,.T.);
#21832=FACE_OUTER_BOUND('',#25932,.T.);
#21833=FACE_OUTER_BOUND('',#25933,.T.);
#21834=FACE_OUTER_BOUND('',#25934,.T.);
#21835=FACE_OUTER_BOUND('',#25935,.T.);
#21836=FACE_OUTER_BOUND('',#25936,.T.);
#21837=FACE_OUTER_BOUND('',#25937,.T.);
#21838=FACE_OUTER_BOUND('',#25938,.T.);
#21839=FACE_OUTER_BOUND('',#25939,.T.);
#21840=FACE_OUTER_BOUND('',#25940,.T.);
#21841=FACE_OUTER_BOUND('',#25941,.T.);
#21842=FACE_OUTER_BOUND('',#25942,.T.);
#21843=FACE_OUTER_BOUND('',#25943,.T.);
#21844=FACE_OUTER_BOUND('',#25944,.T.);
#21845=FACE_OUTER_BOUND('',#25945,.T.);
#21846=FACE_OUTER_BOUND('',#25946,.T.);
#21847=FACE_OUTER_BOUND('',#25947,.T.);
#21848=FACE_OUTER_BOUND('',#25948,.T.);
#21849=FACE_OUTER_BOUND('',#25949,.T.);
#21850=FACE_OUTER_BOUND('',#25950,.T.);
#21851=FACE_OUTER_BOUND('',#25951,.T.);
#21852=FACE_OUTER_BOUND('',#25952,.T.);
#21853=FACE_OUTER_BOUND('',#25953,.T.);
#21854=FACE_OUTER_BOUND('',#25954,.T.);
#21855=FACE_OUTER_BOUND('',#25955,.T.);
#21856=FACE_OUTER_BOUND('',#25956,.T.);
#21857=FACE_OUTER_BOUND('',#25957,.T.);
#21858=FACE_OUTER_BOUND('',#25958,.T.);
#21859=FACE_OUTER_BOUND('',#25959,.T.);
#21860=FACE_OUTER_BOUND('',#25960,.T.);
#21861=FACE_OUTER_BOUND('',#25961,.T.);
#21862=FACE_OUTER_BOUND('',#25962,.T.);
#21863=FACE_OUTER_BOUND('',#25963,.T.);
#21864=FACE_OUTER_BOUND('',#25964,.T.);
#21865=FACE_OUTER_BOUND('',#25965,.T.);
#21866=FACE_OUTER_BOUND('',#25966,.T.);
#21867=FACE_OUTER_BOUND('',#25967,.T.);
#21868=FACE_OUTER_BOUND('',#25968,.T.);
#21869=FACE_OUTER_BOUND('',#25969,.T.);
#21870=FACE_OUTER_BOUND('',#25970,.T.);
#21871=FACE_OUTER_BOUND('',#25971,.T.);
#21872=FACE_OUTER_BOUND('',#25972,.T.);
#21873=FACE_OUTER_BOUND('',#25973,.T.);
#21874=FACE_OUTER_BOUND('',#25974,.T.);
#21875=FACE_OUTER_BOUND('',#25975,.T.);
#21876=FACE_OUTER_BOUND('',#25976,.T.);
#21877=FACE_OUTER_BOUND('',#25977,.T.);
#21878=FACE_OUTER_BOUND('',#25978,.T.);
#21879=FACE_OUTER_BOUND('',#25979,.T.);
#21880=FACE_OUTER_BOUND('',#25980,.T.);
#21881=FACE_OUTER_BOUND('',#25981,.T.);
#21882=FACE_OUTER_BOUND('',#25982,.T.);
#21883=FACE_OUTER_BOUND('',#25983,.T.);
#21884=FACE_OUTER_BOUND('',#25984,.T.);
#21885=FACE_OUTER_BOUND('',#25985,.T.);
#21886=FACE_OUTER_BOUND('',#25986,.T.);
#21887=FACE_OUTER_BOUND('',#25987,.T.);
#21888=FACE_OUTER_BOUND('',#25988,.T.);
#21889=FACE_OUTER_BOUND('',#25989,.T.);
#21890=FACE_OUTER_BOUND('',#25990,.T.);
#21891=FACE_OUTER_BOUND('',#25991,.T.);
#21892=FACE_OUTER_BOUND('',#25992,.T.);
#21893=FACE_OUTER_BOUND('',#25993,.T.);
#21894=FACE_OUTER_BOUND('',#25994,.T.);
#21895=FACE_OUTER_BOUND('',#25995,.T.);
#21896=FACE_OUTER_BOUND('',#25996,.T.);
#21897=FACE_OUTER_BOUND('',#25997,.T.);
#21898=FACE_OUTER_BOUND('',#25998,.T.);
#21899=FACE_OUTER_BOUND('',#25999,.T.);
#21900=FACE_OUTER_BOUND('',#26000,.T.);
#21901=FACE_OUTER_BOUND('',#26001,.T.);
#21902=FACE_OUTER_BOUND('',#26002,.T.);
#21903=FACE_OUTER_BOUND('',#26003,.T.);
#21904=FACE_OUTER_BOUND('',#26004,.T.);
#21905=FACE_OUTER_BOUND('',#26005,.T.);
#21906=FACE_OUTER_BOUND('',#26006,.T.);
#21907=FACE_OUTER_BOUND('',#26007,.T.);
#21908=FACE_OUTER_BOUND('',#26008,.T.);
#21909=FACE_OUTER_BOUND('',#26009,.T.);
#21910=FACE_OUTER_BOUND('',#26010,.T.);
#21911=FACE_OUTER_BOUND('',#26011,.T.);
#21912=FACE_OUTER_BOUND('',#26012,.T.);
#21913=FACE_OUTER_BOUND('',#26013,.T.);
#21914=FACE_OUTER_BOUND('',#26014,.T.);
#21915=FACE_OUTER_BOUND('',#26015,.T.);
#21916=FACE_OUTER_BOUND('',#26016,.T.);
#21917=FACE_OUTER_BOUND('',#26017,.T.);
#21918=FACE_OUTER_BOUND('',#26018,.T.);
#21919=FACE_OUTER_BOUND('',#26019,.T.);
#21920=FACE_OUTER_BOUND('',#26020,.T.);
#21921=FACE_OUTER_BOUND('',#26021,.T.);
#21922=FACE_OUTER_BOUND('',#26022,.T.);
#21923=FACE_OUTER_BOUND('',#26023,.T.);
#21924=FACE_OUTER_BOUND('',#26024,.T.);
#21925=FACE_OUTER_BOUND('',#26025,.T.);
#21926=FACE_OUTER_BOUND('',#26026,.T.);
#21927=FACE_OUTER_BOUND('',#26027,.T.);
#21928=FACE_OUTER_BOUND('',#26028,.T.);
#21929=FACE_OUTER_BOUND('',#26029,.T.);
#21930=FACE_OUTER_BOUND('',#26030,.T.);
#21931=FACE_OUTER_BOUND('',#26031,.T.);
#21932=FACE_OUTER_BOUND('',#26032,.T.);
#21933=FACE_OUTER_BOUND('',#26033,.T.);
#21934=FACE_OUTER_BOUND('',#26034,.T.);
#21935=FACE_OUTER_BOUND('',#26035,.T.);
#21936=FACE_OUTER_BOUND('',#26036,.T.);
#21937=FACE_OUTER_BOUND('',#26037,.T.);
#21938=FACE_OUTER_BOUND('',#26038,.T.);
#21939=FACE_OUTER_BOUND('',#26039,.T.);
#21940=FACE_OUTER_BOUND('',#26040,.T.);
#21941=FACE_OUTER_BOUND('',#26041,.T.);
#21942=FACE_OUTER_BOUND('',#26042,.T.);
#21943=FACE_OUTER_BOUND('',#26043,.T.);
#21944=FACE_OUTER_BOUND('',#26044,.T.);
#21945=FACE_OUTER_BOUND('',#26045,.T.);
#21946=FACE_OUTER_BOUND('',#26046,.T.);
#21947=FACE_OUTER_BOUND('',#26047,.T.);
#21948=FACE_OUTER_BOUND('',#26048,.T.);
#21949=FACE_OUTER_BOUND('',#26049,.T.);
#21950=FACE_OUTER_BOUND('',#26050,.T.);
#21951=FACE_OUTER_BOUND('',#26051,.T.);
#21952=FACE_OUTER_BOUND('',#26052,.T.);
#21953=FACE_OUTER_BOUND('',#26053,.T.);
#21954=FACE_OUTER_BOUND('',#26054,.T.);
#21955=FACE_OUTER_BOUND('',#26055,.T.);
#21956=FACE_OUTER_BOUND('',#26057,.T.);
#21957=FACE_OUTER_BOUND('',#26058,.T.);
#21958=FACE_OUTER_BOUND('',#26059,.T.);
#21959=FACE_OUTER_BOUND('',#26060,.T.);
#21960=FACE_OUTER_BOUND('',#26061,.T.);
#21961=FACE_OUTER_BOUND('',#26062,.T.);
#21962=FACE_OUTER_BOUND('',#26063,.T.);
#21963=FACE_OUTER_BOUND('',#26064,.T.);
#21964=FACE_OUTER_BOUND('',#26065,.T.);
#21965=FACE_OUTER_BOUND('',#26066,.T.);
#21966=FACE_OUTER_BOUND('',#26067,.T.);
#21967=FACE_OUTER_BOUND('',#26068,.T.);
#21968=FACE_OUTER_BOUND('',#26069,.T.);
#21969=FACE_OUTER_BOUND('',#26070,.T.);
#21970=FACE_OUTER_BOUND('',#26071,.T.);
#21971=FACE_OUTER_BOUND('',#26072,.T.);
#21972=FACE_OUTER_BOUND('',#26073,.T.);
#21973=FACE_OUTER_BOUND('',#26074,.T.);
#21974=FACE_OUTER_BOUND('',#26075,.T.);
#21975=FACE_OUTER_BOUND('',#26076,.T.);
#21976=FACE_OUTER_BOUND('',#26077,.T.);
#21977=FACE_OUTER_BOUND('',#26078,.T.);
#21978=FACE_OUTER_BOUND('',#26079,.T.);
#21979=FACE_OUTER_BOUND('',#26080,.T.);
#21980=FACE_OUTER_BOUND('',#26081,.T.);
#21981=FACE_OUTER_BOUND('',#26082,.T.);
#21982=FACE_OUTER_BOUND('',#26083,.T.);
#21983=FACE_OUTER_BOUND('',#26084,.T.);
#21984=FACE_OUTER_BOUND('',#26085,.T.);
#21985=FACE_OUTER_BOUND('',#26086,.T.);
#21986=FACE_OUTER_BOUND('',#26087,.T.);
#21987=FACE_OUTER_BOUND('',#26088,.T.);
#21988=FACE_OUTER_BOUND('',#26089,.T.);
#21989=FACE_OUTER_BOUND('',#26090,.T.);
#21990=FACE_OUTER_BOUND('',#26091,.T.);
#21991=FACE_OUTER_BOUND('',#26092,.T.);
#21992=FACE_OUTER_BOUND('',#26093,.T.);
#21993=FACE_OUTER_BOUND('',#26094,.T.);
#21994=FACE_OUTER_BOUND('',#26095,.T.);
#21995=FACE_OUTER_BOUND('',#26096,.T.);
#21996=FACE_OUTER_BOUND('',#26097,.T.);
#21997=FACE_OUTER_BOUND('',#26098,.T.);
#21998=FACE_OUTER_BOUND('',#26099,.T.);
#21999=FACE_OUTER_BOUND('',#26100,.T.);
#22000=FACE_OUTER_BOUND('',#26101,.T.);
#22001=FACE_OUTER_BOUND('',#26102,.T.);
#22002=FACE_OUTER_BOUND('',#26103,.T.);
#22003=FACE_OUTER_BOUND('',#26104,.T.);
#22004=FACE_OUTER_BOUND('',#26105,.T.);
#22005=FACE_OUTER_BOUND('',#26106,.T.);
#22006=FACE_OUTER_BOUND('',#26107,.T.);
#22007=FACE_OUTER_BOUND('',#26108,.T.);
#22008=FACE_OUTER_BOUND('',#26109,.T.);
#22009=FACE_OUTER_BOUND('',#26110,.T.);
#22010=FACE_OUTER_BOUND('',#26111,.T.);
#22011=FACE_OUTER_BOUND('',#26112,.T.);
#22012=FACE_OUTER_BOUND('',#26113,.T.);
#22013=FACE_OUTER_BOUND('',#26114,.T.);
#22014=FACE_OUTER_BOUND('',#26115,.T.);
#22015=FACE_OUTER_BOUND('',#26116,.T.);
#22016=FACE_OUTER_BOUND('',#26117,.T.);
#22017=FACE_OUTER_BOUND('',#26118,.T.);
#22018=FACE_OUTER_BOUND('',#26119,.T.);
#22019=FACE_OUTER_BOUND('',#26120,.T.);
#22020=FACE_OUTER_BOUND('',#26121,.T.);
#22021=FACE_OUTER_BOUND('',#26122,.T.);
#22022=FACE_OUTER_BOUND('',#26123,.T.);
#22023=FACE_OUTER_BOUND('',#26124,.T.);
#22024=FACE_OUTER_BOUND('',#26125,.T.);
#22025=FACE_OUTER_BOUND('',#26126,.T.);
#22026=FACE_OUTER_BOUND('',#26127,.T.);
#22027=FACE_OUTER_BOUND('',#26128,.T.);
#22028=FACE_OUTER_BOUND('',#26129,.T.);
#22029=FACE_OUTER_BOUND('',#26130,.T.);
#22030=FACE_OUTER_BOUND('',#26131,.T.);
#22031=FACE_OUTER_BOUND('',#26132,.T.);
#22032=FACE_OUTER_BOUND('',#26133,.T.);
#22033=FACE_OUTER_BOUND('',#26134,.T.);
#22034=FACE_OUTER_BOUND('',#26135,.T.);
#22035=FACE_OUTER_BOUND('',#26136,.T.);
#22036=FACE_OUTER_BOUND('',#26137,.T.);
#22037=FACE_OUTER_BOUND('',#26138,.T.);
#22038=FACE_OUTER_BOUND('',#26139,.T.);
#22039=FACE_OUTER_BOUND('',#26140,.T.);
#22040=FACE_OUTER_BOUND('',#26141,.T.);
#22041=FACE_OUTER_BOUND('',#26142,.T.);
#22042=FACE_OUTER_BOUND('',#26143,.T.);
#22043=FACE_OUTER_BOUND('',#26144,.T.);
#22044=FACE_OUTER_BOUND('',#26145,.T.);
#22045=FACE_OUTER_BOUND('',#26146,.T.);
#22046=FACE_OUTER_BOUND('',#26147,.T.);
#22047=FACE_OUTER_BOUND('',#26148,.T.);
#22048=FACE_OUTER_BOUND('',#26149,.T.);
#22049=FACE_OUTER_BOUND('',#26150,.T.);
#22050=FACE_OUTER_BOUND('',#26151,.T.);
#22051=FACE_OUTER_BOUND('',#26152,.T.);
#22052=FACE_OUTER_BOUND('',#26153,.T.);
#22053=FACE_OUTER_BOUND('',#26154,.T.);
#22054=FACE_OUTER_BOUND('',#26155,.T.);
#22055=FACE_OUTER_BOUND('',#26156,.T.);
#22056=FACE_OUTER_BOUND('',#26157,.T.);
#22057=FACE_OUTER_BOUND('',#26158,.T.);
#22058=FACE_OUTER_BOUND('',#26159,.T.);
#22059=FACE_OUTER_BOUND('',#26160,.T.);
#22060=FACE_OUTER_BOUND('',#26161,.T.);
#22061=FACE_OUTER_BOUND('',#26162,.T.);
#22062=FACE_OUTER_BOUND('',#26163,.T.);
#22063=FACE_OUTER_BOUND('',#26164,.T.);
#22064=FACE_OUTER_BOUND('',#26165,.T.);
#22065=FACE_OUTER_BOUND('',#26166,.T.);
#22066=FACE_OUTER_BOUND('',#26167,.T.);
#22067=FACE_OUTER_BOUND('',#26168,.T.);
#22068=FACE_OUTER_BOUND('',#26169,.T.);
#22069=FACE_OUTER_BOUND('',#26170,.T.);
#22070=FACE_OUTER_BOUND('',#26171,.T.);
#22071=FACE_OUTER_BOUND('',#26172,.T.);
#22072=FACE_OUTER_BOUND('',#26173,.T.);
#22073=FACE_OUTER_BOUND('',#26174,.T.);
#22074=FACE_OUTER_BOUND('',#26175,.T.);
#22075=FACE_OUTER_BOUND('',#26176,.T.);
#22076=FACE_OUTER_BOUND('',#26177,.T.);
#22077=FACE_OUTER_BOUND('',#26178,.T.);
#22078=FACE_OUTER_BOUND('',#26179,.T.);
#22079=FACE_OUTER_BOUND('',#26180,.T.);
#22080=FACE_OUTER_BOUND('',#26181,.T.);
#22081=FACE_OUTER_BOUND('',#26182,.T.);
#22082=FACE_OUTER_BOUND('',#26183,.T.);
#22083=FACE_OUTER_BOUND('',#26184,.T.);
#22084=FACE_OUTER_BOUND('',#26185,.T.);
#22085=FACE_OUTER_BOUND('',#26186,.T.);
#22086=FACE_OUTER_BOUND('',#26187,.T.);
#22087=FACE_OUTER_BOUND('',#26188,.T.);
#22088=FACE_OUTER_BOUND('',#26189,.T.);
#22089=FACE_OUTER_BOUND('',#26190,.T.);
#22090=FACE_OUTER_BOUND('',#26191,.T.);
#22091=FACE_OUTER_BOUND('',#26192,.T.);
#22092=FACE_OUTER_BOUND('',#26193,.T.);
#22093=FACE_OUTER_BOUND('',#26194,.T.);
#22094=FACE_OUTER_BOUND('',#26195,.T.);
#22095=FACE_OUTER_BOUND('',#26196,.T.);
#22096=FACE_OUTER_BOUND('',#26197,.T.);
#22097=FACE_OUTER_BOUND('',#26198,.T.);
#22098=FACE_OUTER_BOUND('',#26199,.T.);
#22099=FACE_OUTER_BOUND('',#26200,.T.);
#22100=FACE_OUTER_BOUND('',#26201,.T.);
#22101=FACE_OUTER_BOUND('',#26202,.T.);
#22102=FACE_OUTER_BOUND('',#26203,.T.);
#22103=FACE_OUTER_BOUND('',#26204,.T.);
#22104=FACE_OUTER_BOUND('',#26205,.T.);
#22105=FACE_OUTER_BOUND('',#26206,.T.);
#22106=FACE_OUTER_BOUND('',#26207,.T.);
#22107=FACE_OUTER_BOUND('',#26208,.T.);
#22108=FACE_OUTER_BOUND('',#26209,.T.);
#22109=FACE_OUTER_BOUND('',#26210,.T.);
#22110=FACE_OUTER_BOUND('',#26211,.T.);
#22111=FACE_OUTER_BOUND('',#26212,.T.);
#22112=FACE_OUTER_BOUND('',#26213,.T.);
#22113=FACE_OUTER_BOUND('',#26214,.T.);
#22114=FACE_OUTER_BOUND('',#26215,.T.);
#22115=FACE_OUTER_BOUND('',#26216,.T.);
#22116=FACE_OUTER_BOUND('',#26217,.T.);
#22117=FACE_OUTER_BOUND('',#26218,.T.);
#22118=FACE_OUTER_BOUND('',#26219,.T.);
#22119=FACE_OUTER_BOUND('',#26220,.T.);
#22120=FACE_OUTER_BOUND('',#26221,.T.);
#22121=FACE_OUTER_BOUND('',#26222,.T.);
#22122=FACE_OUTER_BOUND('',#26223,.T.);
#22123=FACE_OUTER_BOUND('',#26224,.T.);
#22124=FACE_OUTER_BOUND('',#26225,.T.);
#22125=FACE_OUTER_BOUND('',#26226,.T.);
#22126=FACE_OUTER_BOUND('',#26227,.T.);
#22127=FACE_OUTER_BOUND('',#26228,.T.);
#22128=FACE_OUTER_BOUND('',#26229,.T.);
#22129=FACE_OUTER_BOUND('',#26230,.T.);
#22130=FACE_OUTER_BOUND('',#26231,.T.);
#22131=FACE_OUTER_BOUND('',#26232,.T.);
#22132=FACE_OUTER_BOUND('',#26233,.T.);
#22133=FACE_OUTER_BOUND('',#26234,.T.);
#22134=FACE_OUTER_BOUND('',#26235,.T.);
#22135=FACE_OUTER_BOUND('',#26236,.T.);
#22136=FACE_OUTER_BOUND('',#26237,.T.);
#22137=FACE_OUTER_BOUND('',#26238,.T.);
#22138=FACE_OUTER_BOUND('',#26239,.T.);
#22139=FACE_OUTER_BOUND('',#26240,.T.);
#22140=FACE_OUTER_BOUND('',#26241,.T.);
#22141=FACE_OUTER_BOUND('',#26242,.T.);
#22142=FACE_OUTER_BOUND('',#26243,.T.);
#22143=FACE_OUTER_BOUND('',#26244,.T.);
#22144=FACE_OUTER_BOUND('',#26245,.T.);
#22145=FACE_OUTER_BOUND('',#26246,.T.);
#22146=FACE_OUTER_BOUND('',#26247,.T.);
#22147=FACE_OUTER_BOUND('',#26248,.T.);
#22148=FACE_OUTER_BOUND('',#26249,.T.);
#22149=FACE_OUTER_BOUND('',#26250,.T.);
#22150=FACE_OUTER_BOUND('',#26251,.T.);
#22151=FACE_OUTER_BOUND('',#26252,.T.);
#22152=FACE_OUTER_BOUND('',#26253,.T.);
#22153=FACE_OUTER_BOUND('',#26254,.T.);
#22154=FACE_OUTER_BOUND('',#26255,.T.);
#22155=FACE_OUTER_BOUND('',#26256,.T.);
#22156=FACE_OUTER_BOUND('',#26257,.T.);
#22157=FACE_OUTER_BOUND('',#26258,.T.);
#22158=FACE_OUTER_BOUND('',#26259,.T.);
#22159=FACE_OUTER_BOUND('',#26260,.T.);
#22160=FACE_OUTER_BOUND('',#26261,.T.);
#22161=FACE_OUTER_BOUND('',#26262,.T.);
#22162=FACE_OUTER_BOUND('',#26263,.T.);
#22163=FACE_OUTER_BOUND('',#26264,.T.);
#22164=FACE_OUTER_BOUND('',#26265,.T.);
#22165=FACE_OUTER_BOUND('',#26266,.T.);
#22166=FACE_OUTER_BOUND('',#26267,.T.);
#22167=FACE_OUTER_BOUND('',#26268,.T.);
#22168=FACE_OUTER_BOUND('',#26269,.T.);
#22169=FACE_OUTER_BOUND('',#26270,.T.);
#22170=FACE_OUTER_BOUND('',#26271,.T.);
#22171=FACE_OUTER_BOUND('',#26272,.T.);
#22172=FACE_OUTER_BOUND('',#26273,.T.);
#22173=FACE_OUTER_BOUND('',#26274,.T.);
#22174=FACE_OUTER_BOUND('',#26275,.T.);
#22175=FACE_OUTER_BOUND('',#26276,.T.);
#22176=FACE_OUTER_BOUND('',#26277,.T.);
#22177=FACE_OUTER_BOUND('',#26278,.T.);
#22178=FACE_OUTER_BOUND('',#26279,.T.);
#22179=FACE_OUTER_BOUND('',#26280,.T.);
#22180=FACE_OUTER_BOUND('',#26281,.T.);
#22181=FACE_OUTER_BOUND('',#26282,.T.);
#22182=FACE_OUTER_BOUND('',#26283,.T.);
#22183=FACE_OUTER_BOUND('',#26284,.T.);
#22184=FACE_OUTER_BOUND('',#26285,.T.);
#22185=FACE_OUTER_BOUND('',#26286,.T.);
#22186=FACE_OUTER_BOUND('',#26287,.T.);
#22187=FACE_OUTER_BOUND('',#26288,.T.);
#22188=FACE_OUTER_BOUND('',#26289,.T.);
#22189=FACE_OUTER_BOUND('',#26290,.T.);
#22190=FACE_OUTER_BOUND('',#26291,.T.);
#22191=FACE_OUTER_BOUND('',#26292,.T.);
#22192=FACE_OUTER_BOUND('',#26293,.T.);
#22193=FACE_OUTER_BOUND('',#26294,.T.);
#22194=FACE_OUTER_BOUND('',#26295,.T.);
#22195=FACE_OUTER_BOUND('',#26296,.T.);
#22196=FACE_OUTER_BOUND('',#26297,.T.);
#22197=FACE_OUTER_BOUND('',#26298,.T.);
#22198=FACE_OUTER_BOUND('',#26299,.T.);
#22199=FACE_OUTER_BOUND('',#26300,.T.);
#22200=FACE_OUTER_BOUND('',#26301,.T.);
#22201=FACE_OUTER_BOUND('',#26302,.T.);
#22202=FACE_OUTER_BOUND('',#26303,.T.);
#22203=FACE_OUTER_BOUND('',#26304,.T.);
#22204=FACE_OUTER_BOUND('',#26305,.T.);
#22205=FACE_OUTER_BOUND('',#26306,.T.);
#22206=FACE_OUTER_BOUND('',#26307,.T.);
#22207=FACE_OUTER_BOUND('',#26308,.T.);
#22208=FACE_OUTER_BOUND('',#26309,.T.);
#22209=FACE_OUTER_BOUND('',#26310,.T.);
#22210=FACE_OUTER_BOUND('',#26311,.T.);
#22211=FACE_OUTER_BOUND('',#26312,.T.);
#22212=FACE_OUTER_BOUND('',#26313,.T.);
#22213=FACE_OUTER_BOUND('',#26314,.T.);
#22214=FACE_OUTER_BOUND('',#26315,.T.);
#22215=FACE_OUTER_BOUND('',#26316,.T.);
#22216=FACE_OUTER_BOUND('',#26317,.T.);
#22217=FACE_OUTER_BOUND('',#26318,.T.);
#22218=FACE_OUTER_BOUND('',#26319,.T.);
#22219=FACE_OUTER_BOUND('',#26320,.T.);
#22220=FACE_OUTER_BOUND('',#26321,.T.);
#22221=FACE_OUTER_BOUND('',#26322,.T.);
#22222=FACE_OUTER_BOUND('',#26323,.T.);
#22223=FACE_OUTER_BOUND('',#26324,.T.);
#22224=FACE_OUTER_BOUND('',#26325,.T.);
#22225=FACE_OUTER_BOUND('',#26326,.T.);
#22226=FACE_OUTER_BOUND('',#26327,.T.);
#22227=FACE_OUTER_BOUND('',#26328,.T.);
#22228=FACE_OUTER_BOUND('',#26329,.T.);
#22229=FACE_OUTER_BOUND('',#26330,.T.);
#22230=FACE_OUTER_BOUND('',#26331,.T.);
#22231=FACE_OUTER_BOUND('',#26332,.T.);
#22232=FACE_OUTER_BOUND('',#26333,.T.);
#22233=FACE_OUTER_BOUND('',#26334,.T.);
#22234=FACE_OUTER_BOUND('',#26335,.T.);
#22235=FACE_OUTER_BOUND('',#26336,.T.);
#22236=FACE_OUTER_BOUND('',#26337,.T.);
#22237=FACE_OUTER_BOUND('',#26338,.T.);
#22238=FACE_OUTER_BOUND('',#26339,.T.);
#22239=FACE_OUTER_BOUND('',#26340,.T.);
#22240=FACE_OUTER_BOUND('',#26341,.T.);
#22241=FACE_OUTER_BOUND('',#26342,.T.);
#22242=FACE_OUTER_BOUND('',#26343,.T.);
#22243=FACE_OUTER_BOUND('',#26344,.T.);
#22244=FACE_OUTER_BOUND('',#26345,.T.);
#22245=FACE_OUTER_BOUND('',#26346,.T.);
#22246=FACE_OUTER_BOUND('',#26347,.T.);
#22247=FACE_OUTER_BOUND('',#26348,.T.);
#22248=FACE_OUTER_BOUND('',#26349,.T.);
#22249=FACE_OUTER_BOUND('',#26350,.T.);
#22250=FACE_OUTER_BOUND('',#26351,.T.);
#22251=FACE_OUTER_BOUND('',#26352,.T.);
#22252=FACE_OUTER_BOUND('',#26353,.T.);
#22253=FACE_OUTER_BOUND('',#26354,.T.);
#22254=FACE_OUTER_BOUND('',#26355,.T.);
#22255=FACE_OUTER_BOUND('',#26356,.T.);
#22256=FACE_OUTER_BOUND('',#26357,.T.);
#22257=FACE_OUTER_BOUND('',#26358,.T.);
#22258=FACE_OUTER_BOUND('',#26359,.T.);
#22259=FACE_OUTER_BOUND('',#26360,.T.);
#22260=FACE_OUTER_BOUND('',#26361,.T.);
#22261=FACE_OUTER_BOUND('',#26362,.T.);
#22262=FACE_OUTER_BOUND('',#26363,.T.);
#22263=FACE_OUTER_BOUND('',#26364,.T.);
#22264=FACE_OUTER_BOUND('',#26365,.T.);
#22265=FACE_OUTER_BOUND('',#26366,.T.);
#22266=FACE_OUTER_BOUND('',#26367,.T.);
#22267=FACE_OUTER_BOUND('',#26368,.T.);
#22268=FACE_OUTER_BOUND('',#26369,.T.);
#22269=FACE_OUTER_BOUND('',#26370,.T.);
#22270=FACE_OUTER_BOUND('',#26371,.T.);
#22271=FACE_OUTER_BOUND('',#26372,.T.);
#22272=FACE_OUTER_BOUND('',#26373,.T.);
#22273=FACE_OUTER_BOUND('',#26374,.T.);
#22274=FACE_OUTER_BOUND('',#26375,.T.);
#22275=FACE_OUTER_BOUND('',#26376,.T.);
#22276=FACE_OUTER_BOUND('',#26377,.T.);
#22277=FACE_OUTER_BOUND('',#26378,.T.);
#22278=FACE_OUTER_BOUND('',#26379,.T.);
#22279=FACE_OUTER_BOUND('',#26380,.T.);
#22280=FACE_OUTER_BOUND('',#26381,.T.);
#22281=FACE_OUTER_BOUND('',#26382,.T.);
#22282=FACE_OUTER_BOUND('',#26383,.T.);
#22283=FACE_OUTER_BOUND('',#26384,.T.);
#22284=FACE_OUTER_BOUND('',#26385,.T.);
#22285=FACE_OUTER_BOUND('',#26386,.T.);
#22286=FACE_OUTER_BOUND('',#26387,.T.);
#22287=FACE_OUTER_BOUND('',#26388,.T.);
#22288=FACE_OUTER_BOUND('',#26389,.T.);
#22289=FACE_OUTER_BOUND('',#26390,.T.);
#22290=FACE_OUTER_BOUND('',#26391,.T.);
#22291=FACE_OUTER_BOUND('',#26392,.T.);
#22292=FACE_OUTER_BOUND('',#26393,.T.);
#22293=FACE_OUTER_BOUND('',#26394,.T.);
#22294=FACE_OUTER_BOUND('',#26395,.T.);
#22295=FACE_OUTER_BOUND('',#26396,.T.);
#22296=FACE_OUTER_BOUND('',#26397,.T.);
#22297=FACE_OUTER_BOUND('',#26398,.T.);
#22298=FACE_OUTER_BOUND('',#26399,.T.);
#22299=FACE_OUTER_BOUND('',#26400,.T.);
#22300=FACE_OUTER_BOUND('',#26401,.T.);
#22301=FACE_OUTER_BOUND('',#26402,.T.);
#22302=FACE_OUTER_BOUND('',#26403,.T.);
#22303=FACE_OUTER_BOUND('',#26404,.T.);
#22304=FACE_OUTER_BOUND('',#26405,.T.);
#22305=FACE_OUTER_BOUND('',#26406,.T.);
#22306=FACE_OUTER_BOUND('',#26407,.T.);
#22307=FACE_OUTER_BOUND('',#26408,.T.);
#22308=FACE_OUTER_BOUND('',#26409,.T.);
#22309=FACE_OUTER_BOUND('',#26410,.T.);
#22310=FACE_OUTER_BOUND('',#26411,.T.);
#22311=FACE_OUTER_BOUND('',#26412,.T.);
#22312=FACE_OUTER_BOUND('',#26413,.T.);
#22313=FACE_OUTER_BOUND('',#26414,.T.);
#22314=FACE_OUTER_BOUND('',#26415,.T.);
#22315=FACE_OUTER_BOUND('',#26416,.T.);
#22316=FACE_OUTER_BOUND('',#26417,.T.);
#22317=FACE_OUTER_BOUND('',#26418,.T.);
#22318=FACE_OUTER_BOUND('',#26419,.T.);
#22319=FACE_OUTER_BOUND('',#26420,.T.);
#22320=FACE_OUTER_BOUND('',#26421,.T.);
#22321=FACE_OUTER_BOUND('',#26422,.T.);
#22322=FACE_OUTER_BOUND('',#26423,.T.);
#22323=FACE_OUTER_BOUND('',#26424,.T.);
#22324=FACE_OUTER_BOUND('',#26425,.T.);
#22325=FACE_OUTER_BOUND('',#26426,.T.);
#22326=FACE_OUTER_BOUND('',#26427,.T.);
#22327=FACE_OUTER_BOUND('',#26428,.T.);
#22328=FACE_OUTER_BOUND('',#26429,.T.);
#22329=FACE_OUTER_BOUND('',#26430,.T.);
#22330=FACE_OUTER_BOUND('',#26431,.T.);
#22331=FACE_OUTER_BOUND('',#26432,.T.);
#22332=FACE_OUTER_BOUND('',#26433,.T.);
#22333=FACE_OUTER_BOUND('',#26434,.T.);
#22334=FACE_OUTER_BOUND('',#26435,.T.);
#22335=FACE_OUTER_BOUND('',#26436,.T.);
#22336=FACE_OUTER_BOUND('',#26437,.T.);
#22337=FACE_OUTER_BOUND('',#26438,.T.);
#22338=FACE_OUTER_BOUND('',#26439,.T.);
#22339=FACE_OUTER_BOUND('',#26440,.T.);
#22340=FACE_OUTER_BOUND('',#26441,.T.);
#22341=FACE_OUTER_BOUND('',#26442,.T.);
#22342=FACE_OUTER_BOUND('',#26443,.T.);
#22343=FACE_OUTER_BOUND('',#26444,.T.);
#22344=FACE_OUTER_BOUND('',#26445,.T.);
#22345=FACE_OUTER_BOUND('',#26446,.T.);
#22346=FACE_OUTER_BOUND('',#26447,.T.);
#22347=FACE_OUTER_BOUND('',#26448,.T.);
#22348=FACE_OUTER_BOUND('',#26449,.T.);
#22349=FACE_OUTER_BOUND('',#26450,.T.);
#22350=FACE_OUTER_BOUND('',#26451,.T.);
#22351=FACE_OUTER_BOUND('',#26452,.T.);
#22352=FACE_OUTER_BOUND('',#26453,.T.);
#22353=FACE_OUTER_BOUND('',#26454,.T.);
#22354=FACE_OUTER_BOUND('',#26455,.T.);
#22355=FACE_OUTER_BOUND('',#26456,.T.);
#22356=FACE_OUTER_BOUND('',#26457,.T.);
#22357=FACE_OUTER_BOUND('',#26458,.T.);
#22358=FACE_OUTER_BOUND('',#26459,.T.);
#22359=FACE_OUTER_BOUND('',#26460,.T.);
#22360=FACE_OUTER_BOUND('',#26461,.T.);
#22361=FACE_OUTER_BOUND('',#26462,.T.);
#22362=FACE_OUTER_BOUND('',#26463,.T.);
#22363=FACE_OUTER_BOUND('',#26464,.T.);
#22364=FACE_OUTER_BOUND('',#26465,.T.);
#22365=FACE_OUTER_BOUND('',#26466,.T.);
#22366=FACE_OUTER_BOUND('',#26467,.T.);
#22367=FACE_OUTER_BOUND('',#26468,.T.);
#22368=FACE_OUTER_BOUND('',#26469,.T.);
#22369=FACE_OUTER_BOUND('',#26470,.T.);
#22370=FACE_OUTER_BOUND('',#26471,.T.);
#22371=FACE_OUTER_BOUND('',#26472,.T.);
#22372=FACE_OUTER_BOUND('',#26473,.T.);
#22373=FACE_OUTER_BOUND('',#26474,.T.);
#22374=FACE_OUTER_BOUND('',#26475,.T.);
#22375=FACE_OUTER_BOUND('',#26476,.T.);
#22376=FACE_OUTER_BOUND('',#26477,.T.);
#22377=FACE_OUTER_BOUND('',#26478,.T.);
#22378=FACE_OUTER_BOUND('',#26479,.T.);
#22379=FACE_OUTER_BOUND('',#26480,.T.);
#22380=FACE_OUTER_BOUND('',#26481,.T.);
#22381=FACE_OUTER_BOUND('',#26482,.T.);
#22382=FACE_OUTER_BOUND('',#26483,.T.);
#22383=FACE_OUTER_BOUND('',#26484,.T.);
#22384=FACE_OUTER_BOUND('',#26485,.T.);
#22385=FACE_OUTER_BOUND('',#26486,.T.);
#22386=FACE_OUTER_BOUND('',#26487,.T.);
#22387=FACE_OUTER_BOUND('',#26488,.T.);
#22388=FACE_OUTER_BOUND('',#26489,.T.);
#22389=FACE_OUTER_BOUND('',#26490,.T.);
#22390=FACE_OUTER_BOUND('',#26491,.T.);
#22391=FACE_OUTER_BOUND('',#26492,.T.);
#22392=FACE_OUTER_BOUND('',#26493,.T.);
#22393=FACE_OUTER_BOUND('',#26494,.T.);
#22394=FACE_OUTER_BOUND('',#26495,.T.);
#22395=FACE_OUTER_BOUND('',#26496,.T.);
#22396=FACE_OUTER_BOUND('',#26497,.T.);
#22397=FACE_OUTER_BOUND('',#26498,.T.);
#22398=FACE_OUTER_BOUND('',#26499,.T.);
#22399=FACE_OUTER_BOUND('',#26500,.T.);
#22400=FACE_OUTER_BOUND('',#26501,.T.);
#22401=FACE_OUTER_BOUND('',#26502,.T.);
#22402=FACE_OUTER_BOUND('',#26503,.T.);
#22403=FACE_OUTER_BOUND('',#26504,.T.);
#22404=FACE_OUTER_BOUND('',#26505,.T.);
#22405=FACE_OUTER_BOUND('',#26506,.T.);
#22406=FACE_OUTER_BOUND('',#26507,.T.);
#22407=FACE_OUTER_BOUND('',#26508,.T.);
#22408=FACE_OUTER_BOUND('',#26509,.T.);
#22409=FACE_OUTER_BOUND('',#26510,.T.);
#22410=FACE_OUTER_BOUND('',#26511,.T.);
#22411=FACE_OUTER_BOUND('',#26512,.T.);
#22412=FACE_OUTER_BOUND('',#26513,.T.);
#22413=FACE_OUTER_BOUND('',#26514,.T.);
#22414=FACE_OUTER_BOUND('',#26515,.T.);
#22415=FACE_OUTER_BOUND('',#26516,.T.);
#22416=FACE_OUTER_BOUND('',#26517,.T.);
#22417=FACE_OUTER_BOUND('',#26518,.T.);
#22418=FACE_OUTER_BOUND('',#26519,.T.);
#22419=FACE_OUTER_BOUND('',#26520,.T.);
#22420=FACE_OUTER_BOUND('',#26521,.T.);
#22421=FACE_OUTER_BOUND('',#26522,.T.);
#22422=FACE_OUTER_BOUND('',#26523,.T.);
#22423=FACE_OUTER_BOUND('',#26524,.T.);
#22424=FACE_OUTER_BOUND('',#26525,.T.);
#22425=FACE_OUTER_BOUND('',#26526,.T.);
#22426=FACE_OUTER_BOUND('',#26527,.T.);
#22427=FACE_OUTER_BOUND('',#26528,.T.);
#22428=FACE_OUTER_BOUND('',#26529,.T.);
#22429=FACE_OUTER_BOUND('',#26530,.T.);
#22430=FACE_OUTER_BOUND('',#26531,.T.);
#22431=FACE_OUTER_BOUND('',#26532,.T.);
#22432=FACE_OUTER_BOUND('',#26533,.T.);
#22433=FACE_OUTER_BOUND('',#26534,.T.);
#22434=FACE_OUTER_BOUND('',#26535,.T.);
#22435=FACE_OUTER_BOUND('',#26536,.T.);
#22436=FACE_OUTER_BOUND('',#26537,.T.);
#22437=FACE_OUTER_BOUND('',#26538,.T.);
#22438=FACE_OUTER_BOUND('',#26539,.T.);
#22439=FACE_OUTER_BOUND('',#26540,.T.);
#22440=FACE_OUTER_BOUND('',#26541,.T.);
#22441=FACE_OUTER_BOUND('',#26542,.T.);
#22442=FACE_OUTER_BOUND('',#26543,.T.);
#22443=FACE_OUTER_BOUND('',#26544,.T.);
#22444=FACE_OUTER_BOUND('',#26545,.T.);
#22445=FACE_OUTER_BOUND('',#26546,.T.);
#22446=FACE_OUTER_BOUND('',#26547,.T.);
#22447=FACE_OUTER_BOUND('',#26548,.T.);
#22448=FACE_OUTER_BOUND('',#26549,.T.);
#22449=FACE_OUTER_BOUND('',#26550,.T.);
#22450=FACE_OUTER_BOUND('',#26551,.T.);
#22451=FACE_OUTER_BOUND('',#26552,.T.);
#22452=FACE_OUTER_BOUND('',#26553,.T.);
#22453=FACE_OUTER_BOUND('',#26554,.T.);
#22454=FACE_OUTER_BOUND('',#26555,.T.);
#22455=FACE_OUTER_BOUND('',#26556,.T.);
#22456=FACE_OUTER_BOUND('',#26557,.T.);
#22457=FACE_OUTER_BOUND('',#26558,.T.);
#22458=FACE_OUTER_BOUND('',#26559,.T.);
#22459=FACE_OUTER_BOUND('',#26560,.T.);
#22460=FACE_OUTER_BOUND('',#26561,.T.);
#22461=FACE_OUTER_BOUND('',#26562,.T.);
#22462=FACE_OUTER_BOUND('',#26563,.T.);
#22463=FACE_OUTER_BOUND('',#26564,.T.);
#22464=FACE_OUTER_BOUND('',#26565,.T.);
#22465=FACE_OUTER_BOUND('',#26566,.T.);
#22466=FACE_OUTER_BOUND('',#26567,.T.);
#22467=FACE_OUTER_BOUND('',#26568,.T.);
#22468=FACE_OUTER_BOUND('',#26569,.T.);
#22469=FACE_OUTER_BOUND('',#26570,.T.);
#22470=FACE_OUTER_BOUND('',#26571,.T.);
#22471=FACE_OUTER_BOUND('',#26572,.T.);
#22472=FACE_OUTER_BOUND('',#26573,.T.);
#22473=FACE_OUTER_BOUND('',#26574,.T.);
#22474=FACE_OUTER_BOUND('',#26575,.T.);
#22475=FACE_OUTER_BOUND('',#26576,.T.);
#22476=FACE_OUTER_BOUND('',#26577,.T.);
#22477=FACE_OUTER_BOUND('',#26578,.T.);
#22478=FACE_OUTER_BOUND('',#26579,.T.);
#22479=FACE_OUTER_BOUND('',#26580,.T.);
#22480=FACE_OUTER_BOUND('',#26581,.T.);
#22481=FACE_OUTER_BOUND('',#26582,.T.);
#22482=FACE_OUTER_BOUND('',#26583,.T.);
#22483=FACE_OUTER_BOUND('',#26584,.T.);
#22484=FACE_OUTER_BOUND('',#26585,.T.);
#22485=FACE_OUTER_BOUND('',#26586,.T.);
#22486=FACE_OUTER_BOUND('',#26587,.T.);
#22487=FACE_OUTER_BOUND('',#26588,.T.);
#22488=FACE_OUTER_BOUND('',#26589,.T.);
#22489=FACE_OUTER_BOUND('',#26590,.T.);
#22490=FACE_OUTER_BOUND('',#26591,.T.);
#22491=FACE_OUTER_BOUND('',#26592,.T.);
#22492=FACE_OUTER_BOUND('',#26593,.T.);
#22493=FACE_OUTER_BOUND('',#26594,.T.);
#22494=FACE_OUTER_BOUND('',#26595,.T.);
#22495=FACE_OUTER_BOUND('',#26596,.T.);
#22496=FACE_OUTER_BOUND('',#26597,.T.);
#22497=FACE_OUTER_BOUND('',#26598,.T.);
#22498=FACE_OUTER_BOUND('',#26599,.T.);
#22499=FACE_OUTER_BOUND('',#26600,.T.);
#22500=FACE_OUTER_BOUND('',#26601,.T.);
#22501=FACE_OUTER_BOUND('',#26602,.T.);
#22502=FACE_OUTER_BOUND('',#26603,.T.);
#22503=FACE_OUTER_BOUND('',#26604,.T.);
#22504=FACE_OUTER_BOUND('',#26605,.T.);
#22505=FACE_OUTER_BOUND('',#26606,.T.);
#22506=FACE_OUTER_BOUND('',#26607,.T.);
#22507=FACE_OUTER_BOUND('',#26608,.T.);
#22508=FACE_OUTER_BOUND('',#26609,.T.);
#22509=FACE_OUTER_BOUND('',#26610,.T.);
#22510=FACE_OUTER_BOUND('',#26611,.T.);
#22511=FACE_OUTER_BOUND('',#26612,.T.);
#22512=FACE_OUTER_BOUND('',#26613,.T.);
#22513=FACE_OUTER_BOUND('',#26614,.T.);
#22514=FACE_OUTER_BOUND('',#26615,.T.);
#22515=FACE_OUTER_BOUND('',#26616,.T.);
#22516=FACE_OUTER_BOUND('',#26617,.T.);
#22517=FACE_OUTER_BOUND('',#26618,.T.);
#22518=FACE_OUTER_BOUND('',#26619,.T.);
#22519=FACE_OUTER_BOUND('',#26620,.T.);
#22520=FACE_OUTER_BOUND('',#26621,.T.);
#22521=FACE_OUTER_BOUND('',#26622,.T.);
#22522=FACE_OUTER_BOUND('',#26623,.T.);
#22523=FACE_OUTER_BOUND('',#26624,.T.);
#22524=FACE_OUTER_BOUND('',#26625,.T.);
#22525=FACE_OUTER_BOUND('',#26626,.T.);
#22526=FACE_OUTER_BOUND('',#26627,.T.);
#22527=FACE_OUTER_BOUND('',#26628,.T.);
#22528=FACE_OUTER_BOUND('',#26629,.T.);
#22529=FACE_OUTER_BOUND('',#26630,.T.);
#22530=FACE_OUTER_BOUND('',#26631,.T.);
#22531=FACE_OUTER_BOUND('',#26632,.T.);
#22532=FACE_OUTER_BOUND('',#26633,.T.);
#22533=FACE_OUTER_BOUND('',#26634,.T.);
#22534=FACE_OUTER_BOUND('',#26635,.T.);
#22535=FACE_OUTER_BOUND('',#26636,.T.);
#22536=FACE_OUTER_BOUND('',#26637,.T.);
#22537=FACE_OUTER_BOUND('',#26638,.T.);
#22538=FACE_OUTER_BOUND('',#26639,.T.);
#22539=FACE_OUTER_BOUND('',#26640,.T.);
#22540=FACE_OUTER_BOUND('',#26641,.T.);
#22541=FACE_OUTER_BOUND('',#26642,.T.);
#22542=FACE_OUTER_BOUND('',#26643,.T.);
#22543=FACE_OUTER_BOUND('',#26644,.T.);
#22544=FACE_OUTER_BOUND('',#26645,.T.);
#22545=FACE_OUTER_BOUND('',#26646,.T.);
#22546=FACE_OUTER_BOUND('',#26647,.T.);
#22547=FACE_OUTER_BOUND('',#26648,.T.);
#22548=FACE_OUTER_BOUND('',#26649,.T.);
#22549=FACE_OUTER_BOUND('',#26650,.T.);
#22550=FACE_OUTER_BOUND('',#26651,.T.);
#22551=FACE_OUTER_BOUND('',#26652,.T.);
#22552=FACE_OUTER_BOUND('',#26653,.T.);
#22553=FACE_OUTER_BOUND('',#26654,.T.);
#22554=FACE_OUTER_BOUND('',#26655,.T.);
#22555=FACE_OUTER_BOUND('',#26656,.T.);
#22556=FACE_OUTER_BOUND('',#26657,.T.);
#22557=FACE_OUTER_BOUND('',#26658,.T.);
#22558=FACE_OUTER_BOUND('',#26659,.T.);
#22559=FACE_OUTER_BOUND('',#26660,.T.);
#22560=FACE_OUTER_BOUND('',#26661,.T.);
#22561=FACE_OUTER_BOUND('',#26662,.T.);
#22562=FACE_OUTER_BOUND('',#26663,.T.);
#22563=FACE_OUTER_BOUND('',#26664,.T.);
#22564=FACE_OUTER_BOUND('',#26665,.T.);
#22565=FACE_OUTER_BOUND('',#26666,.T.);
#22566=FACE_OUTER_BOUND('',#26667,.T.);
#22567=FACE_OUTER_BOUND('',#26668,.T.);
#22568=FACE_OUTER_BOUND('',#26669,.T.);
#22569=FACE_OUTER_BOUND('',#26670,.T.);
#22570=FACE_OUTER_BOUND('',#26671,.T.);
#22571=FACE_OUTER_BOUND('',#26672,.T.);
#22572=FACE_OUTER_BOUND('',#26673,.T.);
#22573=FACE_OUTER_BOUND('',#26674,.T.);
#22574=FACE_OUTER_BOUND('',#26675,.T.);
#22575=FACE_OUTER_BOUND('',#26676,.T.);
#22576=FACE_OUTER_BOUND('',#26677,.T.);
#22577=FACE_OUTER_BOUND('',#26678,.T.);
#22578=FACE_OUTER_BOUND('',#26679,.T.);
#22579=FACE_OUTER_BOUND('',#26680,.T.);
#22580=FACE_OUTER_BOUND('',#26681,.T.);
#22581=FACE_OUTER_BOUND('',#26682,.T.);
#22582=FACE_OUTER_BOUND('',#26683,.T.);
#22583=FACE_OUTER_BOUND('',#26684,.T.);
#22584=FACE_OUTER_BOUND('',#26685,.T.);
#22585=FACE_OUTER_BOUND('',#26686,.T.);
#22586=FACE_OUTER_BOUND('',#26687,.T.);
#22587=FACE_OUTER_BOUND('',#26688,.T.);
#22588=FACE_OUTER_BOUND('',#26689,.T.);
#22589=FACE_OUTER_BOUND('',#26690,.T.);
#22590=FACE_OUTER_BOUND('',#26691,.T.);
#22591=FACE_OUTER_BOUND('',#26692,.T.);
#22592=FACE_OUTER_BOUND('',#26693,.T.);
#22593=FACE_OUTER_BOUND('',#26694,.T.);
#22594=FACE_OUTER_BOUND('',#26695,.T.);
#22595=FACE_OUTER_BOUND('',#26696,.T.);
#22596=FACE_OUTER_BOUND('',#26697,.T.);
#22597=FACE_OUTER_BOUND('',#26698,.T.);
#22598=FACE_OUTER_BOUND('',#26699,.T.);
#22599=FACE_OUTER_BOUND('',#26700,.T.);
#22600=FACE_OUTER_BOUND('',#26701,.T.);
#22601=FACE_OUTER_BOUND('',#26702,.T.);
#22602=FACE_OUTER_BOUND('',#26703,.T.);
#22603=FACE_OUTER_BOUND('',#26704,.T.);
#22604=FACE_OUTER_BOUND('',#26705,.T.);
#22605=FACE_OUTER_BOUND('',#26706,.T.);
#22606=FACE_OUTER_BOUND('',#26707,.T.);
#22607=FACE_OUTER_BOUND('',#26708,.T.);
#22608=FACE_OUTER_BOUND('',#26709,.T.);
#22609=FACE_OUTER_BOUND('',#26710,.T.);
#22610=FACE_OUTER_BOUND('',#26711,.T.);
#22611=FACE_OUTER_BOUND('',#26712,.T.);
#22612=FACE_OUTER_BOUND('',#26713,.T.);
#22613=FACE_OUTER_BOUND('',#26714,.T.);
#22614=FACE_OUTER_BOUND('',#26715,.T.);
#22615=FACE_OUTER_BOUND('',#26716,.T.);
#22616=FACE_OUTER_BOUND('',#26717,.T.);
#22617=FACE_OUTER_BOUND('',#26718,.T.);
#22618=FACE_OUTER_BOUND('',#26719,.T.);
#22619=FACE_OUTER_BOUND('',#26720,.T.);
#22620=FACE_OUTER_BOUND('',#26721,.T.);
#22621=FACE_OUTER_BOUND('',#26722,.T.);
#22622=FACE_OUTER_BOUND('',#26723,.T.);
#22623=FACE_OUTER_BOUND('',#26724,.T.);
#22624=FACE_OUTER_BOUND('',#26725,.T.);
#22625=FACE_OUTER_BOUND('',#26726,.T.);
#22626=FACE_OUTER_BOUND('',#26727,.T.);
#22627=FACE_OUTER_BOUND('',#26728,.T.);
#22628=FACE_OUTER_BOUND('',#26729,.T.);
#22629=FACE_OUTER_BOUND('',#26730,.T.);
#22630=FACE_OUTER_BOUND('',#26731,.T.);
#22631=FACE_OUTER_BOUND('',#26732,.T.);
#22632=FACE_OUTER_BOUND('',#26733,.T.);
#22633=FACE_OUTER_BOUND('',#26734,.T.);
#22634=FACE_OUTER_BOUND('',#26735,.T.);
#22635=FACE_OUTER_BOUND('',#26736,.T.);
#22636=FACE_OUTER_BOUND('',#26737,.T.);
#22637=FACE_OUTER_BOUND('',#26738,.T.);
#22638=FACE_OUTER_BOUND('',#26739,.T.);
#22639=FACE_OUTER_BOUND('',#26740,.T.);
#22640=FACE_OUTER_BOUND('',#26741,.T.);
#22641=FACE_OUTER_BOUND('',#26742,.T.);
#22642=FACE_OUTER_BOUND('',#26743,.T.);
#22643=FACE_OUTER_BOUND('',#26744,.T.);
#22644=FACE_OUTER_BOUND('',#26745,.T.);
#22645=FACE_OUTER_BOUND('',#26746,.T.);
#22646=FACE_OUTER_BOUND('',#26747,.T.);
#22647=FACE_OUTER_BOUND('',#26748,.T.);
#22648=FACE_OUTER_BOUND('',#26749,.T.);
#22649=FACE_OUTER_BOUND('',#26750,.T.);
#22650=FACE_OUTER_BOUND('',#26751,.T.);
#22651=FACE_OUTER_BOUND('',#26752,.T.);
#22652=FACE_OUTER_BOUND('',#26753,.T.);
#22653=FACE_OUTER_BOUND('',#26754,.T.);
#22654=FACE_OUTER_BOUND('',#26755,.T.);
#22655=FACE_OUTER_BOUND('',#26756,.T.);
#22656=FACE_OUTER_BOUND('',#26757,.T.);
#22657=FACE_OUTER_BOUND('',#26758,.T.);
#22658=FACE_OUTER_BOUND('',#26759,.T.);
#22659=FACE_OUTER_BOUND('',#26760,.T.);
#22660=FACE_OUTER_BOUND('',#26761,.T.);
#22661=FACE_OUTER_BOUND('',#26762,.T.);
#22662=FACE_OUTER_BOUND('',#26763,.T.);
#22663=FACE_OUTER_BOUND('',#26764,.T.);
#22664=FACE_OUTER_BOUND('',#26765,.T.);
#22665=FACE_OUTER_BOUND('',#26766,.T.);
#22666=FACE_OUTER_BOUND('',#26767,.T.);
#22667=FACE_OUTER_BOUND('',#26768,.T.);
#22668=FACE_OUTER_BOUND('',#26769,.T.);
#22669=FACE_OUTER_BOUND('',#26770,.T.);
#22670=FACE_OUTER_BOUND('',#26771,.T.);
#22671=FACE_OUTER_BOUND('',#26772,.T.);
#22672=FACE_OUTER_BOUND('',#26773,.T.);
#22673=FACE_OUTER_BOUND('',#26774,.T.);
#22674=FACE_OUTER_BOUND('',#26775,.T.);
#22675=FACE_OUTER_BOUND('',#26776,.T.);
#22676=FACE_OUTER_BOUND('',#26777,.T.);
#22677=FACE_OUTER_BOUND('',#26778,.T.);
#22678=FACE_OUTER_BOUND('',#26779,.T.);
#22679=FACE_OUTER_BOUND('',#26780,.T.);
#22680=FACE_OUTER_BOUND('',#26781,.T.);
#22681=FACE_OUTER_BOUND('',#26782,.T.);
#22682=FACE_OUTER_BOUND('',#26783,.T.);
#22683=FACE_OUTER_BOUND('',#26784,.T.);
#22684=FACE_OUTER_BOUND('',#26785,.T.);
#22685=FACE_OUTER_BOUND('',#26786,.T.);
#22686=FACE_OUTER_BOUND('',#26787,.T.);
#22687=FACE_OUTER_BOUND('',#26788,.T.);
#22688=FACE_OUTER_BOUND('',#26789,.T.);
#22689=FACE_OUTER_BOUND('',#26790,.T.);
#22690=FACE_OUTER_BOUND('',#26791,.T.);
#22691=FACE_OUTER_BOUND('',#26792,.T.);
#22692=FACE_OUTER_BOUND('',#26793,.T.);
#22693=FACE_OUTER_BOUND('',#26794,.T.);
#22694=FACE_OUTER_BOUND('',#26795,.T.);
#22695=FACE_OUTER_BOUND('',#26796,.T.);
#22696=FACE_OUTER_BOUND('',#26797,.T.);
#22697=FACE_OUTER_BOUND('',#26798,.T.);
#22698=FACE_OUTER_BOUND('',#26799,.T.);
#22699=FACE_OUTER_BOUND('',#26800,.T.);
#22700=FACE_OUTER_BOUND('',#26801,.T.);
#22701=FACE_OUTER_BOUND('',#26802,.T.);
#22702=FACE_OUTER_BOUND('',#26803,.T.);
#22703=FACE_OUTER_BOUND('',#26804,.T.);
#22704=FACE_OUTER_BOUND('',#26805,.T.);
#22705=FACE_OUTER_BOUND('',#26806,.T.);
#22706=FACE_OUTER_BOUND('',#26807,.T.);
#22707=FACE_OUTER_BOUND('',#26808,.T.);
#22708=FACE_OUTER_BOUND('',#26809,.T.);
#22709=FACE_OUTER_BOUND('',#26810,.T.);
#22710=FACE_OUTER_BOUND('',#26811,.T.);
#22711=FACE_OUTER_BOUND('',#26812,.T.);
#22712=FACE_OUTER_BOUND('',#26813,.T.);
#22713=FACE_OUTER_BOUND('',#26814,.T.);
#22714=FACE_OUTER_BOUND('',#26815,.T.);
#22715=FACE_OUTER_BOUND('',#26816,.T.);
#22716=FACE_OUTER_BOUND('',#26817,.T.);
#22717=FACE_OUTER_BOUND('',#26818,.T.);
#22718=FACE_OUTER_BOUND('',#26819,.T.);
#22719=FACE_OUTER_BOUND('',#26820,.T.);
#22720=FACE_OUTER_BOUND('',#26821,.T.);
#22721=FACE_OUTER_BOUND('',#26822,.T.);
#22722=FACE_OUTER_BOUND('',#26823,.T.);
#22723=FACE_OUTER_BOUND('',#26824,.T.);
#22724=FACE_OUTER_BOUND('',#26825,.T.);
#22725=FACE_OUTER_BOUND('',#26826,.T.);
#22726=FACE_OUTER_BOUND('',#26827,.T.);
#22727=FACE_OUTER_BOUND('',#26828,.T.);
#22728=FACE_OUTER_BOUND('',#26829,.T.);
#22729=FACE_OUTER_BOUND('',#26830,.T.);
#22730=FACE_OUTER_BOUND('',#26831,.T.);
#22731=FACE_OUTER_BOUND('',#26832,.T.);
#22732=FACE_OUTER_BOUND('',#26833,.T.);
#22733=FACE_OUTER_BOUND('',#26834,.T.);
#22734=FACE_OUTER_BOUND('',#26835,.T.);
#22735=FACE_OUTER_BOUND('',#26836,.T.);
#22736=FACE_OUTER_BOUND('',#26837,.T.);
#22737=FACE_OUTER_BOUND('',#26838,.T.);
#22738=FACE_OUTER_BOUND('',#26839,.T.);
#22739=FACE_OUTER_BOUND('',#26840,.T.);
#22740=FACE_OUTER_BOUND('',#26841,.T.);
#22741=FACE_OUTER_BOUND('',#26842,.T.);
#22742=FACE_OUTER_BOUND('',#26843,.T.);
#22743=FACE_OUTER_BOUND('',#26844,.T.);
#22744=FACE_OUTER_BOUND('',#26845,.T.);
#22745=FACE_OUTER_BOUND('',#26846,.T.);
#22746=FACE_OUTER_BOUND('',#26847,.T.);
#22747=FACE_OUTER_BOUND('',#26848,.T.);
#22748=FACE_OUTER_BOUND('',#26849,.T.);
#22749=FACE_OUTER_BOUND('',#26850,.T.);
#22750=FACE_OUTER_BOUND('',#26851,.T.);
#22751=FACE_OUTER_BOUND('',#26852,.T.);
#22752=FACE_OUTER_BOUND('',#26853,.T.);
#22753=FACE_OUTER_BOUND('',#26854,.T.);
#22754=FACE_OUTER_BOUND('',#26855,.T.);
#22755=FACE_OUTER_BOUND('',#26856,.T.);
#22756=FACE_OUTER_BOUND('',#26857,.T.);
#22757=FACE_OUTER_BOUND('',#26858,.T.);
#22758=FACE_OUTER_BOUND('',#26859,.T.);
#22759=FACE_OUTER_BOUND('',#26860,.T.);
#22760=FACE_OUTER_BOUND('',#26861,.T.);
#22761=FACE_OUTER_BOUND('',#26862,.T.);
#22762=FACE_OUTER_BOUND('',#26863,.T.);
#22763=FACE_OUTER_BOUND('',#26864,.T.);
#22764=FACE_OUTER_BOUND('',#26865,.T.);
#22765=FACE_OUTER_BOUND('',#26866,.T.);
#22766=FACE_OUTER_BOUND('',#26867,.T.);
#22767=FACE_OUTER_BOUND('',#26868,.T.);
#22768=FACE_OUTER_BOUND('',#26869,.T.);
#22769=FACE_OUTER_BOUND('',#26870,.T.);
#22770=FACE_OUTER_BOUND('',#26871,.T.);
#22771=FACE_OUTER_BOUND('',#26872,.T.);
#22772=FACE_OUTER_BOUND('',#26873,.T.);
#22773=FACE_OUTER_BOUND('',#26874,.T.);
#22774=FACE_OUTER_BOUND('',#26875,.T.);
#22775=FACE_OUTER_BOUND('',#26876,.T.);
#22776=FACE_OUTER_BOUND('',#26877,.T.);
#22777=FACE_OUTER_BOUND('',#26878,.T.);
#22778=FACE_OUTER_BOUND('',#26879,.T.);
#22779=FACE_OUTER_BOUND('',#26880,.T.);
#22780=FACE_OUTER_BOUND('',#26881,.T.);
#22781=FACE_OUTER_BOUND('',#26882,.T.);
#22782=FACE_OUTER_BOUND('',#26883,.T.);
#22783=FACE_OUTER_BOUND('',#26884,.T.);
#22784=FACE_OUTER_BOUND('',#26885,.T.);
#22785=FACE_OUTER_BOUND('',#26886,.T.);
#22786=FACE_OUTER_BOUND('',#26887,.T.);
#22787=FACE_OUTER_BOUND('',#26888,.T.);
#22788=FACE_OUTER_BOUND('',#26889,.T.);
#22789=FACE_OUTER_BOUND('',#26890,.T.);
#22790=FACE_OUTER_BOUND('',#26891,.T.);
#22791=FACE_OUTER_BOUND('',#26892,.T.);
#22792=FACE_OUTER_BOUND('',#26893,.T.);
#22793=FACE_OUTER_BOUND('',#26894,.T.);
#22794=FACE_OUTER_BOUND('',#26895,.T.);
#22795=FACE_OUTER_BOUND('',#26896,.T.);
#22796=FACE_OUTER_BOUND('',#26897,.T.);
#22797=FACE_OUTER_BOUND('',#26898,.T.);
#22798=FACE_OUTER_BOUND('',#26899,.T.);
#22799=FACE_OUTER_BOUND('',#26900,.T.);
#22800=FACE_OUTER_BOUND('',#26901,.T.);
#22801=FACE_OUTER_BOUND('',#26902,.T.);
#22802=FACE_OUTER_BOUND('',#26903,.T.);
#22803=FACE_OUTER_BOUND('',#26904,.T.);
#22804=FACE_OUTER_BOUND('',#26905,.T.);
#22805=FACE_OUTER_BOUND('',#26906,.T.);
#22806=FACE_OUTER_BOUND('',#26907,.T.);
#22807=FACE_OUTER_BOUND('',#26908,.T.);
#22808=FACE_OUTER_BOUND('',#26909,.T.);
#22809=FACE_OUTER_BOUND('',#26910,.T.);
#22810=FACE_OUTER_BOUND('',#26911,.T.);
#22811=FACE_OUTER_BOUND('',#26912,.T.);
#22812=FACE_OUTER_BOUND('',#26913,.T.);
#22813=FACE_OUTER_BOUND('',#26914,.T.);
#22814=FACE_OUTER_BOUND('',#26915,.T.);
#22815=FACE_OUTER_BOUND('',#26916,.T.);
#22816=FACE_OUTER_BOUND('',#26917,.T.);
#22817=FACE_OUTER_BOUND('',#26918,.T.);
#22818=FACE_OUTER_BOUND('',#26919,.T.);
#22819=FACE_OUTER_BOUND('',#26920,.T.);
#22820=FACE_OUTER_BOUND('',#26921,.T.);
#22821=FACE_OUTER_BOUND('',#26922,.T.);
#22822=FACE_OUTER_BOUND('',#26923,.T.);
#22823=FACE_OUTER_BOUND('',#26924,.T.);
#22824=FACE_OUTER_BOUND('',#26925,.T.);
#22825=FACE_OUTER_BOUND('',#26926,.T.);
#22826=FACE_OUTER_BOUND('',#26927,.T.);
#22827=FACE_OUTER_BOUND('',#26928,.T.);
#22828=FACE_OUTER_BOUND('',#26929,.T.);
#22829=FACE_OUTER_BOUND('',#26930,.T.);
#22830=FACE_OUTER_BOUND('',#26931,.T.);
#22831=FACE_OUTER_BOUND('',#26932,.T.);
#22832=FACE_OUTER_BOUND('',#26933,.T.);
#22833=FACE_OUTER_BOUND('',#26934,.T.);
#22834=FACE_OUTER_BOUND('',#26935,.T.);
#22835=FACE_OUTER_BOUND('',#26936,.T.);
#22836=FACE_OUTER_BOUND('',#26937,.T.);
#22837=FACE_OUTER_BOUND('',#26938,.T.);
#22838=FACE_OUTER_BOUND('',#26939,.T.);
#22839=FACE_OUTER_BOUND('',#26940,.T.);
#22840=FACE_OUTER_BOUND('',#26941,.T.);
#22841=FACE_OUTER_BOUND('',#26942,.T.);
#22842=FACE_OUTER_BOUND('',#26943,.T.);
#22843=FACE_OUTER_BOUND('',#26944,.T.);
#22844=FACE_OUTER_BOUND('',#26945,.T.);
#22845=FACE_OUTER_BOUND('',#26946,.T.);
#22846=FACE_OUTER_BOUND('',#26947,.T.);
#22847=FACE_OUTER_BOUND('',#26948,.T.);
#22848=FACE_OUTER_BOUND('',#26949,.T.);
#22849=FACE_OUTER_BOUND('',#26950,.T.);
#22850=FACE_OUTER_BOUND('',#26951,.T.);
#22851=FACE_OUTER_BOUND('',#26952,.T.);
#22852=FACE_OUTER_BOUND('',#26953,.T.);
#22853=FACE_OUTER_BOUND('',#26954,.T.);
#22854=FACE_OUTER_BOUND('',#26955,.T.);
#22855=FACE_OUTER_BOUND('',#26956,.T.);
#22856=FACE_OUTER_BOUND('',#26957,.T.);
#22857=FACE_OUTER_BOUND('',#26958,.T.);
#22858=FACE_OUTER_BOUND('',#26959,.T.);
#22859=FACE_OUTER_BOUND('',#26960,.T.);
#22860=FACE_OUTER_BOUND('',#26961,.T.);
#22861=FACE_OUTER_BOUND('',#26962,.T.);
#22862=FACE_OUTER_BOUND('',#26963,.T.);
#22863=FACE_OUTER_BOUND('',#26964,.T.);
#22864=FACE_OUTER_BOUND('',#26965,.T.);
#22865=FACE_OUTER_BOUND('',#26966,.T.);
#22866=FACE_OUTER_BOUND('',#26967,.T.);
#22867=FACE_OUTER_BOUND('',#26968,.T.);
#22868=FACE_OUTER_BOUND('',#26969,.T.);
#22869=FACE_OUTER_BOUND('',#26970,.T.);
#22870=FACE_OUTER_BOUND('',#26971,.T.);
#22871=FACE_OUTER_BOUND('',#26972,.T.);
#22872=FACE_OUTER_BOUND('',#26973,.T.);
#22873=FACE_OUTER_BOUND('',#26974,.T.);
#22874=FACE_OUTER_BOUND('',#26975,.T.);
#22875=FACE_OUTER_BOUND('',#26976,.T.);
#22876=FACE_OUTER_BOUND('',#26977,.T.);
#22877=FACE_OUTER_BOUND('',#26978,.T.);
#22878=FACE_OUTER_BOUND('',#26979,.T.);
#22879=FACE_OUTER_BOUND('',#26980,.T.);
#22880=FACE_OUTER_BOUND('',#26981,.T.);
#22881=FACE_OUTER_BOUND('',#26982,.T.);
#22882=FACE_OUTER_BOUND('',#26983,.T.);
#22883=FACE_OUTER_BOUND('',#26984,.T.);
#22884=FACE_OUTER_BOUND('',#26985,.T.);
#22885=FACE_OUTER_BOUND('',#26986,.T.);
#22886=FACE_OUTER_BOUND('',#26987,.T.);
#22887=FACE_OUTER_BOUND('',#26988,.T.);
#22888=FACE_OUTER_BOUND('',#26989,.T.);
#22889=FACE_OUTER_BOUND('',#26990,.T.);
#22890=FACE_OUTER_BOUND('',#26991,.T.);
#22891=FACE_OUTER_BOUND('',#26992,.T.);
#22892=FACE_OUTER_BOUND('',#26993,.T.);
#22893=FACE_OUTER_BOUND('',#26994,.T.);
#22894=FACE_OUTER_BOUND('',#26995,.T.);
#22895=FACE_OUTER_BOUND('',#26996,.T.);
#22896=FACE_OUTER_BOUND('',#26997,.T.);
#22897=FACE_OUTER_BOUND('',#26998,.T.);
#22898=FACE_OUTER_BOUND('',#26999,.T.);
#22899=FACE_OUTER_BOUND('',#27000,.T.);
#22900=FACE_OUTER_BOUND('',#27001,.T.);
#22901=FACE_OUTER_BOUND('',#27002,.T.);
#22902=FACE_OUTER_BOUND('',#27003,.T.);
#22903=FACE_OUTER_BOUND('',#27004,.T.);
#22904=FACE_OUTER_BOUND('',#27005,.T.);
#22905=FACE_OUTER_BOUND('',#27006,.T.);
#22906=FACE_OUTER_BOUND('',#27007,.T.);
#22907=FACE_OUTER_BOUND('',#27008,.T.);
#22908=FACE_OUTER_BOUND('',#27009,.T.);
#22909=FACE_OUTER_BOUND('',#27010,.T.);
#22910=FACE_OUTER_BOUND('',#27011,.T.);
#22911=FACE_OUTER_BOUND('',#27012,.T.);
#22912=FACE_OUTER_BOUND('',#27013,.T.);
#22913=FACE_OUTER_BOUND('',#27014,.T.);
#22914=FACE_OUTER_BOUND('',#27015,.T.);
#22915=FACE_OUTER_BOUND('',#27016,.T.);
#22916=FACE_OUTER_BOUND('',#27017,.T.);
#22917=FACE_OUTER_BOUND('',#27018,.T.);
#22918=FACE_OUTER_BOUND('',#27019,.T.);
#22919=FACE_OUTER_BOUND('',#27020,.T.);
#22920=FACE_OUTER_BOUND('',#27021,.T.);
#22921=FACE_OUTER_BOUND('',#27022,.T.);
#22922=FACE_OUTER_BOUND('',#27023,.T.);
#22923=FACE_OUTER_BOUND('',#27024,.T.);
#22924=FACE_OUTER_BOUND('',#27025,.T.);
#22925=FACE_OUTER_BOUND('',#27026,.T.);
#22926=FACE_OUTER_BOUND('',#27027,.T.);
#22927=FACE_OUTER_BOUND('',#27028,.T.);
#22928=FACE_OUTER_BOUND('',#27029,.T.);
#22929=FACE_OUTER_BOUND('',#27030,.T.);
#22930=FACE_OUTER_BOUND('',#27031,.T.);
#22931=FACE_OUTER_BOUND('',#27032,.T.);
#22932=FACE_OUTER_BOUND('',#27033,.T.);
#22933=FACE_OUTER_BOUND('',#27034,.T.);
#22934=FACE_OUTER_BOUND('',#27035,.T.);
#22935=FACE_OUTER_BOUND('',#27036,.T.);
#22936=FACE_OUTER_BOUND('',#27037,.T.);
#22937=FACE_OUTER_BOUND('',#27038,.T.);
#22938=FACE_OUTER_BOUND('',#27039,.T.);
#22939=FACE_OUTER_BOUND('',#27040,.T.);
#22940=FACE_OUTER_BOUND('',#27041,.T.);
#22941=FACE_OUTER_BOUND('',#27042,.T.);
#22942=FACE_OUTER_BOUND('',#27043,.T.);
#22943=FACE_OUTER_BOUND('',#27044,.T.);
#22944=FACE_OUTER_BOUND('',#27045,.T.);
#22945=FACE_OUTER_BOUND('',#27046,.T.);
#22946=FACE_OUTER_BOUND('',#27047,.T.);
#22947=FACE_OUTER_BOUND('',#27048,.T.);
#22948=FACE_OUTER_BOUND('',#27049,.T.);
#22949=FACE_OUTER_BOUND('',#27050,.T.);
#22950=FACE_OUTER_BOUND('',#27051,.T.);
#22951=FACE_OUTER_BOUND('',#27052,.T.);
#22952=FACE_OUTER_BOUND('',#27053,.T.);
#22953=FACE_OUTER_BOUND('',#27054,.T.);
#22954=FACE_OUTER_BOUND('',#27055,.T.);
#22955=FACE_OUTER_BOUND('',#27056,.T.);
#22956=FACE_OUTER_BOUND('',#27057,.T.);
#22957=FACE_OUTER_BOUND('',#27058,.T.);
#22958=FACE_OUTER_BOUND('',#27059,.T.);
#22959=FACE_OUTER_BOUND('',#27060,.T.);
#22960=FACE_OUTER_BOUND('',#27061,.T.);
#22961=FACE_OUTER_BOUND('',#27062,.T.);
#22962=FACE_OUTER_BOUND('',#27063,.T.);
#22963=FACE_OUTER_BOUND('',#27064,.T.);
#22964=FACE_OUTER_BOUND('',#27065,.T.);
#22965=FACE_OUTER_BOUND('',#27066,.T.);
#22966=FACE_OUTER_BOUND('',#27067,.T.);
#22967=FACE_OUTER_BOUND('',#27068,.T.);
#22968=FACE_OUTER_BOUND('',#27069,.T.);
#22969=FACE_OUTER_BOUND('',#27070,.T.);
#22970=FACE_OUTER_BOUND('',#27071,.T.);
#22971=FACE_OUTER_BOUND('',#27072,.T.);
#22972=FACE_OUTER_BOUND('',#27073,.T.);
#22973=FACE_OUTER_BOUND('',#27074,.T.);
#22974=FACE_OUTER_BOUND('',#27075,.T.);
#22975=FACE_OUTER_BOUND('',#27076,.T.);
#22976=FACE_OUTER_BOUND('',#27077,.T.);
#22977=FACE_OUTER_BOUND('',#27078,.T.);
#22978=FACE_OUTER_BOUND('',#27079,.T.);
#22979=FACE_OUTER_BOUND('',#27080,.T.);
#22980=FACE_OUTER_BOUND('',#27081,.T.);
#22981=FACE_OUTER_BOUND('',#27082,.T.);
#22982=FACE_OUTER_BOUND('',#27083,.T.);
#22983=FACE_OUTER_BOUND('',#27084,.T.);
#22984=FACE_OUTER_BOUND('',#27085,.T.);
#22985=FACE_OUTER_BOUND('',#27086,.T.);
#22986=FACE_OUTER_BOUND('',#27087,.T.);
#22987=FACE_OUTER_BOUND('',#27088,.T.);
#22988=FACE_OUTER_BOUND('',#27089,.T.);
#22989=FACE_OUTER_BOUND('',#27090,.T.);
#22990=FACE_OUTER_BOUND('',#27091,.T.);
#22991=FACE_OUTER_BOUND('',#27092,.T.);
#22992=FACE_OUTER_BOUND('',#27093,.T.);
#22993=FACE_OUTER_BOUND('',#27094,.T.);
#22994=FACE_OUTER_BOUND('',#27095,.T.);
#22995=FACE_OUTER_BOUND('',#27096,.T.);
#22996=FACE_OUTER_BOUND('',#27097,.T.);
#22997=FACE_OUTER_BOUND('',#27098,.T.);
#22998=FACE_OUTER_BOUND('',#27099,.T.);
#22999=FACE_OUTER_BOUND('',#27100,.T.);
#23000=FACE_OUTER_BOUND('',#27101,.T.);
#23001=FACE_OUTER_BOUND('',#27102,.T.);
#23002=FACE_OUTER_BOUND('',#27103,.T.);
#23003=FACE_OUTER_BOUND('',#27104,.T.);
#23004=FACE_OUTER_BOUND('',#27105,.T.);
#23005=FACE_OUTER_BOUND('',#27106,.T.);
#23006=FACE_OUTER_BOUND('',#27107,.T.);
#23007=FACE_OUTER_BOUND('',#27108,.T.);
#23008=FACE_OUTER_BOUND('',#27109,.T.);
#23009=FACE_OUTER_BOUND('',#27110,.T.);
#23010=FACE_OUTER_BOUND('',#27111,.T.);
#23011=FACE_OUTER_BOUND('',#27112,.T.);
#23012=FACE_OUTER_BOUND('',#27113,.T.);
#23013=FACE_OUTER_BOUND('',#27114,.T.);
#23014=FACE_OUTER_BOUND('',#27115,.T.);
#23015=FACE_OUTER_BOUND('',#27116,.T.);
#23016=FACE_OUTER_BOUND('',#27117,.T.);
#23017=FACE_OUTER_BOUND('',#27118,.T.);
#23018=FACE_OUTER_BOUND('',#27119,.T.);
#23019=FACE_OUTER_BOUND('',#27120,.T.);
#23020=FACE_OUTER_BOUND('',#27121,.T.);
#23021=FACE_OUTER_BOUND('',#27122,.T.);
#23022=FACE_OUTER_BOUND('',#27123,.T.);
#23023=FACE_OUTER_BOUND('',#27124,.T.);
#23024=FACE_OUTER_BOUND('',#27125,.T.);
#23025=FACE_OUTER_BOUND('',#27126,.T.);
#23026=FACE_OUTER_BOUND('',#27127,.T.);
#23027=FACE_OUTER_BOUND('',#27128,.T.);
#23028=FACE_OUTER_BOUND('',#27129,.T.);
#23029=FACE_OUTER_BOUND('',#27130,.T.);
#23030=FACE_OUTER_BOUND('',#27131,.T.);
#23031=FACE_OUTER_BOUND('',#27132,.T.);
#23032=FACE_OUTER_BOUND('',#27133,.T.);
#23033=FACE_OUTER_BOUND('',#27134,.T.);
#23034=FACE_OUTER_BOUND('',#27135,.T.);
#23035=FACE_OUTER_BOUND('',#27136,.T.);
#23036=FACE_OUTER_BOUND('',#27137,.T.);
#23037=FACE_OUTER_BOUND('',#27138,.T.);
#23038=FACE_OUTER_BOUND('',#27139,.T.);
#23039=FACE_OUTER_BOUND('',#27140,.T.);
#23040=FACE_OUTER_BOUND('',#27141,.T.);
#23041=FACE_OUTER_BOUND('',#27142,.T.);
#23042=FACE_OUTER_BOUND('',#27143,.T.);
#23043=FACE_OUTER_BOUND('',#27144,.T.);
#23044=FACE_OUTER_BOUND('',#27145,.T.);
#23045=FACE_OUTER_BOUND('',#27146,.T.);
#23046=FACE_OUTER_BOUND('',#27147,.T.);
#23047=FACE_OUTER_BOUND('',#27148,.T.);
#23048=FACE_OUTER_BOUND('',#27149,.T.);
#23049=FACE_OUTER_BOUND('',#27150,.T.);
#23050=FACE_OUTER_BOUND('',#27151,.T.);
#23051=FACE_OUTER_BOUND('',#27152,.T.);
#23052=FACE_OUTER_BOUND('',#27153,.T.);
#23053=FACE_OUTER_BOUND('',#27154,.T.);
#23054=FACE_OUTER_BOUND('',#27155,.T.);
#23055=FACE_OUTER_BOUND('',#27156,.T.);
#23056=FACE_OUTER_BOUND('',#27157,.T.);
#23057=FACE_OUTER_BOUND('',#27158,.T.);
#23058=FACE_OUTER_BOUND('',#27159,.T.);
#23059=FACE_OUTER_BOUND('',#27160,.T.);
#23060=FACE_OUTER_BOUND('',#27161,.T.);
#23061=FACE_OUTER_BOUND('',#27162,.T.);
#23062=FACE_OUTER_BOUND('',#27163,.T.);
#23063=FACE_OUTER_BOUND('',#27164,.T.);
#23064=FACE_OUTER_BOUND('',#27165,.T.);
#23065=FACE_OUTER_BOUND('',#27166,.T.);
#23066=FACE_OUTER_BOUND('',#27167,.T.);
#23067=FACE_OUTER_BOUND('',#27168,.T.);
#23068=FACE_OUTER_BOUND('',#27169,.T.);
#23069=FACE_OUTER_BOUND('',#27170,.T.);
#23070=FACE_OUTER_BOUND('',#27171,.T.);
#23071=FACE_OUTER_BOUND('',#27172,.T.);
#23072=FACE_OUTER_BOUND('',#27173,.T.);
#23073=FACE_OUTER_BOUND('',#27174,.T.);
#23074=FACE_OUTER_BOUND('',#27175,.T.);
#23075=FACE_OUTER_BOUND('',#27176,.T.);
#23076=FACE_OUTER_BOUND('',#27177,.T.);
#23077=FACE_OUTER_BOUND('',#27178,.T.);
#23078=FACE_OUTER_BOUND('',#27179,.T.);
#23079=FACE_OUTER_BOUND('',#27180,.T.);
#23080=FACE_OUTER_BOUND('',#27181,.T.);
#23081=FACE_OUTER_BOUND('',#27182,.T.);
#23082=FACE_OUTER_BOUND('',#27183,.T.);
#23083=FACE_OUTER_BOUND('',#27184,.T.);
#23084=FACE_OUTER_BOUND('',#27185,.T.);
#23085=FACE_OUTER_BOUND('',#27186,.T.);
#23086=FACE_OUTER_BOUND('',#27187,.T.);
#23087=FACE_OUTER_BOUND('',#27188,.T.);
#23088=FACE_OUTER_BOUND('',#27189,.T.);
#23089=FACE_OUTER_BOUND('',#27190,.T.);
#23090=FACE_OUTER_BOUND('',#27191,.T.);
#23091=FACE_OUTER_BOUND('',#27192,.T.);
#23092=FACE_OUTER_BOUND('',#27193,.T.);
#23093=FACE_OUTER_BOUND('',#27194,.T.);
#23094=FACE_OUTER_BOUND('',#27195,.T.);
#23095=FACE_OUTER_BOUND('',#27196,.T.);
#23096=FACE_OUTER_BOUND('',#27197,.T.);
#23097=FACE_OUTER_BOUND('',#27198,.T.);
#23098=FACE_OUTER_BOUND('',#27199,.T.);
#23099=FACE_OUTER_BOUND('',#27200,.T.);
#23100=FACE_OUTER_BOUND('',#27201,.T.);
#23101=FACE_OUTER_BOUND('',#27202,.T.);
#23102=FACE_OUTER_BOUND('',#27203,.T.);
#23103=FACE_OUTER_BOUND('',#27204,.T.);
#23104=FACE_OUTER_BOUND('',#27205,.T.);
#23105=FACE_OUTER_BOUND('',#27206,.T.);
#23106=FACE_OUTER_BOUND('',#27207,.T.);
#23107=FACE_OUTER_BOUND('',#27208,.T.);
#23108=FACE_OUTER_BOUND('',#27209,.T.);
#23109=FACE_OUTER_BOUND('',#27210,.T.);
#23110=FACE_OUTER_BOUND('',#27211,.T.);
#23111=FACE_OUTER_BOUND('',#27212,.T.);
#23112=FACE_OUTER_BOUND('',#27213,.T.);
#23113=FACE_OUTER_BOUND('',#27214,.T.);
#23114=FACE_OUTER_BOUND('',#27215,.T.);
#23115=FACE_OUTER_BOUND('',#27216,.T.);
#23116=FACE_OUTER_BOUND('',#27217,.T.);
#23117=FACE_OUTER_BOUND('',#27218,.T.);
#23118=FACE_OUTER_BOUND('',#27219,.T.);
#23119=FACE_OUTER_BOUND('',#27220,.T.);
#23120=FACE_OUTER_BOUND('',#27221,.T.);
#23121=FACE_OUTER_BOUND('',#27222,.T.);
#23122=FACE_OUTER_BOUND('',#27223,.T.);
#23123=FACE_OUTER_BOUND('',#27224,.T.);
#23124=FACE_OUTER_BOUND('',#27225,.T.);
#23125=FACE_OUTER_BOUND('',#27226,.T.);
#23126=FACE_OUTER_BOUND('',#27227,.T.);
#23127=FACE_OUTER_BOUND('',#27228,.T.);
#23128=FACE_OUTER_BOUND('',#27229,.T.);
#23129=FACE_OUTER_BOUND('',#27230,.T.);
#23130=FACE_OUTER_BOUND('',#27231,.T.);
#23131=FACE_OUTER_BOUND('',#27232,.T.);
#23132=FACE_OUTER_BOUND('',#27233,.T.);
#23133=FACE_OUTER_BOUND('',#27234,.T.);
#23134=FACE_OUTER_BOUND('',#27235,.T.);
#23135=FACE_OUTER_BOUND('',#27236,.T.);
#23136=FACE_OUTER_BOUND('',#27237,.T.);
#23137=FACE_OUTER_BOUND('',#27238,.T.);
#23138=FACE_OUTER_BOUND('',#27239,.T.);
#23139=FACE_OUTER_BOUND('',#27240,.T.);
#23140=FACE_OUTER_BOUND('',#27241,.T.);
#23141=FACE_OUTER_BOUND('',#27242,.T.);
#23142=FACE_OUTER_BOUND('',#27243,.T.);
#23143=FACE_OUTER_BOUND('',#27244,.T.);
#23144=FACE_OUTER_BOUND('',#27245,.T.);
#23145=FACE_OUTER_BOUND('',#27246,.T.);
#23146=FACE_OUTER_BOUND('',#27247,.T.);
#23147=FACE_OUTER_BOUND('',#27248,.T.);
#23148=FACE_OUTER_BOUND('',#27249,.T.);
#23149=FACE_OUTER_BOUND('',#27250,.T.);
#23150=FACE_OUTER_BOUND('',#27251,.T.);
#23151=FACE_OUTER_BOUND('',#27252,.T.);
#23152=FACE_OUTER_BOUND('',#27253,.T.);
#23153=FACE_OUTER_BOUND('',#27254,.T.);
#23154=FACE_OUTER_BOUND('',#27255,.T.);
#23155=FACE_OUTER_BOUND('',#27256,.T.);
#23156=FACE_OUTER_BOUND('',#27257,.T.);
#23157=FACE_OUTER_BOUND('',#27258,.T.);
#23158=FACE_OUTER_BOUND('',#27259,.T.);
#23159=FACE_OUTER_BOUND('',#27260,.T.);
#23160=FACE_OUTER_BOUND('',#27261,.T.);
#23161=FACE_OUTER_BOUND('',#27262,.T.);
#23162=FACE_OUTER_BOUND('',#27263,.T.);
#23163=FACE_OUTER_BOUND('',#27264,.T.);
#23164=FACE_OUTER_BOUND('',#27265,.T.);
#23165=FACE_OUTER_BOUND('',#27266,.T.);
#23166=FACE_OUTER_BOUND('',#27267,.T.);
#23167=FACE_OUTER_BOUND('',#27268,.T.);
#23168=FACE_OUTER_BOUND('',#27269,.T.);
#23169=FACE_OUTER_BOUND('',#27270,.T.);
#23170=FACE_OUTER_BOUND('',#27271,.T.);
#23171=FACE_OUTER_BOUND('',#27272,.T.);
#23172=FACE_OUTER_BOUND('',#27273,.T.);
#23173=FACE_OUTER_BOUND('',#27274,.T.);
#23174=FACE_OUTER_BOUND('',#27275,.T.);
#23175=FACE_OUTER_BOUND('',#27276,.T.);
#23176=FACE_OUTER_BOUND('',#27277,.T.);
#23177=FACE_OUTER_BOUND('',#27278,.T.);
#23178=FACE_OUTER_BOUND('',#27279,.T.);
#23179=FACE_OUTER_BOUND('',#27280,.T.);
#23180=FACE_OUTER_BOUND('',#27281,.T.);
#23181=FACE_OUTER_BOUND('',#27282,.T.);
#23182=FACE_OUTER_BOUND('',#27283,.T.);
#23183=FACE_OUTER_BOUND('',#27284,.T.);
#23184=FACE_OUTER_BOUND('',#27285,.T.);
#23185=FACE_OUTER_BOUND('',#27286,.T.);
#23186=FACE_OUTER_BOUND('',#27287,.T.);
#23187=FACE_OUTER_BOUND('',#27288,.T.);
#23188=FACE_OUTER_BOUND('',#27289,.T.);
#23189=FACE_OUTER_BOUND('',#27290,.T.);
#23190=FACE_OUTER_BOUND('',#27291,.T.);
#23191=FACE_OUTER_BOUND('',#27292,.T.);
#23192=FACE_OUTER_BOUND('',#27293,.T.);
#23193=FACE_OUTER_BOUND('',#27294,.T.);
#23194=FACE_OUTER_BOUND('',#27295,.T.);
#23195=FACE_OUTER_BOUND('',#27296,.T.);
#23196=FACE_OUTER_BOUND('',#27297,.T.);
#23197=FACE_OUTER_BOUND('',#27298,.T.);
#23198=FACE_OUTER_BOUND('',#27299,.T.);
#23199=FACE_OUTER_BOUND('',#27300,.T.);
#23200=FACE_OUTER_BOUND('',#27301,.T.);
#23201=FACE_OUTER_BOUND('',#27302,.T.);
#23202=FACE_OUTER_BOUND('',#27303,.T.);
#23203=FACE_OUTER_BOUND('',#27304,.T.);
#23204=FACE_OUTER_BOUND('',#27305,.T.);
#23205=FACE_OUTER_BOUND('',#27306,.T.);
#23206=FACE_OUTER_BOUND('',#27307,.T.);
#23207=FACE_OUTER_BOUND('',#27308,.T.);
#23208=FACE_OUTER_BOUND('',#27309,.T.);
#23209=FACE_OUTER_BOUND('',#27310,.T.);
#23210=FACE_OUTER_BOUND('',#27311,.T.);
#23211=FACE_OUTER_BOUND('',#27312,.T.);
#23212=FACE_OUTER_BOUND('',#27313,.T.);
#23213=FACE_OUTER_BOUND('',#27314,.T.);
#23214=FACE_OUTER_BOUND('',#27315,.T.);
#23215=FACE_OUTER_BOUND('',#27316,.T.);
#23216=FACE_OUTER_BOUND('',#27317,.T.);
#23217=FACE_OUTER_BOUND('',#27318,.T.);
#23218=FACE_OUTER_BOUND('',#27319,.T.);
#23219=FACE_OUTER_BOUND('',#27320,.T.);
#23220=FACE_OUTER_BOUND('',#27321,.T.);
#23221=FACE_OUTER_BOUND('',#27322,.T.);
#23222=FACE_OUTER_BOUND('',#27323,.T.);
#23223=FACE_OUTER_BOUND('',#27324,.T.);
#23224=FACE_OUTER_BOUND('',#27325,.T.);
#23225=FACE_OUTER_BOUND('',#27326,.T.);
#23226=FACE_OUTER_BOUND('',#27327,.T.);
#23227=FACE_OUTER_BOUND('',#27328,.T.);
#23228=FACE_OUTER_BOUND('',#27329,.T.);
#23229=FACE_OUTER_BOUND('',#27330,.T.);
#23230=FACE_OUTER_BOUND('',#27331,.T.);
#23231=FACE_OUTER_BOUND('',#27332,.T.);
#23232=FACE_OUTER_BOUND('',#27333,.T.);
#23233=FACE_OUTER_BOUND('',#27334,.T.);
#23234=FACE_OUTER_BOUND('',#27335,.T.);
#23235=FACE_OUTER_BOUND('',#27336,.T.);
#23236=FACE_OUTER_BOUND('',#27337,.T.);
#23237=FACE_OUTER_BOUND('',#27338,.T.);
#23238=FACE_OUTER_BOUND('',#27339,.T.);
#23239=FACE_OUTER_BOUND('',#27340,.T.);
#23240=FACE_OUTER_BOUND('',#27341,.T.);
#23241=FACE_OUTER_BOUND('',#27342,.T.);
#23242=FACE_OUTER_BOUND('',#27343,.T.);
#23243=FACE_OUTER_BOUND('',#27344,.T.);
#23244=FACE_OUTER_BOUND('',#27345,.T.);
#23245=FACE_OUTER_BOUND('',#27346,.T.);
#23246=FACE_OUTER_BOUND('',#27347,.T.);
#23247=FACE_OUTER_BOUND('',#27348,.T.);
#23248=FACE_OUTER_BOUND('',#27349,.T.);
#23249=FACE_OUTER_BOUND('',#27350,.T.);
#23250=FACE_OUTER_BOUND('',#27351,.T.);
#23251=FACE_OUTER_BOUND('',#27352,.T.);
#23252=FACE_OUTER_BOUND('',#27353,.T.);
#23253=FACE_OUTER_BOUND('',#27354,.T.);
#23254=FACE_OUTER_BOUND('',#27355,.T.);
#23255=FACE_OUTER_BOUND('',#27356,.T.);
#23256=FACE_OUTER_BOUND('',#27357,.T.);
#23257=FACE_OUTER_BOUND('',#27358,.T.);
#23258=FACE_OUTER_BOUND('',#27359,.T.);
#23259=FACE_OUTER_BOUND('',#27360,.T.);
#23260=FACE_OUTER_BOUND('',#27361,.T.);
#23261=FACE_OUTER_BOUND('',#27362,.T.);
#23262=FACE_OUTER_BOUND('',#27363,.T.);
#23263=FACE_OUTER_BOUND('',#27364,.T.);
#23264=FACE_OUTER_BOUND('',#27365,.T.);
#23265=FACE_OUTER_BOUND('',#27366,.T.);
#23266=FACE_OUTER_BOUND('',#27367,.T.);
#23267=FACE_OUTER_BOUND('',#27368,.T.);
#23268=FACE_OUTER_BOUND('',#27369,.T.);
#23269=FACE_OUTER_BOUND('',#27370,.T.);
#23270=FACE_OUTER_BOUND('',#27371,.T.);
#23271=FACE_OUTER_BOUND('',#27372,.T.);
#23272=FACE_OUTER_BOUND('',#27373,.T.);
#23273=FACE_OUTER_BOUND('',#27374,.T.);
#23274=FACE_OUTER_BOUND('',#27375,.T.);
#23275=FACE_OUTER_BOUND('',#27376,.T.);
#23276=FACE_OUTER_BOUND('',#27377,.T.);
#23277=FACE_OUTER_BOUND('',#27378,.T.);
#23278=FACE_OUTER_BOUND('',#27379,.T.);
#23279=FACE_OUTER_BOUND('',#27380,.T.);
#23280=FACE_OUTER_BOUND('',#27381,.T.);
#23281=FACE_OUTER_BOUND('',#27382,.T.);
#23282=FACE_OUTER_BOUND('',#27383,.T.);
#23283=FACE_OUTER_BOUND('',#27384,.T.);
#23284=FACE_OUTER_BOUND('',#27385,.T.);
#23285=FACE_OUTER_BOUND('',#27386,.T.);
#23286=FACE_OUTER_BOUND('',#27387,.T.);
#23287=FACE_OUTER_BOUND('',#27388,.T.);
#23288=FACE_OUTER_BOUND('',#27389,.T.);
#23289=FACE_OUTER_BOUND('',#27390,.T.);
#23290=FACE_OUTER_BOUND('',#27391,.T.);
#23291=FACE_OUTER_BOUND('',#27392,.T.);
#23292=FACE_OUTER_BOUND('',#27393,.T.);
#23293=FACE_OUTER_BOUND('',#27394,.T.);
#23294=FACE_OUTER_BOUND('',#27395,.T.);
#23295=FACE_OUTER_BOUND('',#27396,.T.);
#23296=FACE_OUTER_BOUND('',#27397,.T.);
#23297=FACE_OUTER_BOUND('',#27398,.T.);
#23298=FACE_OUTER_BOUND('',#27399,.T.);
#23299=FACE_OUTER_BOUND('',#27400,.T.);
#23300=FACE_OUTER_BOUND('',#27401,.T.);
#23301=FACE_OUTER_BOUND('',#27402,.T.);
#23302=FACE_OUTER_BOUND('',#27403,.T.);
#23303=FACE_OUTER_BOUND('',#27404,.T.);
#23304=FACE_OUTER_BOUND('',#27405,.T.);
#23305=FACE_OUTER_BOUND('',#27406,.T.);
#23306=FACE_OUTER_BOUND('',#27407,.T.);
#23307=FACE_OUTER_BOUND('',#27408,.T.);
#23308=FACE_OUTER_BOUND('',#27409,.T.);
#23309=FACE_OUTER_BOUND('',#27410,.T.);
#23310=FACE_OUTER_BOUND('',#27411,.T.);
#23311=FACE_OUTER_BOUND('',#27412,.T.);
#23312=FACE_OUTER_BOUND('',#27413,.T.);
#23313=FACE_OUTER_BOUND('',#27414,.T.);
#23314=FACE_OUTER_BOUND('',#27415,.T.);
#23315=FACE_OUTER_BOUND('',#27416,.T.);
#23316=FACE_OUTER_BOUND('',#27417,.T.);
#23317=FACE_OUTER_BOUND('',#27418,.T.);
#23318=FACE_OUTER_BOUND('',#27419,.T.);
#23319=FACE_OUTER_BOUND('',#27420,.T.);
#23320=FACE_OUTER_BOUND('',#27421,.T.);
#23321=FACE_OUTER_BOUND('',#27422,.T.);
#23322=FACE_OUTER_BOUND('',#27423,.T.);
#23323=FACE_OUTER_BOUND('',#27424,.T.);
#23324=FACE_OUTER_BOUND('',#27425,.T.);
#23325=FACE_OUTER_BOUND('',#27426,.T.);
#23326=FACE_OUTER_BOUND('',#27427,.T.);
#23327=FACE_OUTER_BOUND('',#27428,.T.);
#23328=FACE_OUTER_BOUND('',#27429,.T.);
#23329=FACE_OUTER_BOUND('',#27430,.T.);
#23330=FACE_OUTER_BOUND('',#27431,.T.);
#23331=FACE_OUTER_BOUND('',#27432,.T.);
#23332=FACE_OUTER_BOUND('',#27433,.T.);
#23333=FACE_OUTER_BOUND('',#27434,.T.);
#23334=FACE_OUTER_BOUND('',#27435,.T.);
#23335=FACE_OUTER_BOUND('',#27436,.T.);
#23336=FACE_OUTER_BOUND('',#27437,.T.);
#23337=FACE_OUTER_BOUND('',#27438,.T.);
#23338=FACE_OUTER_BOUND('',#27439,.T.);
#23339=FACE_OUTER_BOUND('',#27440,.T.);
#23340=FACE_OUTER_BOUND('',#27441,.T.);
#23341=FACE_OUTER_BOUND('',#27442,.T.);
#23342=FACE_OUTER_BOUND('',#27443,.T.);
#23343=FACE_OUTER_BOUND('',#27444,.T.);
#23344=FACE_OUTER_BOUND('',#27445,.T.);
#23345=FACE_OUTER_BOUND('',#27446,.T.);
#23346=FACE_OUTER_BOUND('',#27447,.T.);
#23347=FACE_OUTER_BOUND('',#27448,.T.);
#23348=FACE_OUTER_BOUND('',#27449,.T.);
#23349=FACE_OUTER_BOUND('',#27450,.T.);
#23350=FACE_OUTER_BOUND('',#27451,.T.);
#23351=FACE_OUTER_BOUND('',#27452,.T.);
#23352=FACE_OUTER_BOUND('',#27453,.T.);
#23353=FACE_OUTER_BOUND('',#27454,.T.);
#23354=FACE_OUTER_BOUND('',#27455,.T.);
#23355=FACE_OUTER_BOUND('',#27456,.T.);
#23356=FACE_OUTER_BOUND('',#27457,.T.);
#23357=FACE_OUTER_BOUND('',#27458,.T.);
#23358=FACE_OUTER_BOUND('',#27459,.T.);
#23359=FACE_OUTER_BOUND('',#27460,.T.);
#23360=FACE_OUTER_BOUND('',#27461,.T.);
#23361=FACE_OUTER_BOUND('',#27462,.T.);
#23362=FACE_OUTER_BOUND('',#27463,.T.);
#23363=FACE_OUTER_BOUND('',#27464,.T.);
#23364=FACE_OUTER_BOUND('',#27465,.T.);
#23365=FACE_OUTER_BOUND('',#27466,.T.);
#23366=FACE_OUTER_BOUND('',#27467,.T.);
#23367=FACE_OUTER_BOUND('',#27468,.T.);
#23368=FACE_OUTER_BOUND('',#27469,.T.);
#23369=FACE_OUTER_BOUND('',#27470,.T.);
#23370=FACE_OUTER_BOUND('',#27471,.T.);
#23371=FACE_OUTER_BOUND('',#27472,.T.);
#23372=FACE_OUTER_BOUND('',#27473,.T.);
#23373=FACE_OUTER_BOUND('',#27474,.T.);
#23374=FACE_OUTER_BOUND('',#27475,.T.);
#23375=FACE_OUTER_BOUND('',#27476,.T.);
#23376=FACE_OUTER_BOUND('',#27477,.T.);
#23377=FACE_OUTER_BOUND('',#27478,.T.);
#23378=FACE_OUTER_BOUND('',#27479,.T.);
#23379=FACE_OUTER_BOUND('',#27480,.T.);
#23380=FACE_OUTER_BOUND('',#27481,.T.);
#23381=FACE_OUTER_BOUND('',#27482,.T.);
#23382=FACE_OUTER_BOUND('',#27483,.T.);
#23383=FACE_OUTER_BOUND('',#27484,.T.);
#23384=FACE_OUTER_BOUND('',#27485,.T.);
#23385=FACE_OUTER_BOUND('',#27486,.T.);
#23386=FACE_OUTER_BOUND('',#27487,.T.);
#23387=FACE_OUTER_BOUND('',#27488,.T.);
#23388=FACE_OUTER_BOUND('',#27489,.T.);
#23389=FACE_OUTER_BOUND('',#27490,.T.);
#23390=FACE_OUTER_BOUND('',#27491,.T.);
#23391=FACE_OUTER_BOUND('',#27492,.T.);
#23392=FACE_OUTER_BOUND('',#27493,.T.);
#23393=FACE_OUTER_BOUND('',#27494,.T.);
#23394=FACE_OUTER_BOUND('',#27495,.T.);
#23395=FACE_OUTER_BOUND('',#27496,.T.);
#23396=FACE_OUTER_BOUND('',#27497,.T.);
#23397=FACE_OUTER_BOUND('',#27498,.T.);
#23398=FACE_OUTER_BOUND('',#27499,.T.);
#23399=FACE_OUTER_BOUND('',#27500,.T.);
#23400=FACE_OUTER_BOUND('',#27501,.T.);
#23401=FACE_OUTER_BOUND('',#27502,.T.);
#23402=FACE_OUTER_BOUND('',#27503,.T.);
#23403=FACE_OUTER_BOUND('',#27504,.T.);
#23404=FACE_OUTER_BOUND('',#27505,.T.);
#23405=FACE_OUTER_BOUND('',#27506,.T.);
#23406=FACE_OUTER_BOUND('',#27507,.T.);
#23407=FACE_OUTER_BOUND('',#27508,.T.);
#23408=FACE_OUTER_BOUND('',#27509,.T.);
#23409=FACE_OUTER_BOUND('',#27510,.T.);
#23410=FACE_OUTER_BOUND('',#27511,.T.);
#23411=FACE_OUTER_BOUND('',#27512,.T.);
#23412=FACE_OUTER_BOUND('',#27513,.T.);
#23413=FACE_OUTER_BOUND('',#27514,.T.);
#23414=FACE_OUTER_BOUND('',#27515,.T.);
#23415=FACE_OUTER_BOUND('',#27516,.T.);
#23416=FACE_OUTER_BOUND('',#27517,.T.);
#23417=FACE_OUTER_BOUND('',#27518,.T.);
#23418=FACE_OUTER_BOUND('',#27519,.T.);
#23419=FACE_OUTER_BOUND('',#27520,.T.);
#23420=FACE_OUTER_BOUND('',#27521,.T.);
#23421=FACE_OUTER_BOUND('',#27522,.T.);
#23422=FACE_OUTER_BOUND('',#27523,.T.);
#23423=FACE_OUTER_BOUND('',#27524,.T.);
#23424=FACE_OUTER_BOUND('',#27525,.T.);
#23425=FACE_OUTER_BOUND('',#27526,.T.);
#23426=FACE_OUTER_BOUND('',#27527,.T.);
#23427=FACE_OUTER_BOUND('',#27528,.T.);
#23428=FACE_OUTER_BOUND('',#27529,.T.);
#23429=FACE_OUTER_BOUND('',#27530,.T.);
#23430=FACE_OUTER_BOUND('',#27531,.T.);
#23431=FACE_OUTER_BOUND('',#27532,.T.);
#23432=FACE_OUTER_BOUND('',#27533,.T.);
#23433=FACE_OUTER_BOUND('',#27534,.T.);
#23434=FACE_OUTER_BOUND('',#27535,.T.);
#23435=FACE_OUTER_BOUND('',#27536,.T.);
#23436=FACE_OUTER_BOUND('',#27537,.T.);
#23437=FACE_OUTER_BOUND('',#27538,.T.);
#23438=FACE_OUTER_BOUND('',#27539,.T.);
#23439=FACE_OUTER_BOUND('',#27540,.T.);
#23440=FACE_OUTER_BOUND('',#27541,.T.);
#23441=FACE_OUTER_BOUND('',#27542,.T.);
#23442=FACE_OUTER_BOUND('',#27543,.T.);
#23443=FACE_OUTER_BOUND('',#27544,.T.);
#23444=FACE_OUTER_BOUND('',#27545,.T.);
#23445=FACE_OUTER_BOUND('',#27546,.T.);
#23446=FACE_OUTER_BOUND('',#27547,.T.);
#23447=FACE_OUTER_BOUND('',#27548,.T.);
#23448=FACE_OUTER_BOUND('',#27549,.T.);
#23449=FACE_OUTER_BOUND('',#27550,.T.);
#23450=FACE_OUTER_BOUND('',#27551,.T.);
#23451=FACE_OUTER_BOUND('',#27552,.T.);
#23452=FACE_OUTER_BOUND('',#27553,.T.);
#23453=FACE_OUTER_BOUND('',#27554,.T.);
#23454=FACE_OUTER_BOUND('',#27555,.T.);
#23455=FACE_OUTER_BOUND('',#27556,.T.);
#23456=FACE_OUTER_BOUND('',#27557,.T.);
#23457=FACE_OUTER_BOUND('',#27558,.T.);
#23458=FACE_OUTER_BOUND('',#27559,.T.);
#23459=FACE_OUTER_BOUND('',#27560,.T.);
#23460=FACE_OUTER_BOUND('',#27561,.T.);
#23461=FACE_OUTER_BOUND('',#27562,.T.);
#23462=FACE_OUTER_BOUND('',#27563,.T.);
#23463=FACE_OUTER_BOUND('',#27564,.T.);
#23464=FACE_OUTER_BOUND('',#27565,.T.);
#23465=FACE_OUTER_BOUND('',#27566,.T.);
#23466=FACE_OUTER_BOUND('',#27567,.T.);
#23467=FACE_OUTER_BOUND('',#27568,.T.);
#23468=FACE_OUTER_BOUND('',#27569,.T.);
#23469=FACE_OUTER_BOUND('',#27570,.T.);
#23470=FACE_OUTER_BOUND('',#27571,.T.);
#23471=FACE_OUTER_BOUND('',#27572,.T.);
#23472=FACE_OUTER_BOUND('',#27573,.T.);
#23473=FACE_OUTER_BOUND('',#27574,.T.);
#23474=FACE_OUTER_BOUND('',#27575,.T.);
#23475=FACE_OUTER_BOUND('',#27576,.T.);
#23476=FACE_OUTER_BOUND('',#27577,.T.);
#23477=FACE_OUTER_BOUND('',#27578,.T.);
#23478=FACE_OUTER_BOUND('',#27579,.T.);
#23479=FACE_OUTER_BOUND('',#27580,.T.);
#23480=FACE_OUTER_BOUND('',#27581,.T.);
#23481=FACE_OUTER_BOUND('',#27582,.T.);
#23482=FACE_OUTER_BOUND('',#27583,.T.);
#23483=FACE_OUTER_BOUND('',#27584,.T.);
#23484=FACE_OUTER_BOUND('',#27585,.T.);
#23485=FACE_OUTER_BOUND('',#27586,.T.);
#23486=FACE_OUTER_BOUND('',#27587,.T.);
#23487=FACE_OUTER_BOUND('',#27588,.T.);
#23488=FACE_OUTER_BOUND('',#27589,.T.);
#23489=FACE_OUTER_BOUND('',#27590,.T.);
#23490=FACE_OUTER_BOUND('',#27591,.T.);
#23491=FACE_OUTER_BOUND('',#27592,.T.);
#23492=FACE_OUTER_BOUND('',#27593,.T.);
#23493=FACE_OUTER_BOUND('',#27594,.T.);
#23494=FACE_OUTER_BOUND('',#27595,.T.);
#23495=FACE_OUTER_BOUND('',#27596,.T.);
#23496=FACE_OUTER_BOUND('',#27597,.T.);
#23497=FACE_OUTER_BOUND('',#27598,.T.);
#23498=FACE_OUTER_BOUND('',#27599,.T.);
#23499=FACE_OUTER_BOUND('',#27600,.T.);
#23500=FACE_OUTER_BOUND('',#27601,.T.);
#23501=FACE_OUTER_BOUND('',#27602,.T.);
#23502=FACE_OUTER_BOUND('',#27603,.T.);
#23503=FACE_OUTER_BOUND('',#27604,.T.);
#23504=FACE_OUTER_BOUND('',#27605,.T.);
#23505=FACE_OUTER_BOUND('',#27606,.T.);
#23506=FACE_OUTER_BOUND('',#27607,.T.);
#23507=FACE_OUTER_BOUND('',#27608,.T.);
#23508=FACE_OUTER_BOUND('',#27609,.T.);
#23509=FACE_OUTER_BOUND('',#27610,.T.);
#23510=FACE_OUTER_BOUND('',#27611,.T.);
#23511=FACE_OUTER_BOUND('',#27612,.T.);
#23512=FACE_OUTER_BOUND('',#27613,.T.);
#23513=FACE_OUTER_BOUND('',#27614,.T.);
#23514=FACE_OUTER_BOUND('',#27615,.T.);
#23515=FACE_OUTER_BOUND('',#27616,.T.);
#23516=FACE_OUTER_BOUND('',#27617,.T.);
#23517=FACE_OUTER_BOUND('',#27618,.T.);
#23518=FACE_OUTER_BOUND('',#27619,.T.);
#23519=FACE_OUTER_BOUND('',#27620,.T.);
#23520=FACE_OUTER_BOUND('',#27621,.T.);
#23521=FACE_OUTER_BOUND('',#27622,.T.);
#23522=FACE_OUTER_BOUND('',#27623,.T.);
#23523=FACE_OUTER_BOUND('',#27624,.T.);
#23524=FACE_OUTER_BOUND('',#27625,.T.);
#23525=FACE_OUTER_BOUND('',#27626,.T.);
#23526=FACE_OUTER_BOUND('',#27627,.T.);
#23527=FACE_OUTER_BOUND('',#27628,.T.);
#23528=FACE_OUTER_BOUND('',#27629,.T.);
#23529=FACE_OUTER_BOUND('',#27630,.T.);
#23530=FACE_OUTER_BOUND('',#27631,.T.);
#23531=FACE_OUTER_BOUND('',#27632,.T.);
#23532=FACE_OUTER_BOUND('',#27633,.T.);
#23533=FACE_OUTER_BOUND('',#27634,.T.);
#23534=FACE_OUTER_BOUND('',#27635,.T.);
#23535=FACE_OUTER_BOUND('',#27636,.T.);
#23536=FACE_OUTER_BOUND('',#27637,.T.);
#23537=FACE_OUTER_BOUND('',#27638,.T.);
#23538=FACE_OUTER_BOUND('',#27639,.T.);
#23539=FACE_OUTER_BOUND('',#27640,.T.);
#23540=FACE_OUTER_BOUND('',#27641,.T.);
#23541=FACE_OUTER_BOUND('',#27642,.T.);
#23542=FACE_OUTER_BOUND('',#27643,.T.);
#23543=FACE_OUTER_BOUND('',#27644,.T.);
#23544=FACE_OUTER_BOUND('',#27645,.T.);
#23545=FACE_OUTER_BOUND('',#27646,.T.);
#23546=FACE_OUTER_BOUND('',#27647,.T.);
#23547=FACE_OUTER_BOUND('',#27648,.T.);
#23548=FACE_OUTER_BOUND('',#27649,.T.);
#23549=FACE_OUTER_BOUND('',#27650,.T.);
#23550=FACE_OUTER_BOUND('',#27651,.T.);
#23551=FACE_OUTER_BOUND('',#27652,.T.);
#23552=FACE_OUTER_BOUND('',#27653,.T.);
#23553=FACE_OUTER_BOUND('',#27654,.T.);
#23554=FACE_OUTER_BOUND('',#27655,.T.);
#23555=FACE_OUTER_BOUND('',#27656,.T.);
#23556=FACE_OUTER_BOUND('',#27657,.T.);
#23557=FACE_OUTER_BOUND('',#27658,.T.);
#23558=FACE_OUTER_BOUND('',#27659,.T.);
#23559=FACE_OUTER_BOUND('',#27660,.T.);
#23560=FACE_OUTER_BOUND('',#27661,.T.);
#23561=FACE_OUTER_BOUND('',#27662,.T.);
#23562=FACE_OUTER_BOUND('',#27663,.T.);
#23563=FACE_OUTER_BOUND('',#27664,.T.);
#23564=FACE_OUTER_BOUND('',#27665,.T.);
#23565=FACE_OUTER_BOUND('',#27666,.T.);
#23566=FACE_OUTER_BOUND('',#27667,.T.);
#23567=FACE_OUTER_BOUND('',#27668,.T.);
#23568=FACE_OUTER_BOUND('',#27669,.T.);
#23569=FACE_OUTER_BOUND('',#27670,.T.);
#23570=FACE_OUTER_BOUND('',#27671,.T.);
#23571=FACE_OUTER_BOUND('',#27672,.T.);
#23572=FACE_OUTER_BOUND('',#27673,.T.);
#23573=FACE_OUTER_BOUND('',#27674,.T.);
#23574=FACE_OUTER_BOUND('',#27675,.T.);
#23575=FACE_OUTER_BOUND('',#27676,.T.);
#23576=FACE_OUTER_BOUND('',#27677,.T.);
#23577=FACE_OUTER_BOUND('',#27678,.T.);
#23578=FACE_OUTER_BOUND('',#27679,.T.);
#23579=FACE_OUTER_BOUND('',#27680,.T.);
#23580=FACE_OUTER_BOUND('',#27681,.T.);
#23581=FACE_OUTER_BOUND('',#27682,.T.);
#23582=FACE_OUTER_BOUND('',#27683,.T.);
#23583=FACE_OUTER_BOUND('',#27684,.T.);
#23584=FACE_OUTER_BOUND('',#27685,.T.);
#23585=FACE_OUTER_BOUND('',#27686,.T.);
#23586=FACE_OUTER_BOUND('',#27687,.T.);
#23587=FACE_OUTER_BOUND('',#27688,.T.);
#23588=FACE_OUTER_BOUND('',#27689,.T.);
#23589=FACE_OUTER_BOUND('',#27690,.T.);
#23590=FACE_OUTER_BOUND('',#27691,.T.);
#23591=FACE_OUTER_BOUND('',#27692,.T.);
#23592=FACE_OUTER_BOUND('',#27693,.T.);
#23593=FACE_OUTER_BOUND('',#27694,.T.);
#23594=FACE_OUTER_BOUND('',#27695,.T.);
#23595=FACE_OUTER_BOUND('',#27696,.T.);
#23596=FACE_OUTER_BOUND('',#27697,.T.);
#23597=FACE_OUTER_BOUND('',#27698,.T.);
#23598=FACE_OUTER_BOUND('',#27699,.T.);
#23599=FACE_OUTER_BOUND('',#27700,.T.);
#23600=FACE_OUTER_BOUND('',#27701,.T.);
#23601=FACE_OUTER_BOUND('',#27702,.T.);
#23602=FACE_OUTER_BOUND('',#27703,.T.);
#23603=FACE_OUTER_BOUND('',#27704,.T.);
#23604=FACE_OUTER_BOUND('',#27705,.T.);
#23605=FACE_OUTER_BOUND('',#27706,.T.);
#23606=FACE_OUTER_BOUND('',#27707,.T.);
#23607=FACE_OUTER_BOUND('',#27708,.T.);
#23608=FACE_OUTER_BOUND('',#27709,.T.);
#23609=FACE_OUTER_BOUND('',#27710,.T.);
#23610=FACE_OUTER_BOUND('',#27711,.T.);
#23611=FACE_OUTER_BOUND('',#27712,.T.);
#23612=FACE_OUTER_BOUND('',#27713,.T.);
#23613=FACE_OUTER_BOUND('',#27714,.T.);
#23614=FACE_OUTER_BOUND('',#27715,.T.);
#23615=FACE_OUTER_BOUND('',#27716,.T.);
#23616=FACE_OUTER_BOUND('',#27717,.T.);
#23617=FACE_OUTER_BOUND('',#27718,.T.);
#23618=FACE_OUTER_BOUND('',#27719,.T.);
#23619=FACE_OUTER_BOUND('',#27720,.T.);
#23620=FACE_OUTER_BOUND('',#27721,.T.);
#23621=FACE_OUTER_BOUND('',#27722,.T.);
#23622=FACE_OUTER_BOUND('',#27723,.T.);
#23623=FACE_OUTER_BOUND('',#27724,.T.);
#23624=FACE_OUTER_BOUND('',#27725,.T.);
#23625=FACE_OUTER_BOUND('',#27726,.T.);
#23626=FACE_OUTER_BOUND('',#27727,.T.);
#23627=FACE_OUTER_BOUND('',#27728,.T.);
#23628=FACE_OUTER_BOUND('',#27729,.T.);
#23629=FACE_OUTER_BOUND('',#27730,.T.);
#23630=FACE_OUTER_BOUND('',#27731,.T.);
#23631=FACE_OUTER_BOUND('',#27732,.T.);
#23632=FACE_OUTER_BOUND('',#27733,.T.);
#23633=FACE_OUTER_BOUND('',#27734,.T.);
#23634=FACE_OUTER_BOUND('',#27735,.T.);
#23635=FACE_OUTER_BOUND('',#27736,.T.);
#23636=FACE_OUTER_BOUND('',#27737,.T.);
#23637=FACE_OUTER_BOUND('',#27738,.T.);
#23638=FACE_OUTER_BOUND('',#27739,.T.);
#23639=FACE_OUTER_BOUND('',#27740,.T.);
#23640=FACE_OUTER_BOUND('',#27741,.T.);
#23641=FACE_OUTER_BOUND('',#27742,.T.);
#23642=FACE_OUTER_BOUND('',#27743,.T.);
#23643=FACE_OUTER_BOUND('',#27744,.T.);
#23644=FACE_OUTER_BOUND('',#27745,.T.);
#23645=FACE_OUTER_BOUND('',#27746,.T.);
#23646=FACE_OUTER_BOUND('',#27747,.T.);
#23647=FACE_OUTER_BOUND('',#27748,.T.);
#23648=FACE_OUTER_BOUND('',#27749,.T.);
#23649=FACE_OUTER_BOUND('',#27750,.T.);
#23650=FACE_OUTER_BOUND('',#27751,.T.);
#23651=FACE_OUTER_BOUND('',#27752,.T.);
#23652=FACE_OUTER_BOUND('',#27753,.T.);
#23653=FACE_OUTER_BOUND('',#27754,.T.);
#23654=FACE_OUTER_BOUND('',#27755,.T.);
#23655=FACE_OUTER_BOUND('',#27756,.T.);
#23656=FACE_OUTER_BOUND('',#27757,.T.);
#23657=FACE_OUTER_BOUND('',#27758,.T.);
#23658=FACE_OUTER_BOUND('',#27759,.T.);
#23659=FACE_OUTER_BOUND('',#27760,.T.);
#23660=FACE_OUTER_BOUND('',#27761,.T.);
#23661=FACE_OUTER_BOUND('',#27762,.T.);
#23662=FACE_OUTER_BOUND('',#27763,.T.);
#23663=FACE_OUTER_BOUND('',#27764,.T.);
#23664=FACE_OUTER_BOUND('',#27765,.T.);
#23665=FACE_OUTER_BOUND('',#27766,.T.);
#23666=FACE_OUTER_BOUND('',#27767,.T.);
#23667=FACE_OUTER_BOUND('',#27768,.T.);
#23668=FACE_OUTER_BOUND('',#27769,.T.);
#23669=FACE_OUTER_BOUND('',#27770,.T.);
#23670=FACE_OUTER_BOUND('',#27771,.T.);
#23671=FACE_OUTER_BOUND('',#27772,.T.);
#23672=FACE_OUTER_BOUND('',#27773,.T.);
#23673=FACE_OUTER_BOUND('',#27774,.T.);
#23674=FACE_OUTER_BOUND('',#27775,.T.);
#23675=FACE_OUTER_BOUND('',#27776,.T.);
#23676=FACE_OUTER_BOUND('',#27777,.T.);
#23677=FACE_OUTER_BOUND('',#27778,.T.);
#23678=FACE_OUTER_BOUND('',#27779,.T.);
#23679=FACE_OUTER_BOUND('',#27780,.T.);
#23680=FACE_OUTER_BOUND('',#27781,.T.);
#23681=FACE_OUTER_BOUND('',#27782,.T.);
#23682=FACE_OUTER_BOUND('',#27783,.T.);
#23683=FACE_OUTER_BOUND('',#27784,.T.);
#23684=FACE_OUTER_BOUND('',#27785,.T.);
#23685=FACE_OUTER_BOUND('',#27786,.T.);
#23686=FACE_OUTER_BOUND('',#27787,.T.);
#23687=FACE_OUTER_BOUND('',#27788,.T.);
#23688=FACE_OUTER_BOUND('',#27789,.T.);
#23689=FACE_OUTER_BOUND('',#27790,.T.);
#23690=FACE_OUTER_BOUND('',#27791,.T.);
#23691=FACE_OUTER_BOUND('',#27792,.T.);
#23692=FACE_OUTER_BOUND('',#27793,.T.);
#23693=FACE_OUTER_BOUND('',#27794,.T.);
#23694=FACE_OUTER_BOUND('',#27795,.T.);
#23695=FACE_OUTER_BOUND('',#27796,.T.);
#23696=FACE_OUTER_BOUND('',#27797,.T.);
#23697=FACE_OUTER_BOUND('',#27798,.T.);
#23698=FACE_OUTER_BOUND('',#27799,.T.);
#23699=FACE_OUTER_BOUND('',#27800,.T.);
#23700=FACE_OUTER_BOUND('',#27801,.T.);
#23701=FACE_OUTER_BOUND('',#27803,.T.);
#23702=FACE_OUTER_BOUND('',#28241,.T.);
#23703=FACE_OUTER_BOUND('',#28242,.T.);
#23704=FACE_OUTER_BOUND('',#28243,.T.);
#23705=FACE_OUTER_BOUND('',#28244,.T.);
#23706=FACE_OUTER_BOUND('',#28245,.T.);
#23707=FACE_OUTER_BOUND('',#28683,.T.);
#23708=FACE_OUTER_BOUND('',#28685,.T.);
#23709=FACE_OUTER_BOUND('',#28686,.T.);
#23710=FACE_OUTER_BOUND('',#28687,.T.);
#23711=FACE_OUTER_BOUND('',#28688,.T.);
#23712=FACE_OUTER_BOUND('',#28689,.T.);
#23713=FACE_OUTER_BOUND('',#28690,.T.);
#23714=FACE_OUTER_BOUND('',#28691,.T.);
#23715=FACE_OUTER_BOUND('',#28692,.T.);
#23716=FACE_OUTER_BOUND('',#28693,.T.);
#23717=FACE_OUTER_BOUND('',#28694,.T.);
#23718=FACE_OUTER_BOUND('',#28695,.T.);
#23719=FACE_OUTER_BOUND('',#28696,.T.);
#23720=FACE_OUTER_BOUND('',#28697,.T.);
#23721=FACE_OUTER_BOUND('',#28699,.T.);
#23722=FACE_OUTER_BOUND('',#28956,.T.);
#23723=FACE_OUTER_BOUND('',#28957,.T.);
#23724=FACE_OUTER_BOUND('',#28958,.T.);
#23725=FACE_OUTER_BOUND('',#28959,.T.);
#23726=FACE_OUTER_BOUND('',#28960,.T.);
#23727=FACE_OUTER_BOUND('',#29217,.T.);
#24943=EDGE_LOOP('',(#57171,#57172,#57173));
#24944=EDGE_LOOP('',(#57174,#57175,#57176,#57177,#57178));
#24945=EDGE_LOOP('',(#57179,#57180,#57181,#57182));
#24946=EDGE_LOOP('',(#57183,#57184,#57185,#57186,#57187));
#24947=EDGE_LOOP('',(#57188,#57189,#57190,#57191,#57192));
#24948=EDGE_LOOP('',(#57193,#57194,#57195,#57196,#57197));
#24949=EDGE_LOOP('',(#57198,#57199,#57200,#57201));
#24950=EDGE_LOOP('',(#57202,#57203,#57204,#57205));
#24951=EDGE_LOOP('',(#57206,#57207,#57208,#57209));
#24952=EDGE_LOOP('',(#57210,#57211,#57212,#57213,#57214,#57215,#57216,#57217,
#57218,#57219,#57220,#57221));
#24953=EDGE_LOOP('',(#57222,#57223,#57224,#57225));
#24954=EDGE_LOOP('',(#57226,#57227,#57228,#57229));
#24955=EDGE_LOOP('',(#57230,#57231,#57232,#57233));
#24956=EDGE_LOOP('',(#57234,#57235,#57236,#57237));
#24957=EDGE_LOOP('',(#57238,#57239,#57240,#57241));
#24958=EDGE_LOOP('',(#57242,#57243,#57244,#57245,#57246,#57247,#57248,#57249,
#57250,#57251,#57252,#57253));
#24959=EDGE_LOOP('',(#57254,#57255,#57256,#57257));
#24960=EDGE_LOOP('',(#57258,#57259,#57260,#57261));
#24961=EDGE_LOOP('',(#57262,#57263,#57264,#57265));
#24962=EDGE_LOOP('',(#57266,#57267,#57268,#57269));
#24963=EDGE_LOOP('',(#57270,#57271,#57272,#57273));
#24964=EDGE_LOOP('',(#57274,#57275,#57276,#57277));
#24965=EDGE_LOOP('',(#57278,#57279,#57280,#57281));
#24966=EDGE_LOOP('',(#57282,#57283,#57284,#57285,#57286));
#24967=EDGE_LOOP('',(#57287,#57288,#57289,#57290,#57291));
#24968=EDGE_LOOP('',(#57292,#57293,#57294,#57295));
#24969=EDGE_LOOP('',(#57296,#57297,#57298,#57299));
#24970=EDGE_LOOP('',(#57300,#57301,#57302,#57303));
#24971=EDGE_LOOP('',(#57304,#57305,#57306,#57307,#57308,#57309,#57310,#57311,
#57312,#57313,#57314,#57315));
#24972=EDGE_LOOP('',(#57316,#57317,#57318,#57319,#57320,#57321));
#24973=EDGE_LOOP('',(#57322,#57323,#57324,#57325));
#24974=EDGE_LOOP('',(#57326,#57327,#57328,#57329,#57330,#57331,#57332));
#24975=EDGE_LOOP('',(#57333,#57334,#57335,#57336,#57337));
#24976=EDGE_LOOP('',(#57338,#57339,#57340,#57341,#57342));
#24977=EDGE_LOOP('',(#57343,#57344,#57345,#57346,#57347,#57348));
#24978=EDGE_LOOP('',(#57349,#57350,#57351,#57352));
#24979=EDGE_LOOP('',(#57353,#57354,#57355,#57356));
#24980=EDGE_LOOP('',(#57357,#57358,#57359,#57360,#57361,#57362));
#24981=EDGE_LOOP('',(#57363,#57364));
#24982=EDGE_LOOP('',(#57365,#57366,#57367));
#24983=EDGE_LOOP('',(#57368));
#24984=EDGE_LOOP('',(#57369));
#24985=EDGE_LOOP('',(#57370,#57371,#57372,#57373,#57374,#57375,#57376,#57377));
#24986=EDGE_LOOP('',(#57378));
#24987=EDGE_LOOP('',(#57379,#57380,#57381,#57382,#57383,#57384,#57385));
#24988=EDGE_LOOP('',(#57386,#57387,#57388));
#24989=EDGE_LOOP('',(#57389,#57390,#57391,#57392,#57393,#57394));
#24990=EDGE_LOOP('',(#57395,#57396,#57397,#57398,#57399,#57400));
#24991=EDGE_LOOP('',(#57401,#57402,#57403,#57404,#57405,#57406));
#24992=EDGE_LOOP('',(#57407));
#24993=EDGE_LOOP('',(#57408));
#24994=EDGE_LOOP('',(#57409));
#24995=EDGE_LOOP('',(#57410,#57411,#57412,#57413));
#24996=EDGE_LOOP('',(#57414));
#24997=EDGE_LOOP('',(#57415,#57416,#57417,#57418));
#24998=EDGE_LOOP('',(#57419,#57420,#57421,#57422,#57423));
#24999=EDGE_LOOP('',(#57424,#57425,#57426,#57427));
#25000=EDGE_LOOP('',(#57428,#57429,#57430,#57431,#57432));
#25001=EDGE_LOOP('',(#57433,#57434,#57435,#57436));
#25002=EDGE_LOOP('',(#57437,#57438,#57439,#57440));
#25003=EDGE_LOOP('',(#57441,#57442,#57443,#57444,#57445));
#25004=EDGE_LOOP('',(#57446,#57447,#57448,#57449));
#25005=EDGE_LOOP('',(#57450,#57451,#57452,#57453,#57454));
#25006=EDGE_LOOP('',(#57455,#57456,#57457,#57458));
#25007=EDGE_LOOP('',(#57459,#57460,#57461,#57462));
#25008=EDGE_LOOP('',(#57463,#57464,#57465,#57466));
#25009=EDGE_LOOP('',(#57467,#57468,#57469,#57470));
#25010=EDGE_LOOP('',(#57471,#57472,#57473,#57474,#57475));
#25011=EDGE_LOOP('',(#57476,#57477,#57478,#57479));
#25012=EDGE_LOOP('',(#57480,#57481,#57482,#57483));
#25013=EDGE_LOOP('',(#57484,#57485,#57486,#57487));
#25014=EDGE_LOOP('',(#57488,#57489,#57490,#57491));
#25015=EDGE_LOOP('',(#57492,#57493,#57494,#57495));
#25016=EDGE_LOOP('',(#57496,#57497,#57498,#57499));
#25017=EDGE_LOOP('',(#57500,#57501,#57502,#57503));
#25018=EDGE_LOOP('',(#57504,#57505,#57506,#57507));
#25019=EDGE_LOOP('',(#57508,#57509,#57510,#57511));
#25020=EDGE_LOOP('',(#57512,#57513,#57514,#57515));
#25021=EDGE_LOOP('',(#57516,#57517,#57518,#57519));
#25022=EDGE_LOOP('',(#57520,#57521,#57522,#57523));
#25023=EDGE_LOOP('',(#57524,#57525,#57526,#57527));
#25024=EDGE_LOOP('',(#57528,#57529,#57530,#57531));
#25025=EDGE_LOOP('',(#57532,#57533,#57534,#57535));
#25026=EDGE_LOOP('',(#57536,#57537,#57538,#57539));
#25027=EDGE_LOOP('',(#57540,#57541,#57542,#57543));
#25028=EDGE_LOOP('',(#57544,#57545,#57546,#57547));
#25029=EDGE_LOOP('',(#57548,#57549,#57550,#57551,#57552));
#25030=EDGE_LOOP('',(#57553,#57554,#57555,#57556));
#25031=EDGE_LOOP('',(#57557,#57558,#57559,#57560,#57561));
#25032=EDGE_LOOP('',(#57562,#57563,#57564,#57565));
#25033=EDGE_LOOP('',(#57566,#57567,#57568,#57569));
#25034=EDGE_LOOP('',(#57570,#57571,#57572,#57573,#57574));
#25035=EDGE_LOOP('',(#57575,#57576,#57577,#57578));
#25036=EDGE_LOOP('',(#57579,#57580,#57581,#57582,#57583));
#25037=EDGE_LOOP('',(#57584,#57585,#57586,#57587));
#25038=EDGE_LOOP('',(#57588,#57589,#57590,#57591));
#25039=EDGE_LOOP('',(#57592,#57593,#57594,#57595,#57596));
#25040=EDGE_LOOP('',(#57597,#57598,#57599,#57600));
#25041=EDGE_LOOP('',(#57601,#57602,#57603,#57604,#57605));
#25042=EDGE_LOOP('',(#57606,#57607,#57608,#57609));
#25043=EDGE_LOOP('',(#57610,#57611,#57612,#57613));
#25044=EDGE_LOOP('',(#57614,#57615,#57616,#57617));
#25045=EDGE_LOOP('',(#57618,#57619,#57620,#57621,#57622));
#25046=EDGE_LOOP('',(#57623,#57624,#57625,#57626,#57627));
#25047=EDGE_LOOP('',(#57628,#57629,#57630));
#25048=EDGE_LOOP('',(#57631,#57632,#57633,#57634));
#25049=EDGE_LOOP('',(#57635,#57636,#57637,#57638));
#25050=EDGE_LOOP('',(#57639,#57640,#57641,#57642));
#25051=EDGE_LOOP('',(#57643,#57644,#57645,#57646));
#25052=EDGE_LOOP('',(#57647,#57648,#57649,#57650));
#25053=EDGE_LOOP('',(#57651,#57652,#57653,#57654,#57655));
#25054=EDGE_LOOP('',(#57656,#57657,#57658,#57659));
#25055=EDGE_LOOP('',(#57660,#57661,#57662,#57663,#57664));
#25056=EDGE_LOOP('',(#57665,#57666,#57667,#57668));
#25057=EDGE_LOOP('',(#57669,#57670,#57671,#57672));
#25058=EDGE_LOOP('',(#57673,#57674,#57675,#57676,#57677));
#25059=EDGE_LOOP('',(#57678,#57679,#57680,#57681));
#25060=EDGE_LOOP('',(#57682,#57683,#57684,#57685,#57686));
#25061=EDGE_LOOP('',(#57687,#57688,#57689,#57690));
#25062=EDGE_LOOP('',(#57691,#57692,#57693,#57694));
#25063=EDGE_LOOP('',(#57695,#57696,#57697,#57698,#57699));
#25064=EDGE_LOOP('',(#57700,#57701,#57702,#57703));
#25065=EDGE_LOOP('',(#57704,#57705,#57706,#57707,#57708));
#25066=EDGE_LOOP('',(#57709,#57710,#57711,#57712));
#25067=EDGE_LOOP('',(#57713,#57714,#57715,#57716));
#25068=EDGE_LOOP('',(#57717,#57718,#57719,#57720,#57721));
#25069=EDGE_LOOP('',(#57722,#57723,#57724,#57725));
#25070=EDGE_LOOP('',(#57726,#57727,#57728,#57729,#57730));
#25071=EDGE_LOOP('',(#57731,#57732,#57733,#57734));
#25072=EDGE_LOOP('',(#57735,#57736,#57737,#57738));
#25073=EDGE_LOOP('',(#57739,#57740,#57741,#57742));
#25074=EDGE_LOOP('',(#57743,#57744,#57745,#57746));
#25075=EDGE_LOOP('',(#57747,#57748,#57749,#57750));
#25076=EDGE_LOOP('',(#57751,#57752,#57753,#57754));
#25077=EDGE_LOOP('',(#57755,#57756,#57757,#57758));
#25078=EDGE_LOOP('',(#57759,#57760,#57761,#57762));
#25079=EDGE_LOOP('',(#57763,#57764,#57765,#57766));
#25080=EDGE_LOOP('',(#57767,#57768,#57769,#57770));
#25081=EDGE_LOOP('',(#57771,#57772,#57773,#57774));
#25082=EDGE_LOOP('',(#57775,#57776,#57777,#57778));
#25083=EDGE_LOOP('',(#57779,#57780,#57781,#57782));
#25084=EDGE_LOOP('',(#57783,#57784,#57785,#57786));
#25085=EDGE_LOOP('',(#57787,#57788,#57789,#57790));
#25086=EDGE_LOOP('',(#57791,#57792,#57793,#57794));
#25087=EDGE_LOOP('',(#57795,#57796,#57797,#57798));
#25088=EDGE_LOOP('',(#57799,#57800,#57801,#57802));
#25089=EDGE_LOOP('',(#57803,#57804,#57805,#57806));
#25090=EDGE_LOOP('',(#57807,#57808,#57809,#57810));
#25091=EDGE_LOOP('',(#57811,#57812,#57813,#57814));
#25092=EDGE_LOOP('',(#57815,#57816,#57817,#57818));
#25093=EDGE_LOOP('',(#57819,#57820,#57821,#57822));
#25094=EDGE_LOOP('',(#57823,#57824,#57825,#57826));
#25095=EDGE_LOOP('',(#57827,#57828,#57829,#57830));
#25096=EDGE_LOOP('',(#57831,#57832,#57833,#57834));
#25097=EDGE_LOOP('',(#57835,#57836,#57837,#57838));
#25098=EDGE_LOOP('',(#57839,#57840,#57841,#57842,#57843));
#25099=EDGE_LOOP('',(#57844,#57845,#57846,#57847,#57848));
#25100=EDGE_LOOP('',(#57849,#57850,#57851));
#25101=EDGE_LOOP('',(#57852,#57853,#57854,#57855));
#25102=EDGE_LOOP('',(#57856,#57857,#57858,#57859,#57860));
#25103=EDGE_LOOP('',(#57861,#57862,#57863,#57864));
#25104=EDGE_LOOP('',(#57865,#57866,#57867,#57868,#57869));
#25105=EDGE_LOOP('',(#57870,#57871,#57872,#57873));
#25106=EDGE_LOOP('',(#57874,#57875,#57876,#57877));
#25107=EDGE_LOOP('',(#57878,#57879,#57880,#57881));
#25108=EDGE_LOOP('',(#57882,#57883,#57884,#57885));
#25109=EDGE_LOOP('',(#57886,#57887,#57888,#57889));
#25110=EDGE_LOOP('',(#57890,#57891,#57892,#57893));
#25111=EDGE_LOOP('',(#57894,#57895,#57896,#57897));
#25112=EDGE_LOOP('',(#57898,#57899,#57900,#57901));
#25113=EDGE_LOOP('',(#57902,#57903,#57904,#57905));
#25114=EDGE_LOOP('',(#57906,#57907,#57908,#57909));
#25115=EDGE_LOOP('',(#57910,#57911,#57912,#57913));
#25116=EDGE_LOOP('',(#57914,#57915,#57916,#57917));
#25117=EDGE_LOOP('',(#57918,#57919,#57920,#57921));
#25118=EDGE_LOOP('',(#57922,#57923,#57924,#57925));
#25119=EDGE_LOOP('',(#57926,#57927,#57928,#57929));
#25120=EDGE_LOOP('',(#57930,#57931,#57932,#57933));
#25121=EDGE_LOOP('',(#57934,#57935,#57936,#57937));
#25122=EDGE_LOOP('',(#57938,#57939,#57940,#57941));
#25123=EDGE_LOOP('',(#57942,#57943,#57944,#57945));
#25124=EDGE_LOOP('',(#57946,#57947,#57948,#57949));
#25125=EDGE_LOOP('',(#57950,#57951,#57952,#57953));
#25126=EDGE_LOOP('',(#57954,#57955,#57956,#57957));
#25127=EDGE_LOOP('',(#57958,#57959,#57960,#57961));
#25128=EDGE_LOOP('',(#57962,#57963,#57964,#57965));
#25129=EDGE_LOOP('',(#57966,#57967,#57968,#57969));
#25130=EDGE_LOOP('',(#57970,#57971,#57972,#57973));
#25131=EDGE_LOOP('',(#57974,#57975,#57976,#57977));
#25132=EDGE_LOOP('',(#57978,#57979,#57980,#57981));
#25133=EDGE_LOOP('',(#57982,#57983,#57984,#57985));
#25134=EDGE_LOOP('',(#57986,#57987,#57988,#57989));
#25135=EDGE_LOOP('',(#57990,#57991,#57992,#57993));
#25136=EDGE_LOOP('',(#57994,#57995,#57996,#57997));
#25137=EDGE_LOOP('',(#57998,#57999,#58000,#58001));
#25138=EDGE_LOOP('',(#58002,#58003,#58004,#58005));
#25139=EDGE_LOOP('',(#58006,#58007,#58008,#58009,#58010));
#25140=EDGE_LOOP('',(#58011,#58012,#58013,#58014));
#25141=EDGE_LOOP('',(#58015,#58016,#58017,#58018,#58019));
#25142=EDGE_LOOP('',(#58020,#58021,#58022,#58023));
#25143=EDGE_LOOP('',(#58024,#58025,#58026,#58027));
#25144=EDGE_LOOP('',(#58028,#58029,#58030,#58031,#58032));
#25145=EDGE_LOOP('',(#58033,#58034,#58035,#58036));
#25146=EDGE_LOOP('',(#58037,#58038,#58039,#58040,#58041));
#25147=EDGE_LOOP('',(#58042,#58043,#58044,#58045));
#25148=EDGE_LOOP('',(#58046,#58047,#58048,#58049));
#25149=EDGE_LOOP('',(#58050,#58051,#58052,#58053));
#25150=EDGE_LOOP('',(#58054,#58055,#58056,#58057));
#25151=EDGE_LOOP('',(#58058,#58059,#58060,#58061));
#25152=EDGE_LOOP('',(#58062,#58063,#58064,#58065));
#25153=EDGE_LOOP('',(#58066,#58067,#58068,#58069));
#25154=EDGE_LOOP('',(#58070,#58071,#58072,#58073));
#25155=EDGE_LOOP('',(#58074,#58075,#58076,#58077));
#25156=EDGE_LOOP('',(#58078,#58079,#58080,#58081));
#25157=EDGE_LOOP('',(#58082,#58083,#58084,#58085));
#25158=EDGE_LOOP('',(#58086,#58087,#58088,#58089));
#25159=EDGE_LOOP('',(#58090,#58091,#58092,#58093));
#25160=EDGE_LOOP('',(#58094,#58095,#58096,#58097));
#25161=EDGE_LOOP('',(#58098,#58099,#58100,#58101));
#25162=EDGE_LOOP('',(#58102,#58103,#58104,#58105));
#25163=EDGE_LOOP('',(#58106,#58107,#58108,#58109));
#25164=EDGE_LOOP('',(#58110,#58111,#58112,#58113));
#25165=EDGE_LOOP('',(#58114,#58115,#58116,#58117));
#25166=EDGE_LOOP('',(#58118,#58119,#58120,#58121));
#25167=EDGE_LOOP('',(#58122,#58123,#58124,#58125));
#25168=EDGE_LOOP('',(#58126,#58127,#58128,#58129));
#25169=EDGE_LOOP('',(#58130,#58131,#58132,#58133));
#25170=EDGE_LOOP('',(#58134,#58135,#58136,#58137));
#25171=EDGE_LOOP('',(#58138,#58139,#58140,#58141));
#25172=EDGE_LOOP('',(#58142,#58143,#58144,#58145));
#25173=EDGE_LOOP('',(#58146,#58147,#58148,#58149));
#25174=EDGE_LOOP('',(#58150,#58151,#58152,#58153));
#25175=EDGE_LOOP('',(#58154,#58155,#58156,#58157));
#25176=EDGE_LOOP('',(#58158,#58159,#58160,#58161));
#25177=EDGE_LOOP('',(#58162,#58163,#58164,#58165));
#25178=EDGE_LOOP('',(#58166,#58167,#58168,#58169));
#25179=EDGE_LOOP('',(#58170,#58171,#58172,#58173));
#25180=EDGE_LOOP('',(#58174,#58175,#58176,#58177));
#25181=EDGE_LOOP('',(#58178,#58179,#58180,#58181));
#25182=EDGE_LOOP('',(#58182,#58183,#58184,#58185));
#25183=EDGE_LOOP('',(#58186,#58187,#58188,#58189));
#25184=EDGE_LOOP('',(#58190,#58191,#58192,#58193));
#25185=EDGE_LOOP('',(#58194,#58195,#58196,#58197));
#25186=EDGE_LOOP('',(#58198,#58199,#58200,#58201));
#25187=EDGE_LOOP('',(#58202,#58203,#58204,#58205));
#25188=EDGE_LOOP('',(#58206,#58207,#58208));
#25189=EDGE_LOOP('',(#58209,#58210,#58211,#58212));
#25190=EDGE_LOOP('',(#58213,#58214,#58215,#58216));
#25191=EDGE_LOOP('',(#58217,#58218,#58219,#58220,#58221));
#25192=EDGE_LOOP('',(#58222,#58223,#58224,#58225,#58226));
#25193=EDGE_LOOP('',(#58227,#58228,#58229,#58230));
#25194=EDGE_LOOP('',(#58231,#58232,#58233,#58234));
#25195=EDGE_LOOP('',(#58235,#58236,#58237,#58238));
#25196=EDGE_LOOP('',(#58239,#58240,#58241,#58242));
#25197=EDGE_LOOP('',(#58243,#58244,#58245,#58246));
#25198=EDGE_LOOP('',(#58247,#58248,#58249,#58250));
#25199=EDGE_LOOP('',(#58251,#58252,#58253,#58254));
#25200=EDGE_LOOP('',(#58255,#58256,#58257,#58258));
#25201=EDGE_LOOP('',(#58259,#58260,#58261,#58262));
#25202=EDGE_LOOP('',(#58263,#58264,#58265,#58266));
#25203=EDGE_LOOP('',(#58267,#58268,#58269,#58270));
#25204=EDGE_LOOP('',(#58271,#58272,#58273,#58274));
#25205=EDGE_LOOP('',(#58275,#58276,#58277,#58278));
#25206=EDGE_LOOP('',(#58279,#58280,#58281,#58282));
#25207=EDGE_LOOP('',(#58283,#58284,#58285,#58286));
#25208=EDGE_LOOP('',(#58287,#58288,#58289,#58290));
#25209=EDGE_LOOP('',(#58291,#58292,#58293,#58294));
#25210=EDGE_LOOP('',(#58295,#58296,#58297,#58298));
#25211=EDGE_LOOP('',(#58299,#58300,#58301,#58302));
#25212=EDGE_LOOP('',(#58303,#58304,#58305,#58306));
#25213=EDGE_LOOP('',(#58307,#58308,#58309,#58310));
#25214=EDGE_LOOP('',(#58311,#58312,#58313,#58314));
#25215=EDGE_LOOP('',(#58315,#58316,#58317,#58318));
#25216=EDGE_LOOP('',(#58319,#58320,#58321,#58322));
#25217=EDGE_LOOP('',(#58323,#58324,#58325,#58326));
#25218=EDGE_LOOP('',(#58327,#58328,#58329,#58330));
#25219=EDGE_LOOP('',(#58331,#58332,#58333,#58334));
#25220=EDGE_LOOP('',(#58335,#58336,#58337,#58338));
#25221=EDGE_LOOP('',(#58339,#58340,#58341,#58342));
#25222=EDGE_LOOP('',(#58343,#58344,#58345,#58346));
#25223=EDGE_LOOP('',(#58347,#58348,#58349,#58350));
#25224=EDGE_LOOP('',(#58351,#58352,#58353,#58354));
#25225=EDGE_LOOP('',(#58355,#58356,#58357,#58358));
#25226=EDGE_LOOP('',(#58359,#58360,#58361,#58362));
#25227=EDGE_LOOP('',(#58363,#58364,#58365,#58366));
#25228=EDGE_LOOP('',(#58367,#58368,#58369,#58370));
#25229=EDGE_LOOP('',(#58371,#58372,#58373,#58374));
#25230=EDGE_LOOP('',(#58375,#58376,#58377,#58378));
#25231=EDGE_LOOP('',(#58379,#58380,#58381,#58382));
#25232=EDGE_LOOP('',(#58383,#58384,#58385,#58386));
#25233=EDGE_LOOP('',(#58387,#58388,#58389,#58390));
#25234=EDGE_LOOP('',(#58391,#58392,#58393,#58394));
#25235=EDGE_LOOP('',(#58395,#58396,#58397,#58398,#58399));
#25236=EDGE_LOOP('',(#58400,#58401,#58402,#58403,#58404));
#25237=EDGE_LOOP('',(#58405,#58406,#58407));
#25238=EDGE_LOOP('',(#58408,#58409,#58410,#58411));
#25239=EDGE_LOOP('',(#58412,#58413,#58414,#58415));
#25240=EDGE_LOOP('',(#58416,#58417,#58418,#58419,#58420));
#25241=EDGE_LOOP('',(#58421,#58422,#58423,#58424,#58425));
#25242=EDGE_LOOP('',(#58426,#58427,#58428));
#25243=EDGE_LOOP('',(#58429,#58430,#58431,#58432));
#25244=EDGE_LOOP('',(#58433,#58434,#58435,#58436));
#25245=EDGE_LOOP('',(#58437,#58438,#58439,#58440));
#25246=EDGE_LOOP('',(#58441,#58442,#58443,#58444));
#25247=EDGE_LOOP('',(#58445,#58446,#58447,#58448));
#25248=EDGE_LOOP('',(#58449,#58450,#58451,#58452));
#25249=EDGE_LOOP('',(#58453,#58454,#58455,#58456));
#25250=EDGE_LOOP('',(#58457,#58458,#58459,#58460));
#25251=EDGE_LOOP('',(#58461,#58462,#58463,#58464));
#25252=EDGE_LOOP('',(#58465,#58466,#58467,#58468));
#25253=EDGE_LOOP('',(#58469,#58470,#58471,#58472));
#25254=EDGE_LOOP('',(#58473,#58474,#58475,#58476));
#25255=EDGE_LOOP('',(#58477,#58478,#58479,#58480));
#25256=EDGE_LOOP('',(#58481,#58482,#58483,#58484));
#25257=EDGE_LOOP('',(#58485,#58486,#58487,#58488));
#25258=EDGE_LOOP('',(#58489,#58490,#58491,#58492));
#25259=EDGE_LOOP('',(#58493,#58494,#58495,#58496));
#25260=EDGE_LOOP('',(#58497,#58498,#58499,#58500));
#25261=EDGE_LOOP('',(#58501,#58502,#58503,#58504));
#25262=EDGE_LOOP('',(#58505,#58506,#58507,#58508));
#25263=EDGE_LOOP('',(#58509,#58510,#58511,#58512));
#25264=EDGE_LOOP('',(#58513,#58514,#58515,#58516));
#25265=EDGE_LOOP('',(#58517,#58518,#58519,#58520));
#25266=EDGE_LOOP('',(#58521,#58522,#58523,#58524));
#25267=EDGE_LOOP('',(#58525,#58526,#58527,#58528));
#25268=EDGE_LOOP('',(#58529,#58530,#58531,#58532));
#25269=EDGE_LOOP('',(#58533,#58534,#58535,#58536));
#25270=EDGE_LOOP('',(#58537,#58538,#58539,#58540));
#25271=EDGE_LOOP('',(#58541,#58542,#58543,#58544));
#25272=EDGE_LOOP('',(#58545,#58546,#58547,#58548));
#25273=EDGE_LOOP('',(#58549,#58550,#58551,#58552));
#25274=EDGE_LOOP('',(#58553,#58554,#58555,#58556));
#25275=EDGE_LOOP('',(#58557,#58558,#58559,#58560));
#25276=EDGE_LOOP('',(#58561,#58562,#58563,#58564));
#25277=EDGE_LOOP('',(#58565,#58566,#58567,#58568));
#25278=EDGE_LOOP('',(#58569,#58570,#58571,#58572));
#25279=EDGE_LOOP('',(#58573,#58574,#58575,#58576));
#25280=EDGE_LOOP('',(#58577,#58578,#58579,#58580));
#25281=EDGE_LOOP('',(#58581,#58582,#58583,#58584));
#25282=EDGE_LOOP('',(#58585,#58586,#58587,#58588));
#25283=EDGE_LOOP('',(#58589,#58590,#58591,#58592));
#25284=EDGE_LOOP('',(#58593,#58594,#58595,#58596));
#25285=EDGE_LOOP('',(#58597,#58598,#58599,#58600));
#25286=EDGE_LOOP('',(#58601,#58602,#58603,#58604));
#25287=EDGE_LOOP('',(#58605,#58606,#58607,#58608));
#25288=EDGE_LOOP('',(#58609,#58610,#58611,#58612));
#25289=EDGE_LOOP('',(#58613,#58614,#58615,#58616));
#25290=EDGE_LOOP('',(#58617,#58618,#58619,#58620));
#25291=EDGE_LOOP('',(#58621,#58622,#58623,#58624));
#25292=EDGE_LOOP('',(#58625,#58626,#58627,#58628));
#25293=EDGE_LOOP('',(#58629,#58630,#58631,#58632));
#25294=EDGE_LOOP('',(#58633,#58634,#58635,#58636));
#25295=EDGE_LOOP('',(#58637,#58638,#58639,#58640));
#25296=EDGE_LOOP('',(#58641,#58642,#58643,#58644));
#25297=EDGE_LOOP('',(#58645,#58646,#58647,#58648));
#25298=EDGE_LOOP('',(#58649,#58650,#58651,#58652));
#25299=EDGE_LOOP('',(#58653,#58654,#58655,#58656));
#25300=EDGE_LOOP('',(#58657,#58658,#58659,#58660));
#25301=EDGE_LOOP('',(#58661,#58662,#58663,#58664));
#25302=EDGE_LOOP('',(#58665,#58666,#58667,#58668));
#25303=EDGE_LOOP('',(#58669,#58670,#58671,#58672));
#25304=EDGE_LOOP('',(#58673,#58674,#58675,#58676));
#25305=EDGE_LOOP('',(#58677,#58678,#58679,#58680));
#25306=EDGE_LOOP('',(#58681,#58682,#58683,#58684));
#25307=EDGE_LOOP('',(#58685,#58686,#58687,#58688));
#25308=EDGE_LOOP('',(#58689,#58690,#58691,#58692));
#25309=EDGE_LOOP('',(#58693,#58694,#58695,#58696));
#25310=EDGE_LOOP('',(#58697,#58698,#58699,#58700));
#25311=EDGE_LOOP('',(#58701,#58702,#58703,#58704));
#25312=EDGE_LOOP('',(#58705,#58706,#58707,#58708));
#25313=EDGE_LOOP('',(#58709,#58710,#58711,#58712));
#25314=EDGE_LOOP('',(#58713,#58714,#58715,#58716));
#25315=EDGE_LOOP('',(#58717,#58718,#58719,#58720));
#25316=EDGE_LOOP('',(#58721,#58722,#58723,#58724));
#25317=EDGE_LOOP('',(#58725,#58726,#58727,#58728));
#25318=EDGE_LOOP('',(#58729,#58730,#58731,#58732));
#25319=EDGE_LOOP('',(#58733,#58734,#58735,#58736));
#25320=EDGE_LOOP('',(#58737,#58738,#58739,#58740));
#25321=EDGE_LOOP('',(#58741,#58742,#58743,#58744));
#25322=EDGE_LOOP('',(#58745,#58746,#58747,#58748));
#25323=EDGE_LOOP('',(#58749,#58750,#58751,#58752));
#25324=EDGE_LOOP('',(#58753,#58754,#58755,#58756));
#25325=EDGE_LOOP('',(#58757,#58758,#58759,#58760));
#25326=EDGE_LOOP('',(#58761,#58762,#58763,#58764));
#25327=EDGE_LOOP('',(#58765,#58766,#58767,#58768));
#25328=EDGE_LOOP('',(#58769,#58770,#58771,#58772));
#25329=EDGE_LOOP('',(#58773,#58774,#58775,#58776));
#25330=EDGE_LOOP('',(#58777,#58778,#58779,#58780));
#25331=EDGE_LOOP('',(#58781,#58782,#58783,#58784));
#25332=EDGE_LOOP('',(#58785,#58786,#58787,#58788));
#25333=EDGE_LOOP('',(#58789,#58790,#58791,#58792));
#25334=EDGE_LOOP('',(#58793,#58794,#58795,#58796));
#25335=EDGE_LOOP('',(#58797,#58798,#58799,#58800));
#25336=EDGE_LOOP('',(#58801,#58802,#58803,#58804));
#25337=EDGE_LOOP('',(#58805,#58806,#58807,#58808));
#25338=EDGE_LOOP('',(#58809,#58810,#58811,#58812));
#25339=EDGE_LOOP('',(#58813,#58814,#58815,#58816));
#25340=EDGE_LOOP('',(#58817,#58818,#58819,#58820));
#25341=EDGE_LOOP('',(#58821,#58822,#58823,#58824));
#25342=EDGE_LOOP('',(#58825,#58826,#58827,#58828));
#25343=EDGE_LOOP('',(#58829,#58830,#58831,#58832));
#25344=EDGE_LOOP('',(#58833,#58834,#58835,#58836));
#25345=EDGE_LOOP('',(#58837,#58838,#58839,#58840));
#25346=EDGE_LOOP('',(#58841,#58842,#58843,#58844));
#25347=EDGE_LOOP('',(#58845,#58846,#58847,#58848));
#25348=EDGE_LOOP('',(#58849,#58850,#58851,#58852));
#25349=EDGE_LOOP('',(#58853,#58854,#58855,#58856));
#25350=EDGE_LOOP('',(#58857,#58858,#58859,#58860));
#25351=EDGE_LOOP('',(#58861,#58862,#58863,#58864));
#25352=EDGE_LOOP('',(#58865,#58866,#58867,#58868));
#25353=EDGE_LOOP('',(#58869,#58870,#58871,#58872));
#25354=EDGE_LOOP('',(#58873,#58874,#58875,#58876));
#25355=EDGE_LOOP('',(#58877,#58878,#58879,#58880));
#25356=EDGE_LOOP('',(#58881,#58882,#58883,#58884));
#25357=EDGE_LOOP('',(#58885,#58886,#58887,#58888));
#25358=EDGE_LOOP('',(#58889,#58890,#58891,#58892));
#25359=EDGE_LOOP('',(#58893,#58894,#58895,#58896));
#25360=EDGE_LOOP('',(#58897,#58898,#58899,#58900));
#25361=EDGE_LOOP('',(#58901,#58902,#58903,#58904));
#25362=EDGE_LOOP('',(#58905,#58906,#58907,#58908));
#25363=EDGE_LOOP('',(#58909,#58910,#58911,#58912));
#25364=EDGE_LOOP('',(#58913,#58914,#58915,#58916));
#25365=EDGE_LOOP('',(#58917,#58918,#58919,#58920));
#25366=EDGE_LOOP('',(#58921,#58922,#58923,#58924));
#25367=EDGE_LOOP('',(#58925,#58926,#58927,#58928));
#25368=EDGE_LOOP('',(#58929,#58930,#58931,#58932));
#25369=EDGE_LOOP('',(#58933,#58934,#58935,#58936));
#25370=EDGE_LOOP('',(#58937,#58938,#58939,#58940));
#25371=EDGE_LOOP('',(#58941,#58942,#58943,#58944));
#25372=EDGE_LOOP('',(#58945,#58946,#58947,#58948));
#25373=EDGE_LOOP('',(#58949,#58950,#58951,#58952));
#25374=EDGE_LOOP('',(#58953,#58954,#58955,#58956));
#25375=EDGE_LOOP('',(#58957,#58958,#58959,#58960));
#25376=EDGE_LOOP('',(#58961,#58962,#58963,#58964));
#25377=EDGE_LOOP('',(#58965,#58966,#58967,#58968));
#25378=EDGE_LOOP('',(#58969,#58970,#58971,#58972));
#25379=EDGE_LOOP('',(#58973,#58974,#58975,#58976));
#25380=EDGE_LOOP('',(#58977,#58978,#58979,#58980));
#25381=EDGE_LOOP('',(#58981,#58982,#58983,#58984));
#25382=EDGE_LOOP('',(#58985,#58986,#58987,#58988));
#25383=EDGE_LOOP('',(#58989,#58990,#58991,#58992));
#25384=EDGE_LOOP('',(#58993,#58994,#58995,#58996));
#25385=EDGE_LOOP('',(#58997,#58998,#58999,#59000));
#25386=EDGE_LOOP('',(#59001,#59002,#59003,#59004));
#25387=EDGE_LOOP('',(#59005,#59006,#59007,#59008));
#25388=EDGE_LOOP('',(#59009,#59010,#59011,#59012));
#25389=EDGE_LOOP('',(#59013,#59014,#59015,#59016));
#25390=EDGE_LOOP('',(#59017,#59018,#59019,#59020));
#25391=EDGE_LOOP('',(#59021,#59022,#59023,#59024));
#25392=EDGE_LOOP('',(#59025,#59026,#59027,#59028));
#25393=EDGE_LOOP('',(#59029,#59030,#59031,#59032));
#25394=EDGE_LOOP('',(#59033,#59034,#59035,#59036));
#25395=EDGE_LOOP('',(#59037,#59038,#59039,#59040));
#25396=EDGE_LOOP('',(#59041,#59042,#59043,#59044));
#25397=EDGE_LOOP('',(#59045,#59046,#59047,#59048));
#25398=EDGE_LOOP('',(#59049,#59050,#59051,#59052));
#25399=EDGE_LOOP('',(#59053,#59054,#59055,#59056));
#25400=EDGE_LOOP('',(#59057,#59058,#59059,#59060));
#25401=EDGE_LOOP('',(#59061,#59062,#59063,#59064));
#25402=EDGE_LOOP('',(#59065,#59066,#59067,#59068));
#25403=EDGE_LOOP('',(#59069,#59070,#59071,#59072));
#25404=EDGE_LOOP('',(#59073,#59074,#59075,#59076));
#25405=EDGE_LOOP('',(#59077,#59078,#59079,#59080));
#25406=EDGE_LOOP('',(#59081,#59082,#59083,#59084));
#25407=EDGE_LOOP('',(#59085,#59086,#59087,#59088));
#25408=EDGE_LOOP('',(#59089,#59090,#59091,#59092));
#25409=EDGE_LOOP('',(#59093,#59094,#59095,#59096));
#25410=EDGE_LOOP('',(#59097,#59098,#59099,#59100));
#25411=EDGE_LOOP('',(#59101,#59102,#59103,#59104));
#25412=EDGE_LOOP('',(#59105,#59106,#59107,#59108));
#25413=EDGE_LOOP('',(#59109,#59110,#59111,#59112));
#25414=EDGE_LOOP('',(#59113,#59114,#59115,#59116));
#25415=EDGE_LOOP('',(#59117,#59118,#59119,#59120));
#25416=EDGE_LOOP('',(#59121,#59122,#59123,#59124));
#25417=EDGE_LOOP('',(#59125,#59126,#59127,#59128));
#25418=EDGE_LOOP('',(#59129,#59130,#59131,#59132));
#25419=EDGE_LOOP('',(#59133,#59134,#59135,#59136));
#25420=EDGE_LOOP('',(#59137,#59138,#59139,#59140));
#25421=EDGE_LOOP('',(#59141,#59142,#59143,#59144));
#25422=EDGE_LOOP('',(#59145,#59146,#59147,#59148));
#25423=EDGE_LOOP('',(#59149,#59150,#59151,#59152));
#25424=EDGE_LOOP('',(#59153,#59154,#59155,#59156));
#25425=EDGE_LOOP('',(#59157,#59158,#59159,#59160));
#25426=EDGE_LOOP('',(#59161,#59162,#59163,#59164));
#25427=EDGE_LOOP('',(#59165,#59166,#59167,#59168));
#25428=EDGE_LOOP('',(#59169,#59170,#59171,#59172));
#25429=EDGE_LOOP('',(#59173,#59174,#59175,#59176));
#25430=EDGE_LOOP('',(#59177,#59178,#59179,#59180));
#25431=EDGE_LOOP('',(#59181,#59182,#59183,#59184));
#25432=EDGE_LOOP('',(#59185,#59186,#59187,#59188));
#25433=EDGE_LOOP('',(#59189,#59190,#59191,#59192));
#25434=EDGE_LOOP('',(#59193,#59194,#59195,#59196));
#25435=EDGE_LOOP('',(#59197,#59198,#59199,#59200));
#25436=EDGE_LOOP('',(#59201,#59202,#59203,#59204));
#25437=EDGE_LOOP('',(#59205,#59206,#59207,#59208));
#25438=EDGE_LOOP('',(#59209,#59210,#59211,#59212));
#25439=EDGE_LOOP('',(#59213,#59214,#59215,#59216));
#25440=EDGE_LOOP('',(#59217,#59218,#59219,#59220));
#25441=EDGE_LOOP('',(#59221,#59222,#59223,#59224));
#25442=EDGE_LOOP('',(#59225,#59226,#59227,#59228));
#25443=EDGE_LOOP('',(#59229,#59230,#59231,#59232));
#25444=EDGE_LOOP('',(#59233,#59234,#59235,#59236));
#25445=EDGE_LOOP('',(#59237,#59238,#59239,#59240));
#25446=EDGE_LOOP('',(#59241,#59242,#59243,#59244));
#25447=EDGE_LOOP('',(#59245,#59246,#59247,#59248));
#25448=EDGE_LOOP('',(#59249,#59250,#59251,#59252));
#25449=EDGE_LOOP('',(#59253,#59254,#59255,#59256));
#25450=EDGE_LOOP('',(#59257,#59258,#59259,#59260));
#25451=EDGE_LOOP('',(#59261,#59262,#59263,#59264));
#25452=EDGE_LOOP('',(#59265,#59266,#59267,#59268));
#25453=EDGE_LOOP('',(#59269,#59270,#59271,#59272));
#25454=EDGE_LOOP('',(#59273,#59274,#59275,#59276));
#25455=EDGE_LOOP('',(#59277,#59278,#59279,#59280));
#25456=EDGE_LOOP('',(#59281,#59282,#59283,#59284));
#25457=EDGE_LOOP('',(#59285,#59286,#59287,#59288));
#25458=EDGE_LOOP('',(#59289,#59290,#59291,#59292));
#25459=EDGE_LOOP('',(#59293,#59294,#59295,#59296));
#25460=EDGE_LOOP('',(#59297,#59298,#59299,#59300));
#25461=EDGE_LOOP('',(#59301,#59302,#59303,#59304));
#25462=EDGE_LOOP('',(#59305,#59306,#59307,#59308));
#25463=EDGE_LOOP('',(#59309,#59310,#59311,#59312));
#25464=EDGE_LOOP('',(#59313,#59314,#59315,#59316));
#25465=EDGE_LOOP('',(#59317,#59318,#59319,#59320));
#25466=EDGE_LOOP('',(#59321,#59322,#59323,#59324));
#25467=EDGE_LOOP('',(#59325,#59326,#59327,#59328));
#25468=EDGE_LOOP('',(#59329,#59330,#59331,#59332));
#25469=EDGE_LOOP('',(#59333,#59334,#59335,#59336));
#25470=EDGE_LOOP('',(#59337,#59338,#59339,#59340));
#25471=EDGE_LOOP('',(#59341,#59342,#59343,#59344));
#25472=EDGE_LOOP('',(#59345,#59346,#59347,#59348));
#25473=EDGE_LOOP('',(#59349,#59350,#59351,#59352));
#25474=EDGE_LOOP('',(#59353,#59354,#59355,#59356));
#25475=EDGE_LOOP('',(#59357,#59358,#59359,#59360));
#25476=EDGE_LOOP('',(#59361,#59362,#59363,#59364));
#25477=EDGE_LOOP('',(#59365,#59366,#59367,#59368));
#25478=EDGE_LOOP('',(#59369,#59370,#59371,#59372));
#25479=EDGE_LOOP('',(#59373,#59374,#59375,#59376));
#25480=EDGE_LOOP('',(#59377,#59378,#59379,#59380));
#25481=EDGE_LOOP('',(#59381,#59382,#59383,#59384));
#25482=EDGE_LOOP('',(#59385,#59386,#59387,#59388));
#25483=EDGE_LOOP('',(#59389,#59390,#59391,#59392));
#25484=EDGE_LOOP('',(#59393,#59394,#59395,#59396));
#25485=EDGE_LOOP('',(#59397,#59398,#59399,#59400));
#25486=EDGE_LOOP('',(#59401,#59402,#59403,#59404));
#25487=EDGE_LOOP('',(#59405,#59406,#59407,#59408));
#25488=EDGE_LOOP('',(#59409,#59410,#59411,#59412));
#25489=EDGE_LOOP('',(#59413,#59414,#59415,#59416));
#25490=EDGE_LOOP('',(#59417,#59418,#59419,#59420));
#25491=EDGE_LOOP('',(#59421,#59422,#59423,#59424));
#25492=EDGE_LOOP('',(#59425,#59426,#59427,#59428));
#25493=EDGE_LOOP('',(#59429,#59430,#59431,#59432));
#25494=EDGE_LOOP('',(#59433,#59434,#59435,#59436));
#25495=EDGE_LOOP('',(#59437,#59438,#59439,#59440));
#25496=EDGE_LOOP('',(#59441,#59442,#59443,#59444));
#25497=EDGE_LOOP('',(#59445,#59446,#59447,#59448));
#25498=EDGE_LOOP('',(#59449,#59450,#59451,#59452));
#25499=EDGE_LOOP('',(#59453,#59454,#59455,#59456));
#25500=EDGE_LOOP('',(#59457,#59458,#59459,#59460));
#25501=EDGE_LOOP('',(#59461,#59462,#59463,#59464));
#25502=EDGE_LOOP('',(#59465,#59466,#59467,#59468));
#25503=EDGE_LOOP('',(#59469,#59470,#59471,#59472));
#25504=EDGE_LOOP('',(#59473,#59474,#59475,#59476));
#25505=EDGE_LOOP('',(#59477,#59478,#59479,#59480));
#25506=EDGE_LOOP('',(#59481,#59482,#59483,#59484));
#25507=EDGE_LOOP('',(#59485,#59486,#59487,#59488));
#25508=EDGE_LOOP('',(#59489,#59490,#59491,#59492));
#25509=EDGE_LOOP('',(#59493,#59494,#59495,#59496));
#25510=EDGE_LOOP('',(#59497,#59498,#59499,#59500));
#25511=EDGE_LOOP('',(#59501,#59502,#59503,#59504));
#25512=EDGE_LOOP('',(#59505,#59506,#59507,#59508));
#25513=EDGE_LOOP('',(#59509,#59510,#59511,#59512));
#25514=EDGE_LOOP('',(#59513,#59514,#59515,#59516));
#25515=EDGE_LOOP('',(#59517,#59518,#59519,#59520));
#25516=EDGE_LOOP('',(#59521,#59522,#59523,#59524));
#25517=EDGE_LOOP('',(#59525,#59526,#59527,#59528));
#25518=EDGE_LOOP('',(#59529,#59530,#59531,#59532));
#25519=EDGE_LOOP('',(#59533,#59534,#59535,#59536));
#25520=EDGE_LOOP('',(#59537,#59538,#59539,#59540));
#25521=EDGE_LOOP('',(#59541,#59542,#59543,#59544));
#25522=EDGE_LOOP('',(#59545,#59546,#59547,#59548));
#25523=EDGE_LOOP('',(#59549,#59550,#59551,#59552));
#25524=EDGE_LOOP('',(#59553,#59554,#59555,#59556,#59557));
#25525=EDGE_LOOP('',(#59558,#59559,#59560,#59561));
#25526=EDGE_LOOP('',(#59562,#59563,#59564,#59565));
#25527=EDGE_LOOP('',(#59566,#59567,#59568,#59569));
#25528=EDGE_LOOP('',(#59570,#59571,#59572,#59573));
#25529=EDGE_LOOP('',(#59574,#59575,#59576,#59577,#59578));
#25530=EDGE_LOOP('',(#59579,#59580,#59581,#59582));
#25531=EDGE_LOOP('',(#59583,#59584,#59585,#59586,#59587));
#25532=EDGE_LOOP('',(#59588,#59589,#59590,#59591));
#25533=EDGE_LOOP('',(#59592,#59593,#59594,#59595));
#25534=EDGE_LOOP('',(#59596,#59597,#59598,#59599,#59600));
#25535=EDGE_LOOP('',(#59601,#59602,#59603,#59604));
#25536=EDGE_LOOP('',(#59605,#59606,#59607,#59608,#59609));
#25537=EDGE_LOOP('',(#59610,#59611,#59612,#59613));
#25538=EDGE_LOOP('',(#59614,#59615,#59616,#59617));
#25539=EDGE_LOOP('',(#59618,#59619,#59620,#59621,#59622));
#25540=EDGE_LOOP('',(#59623,#59624,#59625,#59626));
#25541=EDGE_LOOP('',(#59627,#59628,#59629,#59630,#59631));
#25542=EDGE_LOOP('',(#59632,#59633,#59634,#59635));
#25543=EDGE_LOOP('',(#59636,#59637,#59638,#59639));
#25544=EDGE_LOOP('',(#59640,#59641,#59642,#59643,#59644));
#25545=EDGE_LOOP('',(#59645,#59646,#59647,#59648));
#25546=EDGE_LOOP('',(#59649,#59650,#59651,#59652,#59653));
#25547=EDGE_LOOP('',(#59654,#59655,#59656,#59657));
#25548=EDGE_LOOP('',(#59658,#59659,#59660,#59661,#59662));
#25549=EDGE_LOOP('',(#59663,#59664,#59665,#59666));
#25550=EDGE_LOOP('',(#59667,#59668,#59669,#59670));
#25551=EDGE_LOOP('',(#59671,#59672,#59673,#59674,#59675));
#25552=EDGE_LOOP('',(#59676,#59677,#59678,#59679,#59680));
#25553=EDGE_LOOP('',(#59681,#59682,#59683,#59684,#59685));
#25554=EDGE_LOOP('',(#59686,#59687,#59688,#59689));
#25555=EDGE_LOOP('',(#59690,#59691,#59692,#59693));
#25556=EDGE_LOOP('',(#59694,#59695,#59696,#59697,#59698));
#25557=EDGE_LOOP('',(#59699,#59700,#59701,#59702,#59703));
#25558=EDGE_LOOP('',(#59704,#59705,#59706,#59707));
#25559=EDGE_LOOP('',(#59708,#59709,#59710,#59711,#59712));
#25560=EDGE_LOOP('',(#59713,#59714,#59715,#59716));
#25561=EDGE_LOOP('',(#59717,#59718,#59719,#59720,#59721));
#25562=EDGE_LOOP('',(#59722,#59723,#59724,#59725));
#25563=EDGE_LOOP('',(#59726,#59727,#59728,#59729));
#25564=EDGE_LOOP('',(#59730,#59731,#59732,#59733,#59734));
#25565=EDGE_LOOP('',(#59735,#59736,#59737,#59738));
#25566=EDGE_LOOP('',(#59739,#59740,#59741,#59742,#59743));
#25567=EDGE_LOOP('',(#59744,#59745,#59746,#59747));
#25568=EDGE_LOOP('',(#59748,#59749,#59750,#59751));
#25569=EDGE_LOOP('',(#59752,#59753,#59754,#59755,#59756));
#25570=EDGE_LOOP('',(#59757,#59758,#59759,#59760));
#25571=EDGE_LOOP('',(#59761,#59762,#59763,#59764,#59765));
#25572=EDGE_LOOP('',(#59766,#59767,#59768,#59769));
#25573=EDGE_LOOP('',(#59770,#59771,#59772,#59773));
#25574=EDGE_LOOP('',(#59774,#59775,#59776,#59777));
#25575=EDGE_LOOP('',(#59778,#59779,#59780,#59781));
#25576=EDGE_LOOP('',(#59782,#59783,#59784,#59785));
#25577=EDGE_LOOP('',(#59786,#59787,#59788,#59789));
#25578=EDGE_LOOP('',(#59790,#59791,#59792,#59793));
#25579=EDGE_LOOP('',(#59794,#59795,#59796,#59797));
#25580=EDGE_LOOP('',(#59798,#59799,#59800,#59801));
#25581=EDGE_LOOP('',(#59802,#59803,#59804,#59805));
#25582=EDGE_LOOP('',(#59806,#59807,#59808,#59809));
#25583=EDGE_LOOP('',(#59810,#59811,#59812,#59813));
#25584=EDGE_LOOP('',(#59814,#59815,#59816,#59817));
#25585=EDGE_LOOP('',(#59818,#59819,#59820,#59821));
#25586=EDGE_LOOP('',(#59822,#59823,#59824,#59825));
#25587=EDGE_LOOP('',(#59826,#59827,#59828,#59829));
#25588=EDGE_LOOP('',(#59830,#59831,#59832,#59833));
#25589=EDGE_LOOP('',(#59834,#59835,#59836,#59837));
#25590=EDGE_LOOP('',(#59838,#59839,#59840,#59841));
#25591=EDGE_LOOP('',(#59842,#59843,#59844,#59845));
#25592=EDGE_LOOP('',(#59846,#59847,#59848,#59849));
#25593=EDGE_LOOP('',(#59850,#59851,#59852,#59853));
#25594=EDGE_LOOP('',(#59854,#59855,#59856,#59857));
#25595=EDGE_LOOP('',(#59858,#59859,#59860,#59861));
#25596=EDGE_LOOP('',(#59862,#59863,#59864,#59865));
#25597=EDGE_LOOP('',(#59866,#59867,#59868,#59869));
#25598=EDGE_LOOP('',(#59870,#59871,#59872,#59873));
#25599=EDGE_LOOP('',(#59874,#59875,#59876,#59877));
#25600=EDGE_LOOP('',(#59878,#59879,#59880,#59881));
#25601=EDGE_LOOP('',(#59882,#59883,#59884,#59885));
#25602=EDGE_LOOP('',(#59886,#59887,#59888,#59889));
#25603=EDGE_LOOP('',(#59890,#59891,#59892,#59893));
#25604=EDGE_LOOP('',(#59894,#59895,#59896,#59897));
#25605=EDGE_LOOP('',(#59898,#59899,#59900,#59901,#59902));
#25606=EDGE_LOOP('',(#59903,#59904,#59905,#59906));
#25607=EDGE_LOOP('',(#59907,#59908,#59909,#59910));
#25608=EDGE_LOOP('',(#59911,#59912,#59913,#59914,#59915));
#25609=EDGE_LOOP('',(#59916,#59917,#59918,#59919,#59920));
#25610=EDGE_LOOP('',(#59921,#59922,#59923,#59924,#59925));
#25611=EDGE_LOOP('',(#59926,#59927,#59928,#59929));
#25612=EDGE_LOOP('',(#59930,#59931,#59932,#59933));
#25613=EDGE_LOOP('',(#59934,#59935,#59936,#59937,#59938));
#25614=EDGE_LOOP('',(#59939,#59940,#59941,#59942,#59943));
#25615=EDGE_LOOP('',(#59944,#59945,#59946,#59947));
#25616=EDGE_LOOP('',(#59948,#59949,#59950,#59951));
#25617=EDGE_LOOP('',(#59952,#59953,#59954,#59955));
#25618=EDGE_LOOP('',(#59956,#59957,#59958,#59959));
#25619=EDGE_LOOP('',(#59960,#59961,#59962,#59963));
#25620=EDGE_LOOP('',(#59964,#59965,#59966,#59967));
#25621=EDGE_LOOP('',(#59968,#59969,#59970,#59971));
#25622=EDGE_LOOP('',(#59972,#59973,#59974,#59975));
#25623=EDGE_LOOP('',(#59976,#59977,#59978,#59979));
#25624=EDGE_LOOP('',(#59980,#59981,#59982,#59983));
#25625=EDGE_LOOP('',(#59984,#59985,#59986,#59987));
#25626=EDGE_LOOP('',(#59988,#59989,#59990,#59991));
#25627=EDGE_LOOP('',(#59992,#59993,#59994,#59995));
#25628=EDGE_LOOP('',(#59996,#59997,#59998,#59999));
#25629=EDGE_LOOP('',(#60000,#60001,#60002,#60003));
#25630=EDGE_LOOP('',(#60004,#60005,#60006,#60007));
#25631=EDGE_LOOP('',(#60008,#60009,#60010,#60011));
#25632=EDGE_LOOP('',(#60012,#60013,#60014,#60015));
#25633=EDGE_LOOP('',(#60016,#60017,#60018,#60019,#60020));
#25634=EDGE_LOOP('',(#60021,#60022,#60023,#60024,#60025));
#25635=EDGE_LOOP('',(#60026,#60027,#60028));
#25636=EDGE_LOOP('',(#60029,#60030,#60031,#60032));
#25637=EDGE_LOOP('',(#60033,#60034,#60035,#60036,#60037));
#25638=EDGE_LOOP('',(#60038,#60039,#60040,#60041));
#25639=EDGE_LOOP('',(#60042,#60043,#60044,#60045,#60046));
#25640=EDGE_LOOP('',(#60047,#60048,#60049,#60050));
#25641=EDGE_LOOP('',(#60051,#60052,#60053,#60054));
#25642=EDGE_LOOP('',(#60055,#60056,#60057,#60058,#60059));
#25643=EDGE_LOOP('',(#60060,#60061,#60062,#60063));
#25644=EDGE_LOOP('',(#60064,#60065,#60066,#60067,#60068));
#25645=EDGE_LOOP('',(#60069,#60070,#60071,#60072));
#25646=EDGE_LOOP('',(#60073,#60074,#60075,#60076));
#25647=EDGE_LOOP('',(#60077,#60078,#60079,#60080));
#25648=EDGE_LOOP('',(#60081,#60082,#60083,#60084,#60085));
#25649=EDGE_LOOP('',(#60086,#60087,#60088,#60089,#60090));
#25650=EDGE_LOOP('',(#60091,#60092,#60093));
#25651=EDGE_LOOP('',(#60094,#60095,#60096,#60097));
#25652=EDGE_LOOP('',(#60098,#60099,#60100,#60101));
#25653=EDGE_LOOP('',(#60102,#60103,#60104,#60105));
#25654=EDGE_LOOP('',(#60106,#60107,#60108,#60109));
#25655=EDGE_LOOP('',(#60110,#60111,#60112,#60113));
#25656=EDGE_LOOP('',(#60114,#60115,#60116,#60117));
#25657=EDGE_LOOP('',(#60118,#60119,#60120,#60121));
#25658=EDGE_LOOP('',(#60122,#60123,#60124,#60125));
#25659=EDGE_LOOP('',(#60126,#60127,#60128,#60129));
#25660=EDGE_LOOP('',(#60130,#60131,#60132,#60133));
#25661=EDGE_LOOP('',(#60134,#60135,#60136,#60137));
#25662=EDGE_LOOP('',(#60138,#60139,#60140,#60141));
#25663=EDGE_LOOP('',(#60142,#60143,#60144,#60145));
#25664=EDGE_LOOP('',(#60146,#60147,#60148,#60149));
#25665=EDGE_LOOP('',(#60150,#60151,#60152,#60153));
#25666=EDGE_LOOP('',(#60154,#60155,#60156,#60157));
#25667=EDGE_LOOP('',(#60158,#60159,#60160,#60161));
#25668=EDGE_LOOP('',(#60162,#60163,#60164,#60165));
#25669=EDGE_LOOP('',(#60166,#60167,#60168,#60169));
#25670=EDGE_LOOP('',(#60170,#60171,#60172,#60173));
#25671=EDGE_LOOP('',(#60174,#60175,#60176,#60177));
#25672=EDGE_LOOP('',(#60178,#60179,#60180,#60181));
#25673=EDGE_LOOP('',(#60182,#60183,#60184,#60185));
#25674=EDGE_LOOP('',(#60186,#60187,#60188,#60189));
#25675=EDGE_LOOP('',(#60190,#60191,#60192,#60193));
#25676=EDGE_LOOP('',(#60194,#60195,#60196,#60197));
#25677=EDGE_LOOP('',(#60198,#60199,#60200,#60201));
#25678=EDGE_LOOP('',(#60202,#60203,#60204,#60205));
#25679=EDGE_LOOP('',(#60206,#60207,#60208,#60209));
#25680=EDGE_LOOP('',(#60210,#60211,#60212,#60213));
#25681=EDGE_LOOP('',(#60214,#60215,#60216,#60217));
#25682=EDGE_LOOP('',(#60218,#60219,#60220,#60221));
#25683=EDGE_LOOP('',(#60222,#60223,#60224,#60225));
#25684=EDGE_LOOP('',(#60226,#60227,#60228,#60229));
#25685=EDGE_LOOP('',(#60230,#60231,#60232,#60233));
#25686=EDGE_LOOP('',(#60234,#60235,#60236,#60237));
#25687=EDGE_LOOP('',(#60238,#60239,#60240,#60241));
#25688=EDGE_LOOP('',(#60242,#60243,#60244,#60245));
#25689=EDGE_LOOP('',(#60246,#60247,#60248,#60249));
#25690=EDGE_LOOP('',(#60250,#60251,#60252,#60253));
#25691=EDGE_LOOP('',(#60254,#60255,#60256,#60257));
#25692=EDGE_LOOP('',(#60258,#60259,#60260,#60261));
#25693=EDGE_LOOP('',(#60262,#60263,#60264,#60265,#60266));
#25694=EDGE_LOOP('',(#60267,#60268,#60269,#60270,#60271));
#25695=EDGE_LOOP('',(#60272,#60273,#60274));
#25696=EDGE_LOOP('',(#60275,#60276,#60277,#60278));
#25697=EDGE_LOOP('',(#60279,#60280,#60281,#60282));
#25698=EDGE_LOOP('',(#60283,#60284,#60285,#60286,#60287));
#25699=EDGE_LOOP('',(#60288,#60289,#60290,#60291,#60292));
#25700=EDGE_LOOP('',(#60293,#60294,#60295));
#25701=EDGE_LOOP('',(#60296,#60297,#60298,#60299));
#25702=EDGE_LOOP('',(#60300,#60301,#60302,#60303));
#25703=EDGE_LOOP('',(#60304,#60305,#60306,#60307));
#25704=EDGE_LOOP('',(#60308,#60309,#60310,#60311));
#25705=EDGE_LOOP('',(#60312,#60313,#60314,#60315));
#25706=EDGE_LOOP('',(#60316,#60317,#60318,#60319));
#25707=EDGE_LOOP('',(#60320,#60321,#60322,#60323));
#25708=EDGE_LOOP('',(#60324,#60325,#60326,#60327));
#25709=EDGE_LOOP('',(#60328,#60329,#60330,#60331));
#25710=EDGE_LOOP('',(#60332,#60333,#60334,#60335));
#25711=EDGE_LOOP('',(#60336,#60337,#60338,#60339));
#25712=EDGE_LOOP('',(#60340,#60341,#60342,#60343));
#25713=EDGE_LOOP('',(#60344,#60345,#60346,#60347));
#25714=EDGE_LOOP('',(#60348,#60349,#60350,#60351));
#25715=EDGE_LOOP('',(#60352,#60353,#60354,#60355));
#25716=EDGE_LOOP('',(#60356,#60357,#60358,#60359));
#25717=EDGE_LOOP('',(#60360,#60361,#60362,#60363));
#25718=EDGE_LOOP('',(#60364,#60365,#60366,#60367));
#25719=EDGE_LOOP('',(#60368,#60369,#60370,#60371));
#25720=EDGE_LOOP('',(#60372,#60373,#60374,#60375));
#25721=EDGE_LOOP('',(#60376,#60377,#60378,#60379));
#25722=EDGE_LOOP('',(#60380,#60381,#60382,#60383));
#25723=EDGE_LOOP('',(#60384,#60385,#60386,#60387));
#25724=EDGE_LOOP('',(#60388,#60389,#60390,#60391));
#25725=EDGE_LOOP('',(#60392,#60393,#60394,#60395));
#25726=EDGE_LOOP('',(#60396,#60397,#60398,#60399));
#25727=EDGE_LOOP('',(#60400,#60401,#60402,#60403));
#25728=EDGE_LOOP('',(#60404,#60405,#60406,#60407));
#25729=EDGE_LOOP('',(#60408,#60409,#60410,#60411));
#25730=EDGE_LOOP('',(#60412,#60413,#60414,#60415));
#25731=EDGE_LOOP('',(#60416,#60417,#60418,#60419));
#25732=EDGE_LOOP('',(#60420,#60421,#60422,#60423));
#25733=EDGE_LOOP('',(#60424,#60425,#60426,#60427));
#25734=EDGE_LOOP('',(#60428,#60429,#60430,#60431));
#25735=EDGE_LOOP('',(#60432,#60433,#60434,#60435));
#25736=EDGE_LOOP('',(#60436,#60437,#60438,#60439));
#25737=EDGE_LOOP('',(#60440,#60441,#60442,#60443));
#25738=EDGE_LOOP('',(#60444,#60445,#60446,#60447,#60448));
#25739=EDGE_LOOP('',(#60449,#60450,#60451,#60452));
#25740=EDGE_LOOP('',(#60453,#60454,#60455,#60456,#60457));
#25741=EDGE_LOOP('',(#60458,#60459,#60460,#60461));
#25742=EDGE_LOOP('',(#60462,#60463,#60464,#60465));
#25743=EDGE_LOOP('',(#60466,#60467,#60468,#60469));
#25744=EDGE_LOOP('',(#60470,#60471,#60472,#60473,#60474));
#25745=EDGE_LOOP('',(#60475,#60476,#60477,#60478,#60479));
#25746=EDGE_LOOP('',(#60480,#60481,#60482));
#25747=EDGE_LOOP('',(#60483,#60484,#60485,#60486));
#25748=EDGE_LOOP('',(#60487,#60488,#60489,#60490));
#25749=EDGE_LOOP('',(#60491,#60492,#60493,#60494));
#25750=EDGE_LOOP('',(#60495,#60496,#60497,#60498));
#25751=EDGE_LOOP('',(#60499,#60500,#60501,#60502));
#25752=EDGE_LOOP('',(#60503,#60504,#60505,#60506));
#25753=EDGE_LOOP('',(#60507,#60508,#60509,#60510));
#25754=EDGE_LOOP('',(#60511,#60512,#60513,#60514));
#25755=EDGE_LOOP('',(#60515,#60516,#60517,#60518));
#25756=EDGE_LOOP('',(#60519,#60520,#60521,#60522));
#25757=EDGE_LOOP('',(#60523,#60524,#60525,#60526));
#25758=EDGE_LOOP('',(#60527,#60528,#60529,#60530));
#25759=EDGE_LOOP('',(#60531,#60532,#60533,#60534));
#25760=EDGE_LOOP('',(#60535,#60536,#60537,#60538));
#25761=EDGE_LOOP('',(#60539,#60540,#60541,#60542));
#25762=EDGE_LOOP('',(#60543,#60544,#60545,#60546));
#25763=EDGE_LOOP('',(#60547,#60548,#60549,#60550));
#25764=EDGE_LOOP('',(#60551,#60552,#60553,#60554));
#25765=EDGE_LOOP('',(#60555,#60556,#60557,#60558));
#25766=EDGE_LOOP('',(#60559,#60560,#60561,#60562));
#25767=EDGE_LOOP('',(#60563,#60564,#60565,#60566));
#25768=EDGE_LOOP('',(#60567,#60568,#60569,#60570));
#25769=EDGE_LOOP('',(#60571,#60572,#60573,#60574));
#25770=EDGE_LOOP('',(#60575,#60576,#60577,#60578));
#25771=EDGE_LOOP('',(#60579,#60580,#60581,#60582));
#25772=EDGE_LOOP('',(#60583,#60584,#60585,#60586));
#25773=EDGE_LOOP('',(#60587,#60588,#60589,#60590));
#25774=EDGE_LOOP('',(#60591,#60592,#60593,#60594));
#25775=EDGE_LOOP('',(#60595,#60596,#60597,#60598));
#25776=EDGE_LOOP('',(#60599,#60600,#60601,#60602));
#25777=EDGE_LOOP('',(#60603,#60604,#60605,#60606));
#25778=EDGE_LOOP('',(#60607,#60608,#60609,#60610));
#25779=EDGE_LOOP('',(#60611,#60612,#60613,#60614));
#25780=EDGE_LOOP('',(#60615,#60616,#60617,#60618));
#25781=EDGE_LOOP('',(#60619,#60620,#60621,#60622));
#25782=EDGE_LOOP('',(#60623,#60624,#60625,#60626));
#25783=EDGE_LOOP('',(#60627,#60628,#60629,#60630));
#25784=EDGE_LOOP('',(#60631,#60632,#60633,#60634));
#25785=EDGE_LOOP('',(#60635,#60636,#60637,#60638));
#25786=EDGE_LOOP('',(#60639,#60640,#60641,#60642));
#25787=EDGE_LOOP('',(#60643,#60644,#60645,#60646));
#25788=EDGE_LOOP('',(#60647,#60648,#60649,#60650));
#25789=EDGE_LOOP('',(#60651,#60652,#60653,#60654));
#25790=EDGE_LOOP('',(#60655,#60656,#60657,#60658));
#25791=EDGE_LOOP('',(#60659,#60660,#60661,#60662));
#25792=EDGE_LOOP('',(#60663,#60664,#60665,#60666));
#25793=EDGE_LOOP('',(#60667,#60668,#60669,#60670));
#25794=EDGE_LOOP('',(#60671,#60672,#60673,#60674));
#25795=EDGE_LOOP('',(#60675,#60676,#60677,#60678));
#25796=EDGE_LOOP('',(#60679,#60680,#60681,#60682));
#25797=EDGE_LOOP('',(#60683,#60684,#60685,#60686));
#25798=EDGE_LOOP('',(#60687,#60688,#60689,#60690));
#25799=EDGE_LOOP('',(#60691,#60692,#60693,#60694));
#25800=EDGE_LOOP('',(#60695,#60696,#60697,#60698));
#25801=EDGE_LOOP('',(#60699,#60700,#60701,#60702));
#25802=EDGE_LOOP('',(#60703,#60704,#60705,#60706));
#25803=EDGE_LOOP('',(#60707,#60708,#60709,#60710));
#25804=EDGE_LOOP('',(#60711,#60712,#60713,#60714));
#25805=EDGE_LOOP('',(#60715,#60716,#60717,#60718));
#25806=EDGE_LOOP('',(#60719,#60720,#60721,#60722));
#25807=EDGE_LOOP('',(#60723,#60724,#60725,#60726));
#25808=EDGE_LOOP('',(#60727,#60728,#60729,#60730));
#25809=EDGE_LOOP('',(#60731,#60732,#60733,#60734));
#25810=EDGE_LOOP('',(#60735,#60736,#60737,#60738));
#25811=EDGE_LOOP('',(#60739,#60740,#60741,#60742));
#25812=EDGE_LOOP('',(#60743,#60744,#60745,#60746));
#25813=EDGE_LOOP('',(#60747,#60748,#60749,#60750));
#25814=EDGE_LOOP('',(#60751,#60752,#60753,#60754));
#25815=EDGE_LOOP('',(#60755,#60756,#60757,#60758));
#25816=EDGE_LOOP('',(#60759,#60760,#60761,#60762));
#25817=EDGE_LOOP('',(#60763,#60764,#60765,#60766));
#25818=EDGE_LOOP('',(#60767,#60768,#60769,#60770));
#25819=EDGE_LOOP('',(#60771,#60772,#60773,#60774));
#25820=EDGE_LOOP('',(#60775,#60776,#60777,#60778));
#25821=EDGE_LOOP('',(#60779,#60780,#60781,#60782));
#25822=EDGE_LOOP('',(#60783,#60784,#60785,#60786));
#25823=EDGE_LOOP('',(#60787,#60788,#60789,#60790));
#25824=EDGE_LOOP('',(#60791,#60792,#60793,#60794));
#25825=EDGE_LOOP('',(#60795,#60796,#60797,#60798));
#25826=EDGE_LOOP('',(#60799,#60800,#60801,#60802));
#25827=EDGE_LOOP('',(#60803,#60804,#60805,#60806));
#25828=EDGE_LOOP('',(#60807,#60808,#60809,#60810));
#25829=EDGE_LOOP('',(#60811,#60812,#60813,#60814));
#25830=EDGE_LOOP('',(#60815,#60816,#60817,#60818));
#25831=EDGE_LOOP('',(#60819,#60820,#60821,#60822));
#25832=EDGE_LOOP('',(#60823,#60824,#60825,#60826));
#25833=EDGE_LOOP('',(#60827,#60828,#60829,#60830));
#25834=EDGE_LOOP('',(#60831,#60832,#60833,#60834));
#25835=EDGE_LOOP('',(#60835,#60836,#60837,#60838));
#25836=EDGE_LOOP('',(#60839,#60840,#60841,#60842));
#25837=EDGE_LOOP('',(#60843,#60844,#60845,#60846));
#25838=EDGE_LOOP('',(#60847,#60848,#60849,#60850));
#25839=EDGE_LOOP('',(#60851,#60852,#60853,#60854));
#25840=EDGE_LOOP('',(#60855,#60856,#60857,#60858));
#25841=EDGE_LOOP('',(#60859,#60860,#60861,#60862));
#25842=EDGE_LOOP('',(#60863,#60864,#60865,#60866));
#25843=EDGE_LOOP('',(#60867,#60868,#60869,#60870));
#25844=EDGE_LOOP('',(#60871,#60872,#60873,#60874));
#25845=EDGE_LOOP('',(#60875,#60876,#60877,#60878));
#25846=EDGE_LOOP('',(#60879,#60880,#60881,#60882));
#25847=EDGE_LOOP('',(#60883,#60884,#60885,#60886));
#25848=EDGE_LOOP('',(#60887,#60888,#60889,#60890));
#25849=EDGE_LOOP('',(#60891,#60892,#60893,#60894));
#25850=EDGE_LOOP('',(#60895,#60896,#60897,#60898));
#25851=EDGE_LOOP('',(#60899,#60900,#60901,#60902));
#25852=EDGE_LOOP('',(#60903,#60904,#60905,#60906));
#25853=EDGE_LOOP('',(#60907,#60908,#60909,#60910));
#25854=EDGE_LOOP('',(#60911,#60912,#60913,#60914));
#25855=EDGE_LOOP('',(#60915,#60916,#60917,#60918));
#25856=EDGE_LOOP('',(#60919,#60920,#60921,#60922));
#25857=EDGE_LOOP('',(#60923,#60924,#60925,#60926));
#25858=EDGE_LOOP('',(#60927,#60928,#60929,#60930));
#25859=EDGE_LOOP('',(#60931,#60932,#60933,#60934));
#25860=EDGE_LOOP('',(#60935,#60936,#60937,#60938));
#25861=EDGE_LOOP('',(#60939,#60940,#60941,#60942));
#25862=EDGE_LOOP('',(#60943,#60944,#60945,#60946));
#25863=EDGE_LOOP('',(#60947,#60948,#60949,#60950));
#25864=EDGE_LOOP('',(#60951,#60952,#60953,#60954));
#25865=EDGE_LOOP('',(#60955,#60956,#60957,#60958));
#25866=EDGE_LOOP('',(#60959,#60960,#60961,#60962));
#25867=EDGE_LOOP('',(#60963,#60964,#60965,#60966));
#25868=EDGE_LOOP('',(#60967,#60968,#60969,#60970));
#25869=EDGE_LOOP('',(#60971,#60972,#60973,#60974));
#25870=EDGE_LOOP('',(#60975,#60976,#60977,#60978));
#25871=EDGE_LOOP('',(#60979,#60980,#60981,#60982));
#25872=EDGE_LOOP('',(#60983,#60984,#60985,#60986));
#25873=EDGE_LOOP('',(#60987,#60988,#60989,#60990));
#25874=EDGE_LOOP('',(#60991,#60992,#60993,#60994));
#25875=EDGE_LOOP('',(#60995,#60996,#60997,#60998));
#25876=EDGE_LOOP('',(#60999,#61000,#61001,#61002));
#25877=EDGE_LOOP('',(#61003,#61004,#61005,#61006));
#25878=EDGE_LOOP('',(#61007,#61008,#61009,#61010));
#25879=EDGE_LOOP('',(#61011,#61012,#61013,#61014));
#25880=EDGE_LOOP('',(#61015,#61016,#61017,#61018));
#25881=EDGE_LOOP('',(#61019,#61020,#61021,#61022));
#25882=EDGE_LOOP('',(#61023,#61024,#61025,#61026));
#25883=EDGE_LOOP('',(#61027,#61028,#61029,#61030));
#25884=EDGE_LOOP('',(#61031,#61032,#61033,#61034));
#25885=EDGE_LOOP('',(#61035,#61036,#61037,#61038));
#25886=EDGE_LOOP('',(#61039,#61040,#61041,#61042));
#25887=EDGE_LOOP('',(#61043,#61044,#61045,#61046));
#25888=EDGE_LOOP('',(#61047,#61048,#61049,#61050));
#25889=EDGE_LOOP('',(#61051,#61052,#61053,#61054));
#25890=EDGE_LOOP('',(#61055,#61056,#61057,#61058));
#25891=EDGE_LOOP('',(#61059,#61060,#61061,#61062));
#25892=EDGE_LOOP('',(#61063,#61064,#61065,#61066));
#25893=EDGE_LOOP('',(#61067,#61068,#61069,#61070));
#25894=EDGE_LOOP('',(#61071,#61072,#61073,#61074));
#25895=EDGE_LOOP('',(#61075,#61076,#61077,#61078));
#25896=EDGE_LOOP('',(#61079,#61080,#61081,#61082));
#25897=EDGE_LOOP('',(#61083,#61084,#61085,#61086));
#25898=EDGE_LOOP('',(#61087,#61088,#61089,#61090));
#25899=EDGE_LOOP('',(#61091,#61092,#61093,#61094));
#25900=EDGE_LOOP('',(#61095,#61096,#61097,#61098));
#25901=EDGE_LOOP('',(#61099,#61100,#61101,#61102));
#25902=EDGE_LOOP('',(#61103,#61104,#61105,#61106));
#25903=EDGE_LOOP('',(#61107,#61108,#61109,#61110));
#25904=EDGE_LOOP('',(#61111,#61112,#61113,#61114));
#25905=EDGE_LOOP('',(#61115,#61116,#61117,#61118));
#25906=EDGE_LOOP('',(#61119,#61120,#61121,#61122));
#25907=EDGE_LOOP('',(#61123,#61124,#61125,#61126));
#25908=EDGE_LOOP('',(#61127,#61128,#61129,#61130));
#25909=EDGE_LOOP('',(#61131,#61132,#61133,#61134));
#25910=EDGE_LOOP('',(#61135,#61136,#61137,#61138));
#25911=EDGE_LOOP('',(#61139,#61140,#61141,#61142));
#25912=EDGE_LOOP('',(#61143,#61144,#61145,#61146));
#25913=EDGE_LOOP('',(#61147,#61148,#61149,#61150));
#25914=EDGE_LOOP('',(#61151,#61152,#61153,#61154));
#25915=EDGE_LOOP('',(#61155,#61156,#61157,#61158));
#25916=EDGE_LOOP('',(#61159,#61160,#61161,#61162));
#25917=EDGE_LOOP('',(#61163,#61164,#61165,#61166));
#25918=EDGE_LOOP('',(#61167,#61168,#61169,#61170));
#25919=EDGE_LOOP('',(#61171,#61172,#61173,#61174));
#25920=EDGE_LOOP('',(#61175,#61176,#61177,#61178));
#25921=EDGE_LOOP('',(#61179,#61180,#61181,#61182));
#25922=EDGE_LOOP('',(#61183,#61184,#61185,#61186));
#25923=EDGE_LOOP('',(#61187,#61188,#61189,#61190));
#25924=EDGE_LOOP('',(#61191,#61192,#61193,#61194));
#25925=EDGE_LOOP('',(#61195,#61196,#61197,#61198));
#25926=EDGE_LOOP('',(#61199,#61200,#61201,#61202));
#25927=EDGE_LOOP('',(#61203,#61204,#61205,#61206));
#25928=EDGE_LOOP('',(#61207,#61208,#61209,#61210));
#25929=EDGE_LOOP('',(#61211,#61212,#61213,#61214));
#25930=EDGE_LOOP('',(#61215,#61216,#61217,#61218));
#25931=EDGE_LOOP('',(#61219,#61220,#61221,#61222));
#25932=EDGE_LOOP('',(#61223,#61224,#61225,#61226));
#25933=EDGE_LOOP('',(#61227,#61228,#61229,#61230));
#25934=EDGE_LOOP('',(#61231,#61232,#61233,#61234));
#25935=EDGE_LOOP('',(#61235,#61236,#61237,#61238));
#25936=EDGE_LOOP('',(#61239,#61240,#61241,#61242));
#25937=EDGE_LOOP('',(#61243,#61244,#61245,#61246));
#25938=EDGE_LOOP('',(#61247,#61248,#61249,#61250));
#25939=EDGE_LOOP('',(#61251,#61252,#61253,#61254));
#25940=EDGE_LOOP('',(#61255,#61256,#61257,#61258));
#25941=EDGE_LOOP('',(#61259,#61260,#61261,#61262));
#25942=EDGE_LOOP('',(#61263,#61264,#61265,#61266));
#25943=EDGE_LOOP('',(#61267,#61268,#61269,#61270));
#25944=EDGE_LOOP('',(#61271,#61272,#61273,#61274));
#25945=EDGE_LOOP('',(#61275,#61276,#61277,#61278));
#25946=EDGE_LOOP('',(#61279,#61280,#61281,#61282));
#25947=EDGE_LOOP('',(#61283,#61284,#61285,#61286));
#25948=EDGE_LOOP('',(#61287,#61288,#61289,#61290));
#25949=EDGE_LOOP('',(#61291,#61292,#61293,#61294));
#25950=EDGE_LOOP('',(#61295,#61296,#61297,#61298));
#25951=EDGE_LOOP('',(#61299,#61300,#61301,#61302));
#25952=EDGE_LOOP('',(#61303,#61304,#61305,#61306));
#25953=EDGE_LOOP('',(#61307,#61308,#61309,#61310));
#25954=EDGE_LOOP('',(#61311,#61312,#61313,#61314));
#25955=EDGE_LOOP('',(#61315,#61316,#61317,#61318));
#25956=EDGE_LOOP('',(#61319,#61320,#61321,#61322));
#25957=EDGE_LOOP('',(#61323,#61324,#61325,#61326));
#25958=EDGE_LOOP('',(#61327,#61328,#61329,#61330));
#25959=EDGE_LOOP('',(#61331,#61332,#61333,#61334));
#25960=EDGE_LOOP('',(#61335,#61336,#61337,#61338));
#25961=EDGE_LOOP('',(#61339,#61340,#61341,#61342));
#25962=EDGE_LOOP('',(#61343,#61344,#61345,#61346));
#25963=EDGE_LOOP('',(#61347,#61348,#61349,#61350));
#25964=EDGE_LOOP('',(#61351,#61352,#61353,#61354));
#25965=EDGE_LOOP('',(#61355,#61356,#61357,#61358));
#25966=EDGE_LOOP('',(#61359,#61360,#61361,#61362));
#25967=EDGE_LOOP('',(#61363,#61364,#61365,#61366));
#25968=EDGE_LOOP('',(#61367,#61368,#61369,#61370));
#25969=EDGE_LOOP('',(#61371,#61372,#61373,#61374));
#25970=EDGE_LOOP('',(#61375,#61376,#61377,#61378));
#25971=EDGE_LOOP('',(#61379,#61380,#61381,#61382));
#25972=EDGE_LOOP('',(#61383,#61384,#61385,#61386));
#25973=EDGE_LOOP('',(#61387,#61388,#61389,#61390));
#25974=EDGE_LOOP('',(#61391,#61392,#61393,#61394));
#25975=EDGE_LOOP('',(#61395,#61396,#61397,#61398));
#25976=EDGE_LOOP('',(#61399,#61400,#61401,#61402));
#25977=EDGE_LOOP('',(#61403,#61404,#61405,#61406));
#25978=EDGE_LOOP('',(#61407,#61408,#61409,#61410));
#25979=EDGE_LOOP('',(#61411,#61412,#61413,#61414));
#25980=EDGE_LOOP('',(#61415,#61416,#61417,#61418));
#25981=EDGE_LOOP('',(#61419,#61420,#61421,#61422));
#25982=EDGE_LOOP('',(#61423,#61424,#61425,#61426));
#25983=EDGE_LOOP('',(#61427,#61428,#61429,#61430));
#25984=EDGE_LOOP('',(#61431,#61432,#61433,#61434));
#25985=EDGE_LOOP('',(#61435,#61436,#61437,#61438));
#25986=EDGE_LOOP('',(#61439,#61440,#61441,#61442));
#25987=EDGE_LOOP('',(#61443,#61444,#61445,#61446));
#25988=EDGE_LOOP('',(#61447,#61448,#61449,#61450));
#25989=EDGE_LOOP('',(#61451,#61452,#61453,#61454));
#25990=EDGE_LOOP('',(#61455,#61456,#61457,#61458));
#25991=EDGE_LOOP('',(#61459,#61460,#61461,#61462));
#25992=EDGE_LOOP('',(#61463,#61464,#61465,#61466));
#25993=EDGE_LOOP('',(#61467,#61468,#61469,#61470));
#25994=EDGE_LOOP('',(#61471,#61472,#61473,#61474));
#25995=EDGE_LOOP('',(#61475,#61476,#61477,#61478));
#25996=EDGE_LOOP('',(#61479,#61480,#61481,#61482));
#25997=EDGE_LOOP('',(#61483,#61484,#61485,#61486));
#25998=EDGE_LOOP('',(#61487,#61488,#61489,#61490));
#25999=EDGE_LOOP('',(#61491,#61492,#61493,#61494));
#26000=EDGE_LOOP('',(#61495,#61496,#61497,#61498));
#26001=EDGE_LOOP('',(#61499,#61500,#61501,#61502));
#26002=EDGE_LOOP('',(#61503,#61504,#61505,#61506));
#26003=EDGE_LOOP('',(#61507,#61508,#61509,#61510));
#26004=EDGE_LOOP('',(#61511,#61512,#61513,#61514));
#26005=EDGE_LOOP('',(#61515,#61516,#61517,#61518));
#26006=EDGE_LOOP('',(#61519,#61520,#61521,#61522));
#26007=EDGE_LOOP('',(#61523,#61524,#61525,#61526));
#26008=EDGE_LOOP('',(#61527,#61528,#61529,#61530));
#26009=EDGE_LOOP('',(#61531,#61532,#61533,#61534));
#26010=EDGE_LOOP('',(#61535,#61536,#61537,#61538));
#26011=EDGE_LOOP('',(#61539,#61540,#61541,#61542));
#26012=EDGE_LOOP('',(#61543,#61544,#61545,#61546));
#26013=EDGE_LOOP('',(#61547,#61548,#61549,#61550));
#26014=EDGE_LOOP('',(#61551,#61552,#61553,#61554));
#26015=EDGE_LOOP('',(#61555,#61556,#61557,#61558));
#26016=EDGE_LOOP('',(#61559,#61560,#61561,#61562));
#26017=EDGE_LOOP('',(#61563,#61564,#61565,#61566));
#26018=EDGE_LOOP('',(#61567,#61568,#61569,#61570));
#26019=EDGE_LOOP('',(#61571,#61572,#61573,#61574));
#26020=EDGE_LOOP('',(#61575,#61576,#61577,#61578));
#26021=EDGE_LOOP('',(#61579,#61580,#61581,#61582));
#26022=EDGE_LOOP('',(#61583,#61584,#61585,#61586));
#26023=EDGE_LOOP('',(#61587,#61588,#61589,#61590));
#26024=EDGE_LOOP('',(#61591,#61592,#61593,#61594));
#26025=EDGE_LOOP('',(#61595,#61596,#61597,#61598));
#26026=EDGE_LOOP('',(#61599,#61600,#61601,#61602));
#26027=EDGE_LOOP('',(#61603,#61604,#61605,#61606));
#26028=EDGE_LOOP('',(#61607,#61608,#61609,#61610));
#26029=EDGE_LOOP('',(#61611,#61612,#61613,#61614));
#26030=EDGE_LOOP('',(#61615,#61616,#61617,#61618));
#26031=EDGE_LOOP('',(#61619,#61620,#61621,#61622));
#26032=EDGE_LOOP('',(#61623,#61624,#61625,#61626));
#26033=EDGE_LOOP('',(#61627,#61628,#61629,#61630));
#26034=EDGE_LOOP('',(#61631,#61632,#61633,#61634));
#26035=EDGE_LOOP('',(#61635,#61636,#61637,#61638));
#26036=EDGE_LOOP('',(#61639,#61640,#61641,#61642));
#26037=EDGE_LOOP('',(#61643,#61644,#61645,#61646));
#26038=EDGE_LOOP('',(#61647,#61648,#61649,#61650));
#26039=EDGE_LOOP('',(#61651,#61652,#61653,#61654));
#26040=EDGE_LOOP('',(#61655,#61656,#61657,#61658));
#26041=EDGE_LOOP('',(#61659,#61660,#61661,#61662));
#26042=EDGE_LOOP('',(#61663,#61664,#61665,#61666));
#26043=EDGE_LOOP('',(#61667,#61668,#61669,#61670));
#26044=EDGE_LOOP('',(#61671,#61672,#61673,#61674));
#26045=EDGE_LOOP('',(#61675,#61676,#61677,#61678));
#26046=EDGE_LOOP('',(#61679,#61680,#61681,#61682));
#26047=EDGE_LOOP('',(#61683,#61684,#61685,#61686));
#26048=EDGE_LOOP('',(#61687,#61688,#61689,#61690));
#26049=EDGE_LOOP('',(#61691,#61692,#61693,#61694));
#26050=EDGE_LOOP('',(#61695,#61696,#61697,#61698));
#26051=EDGE_LOOP('',(#61699,#61700,#61701,#61702));
#26052=EDGE_LOOP('',(#61703,#61704,#61705,#61706));
#26053=EDGE_LOOP('',(#61707,#61708,#61709,#61710));
#26054=EDGE_LOOP('',(#61711,#61712,#61713,#61714));
#26055=EDGE_LOOP('',(#61715));
#26056=EDGE_LOOP('',(#61716));
#26057=EDGE_LOOP('',(#61717,#61718,#61719,#61720));
#26058=EDGE_LOOP('',(#61721,#61722,#61723,#61724));
#26059=EDGE_LOOP('',(#61725,#61726,#61727,#61728));
#26060=EDGE_LOOP('',(#61729,#61730,#61731,#61732));
#26061=EDGE_LOOP('',(#61733,#61734,#61735,#61736));
#26062=EDGE_LOOP('',(#61737,#61738,#61739,#61740));
#26063=EDGE_LOOP('',(#61741,#61742,#61743,#61744));
#26064=EDGE_LOOP('',(#61745,#61746,#61747,#61748));
#26065=EDGE_LOOP('',(#61749,#61750,#61751,#61752));
#26066=EDGE_LOOP('',(#61753,#61754,#61755,#61756));
#26067=EDGE_LOOP('',(#61757,#61758,#61759,#61760));
#26068=EDGE_LOOP('',(#61761,#61762,#61763,#61764));
#26069=EDGE_LOOP('',(#61765,#61766,#61767,#61768));
#26070=EDGE_LOOP('',(#61769,#61770,#61771,#61772));
#26071=EDGE_LOOP('',(#61773,#61774,#61775,#61776));
#26072=EDGE_LOOP('',(#61777,#61778,#61779,#61780));
#26073=EDGE_LOOP('',(#61781,#61782,#61783,#61784));
#26074=EDGE_LOOP('',(#61785,#61786,#61787,#61788));
#26075=EDGE_LOOP('',(#61789,#61790,#61791,#61792));
#26076=EDGE_LOOP('',(#61793,#61794,#61795,#61796));
#26077=EDGE_LOOP('',(#61797,#61798,#61799,#61800));
#26078=EDGE_LOOP('',(#61801,#61802,#61803,#61804));
#26079=EDGE_LOOP('',(#61805,#61806,#61807,#61808));
#26080=EDGE_LOOP('',(#61809,#61810,#61811,#61812));
#26081=EDGE_LOOP('',(#61813,#61814,#61815,#61816));
#26082=EDGE_LOOP('',(#61817,#61818,#61819,#61820));
#26083=EDGE_LOOP('',(#61821,#61822,#61823,#61824));
#26084=EDGE_LOOP('',(#61825,#61826,#61827,#61828));
#26085=EDGE_LOOP('',(#61829,#61830,#61831,#61832));
#26086=EDGE_LOOP('',(#61833,#61834,#61835,#61836));
#26087=EDGE_LOOP('',(#61837,#61838,#61839,#61840));
#26088=EDGE_LOOP('',(#61841,#61842,#61843,#61844));
#26089=EDGE_LOOP('',(#61845,#61846,#61847,#61848));
#26090=EDGE_LOOP('',(#61849,#61850,#61851,#61852));
#26091=EDGE_LOOP('',(#61853,#61854,#61855,#61856));
#26092=EDGE_LOOP('',(#61857,#61858,#61859,#61860));
#26093=EDGE_LOOP('',(#61861,#61862,#61863,#61864));
#26094=EDGE_LOOP('',(#61865,#61866,#61867,#61868));
#26095=EDGE_LOOP('',(#61869,#61870,#61871,#61872));
#26096=EDGE_LOOP('',(#61873,#61874,#61875,#61876));
#26097=EDGE_LOOP('',(#61877,#61878,#61879,#61880));
#26098=EDGE_LOOP('',(#61881,#61882,#61883,#61884));
#26099=EDGE_LOOP('',(#61885,#61886,#61887,#61888));
#26100=EDGE_LOOP('',(#61889,#61890,#61891,#61892));
#26101=EDGE_LOOP('',(#61893,#61894,#61895,#61896));
#26102=EDGE_LOOP('',(#61897,#61898,#61899,#61900));
#26103=EDGE_LOOP('',(#61901,#61902,#61903,#61904));
#26104=EDGE_LOOP('',(#61905,#61906,#61907,#61908));
#26105=EDGE_LOOP('',(#61909,#61910,#61911,#61912));
#26106=EDGE_LOOP('',(#61913,#61914,#61915,#61916));
#26107=EDGE_LOOP('',(#61917,#61918,#61919,#61920));
#26108=EDGE_LOOP('',(#61921,#61922,#61923,#61924));
#26109=EDGE_LOOP('',(#61925,#61926,#61927,#61928));
#26110=EDGE_LOOP('',(#61929,#61930,#61931,#61932));
#26111=EDGE_LOOP('',(#61933,#61934,#61935,#61936));
#26112=EDGE_LOOP('',(#61937,#61938,#61939,#61940));
#26113=EDGE_LOOP('',(#61941,#61942,#61943,#61944));
#26114=EDGE_LOOP('',(#61945,#61946,#61947,#61948));
#26115=EDGE_LOOP('',(#61949,#61950,#61951,#61952));
#26116=EDGE_LOOP('',(#61953,#61954,#61955,#61956));
#26117=EDGE_LOOP('',(#61957,#61958,#61959,#61960));
#26118=EDGE_LOOP('',(#61961,#61962,#61963,#61964));
#26119=EDGE_LOOP('',(#61965,#61966,#61967,#61968));
#26120=EDGE_LOOP('',(#61969,#61970,#61971,#61972));
#26121=EDGE_LOOP('',(#61973,#61974,#61975,#61976));
#26122=EDGE_LOOP('',(#61977,#61978,#61979,#61980));
#26123=EDGE_LOOP('',(#61981,#61982,#61983,#61984));
#26124=EDGE_LOOP('',(#61985,#61986,#61987,#61988));
#26125=EDGE_LOOP('',(#61989,#61990,#61991,#61992));
#26126=EDGE_LOOP('',(#61993,#61994,#61995,#61996));
#26127=EDGE_LOOP('',(#61997,#61998,#61999,#62000));
#26128=EDGE_LOOP('',(#62001,#62002,#62003,#62004));
#26129=EDGE_LOOP('',(#62005,#62006,#62007,#62008));
#26130=EDGE_LOOP('',(#62009,#62010,#62011,#62012));
#26131=EDGE_LOOP('',(#62013,#62014,#62015,#62016));
#26132=EDGE_LOOP('',(#62017,#62018,#62019,#62020));
#26133=EDGE_LOOP('',(#62021,#62022,#62023,#62024));
#26134=EDGE_LOOP('',(#62025,#62026,#62027,#62028));
#26135=EDGE_LOOP('',(#62029,#62030,#62031,#62032));
#26136=EDGE_LOOP('',(#62033,#62034,#62035,#62036));
#26137=EDGE_LOOP('',(#62037,#62038,#62039,#62040));
#26138=EDGE_LOOP('',(#62041,#62042,#62043,#62044));
#26139=EDGE_LOOP('',(#62045,#62046,#62047,#62048));
#26140=EDGE_LOOP('',(#62049,#62050,#62051,#62052));
#26141=EDGE_LOOP('',(#62053,#62054,#62055,#62056));
#26142=EDGE_LOOP('',(#62057,#62058,#62059,#62060));
#26143=EDGE_LOOP('',(#62061,#62062,#62063,#62064));
#26144=EDGE_LOOP('',(#62065,#62066,#62067,#62068));
#26145=EDGE_LOOP('',(#62069,#62070,#62071,#62072));
#26146=EDGE_LOOP('',(#62073,#62074,#62075,#62076));
#26147=EDGE_LOOP('',(#62077,#62078,#62079,#62080));
#26148=EDGE_LOOP('',(#62081,#62082,#62083,#62084));
#26149=EDGE_LOOP('',(#62085,#62086,#62087,#62088));
#26150=EDGE_LOOP('',(#62089,#62090,#62091,#62092));
#26151=EDGE_LOOP('',(#62093,#62094,#62095,#62096));
#26152=EDGE_LOOP('',(#62097,#62098,#62099,#62100));
#26153=EDGE_LOOP('',(#62101,#62102,#62103,#62104));
#26154=EDGE_LOOP('',(#62105,#62106,#62107,#62108));
#26155=EDGE_LOOP('',(#62109,#62110,#62111,#62112));
#26156=EDGE_LOOP('',(#62113,#62114,#62115,#62116));
#26157=EDGE_LOOP('',(#62117,#62118,#62119,#62120));
#26158=EDGE_LOOP('',(#62121,#62122,#62123,#62124));
#26159=EDGE_LOOP('',(#62125,#62126,#62127,#62128));
#26160=EDGE_LOOP('',(#62129,#62130,#62131,#62132));
#26161=EDGE_LOOP('',(#62133,#62134,#62135,#62136));
#26162=EDGE_LOOP('',(#62137,#62138,#62139,#62140));
#26163=EDGE_LOOP('',(#62141,#62142,#62143,#62144));
#26164=EDGE_LOOP('',(#62145,#62146,#62147,#62148));
#26165=EDGE_LOOP('',(#62149,#62150,#62151,#62152));
#26166=EDGE_LOOP('',(#62153,#62154,#62155,#62156));
#26167=EDGE_LOOP('',(#62157,#62158,#62159,#62160));
#26168=EDGE_LOOP('',(#62161,#62162,#62163,#62164));
#26169=EDGE_LOOP('',(#62165,#62166,#62167,#62168));
#26170=EDGE_LOOP('',(#62169,#62170,#62171,#62172));
#26171=EDGE_LOOP('',(#62173,#62174,#62175,#62176));
#26172=EDGE_LOOP('',(#62177,#62178,#62179,#62180));
#26173=EDGE_LOOP('',(#62181,#62182,#62183,#62184));
#26174=EDGE_LOOP('',(#62185,#62186,#62187,#62188));
#26175=EDGE_LOOP('',(#62189,#62190,#62191,#62192));
#26176=EDGE_LOOP('',(#62193,#62194,#62195,#62196));
#26177=EDGE_LOOP('',(#62197,#62198,#62199,#62200));
#26178=EDGE_LOOP('',(#62201,#62202,#62203,#62204));
#26179=EDGE_LOOP('',(#62205,#62206,#62207,#62208));
#26180=EDGE_LOOP('',(#62209,#62210,#62211,#62212));
#26181=EDGE_LOOP('',(#62213,#62214,#62215,#62216));
#26182=EDGE_LOOP('',(#62217,#62218,#62219,#62220));
#26183=EDGE_LOOP('',(#62221,#62222,#62223,#62224));
#26184=EDGE_LOOP('',(#62225,#62226,#62227,#62228));
#26185=EDGE_LOOP('',(#62229,#62230,#62231,#62232));
#26186=EDGE_LOOP('',(#62233,#62234,#62235,#62236));
#26187=EDGE_LOOP('',(#62237,#62238,#62239,#62240));
#26188=EDGE_LOOP('',(#62241,#62242,#62243,#62244));
#26189=EDGE_LOOP('',(#62245,#62246,#62247,#62248));
#26190=EDGE_LOOP('',(#62249,#62250,#62251,#62252));
#26191=EDGE_LOOP('',(#62253,#62254,#62255,#62256));
#26192=EDGE_LOOP('',(#62257,#62258,#62259,#62260));
#26193=EDGE_LOOP('',(#62261,#62262,#62263,#62264));
#26194=EDGE_LOOP('',(#62265,#62266,#62267,#62268));
#26195=EDGE_LOOP('',(#62269,#62270,#62271,#62272));
#26196=EDGE_LOOP('',(#62273,#62274,#62275,#62276));
#26197=EDGE_LOOP('',(#62277,#62278,#62279,#62280));
#26198=EDGE_LOOP('',(#62281,#62282,#62283,#62284));
#26199=EDGE_LOOP('',(#62285,#62286,#62287,#62288));
#26200=EDGE_LOOP('',(#62289,#62290,#62291,#62292));
#26201=EDGE_LOOP('',(#62293,#62294,#62295,#62296));
#26202=EDGE_LOOP('',(#62297,#62298,#62299,#62300));
#26203=EDGE_LOOP('',(#62301,#62302,#62303,#62304));
#26204=EDGE_LOOP('',(#62305,#62306,#62307,#62308));
#26205=EDGE_LOOP('',(#62309,#62310,#62311,#62312));
#26206=EDGE_LOOP('',(#62313,#62314,#62315,#62316));
#26207=EDGE_LOOP('',(#62317,#62318,#62319,#62320));
#26208=EDGE_LOOP('',(#62321,#62322,#62323,#62324));
#26209=EDGE_LOOP('',(#62325,#62326,#62327,#62328));
#26210=EDGE_LOOP('',(#62329,#62330,#62331,#62332));
#26211=EDGE_LOOP('',(#62333,#62334,#62335,#62336));
#26212=EDGE_LOOP('',(#62337,#62338,#62339,#62340));
#26213=EDGE_LOOP('',(#62341,#62342,#62343,#62344));
#26214=EDGE_LOOP('',(#62345,#62346,#62347,#62348));
#26215=EDGE_LOOP('',(#62349,#62350,#62351,#62352));
#26216=EDGE_LOOP('',(#62353,#62354,#62355,#62356));
#26217=EDGE_LOOP('',(#62357,#62358,#62359,#62360));
#26218=EDGE_LOOP('',(#62361,#62362,#62363,#62364));
#26219=EDGE_LOOP('',(#62365,#62366,#62367,#62368));
#26220=EDGE_LOOP('',(#62369,#62370,#62371,#62372));
#26221=EDGE_LOOP('',(#62373,#62374,#62375,#62376));
#26222=EDGE_LOOP('',(#62377,#62378,#62379,#62380));
#26223=EDGE_LOOP('',(#62381,#62382,#62383,#62384));
#26224=EDGE_LOOP('',(#62385,#62386,#62387,#62388));
#26225=EDGE_LOOP('',(#62389,#62390,#62391,#62392));
#26226=EDGE_LOOP('',(#62393,#62394,#62395,#62396));
#26227=EDGE_LOOP('',(#62397,#62398,#62399,#62400));
#26228=EDGE_LOOP('',(#62401,#62402,#62403,#62404));
#26229=EDGE_LOOP('',(#62405,#62406,#62407,#62408));
#26230=EDGE_LOOP('',(#62409,#62410,#62411,#62412));
#26231=EDGE_LOOP('',(#62413,#62414,#62415,#62416));
#26232=EDGE_LOOP('',(#62417,#62418,#62419,#62420));
#26233=EDGE_LOOP('',(#62421,#62422,#62423,#62424));
#26234=EDGE_LOOP('',(#62425,#62426,#62427,#62428));
#26235=EDGE_LOOP('',(#62429,#62430,#62431,#62432));
#26236=EDGE_LOOP('',(#62433,#62434,#62435,#62436));
#26237=EDGE_LOOP('',(#62437,#62438,#62439,#62440));
#26238=EDGE_LOOP('',(#62441,#62442,#62443,#62444));
#26239=EDGE_LOOP('',(#62445,#62446,#62447,#62448));
#26240=EDGE_LOOP('',(#62449,#62450,#62451,#62452));
#26241=EDGE_LOOP('',(#62453,#62454,#62455,#62456));
#26242=EDGE_LOOP('',(#62457,#62458,#62459,#62460));
#26243=EDGE_LOOP('',(#62461,#62462,#62463,#62464));
#26244=EDGE_LOOP('',(#62465,#62466,#62467,#62468));
#26245=EDGE_LOOP('',(#62469,#62470,#62471,#62472));
#26246=EDGE_LOOP('',(#62473,#62474,#62475,#62476));
#26247=EDGE_LOOP('',(#62477,#62478,#62479,#62480));
#26248=EDGE_LOOP('',(#62481,#62482,#62483,#62484));
#26249=EDGE_LOOP('',(#62485,#62486,#62487,#62488));
#26250=EDGE_LOOP('',(#62489,#62490,#62491,#62492));
#26251=EDGE_LOOP('',(#62493,#62494,#62495,#62496));
#26252=EDGE_LOOP('',(#62497,#62498,#62499,#62500));
#26253=EDGE_LOOP('',(#62501,#62502,#62503,#62504));
#26254=EDGE_LOOP('',(#62505,#62506,#62507,#62508));
#26255=EDGE_LOOP('',(#62509,#62510,#62511,#62512));
#26256=EDGE_LOOP('',(#62513,#62514,#62515,#62516));
#26257=EDGE_LOOP('',(#62517,#62518,#62519,#62520));
#26258=EDGE_LOOP('',(#62521,#62522,#62523,#62524));
#26259=EDGE_LOOP('',(#62525,#62526,#62527,#62528));
#26260=EDGE_LOOP('',(#62529,#62530,#62531,#62532));
#26261=EDGE_LOOP('',(#62533,#62534,#62535,#62536));
#26262=EDGE_LOOP('',(#62537,#62538,#62539,#62540));
#26263=EDGE_LOOP('',(#62541,#62542,#62543,#62544));
#26264=EDGE_LOOP('',(#62545,#62546,#62547,#62548));
#26265=EDGE_LOOP('',(#62549,#62550,#62551,#62552));
#26266=EDGE_LOOP('',(#62553,#62554,#62555,#62556));
#26267=EDGE_LOOP('',(#62557,#62558,#62559,#62560));
#26268=EDGE_LOOP('',(#62561,#62562,#62563,#62564));
#26269=EDGE_LOOP('',(#62565,#62566,#62567,#62568));
#26270=EDGE_LOOP('',(#62569,#62570,#62571,#62572));
#26271=EDGE_LOOP('',(#62573,#62574,#62575,#62576));
#26272=EDGE_LOOP('',(#62577,#62578,#62579,#62580));
#26273=EDGE_LOOP('',(#62581,#62582,#62583,#62584));
#26274=EDGE_LOOP('',(#62585,#62586,#62587,#62588));
#26275=EDGE_LOOP('',(#62589,#62590,#62591,#62592));
#26276=EDGE_LOOP('',(#62593,#62594,#62595,#62596));
#26277=EDGE_LOOP('',(#62597,#62598,#62599,#62600));
#26278=EDGE_LOOP('',(#62601,#62602,#62603,#62604));
#26279=EDGE_LOOP('',(#62605,#62606,#62607,#62608));
#26280=EDGE_LOOP('',(#62609,#62610,#62611,#62612));
#26281=EDGE_LOOP('',(#62613,#62614,#62615,#62616));
#26282=EDGE_LOOP('',(#62617,#62618,#62619,#62620));
#26283=EDGE_LOOP('',(#62621,#62622,#62623,#62624));
#26284=EDGE_LOOP('',(#62625,#62626,#62627,#62628));
#26285=EDGE_LOOP('',(#62629,#62630,#62631,#62632));
#26286=EDGE_LOOP('',(#62633,#62634,#62635,#62636));
#26287=EDGE_LOOP('',(#62637,#62638,#62639,#62640));
#26288=EDGE_LOOP('',(#62641,#62642,#62643,#62644));
#26289=EDGE_LOOP('',(#62645,#62646,#62647,#62648));
#26290=EDGE_LOOP('',(#62649,#62650,#62651,#62652));
#26291=EDGE_LOOP('',(#62653,#62654,#62655,#62656));
#26292=EDGE_LOOP('',(#62657,#62658,#62659,#62660));
#26293=EDGE_LOOP('',(#62661,#62662,#62663,#62664));
#26294=EDGE_LOOP('',(#62665,#62666,#62667,#62668));
#26295=EDGE_LOOP('',(#62669,#62670,#62671,#62672));
#26296=EDGE_LOOP('',(#62673,#62674,#62675,#62676));
#26297=EDGE_LOOP('',(#62677,#62678,#62679,#62680));
#26298=EDGE_LOOP('',(#62681,#62682,#62683,#62684));
#26299=EDGE_LOOP('',(#62685,#62686,#62687,#62688));
#26300=EDGE_LOOP('',(#62689,#62690,#62691,#62692));
#26301=EDGE_LOOP('',(#62693,#62694,#62695,#62696));
#26302=EDGE_LOOP('',(#62697,#62698,#62699,#62700));
#26303=EDGE_LOOP('',(#62701,#62702,#62703,#62704));
#26304=EDGE_LOOP('',(#62705,#62706,#62707,#62708));
#26305=EDGE_LOOP('',(#62709,#62710,#62711,#62712));
#26306=EDGE_LOOP('',(#62713,#62714,#62715,#62716));
#26307=EDGE_LOOP('',(#62717,#62718,#62719,#62720));
#26308=EDGE_LOOP('',(#62721,#62722,#62723,#62724));
#26309=EDGE_LOOP('',(#62725,#62726,#62727,#62728));
#26310=EDGE_LOOP('',(#62729,#62730,#62731,#62732));
#26311=EDGE_LOOP('',(#62733,#62734,#62735,#62736));
#26312=EDGE_LOOP('',(#62737,#62738,#62739,#62740));
#26313=EDGE_LOOP('',(#62741,#62742,#62743,#62744));
#26314=EDGE_LOOP('',(#62745,#62746,#62747,#62748));
#26315=EDGE_LOOP('',(#62749,#62750,#62751,#62752));
#26316=EDGE_LOOP('',(#62753,#62754,#62755,#62756));
#26317=EDGE_LOOP('',(#62757,#62758,#62759,#62760));
#26318=EDGE_LOOP('',(#62761,#62762,#62763,#62764));
#26319=EDGE_LOOP('',(#62765,#62766,#62767,#62768));
#26320=EDGE_LOOP('',(#62769,#62770,#62771,#62772));
#26321=EDGE_LOOP('',(#62773,#62774,#62775,#62776));
#26322=EDGE_LOOP('',(#62777,#62778,#62779,#62780));
#26323=EDGE_LOOP('',(#62781,#62782,#62783,#62784));
#26324=EDGE_LOOP('',(#62785,#62786,#62787,#62788));
#26325=EDGE_LOOP('',(#62789,#62790,#62791,#62792));
#26326=EDGE_LOOP('',(#62793,#62794,#62795,#62796));
#26327=EDGE_LOOP('',(#62797,#62798,#62799,#62800));
#26328=EDGE_LOOP('',(#62801,#62802,#62803,#62804));
#26329=EDGE_LOOP('',(#62805,#62806,#62807,#62808));
#26330=EDGE_LOOP('',(#62809,#62810,#62811,#62812));
#26331=EDGE_LOOP('',(#62813,#62814,#62815,#62816));
#26332=EDGE_LOOP('',(#62817,#62818,#62819,#62820));
#26333=EDGE_LOOP('',(#62821,#62822,#62823,#62824));
#26334=EDGE_LOOP('',(#62825,#62826,#62827,#62828));
#26335=EDGE_LOOP('',(#62829,#62830,#62831,#62832));
#26336=EDGE_LOOP('',(#62833,#62834,#62835,#62836));
#26337=EDGE_LOOP('',(#62837,#62838,#62839,#62840));
#26338=EDGE_LOOP('',(#62841,#62842,#62843,#62844));
#26339=EDGE_LOOP('',(#62845,#62846,#62847,#62848));
#26340=EDGE_LOOP('',(#62849,#62850,#62851,#62852));
#26341=EDGE_LOOP('',(#62853,#62854,#62855,#62856));
#26342=EDGE_LOOP('',(#62857,#62858,#62859,#62860));
#26343=EDGE_LOOP('',(#62861,#62862,#62863,#62864));
#26344=EDGE_LOOP('',(#62865,#62866,#62867,#62868));
#26345=EDGE_LOOP('',(#62869,#62870,#62871,#62872));
#26346=EDGE_LOOP('',(#62873,#62874,#62875,#62876));
#26347=EDGE_LOOP('',(#62877,#62878,#62879,#62880));
#26348=EDGE_LOOP('',(#62881,#62882,#62883,#62884));
#26349=EDGE_LOOP('',(#62885,#62886,#62887,#62888));
#26350=EDGE_LOOP('',(#62889,#62890,#62891,#62892));
#26351=EDGE_LOOP('',(#62893,#62894,#62895,#62896));
#26352=EDGE_LOOP('',(#62897,#62898,#62899,#62900));
#26353=EDGE_LOOP('',(#62901,#62902,#62903,#62904));
#26354=EDGE_LOOP('',(#62905,#62906,#62907,#62908));
#26355=EDGE_LOOP('',(#62909,#62910,#62911,#62912));
#26356=EDGE_LOOP('',(#62913,#62914,#62915,#62916));
#26357=EDGE_LOOP('',(#62917,#62918,#62919,#62920));
#26358=EDGE_LOOP('',(#62921,#62922,#62923,#62924));
#26359=EDGE_LOOP('',(#62925,#62926,#62927,#62928));
#26360=EDGE_LOOP('',(#62929,#62930,#62931,#62932));
#26361=EDGE_LOOP('',(#62933,#62934,#62935,#62936));
#26362=EDGE_LOOP('',(#62937,#62938,#62939,#62940));
#26363=EDGE_LOOP('',(#62941,#62942,#62943,#62944));
#26364=EDGE_LOOP('',(#62945,#62946,#62947,#62948));
#26365=EDGE_LOOP('',(#62949,#62950,#62951,#62952));
#26366=EDGE_LOOP('',(#62953,#62954,#62955,#62956));
#26367=EDGE_LOOP('',(#62957,#62958,#62959,#62960));
#26368=EDGE_LOOP('',(#62961,#62962,#62963,#62964));
#26369=EDGE_LOOP('',(#62965,#62966,#62967,#62968));
#26370=EDGE_LOOP('',(#62969,#62970,#62971,#62972));
#26371=EDGE_LOOP('',(#62973,#62974,#62975,#62976));
#26372=EDGE_LOOP('',(#62977,#62978,#62979,#62980));
#26373=EDGE_LOOP('',(#62981,#62982,#62983,#62984));
#26374=EDGE_LOOP('',(#62985,#62986,#62987,#62988));
#26375=EDGE_LOOP('',(#62989,#62990,#62991,#62992));
#26376=EDGE_LOOP('',(#62993,#62994,#62995,#62996));
#26377=EDGE_LOOP('',(#62997,#62998,#62999,#63000));
#26378=EDGE_LOOP('',(#63001,#63002,#63003,#63004));
#26379=EDGE_LOOP('',(#63005,#63006,#63007,#63008));
#26380=EDGE_LOOP('',(#63009,#63010,#63011,#63012));
#26381=EDGE_LOOP('',(#63013,#63014,#63015,#63016));
#26382=EDGE_LOOP('',(#63017,#63018,#63019,#63020));
#26383=EDGE_LOOP('',(#63021,#63022,#63023,#63024));
#26384=EDGE_LOOP('',(#63025,#63026,#63027,#63028));
#26385=EDGE_LOOP('',(#63029,#63030,#63031,#63032));
#26386=EDGE_LOOP('',(#63033,#63034,#63035,#63036));
#26387=EDGE_LOOP('',(#63037,#63038,#63039,#63040));
#26388=EDGE_LOOP('',(#63041,#63042,#63043,#63044));
#26389=EDGE_LOOP('',(#63045,#63046,#63047,#63048));
#26390=EDGE_LOOP('',(#63049,#63050,#63051,#63052));
#26391=EDGE_LOOP('',(#63053,#63054,#63055,#63056));
#26392=EDGE_LOOP('',(#63057,#63058,#63059,#63060));
#26393=EDGE_LOOP('',(#63061,#63062,#63063,#63064));
#26394=EDGE_LOOP('',(#63065,#63066,#63067,#63068));
#26395=EDGE_LOOP('',(#63069,#63070,#63071,#63072));
#26396=EDGE_LOOP('',(#63073,#63074,#63075,#63076));
#26397=EDGE_LOOP('',(#63077,#63078,#63079,#63080));
#26398=EDGE_LOOP('',(#63081,#63082,#63083,#63084));
#26399=EDGE_LOOP('',(#63085,#63086,#63087,#63088));
#26400=EDGE_LOOP('',(#63089,#63090,#63091,#63092));
#26401=EDGE_LOOP('',(#63093,#63094,#63095,#63096));
#26402=EDGE_LOOP('',(#63097,#63098,#63099,#63100));
#26403=EDGE_LOOP('',(#63101,#63102,#63103,#63104));
#26404=EDGE_LOOP('',(#63105,#63106,#63107,#63108));
#26405=EDGE_LOOP('',(#63109,#63110,#63111,#63112));
#26406=EDGE_LOOP('',(#63113,#63114,#63115,#63116));
#26407=EDGE_LOOP('',(#63117,#63118,#63119,#63120));
#26408=EDGE_LOOP('',(#63121,#63122,#63123,#63124));
#26409=EDGE_LOOP('',(#63125,#63126,#63127,#63128));
#26410=EDGE_LOOP('',(#63129,#63130,#63131,#63132));
#26411=EDGE_LOOP('',(#63133,#63134,#63135,#63136));
#26412=EDGE_LOOP('',(#63137,#63138,#63139,#63140));
#26413=EDGE_LOOP('',(#63141,#63142,#63143,#63144));
#26414=EDGE_LOOP('',(#63145,#63146,#63147,#63148));
#26415=EDGE_LOOP('',(#63149,#63150,#63151,#63152));
#26416=EDGE_LOOP('',(#63153,#63154,#63155,#63156));
#26417=EDGE_LOOP('',(#63157,#63158,#63159,#63160));
#26418=EDGE_LOOP('',(#63161,#63162,#63163,#63164));
#26419=EDGE_LOOP('',(#63165,#63166,#63167,#63168));
#26420=EDGE_LOOP('',(#63169,#63170,#63171,#63172));
#26421=EDGE_LOOP('',(#63173,#63174,#63175,#63176));
#26422=EDGE_LOOP('',(#63177,#63178,#63179,#63180));
#26423=EDGE_LOOP('',(#63181,#63182,#63183,#63184));
#26424=EDGE_LOOP('',(#63185,#63186,#63187,#63188));
#26425=EDGE_LOOP('',(#63189,#63190,#63191,#63192));
#26426=EDGE_LOOP('',(#63193,#63194,#63195,#63196));
#26427=EDGE_LOOP('',(#63197,#63198,#63199,#63200));
#26428=EDGE_LOOP('',(#63201,#63202,#63203,#63204));
#26429=EDGE_LOOP('',(#63205,#63206,#63207,#63208));
#26430=EDGE_LOOP('',(#63209,#63210,#63211,#63212));
#26431=EDGE_LOOP('',(#63213,#63214,#63215,#63216));
#26432=EDGE_LOOP('',(#63217,#63218,#63219,#63220));
#26433=EDGE_LOOP('',(#63221,#63222,#63223,#63224));
#26434=EDGE_LOOP('',(#63225,#63226,#63227,#63228));
#26435=EDGE_LOOP('',(#63229,#63230,#63231,#63232));
#26436=EDGE_LOOP('',(#63233,#63234,#63235,#63236));
#26437=EDGE_LOOP('',(#63237,#63238,#63239,#63240));
#26438=EDGE_LOOP('',(#63241,#63242,#63243,#63244));
#26439=EDGE_LOOP('',(#63245,#63246,#63247,#63248));
#26440=EDGE_LOOP('',(#63249,#63250,#63251,#63252));
#26441=EDGE_LOOP('',(#63253,#63254,#63255,#63256));
#26442=EDGE_LOOP('',(#63257,#63258,#63259,#63260));
#26443=EDGE_LOOP('',(#63261,#63262,#63263,#63264));
#26444=EDGE_LOOP('',(#63265,#63266,#63267,#63268));
#26445=EDGE_LOOP('',(#63269,#63270,#63271,#63272));
#26446=EDGE_LOOP('',(#63273,#63274,#63275,#63276));
#26447=EDGE_LOOP('',(#63277,#63278,#63279,#63280));
#26448=EDGE_LOOP('',(#63281,#63282,#63283,#63284));
#26449=EDGE_LOOP('',(#63285,#63286,#63287,#63288));
#26450=EDGE_LOOP('',(#63289,#63290,#63291,#63292));
#26451=EDGE_LOOP('',(#63293,#63294,#63295,#63296));
#26452=EDGE_LOOP('',(#63297,#63298,#63299,#63300));
#26453=EDGE_LOOP('',(#63301,#63302,#63303,#63304));
#26454=EDGE_LOOP('',(#63305,#63306,#63307,#63308));
#26455=EDGE_LOOP('',(#63309,#63310,#63311,#63312));
#26456=EDGE_LOOP('',(#63313,#63314,#63315,#63316));
#26457=EDGE_LOOP('',(#63317,#63318,#63319,#63320));
#26458=EDGE_LOOP('',(#63321,#63322,#63323,#63324));
#26459=EDGE_LOOP('',(#63325,#63326,#63327,#63328));
#26460=EDGE_LOOP('',(#63329,#63330,#63331,#63332));
#26461=EDGE_LOOP('',(#63333,#63334,#63335,#63336));
#26462=EDGE_LOOP('',(#63337,#63338,#63339,#63340));
#26463=EDGE_LOOP('',(#63341,#63342,#63343,#63344));
#26464=EDGE_LOOP('',(#63345,#63346,#63347,#63348));
#26465=EDGE_LOOP('',(#63349,#63350,#63351,#63352));
#26466=EDGE_LOOP('',(#63353,#63354,#63355,#63356));
#26467=EDGE_LOOP('',(#63357,#63358,#63359,#63360));
#26468=EDGE_LOOP('',(#63361,#63362,#63363,#63364));
#26469=EDGE_LOOP('',(#63365,#63366,#63367,#63368));
#26470=EDGE_LOOP('',(#63369,#63370,#63371,#63372));
#26471=EDGE_LOOP('',(#63373,#63374,#63375,#63376));
#26472=EDGE_LOOP('',(#63377,#63378,#63379,#63380));
#26473=EDGE_LOOP('',(#63381,#63382,#63383,#63384));
#26474=EDGE_LOOP('',(#63385,#63386,#63387,#63388));
#26475=EDGE_LOOP('',(#63389,#63390,#63391,#63392));
#26476=EDGE_LOOP('',(#63393,#63394,#63395,#63396));
#26477=EDGE_LOOP('',(#63397,#63398,#63399,#63400));
#26478=EDGE_LOOP('',(#63401,#63402,#63403,#63404));
#26479=EDGE_LOOP('',(#63405,#63406,#63407,#63408));
#26480=EDGE_LOOP('',(#63409,#63410,#63411,#63412));
#26481=EDGE_LOOP('',(#63413,#63414,#63415,#63416));
#26482=EDGE_LOOP('',(#63417,#63418,#63419,#63420));
#26483=EDGE_LOOP('',(#63421,#63422,#63423,#63424));
#26484=EDGE_LOOP('',(#63425,#63426,#63427,#63428));
#26485=EDGE_LOOP('',(#63429,#63430,#63431,#63432));
#26486=EDGE_LOOP('',(#63433,#63434,#63435,#63436));
#26487=EDGE_LOOP('',(#63437,#63438,#63439,#63440));
#26488=EDGE_LOOP('',(#63441,#63442,#63443,#63444));
#26489=EDGE_LOOP('',(#63445,#63446,#63447,#63448));
#26490=EDGE_LOOP('',(#63449,#63450,#63451,#63452));
#26491=EDGE_LOOP('',(#63453,#63454,#63455,#63456));
#26492=EDGE_LOOP('',(#63457,#63458,#63459,#63460));
#26493=EDGE_LOOP('',(#63461,#63462,#63463,#63464));
#26494=EDGE_LOOP('',(#63465,#63466,#63467,#63468));
#26495=EDGE_LOOP('',(#63469,#63470,#63471,#63472));
#26496=EDGE_LOOP('',(#63473,#63474,#63475,#63476));
#26497=EDGE_LOOP('',(#63477,#63478,#63479,#63480));
#26498=EDGE_LOOP('',(#63481,#63482,#63483,#63484));
#26499=EDGE_LOOP('',(#63485,#63486,#63487,#63488));
#26500=EDGE_LOOP('',(#63489,#63490,#63491,#63492));
#26501=EDGE_LOOP('',(#63493,#63494,#63495,#63496));
#26502=EDGE_LOOP('',(#63497,#63498,#63499,#63500));
#26503=EDGE_LOOP('',(#63501,#63502,#63503,#63504));
#26504=EDGE_LOOP('',(#63505,#63506,#63507,#63508));
#26505=EDGE_LOOP('',(#63509,#63510,#63511,#63512));
#26506=EDGE_LOOP('',(#63513,#63514,#63515,#63516));
#26507=EDGE_LOOP('',(#63517,#63518,#63519,#63520));
#26508=EDGE_LOOP('',(#63521,#63522,#63523,#63524));
#26509=EDGE_LOOP('',(#63525,#63526,#63527,#63528));
#26510=EDGE_LOOP('',(#63529,#63530,#63531,#63532));
#26511=EDGE_LOOP('',(#63533,#63534,#63535,#63536));
#26512=EDGE_LOOP('',(#63537,#63538,#63539,#63540));
#26513=EDGE_LOOP('',(#63541,#63542,#63543,#63544));
#26514=EDGE_LOOP('',(#63545,#63546,#63547,#63548));
#26515=EDGE_LOOP('',(#63549,#63550,#63551,#63552));
#26516=EDGE_LOOP('',(#63553,#63554,#63555,#63556));
#26517=EDGE_LOOP('',(#63557,#63558,#63559,#63560));
#26518=EDGE_LOOP('',(#63561,#63562,#63563,#63564));
#26519=EDGE_LOOP('',(#63565,#63566,#63567,#63568));
#26520=EDGE_LOOP('',(#63569,#63570,#63571,#63572));
#26521=EDGE_LOOP('',(#63573,#63574,#63575,#63576));
#26522=EDGE_LOOP('',(#63577,#63578,#63579,#63580));
#26523=EDGE_LOOP('',(#63581,#63582,#63583,#63584));
#26524=EDGE_LOOP('',(#63585,#63586,#63587,#63588));
#26525=EDGE_LOOP('',(#63589,#63590,#63591,#63592));
#26526=EDGE_LOOP('',(#63593,#63594,#63595,#63596));
#26527=EDGE_LOOP('',(#63597,#63598,#63599,#63600));
#26528=EDGE_LOOP('',(#63601,#63602,#63603,#63604));
#26529=EDGE_LOOP('',(#63605,#63606,#63607,#63608));
#26530=EDGE_LOOP('',(#63609,#63610,#63611,#63612));
#26531=EDGE_LOOP('',(#63613,#63614,#63615,#63616));
#26532=EDGE_LOOP('',(#63617,#63618,#63619,#63620));
#26533=EDGE_LOOP('',(#63621,#63622,#63623,#63624));
#26534=EDGE_LOOP('',(#63625,#63626,#63627,#63628));
#26535=EDGE_LOOP('',(#63629,#63630,#63631,#63632));
#26536=EDGE_LOOP('',(#63633,#63634,#63635,#63636));
#26537=EDGE_LOOP('',(#63637,#63638,#63639,#63640));
#26538=EDGE_LOOP('',(#63641,#63642,#63643,#63644));
#26539=EDGE_LOOP('',(#63645,#63646,#63647,#63648));
#26540=EDGE_LOOP('',(#63649,#63650,#63651,#63652));
#26541=EDGE_LOOP('',(#63653,#63654,#63655,#63656));
#26542=EDGE_LOOP('',(#63657,#63658,#63659,#63660));
#26543=EDGE_LOOP('',(#63661,#63662,#63663,#63664));
#26544=EDGE_LOOP('',(#63665,#63666,#63667,#63668));
#26545=EDGE_LOOP('',(#63669,#63670,#63671,#63672));
#26546=EDGE_LOOP('',(#63673,#63674,#63675,#63676));
#26547=EDGE_LOOP('',(#63677,#63678,#63679,#63680));
#26548=EDGE_LOOP('',(#63681,#63682,#63683,#63684));
#26549=EDGE_LOOP('',(#63685,#63686,#63687,#63688));
#26550=EDGE_LOOP('',(#63689,#63690,#63691,#63692));
#26551=EDGE_LOOP('',(#63693,#63694,#63695,#63696));
#26552=EDGE_LOOP('',(#63697,#63698,#63699,#63700));
#26553=EDGE_LOOP('',(#63701,#63702,#63703,#63704));
#26554=EDGE_LOOP('',(#63705,#63706,#63707,#63708));
#26555=EDGE_LOOP('',(#63709,#63710,#63711,#63712));
#26556=EDGE_LOOP('',(#63713,#63714,#63715,#63716));
#26557=EDGE_LOOP('',(#63717,#63718,#63719,#63720));
#26558=EDGE_LOOP('',(#63721,#63722,#63723,#63724));
#26559=EDGE_LOOP('',(#63725,#63726,#63727,#63728));
#26560=EDGE_LOOP('',(#63729,#63730,#63731,#63732));
#26561=EDGE_LOOP('',(#63733,#63734,#63735,#63736));
#26562=EDGE_LOOP('',(#63737,#63738,#63739,#63740));
#26563=EDGE_LOOP('',(#63741,#63742,#63743,#63744));
#26564=EDGE_LOOP('',(#63745,#63746,#63747,#63748));
#26565=EDGE_LOOP('',(#63749,#63750,#63751,#63752));
#26566=EDGE_LOOP('',(#63753,#63754,#63755,#63756));
#26567=EDGE_LOOP('',(#63757,#63758,#63759,#63760));
#26568=EDGE_LOOP('',(#63761,#63762,#63763,#63764));
#26569=EDGE_LOOP('',(#63765,#63766,#63767,#63768));
#26570=EDGE_LOOP('',(#63769,#63770,#63771,#63772));
#26571=EDGE_LOOP('',(#63773,#63774,#63775,#63776));
#26572=EDGE_LOOP('',(#63777,#63778,#63779,#63780));
#26573=EDGE_LOOP('',(#63781,#63782,#63783,#63784));
#26574=EDGE_LOOP('',(#63785,#63786,#63787,#63788));
#26575=EDGE_LOOP('',(#63789,#63790,#63791,#63792));
#26576=EDGE_LOOP('',(#63793,#63794,#63795,#63796));
#26577=EDGE_LOOP('',(#63797,#63798,#63799,#63800));
#26578=EDGE_LOOP('',(#63801,#63802,#63803,#63804));
#26579=EDGE_LOOP('',(#63805,#63806,#63807,#63808));
#26580=EDGE_LOOP('',(#63809,#63810,#63811,#63812));
#26581=EDGE_LOOP('',(#63813,#63814,#63815,#63816));
#26582=EDGE_LOOP('',(#63817,#63818,#63819,#63820));
#26583=EDGE_LOOP('',(#63821,#63822,#63823,#63824));
#26584=EDGE_LOOP('',(#63825,#63826,#63827,#63828));
#26585=EDGE_LOOP('',(#63829,#63830,#63831,#63832));
#26586=EDGE_LOOP('',(#63833,#63834,#63835,#63836));
#26587=EDGE_LOOP('',(#63837,#63838,#63839,#63840));
#26588=EDGE_LOOP('',(#63841,#63842,#63843,#63844));
#26589=EDGE_LOOP('',(#63845,#63846,#63847,#63848));
#26590=EDGE_LOOP('',(#63849,#63850,#63851,#63852));
#26591=EDGE_LOOP('',(#63853,#63854,#63855,#63856));
#26592=EDGE_LOOP('',(#63857,#63858,#63859,#63860));
#26593=EDGE_LOOP('',(#63861,#63862,#63863,#63864));
#26594=EDGE_LOOP('',(#63865,#63866,#63867,#63868));
#26595=EDGE_LOOP('',(#63869,#63870,#63871,#63872));
#26596=EDGE_LOOP('',(#63873,#63874,#63875,#63876));
#26597=EDGE_LOOP('',(#63877,#63878,#63879,#63880));
#26598=EDGE_LOOP('',(#63881,#63882,#63883,#63884));
#26599=EDGE_LOOP('',(#63885,#63886,#63887,#63888));
#26600=EDGE_LOOP('',(#63889,#63890,#63891,#63892));
#26601=EDGE_LOOP('',(#63893,#63894,#63895,#63896));
#26602=EDGE_LOOP('',(#63897,#63898,#63899,#63900));
#26603=EDGE_LOOP('',(#63901,#63902,#63903,#63904));
#26604=EDGE_LOOP('',(#63905,#63906,#63907,#63908));
#26605=EDGE_LOOP('',(#63909,#63910,#63911,#63912));
#26606=EDGE_LOOP('',(#63913,#63914,#63915,#63916));
#26607=EDGE_LOOP('',(#63917,#63918,#63919,#63920));
#26608=EDGE_LOOP('',(#63921,#63922,#63923,#63924));
#26609=EDGE_LOOP('',(#63925,#63926,#63927,#63928));
#26610=EDGE_LOOP('',(#63929,#63930,#63931,#63932));
#26611=EDGE_LOOP('',(#63933,#63934,#63935,#63936));
#26612=EDGE_LOOP('',(#63937,#63938,#63939,#63940));
#26613=EDGE_LOOP('',(#63941,#63942,#63943,#63944));
#26614=EDGE_LOOP('',(#63945,#63946,#63947,#63948));
#26615=EDGE_LOOP('',(#63949,#63950,#63951,#63952));
#26616=EDGE_LOOP('',(#63953,#63954,#63955,#63956));
#26617=EDGE_LOOP('',(#63957,#63958,#63959,#63960));
#26618=EDGE_LOOP('',(#63961,#63962,#63963,#63964));
#26619=EDGE_LOOP('',(#63965,#63966,#63967,#63968));
#26620=EDGE_LOOP('',(#63969,#63970,#63971,#63972));
#26621=EDGE_LOOP('',(#63973,#63974,#63975,#63976));
#26622=EDGE_LOOP('',(#63977,#63978,#63979,#63980));
#26623=EDGE_LOOP('',(#63981,#63982,#63983,#63984));
#26624=EDGE_LOOP('',(#63985,#63986,#63987,#63988));
#26625=EDGE_LOOP('',(#63989,#63990,#63991,#63992));
#26626=EDGE_LOOP('',(#63993,#63994,#63995,#63996));
#26627=EDGE_LOOP('',(#63997,#63998,#63999,#64000));
#26628=EDGE_LOOP('',(#64001,#64002,#64003,#64004));
#26629=EDGE_LOOP('',(#64005,#64006,#64007,#64008));
#26630=EDGE_LOOP('',(#64009,#64010,#64011,#64012));
#26631=EDGE_LOOP('',(#64013,#64014,#64015,#64016));
#26632=EDGE_LOOP('',(#64017,#64018,#64019,#64020));
#26633=EDGE_LOOP('',(#64021,#64022,#64023,#64024));
#26634=EDGE_LOOP('',(#64025,#64026,#64027,#64028));
#26635=EDGE_LOOP('',(#64029,#64030,#64031,#64032));
#26636=EDGE_LOOP('',(#64033,#64034,#64035,#64036));
#26637=EDGE_LOOP('',(#64037,#64038,#64039,#64040));
#26638=EDGE_LOOP('',(#64041,#64042,#64043,#64044));
#26639=EDGE_LOOP('',(#64045,#64046,#64047,#64048));
#26640=EDGE_LOOP('',(#64049,#64050,#64051,#64052));
#26641=EDGE_LOOP('',(#64053,#64054,#64055,#64056));
#26642=EDGE_LOOP('',(#64057,#64058,#64059,#64060));
#26643=EDGE_LOOP('',(#64061,#64062,#64063,#64064));
#26644=EDGE_LOOP('',(#64065,#64066,#64067,#64068));
#26645=EDGE_LOOP('',(#64069,#64070,#64071,#64072));
#26646=EDGE_LOOP('',(#64073,#64074,#64075,#64076));
#26647=EDGE_LOOP('',(#64077,#64078,#64079,#64080));
#26648=EDGE_LOOP('',(#64081,#64082,#64083,#64084));
#26649=EDGE_LOOP('',(#64085,#64086,#64087,#64088));
#26650=EDGE_LOOP('',(#64089,#64090,#64091,#64092));
#26651=EDGE_LOOP('',(#64093,#64094,#64095,#64096));
#26652=EDGE_LOOP('',(#64097,#64098,#64099,#64100));
#26653=EDGE_LOOP('',(#64101,#64102,#64103,#64104));
#26654=EDGE_LOOP('',(#64105,#64106,#64107,#64108));
#26655=EDGE_LOOP('',(#64109,#64110,#64111,#64112));
#26656=EDGE_LOOP('',(#64113,#64114,#64115,#64116));
#26657=EDGE_LOOP('',(#64117,#64118,#64119,#64120));
#26658=EDGE_LOOP('',(#64121,#64122,#64123,#64124));
#26659=EDGE_LOOP('',(#64125,#64126,#64127,#64128));
#26660=EDGE_LOOP('',(#64129,#64130,#64131,#64132));
#26661=EDGE_LOOP('',(#64133,#64134,#64135,#64136));
#26662=EDGE_LOOP('',(#64137,#64138,#64139,#64140));
#26663=EDGE_LOOP('',(#64141,#64142,#64143,#64144));
#26664=EDGE_LOOP('',(#64145,#64146,#64147,#64148));
#26665=EDGE_LOOP('',(#64149,#64150,#64151,#64152));
#26666=EDGE_LOOP('',(#64153,#64154,#64155,#64156));
#26667=EDGE_LOOP('',(#64157,#64158,#64159,#64160));
#26668=EDGE_LOOP('',(#64161,#64162,#64163,#64164));
#26669=EDGE_LOOP('',(#64165,#64166,#64167,#64168));
#26670=EDGE_LOOP('',(#64169,#64170,#64171,#64172));
#26671=EDGE_LOOP('',(#64173,#64174,#64175,#64176));
#26672=EDGE_LOOP('',(#64177,#64178,#64179,#64180));
#26673=EDGE_LOOP('',(#64181,#64182,#64183,#64184));
#26674=EDGE_LOOP('',(#64185,#64186,#64187,#64188));
#26675=EDGE_LOOP('',(#64189,#64190,#64191,#64192));
#26676=EDGE_LOOP('',(#64193,#64194,#64195,#64196));
#26677=EDGE_LOOP('',(#64197,#64198,#64199,#64200));
#26678=EDGE_LOOP('',(#64201,#64202,#64203,#64204));
#26679=EDGE_LOOP('',(#64205,#64206,#64207,#64208));
#26680=EDGE_LOOP('',(#64209,#64210,#64211,#64212));
#26681=EDGE_LOOP('',(#64213,#64214,#64215,#64216));
#26682=EDGE_LOOP('',(#64217,#64218,#64219,#64220));
#26683=EDGE_LOOP('',(#64221,#64222,#64223,#64224));
#26684=EDGE_LOOP('',(#64225,#64226,#64227,#64228));
#26685=EDGE_LOOP('',(#64229,#64230,#64231,#64232));
#26686=EDGE_LOOP('',(#64233,#64234,#64235,#64236));
#26687=EDGE_LOOP('',(#64237,#64238,#64239,#64240));
#26688=EDGE_LOOP('',(#64241,#64242,#64243,#64244));
#26689=EDGE_LOOP('',(#64245,#64246,#64247,#64248));
#26690=EDGE_LOOP('',(#64249,#64250,#64251,#64252));
#26691=EDGE_LOOP('',(#64253,#64254,#64255,#64256));
#26692=EDGE_LOOP('',(#64257,#64258,#64259,#64260));
#26693=EDGE_LOOP('',(#64261,#64262,#64263,#64264));
#26694=EDGE_LOOP('',(#64265,#64266,#64267,#64268));
#26695=EDGE_LOOP('',(#64269,#64270,#64271,#64272));
#26696=EDGE_LOOP('',(#64273,#64274,#64275,#64276));
#26697=EDGE_LOOP('',(#64277,#64278,#64279,#64280));
#26698=EDGE_LOOP('',(#64281,#64282,#64283,#64284));
#26699=EDGE_LOOP('',(#64285,#64286,#64287,#64288));
#26700=EDGE_LOOP('',(#64289,#64290,#64291,#64292));
#26701=EDGE_LOOP('',(#64293,#64294,#64295,#64296));
#26702=EDGE_LOOP('',(#64297,#64298,#64299,#64300));
#26703=EDGE_LOOP('',(#64301,#64302,#64303,#64304));
#26704=EDGE_LOOP('',(#64305,#64306,#64307,#64308));
#26705=EDGE_LOOP('',(#64309,#64310,#64311,#64312));
#26706=EDGE_LOOP('',(#64313,#64314,#64315,#64316));
#26707=EDGE_LOOP('',(#64317,#64318,#64319,#64320));
#26708=EDGE_LOOP('',(#64321,#64322,#64323,#64324));
#26709=EDGE_LOOP('',(#64325,#64326,#64327,#64328));
#26710=EDGE_LOOP('',(#64329,#64330,#64331,#64332));
#26711=EDGE_LOOP('',(#64333,#64334,#64335,#64336));
#26712=EDGE_LOOP('',(#64337,#64338,#64339,#64340));
#26713=EDGE_LOOP('',(#64341,#64342,#64343,#64344));
#26714=EDGE_LOOP('',(#64345,#64346,#64347,#64348));
#26715=EDGE_LOOP('',(#64349,#64350,#64351,#64352));
#26716=EDGE_LOOP('',(#64353,#64354,#64355,#64356));
#26717=EDGE_LOOP('',(#64357,#64358,#64359,#64360));
#26718=EDGE_LOOP('',(#64361,#64362,#64363,#64364));
#26719=EDGE_LOOP('',(#64365,#64366,#64367,#64368));
#26720=EDGE_LOOP('',(#64369,#64370,#64371,#64372));
#26721=EDGE_LOOP('',(#64373,#64374,#64375,#64376));
#26722=EDGE_LOOP('',(#64377,#64378,#64379,#64380));
#26723=EDGE_LOOP('',(#64381,#64382,#64383,#64384));
#26724=EDGE_LOOP('',(#64385,#64386,#64387,#64388));
#26725=EDGE_LOOP('',(#64389,#64390,#64391,#64392));
#26726=EDGE_LOOP('',(#64393,#64394,#64395,#64396));
#26727=EDGE_LOOP('',(#64397,#64398,#64399,#64400));
#26728=EDGE_LOOP('',(#64401,#64402,#64403,#64404));
#26729=EDGE_LOOP('',(#64405,#64406,#64407,#64408));
#26730=EDGE_LOOP('',(#64409,#64410,#64411,#64412));
#26731=EDGE_LOOP('',(#64413,#64414,#64415,#64416));
#26732=EDGE_LOOP('',(#64417,#64418,#64419,#64420));
#26733=EDGE_LOOP('',(#64421,#64422,#64423,#64424));
#26734=EDGE_LOOP('',(#64425,#64426,#64427,#64428));
#26735=EDGE_LOOP('',(#64429,#64430,#64431,#64432));
#26736=EDGE_LOOP('',(#64433,#64434,#64435,#64436));
#26737=EDGE_LOOP('',(#64437,#64438,#64439,#64440));
#26738=EDGE_LOOP('',(#64441,#64442,#64443,#64444));
#26739=EDGE_LOOP('',(#64445,#64446,#64447,#64448));
#26740=EDGE_LOOP('',(#64449,#64450,#64451,#64452));
#26741=EDGE_LOOP('',(#64453,#64454,#64455,#64456));
#26742=EDGE_LOOP('',(#64457,#64458,#64459,#64460));
#26743=EDGE_LOOP('',(#64461,#64462,#64463,#64464));
#26744=EDGE_LOOP('',(#64465,#64466,#64467,#64468));
#26745=EDGE_LOOP('',(#64469,#64470,#64471,#64472));
#26746=EDGE_LOOP('',(#64473,#64474,#64475,#64476));
#26747=EDGE_LOOP('',(#64477,#64478,#64479,#64480));
#26748=EDGE_LOOP('',(#64481,#64482,#64483,#64484));
#26749=EDGE_LOOP('',(#64485,#64486,#64487,#64488));
#26750=EDGE_LOOP('',(#64489,#64490,#64491,#64492));
#26751=EDGE_LOOP('',(#64493,#64494,#64495,#64496));
#26752=EDGE_LOOP('',(#64497,#64498,#64499,#64500));
#26753=EDGE_LOOP('',(#64501,#64502,#64503,#64504));
#26754=EDGE_LOOP('',(#64505,#64506,#64507,#64508));
#26755=EDGE_LOOP('',(#64509,#64510,#64511,#64512));
#26756=EDGE_LOOP('',(#64513,#64514,#64515,#64516));
#26757=EDGE_LOOP('',(#64517,#64518,#64519,#64520));
#26758=EDGE_LOOP('',(#64521,#64522,#64523,#64524));
#26759=EDGE_LOOP('',(#64525,#64526,#64527,#64528));
#26760=EDGE_LOOP('',(#64529,#64530,#64531,#64532));
#26761=EDGE_LOOP('',(#64533,#64534,#64535,#64536));
#26762=EDGE_LOOP('',(#64537,#64538,#64539,#64540));
#26763=EDGE_LOOP('',(#64541,#64542,#64543,#64544));
#26764=EDGE_LOOP('',(#64545,#64546,#64547,#64548));
#26765=EDGE_LOOP('',(#64549,#64550,#64551,#64552));
#26766=EDGE_LOOP('',(#64553,#64554,#64555,#64556));
#26767=EDGE_LOOP('',(#64557,#64558,#64559,#64560));
#26768=EDGE_LOOP('',(#64561,#64562,#64563,#64564));
#26769=EDGE_LOOP('',(#64565,#64566,#64567,#64568));
#26770=EDGE_LOOP('',(#64569,#64570,#64571,#64572));
#26771=EDGE_LOOP('',(#64573,#64574,#64575,#64576));
#26772=EDGE_LOOP('',(#64577,#64578,#64579,#64580));
#26773=EDGE_LOOP('',(#64581,#64582,#64583,#64584));
#26774=EDGE_LOOP('',(#64585,#64586,#64587,#64588));
#26775=EDGE_LOOP('',(#64589,#64590,#64591,#64592));
#26776=EDGE_LOOP('',(#64593,#64594,#64595,#64596));
#26777=EDGE_LOOP('',(#64597,#64598,#64599,#64600));
#26778=EDGE_LOOP('',(#64601,#64602,#64603,#64604));
#26779=EDGE_LOOP('',(#64605,#64606,#64607,#64608));
#26780=EDGE_LOOP('',(#64609,#64610,#64611,#64612));
#26781=EDGE_LOOP('',(#64613,#64614,#64615,#64616));
#26782=EDGE_LOOP('',(#64617,#64618,#64619,#64620));
#26783=EDGE_LOOP('',(#64621,#64622,#64623,#64624));
#26784=EDGE_LOOP('',(#64625,#64626,#64627,#64628));
#26785=EDGE_LOOP('',(#64629,#64630,#64631,#64632));
#26786=EDGE_LOOP('',(#64633,#64634,#64635,#64636));
#26787=EDGE_LOOP('',(#64637,#64638,#64639,#64640));
#26788=EDGE_LOOP('',(#64641,#64642,#64643,#64644));
#26789=EDGE_LOOP('',(#64645,#64646,#64647,#64648));
#26790=EDGE_LOOP('',(#64649,#64650,#64651,#64652));
#26791=EDGE_LOOP('',(#64653,#64654,#64655,#64656));
#26792=EDGE_LOOP('',(#64657,#64658,#64659,#64660));
#26793=EDGE_LOOP('',(#64661,#64662,#64663,#64664));
#26794=EDGE_LOOP('',(#64665,#64666,#64667,#64668));
#26795=EDGE_LOOP('',(#64669,#64670,#64671,#64672));
#26796=EDGE_LOOP('',(#64673,#64674,#64675,#64676));
#26797=EDGE_LOOP('',(#64677,#64678,#64679,#64680));
#26798=EDGE_LOOP('',(#64681,#64682,#64683,#64684));
#26799=EDGE_LOOP('',(#64685,#64686,#64687,#64688));
#26800=EDGE_LOOP('',(#64689,#64690,#64691,#64692));
#26801=EDGE_LOOP('',(#64693,#64694,#64695,#64696));
#26802=EDGE_LOOP('',(#64697,#64698,#64699,#64700));
#26803=EDGE_LOOP('',(#64701,#64702,#64703,#64704));
#26804=EDGE_LOOP('',(#64705,#64706,#64707,#64708));
#26805=EDGE_LOOP('',(#64709,#64710,#64711,#64712));
#26806=EDGE_LOOP('',(#64713,#64714,#64715,#64716));
#26807=EDGE_LOOP('',(#64717,#64718,#64719,#64720));
#26808=EDGE_LOOP('',(#64721,#64722,#64723,#64724));
#26809=EDGE_LOOP('',(#64725,#64726,#64727,#64728));
#26810=EDGE_LOOP('',(#64729,#64730,#64731,#64732));
#26811=EDGE_LOOP('',(#64733,#64734,#64735,#64736));
#26812=EDGE_LOOP('',(#64737,#64738,#64739,#64740));
#26813=EDGE_LOOP('',(#64741,#64742,#64743,#64744));
#26814=EDGE_LOOP('',(#64745,#64746,#64747,#64748));
#26815=EDGE_LOOP('',(#64749,#64750,#64751,#64752));
#26816=EDGE_LOOP('',(#64753,#64754,#64755,#64756));
#26817=EDGE_LOOP('',(#64757,#64758,#64759,#64760));
#26818=EDGE_LOOP('',(#64761,#64762,#64763,#64764));
#26819=EDGE_LOOP('',(#64765,#64766,#64767,#64768));
#26820=EDGE_LOOP('',(#64769,#64770,#64771,#64772));
#26821=EDGE_LOOP('',(#64773,#64774,#64775,#64776));
#26822=EDGE_LOOP('',(#64777,#64778,#64779,#64780));
#26823=EDGE_LOOP('',(#64781,#64782,#64783,#64784));
#26824=EDGE_LOOP('',(#64785,#64786,#64787,#64788));
#26825=EDGE_LOOP('',(#64789,#64790,#64791,#64792));
#26826=EDGE_LOOP('',(#64793,#64794,#64795,#64796));
#26827=EDGE_LOOP('',(#64797,#64798,#64799,#64800));
#26828=EDGE_LOOP('',(#64801,#64802,#64803,#64804));
#26829=EDGE_LOOP('',(#64805,#64806,#64807,#64808));
#26830=EDGE_LOOP('',(#64809,#64810,#64811,#64812));
#26831=EDGE_LOOP('',(#64813,#64814,#64815,#64816));
#26832=EDGE_LOOP('',(#64817,#64818,#64819,#64820));
#26833=EDGE_LOOP('',(#64821,#64822,#64823,#64824));
#26834=EDGE_LOOP('',(#64825,#64826,#64827,#64828));
#26835=EDGE_LOOP('',(#64829,#64830,#64831,#64832));
#26836=EDGE_LOOP('',(#64833,#64834,#64835,#64836));
#26837=EDGE_LOOP('',(#64837,#64838,#64839,#64840));
#26838=EDGE_LOOP('',(#64841,#64842,#64843,#64844));
#26839=EDGE_LOOP('',(#64845,#64846,#64847,#64848));
#26840=EDGE_LOOP('',(#64849,#64850,#64851,#64852));
#26841=EDGE_LOOP('',(#64853,#64854,#64855,#64856));
#26842=EDGE_LOOP('',(#64857,#64858,#64859,#64860));
#26843=EDGE_LOOP('',(#64861,#64862,#64863,#64864));
#26844=EDGE_LOOP('',(#64865,#64866,#64867,#64868));
#26845=EDGE_LOOP('',(#64869,#64870,#64871,#64872));
#26846=EDGE_LOOP('',(#64873,#64874,#64875,#64876));
#26847=EDGE_LOOP('',(#64877,#64878,#64879,#64880));
#26848=EDGE_LOOP('',(#64881,#64882,#64883,#64884));
#26849=EDGE_LOOP('',(#64885,#64886,#64887,#64888));
#26850=EDGE_LOOP('',(#64889,#64890,#64891,#64892));
#26851=EDGE_LOOP('',(#64893,#64894,#64895,#64896));
#26852=EDGE_LOOP('',(#64897,#64898,#64899,#64900));
#26853=EDGE_LOOP('',(#64901,#64902,#64903,#64904));
#26854=EDGE_LOOP('',(#64905,#64906,#64907,#64908));
#26855=EDGE_LOOP('',(#64909,#64910,#64911,#64912));
#26856=EDGE_LOOP('',(#64913,#64914,#64915,#64916));
#26857=EDGE_LOOP('',(#64917,#64918,#64919,#64920));
#26858=EDGE_LOOP('',(#64921,#64922,#64923,#64924));
#26859=EDGE_LOOP('',(#64925,#64926,#64927,#64928));
#26860=EDGE_LOOP('',(#64929,#64930,#64931,#64932));
#26861=EDGE_LOOP('',(#64933,#64934,#64935,#64936));
#26862=EDGE_LOOP('',(#64937,#64938,#64939,#64940));
#26863=EDGE_LOOP('',(#64941,#64942,#64943,#64944));
#26864=EDGE_LOOP('',(#64945,#64946,#64947,#64948));
#26865=EDGE_LOOP('',(#64949,#64950,#64951,#64952));
#26866=EDGE_LOOP('',(#64953,#64954,#64955,#64956));
#26867=EDGE_LOOP('',(#64957,#64958,#64959,#64960));
#26868=EDGE_LOOP('',(#64961,#64962,#64963,#64964));
#26869=EDGE_LOOP('',(#64965,#64966,#64967,#64968));
#26870=EDGE_LOOP('',(#64969,#64970,#64971,#64972));
#26871=EDGE_LOOP('',(#64973,#64974,#64975,#64976));
#26872=EDGE_LOOP('',(#64977,#64978,#64979,#64980));
#26873=EDGE_LOOP('',(#64981,#64982,#64983,#64984));
#26874=EDGE_LOOP('',(#64985,#64986,#64987,#64988));
#26875=EDGE_LOOP('',(#64989,#64990,#64991,#64992));
#26876=EDGE_LOOP('',(#64993,#64994,#64995,#64996));
#26877=EDGE_LOOP('',(#64997,#64998,#64999,#65000));
#26878=EDGE_LOOP('',(#65001,#65002,#65003,#65004));
#26879=EDGE_LOOP('',(#65005,#65006,#65007,#65008));
#26880=EDGE_LOOP('',(#65009,#65010,#65011,#65012));
#26881=EDGE_LOOP('',(#65013,#65014,#65015,#65016));
#26882=EDGE_LOOP('',(#65017,#65018,#65019,#65020));
#26883=EDGE_LOOP('',(#65021,#65022,#65023,#65024));
#26884=EDGE_LOOP('',(#65025,#65026,#65027,#65028));
#26885=EDGE_LOOP('',(#65029,#65030,#65031,#65032));
#26886=EDGE_LOOP('',(#65033,#65034,#65035,#65036));
#26887=EDGE_LOOP('',(#65037,#65038,#65039,#65040));
#26888=EDGE_LOOP('',(#65041,#65042,#65043,#65044));
#26889=EDGE_LOOP('',(#65045,#65046,#65047,#65048));
#26890=EDGE_LOOP('',(#65049,#65050,#65051,#65052));
#26891=EDGE_LOOP('',(#65053,#65054,#65055,#65056));
#26892=EDGE_LOOP('',(#65057,#65058,#65059,#65060));
#26893=EDGE_LOOP('',(#65061,#65062,#65063,#65064));
#26894=EDGE_LOOP('',(#65065,#65066,#65067,#65068));
#26895=EDGE_LOOP('',(#65069,#65070,#65071,#65072));
#26896=EDGE_LOOP('',(#65073,#65074,#65075,#65076));
#26897=EDGE_LOOP('',(#65077,#65078,#65079,#65080));
#26898=EDGE_LOOP('',(#65081,#65082,#65083,#65084));
#26899=EDGE_LOOP('',(#65085,#65086,#65087,#65088));
#26900=EDGE_LOOP('',(#65089,#65090,#65091,#65092));
#26901=EDGE_LOOP('',(#65093,#65094,#65095,#65096));
#26902=EDGE_LOOP('',(#65097,#65098,#65099,#65100));
#26903=EDGE_LOOP('',(#65101,#65102,#65103,#65104));
#26904=EDGE_LOOP('',(#65105,#65106,#65107,#65108));
#26905=EDGE_LOOP('',(#65109,#65110,#65111,#65112));
#26906=EDGE_LOOP('',(#65113,#65114,#65115,#65116));
#26907=EDGE_LOOP('',(#65117,#65118,#65119,#65120));
#26908=EDGE_LOOP('',(#65121,#65122,#65123,#65124));
#26909=EDGE_LOOP('',(#65125,#65126,#65127,#65128));
#26910=EDGE_LOOP('',(#65129,#65130,#65131,#65132));
#26911=EDGE_LOOP('',(#65133,#65134,#65135,#65136));
#26912=EDGE_LOOP('',(#65137,#65138,#65139,#65140));
#26913=EDGE_LOOP('',(#65141,#65142,#65143,#65144));
#26914=EDGE_LOOP('',(#65145,#65146,#65147,#65148));
#26915=EDGE_LOOP('',(#65149,#65150,#65151,#65152));
#26916=EDGE_LOOP('',(#65153,#65154,#65155,#65156));
#26917=EDGE_LOOP('',(#65157,#65158,#65159,#65160));
#26918=EDGE_LOOP('',(#65161,#65162,#65163,#65164));
#26919=EDGE_LOOP('',(#65165,#65166,#65167,#65168));
#26920=EDGE_LOOP('',(#65169,#65170,#65171,#65172));
#26921=EDGE_LOOP('',(#65173,#65174,#65175,#65176));
#26922=EDGE_LOOP('',(#65177,#65178,#65179,#65180));
#26923=EDGE_LOOP('',(#65181,#65182,#65183,#65184));
#26924=EDGE_LOOP('',(#65185,#65186,#65187,#65188));
#26925=EDGE_LOOP('',(#65189,#65190,#65191,#65192));
#26926=EDGE_LOOP('',(#65193,#65194,#65195,#65196));
#26927=EDGE_LOOP('',(#65197,#65198,#65199,#65200));
#26928=EDGE_LOOP('',(#65201,#65202,#65203,#65204));
#26929=EDGE_LOOP('',(#65205,#65206,#65207,#65208));
#26930=EDGE_LOOP('',(#65209,#65210,#65211,#65212));
#26931=EDGE_LOOP('',(#65213,#65214,#65215,#65216));
#26932=EDGE_LOOP('',(#65217,#65218,#65219,#65220));
#26933=EDGE_LOOP('',(#65221,#65222,#65223,#65224));
#26934=EDGE_LOOP('',(#65225,#65226,#65227,#65228));
#26935=EDGE_LOOP('',(#65229,#65230,#65231,#65232));
#26936=EDGE_LOOP('',(#65233,#65234,#65235,#65236));
#26937=EDGE_LOOP('',(#65237,#65238,#65239,#65240));
#26938=EDGE_LOOP('',(#65241,#65242,#65243,#65244));
#26939=EDGE_LOOP('',(#65245,#65246,#65247,#65248));
#26940=EDGE_LOOP('',(#65249,#65250,#65251,#65252));
#26941=EDGE_LOOP('',(#65253,#65254,#65255,#65256));
#26942=EDGE_LOOP('',(#65257,#65258,#65259,#65260));
#26943=EDGE_LOOP('',(#65261,#65262,#65263,#65264));
#26944=EDGE_LOOP('',(#65265,#65266,#65267,#65268));
#26945=EDGE_LOOP('',(#65269,#65270,#65271,#65272));
#26946=EDGE_LOOP('',(#65273,#65274,#65275,#65276));
#26947=EDGE_LOOP('',(#65277,#65278,#65279,#65280));
#26948=EDGE_LOOP('',(#65281,#65282,#65283,#65284));
#26949=EDGE_LOOP('',(#65285,#65286,#65287,#65288));
#26950=EDGE_LOOP('',(#65289,#65290,#65291,#65292));
#26951=EDGE_LOOP('',(#65293,#65294,#65295,#65296));
#26952=EDGE_LOOP('',(#65297,#65298,#65299,#65300));
#26953=EDGE_LOOP('',(#65301,#65302,#65303,#65304));
#26954=EDGE_LOOP('',(#65305,#65306,#65307,#65308));
#26955=EDGE_LOOP('',(#65309,#65310,#65311,#65312));
#26956=EDGE_LOOP('',(#65313,#65314,#65315,#65316));
#26957=EDGE_LOOP('',(#65317,#65318,#65319,#65320));
#26958=EDGE_LOOP('',(#65321,#65322,#65323,#65324));
#26959=EDGE_LOOP('',(#65325,#65326,#65327,#65328));
#26960=EDGE_LOOP('',(#65329,#65330,#65331,#65332));
#26961=EDGE_LOOP('',(#65333,#65334,#65335,#65336));
#26962=EDGE_LOOP('',(#65337,#65338,#65339,#65340));
#26963=EDGE_LOOP('',(#65341,#65342,#65343,#65344));
#26964=EDGE_LOOP('',(#65345,#65346,#65347,#65348));
#26965=EDGE_LOOP('',(#65349,#65350,#65351,#65352));
#26966=EDGE_LOOP('',(#65353,#65354,#65355,#65356));
#26967=EDGE_LOOP('',(#65357,#65358,#65359,#65360));
#26968=EDGE_LOOP('',(#65361,#65362,#65363,#65364));
#26969=EDGE_LOOP('',(#65365,#65366,#65367,#65368));
#26970=EDGE_LOOP('',(#65369,#65370,#65371,#65372));
#26971=EDGE_LOOP('',(#65373,#65374,#65375,#65376));
#26972=EDGE_LOOP('',(#65377,#65378,#65379,#65380));
#26973=EDGE_LOOP('',(#65381,#65382,#65383,#65384));
#26974=EDGE_LOOP('',(#65385,#65386,#65387,#65388));
#26975=EDGE_LOOP('',(#65389,#65390,#65391,#65392));
#26976=EDGE_LOOP('',(#65393,#65394,#65395,#65396));
#26977=EDGE_LOOP('',(#65397,#65398,#65399,#65400));
#26978=EDGE_LOOP('',(#65401,#65402,#65403,#65404));
#26979=EDGE_LOOP('',(#65405,#65406,#65407,#65408));
#26980=EDGE_LOOP('',(#65409,#65410,#65411,#65412));
#26981=EDGE_LOOP('',(#65413,#65414,#65415,#65416));
#26982=EDGE_LOOP('',(#65417,#65418,#65419,#65420));
#26983=EDGE_LOOP('',(#65421,#65422,#65423,#65424));
#26984=EDGE_LOOP('',(#65425,#65426,#65427,#65428));
#26985=EDGE_LOOP('',(#65429,#65430,#65431,#65432));
#26986=EDGE_LOOP('',(#65433,#65434,#65435,#65436));
#26987=EDGE_LOOP('',(#65437,#65438,#65439,#65440));
#26988=EDGE_LOOP('',(#65441,#65442,#65443,#65444));
#26989=EDGE_LOOP('',(#65445,#65446,#65447,#65448));
#26990=EDGE_LOOP('',(#65449,#65450,#65451,#65452));
#26991=EDGE_LOOP('',(#65453,#65454,#65455,#65456));
#26992=EDGE_LOOP('',(#65457,#65458,#65459,#65460));
#26993=EDGE_LOOP('',(#65461,#65462,#65463,#65464));
#26994=EDGE_LOOP('',(#65465,#65466,#65467,#65468));
#26995=EDGE_LOOP('',(#65469,#65470,#65471,#65472));
#26996=EDGE_LOOP('',(#65473,#65474,#65475,#65476));
#26997=EDGE_LOOP('',(#65477,#65478,#65479,#65480));
#26998=EDGE_LOOP('',(#65481,#65482,#65483,#65484));
#26999=EDGE_LOOP('',(#65485,#65486,#65487,#65488));
#27000=EDGE_LOOP('',(#65489,#65490,#65491,#65492));
#27001=EDGE_LOOP('',(#65493,#65494,#65495,#65496));
#27002=EDGE_LOOP('',(#65497,#65498,#65499,#65500));
#27003=EDGE_LOOP('',(#65501,#65502,#65503,#65504));
#27004=EDGE_LOOP('',(#65505,#65506,#65507,#65508));
#27005=EDGE_LOOP('',(#65509,#65510,#65511,#65512));
#27006=EDGE_LOOP('',(#65513,#65514,#65515,#65516));
#27007=EDGE_LOOP('',(#65517,#65518,#65519,#65520));
#27008=EDGE_LOOP('',(#65521,#65522,#65523,#65524));
#27009=EDGE_LOOP('',(#65525,#65526,#65527,#65528));
#27010=EDGE_LOOP('',(#65529,#65530,#65531,#65532));
#27011=EDGE_LOOP('',(#65533,#65534,#65535,#65536));
#27012=EDGE_LOOP('',(#65537,#65538,#65539,#65540));
#27013=EDGE_LOOP('',(#65541,#65542,#65543,#65544));
#27014=EDGE_LOOP('',(#65545,#65546,#65547,#65548));
#27015=EDGE_LOOP('',(#65549,#65550,#65551,#65552));
#27016=EDGE_LOOP('',(#65553,#65554,#65555,#65556));
#27017=EDGE_LOOP('',(#65557,#65558,#65559,#65560));
#27018=EDGE_LOOP('',(#65561,#65562,#65563,#65564));
#27019=EDGE_LOOP('',(#65565,#65566,#65567,#65568));
#27020=EDGE_LOOP('',(#65569,#65570,#65571,#65572));
#27021=EDGE_LOOP('',(#65573,#65574,#65575,#65576));
#27022=EDGE_LOOP('',(#65577,#65578,#65579,#65580));
#27023=EDGE_LOOP('',(#65581,#65582,#65583,#65584));
#27024=EDGE_LOOP('',(#65585,#65586,#65587,#65588));
#27025=EDGE_LOOP('',(#65589,#65590,#65591,#65592));
#27026=EDGE_LOOP('',(#65593,#65594,#65595,#65596));
#27027=EDGE_LOOP('',(#65597,#65598,#65599,#65600));
#27028=EDGE_LOOP('',(#65601,#65602,#65603,#65604));
#27029=EDGE_LOOP('',(#65605,#65606,#65607,#65608));
#27030=EDGE_LOOP('',(#65609,#65610,#65611,#65612));
#27031=EDGE_LOOP('',(#65613,#65614,#65615,#65616));
#27032=EDGE_LOOP('',(#65617,#65618,#65619,#65620));
#27033=EDGE_LOOP('',(#65621,#65622,#65623,#65624));
#27034=EDGE_LOOP('',(#65625,#65626,#65627,#65628));
#27035=EDGE_LOOP('',(#65629,#65630,#65631,#65632));
#27036=EDGE_LOOP('',(#65633,#65634,#65635,#65636));
#27037=EDGE_LOOP('',(#65637,#65638,#65639,#65640));
#27038=EDGE_LOOP('',(#65641,#65642,#65643,#65644));
#27039=EDGE_LOOP('',(#65645,#65646,#65647,#65648));
#27040=EDGE_LOOP('',(#65649,#65650,#65651,#65652));
#27041=EDGE_LOOP('',(#65653,#65654,#65655,#65656));
#27042=EDGE_LOOP('',(#65657,#65658,#65659,#65660));
#27043=EDGE_LOOP('',(#65661,#65662,#65663,#65664));
#27044=EDGE_LOOP('',(#65665,#65666,#65667,#65668));
#27045=EDGE_LOOP('',(#65669,#65670,#65671,#65672));
#27046=EDGE_LOOP('',(#65673,#65674,#65675,#65676));
#27047=EDGE_LOOP('',(#65677,#65678,#65679,#65680));
#27048=EDGE_LOOP('',(#65681,#65682,#65683,#65684));
#27049=EDGE_LOOP('',(#65685,#65686,#65687,#65688));
#27050=EDGE_LOOP('',(#65689,#65690,#65691,#65692));
#27051=EDGE_LOOP('',(#65693,#65694,#65695,#65696));
#27052=EDGE_LOOP('',(#65697,#65698,#65699,#65700));
#27053=EDGE_LOOP('',(#65701,#65702,#65703,#65704));
#27054=EDGE_LOOP('',(#65705,#65706,#65707,#65708));
#27055=EDGE_LOOP('',(#65709,#65710,#65711,#65712));
#27056=EDGE_LOOP('',(#65713,#65714,#65715,#65716));
#27057=EDGE_LOOP('',(#65717,#65718,#65719,#65720));
#27058=EDGE_LOOP('',(#65721,#65722,#65723,#65724));
#27059=EDGE_LOOP('',(#65725,#65726,#65727,#65728));
#27060=EDGE_LOOP('',(#65729,#65730,#65731,#65732));
#27061=EDGE_LOOP('',(#65733,#65734,#65735,#65736));
#27062=EDGE_LOOP('',(#65737,#65738,#65739,#65740));
#27063=EDGE_LOOP('',(#65741,#65742,#65743,#65744));
#27064=EDGE_LOOP('',(#65745,#65746,#65747,#65748));
#27065=EDGE_LOOP('',(#65749,#65750,#65751,#65752));
#27066=EDGE_LOOP('',(#65753,#65754,#65755,#65756));
#27067=EDGE_LOOP('',(#65757,#65758,#65759,#65760));
#27068=EDGE_LOOP('',(#65761,#65762,#65763,#65764));
#27069=EDGE_LOOP('',(#65765,#65766,#65767,#65768));
#27070=EDGE_LOOP('',(#65769,#65770,#65771,#65772));
#27071=EDGE_LOOP('',(#65773,#65774,#65775,#65776));
#27072=EDGE_LOOP('',(#65777,#65778,#65779,#65780));
#27073=EDGE_LOOP('',(#65781,#65782,#65783,#65784));
#27074=EDGE_LOOP('',(#65785,#65786,#65787,#65788));
#27075=EDGE_LOOP('',(#65789,#65790,#65791,#65792));
#27076=EDGE_LOOP('',(#65793,#65794,#65795,#65796));
#27077=EDGE_LOOP('',(#65797,#65798,#65799,#65800));
#27078=EDGE_LOOP('',(#65801,#65802,#65803,#65804));
#27079=EDGE_LOOP('',(#65805,#65806,#65807,#65808));
#27080=EDGE_LOOP('',(#65809,#65810,#65811,#65812));
#27081=EDGE_LOOP('',(#65813,#65814,#65815,#65816));
#27082=EDGE_LOOP('',(#65817,#65818,#65819,#65820));
#27083=EDGE_LOOP('',(#65821,#65822,#65823,#65824));
#27084=EDGE_LOOP('',(#65825,#65826,#65827,#65828));
#27085=EDGE_LOOP('',(#65829,#65830,#65831,#65832));
#27086=EDGE_LOOP('',(#65833,#65834,#65835,#65836));
#27087=EDGE_LOOP('',(#65837,#65838,#65839,#65840));
#27088=EDGE_LOOP('',(#65841,#65842,#65843,#65844));
#27089=EDGE_LOOP('',(#65845,#65846,#65847,#65848));
#27090=EDGE_LOOP('',(#65849,#65850,#65851,#65852));
#27091=EDGE_LOOP('',(#65853,#65854,#65855,#65856));
#27092=EDGE_LOOP('',(#65857,#65858,#65859,#65860));
#27093=EDGE_LOOP('',(#65861,#65862,#65863,#65864));
#27094=EDGE_LOOP('',(#65865,#65866,#65867,#65868));
#27095=EDGE_LOOP('',(#65869,#65870,#65871,#65872));
#27096=EDGE_LOOP('',(#65873,#65874,#65875,#65876));
#27097=EDGE_LOOP('',(#65877,#65878,#65879,#65880));
#27098=EDGE_LOOP('',(#65881,#65882,#65883,#65884));
#27099=EDGE_LOOP('',(#65885,#65886,#65887,#65888));
#27100=EDGE_LOOP('',(#65889,#65890,#65891,#65892));
#27101=EDGE_LOOP('',(#65893,#65894,#65895,#65896));
#27102=EDGE_LOOP('',(#65897,#65898,#65899,#65900));
#27103=EDGE_LOOP('',(#65901,#65902,#65903,#65904));
#27104=EDGE_LOOP('',(#65905,#65906,#65907,#65908));
#27105=EDGE_LOOP('',(#65909,#65910,#65911,#65912));
#27106=EDGE_LOOP('',(#65913,#65914,#65915,#65916));
#27107=EDGE_LOOP('',(#65917,#65918,#65919,#65920));
#27108=EDGE_LOOP('',(#65921,#65922,#65923,#65924));
#27109=EDGE_LOOP('',(#65925,#65926,#65927,#65928));
#27110=EDGE_LOOP('',(#65929,#65930,#65931,#65932));
#27111=EDGE_LOOP('',(#65933,#65934,#65935,#65936));
#27112=EDGE_LOOP('',(#65937,#65938,#65939,#65940));
#27113=EDGE_LOOP('',(#65941,#65942,#65943,#65944));
#27114=EDGE_LOOP('',(#65945,#65946,#65947,#65948));
#27115=EDGE_LOOP('',(#65949,#65950,#65951,#65952));
#27116=EDGE_LOOP('',(#65953,#65954,#65955,#65956));
#27117=EDGE_LOOP('',(#65957,#65958,#65959,#65960));
#27118=EDGE_LOOP('',(#65961,#65962,#65963,#65964));
#27119=EDGE_LOOP('',(#65965,#65966,#65967,#65968));
#27120=EDGE_LOOP('',(#65969,#65970,#65971,#65972));
#27121=EDGE_LOOP('',(#65973,#65974,#65975,#65976));
#27122=EDGE_LOOP('',(#65977,#65978,#65979,#65980));
#27123=EDGE_LOOP('',(#65981,#65982,#65983,#65984));
#27124=EDGE_LOOP('',(#65985,#65986,#65987,#65988));
#27125=EDGE_LOOP('',(#65989,#65990,#65991,#65992));
#27126=EDGE_LOOP('',(#65993,#65994,#65995,#65996));
#27127=EDGE_LOOP('',(#65997,#65998,#65999,#66000));
#27128=EDGE_LOOP('',(#66001,#66002,#66003,#66004));
#27129=EDGE_LOOP('',(#66005,#66006,#66007,#66008));
#27130=EDGE_LOOP('',(#66009,#66010,#66011,#66012));
#27131=EDGE_LOOP('',(#66013,#66014,#66015,#66016));
#27132=EDGE_LOOP('',(#66017,#66018,#66019,#66020));
#27133=EDGE_LOOP('',(#66021,#66022,#66023,#66024));
#27134=EDGE_LOOP('',(#66025,#66026,#66027,#66028));
#27135=EDGE_LOOP('',(#66029,#66030,#66031,#66032));
#27136=EDGE_LOOP('',(#66033,#66034,#66035,#66036));
#27137=EDGE_LOOP('',(#66037,#66038,#66039,#66040));
#27138=EDGE_LOOP('',(#66041,#66042,#66043,#66044));
#27139=EDGE_LOOP('',(#66045,#66046,#66047,#66048));
#27140=EDGE_LOOP('',(#66049,#66050,#66051,#66052));
#27141=EDGE_LOOP('',(#66053,#66054,#66055,#66056));
#27142=EDGE_LOOP('',(#66057,#66058,#66059,#66060));
#27143=EDGE_LOOP('',(#66061,#66062,#66063,#66064));
#27144=EDGE_LOOP('',(#66065,#66066,#66067,#66068));
#27145=EDGE_LOOP('',(#66069,#66070,#66071,#66072));
#27146=EDGE_LOOP('',(#66073,#66074,#66075,#66076));
#27147=EDGE_LOOP('',(#66077,#66078,#66079,#66080));
#27148=EDGE_LOOP('',(#66081,#66082,#66083,#66084));
#27149=EDGE_LOOP('',(#66085,#66086,#66087,#66088));
#27150=EDGE_LOOP('',(#66089,#66090,#66091,#66092));
#27151=EDGE_LOOP('',(#66093,#66094,#66095,#66096));
#27152=EDGE_LOOP('',(#66097,#66098,#66099,#66100));
#27153=EDGE_LOOP('',(#66101,#66102,#66103,#66104));
#27154=EDGE_LOOP('',(#66105,#66106,#66107,#66108));
#27155=EDGE_LOOP('',(#66109,#66110,#66111,#66112));
#27156=EDGE_LOOP('',(#66113,#66114,#66115,#66116));
#27157=EDGE_LOOP('',(#66117,#66118,#66119,#66120));
#27158=EDGE_LOOP('',(#66121,#66122,#66123,#66124));
#27159=EDGE_LOOP('',(#66125,#66126,#66127,#66128));
#27160=EDGE_LOOP('',(#66129,#66130,#66131,#66132));
#27161=EDGE_LOOP('',(#66133,#66134,#66135,#66136));
#27162=EDGE_LOOP('',(#66137,#66138,#66139,#66140));
#27163=EDGE_LOOP('',(#66141,#66142,#66143,#66144));
#27164=EDGE_LOOP('',(#66145,#66146,#66147,#66148));
#27165=EDGE_LOOP('',(#66149,#66150,#66151,#66152));
#27166=EDGE_LOOP('',(#66153,#66154,#66155,#66156));
#27167=EDGE_LOOP('',(#66157,#66158,#66159,#66160));
#27168=EDGE_LOOP('',(#66161,#66162,#66163,#66164));
#27169=EDGE_LOOP('',(#66165,#66166,#66167,#66168));
#27170=EDGE_LOOP('',(#66169,#66170,#66171,#66172));
#27171=EDGE_LOOP('',(#66173,#66174,#66175,#66176));
#27172=EDGE_LOOP('',(#66177,#66178,#66179,#66180));
#27173=EDGE_LOOP('',(#66181,#66182,#66183,#66184));
#27174=EDGE_LOOP('',(#66185,#66186,#66187,#66188));
#27175=EDGE_LOOP('',(#66189,#66190,#66191,#66192));
#27176=EDGE_LOOP('',(#66193,#66194,#66195,#66196));
#27177=EDGE_LOOP('',(#66197,#66198,#66199,#66200));
#27178=EDGE_LOOP('',(#66201,#66202,#66203,#66204));
#27179=EDGE_LOOP('',(#66205,#66206,#66207,#66208));
#27180=EDGE_LOOP('',(#66209,#66210,#66211,#66212));
#27181=EDGE_LOOP('',(#66213,#66214,#66215,#66216));
#27182=EDGE_LOOP('',(#66217,#66218,#66219,#66220));
#27183=EDGE_LOOP('',(#66221,#66222,#66223,#66224));
#27184=EDGE_LOOP('',(#66225,#66226,#66227,#66228));
#27185=EDGE_LOOP('',(#66229,#66230,#66231,#66232));
#27186=EDGE_LOOP('',(#66233,#66234,#66235,#66236));
#27187=EDGE_LOOP('',(#66237,#66238,#66239,#66240));
#27188=EDGE_LOOP('',(#66241,#66242,#66243,#66244));
#27189=EDGE_LOOP('',(#66245,#66246,#66247,#66248));
#27190=EDGE_LOOP('',(#66249,#66250,#66251,#66252));
#27191=EDGE_LOOP('',(#66253,#66254,#66255,#66256));
#27192=EDGE_LOOP('',(#66257,#66258,#66259,#66260));
#27193=EDGE_LOOP('',(#66261,#66262,#66263,#66264));
#27194=EDGE_LOOP('',(#66265,#66266,#66267,#66268));
#27195=EDGE_LOOP('',(#66269,#66270,#66271,#66272));
#27196=EDGE_LOOP('',(#66273,#66274,#66275,#66276));
#27197=EDGE_LOOP('',(#66277,#66278,#66279,#66280));
#27198=EDGE_LOOP('',(#66281,#66282,#66283,#66284));
#27199=EDGE_LOOP('',(#66285,#66286,#66287,#66288));
#27200=EDGE_LOOP('',(#66289,#66290,#66291,#66292));
#27201=EDGE_LOOP('',(#66293,#66294,#66295,#66296));
#27202=EDGE_LOOP('',(#66297,#66298,#66299,#66300));
#27203=EDGE_LOOP('',(#66301,#66302,#66303,#66304));
#27204=EDGE_LOOP('',(#66305,#66306,#66307,#66308));
#27205=EDGE_LOOP('',(#66309,#66310,#66311,#66312));
#27206=EDGE_LOOP('',(#66313,#66314,#66315,#66316));
#27207=EDGE_LOOP('',(#66317,#66318,#66319,#66320));
#27208=EDGE_LOOP('',(#66321,#66322,#66323,#66324));
#27209=EDGE_LOOP('',(#66325,#66326,#66327,#66328));
#27210=EDGE_LOOP('',(#66329,#66330,#66331,#66332));
#27211=EDGE_LOOP('',(#66333,#66334,#66335,#66336));
#27212=EDGE_LOOP('',(#66337,#66338,#66339,#66340));
#27213=EDGE_LOOP('',(#66341,#66342,#66343,#66344));
#27214=EDGE_LOOP('',(#66345,#66346,#66347,#66348));
#27215=EDGE_LOOP('',(#66349,#66350,#66351,#66352));
#27216=EDGE_LOOP('',(#66353,#66354,#66355,#66356));
#27217=EDGE_LOOP('',(#66357,#66358,#66359,#66360));
#27218=EDGE_LOOP('',(#66361,#66362,#66363,#66364));
#27219=EDGE_LOOP('',(#66365,#66366,#66367,#66368));
#27220=EDGE_LOOP('',(#66369,#66370,#66371,#66372));
#27221=EDGE_LOOP('',(#66373,#66374,#66375,#66376));
#27222=EDGE_LOOP('',(#66377,#66378,#66379,#66380));
#27223=EDGE_LOOP('',(#66381,#66382,#66383,#66384));
#27224=EDGE_LOOP('',(#66385,#66386,#66387,#66388));
#27225=EDGE_LOOP('',(#66389,#66390,#66391,#66392));
#27226=EDGE_LOOP('',(#66393,#66394,#66395,#66396));
#27227=EDGE_LOOP('',(#66397,#66398,#66399,#66400));
#27228=EDGE_LOOP('',(#66401,#66402,#66403,#66404));
#27229=EDGE_LOOP('',(#66405,#66406,#66407,#66408));
#27230=EDGE_LOOP('',(#66409,#66410,#66411,#66412));
#27231=EDGE_LOOP('',(#66413,#66414,#66415,#66416));
#27232=EDGE_LOOP('',(#66417,#66418,#66419,#66420));
#27233=EDGE_LOOP('',(#66421,#66422,#66423,#66424));
#27234=EDGE_LOOP('',(#66425,#66426,#66427,#66428));
#27235=EDGE_LOOP('',(#66429,#66430,#66431,#66432));
#27236=EDGE_LOOP('',(#66433,#66434,#66435,#66436));
#27237=EDGE_LOOP('',(#66437,#66438,#66439,#66440));
#27238=EDGE_LOOP('',(#66441,#66442,#66443,#66444));
#27239=EDGE_LOOP('',(#66445,#66446,#66447,#66448));
#27240=EDGE_LOOP('',(#66449,#66450,#66451,#66452));
#27241=EDGE_LOOP('',(#66453,#66454,#66455,#66456));
#27242=EDGE_LOOP('',(#66457,#66458,#66459,#66460));
#27243=EDGE_LOOP('',(#66461,#66462,#66463,#66464));
#27244=EDGE_LOOP('',(#66465,#66466,#66467,#66468));
#27245=EDGE_LOOP('',(#66469,#66470,#66471,#66472));
#27246=EDGE_LOOP('',(#66473,#66474,#66475,#66476));
#27247=EDGE_LOOP('',(#66477,#66478,#66479,#66480));
#27248=EDGE_LOOP('',(#66481,#66482,#66483,#66484));
#27249=EDGE_LOOP('',(#66485,#66486,#66487,#66488));
#27250=EDGE_LOOP('',(#66489,#66490,#66491,#66492));
#27251=EDGE_LOOP('',(#66493,#66494,#66495,#66496));
#27252=EDGE_LOOP('',(#66497,#66498,#66499,#66500));
#27253=EDGE_LOOP('',(#66501,#66502,#66503,#66504));
#27254=EDGE_LOOP('',(#66505,#66506,#66507,#66508));
#27255=EDGE_LOOP('',(#66509,#66510,#66511,#66512));
#27256=EDGE_LOOP('',(#66513,#66514,#66515,#66516));
#27257=EDGE_LOOP('',(#66517,#66518,#66519,#66520));
#27258=EDGE_LOOP('',(#66521,#66522,#66523,#66524));
#27259=EDGE_LOOP('',(#66525,#66526,#66527,#66528));
#27260=EDGE_LOOP('',(#66529,#66530,#66531,#66532));
#27261=EDGE_LOOP('',(#66533,#66534,#66535,#66536));
#27262=EDGE_LOOP('',(#66537,#66538,#66539,#66540));
#27263=EDGE_LOOP('',(#66541,#66542,#66543,#66544));
#27264=EDGE_LOOP('',(#66545,#66546,#66547,#66548));
#27265=EDGE_LOOP('',(#66549,#66550,#66551,#66552));
#27266=EDGE_LOOP('',(#66553,#66554,#66555,#66556));
#27267=EDGE_LOOP('',(#66557,#66558,#66559,#66560));
#27268=EDGE_LOOP('',(#66561,#66562,#66563,#66564));
#27269=EDGE_LOOP('',(#66565,#66566,#66567,#66568));
#27270=EDGE_LOOP('',(#66569,#66570,#66571,#66572));
#27271=EDGE_LOOP('',(#66573,#66574,#66575,#66576));
#27272=EDGE_LOOP('',(#66577,#66578,#66579,#66580));
#27273=EDGE_LOOP('',(#66581,#66582,#66583,#66584));
#27274=EDGE_LOOP('',(#66585,#66586,#66587,#66588));
#27275=EDGE_LOOP('',(#66589,#66590,#66591,#66592));
#27276=EDGE_LOOP('',(#66593,#66594,#66595,#66596));
#27277=EDGE_LOOP('',(#66597,#66598,#66599,#66600));
#27278=EDGE_LOOP('',(#66601,#66602,#66603,#66604));
#27279=EDGE_LOOP('',(#66605,#66606,#66607,#66608));
#27280=EDGE_LOOP('',(#66609,#66610,#66611,#66612));
#27281=EDGE_LOOP('',(#66613,#66614,#66615,#66616));
#27282=EDGE_LOOP('',(#66617,#66618,#66619,#66620));
#27283=EDGE_LOOP('',(#66621,#66622,#66623,#66624));
#27284=EDGE_LOOP('',(#66625,#66626,#66627,#66628));
#27285=EDGE_LOOP('',(#66629,#66630,#66631,#66632));
#27286=EDGE_LOOP('',(#66633,#66634,#66635,#66636));
#27287=EDGE_LOOP('',(#66637,#66638,#66639,#66640));
#27288=EDGE_LOOP('',(#66641,#66642,#66643,#66644));
#27289=EDGE_LOOP('',(#66645,#66646,#66647,#66648));
#27290=EDGE_LOOP('',(#66649,#66650,#66651,#66652));
#27291=EDGE_LOOP('',(#66653,#66654,#66655,#66656));
#27292=EDGE_LOOP('',(#66657,#66658,#66659,#66660));
#27293=EDGE_LOOP('',(#66661,#66662,#66663,#66664));
#27294=EDGE_LOOP('',(#66665,#66666,#66667,#66668));
#27295=EDGE_LOOP('',(#66669,#66670,#66671,#66672));
#27296=EDGE_LOOP('',(#66673,#66674,#66675,#66676));
#27297=EDGE_LOOP('',(#66677,#66678,#66679,#66680));
#27298=EDGE_LOOP('',(#66681,#66682,#66683,#66684));
#27299=EDGE_LOOP('',(#66685,#66686,#66687,#66688));
#27300=EDGE_LOOP('',(#66689,#66690,#66691,#66692));
#27301=EDGE_LOOP('',(#66693,#66694,#66695,#66696));
#27302=EDGE_LOOP('',(#66697,#66698,#66699,#66700));
#27303=EDGE_LOOP('',(#66701,#66702,#66703,#66704));
#27304=EDGE_LOOP('',(#66705,#66706,#66707,#66708));
#27305=EDGE_LOOP('',(#66709,#66710,#66711,#66712));
#27306=EDGE_LOOP('',(#66713,#66714,#66715,#66716));
#27307=EDGE_LOOP('',(#66717,#66718,#66719,#66720));
#27308=EDGE_LOOP('',(#66721,#66722,#66723,#66724));
#27309=EDGE_LOOP('',(#66725,#66726,#66727,#66728));
#27310=EDGE_LOOP('',(#66729,#66730,#66731,#66732));
#27311=EDGE_LOOP('',(#66733,#66734,#66735,#66736));
#27312=EDGE_LOOP('',(#66737,#66738,#66739,#66740));
#27313=EDGE_LOOP('',(#66741,#66742,#66743,#66744));
#27314=EDGE_LOOP('',(#66745,#66746,#66747,#66748));
#27315=EDGE_LOOP('',(#66749,#66750,#66751,#66752));
#27316=EDGE_LOOP('',(#66753,#66754,#66755,#66756));
#27317=EDGE_LOOP('',(#66757,#66758,#66759,#66760));
#27318=EDGE_LOOP('',(#66761,#66762,#66763,#66764));
#27319=EDGE_LOOP('',(#66765,#66766,#66767,#66768));
#27320=EDGE_LOOP('',(#66769,#66770,#66771,#66772));
#27321=EDGE_LOOP('',(#66773,#66774,#66775,#66776));
#27322=EDGE_LOOP('',(#66777,#66778,#66779,#66780));
#27323=EDGE_LOOP('',(#66781,#66782,#66783,#66784));
#27324=EDGE_LOOP('',(#66785,#66786,#66787,#66788));
#27325=EDGE_LOOP('',(#66789,#66790,#66791,#66792));
#27326=EDGE_LOOP('',(#66793,#66794,#66795,#66796));
#27327=EDGE_LOOP('',(#66797,#66798,#66799,#66800));
#27328=EDGE_LOOP('',(#66801,#66802,#66803,#66804));
#27329=EDGE_LOOP('',(#66805,#66806,#66807,#66808));
#27330=EDGE_LOOP('',(#66809,#66810,#66811,#66812));
#27331=EDGE_LOOP('',(#66813,#66814,#66815,#66816));
#27332=EDGE_LOOP('',(#66817,#66818,#66819,#66820));
#27333=EDGE_LOOP('',(#66821,#66822,#66823,#66824));
#27334=EDGE_LOOP('',(#66825,#66826,#66827,#66828));
#27335=EDGE_LOOP('',(#66829,#66830,#66831,#66832));
#27336=EDGE_LOOP('',(#66833,#66834,#66835,#66836));
#27337=EDGE_LOOP('',(#66837,#66838,#66839,#66840));
#27338=EDGE_LOOP('',(#66841,#66842,#66843,#66844));
#27339=EDGE_LOOP('',(#66845,#66846,#66847,#66848));
#27340=EDGE_LOOP('',(#66849,#66850,#66851,#66852));
#27341=EDGE_LOOP('',(#66853,#66854,#66855,#66856));
#27342=EDGE_LOOP('',(#66857,#66858,#66859,#66860));
#27343=EDGE_LOOP('',(#66861,#66862,#66863,#66864));
#27344=EDGE_LOOP('',(#66865,#66866,#66867,#66868));
#27345=EDGE_LOOP('',(#66869,#66870,#66871,#66872));
#27346=EDGE_LOOP('',(#66873,#66874,#66875,#66876));
#27347=EDGE_LOOP('',(#66877,#66878,#66879,#66880));
#27348=EDGE_LOOP('',(#66881,#66882,#66883,#66884));
#27349=EDGE_LOOP('',(#66885,#66886,#66887,#66888));
#27350=EDGE_LOOP('',(#66889,#66890,#66891,#66892));
#27351=EDGE_LOOP('',(#66893,#66894,#66895,#66896));
#27352=EDGE_LOOP('',(#66897,#66898,#66899,#66900));
#27353=EDGE_LOOP('',(#66901,#66902,#66903,#66904));
#27354=EDGE_LOOP('',(#66905,#66906,#66907,#66908));
#27355=EDGE_LOOP('',(#66909,#66910,#66911,#66912));
#27356=EDGE_LOOP('',(#66913,#66914,#66915,#66916));
#27357=EDGE_LOOP('',(#66917,#66918,#66919,#66920));
#27358=EDGE_LOOP('',(#66921,#66922,#66923,#66924));
#27359=EDGE_LOOP('',(#66925,#66926,#66927,#66928));
#27360=EDGE_LOOP('',(#66929,#66930,#66931,#66932));
#27361=EDGE_LOOP('',(#66933,#66934,#66935,#66936));
#27362=EDGE_LOOP('',(#66937,#66938,#66939,#66940));
#27363=EDGE_LOOP('',(#66941,#66942,#66943,#66944));
#27364=EDGE_LOOP('',(#66945,#66946,#66947,#66948));
#27365=EDGE_LOOP('',(#66949,#66950,#66951,#66952));
#27366=EDGE_LOOP('',(#66953,#66954,#66955,#66956));
#27367=EDGE_LOOP('',(#66957,#66958,#66959,#66960));
#27368=EDGE_LOOP('',(#66961,#66962,#66963,#66964));
#27369=EDGE_LOOP('',(#66965,#66966,#66967,#66968));
#27370=EDGE_LOOP('',(#66969,#66970,#66971,#66972));
#27371=EDGE_LOOP('',(#66973,#66974,#66975,#66976));
#27372=EDGE_LOOP('',(#66977,#66978,#66979,#66980));
#27373=EDGE_LOOP('',(#66981,#66982,#66983,#66984));
#27374=EDGE_LOOP('',(#66985,#66986,#66987,#66988));
#27375=EDGE_LOOP('',(#66989,#66990,#66991,#66992));
#27376=EDGE_LOOP('',(#66993,#66994,#66995,#66996));
#27377=EDGE_LOOP('',(#66997,#66998,#66999,#67000));
#27378=EDGE_LOOP('',(#67001,#67002,#67003,#67004));
#27379=EDGE_LOOP('',(#67005,#67006,#67007,#67008));
#27380=EDGE_LOOP('',(#67009,#67010,#67011,#67012));
#27381=EDGE_LOOP('',(#67013,#67014,#67015,#67016));
#27382=EDGE_LOOP('',(#67017,#67018,#67019,#67020));
#27383=EDGE_LOOP('',(#67021,#67022,#67023,#67024));
#27384=EDGE_LOOP('',(#67025,#67026,#67027,#67028));
#27385=EDGE_LOOP('',(#67029,#67030,#67031,#67032));
#27386=EDGE_LOOP('',(#67033,#67034,#67035,#67036));
#27387=EDGE_LOOP('',(#67037,#67038,#67039,#67040));
#27388=EDGE_LOOP('',(#67041,#67042,#67043,#67044));
#27389=EDGE_LOOP('',(#67045,#67046,#67047,#67048));
#27390=EDGE_LOOP('',(#67049,#67050,#67051,#67052));
#27391=EDGE_LOOP('',(#67053,#67054,#67055,#67056));
#27392=EDGE_LOOP('',(#67057,#67058,#67059,#67060));
#27393=EDGE_LOOP('',(#67061,#67062,#67063,#67064));
#27394=EDGE_LOOP('',(#67065,#67066,#67067,#67068));
#27395=EDGE_LOOP('',(#67069,#67070,#67071,#67072));
#27396=EDGE_LOOP('',(#67073,#67074,#67075,#67076));
#27397=EDGE_LOOP('',(#67077,#67078,#67079,#67080));
#27398=EDGE_LOOP('',(#67081,#67082,#67083,#67084));
#27399=EDGE_LOOP('',(#67085,#67086,#67087,#67088));
#27400=EDGE_LOOP('',(#67089,#67090,#67091,#67092));
#27401=EDGE_LOOP('',(#67093,#67094,#67095,#67096));
#27402=EDGE_LOOP('',(#67097,#67098,#67099,#67100));
#27403=EDGE_LOOP('',(#67101,#67102,#67103,#67104));
#27404=EDGE_LOOP('',(#67105,#67106,#67107,#67108));
#27405=EDGE_LOOP('',(#67109,#67110,#67111,#67112));
#27406=EDGE_LOOP('',(#67113,#67114,#67115,#67116));
#27407=EDGE_LOOP('',(#67117,#67118,#67119,#67120));
#27408=EDGE_LOOP('',(#67121,#67122,#67123,#67124));
#27409=EDGE_LOOP('',(#67125,#67126,#67127,#67128));
#27410=EDGE_LOOP('',(#67129,#67130,#67131,#67132));
#27411=EDGE_LOOP('',(#67133,#67134,#67135,#67136));
#27412=EDGE_LOOP('',(#67137,#67138,#67139,#67140));
#27413=EDGE_LOOP('',(#67141,#67142,#67143,#67144));
#27414=EDGE_LOOP('',(#67145,#67146,#67147,#67148));
#27415=EDGE_LOOP('',(#67149,#67150,#67151,#67152));
#27416=EDGE_LOOP('',(#67153,#67154,#67155,#67156));
#27417=EDGE_LOOP('',(#67157,#67158,#67159,#67160));
#27418=EDGE_LOOP('',(#67161,#67162,#67163,#67164));
#27419=EDGE_LOOP('',(#67165,#67166,#67167,#67168));
#27420=EDGE_LOOP('',(#67169,#67170,#67171,#67172));
#27421=EDGE_LOOP('',(#67173,#67174,#67175,#67176));
#27422=EDGE_LOOP('',(#67177,#67178,#67179,#67180));
#27423=EDGE_LOOP('',(#67181,#67182,#67183,#67184));
#27424=EDGE_LOOP('',(#67185,#67186,#67187,#67188));
#27425=EDGE_LOOP('',(#67189,#67190,#67191,#67192));
#27426=EDGE_LOOP('',(#67193,#67194,#67195,#67196));
#27427=EDGE_LOOP('',(#67197,#67198,#67199,#67200));
#27428=EDGE_LOOP('',(#67201,#67202,#67203,#67204));
#27429=EDGE_LOOP('',(#67205,#67206,#67207,#67208));
#27430=EDGE_LOOP('',(#67209,#67210,#67211,#67212));
#27431=EDGE_LOOP('',(#67213,#67214,#67215,#67216));
#27432=EDGE_LOOP('',(#67217,#67218,#67219,#67220));
#27433=EDGE_LOOP('',(#67221,#67222,#67223,#67224));
#27434=EDGE_LOOP('',(#67225,#67226,#67227,#67228));
#27435=EDGE_LOOP('',(#67229,#67230,#67231,#67232));
#27436=EDGE_LOOP('',(#67233,#67234,#67235,#67236));
#27437=EDGE_LOOP('',(#67237,#67238,#67239,#67240));
#27438=EDGE_LOOP('',(#67241,#67242,#67243,#67244));
#27439=EDGE_LOOP('',(#67245,#67246,#67247,#67248));
#27440=EDGE_LOOP('',(#67249,#67250,#67251,#67252));
#27441=EDGE_LOOP('',(#67253,#67254,#67255,#67256));
#27442=EDGE_LOOP('',(#67257,#67258,#67259,#67260));
#27443=EDGE_LOOP('',(#67261,#67262,#67263,#67264));
#27444=EDGE_LOOP('',(#67265,#67266,#67267,#67268));
#27445=EDGE_LOOP('',(#67269,#67270,#67271,#67272));
#27446=EDGE_LOOP('',(#67273,#67274,#67275,#67276));
#27447=EDGE_LOOP('',(#67277,#67278,#67279,#67280));
#27448=EDGE_LOOP('',(#67281,#67282,#67283,#67284));
#27449=EDGE_LOOP('',(#67285,#67286,#67287,#67288));
#27450=EDGE_LOOP('',(#67289,#67290,#67291,#67292));
#27451=EDGE_LOOP('',(#67293,#67294,#67295,#67296));
#27452=EDGE_LOOP('',(#67297,#67298,#67299,#67300));
#27453=EDGE_LOOP('',(#67301,#67302,#67303,#67304));
#27454=EDGE_LOOP('',(#67305,#67306,#67307,#67308));
#27455=EDGE_LOOP('',(#67309,#67310,#67311,#67312));
#27456=EDGE_LOOP('',(#67313,#67314,#67315,#67316));
#27457=EDGE_LOOP('',(#67317,#67318,#67319,#67320));
#27458=EDGE_LOOP('',(#67321,#67322,#67323,#67324));
#27459=EDGE_LOOP('',(#67325,#67326,#67327,#67328));
#27460=EDGE_LOOP('',(#67329,#67330,#67331,#67332));
#27461=EDGE_LOOP('',(#67333,#67334,#67335,#67336));
#27462=EDGE_LOOP('',(#67337,#67338,#67339,#67340));
#27463=EDGE_LOOP('',(#67341,#67342,#67343,#67344));
#27464=EDGE_LOOP('',(#67345,#67346,#67347,#67348));
#27465=EDGE_LOOP('',(#67349,#67350,#67351,#67352));
#27466=EDGE_LOOP('',(#67353,#67354,#67355,#67356));
#27467=EDGE_LOOP('',(#67357,#67358,#67359,#67360));
#27468=EDGE_LOOP('',(#67361,#67362,#67363,#67364));
#27469=EDGE_LOOP('',(#67365,#67366,#67367,#67368));
#27470=EDGE_LOOP('',(#67369,#67370,#67371,#67372));
#27471=EDGE_LOOP('',(#67373,#67374,#67375,#67376));
#27472=EDGE_LOOP('',(#67377,#67378,#67379,#67380));
#27473=EDGE_LOOP('',(#67381,#67382,#67383,#67384));
#27474=EDGE_LOOP('',(#67385,#67386,#67387,#67388));
#27475=EDGE_LOOP('',(#67389,#67390,#67391,#67392));
#27476=EDGE_LOOP('',(#67393,#67394,#67395,#67396));
#27477=EDGE_LOOP('',(#67397,#67398,#67399,#67400));
#27478=EDGE_LOOP('',(#67401,#67402,#67403,#67404));
#27479=EDGE_LOOP('',(#67405,#67406,#67407,#67408));
#27480=EDGE_LOOP('',(#67409,#67410,#67411,#67412));
#27481=EDGE_LOOP('',(#67413,#67414,#67415,#67416));
#27482=EDGE_LOOP('',(#67417,#67418,#67419,#67420));
#27483=EDGE_LOOP('',(#67421,#67422,#67423,#67424));
#27484=EDGE_LOOP('',(#67425,#67426,#67427,#67428));
#27485=EDGE_LOOP('',(#67429,#67430,#67431,#67432));
#27486=EDGE_LOOP('',(#67433,#67434,#67435,#67436));
#27487=EDGE_LOOP('',(#67437,#67438,#67439,#67440));
#27488=EDGE_LOOP('',(#67441,#67442,#67443,#67444));
#27489=EDGE_LOOP('',(#67445,#67446,#67447,#67448));
#27490=EDGE_LOOP('',(#67449,#67450,#67451,#67452));
#27491=EDGE_LOOP('',(#67453,#67454,#67455,#67456));
#27492=EDGE_LOOP('',(#67457,#67458,#67459,#67460));
#27493=EDGE_LOOP('',(#67461,#67462,#67463,#67464));
#27494=EDGE_LOOP('',(#67465,#67466,#67467,#67468));
#27495=EDGE_LOOP('',(#67469,#67470,#67471,#67472));
#27496=EDGE_LOOP('',(#67473,#67474,#67475,#67476));
#27497=EDGE_LOOP('',(#67477,#67478,#67479,#67480));
#27498=EDGE_LOOP('',(#67481,#67482,#67483,#67484));
#27499=EDGE_LOOP('',(#67485,#67486,#67487,#67488));
#27500=EDGE_LOOP('',(#67489,#67490,#67491,#67492));
#27501=EDGE_LOOP('',(#67493,#67494,#67495,#67496));
#27502=EDGE_LOOP('',(#67497,#67498,#67499,#67500));
#27503=EDGE_LOOP('',(#67501,#67502,#67503,#67504));
#27504=EDGE_LOOP('',(#67505,#67506,#67507,#67508));
#27505=EDGE_LOOP('',(#67509,#67510,#67511,#67512));
#27506=EDGE_LOOP('',(#67513,#67514,#67515,#67516));
#27507=EDGE_LOOP('',(#67517,#67518,#67519,#67520));
#27508=EDGE_LOOP('',(#67521,#67522,#67523,#67524));
#27509=EDGE_LOOP('',(#67525,#67526,#67527,#67528));
#27510=EDGE_LOOP('',(#67529,#67530,#67531,#67532));
#27511=EDGE_LOOP('',(#67533,#67534,#67535,#67536));
#27512=EDGE_LOOP('',(#67537,#67538,#67539,#67540));
#27513=EDGE_LOOP('',(#67541,#67542,#67543,#67544));
#27514=EDGE_LOOP('',(#67545,#67546,#67547,#67548));
#27515=EDGE_LOOP('',(#67549,#67550,#67551,#67552));
#27516=EDGE_LOOP('',(#67553,#67554,#67555,#67556));
#27517=EDGE_LOOP('',(#67557,#67558,#67559,#67560));
#27518=EDGE_LOOP('',(#67561,#67562,#67563,#67564));
#27519=EDGE_LOOP('',(#67565,#67566,#67567,#67568));
#27520=EDGE_LOOP('',(#67569,#67570,#67571,#67572));
#27521=EDGE_LOOP('',(#67573,#67574,#67575,#67576));
#27522=EDGE_LOOP('',(#67577,#67578,#67579,#67580));
#27523=EDGE_LOOP('',(#67581,#67582,#67583,#67584));
#27524=EDGE_LOOP('',(#67585,#67586,#67587,#67588));
#27525=EDGE_LOOP('',(#67589,#67590,#67591,#67592));
#27526=EDGE_LOOP('',(#67593,#67594,#67595,#67596));
#27527=EDGE_LOOP('',(#67597,#67598,#67599,#67600));
#27528=EDGE_LOOP('',(#67601,#67602,#67603,#67604));
#27529=EDGE_LOOP('',(#67605,#67606,#67607,#67608));
#27530=EDGE_LOOP('',(#67609,#67610,#67611,#67612));
#27531=EDGE_LOOP('',(#67613,#67614,#67615,#67616));
#27532=EDGE_LOOP('',(#67617,#67618,#67619,#67620));
#27533=EDGE_LOOP('',(#67621,#67622,#67623,#67624));
#27534=EDGE_LOOP('',(#67625,#67626,#67627,#67628));
#27535=EDGE_LOOP('',(#67629,#67630,#67631,#67632));
#27536=EDGE_LOOP('',(#67633,#67634,#67635,#67636));
#27537=EDGE_LOOP('',(#67637,#67638,#67639,#67640));
#27538=EDGE_LOOP('',(#67641,#67642,#67643,#67644));
#27539=EDGE_LOOP('',(#67645,#67646,#67647,#67648));
#27540=EDGE_LOOP('',(#67649,#67650,#67651,#67652));
#27541=EDGE_LOOP('',(#67653,#67654,#67655,#67656));
#27542=EDGE_LOOP('',(#67657,#67658,#67659,#67660));
#27543=EDGE_LOOP('',(#67661,#67662,#67663,#67664));
#27544=EDGE_LOOP('',(#67665,#67666,#67667,#67668));
#27545=EDGE_LOOP('',(#67669,#67670,#67671,#67672));
#27546=EDGE_LOOP('',(#67673,#67674,#67675,#67676));
#27547=EDGE_LOOP('',(#67677,#67678,#67679,#67680));
#27548=EDGE_LOOP('',(#67681,#67682,#67683,#67684));
#27549=EDGE_LOOP('',(#67685,#67686,#67687,#67688));
#27550=EDGE_LOOP('',(#67689,#67690,#67691,#67692));
#27551=EDGE_LOOP('',(#67693,#67694,#67695,#67696));
#27552=EDGE_LOOP('',(#67697,#67698,#67699,#67700));
#27553=EDGE_LOOP('',(#67701,#67702,#67703,#67704));
#27554=EDGE_LOOP('',(#67705,#67706,#67707,#67708));
#27555=EDGE_LOOP('',(#67709,#67710,#67711,#67712));
#27556=EDGE_LOOP('',(#67713,#67714,#67715,#67716));
#27557=EDGE_LOOP('',(#67717,#67718,#67719,#67720));
#27558=EDGE_LOOP('',(#67721,#67722,#67723,#67724));
#27559=EDGE_LOOP('',(#67725,#67726,#67727,#67728));
#27560=EDGE_LOOP('',(#67729,#67730,#67731,#67732));
#27561=EDGE_LOOP('',(#67733,#67734,#67735,#67736));
#27562=EDGE_LOOP('',(#67737,#67738,#67739,#67740));
#27563=EDGE_LOOP('',(#67741,#67742,#67743,#67744));
#27564=EDGE_LOOP('',(#67745,#67746,#67747,#67748));
#27565=EDGE_LOOP('',(#67749,#67750,#67751,#67752));
#27566=EDGE_LOOP('',(#67753,#67754,#67755,#67756));
#27567=EDGE_LOOP('',(#67757,#67758,#67759,#67760));
#27568=EDGE_LOOP('',(#67761,#67762,#67763,#67764));
#27569=EDGE_LOOP('',(#67765,#67766,#67767,#67768));
#27570=EDGE_LOOP('',(#67769,#67770,#67771,#67772));
#27571=EDGE_LOOP('',(#67773,#67774,#67775,#67776));
#27572=EDGE_LOOP('',(#67777,#67778,#67779,#67780));
#27573=EDGE_LOOP('',(#67781,#67782,#67783,#67784));
#27574=EDGE_LOOP('',(#67785,#67786,#67787,#67788));
#27575=EDGE_LOOP('',(#67789,#67790,#67791,#67792));
#27576=EDGE_LOOP('',(#67793,#67794,#67795,#67796));
#27577=EDGE_LOOP('',(#67797,#67798,#67799,#67800));
#27578=EDGE_LOOP('',(#67801,#67802,#67803,#67804));
#27579=EDGE_LOOP('',(#67805,#67806,#67807,#67808));
#27580=EDGE_LOOP('',(#67809,#67810,#67811,#67812));
#27581=EDGE_LOOP('',(#67813,#67814,#67815,#67816));
#27582=EDGE_LOOP('',(#67817,#67818,#67819,#67820));
#27583=EDGE_LOOP('',(#67821,#67822,#67823,#67824));
#27584=EDGE_LOOP('',(#67825,#67826,#67827,#67828));
#27585=EDGE_LOOP('',(#67829,#67830,#67831,#67832));
#27586=EDGE_LOOP('',(#67833,#67834,#67835,#67836));
#27587=EDGE_LOOP('',(#67837,#67838,#67839,#67840));
#27588=EDGE_LOOP('',(#67841,#67842,#67843,#67844));
#27589=EDGE_LOOP('',(#67845,#67846,#67847,#67848));
#27590=EDGE_LOOP('',(#67849,#67850,#67851,#67852));
#27591=EDGE_LOOP('',(#67853,#67854,#67855,#67856));
#27592=EDGE_LOOP('',(#67857,#67858,#67859,#67860));
#27593=EDGE_LOOP('',(#67861,#67862,#67863,#67864));
#27594=EDGE_LOOP('',(#67865,#67866,#67867,#67868));
#27595=EDGE_LOOP('',(#67869,#67870,#67871,#67872));
#27596=EDGE_LOOP('',(#67873,#67874,#67875,#67876));
#27597=EDGE_LOOP('',(#67877,#67878,#67879,#67880));
#27598=EDGE_LOOP('',(#67881,#67882,#67883,#67884));
#27599=EDGE_LOOP('',(#67885,#67886,#67887,#67888));
#27600=EDGE_LOOP('',(#67889,#67890,#67891,#67892));
#27601=EDGE_LOOP('',(#67893,#67894,#67895,#67896));
#27602=EDGE_LOOP('',(#67897,#67898,#67899,#67900));
#27603=EDGE_LOOP('',(#67901,#67902,#67903,#67904));
#27604=EDGE_LOOP('',(#67905,#67906,#67907,#67908));
#27605=EDGE_LOOP('',(#67909,#67910,#67911,#67912));
#27606=EDGE_LOOP('',(#67913,#67914,#67915,#67916));
#27607=EDGE_LOOP('',(#67917,#67918,#67919,#67920));
#27608=EDGE_LOOP('',(#67921,#67922,#67923,#67924));
#27609=EDGE_LOOP('',(#67925,#67926,#67927,#67928));
#27610=EDGE_LOOP('',(#67929,#67930,#67931,#67932));
#27611=EDGE_LOOP('',(#67933,#67934,#67935,#67936));
#27612=EDGE_LOOP('',(#67937,#67938,#67939,#67940));
#27613=EDGE_LOOP('',(#67941,#67942,#67943,#67944));
#27614=EDGE_LOOP('',(#67945,#67946,#67947,#67948));
#27615=EDGE_LOOP('',(#67949,#67950,#67951,#67952));
#27616=EDGE_LOOP('',(#67953,#67954,#67955,#67956));
#27617=EDGE_LOOP('',(#67957,#67958,#67959,#67960));
#27618=EDGE_LOOP('',(#67961,#67962,#67963,#67964));
#27619=EDGE_LOOP('',(#67965,#67966,#67967,#67968));
#27620=EDGE_LOOP('',(#67969,#67970,#67971,#67972));
#27621=EDGE_LOOP('',(#67973,#67974,#67975,#67976));
#27622=EDGE_LOOP('',(#67977,#67978,#67979,#67980));
#27623=EDGE_LOOP('',(#67981,#67982,#67983,#67984));
#27624=EDGE_LOOP('',(#67985,#67986,#67987,#67988));
#27625=EDGE_LOOP('',(#67989,#67990,#67991,#67992));
#27626=EDGE_LOOP('',(#67993,#67994,#67995,#67996));
#27627=EDGE_LOOP('',(#67997,#67998,#67999,#68000));
#27628=EDGE_LOOP('',(#68001,#68002,#68003,#68004));
#27629=EDGE_LOOP('',(#68005,#68006,#68007,#68008));
#27630=EDGE_LOOP('',(#68009,#68010,#68011,#68012));
#27631=EDGE_LOOP('',(#68013,#68014,#68015,#68016));
#27632=EDGE_LOOP('',(#68017,#68018,#68019,#68020));
#27633=EDGE_LOOP('',(#68021,#68022,#68023,#68024));
#27634=EDGE_LOOP('',(#68025,#68026,#68027,#68028));
#27635=EDGE_LOOP('',(#68029,#68030,#68031,#68032));
#27636=EDGE_LOOP('',(#68033,#68034,#68035,#68036));
#27637=EDGE_LOOP('',(#68037,#68038,#68039,#68040));
#27638=EDGE_LOOP('',(#68041,#68042,#68043,#68044));
#27639=EDGE_LOOP('',(#68045,#68046,#68047,#68048));
#27640=EDGE_LOOP('',(#68049,#68050,#68051,#68052));
#27641=EDGE_LOOP('',(#68053,#68054,#68055,#68056));
#27642=EDGE_LOOP('',(#68057,#68058,#68059,#68060));
#27643=EDGE_LOOP('',(#68061,#68062,#68063,#68064));
#27644=EDGE_LOOP('',(#68065,#68066,#68067,#68068));
#27645=EDGE_LOOP('',(#68069,#68070,#68071,#68072));
#27646=EDGE_LOOP('',(#68073,#68074,#68075,#68076));
#27647=EDGE_LOOP('',(#68077,#68078,#68079,#68080));
#27648=EDGE_LOOP('',(#68081,#68082,#68083,#68084));
#27649=EDGE_LOOP('',(#68085,#68086,#68087,#68088));
#27650=EDGE_LOOP('',(#68089,#68090,#68091,#68092));
#27651=EDGE_LOOP('',(#68093,#68094,#68095,#68096));
#27652=EDGE_LOOP('',(#68097,#68098,#68099,#68100));
#27653=EDGE_LOOP('',(#68101,#68102,#68103,#68104));
#27654=EDGE_LOOP('',(#68105,#68106,#68107,#68108));
#27655=EDGE_LOOP('',(#68109,#68110,#68111,#68112));
#27656=EDGE_LOOP('',(#68113,#68114,#68115,#68116));
#27657=EDGE_LOOP('',(#68117,#68118,#68119,#68120));
#27658=EDGE_LOOP('',(#68121,#68122,#68123,#68124));
#27659=EDGE_LOOP('',(#68125,#68126,#68127,#68128));
#27660=EDGE_LOOP('',(#68129,#68130,#68131,#68132));
#27661=EDGE_LOOP('',(#68133,#68134,#68135,#68136));
#27662=EDGE_LOOP('',(#68137,#68138,#68139,#68140));
#27663=EDGE_LOOP('',(#68141,#68142,#68143,#68144));
#27664=EDGE_LOOP('',(#68145,#68146,#68147,#68148));
#27665=EDGE_LOOP('',(#68149,#68150,#68151,#68152));
#27666=EDGE_LOOP('',(#68153,#68154,#68155,#68156));
#27667=EDGE_LOOP('',(#68157,#68158,#68159,#68160));
#27668=EDGE_LOOP('',(#68161,#68162,#68163,#68164));
#27669=EDGE_LOOP('',(#68165,#68166,#68167,#68168));
#27670=EDGE_LOOP('',(#68169,#68170,#68171,#68172));
#27671=EDGE_LOOP('',(#68173,#68174,#68175,#68176));
#27672=EDGE_LOOP('',(#68177,#68178,#68179,#68180));
#27673=EDGE_LOOP('',(#68181,#68182,#68183,#68184));
#27674=EDGE_LOOP('',(#68185,#68186,#68187,#68188));
#27675=EDGE_LOOP('',(#68189,#68190,#68191,#68192));
#27676=EDGE_LOOP('',(#68193,#68194,#68195,#68196));
#27677=EDGE_LOOP('',(#68197,#68198,#68199,#68200));
#27678=EDGE_LOOP('',(#68201,#68202,#68203,#68204));
#27679=EDGE_LOOP('',(#68205,#68206,#68207,#68208));
#27680=EDGE_LOOP('',(#68209,#68210,#68211,#68212));
#27681=EDGE_LOOP('',(#68213,#68214,#68215,#68216));
#27682=EDGE_LOOP('',(#68217,#68218,#68219,#68220));
#27683=EDGE_LOOP('',(#68221,#68222,#68223,#68224));
#27684=EDGE_LOOP('',(#68225,#68226,#68227,#68228));
#27685=EDGE_LOOP('',(#68229,#68230,#68231,#68232));
#27686=EDGE_LOOP('',(#68233,#68234,#68235,#68236));
#27687=EDGE_LOOP('',(#68237,#68238,#68239,#68240));
#27688=EDGE_LOOP('',(#68241,#68242,#68243,#68244));
#27689=EDGE_LOOP('',(#68245,#68246,#68247,#68248));
#27690=EDGE_LOOP('',(#68249,#68250,#68251,#68252));
#27691=EDGE_LOOP('',(#68253,#68254,#68255,#68256));
#27692=EDGE_LOOP('',(#68257,#68258,#68259,#68260));
#27693=EDGE_LOOP('',(#68261,#68262,#68263,#68264));
#27694=EDGE_LOOP('',(#68265,#68266,#68267,#68268));
#27695=EDGE_LOOP('',(#68269,#68270,#68271,#68272));
#27696=EDGE_LOOP('',(#68273,#68274,#68275,#68276));
#27697=EDGE_LOOP('',(#68277,#68278,#68279,#68280));
#27698=EDGE_LOOP('',(#68281,#68282,#68283,#68284));
#27699=EDGE_LOOP('',(#68285,#68286,#68287,#68288));
#27700=EDGE_LOOP('',(#68289,#68290,#68291,#68292));
#27701=EDGE_LOOP('',(#68293,#68294,#68295,#68296));
#27702=EDGE_LOOP('',(#68297,#68298,#68299,#68300));
#27703=EDGE_LOOP('',(#68301,#68302,#68303,#68304));
#27704=EDGE_LOOP('',(#68305,#68306,#68307,#68308));
#27705=EDGE_LOOP('',(#68309,#68310,#68311,#68312));
#27706=EDGE_LOOP('',(#68313,#68314,#68315,#68316));
#27707=EDGE_LOOP('',(#68317,#68318,#68319,#68320));
#27708=EDGE_LOOP('',(#68321,#68322,#68323,#68324));
#27709=EDGE_LOOP('',(#68325,#68326,#68327,#68328));
#27710=EDGE_LOOP('',(#68329,#68330,#68331,#68332));
#27711=EDGE_LOOP('',(#68333,#68334,#68335,#68336));
#27712=EDGE_LOOP('',(#68337,#68338,#68339,#68340));
#27713=EDGE_LOOP('',(#68341,#68342,#68343,#68344));
#27714=EDGE_LOOP('',(#68345,#68346,#68347,#68348));
#27715=EDGE_LOOP('',(#68349,#68350,#68351,#68352));
#27716=EDGE_LOOP('',(#68353,#68354,#68355,#68356));
#27717=EDGE_LOOP('',(#68357,#68358,#68359,#68360));
#27718=EDGE_LOOP('',(#68361,#68362,#68363,#68364));
#27719=EDGE_LOOP('',(#68365,#68366,#68367,#68368));
#27720=EDGE_LOOP('',(#68369,#68370,#68371,#68372));
#27721=EDGE_LOOP('',(#68373,#68374,#68375,#68376));
#27722=EDGE_LOOP('',(#68377,#68378,#68379,#68380));
#27723=EDGE_LOOP('',(#68381,#68382,#68383,#68384));
#27724=EDGE_LOOP('',(#68385,#68386,#68387,#68388));
#27725=EDGE_LOOP('',(#68389,#68390,#68391,#68392));
#27726=EDGE_LOOP('',(#68393,#68394,#68395,#68396));
#27727=EDGE_LOOP('',(#68397,#68398,#68399,#68400));
#27728=EDGE_LOOP('',(#68401,#68402,#68403,#68404));
#27729=EDGE_LOOP('',(#68405,#68406,#68407,#68408));
#27730=EDGE_LOOP('',(#68409,#68410,#68411,#68412));
#27731=EDGE_LOOP('',(#68413,#68414,#68415,#68416));
#27732=EDGE_LOOP('',(#68417,#68418,#68419,#68420));
#27733=EDGE_LOOP('',(#68421,#68422,#68423,#68424));
#27734=EDGE_LOOP('',(#68425,#68426,#68427,#68428));
#27735=EDGE_LOOP('',(#68429,#68430,#68431,#68432));
#27736=EDGE_LOOP('',(#68433,#68434,#68435,#68436));
#27737=EDGE_LOOP('',(#68437,#68438,#68439,#68440));
#27738=EDGE_LOOP('',(#68441,#68442,#68443,#68444));
#27739=EDGE_LOOP('',(#68445,#68446,#68447,#68448));
#27740=EDGE_LOOP('',(#68449,#68450,#68451,#68452));
#27741=EDGE_LOOP('',(#68453,#68454,#68455,#68456));
#27742=EDGE_LOOP('',(#68457,#68458,#68459,#68460));
#27743=EDGE_LOOP('',(#68461,#68462,#68463,#68464));
#27744=EDGE_LOOP('',(#68465,#68466,#68467,#68468));
#27745=EDGE_LOOP('',(#68469,#68470,#68471,#68472));
#27746=EDGE_LOOP('',(#68473,#68474,#68475,#68476));
#27747=EDGE_LOOP('',(#68477,#68478,#68479,#68480));
#27748=EDGE_LOOP('',(#68481,#68482,#68483,#68484));
#27749=EDGE_LOOP('',(#68485,#68486,#68487,#68488));
#27750=EDGE_LOOP('',(#68489,#68490,#68491,#68492));
#27751=EDGE_LOOP('',(#68493,#68494,#68495,#68496));
#27752=EDGE_LOOP('',(#68497,#68498,#68499,#68500));
#27753=EDGE_LOOP('',(#68501,#68502,#68503,#68504));
#27754=EDGE_LOOP('',(#68505,#68506,#68507,#68508));
#27755=EDGE_LOOP('',(#68509,#68510,#68511,#68512));
#27756=EDGE_LOOP('',(#68513,#68514,#68515,#68516));
#27757=EDGE_LOOP('',(#68517,#68518,#68519,#68520));
#27758=EDGE_LOOP('',(#68521,#68522,#68523,#68524));
#27759=EDGE_LOOP('',(#68525,#68526,#68527,#68528));
#27760=EDGE_LOOP('',(#68529,#68530,#68531,#68532));
#27761=EDGE_LOOP('',(#68533,#68534,#68535,#68536));
#27762=EDGE_LOOP('',(#68537,#68538,#68539,#68540));
#27763=EDGE_LOOP('',(#68541,#68542,#68543,#68544));
#27764=EDGE_LOOP('',(#68545,#68546,#68547,#68548));
#27765=EDGE_LOOP('',(#68549,#68550,#68551,#68552));
#27766=EDGE_LOOP('',(#68553,#68554,#68555,#68556));
#27767=EDGE_LOOP('',(#68557,#68558,#68559,#68560));
#27768=EDGE_LOOP('',(#68561,#68562,#68563,#68564));
#27769=EDGE_LOOP('',(#68565,#68566,#68567,#68568));
#27770=EDGE_LOOP('',(#68569,#68570,#68571,#68572));
#27771=EDGE_LOOP('',(#68573,#68574,#68575,#68576));
#27772=EDGE_LOOP('',(#68577,#68578,#68579,#68580));
#27773=EDGE_LOOP('',(#68581,#68582,#68583,#68584));
#27774=EDGE_LOOP('',(#68585,#68586,#68587,#68588));
#27775=EDGE_LOOP('',(#68589,#68590,#68591,#68592));
#27776=EDGE_LOOP('',(#68593,#68594,#68595,#68596));
#27777=EDGE_LOOP('',(#68597,#68598,#68599,#68600));
#27778=EDGE_LOOP('',(#68601,#68602,#68603,#68604));
#27779=EDGE_LOOP('',(#68605,#68606,#68607,#68608));
#27780=EDGE_LOOP('',(#68609,#68610,#68611,#68612));
#27781=EDGE_LOOP('',(#68613,#68614,#68615,#68616));
#27782=EDGE_LOOP('',(#68617,#68618,#68619,#68620));
#27783=EDGE_LOOP('',(#68621,#68622,#68623,#68624));
#27784=EDGE_LOOP('',(#68625,#68626,#68627,#68628));
#27785=EDGE_LOOP('',(#68629,#68630,#68631,#68632));
#27786=EDGE_LOOP('',(#68633,#68634,#68635,#68636));
#27787=EDGE_LOOP('',(#68637,#68638,#68639,#68640));
#27788=EDGE_LOOP('',(#68641,#68642,#68643,#68644));
#27789=EDGE_LOOP('',(#68645,#68646,#68647,#68648));
#27790=EDGE_LOOP('',(#68649,#68650,#68651,#68652));
#27791=EDGE_LOOP('',(#68653,#68654,#68655,#68656));
#27792=EDGE_LOOP('',(#68657,#68658,#68659,#68660));
#27793=EDGE_LOOP('',(#68661,#68662,#68663,#68664));
#27794=EDGE_LOOP('',(#68665,#68666,#68667,#68668));
#27795=EDGE_LOOP('',(#68669,#68670,#68671,#68672));
#27796=EDGE_LOOP('',(#68673,#68674,#68675,#68676));
#27797=EDGE_LOOP('',(#68677,#68678,#68679,#68680));
#27798=EDGE_LOOP('',(#68681,#68682,#68683,#68684));
#27799=EDGE_LOOP('',(#68685,#68686,#68687,#68688));
#27800=EDGE_LOOP('',(#68689,#68690,#68691,#68692));
#27801=EDGE_LOOP('',(#68693));
#27802=EDGE_LOOP('',(#68694));
#27803=EDGE_LOOP('',(#68695));
#27804=EDGE_LOOP('',(#68696,#68697,#68698,#68699));
#27805=EDGE_LOOP('',(#68700,#68701,#68702,#68703));
#27806=EDGE_LOOP('',(#68704,#68705,#68706,#68707));
#27807=EDGE_LOOP('',(#68708,#68709,#68710,#68711));
#27808=EDGE_LOOP('',(#68712,#68713,#68714,#68715));
#27809=EDGE_LOOP('',(#68716,#68717,#68718,#68719));
#27810=EDGE_LOOP('',(#68720,#68721,#68722,#68723));
#27811=EDGE_LOOP('',(#68724,#68725,#68726,#68727));
#27812=EDGE_LOOP('',(#68728,#68729,#68730,#68731));
#27813=EDGE_LOOP('',(#68732,#68733,#68734,#68735));
#27814=EDGE_LOOP('',(#68736,#68737,#68738,#68739));
#27815=EDGE_LOOP('',(#68740,#68741,#68742,#68743));
#27816=EDGE_LOOP('',(#68744,#68745,#68746,#68747));
#27817=EDGE_LOOP('',(#68748,#68749,#68750,#68751));
#27818=EDGE_LOOP('',(#68752,#68753,#68754,#68755));
#27819=EDGE_LOOP('',(#68756,#68757,#68758,#68759));
#27820=EDGE_LOOP('',(#68760,#68761,#68762,#68763));
#27821=EDGE_LOOP('',(#68764,#68765,#68766,#68767));
#27822=EDGE_LOOP('',(#68768,#68769,#68770,#68771));
#27823=EDGE_LOOP('',(#68772,#68773,#68774,#68775));
#27824=EDGE_LOOP('',(#68776,#68777,#68778,#68779));
#27825=EDGE_LOOP('',(#68780,#68781,#68782,#68783));
#27826=EDGE_LOOP('',(#68784,#68785,#68786,#68787));
#27827=EDGE_LOOP('',(#68788,#68789,#68790,#68791));
#27828=EDGE_LOOP('',(#68792,#68793,#68794,#68795));
#27829=EDGE_LOOP('',(#68796,#68797,#68798,#68799));
#27830=EDGE_LOOP('',(#68800,#68801,#68802,#68803));
#27831=EDGE_LOOP('',(#68804,#68805,#68806,#68807));
#27832=EDGE_LOOP('',(#68808,#68809,#68810,#68811));
#27833=EDGE_LOOP('',(#68812,#68813,#68814,#68815));
#27834=EDGE_LOOP('',(#68816,#68817,#68818,#68819));
#27835=EDGE_LOOP('',(#68820,#68821,#68822,#68823));
#27836=EDGE_LOOP('',(#68824,#68825,#68826,#68827));
#27837=EDGE_LOOP('',(#68828,#68829,#68830,#68831));
#27838=EDGE_LOOP('',(#68832,#68833,#68834,#68835));
#27839=EDGE_LOOP('',(#68836,#68837,#68838,#68839));
#27840=EDGE_LOOP('',(#68840,#68841,#68842,#68843));
#27841=EDGE_LOOP('',(#68844,#68845,#68846,#68847));
#27842=EDGE_LOOP('',(#68848,#68849,#68850,#68851));
#27843=EDGE_LOOP('',(#68852,#68853,#68854,#68855));
#27844=EDGE_LOOP('',(#68856,#68857,#68858,#68859));
#27845=EDGE_LOOP('',(#68860,#68861,#68862,#68863));
#27846=EDGE_LOOP('',(#68864,#68865,#68866,#68867));
#27847=EDGE_LOOP('',(#68868,#68869,#68870,#68871));
#27848=EDGE_LOOP('',(#68872,#68873,#68874,#68875));
#27849=EDGE_LOOP('',(#68876,#68877,#68878,#68879));
#27850=EDGE_LOOP('',(#68880,#68881,#68882,#68883));
#27851=EDGE_LOOP('',(#68884,#68885,#68886,#68887));
#27852=EDGE_LOOP('',(#68888,#68889,#68890,#68891));
#27853=EDGE_LOOP('',(#68892,#68893,#68894,#68895));
#27854=EDGE_LOOP('',(#68896,#68897,#68898,#68899));
#27855=EDGE_LOOP('',(#68900,#68901,#68902,#68903));
#27856=EDGE_LOOP('',(#68904,#68905,#68906,#68907));
#27857=EDGE_LOOP('',(#68908,#68909,#68910,#68911));
#27858=EDGE_LOOP('',(#68912,#68913,#68914,#68915));
#27859=EDGE_LOOP('',(#68916,#68917,#68918,#68919));
#27860=EDGE_LOOP('',(#68920,#68921,#68922,#68923));
#27861=EDGE_LOOP('',(#68924,#68925,#68926,#68927));
#27862=EDGE_LOOP('',(#68928,#68929,#68930,#68931));
#27863=EDGE_LOOP('',(#68932,#68933,#68934,#68935));
#27864=EDGE_LOOP('',(#68936,#68937,#68938,#68939));
#27865=EDGE_LOOP('',(#68940,#68941,#68942,#68943));
#27866=EDGE_LOOP('',(#68944,#68945,#68946,#68947));
#27867=EDGE_LOOP('',(#68948,#68949,#68950,#68951));
#27868=EDGE_LOOP('',(#68952,#68953,#68954,#68955));
#27869=EDGE_LOOP('',(#68956,#68957,#68958,#68959));
#27870=EDGE_LOOP('',(#68960,#68961,#68962,#68963));
#27871=EDGE_LOOP('',(#68964,#68965,#68966,#68967));
#27872=EDGE_LOOP('',(#68968,#68969,#68970,#68971));
#27873=EDGE_LOOP('',(#68972,#68973,#68974,#68975));
#27874=EDGE_LOOP('',(#68976,#68977,#68978,#68979));
#27875=EDGE_LOOP('',(#68980,#68981,#68982,#68983));
#27876=EDGE_LOOP('',(#68984,#68985,#68986,#68987));
#27877=EDGE_LOOP('',(#68988,#68989,#68990,#68991));
#27878=EDGE_LOOP('',(#68992,#68993,#68994,#68995));
#27879=EDGE_LOOP('',(#68996,#68997,#68998,#68999));
#27880=EDGE_LOOP('',(#69000,#69001,#69002,#69003));
#27881=EDGE_LOOP('',(#69004,#69005,#69006,#69007));
#27882=EDGE_LOOP('',(#69008,#69009,#69010,#69011));
#27883=EDGE_LOOP('',(#69012,#69013,#69014,#69015));
#27884=EDGE_LOOP('',(#69016,#69017,#69018,#69019));
#27885=EDGE_LOOP('',(#69020,#69021,#69022,#69023));
#27886=EDGE_LOOP('',(#69024,#69025,#69026,#69027));
#27887=EDGE_LOOP('',(#69028,#69029,#69030,#69031));
#27888=EDGE_LOOP('',(#69032,#69033,#69034,#69035));
#27889=EDGE_LOOP('',(#69036,#69037,#69038,#69039));
#27890=EDGE_LOOP('',(#69040,#69041,#69042,#69043));
#27891=EDGE_LOOP('',(#69044,#69045,#69046,#69047));
#27892=EDGE_LOOP('',(#69048,#69049,#69050,#69051));
#27893=EDGE_LOOP('',(#69052,#69053,#69054,#69055));
#27894=EDGE_LOOP('',(#69056,#69057,#69058,#69059));
#27895=EDGE_LOOP('',(#69060,#69061,#69062,#69063));
#27896=EDGE_LOOP('',(#69064,#69065,#69066,#69067));
#27897=EDGE_LOOP('',(#69068,#69069,#69070,#69071));
#27898=EDGE_LOOP('',(#69072,#69073,#69074,#69075));
#27899=EDGE_LOOP('',(#69076,#69077,#69078,#69079));
#27900=EDGE_LOOP('',(#69080,#69081,#69082,#69083));
#27901=EDGE_LOOP('',(#69084,#69085,#69086,#69087));
#27902=EDGE_LOOP('',(#69088,#69089,#69090,#69091));
#27903=EDGE_LOOP('',(#69092,#69093,#69094,#69095));
#27904=EDGE_LOOP('',(#69096,#69097,#69098,#69099));
#27905=EDGE_LOOP('',(#69100,#69101,#69102,#69103));
#27906=EDGE_LOOP('',(#69104,#69105,#69106,#69107));
#27907=EDGE_LOOP('',(#69108,#69109,#69110,#69111));
#27908=EDGE_LOOP('',(#69112,#69113,#69114,#69115));
#27909=EDGE_LOOP('',(#69116,#69117,#69118,#69119));
#27910=EDGE_LOOP('',(#69120,#69121,#69122,#69123));
#27911=EDGE_LOOP('',(#69124,#69125,#69126,#69127));
#27912=EDGE_LOOP('',(#69128,#69129,#69130,#69131));
#27913=EDGE_LOOP('',(#69132,#69133,#69134,#69135));
#27914=EDGE_LOOP('',(#69136,#69137,#69138,#69139));
#27915=EDGE_LOOP('',(#69140,#69141,#69142,#69143));
#27916=EDGE_LOOP('',(#69144,#69145,#69146,#69147));
#27917=EDGE_LOOP('',(#69148,#69149,#69150,#69151));
#27918=EDGE_LOOP('',(#69152,#69153,#69154,#69155));
#27919=EDGE_LOOP('',(#69156,#69157,#69158,#69159));
#27920=EDGE_LOOP('',(#69160,#69161,#69162,#69163));
#27921=EDGE_LOOP('',(#69164,#69165,#69166,#69167));
#27922=EDGE_LOOP('',(#69168,#69169,#69170,#69171));
#27923=EDGE_LOOP('',(#69172,#69173,#69174,#69175));
#27924=EDGE_LOOP('',(#69176,#69177,#69178,#69179));
#27925=EDGE_LOOP('',(#69180,#69181,#69182,#69183));
#27926=EDGE_LOOP('',(#69184,#69185,#69186,#69187));
#27927=EDGE_LOOP('',(#69188,#69189,#69190,#69191));
#27928=EDGE_LOOP('',(#69192,#69193,#69194,#69195));
#27929=EDGE_LOOP('',(#69196,#69197,#69198,#69199));
#27930=EDGE_LOOP('',(#69200,#69201,#69202,#69203));
#27931=EDGE_LOOP('',(#69204,#69205,#69206,#69207));
#27932=EDGE_LOOP('',(#69208,#69209,#69210,#69211));
#27933=EDGE_LOOP('',(#69212,#69213,#69214,#69215));
#27934=EDGE_LOOP('',(#69216,#69217,#69218,#69219));
#27935=EDGE_LOOP('',(#69220,#69221,#69222,#69223));
#27936=EDGE_LOOP('',(#69224,#69225,#69226,#69227));
#27937=EDGE_LOOP('',(#69228,#69229,#69230,#69231));
#27938=EDGE_LOOP('',(#69232,#69233,#69234,#69235));
#27939=EDGE_LOOP('',(#69236,#69237,#69238,#69239));
#27940=EDGE_LOOP('',(#69240,#69241,#69242,#69243));
#27941=EDGE_LOOP('',(#69244,#69245,#69246,#69247));
#27942=EDGE_LOOP('',(#69248,#69249,#69250,#69251));
#27943=EDGE_LOOP('',(#69252,#69253,#69254,#69255));
#27944=EDGE_LOOP('',(#69256,#69257,#69258,#69259));
#27945=EDGE_LOOP('',(#69260,#69261,#69262,#69263));
#27946=EDGE_LOOP('',(#69264,#69265,#69266,#69267));
#27947=EDGE_LOOP('',(#69268,#69269,#69270,#69271));
#27948=EDGE_LOOP('',(#69272,#69273,#69274,#69275));
#27949=EDGE_LOOP('',(#69276,#69277,#69278,#69279));
#27950=EDGE_LOOP('',(#69280,#69281,#69282,#69283));
#27951=EDGE_LOOP('',(#69284,#69285,#69286,#69287));
#27952=EDGE_LOOP('',(#69288,#69289,#69290,#69291));
#27953=EDGE_LOOP('',(#69292,#69293,#69294,#69295));
#27954=EDGE_LOOP('',(#69296,#69297,#69298,#69299));
#27955=EDGE_LOOP('',(#69300,#69301,#69302,#69303));
#27956=EDGE_LOOP('',(#69304,#69305,#69306,#69307));
#27957=EDGE_LOOP('',(#69308,#69309,#69310,#69311));
#27958=EDGE_LOOP('',(#69312,#69313,#69314,#69315));
#27959=EDGE_LOOP('',(#69316,#69317,#69318,#69319));
#27960=EDGE_LOOP('',(#69320,#69321,#69322,#69323));
#27961=EDGE_LOOP('',(#69324,#69325,#69326,#69327));
#27962=EDGE_LOOP('',(#69328,#69329,#69330,#69331));
#27963=EDGE_LOOP('',(#69332,#69333,#69334,#69335));
#27964=EDGE_LOOP('',(#69336,#69337,#69338,#69339));
#27965=EDGE_LOOP('',(#69340,#69341,#69342,#69343));
#27966=EDGE_LOOP('',(#69344,#69345,#69346,#69347));
#27967=EDGE_LOOP('',(#69348,#69349,#69350,#69351));
#27968=EDGE_LOOP('',(#69352,#69353,#69354,#69355));
#27969=EDGE_LOOP('',(#69356,#69357,#69358,#69359));
#27970=EDGE_LOOP('',(#69360,#69361,#69362,#69363));
#27971=EDGE_LOOP('',(#69364,#69365,#69366,#69367));
#27972=EDGE_LOOP('',(#69368,#69369,#69370,#69371));
#27973=EDGE_LOOP('',(#69372,#69373,#69374,#69375));
#27974=EDGE_LOOP('',(#69376,#69377,#69378,#69379));
#27975=EDGE_LOOP('',(#69380,#69381,#69382,#69383));
#27976=EDGE_LOOP('',(#69384,#69385,#69386,#69387));
#27977=EDGE_LOOP('',(#69388,#69389,#69390,#69391));
#27978=EDGE_LOOP('',(#69392,#69393,#69394,#69395));
#27979=EDGE_LOOP('',(#69396,#69397,#69398,#69399));
#27980=EDGE_LOOP('',(#69400,#69401,#69402,#69403));
#27981=EDGE_LOOP('',(#69404,#69405,#69406,#69407));
#27982=EDGE_LOOP('',(#69408,#69409,#69410,#69411));
#27983=EDGE_LOOP('',(#69412,#69413,#69414,#69415));
#27984=EDGE_LOOP('',(#69416,#69417,#69418,#69419));
#27985=EDGE_LOOP('',(#69420,#69421,#69422,#69423));
#27986=EDGE_LOOP('',(#69424,#69425,#69426,#69427));
#27987=EDGE_LOOP('',(#69428,#69429,#69430,#69431));
#27988=EDGE_LOOP('',(#69432,#69433,#69434,#69435));
#27989=EDGE_LOOP('',(#69436,#69437,#69438,#69439));
#27990=EDGE_LOOP('',(#69440,#69441,#69442,#69443));
#27991=EDGE_LOOP('',(#69444,#69445,#69446,#69447));
#27992=EDGE_LOOP('',(#69448,#69449,#69450,#69451));
#27993=EDGE_LOOP('',(#69452,#69453,#69454,#69455));
#27994=EDGE_LOOP('',(#69456,#69457,#69458,#69459));
#27995=EDGE_LOOP('',(#69460,#69461,#69462,#69463));
#27996=EDGE_LOOP('',(#69464,#69465,#69466,#69467));
#27997=EDGE_LOOP('',(#69468,#69469,#69470,#69471));
#27998=EDGE_LOOP('',(#69472,#69473,#69474,#69475));
#27999=EDGE_LOOP('',(#69476,#69477,#69478,#69479));
#28000=EDGE_LOOP('',(#69480,#69481,#69482,#69483));
#28001=EDGE_LOOP('',(#69484,#69485,#69486,#69487));
#28002=EDGE_LOOP('',(#69488,#69489,#69490,#69491));
#28003=EDGE_LOOP('',(#69492,#69493,#69494,#69495));
#28004=EDGE_LOOP('',(#69496,#69497,#69498,#69499));
#28005=EDGE_LOOP('',(#69500,#69501,#69502,#69503));
#28006=EDGE_LOOP('',(#69504,#69505,#69506,#69507));
#28007=EDGE_LOOP('',(#69508,#69509,#69510,#69511));
#28008=EDGE_LOOP('',(#69512,#69513,#69514,#69515));
#28009=EDGE_LOOP('',(#69516,#69517,#69518,#69519));
#28010=EDGE_LOOP('',(#69520,#69521,#69522,#69523));
#28011=EDGE_LOOP('',(#69524,#69525,#69526,#69527));
#28012=EDGE_LOOP('',(#69528,#69529,#69530,#69531));
#28013=EDGE_LOOP('',(#69532,#69533,#69534,#69535));
#28014=EDGE_LOOP('',(#69536,#69537,#69538,#69539));
#28015=EDGE_LOOP('',(#69540,#69541,#69542,#69543));
#28016=EDGE_LOOP('',(#69544,#69545,#69546,#69547));
#28017=EDGE_LOOP('',(#69548,#69549,#69550,#69551));
#28018=EDGE_LOOP('',(#69552,#69553,#69554,#69555));
#28019=EDGE_LOOP('',(#69556,#69557,#69558,#69559));
#28020=EDGE_LOOP('',(#69560,#69561,#69562,#69563));
#28021=EDGE_LOOP('',(#69564,#69565,#69566,#69567));
#28022=EDGE_LOOP('',(#69568,#69569,#69570,#69571));
#28023=EDGE_LOOP('',(#69572,#69573,#69574,#69575));
#28024=EDGE_LOOP('',(#69576,#69577,#69578,#69579));
#28025=EDGE_LOOP('',(#69580,#69581,#69582,#69583));
#28026=EDGE_LOOP('',(#69584,#69585,#69586,#69587));
#28027=EDGE_LOOP('',(#69588,#69589,#69590,#69591));
#28028=EDGE_LOOP('',(#69592,#69593,#69594,#69595));
#28029=EDGE_LOOP('',(#69596,#69597,#69598,#69599));
#28030=EDGE_LOOP('',(#69600,#69601,#69602,#69603));
#28031=EDGE_LOOP('',(#69604,#69605,#69606,#69607));
#28032=EDGE_LOOP('',(#69608,#69609,#69610,#69611));
#28033=EDGE_LOOP('',(#69612,#69613,#69614,#69615));
#28034=EDGE_LOOP('',(#69616,#69617,#69618,#69619));
#28035=EDGE_LOOP('',(#69620,#69621,#69622,#69623));
#28036=EDGE_LOOP('',(#69624,#69625,#69626,#69627));
#28037=EDGE_LOOP('',(#69628,#69629,#69630,#69631));
#28038=EDGE_LOOP('',(#69632,#69633,#69634,#69635));
#28039=EDGE_LOOP('',(#69636,#69637,#69638,#69639));
#28040=EDGE_LOOP('',(#69640,#69641,#69642,#69643));
#28041=EDGE_LOOP('',(#69644,#69645,#69646,#69647));
#28042=EDGE_LOOP('',(#69648,#69649,#69650,#69651));
#28043=EDGE_LOOP('',(#69652,#69653,#69654,#69655));
#28044=EDGE_LOOP('',(#69656,#69657,#69658,#69659));
#28045=EDGE_LOOP('',(#69660,#69661,#69662,#69663));
#28046=EDGE_LOOP('',(#69664,#69665,#69666,#69667));
#28047=EDGE_LOOP('',(#69668,#69669,#69670,#69671));
#28048=EDGE_LOOP('',(#69672,#69673,#69674,#69675));
#28049=EDGE_LOOP('',(#69676,#69677,#69678,#69679));
#28050=EDGE_LOOP('',(#69680,#69681,#69682,#69683));
#28051=EDGE_LOOP('',(#69684,#69685,#69686,#69687));
#28052=EDGE_LOOP('',(#69688,#69689,#69690,#69691));
#28053=EDGE_LOOP('',(#69692,#69693,#69694,#69695));
#28054=EDGE_LOOP('',(#69696,#69697,#69698,#69699));
#28055=EDGE_LOOP('',(#69700,#69701,#69702,#69703));
#28056=EDGE_LOOP('',(#69704,#69705,#69706,#69707));
#28057=EDGE_LOOP('',(#69708,#69709,#69710,#69711));
#28058=EDGE_LOOP('',(#69712,#69713,#69714,#69715));
#28059=EDGE_LOOP('',(#69716,#69717,#69718,#69719));
#28060=EDGE_LOOP('',(#69720,#69721,#69722,#69723));
#28061=EDGE_LOOP('',(#69724,#69725,#69726,#69727));
#28062=EDGE_LOOP('',(#69728,#69729,#69730,#69731));
#28063=EDGE_LOOP('',(#69732,#69733,#69734,#69735));
#28064=EDGE_LOOP('',(#69736,#69737,#69738,#69739));
#28065=EDGE_LOOP('',(#69740,#69741,#69742,#69743));
#28066=EDGE_LOOP('',(#69744,#69745,#69746,#69747));
#28067=EDGE_LOOP('',(#69748,#69749,#69750,#69751));
#28068=EDGE_LOOP('',(#69752,#69753,#69754,#69755));
#28069=EDGE_LOOP('',(#69756,#69757,#69758,#69759));
#28070=EDGE_LOOP('',(#69760,#69761,#69762,#69763));
#28071=EDGE_LOOP('',(#69764,#69765,#69766,#69767));
#28072=EDGE_LOOP('',(#69768,#69769,#69770,#69771));
#28073=EDGE_LOOP('',(#69772,#69773,#69774,#69775));
#28074=EDGE_LOOP('',(#69776,#69777,#69778,#69779));
#28075=EDGE_LOOP('',(#69780,#69781,#69782,#69783));
#28076=EDGE_LOOP('',(#69784,#69785,#69786,#69787));
#28077=EDGE_LOOP('',(#69788,#69789,#69790,#69791));
#28078=EDGE_LOOP('',(#69792,#69793,#69794,#69795));
#28079=EDGE_LOOP('',(#69796,#69797,#69798,#69799));
#28080=EDGE_LOOP('',(#69800,#69801,#69802,#69803));
#28081=EDGE_LOOP('',(#69804,#69805,#69806,#69807));
#28082=EDGE_LOOP('',(#69808,#69809,#69810,#69811));
#28083=EDGE_LOOP('',(#69812,#69813,#69814,#69815));
#28084=EDGE_LOOP('',(#69816,#69817,#69818,#69819));
#28085=EDGE_LOOP('',(#69820,#69821,#69822,#69823));
#28086=EDGE_LOOP('',(#69824,#69825,#69826,#69827));
#28087=EDGE_LOOP('',(#69828,#69829,#69830,#69831));
#28088=EDGE_LOOP('',(#69832,#69833,#69834,#69835));
#28089=EDGE_LOOP('',(#69836,#69837,#69838,#69839));
#28090=EDGE_LOOP('',(#69840,#69841,#69842,#69843));
#28091=EDGE_LOOP('',(#69844,#69845,#69846,#69847));
#28092=EDGE_LOOP('',(#69848,#69849,#69850,#69851));
#28093=EDGE_LOOP('',(#69852,#69853,#69854,#69855));
#28094=EDGE_LOOP('',(#69856,#69857,#69858,#69859));
#28095=EDGE_LOOP('',(#69860,#69861,#69862,#69863));
#28096=EDGE_LOOP('',(#69864,#69865,#69866,#69867));
#28097=EDGE_LOOP('',(#69868,#69869,#69870,#69871));
#28098=EDGE_LOOP('',(#69872,#69873,#69874,#69875));
#28099=EDGE_LOOP('',(#69876,#69877,#69878,#69879));
#28100=EDGE_LOOP('',(#69880,#69881,#69882,#69883));
#28101=EDGE_LOOP('',(#69884,#69885,#69886,#69887));
#28102=EDGE_LOOP('',(#69888,#69889,#69890,#69891));
#28103=EDGE_LOOP('',(#69892,#69893,#69894,#69895));
#28104=EDGE_LOOP('',(#69896,#69897,#69898,#69899));
#28105=EDGE_LOOP('',(#69900,#69901,#69902,#69903));
#28106=EDGE_LOOP('',(#69904,#69905,#69906,#69907));
#28107=EDGE_LOOP('',(#69908,#69909,#69910,#69911));
#28108=EDGE_LOOP('',(#69912,#69913,#69914,#69915));
#28109=EDGE_LOOP('',(#69916,#69917,#69918,#69919));
#28110=EDGE_LOOP('',(#69920,#69921,#69922,#69923));
#28111=EDGE_LOOP('',(#69924,#69925,#69926,#69927));
#28112=EDGE_LOOP('',(#69928,#69929,#69930,#69931));
#28113=EDGE_LOOP('',(#69932,#69933,#69934,#69935));
#28114=EDGE_LOOP('',(#69936,#69937,#69938,#69939));
#28115=EDGE_LOOP('',(#69940,#69941,#69942,#69943));
#28116=EDGE_LOOP('',(#69944,#69945,#69946,#69947));
#28117=EDGE_LOOP('',(#69948,#69949,#69950,#69951));
#28118=EDGE_LOOP('',(#69952,#69953,#69954,#69955));
#28119=EDGE_LOOP('',(#69956,#69957,#69958,#69959));
#28120=EDGE_LOOP('',(#69960,#69961,#69962,#69963));
#28121=EDGE_LOOP('',(#69964,#69965,#69966,#69967));
#28122=EDGE_LOOP('',(#69968,#69969,#69970,#69971));
#28123=EDGE_LOOP('',(#69972,#69973,#69974,#69975));
#28124=EDGE_LOOP('',(#69976,#69977,#69978,#69979));
#28125=EDGE_LOOP('',(#69980,#69981,#69982,#69983));
#28126=EDGE_LOOP('',(#69984,#69985,#69986,#69987));
#28127=EDGE_LOOP('',(#69988,#69989,#69990,#69991));
#28128=EDGE_LOOP('',(#69992,#69993,#69994,#69995));
#28129=EDGE_LOOP('',(#69996,#69997,#69998,#69999));
#28130=EDGE_LOOP('',(#70000,#70001,#70002,#70003));
#28131=EDGE_LOOP('',(#70004,#70005,#70006,#70007));
#28132=EDGE_LOOP('',(#70008,#70009,#70010,#70011));
#28133=EDGE_LOOP('',(#70012,#70013,#70014,#70015));
#28134=EDGE_LOOP('',(#70016,#70017,#70018,#70019));
#28135=EDGE_LOOP('',(#70020,#70021,#70022,#70023));
#28136=EDGE_LOOP('',(#70024,#70025,#70026,#70027));
#28137=EDGE_LOOP('',(#70028,#70029,#70030,#70031));
#28138=EDGE_LOOP('',(#70032,#70033,#70034,#70035));
#28139=EDGE_LOOP('',(#70036,#70037,#70038,#70039));
#28140=EDGE_LOOP('',(#70040,#70041,#70042,#70043));
#28141=EDGE_LOOP('',(#70044,#70045,#70046,#70047));
#28142=EDGE_LOOP('',(#70048,#70049,#70050,#70051));
#28143=EDGE_LOOP('',(#70052,#70053,#70054,#70055));
#28144=EDGE_LOOP('',(#70056,#70057,#70058,#70059));
#28145=EDGE_LOOP('',(#70060,#70061,#70062,#70063));
#28146=EDGE_LOOP('',(#70064,#70065,#70066,#70067));
#28147=EDGE_LOOP('',(#70068,#70069,#70070,#70071));
#28148=EDGE_LOOP('',(#70072,#70073,#70074,#70075));
#28149=EDGE_LOOP('',(#70076,#70077,#70078,#70079));
#28150=EDGE_LOOP('',(#70080,#70081,#70082,#70083));
#28151=EDGE_LOOP('',(#70084,#70085,#70086,#70087));
#28152=EDGE_LOOP('',(#70088,#70089,#70090,#70091));
#28153=EDGE_LOOP('',(#70092,#70093,#70094,#70095));
#28154=EDGE_LOOP('',(#70096,#70097,#70098,#70099));
#28155=EDGE_LOOP('',(#70100,#70101,#70102,#70103));
#28156=EDGE_LOOP('',(#70104,#70105,#70106,#70107));
#28157=EDGE_LOOP('',(#70108,#70109,#70110,#70111));
#28158=EDGE_LOOP('',(#70112,#70113,#70114,#70115));
#28159=EDGE_LOOP('',(#70116,#70117,#70118,#70119));
#28160=EDGE_LOOP('',(#70120,#70121,#70122,#70123));
#28161=EDGE_LOOP('',(#70124,#70125,#70126,#70127));
#28162=EDGE_LOOP('',(#70128,#70129,#70130,#70131));
#28163=EDGE_LOOP('',(#70132,#70133,#70134,#70135));
#28164=EDGE_LOOP('',(#70136,#70137,#70138,#70139));
#28165=EDGE_LOOP('',(#70140,#70141,#70142,#70143));
#28166=EDGE_LOOP('',(#70144,#70145,#70146,#70147));
#28167=EDGE_LOOP('',(#70148,#70149,#70150,#70151));
#28168=EDGE_LOOP('',(#70152,#70153,#70154,#70155));
#28169=EDGE_LOOP('',(#70156,#70157,#70158,#70159));
#28170=EDGE_LOOP('',(#70160,#70161,#70162,#70163));
#28171=EDGE_LOOP('',(#70164,#70165,#70166,#70167));
#28172=EDGE_LOOP('',(#70168,#70169,#70170,#70171));
#28173=EDGE_LOOP('',(#70172,#70173,#70174,#70175));
#28174=EDGE_LOOP('',(#70176,#70177,#70178,#70179));
#28175=EDGE_LOOP('',(#70180,#70181,#70182,#70183));
#28176=EDGE_LOOP('',(#70184,#70185,#70186,#70187));
#28177=EDGE_LOOP('',(#70188,#70189,#70190,#70191));
#28178=EDGE_LOOP('',(#70192,#70193,#70194,#70195));
#28179=EDGE_LOOP('',(#70196,#70197,#70198,#70199));
#28180=EDGE_LOOP('',(#70200,#70201,#70202,#70203));
#28181=EDGE_LOOP('',(#70204,#70205,#70206,#70207));
#28182=EDGE_LOOP('',(#70208,#70209,#70210,#70211));
#28183=EDGE_LOOP('',(#70212,#70213,#70214,#70215));
#28184=EDGE_LOOP('',(#70216,#70217,#70218,#70219));
#28185=EDGE_LOOP('',(#70220,#70221,#70222,#70223));
#28186=EDGE_LOOP('',(#70224,#70225,#70226,#70227));
#28187=EDGE_LOOP('',(#70228,#70229,#70230,#70231));
#28188=EDGE_LOOP('',(#70232,#70233,#70234,#70235));
#28189=EDGE_LOOP('',(#70236,#70237,#70238,#70239));
#28190=EDGE_LOOP('',(#70240,#70241,#70242,#70243));
#28191=EDGE_LOOP('',(#70244,#70245,#70246,#70247));
#28192=EDGE_LOOP('',(#70248,#70249,#70250,#70251));
#28193=EDGE_LOOP('',(#70252,#70253,#70254,#70255));
#28194=EDGE_LOOP('',(#70256,#70257,#70258,#70259));
#28195=EDGE_LOOP('',(#70260,#70261,#70262,#70263));
#28196=EDGE_LOOP('',(#70264,#70265,#70266,#70267));
#28197=EDGE_LOOP('',(#70268,#70269,#70270,#70271));
#28198=EDGE_LOOP('',(#70272,#70273,#70274,#70275));
#28199=EDGE_LOOP('',(#70276,#70277,#70278,#70279));
#28200=EDGE_LOOP('',(#70280,#70281,#70282,#70283));
#28201=EDGE_LOOP('',(#70284,#70285,#70286,#70287));
#28202=EDGE_LOOP('',(#70288,#70289,#70290,#70291));
#28203=EDGE_LOOP('',(#70292,#70293,#70294,#70295));
#28204=EDGE_LOOP('',(#70296,#70297,#70298,#70299));
#28205=EDGE_LOOP('',(#70300,#70301,#70302,#70303));
#28206=EDGE_LOOP('',(#70304,#70305,#70306,#70307));
#28207=EDGE_LOOP('',(#70308,#70309,#70310,#70311));
#28208=EDGE_LOOP('',(#70312,#70313,#70314,#70315));
#28209=EDGE_LOOP('',(#70316,#70317,#70318,#70319));
#28210=EDGE_LOOP('',(#70320,#70321,#70322,#70323));
#28211=EDGE_LOOP('',(#70324,#70325,#70326,#70327));
#28212=EDGE_LOOP('',(#70328,#70329,#70330,#70331));
#28213=EDGE_LOOP('',(#70332,#70333,#70334,#70335));
#28214=EDGE_LOOP('',(#70336,#70337,#70338,#70339));
#28215=EDGE_LOOP('',(#70340,#70341,#70342,#70343));
#28216=EDGE_LOOP('',(#70344,#70345,#70346,#70347));
#28217=EDGE_LOOP('',(#70348,#70349,#70350,#70351));
#28218=EDGE_LOOP('',(#70352,#70353,#70354,#70355));
#28219=EDGE_LOOP('',(#70356,#70357,#70358,#70359));
#28220=EDGE_LOOP('',(#70360,#70361,#70362,#70363));
#28221=EDGE_LOOP('',(#70364,#70365,#70366,#70367));
#28222=EDGE_LOOP('',(#70368,#70369,#70370,#70371));
#28223=EDGE_LOOP('',(#70372,#70373,#70374,#70375));
#28224=EDGE_LOOP('',(#70376,#70377,#70378,#70379));
#28225=EDGE_LOOP('',(#70380,#70381,#70382,#70383));
#28226=EDGE_LOOP('',(#70384,#70385,#70386,#70387));
#28227=EDGE_LOOP('',(#70388,#70389,#70390,#70391));
#28228=EDGE_LOOP('',(#70392,#70393,#70394,#70395));
#28229=EDGE_LOOP('',(#70396,#70397,#70398,#70399));
#28230=EDGE_LOOP('',(#70400,#70401,#70402,#70403));
#28231=EDGE_LOOP('',(#70404,#70405,#70406,#70407));
#28232=EDGE_LOOP('',(#70408,#70409,#70410,#70411));
#28233=EDGE_LOOP('',(#70412,#70413,#70414,#70415));
#28234=EDGE_LOOP('',(#70416,#70417,#70418,#70419));
#28235=EDGE_LOOP('',(#70420,#70421,#70422,#70423));
#28236=EDGE_LOOP('',(#70424,#70425,#70426,#70427));
#28237=EDGE_LOOP('',(#70428,#70429,#70430,#70431));
#28238=EDGE_LOOP('',(#70432,#70433,#70434,#70435));
#28239=EDGE_LOOP('',(#70436,#70437,#70438,#70439));
#28240=EDGE_LOOP('',(#70440,#70441,#70442,#70443));
#28241=EDGE_LOOP('',(#70444,#70445,#70446,#70447));
#28242=EDGE_LOOP('',(#70448,#70449,#70450,#70451));
#28243=EDGE_LOOP('',(#70452,#70453,#70454,#70455));
#28244=EDGE_LOOP('',(#70456,#70457,#70458,#70459));
#28245=EDGE_LOOP('',(#70460));
#28246=EDGE_LOOP('',(#70461,#70462,#70463,#70464));
#28247=EDGE_LOOP('',(#70465,#70466,#70467,#70468));
#28248=EDGE_LOOP('',(#70469,#70470,#70471,#70472));
#28249=EDGE_LOOP('',(#70473,#70474,#70475,#70476));
#28250=EDGE_LOOP('',(#70477,#70478,#70479,#70480));
#28251=EDGE_LOOP('',(#70481,#70482,#70483,#70484));
#28252=EDGE_LOOP('',(#70485,#70486,#70487,#70488));
#28253=EDGE_LOOP('',(#70489,#70490,#70491,#70492));
#28254=EDGE_LOOP('',(#70493,#70494,#70495,#70496));
#28255=EDGE_LOOP('',(#70497,#70498,#70499,#70500));
#28256=EDGE_LOOP('',(#70501,#70502,#70503,#70504));
#28257=EDGE_LOOP('',(#70505,#70506,#70507,#70508));
#28258=EDGE_LOOP('',(#70509,#70510,#70511,#70512));
#28259=EDGE_LOOP('',(#70513,#70514,#70515,#70516));
#28260=EDGE_LOOP('',(#70517,#70518,#70519,#70520));
#28261=EDGE_LOOP('',(#70521,#70522,#70523,#70524));
#28262=EDGE_LOOP('',(#70525,#70526,#70527,#70528));
#28263=EDGE_LOOP('',(#70529,#70530,#70531,#70532));
#28264=EDGE_LOOP('',(#70533,#70534,#70535,#70536));
#28265=EDGE_LOOP('',(#70537,#70538,#70539,#70540));
#28266=EDGE_LOOP('',(#70541,#70542,#70543,#70544));
#28267=EDGE_LOOP('',(#70545,#70546,#70547,#70548));
#28268=EDGE_LOOP('',(#70549,#70550,#70551,#70552));
#28269=EDGE_LOOP('',(#70553,#70554,#70555,#70556));
#28270=EDGE_LOOP('',(#70557,#70558,#70559,#70560));
#28271=EDGE_LOOP('',(#70561,#70562,#70563,#70564));
#28272=EDGE_LOOP('',(#70565,#70566,#70567,#70568));
#28273=EDGE_LOOP('',(#70569,#70570,#70571,#70572));
#28274=EDGE_LOOP('',(#70573,#70574,#70575,#70576));
#28275=EDGE_LOOP('',(#70577,#70578,#70579,#70580));
#28276=EDGE_LOOP('',(#70581,#70582,#70583,#70584));
#28277=EDGE_LOOP('',(#70585,#70586,#70587,#70588));
#28278=EDGE_LOOP('',(#70589,#70590,#70591,#70592));
#28279=EDGE_LOOP('',(#70593,#70594,#70595,#70596));
#28280=EDGE_LOOP('',(#70597,#70598,#70599,#70600));
#28281=EDGE_LOOP('',(#70601,#70602,#70603,#70604));
#28282=EDGE_LOOP('',(#70605,#70606,#70607,#70608));
#28283=EDGE_LOOP('',(#70609,#70610,#70611,#70612));
#28284=EDGE_LOOP('',(#70613,#70614,#70615,#70616));
#28285=EDGE_LOOP('',(#70617,#70618,#70619,#70620));
#28286=EDGE_LOOP('',(#70621,#70622,#70623,#70624));
#28287=EDGE_LOOP('',(#70625,#70626,#70627,#70628));
#28288=EDGE_LOOP('',(#70629,#70630,#70631,#70632));
#28289=EDGE_LOOP('',(#70633,#70634,#70635,#70636));
#28290=EDGE_LOOP('',(#70637,#70638,#70639,#70640));
#28291=EDGE_LOOP('',(#70641,#70642,#70643,#70644));
#28292=EDGE_LOOP('',(#70645,#70646,#70647,#70648));
#28293=EDGE_LOOP('',(#70649,#70650,#70651,#70652));
#28294=EDGE_LOOP('',(#70653,#70654,#70655,#70656));
#28295=EDGE_LOOP('',(#70657,#70658,#70659,#70660));
#28296=EDGE_LOOP('',(#70661,#70662,#70663,#70664));
#28297=EDGE_LOOP('',(#70665,#70666,#70667,#70668));
#28298=EDGE_LOOP('',(#70669,#70670,#70671,#70672));
#28299=EDGE_LOOP('',(#70673,#70674,#70675,#70676));
#28300=EDGE_LOOP('',(#70677,#70678,#70679,#70680));
#28301=EDGE_LOOP('',(#70681,#70682,#70683,#70684));
#28302=EDGE_LOOP('',(#70685,#70686,#70687,#70688));
#28303=EDGE_LOOP('',(#70689,#70690,#70691,#70692));
#28304=EDGE_LOOP('',(#70693,#70694,#70695,#70696));
#28305=EDGE_LOOP('',(#70697,#70698,#70699,#70700));
#28306=EDGE_LOOP('',(#70701,#70702,#70703,#70704));
#28307=EDGE_LOOP('',(#70705,#70706,#70707,#70708));
#28308=EDGE_LOOP('',(#70709,#70710,#70711,#70712));
#28309=EDGE_LOOP('',(#70713,#70714,#70715,#70716));
#28310=EDGE_LOOP('',(#70717,#70718,#70719,#70720));
#28311=EDGE_LOOP('',(#70721,#70722,#70723,#70724));
#28312=EDGE_LOOP('',(#70725,#70726,#70727,#70728));
#28313=EDGE_LOOP('',(#70729,#70730,#70731,#70732));
#28314=EDGE_LOOP('',(#70733,#70734,#70735,#70736));
#28315=EDGE_LOOP('',(#70737,#70738,#70739,#70740));
#28316=EDGE_LOOP('',(#70741,#70742,#70743,#70744));
#28317=EDGE_LOOP('',(#70745,#70746,#70747,#70748));
#28318=EDGE_LOOP('',(#70749,#70750,#70751,#70752));
#28319=EDGE_LOOP('',(#70753,#70754,#70755,#70756));
#28320=EDGE_LOOP('',(#70757,#70758,#70759,#70760));
#28321=EDGE_LOOP('',(#70761,#70762,#70763,#70764));
#28322=EDGE_LOOP('',(#70765,#70766,#70767,#70768));
#28323=EDGE_LOOP('',(#70769,#70770,#70771,#70772));
#28324=EDGE_LOOP('',(#70773,#70774,#70775,#70776));
#28325=EDGE_LOOP('',(#70777,#70778,#70779,#70780));
#28326=EDGE_LOOP('',(#70781,#70782,#70783,#70784));
#28327=EDGE_LOOP('',(#70785,#70786,#70787,#70788));
#28328=EDGE_LOOP('',(#70789,#70790,#70791,#70792));
#28329=EDGE_LOOP('',(#70793,#70794,#70795,#70796));
#28330=EDGE_LOOP('',(#70797,#70798,#70799,#70800));
#28331=EDGE_LOOP('',(#70801,#70802,#70803,#70804));
#28332=EDGE_LOOP('',(#70805,#70806,#70807,#70808));
#28333=EDGE_LOOP('',(#70809,#70810,#70811,#70812));
#28334=EDGE_LOOP('',(#70813,#70814,#70815,#70816));
#28335=EDGE_LOOP('',(#70817,#70818,#70819,#70820));
#28336=EDGE_LOOP('',(#70821,#70822,#70823,#70824));
#28337=EDGE_LOOP('',(#70825,#70826,#70827,#70828));
#28338=EDGE_LOOP('',(#70829,#70830,#70831,#70832));
#28339=EDGE_LOOP('',(#70833,#70834,#70835,#70836));
#28340=EDGE_LOOP('',(#70837,#70838,#70839,#70840));
#28341=EDGE_LOOP('',(#70841,#70842,#70843,#70844));
#28342=EDGE_LOOP('',(#70845,#70846,#70847,#70848));
#28343=EDGE_LOOP('',(#70849,#70850,#70851,#70852));
#28344=EDGE_LOOP('',(#70853,#70854,#70855,#70856));
#28345=EDGE_LOOP('',(#70857,#70858,#70859,#70860));
#28346=EDGE_LOOP('',(#70861,#70862,#70863,#70864));
#28347=EDGE_LOOP('',(#70865,#70866,#70867,#70868));
#28348=EDGE_LOOP('',(#70869,#70870,#70871,#70872));
#28349=EDGE_LOOP('',(#70873,#70874,#70875,#70876));
#28350=EDGE_LOOP('',(#70877,#70878,#70879,#70880));
#28351=EDGE_LOOP('',(#70881,#70882,#70883,#70884));
#28352=EDGE_LOOP('',(#70885,#70886,#70887,#70888));
#28353=EDGE_LOOP('',(#70889,#70890,#70891,#70892));
#28354=EDGE_LOOP('',(#70893,#70894,#70895,#70896));
#28355=EDGE_LOOP('',(#70897,#70898,#70899,#70900));
#28356=EDGE_LOOP('',(#70901,#70902,#70903,#70904));
#28357=EDGE_LOOP('',(#70905,#70906,#70907,#70908));
#28358=EDGE_LOOP('',(#70909,#70910,#70911,#70912));
#28359=EDGE_LOOP('',(#70913,#70914,#70915,#70916));
#28360=EDGE_LOOP('',(#70917,#70918,#70919,#70920));
#28361=EDGE_LOOP('',(#70921,#70922,#70923,#70924));
#28362=EDGE_LOOP('',(#70925,#70926,#70927,#70928));
#28363=EDGE_LOOP('',(#70929,#70930,#70931,#70932));
#28364=EDGE_LOOP('',(#70933,#70934,#70935,#70936));
#28365=EDGE_LOOP('',(#70937,#70938,#70939,#70940));
#28366=EDGE_LOOP('',(#70941,#70942,#70943,#70944));
#28367=EDGE_LOOP('',(#70945,#70946,#70947,#70948));
#28368=EDGE_LOOP('',(#70949,#70950,#70951,#70952));
#28369=EDGE_LOOP('',(#70953,#70954,#70955,#70956));
#28370=EDGE_LOOP('',(#70957,#70958,#70959,#70960));
#28371=EDGE_LOOP('',(#70961,#70962,#70963,#70964));
#28372=EDGE_LOOP('',(#70965,#70966,#70967,#70968));
#28373=EDGE_LOOP('',(#70969,#70970,#70971,#70972));
#28374=EDGE_LOOP('',(#70973,#70974,#70975,#70976));
#28375=EDGE_LOOP('',(#70977,#70978,#70979,#70980));
#28376=EDGE_LOOP('',(#70981,#70982,#70983,#70984));
#28377=EDGE_LOOP('',(#70985,#70986,#70987,#70988));
#28378=EDGE_LOOP('',(#70989,#70990,#70991,#70992));
#28379=EDGE_LOOP('',(#70993,#70994,#70995,#70996));
#28380=EDGE_LOOP('',(#70997,#70998,#70999,#71000));
#28381=EDGE_LOOP('',(#71001,#71002,#71003,#71004));
#28382=EDGE_LOOP('',(#71005,#71006,#71007,#71008));
#28383=EDGE_LOOP('',(#71009,#71010,#71011,#71012));
#28384=EDGE_LOOP('',(#71013,#71014,#71015,#71016));
#28385=EDGE_LOOP('',(#71017,#71018,#71019,#71020));
#28386=EDGE_LOOP('',(#71021,#71022,#71023,#71024));
#28387=EDGE_LOOP('',(#71025,#71026,#71027,#71028));
#28388=EDGE_LOOP('',(#71029,#71030,#71031,#71032));
#28389=EDGE_LOOP('',(#71033,#71034,#71035,#71036));
#28390=EDGE_LOOP('',(#71037,#71038,#71039,#71040));
#28391=EDGE_LOOP('',(#71041,#71042,#71043,#71044));
#28392=EDGE_LOOP('',(#71045,#71046,#71047,#71048));
#28393=EDGE_LOOP('',(#71049,#71050,#71051,#71052));
#28394=EDGE_LOOP('',(#71053,#71054,#71055,#71056));
#28395=EDGE_LOOP('',(#71057,#71058,#71059,#71060));
#28396=EDGE_LOOP('',(#71061,#71062,#71063,#71064));
#28397=EDGE_LOOP('',(#71065,#71066,#71067,#71068));
#28398=EDGE_LOOP('',(#71069,#71070,#71071,#71072));
#28399=EDGE_LOOP('',(#71073,#71074,#71075,#71076));
#28400=EDGE_LOOP('',(#71077,#71078,#71079,#71080));
#28401=EDGE_LOOP('',(#71081,#71082,#71083,#71084));
#28402=EDGE_LOOP('',(#71085,#71086,#71087,#71088));
#28403=EDGE_LOOP('',(#71089,#71090,#71091,#71092));
#28404=EDGE_LOOP('',(#71093,#71094,#71095,#71096));
#28405=EDGE_LOOP('',(#71097,#71098,#71099,#71100));
#28406=EDGE_LOOP('',(#71101,#71102,#71103,#71104));
#28407=EDGE_LOOP('',(#71105,#71106,#71107,#71108));
#28408=EDGE_LOOP('',(#71109,#71110,#71111,#71112));
#28409=EDGE_LOOP('',(#71113,#71114,#71115,#71116));
#28410=EDGE_LOOP('',(#71117,#71118,#71119,#71120));
#28411=EDGE_LOOP('',(#71121,#71122,#71123,#71124));
#28412=EDGE_LOOP('',(#71125,#71126,#71127,#71128));
#28413=EDGE_LOOP('',(#71129,#71130,#71131,#71132));
#28414=EDGE_LOOP('',(#71133,#71134,#71135,#71136));
#28415=EDGE_LOOP('',(#71137,#71138,#71139,#71140));
#28416=EDGE_LOOP('',(#71141,#71142,#71143,#71144));
#28417=EDGE_LOOP('',(#71145,#71146,#71147,#71148));
#28418=EDGE_LOOP('',(#71149,#71150,#71151,#71152));
#28419=EDGE_LOOP('',(#71153,#71154,#71155,#71156));
#28420=EDGE_LOOP('',(#71157,#71158,#71159,#71160));
#28421=EDGE_LOOP('',(#71161,#71162,#71163,#71164));
#28422=EDGE_LOOP('',(#71165,#71166,#71167,#71168));
#28423=EDGE_LOOP('',(#71169,#71170,#71171,#71172));
#28424=EDGE_LOOP('',(#71173,#71174,#71175,#71176));
#28425=EDGE_LOOP('',(#71177,#71178,#71179,#71180));
#28426=EDGE_LOOP('',(#71181,#71182,#71183,#71184));
#28427=EDGE_LOOP('',(#71185,#71186,#71187,#71188));
#28428=EDGE_LOOP('',(#71189,#71190,#71191,#71192));
#28429=EDGE_LOOP('',(#71193,#71194,#71195,#71196));
#28430=EDGE_LOOP('',(#71197,#71198,#71199,#71200));
#28431=EDGE_LOOP('',(#71201,#71202,#71203,#71204));
#28432=EDGE_LOOP('',(#71205,#71206,#71207,#71208));
#28433=EDGE_LOOP('',(#71209,#71210,#71211,#71212));
#28434=EDGE_LOOP('',(#71213,#71214,#71215,#71216));
#28435=EDGE_LOOP('',(#71217,#71218,#71219,#71220));
#28436=EDGE_LOOP('',(#71221,#71222,#71223,#71224));
#28437=EDGE_LOOP('',(#71225,#71226,#71227,#71228));
#28438=EDGE_LOOP('',(#71229,#71230,#71231,#71232));
#28439=EDGE_LOOP('',(#71233,#71234,#71235,#71236));
#28440=EDGE_LOOP('',(#71237,#71238,#71239,#71240));
#28441=EDGE_LOOP('',(#71241,#71242,#71243,#71244));
#28442=EDGE_LOOP('',(#71245,#71246,#71247,#71248));
#28443=EDGE_LOOP('',(#71249,#71250,#71251,#71252));
#28444=EDGE_LOOP('',(#71253,#71254,#71255,#71256));
#28445=EDGE_LOOP('',(#71257,#71258,#71259,#71260));
#28446=EDGE_LOOP('',(#71261,#71262,#71263,#71264));
#28447=EDGE_LOOP('',(#71265,#71266,#71267,#71268));
#28448=EDGE_LOOP('',(#71269,#71270,#71271,#71272));
#28449=EDGE_LOOP('',(#71273,#71274,#71275,#71276));
#28450=EDGE_LOOP('',(#71277,#71278,#71279,#71280));
#28451=EDGE_LOOP('',(#71281,#71282,#71283,#71284));
#28452=EDGE_LOOP('',(#71285,#71286,#71287,#71288));
#28453=EDGE_LOOP('',(#71289,#71290,#71291,#71292));
#28454=EDGE_LOOP('',(#71293,#71294,#71295,#71296));
#28455=EDGE_LOOP('',(#71297,#71298,#71299,#71300));
#28456=EDGE_LOOP('',(#71301,#71302,#71303,#71304));
#28457=EDGE_LOOP('',(#71305,#71306,#71307,#71308));
#28458=EDGE_LOOP('',(#71309,#71310,#71311,#71312));
#28459=EDGE_LOOP('',(#71313,#71314,#71315,#71316));
#28460=EDGE_LOOP('',(#71317,#71318,#71319,#71320));
#28461=EDGE_LOOP('',(#71321,#71322,#71323,#71324));
#28462=EDGE_LOOP('',(#71325,#71326,#71327,#71328));
#28463=EDGE_LOOP('',(#71329,#71330,#71331,#71332));
#28464=EDGE_LOOP('',(#71333,#71334,#71335,#71336));
#28465=EDGE_LOOP('',(#71337,#71338,#71339,#71340));
#28466=EDGE_LOOP('',(#71341,#71342,#71343,#71344));
#28467=EDGE_LOOP('',(#71345,#71346,#71347,#71348));
#28468=EDGE_LOOP('',(#71349,#71350,#71351,#71352));
#28469=EDGE_LOOP('',(#71353,#71354,#71355,#71356));
#28470=EDGE_LOOP('',(#71357,#71358,#71359,#71360));
#28471=EDGE_LOOP('',(#71361,#71362,#71363,#71364));
#28472=EDGE_LOOP('',(#71365,#71366,#71367,#71368));
#28473=EDGE_LOOP('',(#71369,#71370,#71371,#71372));
#28474=EDGE_LOOP('',(#71373,#71374,#71375,#71376));
#28475=EDGE_LOOP('',(#71377,#71378,#71379,#71380));
#28476=EDGE_LOOP('',(#71381,#71382,#71383,#71384));
#28477=EDGE_LOOP('',(#71385,#71386,#71387,#71388));
#28478=EDGE_LOOP('',(#71389,#71390,#71391,#71392));
#28479=EDGE_LOOP('',(#71393,#71394,#71395,#71396));
#28480=EDGE_LOOP('',(#71397,#71398,#71399,#71400));
#28481=EDGE_LOOP('',(#71401,#71402,#71403,#71404));
#28482=EDGE_LOOP('',(#71405,#71406,#71407,#71408));
#28483=EDGE_LOOP('',(#71409,#71410,#71411,#71412));
#28484=EDGE_LOOP('',(#71413,#71414,#71415,#71416));
#28485=EDGE_LOOP('',(#71417,#71418,#71419,#71420));
#28486=EDGE_LOOP('',(#71421,#71422,#71423,#71424));
#28487=EDGE_LOOP('',(#71425,#71426,#71427,#71428));
#28488=EDGE_LOOP('',(#71429,#71430,#71431,#71432));
#28489=EDGE_LOOP('',(#71433,#71434,#71435,#71436));
#28490=EDGE_LOOP('',(#71437,#71438,#71439,#71440));
#28491=EDGE_LOOP('',(#71441,#71442,#71443,#71444));
#28492=EDGE_LOOP('',(#71445,#71446,#71447,#71448));
#28493=EDGE_LOOP('',(#71449,#71450,#71451,#71452));
#28494=EDGE_LOOP('',(#71453,#71454,#71455,#71456));
#28495=EDGE_LOOP('',(#71457,#71458,#71459,#71460));
#28496=EDGE_LOOP('',(#71461,#71462,#71463,#71464));
#28497=EDGE_LOOP('',(#71465,#71466,#71467,#71468));
#28498=EDGE_LOOP('',(#71469,#71470,#71471,#71472));
#28499=EDGE_LOOP('',(#71473,#71474,#71475,#71476));
#28500=EDGE_LOOP('',(#71477,#71478,#71479,#71480));
#28501=EDGE_LOOP('',(#71481,#71482,#71483,#71484));
#28502=EDGE_LOOP('',(#71485,#71486,#71487,#71488));
#28503=EDGE_LOOP('',(#71489,#71490,#71491,#71492));
#28504=EDGE_LOOP('',(#71493,#71494,#71495,#71496));
#28505=EDGE_LOOP('',(#71497,#71498,#71499,#71500));
#28506=EDGE_LOOP('',(#71501,#71502,#71503,#71504));
#28507=EDGE_LOOP('',(#71505,#71506,#71507,#71508));
#28508=EDGE_LOOP('',(#71509,#71510,#71511,#71512));
#28509=EDGE_LOOP('',(#71513,#71514,#71515,#71516));
#28510=EDGE_LOOP('',(#71517,#71518,#71519,#71520));
#28511=EDGE_LOOP('',(#71521,#71522,#71523,#71524));
#28512=EDGE_LOOP('',(#71525,#71526,#71527,#71528));
#28513=EDGE_LOOP('',(#71529,#71530,#71531,#71532));
#28514=EDGE_LOOP('',(#71533,#71534,#71535,#71536));
#28515=EDGE_LOOP('',(#71537,#71538,#71539,#71540));
#28516=EDGE_LOOP('',(#71541,#71542,#71543,#71544));
#28517=EDGE_LOOP('',(#71545,#71546,#71547,#71548));
#28518=EDGE_LOOP('',(#71549,#71550,#71551,#71552));
#28519=EDGE_LOOP('',(#71553,#71554,#71555,#71556));
#28520=EDGE_LOOP('',(#71557,#71558,#71559,#71560));
#28521=EDGE_LOOP('',(#71561,#71562,#71563,#71564));
#28522=EDGE_LOOP('',(#71565,#71566,#71567,#71568));
#28523=EDGE_LOOP('',(#71569,#71570,#71571,#71572));
#28524=EDGE_LOOP('',(#71573,#71574,#71575,#71576));
#28525=EDGE_LOOP('',(#71577,#71578,#71579,#71580));
#28526=EDGE_LOOP('',(#71581,#71582,#71583,#71584));
#28527=EDGE_LOOP('',(#71585,#71586,#71587,#71588));
#28528=EDGE_LOOP('',(#71589,#71590,#71591,#71592));
#28529=EDGE_LOOP('',(#71593,#71594,#71595,#71596));
#28530=EDGE_LOOP('',(#71597,#71598,#71599,#71600));
#28531=EDGE_LOOP('',(#71601,#71602,#71603,#71604));
#28532=EDGE_LOOP('',(#71605,#71606,#71607,#71608));
#28533=EDGE_LOOP('',(#71609,#71610,#71611,#71612));
#28534=EDGE_LOOP('',(#71613,#71614,#71615,#71616));
#28535=EDGE_LOOP('',(#71617,#71618,#71619,#71620));
#28536=EDGE_LOOP('',(#71621,#71622,#71623,#71624));
#28537=EDGE_LOOP('',(#71625,#71626,#71627,#71628));
#28538=EDGE_LOOP('',(#71629,#71630,#71631,#71632));
#28539=EDGE_LOOP('',(#71633,#71634,#71635,#71636));
#28540=EDGE_LOOP('',(#71637,#71638,#71639,#71640));
#28541=EDGE_LOOP('',(#71641,#71642,#71643,#71644));
#28542=EDGE_LOOP('',(#71645,#71646,#71647,#71648));
#28543=EDGE_LOOP('',(#71649,#71650,#71651,#71652));
#28544=EDGE_LOOP('',(#71653,#71654,#71655,#71656));
#28545=EDGE_LOOP('',(#71657,#71658,#71659,#71660));
#28546=EDGE_LOOP('',(#71661,#71662,#71663,#71664));
#28547=EDGE_LOOP('',(#71665,#71666,#71667,#71668));
#28548=EDGE_LOOP('',(#71669,#71670,#71671,#71672));
#28549=EDGE_LOOP('',(#71673,#71674,#71675,#71676));
#28550=EDGE_LOOP('',(#71677,#71678,#71679,#71680));
#28551=EDGE_LOOP('',(#71681,#71682,#71683,#71684));
#28552=EDGE_LOOP('',(#71685,#71686,#71687,#71688));
#28553=EDGE_LOOP('',(#71689,#71690,#71691,#71692));
#28554=EDGE_LOOP('',(#71693,#71694,#71695,#71696));
#28555=EDGE_LOOP('',(#71697,#71698,#71699,#71700));
#28556=EDGE_LOOP('',(#71701,#71702,#71703,#71704));
#28557=EDGE_LOOP('',(#71705,#71706,#71707,#71708));
#28558=EDGE_LOOP('',(#71709,#71710,#71711,#71712));
#28559=EDGE_LOOP('',(#71713,#71714,#71715,#71716));
#28560=EDGE_LOOP('',(#71717,#71718,#71719,#71720));
#28561=EDGE_LOOP('',(#71721,#71722,#71723,#71724));
#28562=EDGE_LOOP('',(#71725,#71726,#71727,#71728));
#28563=EDGE_LOOP('',(#71729,#71730,#71731,#71732));
#28564=EDGE_LOOP('',(#71733,#71734,#71735,#71736));
#28565=EDGE_LOOP('',(#71737,#71738,#71739,#71740));
#28566=EDGE_LOOP('',(#71741,#71742,#71743,#71744));
#28567=EDGE_LOOP('',(#71745,#71746,#71747,#71748));
#28568=EDGE_LOOP('',(#71749,#71750,#71751,#71752));
#28569=EDGE_LOOP('',(#71753,#71754,#71755,#71756));
#28570=EDGE_LOOP('',(#71757,#71758,#71759,#71760));
#28571=EDGE_LOOP('',(#71761,#71762,#71763,#71764));
#28572=EDGE_LOOP('',(#71765,#71766,#71767,#71768));
#28573=EDGE_LOOP('',(#71769,#71770,#71771,#71772));
#28574=EDGE_LOOP('',(#71773,#71774,#71775,#71776));
#28575=EDGE_LOOP('',(#71777,#71778,#71779,#71780));
#28576=EDGE_LOOP('',(#71781,#71782,#71783,#71784));
#28577=EDGE_LOOP('',(#71785,#71786,#71787,#71788));
#28578=EDGE_LOOP('',(#71789,#71790,#71791,#71792));
#28579=EDGE_LOOP('',(#71793,#71794,#71795,#71796));
#28580=EDGE_LOOP('',(#71797,#71798,#71799,#71800));
#28581=EDGE_LOOP('',(#71801,#71802,#71803,#71804));
#28582=EDGE_LOOP('',(#71805,#71806,#71807,#71808));
#28583=EDGE_LOOP('',(#71809,#71810,#71811,#71812));
#28584=EDGE_LOOP('',(#71813,#71814,#71815,#71816));
#28585=EDGE_LOOP('',(#71817,#71818,#71819,#71820));
#28586=EDGE_LOOP('',(#71821,#71822,#71823,#71824));
#28587=EDGE_LOOP('',(#71825,#71826,#71827,#71828));
#28588=EDGE_LOOP('',(#71829,#71830,#71831,#71832));
#28589=EDGE_LOOP('',(#71833,#71834,#71835,#71836));
#28590=EDGE_LOOP('',(#71837,#71838,#71839,#71840));
#28591=EDGE_LOOP('',(#71841,#71842,#71843,#71844));
#28592=EDGE_LOOP('',(#71845,#71846,#71847,#71848));
#28593=EDGE_LOOP('',(#71849,#71850,#71851,#71852));
#28594=EDGE_LOOP('',(#71853,#71854,#71855,#71856));
#28595=EDGE_LOOP('',(#71857,#71858,#71859,#71860));
#28596=EDGE_LOOP('',(#71861,#71862,#71863,#71864));
#28597=EDGE_LOOP('',(#71865,#71866,#71867,#71868));
#28598=EDGE_LOOP('',(#71869,#71870,#71871,#71872));
#28599=EDGE_LOOP('',(#71873,#71874,#71875,#71876));
#28600=EDGE_LOOP('',(#71877,#71878,#71879,#71880));
#28601=EDGE_LOOP('',(#71881,#71882,#71883,#71884));
#28602=EDGE_LOOP('',(#71885,#71886,#71887,#71888));
#28603=EDGE_LOOP('',(#71889,#71890,#71891,#71892));
#28604=EDGE_LOOP('',(#71893,#71894,#71895,#71896));
#28605=EDGE_LOOP('',(#71897,#71898,#71899,#71900));
#28606=EDGE_LOOP('',(#71901,#71902,#71903,#71904));
#28607=EDGE_LOOP('',(#71905,#71906,#71907,#71908));
#28608=EDGE_LOOP('',(#71909,#71910,#71911,#71912));
#28609=EDGE_LOOP('',(#71913,#71914,#71915,#71916));
#28610=EDGE_LOOP('',(#71917,#71918,#71919,#71920));
#28611=EDGE_LOOP('',(#71921,#71922,#71923,#71924));
#28612=EDGE_LOOP('',(#71925,#71926,#71927,#71928));
#28613=EDGE_LOOP('',(#71929,#71930,#71931,#71932));
#28614=EDGE_LOOP('',(#71933,#71934,#71935,#71936));
#28615=EDGE_LOOP('',(#71937,#71938,#71939,#71940));
#28616=EDGE_LOOP('',(#71941,#71942,#71943,#71944));
#28617=EDGE_LOOP('',(#71945,#71946,#71947,#71948));
#28618=EDGE_LOOP('',(#71949,#71950,#71951,#71952));
#28619=EDGE_LOOP('',(#71953,#71954,#71955,#71956));
#28620=EDGE_LOOP('',(#71957,#71958,#71959,#71960));
#28621=EDGE_LOOP('',(#71961,#71962,#71963,#71964));
#28622=EDGE_LOOP('',(#71965,#71966,#71967,#71968));
#28623=EDGE_LOOP('',(#71969,#71970,#71971,#71972));
#28624=EDGE_LOOP('',(#71973,#71974,#71975,#71976));
#28625=EDGE_LOOP('',(#71977,#71978,#71979,#71980));
#28626=EDGE_LOOP('',(#71981,#71982,#71983,#71984));
#28627=EDGE_LOOP('',(#71985,#71986,#71987,#71988));
#28628=EDGE_LOOP('',(#71989,#71990,#71991,#71992));
#28629=EDGE_LOOP('',(#71993,#71994,#71995,#71996));
#28630=EDGE_LOOP('',(#71997,#71998,#71999,#72000));
#28631=EDGE_LOOP('',(#72001,#72002,#72003,#72004));
#28632=EDGE_LOOP('',(#72005,#72006,#72007,#72008));
#28633=EDGE_LOOP('',(#72009,#72010,#72011,#72012));
#28634=EDGE_LOOP('',(#72013,#72014,#72015,#72016));
#28635=EDGE_LOOP('',(#72017,#72018,#72019,#72020));
#28636=EDGE_LOOP('',(#72021,#72022,#72023,#72024));
#28637=EDGE_LOOP('',(#72025,#72026,#72027,#72028));
#28638=EDGE_LOOP('',(#72029,#72030,#72031,#72032));
#28639=EDGE_LOOP('',(#72033,#72034,#72035,#72036));
#28640=EDGE_LOOP('',(#72037,#72038,#72039,#72040));
#28641=EDGE_LOOP('',(#72041,#72042,#72043,#72044));
#28642=EDGE_LOOP('',(#72045,#72046,#72047,#72048));
#28643=EDGE_LOOP('',(#72049,#72050,#72051,#72052));
#28644=EDGE_LOOP('',(#72053,#72054,#72055,#72056));
#28645=EDGE_LOOP('',(#72057,#72058,#72059,#72060));
#28646=EDGE_LOOP('',(#72061,#72062,#72063,#72064));
#28647=EDGE_LOOP('',(#72065,#72066,#72067,#72068));
#28648=EDGE_LOOP('',(#72069,#72070,#72071,#72072));
#28649=EDGE_LOOP('',(#72073,#72074,#72075,#72076));
#28650=EDGE_LOOP('',(#72077,#72078,#72079,#72080));
#28651=EDGE_LOOP('',(#72081,#72082,#72083,#72084));
#28652=EDGE_LOOP('',(#72085,#72086,#72087,#72088));
#28653=EDGE_LOOP('',(#72089,#72090,#72091,#72092));
#28654=EDGE_LOOP('',(#72093,#72094,#72095,#72096));
#28655=EDGE_LOOP('',(#72097,#72098,#72099,#72100));
#28656=EDGE_LOOP('',(#72101,#72102,#72103,#72104));
#28657=EDGE_LOOP('',(#72105,#72106,#72107,#72108));
#28658=EDGE_LOOP('',(#72109,#72110,#72111,#72112));
#28659=EDGE_LOOP('',(#72113,#72114,#72115,#72116));
#28660=EDGE_LOOP('',(#72117,#72118,#72119,#72120));
#28661=EDGE_LOOP('',(#72121,#72122,#72123,#72124));
#28662=EDGE_LOOP('',(#72125,#72126,#72127,#72128));
#28663=EDGE_LOOP('',(#72129,#72130,#72131,#72132));
#28664=EDGE_LOOP('',(#72133,#72134,#72135,#72136));
#28665=EDGE_LOOP('',(#72137,#72138,#72139,#72140));
#28666=EDGE_LOOP('',(#72141,#72142,#72143,#72144));
#28667=EDGE_LOOP('',(#72145,#72146,#72147,#72148));
#28668=EDGE_LOOP('',(#72149,#72150,#72151,#72152));
#28669=EDGE_LOOP('',(#72153,#72154,#72155,#72156));
#28670=EDGE_LOOP('',(#72157,#72158,#72159,#72160));
#28671=EDGE_LOOP('',(#72161,#72162,#72163,#72164));
#28672=EDGE_LOOP('',(#72165,#72166,#72167,#72168));
#28673=EDGE_LOOP('',(#72169,#72170,#72171,#72172));
#28674=EDGE_LOOP('',(#72173,#72174,#72175,#72176));
#28675=EDGE_LOOP('',(#72177,#72178,#72179,#72180));
#28676=EDGE_LOOP('',(#72181,#72182,#72183,#72184));
#28677=EDGE_LOOP('',(#72185,#72186,#72187,#72188));
#28678=EDGE_LOOP('',(#72189,#72190,#72191,#72192));
#28679=EDGE_LOOP('',(#72193,#72194,#72195,#72196));
#28680=EDGE_LOOP('',(#72197,#72198,#72199,#72200));
#28681=EDGE_LOOP('',(#72201,#72202,#72203,#72204));
#28682=EDGE_LOOP('',(#72205,#72206,#72207,#72208));
#28683=EDGE_LOOP('',(#72209));
#28684=EDGE_LOOP('',(#72210));
#28685=EDGE_LOOP('',(#72211,#72212,#72213,#72214));
#28686=EDGE_LOOP('',(#72215,#72216,#72217,#72218));
#28687=EDGE_LOOP('',(#72219,#72220,#72221,#72222));
#28688=EDGE_LOOP('',(#72223,#72224,#72225,#72226));
#28689=EDGE_LOOP('',(#72227,#72228,#72229,#72230));
#28690=EDGE_LOOP('',(#72231,#72232,#72233,#72234));
#28691=EDGE_LOOP('',(#72235,#72236,#72237,#72238));
#28692=EDGE_LOOP('',(#72239,#72240,#72241,#72242,#72243,#72244));
#28693=EDGE_LOOP('',(#72245,#72246,#72247,#72248));
#28694=EDGE_LOOP('',(#72249,#72250,#72251,#72252,#72253,#72254));
#28695=EDGE_LOOP('',(#72255,#72256,#72257,#72258));
#28696=EDGE_LOOP('',(#72259,#72260,#72261,#72262));
#28697=EDGE_LOOP('',(#72263));
#28698=EDGE_LOOP('',(#72264));
#28699=EDGE_LOOP('',(#72265));
#28700=EDGE_LOOP('',(#72266,#72267,#72268,#72269));
#28701=EDGE_LOOP('',(#72270,#72271,#72272,#72273));
#28702=EDGE_LOOP('',(#72274,#72275,#72276,#72277));
#28703=EDGE_LOOP('',(#72278,#72279,#72280,#72281));
#28704=EDGE_LOOP('',(#72282,#72283,#72284,#72285));
#28705=EDGE_LOOP('',(#72286,#72287,#72288,#72289));
#28706=EDGE_LOOP('',(#72290,#72291,#72292,#72293));
#28707=EDGE_LOOP('',(#72294,#72295,#72296,#72297));
#28708=EDGE_LOOP('',(#72298,#72299,#72300,#72301));
#28709=EDGE_LOOP('',(#72302,#72303,#72304,#72305));
#28710=EDGE_LOOP('',(#72306,#72307,#72308,#72309));
#28711=EDGE_LOOP('',(#72310,#72311,#72312,#72313));
#28712=EDGE_LOOP('',(#72314,#72315,#72316,#72317));
#28713=EDGE_LOOP('',(#72318,#72319,#72320,#72321));
#28714=EDGE_LOOP('',(#72322,#72323,#72324,#72325));
#28715=EDGE_LOOP('',(#72326,#72327,#72328,#72329));
#28716=EDGE_LOOP('',(#72330,#72331,#72332,#72333));
#28717=EDGE_LOOP('',(#72334,#72335,#72336,#72337));
#28718=EDGE_LOOP('',(#72338,#72339,#72340,#72341));
#28719=EDGE_LOOP('',(#72342,#72343,#72344,#72345));
#28720=EDGE_LOOP('',(#72346,#72347,#72348,#72349));
#28721=EDGE_LOOP('',(#72350,#72351,#72352,#72353));
#28722=EDGE_LOOP('',(#72354,#72355,#72356,#72357));
#28723=EDGE_LOOP('',(#72358,#72359,#72360,#72361));
#28724=EDGE_LOOP('',(#72362,#72363,#72364,#72365));
#28725=EDGE_LOOP('',(#72366,#72367,#72368,#72369));
#28726=EDGE_LOOP('',(#72370,#72371,#72372,#72373));
#28727=EDGE_LOOP('',(#72374,#72375,#72376,#72377));
#28728=EDGE_LOOP('',(#72378,#72379,#72380,#72381));
#28729=EDGE_LOOP('',(#72382,#72383,#72384,#72385));
#28730=EDGE_LOOP('',(#72386,#72387,#72388,#72389));
#28731=EDGE_LOOP('',(#72390,#72391,#72392,#72393));
#28732=EDGE_LOOP('',(#72394,#72395,#72396,#72397));
#28733=EDGE_LOOP('',(#72398,#72399,#72400,#72401));
#28734=EDGE_LOOP('',(#72402,#72403,#72404,#72405));
#28735=EDGE_LOOP('',(#72406,#72407,#72408,#72409));
#28736=EDGE_LOOP('',(#72410,#72411,#72412,#72413));
#28737=EDGE_LOOP('',(#72414,#72415,#72416,#72417));
#28738=EDGE_LOOP('',(#72418,#72419,#72420,#72421));
#28739=EDGE_LOOP('',(#72422,#72423,#72424,#72425));
#28740=EDGE_LOOP('',(#72426,#72427,#72428,#72429));
#28741=EDGE_LOOP('',(#72430,#72431,#72432,#72433));
#28742=EDGE_LOOP('',(#72434,#72435,#72436,#72437));
#28743=EDGE_LOOP('',(#72438,#72439,#72440,#72441));
#28744=EDGE_LOOP('',(#72442,#72443,#72444,#72445));
#28745=EDGE_LOOP('',(#72446,#72447,#72448,#72449));
#28746=EDGE_LOOP('',(#72450,#72451,#72452,#72453));
#28747=EDGE_LOOP('',(#72454,#72455,#72456,#72457));
#28748=EDGE_LOOP('',(#72458,#72459,#72460,#72461));
#28749=EDGE_LOOP('',(#72462,#72463,#72464,#72465));
#28750=EDGE_LOOP('',(#72466,#72467,#72468,#72469));
#28751=EDGE_LOOP('',(#72470,#72471,#72472,#72473));
#28752=EDGE_LOOP('',(#72474,#72475,#72476,#72477));
#28753=EDGE_LOOP('',(#72478,#72479,#72480,#72481));
#28754=EDGE_LOOP('',(#72482,#72483,#72484,#72485));
#28755=EDGE_LOOP('',(#72486,#72487,#72488,#72489));
#28756=EDGE_LOOP('',(#72490,#72491,#72492,#72493));
#28757=EDGE_LOOP('',(#72494,#72495,#72496,#72497));
#28758=EDGE_LOOP('',(#72498,#72499,#72500,#72501));
#28759=EDGE_LOOP('',(#72502,#72503,#72504,#72505));
#28760=EDGE_LOOP('',(#72506,#72507,#72508,#72509));
#28761=EDGE_LOOP('',(#72510,#72511,#72512,#72513));
#28762=EDGE_LOOP('',(#72514,#72515,#72516,#72517));
#28763=EDGE_LOOP('',(#72518,#72519,#72520,#72521));
#28764=EDGE_LOOP('',(#72522,#72523,#72524,#72525));
#28765=EDGE_LOOP('',(#72526,#72527,#72528,#72529));
#28766=EDGE_LOOP('',(#72530,#72531,#72532,#72533));
#28767=EDGE_LOOP('',(#72534,#72535,#72536,#72537));
#28768=EDGE_LOOP('',(#72538,#72539,#72540,#72541));
#28769=EDGE_LOOP('',(#72542,#72543,#72544,#72545));
#28770=EDGE_LOOP('',(#72546,#72547,#72548,#72549));
#28771=EDGE_LOOP('',(#72550,#72551,#72552,#72553,#72554));
#28772=EDGE_LOOP('',(#72555,#72556,#72557,#72558,#72559));
#28773=EDGE_LOOP('',(#72560,#72561,#72562,#72563));
#28774=EDGE_LOOP('',(#72564,#72565,#72566,#72567));
#28775=EDGE_LOOP('',(#72568,#72569,#72570,#72571));
#28776=EDGE_LOOP('',(#72572,#72573,#72574,#72575));
#28777=EDGE_LOOP('',(#72576,#72577,#72578,#72579));
#28778=EDGE_LOOP('',(#72580,#72581,#72582,#72583));
#28779=EDGE_LOOP('',(#72584,#72585,#72586,#72587));
#28780=EDGE_LOOP('',(#72588,#72589,#72590,#72591));
#28781=EDGE_LOOP('',(#72592,#72593,#72594,#72595));
#28782=EDGE_LOOP('',(#72596,#72597,#72598,#72599));
#28783=EDGE_LOOP('',(#72600,#72601,#72602,#72603,#72604));
#28784=EDGE_LOOP('',(#72605,#72606,#72607,#72608));
#28785=EDGE_LOOP('',(#72609,#72610,#72611,#72612));
#28786=EDGE_LOOP('',(#72613,#72614,#72615,#72616));
#28787=EDGE_LOOP('',(#72617,#72618,#72619,#72620));
#28788=EDGE_LOOP('',(#72621,#72622,#72623,#72624));
#28789=EDGE_LOOP('',(#72625,#72626,#72627,#72628));
#28790=EDGE_LOOP('',(#72629,#72630,#72631,#72632));
#28791=EDGE_LOOP('',(#72633,#72634,#72635,#72636));
#28792=EDGE_LOOP('',(#72637,#72638,#72639,#72640));
#28793=EDGE_LOOP('',(#72641,#72642,#72643,#72644));
#28794=EDGE_LOOP('',(#72645,#72646,#72647,#72648));
#28795=EDGE_LOOP('',(#72649,#72650,#72651,#72652));
#28796=EDGE_LOOP('',(#72653,#72654,#72655,#72656));
#28797=EDGE_LOOP('',(#72657,#72658,#72659,#72660));
#28798=EDGE_LOOP('',(#72661,#72662,#72663,#72664));
#28799=EDGE_LOOP('',(#72665,#72666,#72667,#72668));
#28800=EDGE_LOOP('',(#72669,#72670,#72671,#72672));
#28801=EDGE_LOOP('',(#72673,#72674,#72675,#72676));
#28802=EDGE_LOOP('',(#72677,#72678,#72679,#72680));
#28803=EDGE_LOOP('',(#72681,#72682,#72683,#72684));
#28804=EDGE_LOOP('',(#72685,#72686,#72687,#72688));
#28805=EDGE_LOOP('',(#72689,#72690,#72691,#72692,#72693));
#28806=EDGE_LOOP('',(#72694,#72695,#72696,#72697));
#28807=EDGE_LOOP('',(#72698,#72699,#72700,#72701));
#28808=EDGE_LOOP('',(#72702,#72703,#72704,#72705));
#28809=EDGE_LOOP('',(#72706,#72707,#72708,#72709));
#28810=EDGE_LOOP('',(#72710,#72711,#72712,#72713));
#28811=EDGE_LOOP('',(#72714,#72715,#72716,#72717));
#28812=EDGE_LOOP('',(#72718,#72719,#72720,#72721));
#28813=EDGE_LOOP('',(#72722,#72723,#72724,#72725));
#28814=EDGE_LOOP('',(#72726,#72727,#72728,#72729));
#28815=EDGE_LOOP('',(#72730,#72731,#72732,#72733));
#28816=EDGE_LOOP('',(#72734,#72735,#72736,#72737));
#28817=EDGE_LOOP('',(#72738,#72739,#72740,#72741,#72742));
#28818=EDGE_LOOP('',(#72743,#72744,#72745,#72746));
#28819=EDGE_LOOP('',(#72747,#72748,#72749,#72750));
#28820=EDGE_LOOP('',(#72751,#72752,#72753,#72754));
#28821=EDGE_LOOP('',(#72755,#72756,#72757,#72758));
#28822=EDGE_LOOP('',(#72759,#72760,#72761,#72762));
#28823=EDGE_LOOP('',(#72763,#72764,#72765,#72766));
#28824=EDGE_LOOP('',(#72767,#72768,#72769,#72770));
#28825=EDGE_LOOP('',(#72771,#72772,#72773));
#28826=EDGE_LOOP('',(#72774,#72775,#72776,#72777));
#28827=EDGE_LOOP('',(#72778,#72779,#72780,#72781));
#28828=EDGE_LOOP('',(#72782,#72783,#72784));
#28829=EDGE_LOOP('',(#72785,#72786,#72787,#72788));
#28830=EDGE_LOOP('',(#72789,#72790,#72791,#72792));
#28831=EDGE_LOOP('',(#72793,#72794,#72795,#72796));
#28832=EDGE_LOOP('',(#72797,#72798,#72799,#72800));
#28833=EDGE_LOOP('',(#72801,#72802,#72803));
#28834=EDGE_LOOP('',(#72804,#72805,#72806));
#28835=EDGE_LOOP('',(#72807,#72808,#72809,#72810));
#28836=EDGE_LOOP('',(#72811,#72812,#72813,#72814));
#28837=EDGE_LOOP('',(#72815,#72816,#72817,#72818));
#28838=EDGE_LOOP('',(#72819,#72820,#72821,#72822));
#28839=EDGE_LOOP('',(#72823,#72824,#72825,#72826));
#28840=EDGE_LOOP('',(#72827,#72828,#72829,#72830));
#28841=EDGE_LOOP('',(#72831,#72832,#72833,#72834));
#28842=EDGE_LOOP('',(#72835,#72836,#72837,#72838));
#28843=EDGE_LOOP('',(#72839,#72840,#72841,#72842));
#28844=EDGE_LOOP('',(#72843,#72844,#72845,#72846));
#28845=EDGE_LOOP('',(#72847,#72848,#72849,#72850));
#28846=EDGE_LOOP('',(#72851,#72852,#72853));
#28847=EDGE_LOOP('',(#72854,#72855,#72856));
#28848=EDGE_LOOP('',(#72857,#72858,#72859,#72860));
#28849=EDGE_LOOP('',(#72861,#72862,#72863,#72864));
#28850=EDGE_LOOP('',(#72865,#72866,#72867,#72868));
#28851=EDGE_LOOP('',(#72869,#72870,#72871,#72872));
#28852=EDGE_LOOP('',(#72873,#72874,#72875,#72876,#72877));
#28853=EDGE_LOOP('',(#72878,#72879,#72880,#72881));
#28854=EDGE_LOOP('',(#72882,#72883,#72884,#72885));
#28855=EDGE_LOOP('',(#72886,#72887,#72888,#72889,#72890));
#28856=EDGE_LOOP('',(#72891,#72892,#72893,#72894));
#28857=EDGE_LOOP('',(#72895,#72896,#72897,#72898));
#28858=EDGE_LOOP('',(#72899,#72900,#72901,#72902));
#28859=EDGE_LOOP('',(#72903,#72904,#72905,#72906));
#28860=EDGE_LOOP('',(#72907,#72908,#72909,#72910));
#28861=EDGE_LOOP('',(#72911,#72912,#72913,#72914));
#28862=EDGE_LOOP('',(#72915,#72916,#72917,#72918));
#28863=EDGE_LOOP('',(#72919,#72920,#72921,#72922));
#28864=EDGE_LOOP('',(#72923,#72924,#72925,#72926));
#28865=EDGE_LOOP('',(#72927,#72928,#72929,#72930));
#28866=EDGE_LOOP('',(#72931,#72932,#72933,#72934,#72935));
#28867=EDGE_LOOP('',(#72936,#72937,#72938,#72939,#72940));
#28868=EDGE_LOOP('',(#72941,#72942,#72943,#72944));
#28869=EDGE_LOOP('',(#72945,#72946,#72947,#72948));
#28870=EDGE_LOOP('',(#72949,#72950,#72951,#72952));
#28871=EDGE_LOOP('',(#72953,#72954,#72955,#72956));
#28872=EDGE_LOOP('',(#72957,#72958,#72959,#72960));
#28873=EDGE_LOOP('',(#72961,#72962,#72963,#72964));
#28874=EDGE_LOOP('',(#72965,#72966,#72967,#72968));
#28875=EDGE_LOOP('',(#72969,#72970,#72971,#72972));
#28876=EDGE_LOOP('',(#72973,#72974,#72975,#72976));
#28877=EDGE_LOOP('',(#72977,#72978,#72979,#72980));
#28878=EDGE_LOOP('',(#72981,#72982,#72983,#72984,#72985));
#28879=EDGE_LOOP('',(#72986,#72987,#72988,#72989));
#28880=EDGE_LOOP('',(#72990,#72991,#72992,#72993));
#28881=EDGE_LOOP('',(#72994,#72995,#72996,#72997));
#28882=EDGE_LOOP('',(#72998,#72999,#73000,#73001));
#28883=EDGE_LOOP('',(#73002,#73003,#73004,#73005));
#28884=EDGE_LOOP('',(#73006,#73007,#73008,#73009));
#28885=EDGE_LOOP('',(#73010,#73011,#73012,#73013));
#28886=EDGE_LOOP('',(#73014,#73015,#73016,#73017));
#28887=EDGE_LOOP('',(#73018,#73019,#73020,#73021));
#28888=EDGE_LOOP('',(#73022,#73023,#73024,#73025));
#28889=EDGE_LOOP('',(#73026,#73027,#73028,#73029));
#28890=EDGE_LOOP('',(#73030,#73031,#73032,#73033));
#28891=EDGE_LOOP('',(#73034,#73035,#73036,#73037));
#28892=EDGE_LOOP('',(#73038,#73039,#73040,#73041));
#28893=EDGE_LOOP('',(#73042,#73043,#73044,#73045));
#28894=EDGE_LOOP('',(#73046,#73047,#73048,#73049));
#28895=EDGE_LOOP('',(#73050,#73051,#73052,#73053));
#28896=EDGE_LOOP('',(#73054,#73055,#73056,#73057));
#28897=EDGE_LOOP('',(#73058,#73059,#73060,#73061));
#28898=EDGE_LOOP('',(#73062,#73063,#73064,#73065));
#28899=EDGE_LOOP('',(#73066,#73067,#73068,#73069));
#28900=EDGE_LOOP('',(#73070,#73071,#73072,#73073));
#28901=EDGE_LOOP('',(#73074,#73075,#73076,#73077));
#28902=EDGE_LOOP('',(#73078,#73079,#73080,#73081));
#28903=EDGE_LOOP('',(#73082,#73083,#73084,#73085));
#28904=EDGE_LOOP('',(#73086,#73087,#73088,#73089));
#28905=EDGE_LOOP('',(#73090,#73091,#73092,#73093));
#28906=EDGE_LOOP('',(#73094,#73095,#73096,#73097));
#28907=EDGE_LOOP('',(#73098,#73099,#73100,#73101));
#28908=EDGE_LOOP('',(#73102,#73103,#73104,#73105));
#28909=EDGE_LOOP('',(#73106,#73107,#73108,#73109));
#28910=EDGE_LOOP('',(#73110,#73111,#73112,#73113));
#28911=EDGE_LOOP('',(#73114,#73115,#73116,#73117));
#28912=EDGE_LOOP('',(#73118,#73119,#73120,#73121));
#28913=EDGE_LOOP('',(#73122,#73123,#73124,#73125));
#28914=EDGE_LOOP('',(#73126,#73127,#73128,#73129));
#28915=EDGE_LOOP('',(#73130,#73131,#73132,#73133));
#28916=EDGE_LOOP('',(#73134,#73135,#73136,#73137));
#28917=EDGE_LOOP('',(#73138,#73139,#73140,#73141));
#28918=EDGE_LOOP('',(#73142,#73143,#73144,#73145));
#28919=EDGE_LOOP('',(#73146,#73147,#73148,#73149));
#28920=EDGE_LOOP('',(#73150,#73151,#73152,#73153));
#28921=EDGE_LOOP('',(#73154,#73155,#73156,#73157));
#28922=EDGE_LOOP('',(#73158,#73159,#73160,#73161));
#28923=EDGE_LOOP('',(#73162,#73163,#73164,#73165));
#28924=EDGE_LOOP('',(#73166,#73167,#73168,#73169));
#28925=EDGE_LOOP('',(#73170,#73171,#73172,#73173));
#28926=EDGE_LOOP('',(#73174,#73175,#73176,#73177));
#28927=EDGE_LOOP('',(#73178,#73179,#73180,#73181));
#28928=EDGE_LOOP('',(#73182,#73183,#73184,#73185));
#28929=EDGE_LOOP('',(#73186,#73187,#73188,#73189));
#28930=EDGE_LOOP('',(#73190,#73191,#73192,#73193));
#28931=EDGE_LOOP('',(#73194,#73195,#73196,#73197));
#28932=EDGE_LOOP('',(#73198,#73199,#73200,#73201));
#28933=EDGE_LOOP('',(#73202,#73203,#73204,#73205));
#28934=EDGE_LOOP('',(#73206,#73207,#73208,#73209));
#28935=EDGE_LOOP('',(#73210,#73211,#73212,#73213));
#28936=EDGE_LOOP('',(#73214,#73215,#73216,#73217));
#28937=EDGE_LOOP('',(#73218,#73219,#73220,#73221));
#28938=EDGE_LOOP('',(#73222,#73223,#73224,#73225));
#28939=EDGE_LOOP('',(#73226,#73227,#73228,#73229));
#28940=EDGE_LOOP('',(#73230,#73231,#73232,#73233));
#28941=EDGE_LOOP('',(#73234,#73235,#73236,#73237));
#28942=EDGE_LOOP('',(#73238,#73239,#73240,#73241));
#28943=EDGE_LOOP('',(#73242,#73243,#73244,#73245));
#28944=EDGE_LOOP('',(#73246,#73247,#73248,#73249));
#28945=EDGE_LOOP('',(#73250,#73251,#73252,#73253));
#28946=EDGE_LOOP('',(#73254,#73255,#73256,#73257));
#28947=EDGE_LOOP('',(#73258,#73259,#73260,#73261));
#28948=EDGE_LOOP('',(#73262,#73263,#73264,#73265));
#28949=EDGE_LOOP('',(#73266,#73267,#73268,#73269));
#28950=EDGE_LOOP('',(#73270,#73271,#73272,#73273));
#28951=EDGE_LOOP('',(#73274,#73275,#73276,#73277));
#28952=EDGE_LOOP('',(#73278,#73279,#73280,#73281));
#28953=EDGE_LOOP('',(#73282,#73283,#73284,#73285));
#28954=EDGE_LOOP('',(#73286,#73287,#73288,#73289));
#28955=EDGE_LOOP('',(#73290,#73291,#73292,#73293));
#28956=EDGE_LOOP('',(#73294,#73295,#73296,#73297));
#28957=EDGE_LOOP('',(#73298,#73299,#73300,#73301));
#28958=EDGE_LOOP('',(#73302,#73303,#73304,#73305));
#28959=EDGE_LOOP('',(#73306,#73307,#73308,#73309));
#28960=EDGE_LOOP('',(#73310));
#28961=EDGE_LOOP('',(#73311,#73312,#73313,#73314));
#28962=EDGE_LOOP('',(#73315,#73316,#73317,#73318));
#28963=EDGE_LOOP('',(#73319,#73320,#73321,#73322));
#28964=EDGE_LOOP('',(#73323,#73324,#73325,#73326));
#28965=EDGE_LOOP('',(#73327,#73328,#73329,#73330));
#28966=EDGE_LOOP('',(#73331,#73332,#73333,#73334));
#28967=EDGE_LOOP('',(#73335,#73336,#73337,#73338));
#28968=EDGE_LOOP('',(#73339,#73340,#73341,#73342));
#28969=EDGE_LOOP('',(#73343,#73344,#73345,#73346));
#28970=EDGE_LOOP('',(#73347,#73348,#73349,#73350));
#28971=EDGE_LOOP('',(#73351,#73352,#73353,#73354));
#28972=EDGE_LOOP('',(#73355,#73356,#73357,#73358));
#28973=EDGE_LOOP('',(#73359,#73360,#73361,#73362));
#28974=EDGE_LOOP('',(#73363,#73364,#73365,#73366));
#28975=EDGE_LOOP('',(#73367,#73368,#73369,#73370));
#28976=EDGE_LOOP('',(#73371,#73372,#73373,#73374));
#28977=EDGE_LOOP('',(#73375,#73376,#73377,#73378));
#28978=EDGE_LOOP('',(#73379,#73380,#73381,#73382));
#28979=EDGE_LOOP('',(#73383,#73384,#73385,#73386));
#28980=EDGE_LOOP('',(#73387,#73388,#73389,#73390));
#28981=EDGE_LOOP('',(#73391,#73392,#73393,#73394));
#28982=EDGE_LOOP('',(#73395,#73396,#73397,#73398));
#28983=EDGE_LOOP('',(#73399,#73400,#73401,#73402));
#28984=EDGE_LOOP('',(#73403,#73404,#73405,#73406));
#28985=EDGE_LOOP('',(#73407,#73408,#73409,#73410));
#28986=EDGE_LOOP('',(#73411,#73412,#73413,#73414));
#28987=EDGE_LOOP('',(#73415,#73416,#73417,#73418));
#28988=EDGE_LOOP('',(#73419,#73420,#73421,#73422));
#28989=EDGE_LOOP('',(#73423,#73424,#73425,#73426));
#28990=EDGE_LOOP('',(#73427,#73428,#73429,#73430));
#28991=EDGE_LOOP('',(#73431,#73432,#73433,#73434));
#28992=EDGE_LOOP('',(#73435,#73436,#73437,#73438));
#28993=EDGE_LOOP('',(#73439,#73440,#73441,#73442));
#28994=EDGE_LOOP('',(#73443,#73444,#73445,#73446));
#28995=EDGE_LOOP('',(#73447,#73448,#73449,#73450));
#28996=EDGE_LOOP('',(#73451,#73452,#73453,#73454));
#28997=EDGE_LOOP('',(#73455,#73456,#73457,#73458));
#28998=EDGE_LOOP('',(#73459,#73460,#73461,#73462));
#28999=EDGE_LOOP('',(#73463,#73464,#73465,#73466));
#29000=EDGE_LOOP('',(#73467,#73468,#73469,#73470));
#29001=EDGE_LOOP('',(#73471,#73472,#73473,#73474));
#29002=EDGE_LOOP('',(#73475,#73476,#73477,#73478));
#29003=EDGE_LOOP('',(#73479,#73480,#73481,#73482));
#29004=EDGE_LOOP('',(#73483,#73484,#73485,#73486));
#29005=EDGE_LOOP('',(#73487,#73488,#73489,#73490));
#29006=EDGE_LOOP('',(#73491,#73492,#73493,#73494));
#29007=EDGE_LOOP('',(#73495,#73496,#73497,#73498));
#29008=EDGE_LOOP('',(#73499,#73500,#73501,#73502));
#29009=EDGE_LOOP('',(#73503,#73504,#73505,#73506));
#29010=EDGE_LOOP('',(#73507,#73508,#73509,#73510));
#29011=EDGE_LOOP('',(#73511,#73512,#73513,#73514));
#29012=EDGE_LOOP('',(#73515,#73516,#73517,#73518));
#29013=EDGE_LOOP('',(#73519,#73520,#73521,#73522));
#29014=EDGE_LOOP('',(#73523,#73524,#73525,#73526));
#29015=EDGE_LOOP('',(#73527,#73528,#73529,#73530));
#29016=EDGE_LOOP('',(#73531,#73532,#73533,#73534));
#29017=EDGE_LOOP('',(#73535,#73536,#73537,#73538));
#29018=EDGE_LOOP('',(#73539,#73540,#73541,#73542));
#29019=EDGE_LOOP('',(#73543,#73544,#73545,#73546));
#29020=EDGE_LOOP('',(#73547,#73548,#73549,#73550));
#29021=EDGE_LOOP('',(#73551,#73552,#73553,#73554));
#29022=EDGE_LOOP('',(#73555,#73556,#73557,#73558));
#29023=EDGE_LOOP('',(#73559,#73560,#73561,#73562));
#29024=EDGE_LOOP('',(#73563,#73564,#73565,#73566));
#29025=EDGE_LOOP('',(#73567,#73568,#73569,#73570));
#29026=EDGE_LOOP('',(#73571,#73572,#73573,#73574));
#29027=EDGE_LOOP('',(#73575,#73576,#73577,#73578));
#29028=EDGE_LOOP('',(#73579,#73580,#73581,#73582));
#29029=EDGE_LOOP('',(#73583,#73584,#73585,#73586));
#29030=EDGE_LOOP('',(#73587,#73588,#73589,#73590));
#29031=EDGE_LOOP('',(#73591,#73592,#73593,#73594));
#29032=EDGE_LOOP('',(#73595,#73596,#73597,#73598));
#29033=EDGE_LOOP('',(#73599,#73600,#73601,#73602));
#29034=EDGE_LOOP('',(#73603,#73604,#73605,#73606));
#29035=EDGE_LOOP('',(#73607,#73608,#73609,#73610));
#29036=EDGE_LOOP('',(#73611,#73612,#73613,#73614));
#29037=EDGE_LOOP('',(#73615,#73616,#73617,#73618));
#29038=EDGE_LOOP('',(#73619,#73620,#73621,#73622));
#29039=EDGE_LOOP('',(#73623,#73624,#73625,#73626));
#29040=EDGE_LOOP('',(#73627,#73628,#73629,#73630));
#29041=EDGE_LOOP('',(#73631,#73632,#73633,#73634));
#29042=EDGE_LOOP('',(#73635,#73636,#73637,#73638));
#29043=EDGE_LOOP('',(#73639,#73640,#73641,#73642));
#29044=EDGE_LOOP('',(#73643,#73644,#73645,#73646));
#29045=EDGE_LOOP('',(#73647,#73648,#73649,#73650));
#29046=EDGE_LOOP('',(#73651,#73652,#73653,#73654));
#29047=EDGE_LOOP('',(#73655,#73656,#73657,#73658));
#29048=EDGE_LOOP('',(#73659,#73660,#73661,#73662));
#29049=EDGE_LOOP('',(#73663,#73664,#73665,#73666));
#29050=EDGE_LOOP('',(#73667,#73668,#73669,#73670));
#29051=EDGE_LOOP('',(#73671,#73672,#73673,#73674));
#29052=EDGE_LOOP('',(#73675,#73676,#73677,#73678));
#29053=EDGE_LOOP('',(#73679,#73680,#73681,#73682));
#29054=EDGE_LOOP('',(#73683,#73684,#73685,#73686));
#29055=EDGE_LOOP('',(#73687,#73688,#73689,#73690));
#29056=EDGE_LOOP('',(#73691,#73692,#73693,#73694));
#29057=EDGE_LOOP('',(#73695,#73696,#73697,#73698));
#29058=EDGE_LOOP('',(#73699,#73700,#73701,#73702));
#29059=EDGE_LOOP('',(#73703,#73704,#73705,#73706));
#29060=EDGE_LOOP('',(#73707,#73708,#73709,#73710));
#29061=EDGE_LOOP('',(#73711,#73712,#73713,#73714));
#29062=EDGE_LOOP('',(#73715,#73716,#73717,#73718));
#29063=EDGE_LOOP('',(#73719,#73720,#73721,#73722));
#29064=EDGE_LOOP('',(#73723,#73724,#73725,#73726));
#29065=EDGE_LOOP('',(#73727,#73728,#73729,#73730));
#29066=EDGE_LOOP('',(#73731,#73732,#73733,#73734));
#29067=EDGE_LOOP('',(#73735,#73736,#73737,#73738));
#29068=EDGE_LOOP('',(#73739,#73740,#73741,#73742));
#29069=EDGE_LOOP('',(#73743,#73744,#73745,#73746));
#29070=EDGE_LOOP('',(#73747,#73748,#73749,#73750));
#29071=EDGE_LOOP('',(#73751,#73752,#73753,#73754));
#29072=EDGE_LOOP('',(#73755,#73756,#73757,#73758));
#29073=EDGE_LOOP('',(#73759,#73760,#73761,#73762));
#29074=EDGE_LOOP('',(#73763,#73764,#73765,#73766));
#29075=EDGE_LOOP('',(#73767,#73768,#73769,#73770));
#29076=EDGE_LOOP('',(#73771,#73772,#73773,#73774));
#29077=EDGE_LOOP('',(#73775,#73776,#73777,#73778));
#29078=EDGE_LOOP('',(#73779,#73780,#73781,#73782));
#29079=EDGE_LOOP('',(#73783,#73784,#73785,#73786));
#29080=EDGE_LOOP('',(#73787,#73788,#73789,#73790));
#29081=EDGE_LOOP('',(#73791,#73792,#73793,#73794));
#29082=EDGE_LOOP('',(#73795,#73796,#73797,#73798));
#29083=EDGE_LOOP('',(#73799,#73800,#73801,#73802));
#29084=EDGE_LOOP('',(#73803,#73804,#73805,#73806));
#29085=EDGE_LOOP('',(#73807,#73808,#73809,#73810));
#29086=EDGE_LOOP('',(#73811,#73812,#73813,#73814));
#29087=EDGE_LOOP('',(#73815,#73816,#73817,#73818));
#29088=EDGE_LOOP('',(#73819,#73820,#73821,#73822));
#29089=EDGE_LOOP('',(#73823,#73824,#73825,#73826));
#29090=EDGE_LOOP('',(#73827,#73828,#73829,#73830));
#29091=EDGE_LOOP('',(#73831,#73832,#73833,#73834));
#29092=EDGE_LOOP('',(#73835,#73836,#73837,#73838));
#29093=EDGE_LOOP('',(#73839,#73840,#73841,#73842));
#29094=EDGE_LOOP('',(#73843,#73844,#73845,#73846));
#29095=EDGE_LOOP('',(#73847,#73848,#73849,#73850));
#29096=EDGE_LOOP('',(#73851,#73852,#73853,#73854));
#29097=EDGE_LOOP('',(#73855,#73856,#73857,#73858));
#29098=EDGE_LOOP('',(#73859,#73860,#73861,#73862));
#29099=EDGE_LOOP('',(#73863,#73864,#73865,#73866));
#29100=EDGE_LOOP('',(#73867,#73868,#73869,#73870));
#29101=EDGE_LOOP('',(#73871,#73872,#73873,#73874));
#29102=EDGE_LOOP('',(#73875,#73876,#73877,#73878));
#29103=EDGE_LOOP('',(#73879,#73880,#73881,#73882));
#29104=EDGE_LOOP('',(#73883,#73884,#73885,#73886));
#29105=EDGE_LOOP('',(#73887,#73888,#73889,#73890));
#29106=EDGE_LOOP('',(#73891,#73892,#73893,#73894));
#29107=EDGE_LOOP('',(#73895,#73896,#73897,#73898));
#29108=EDGE_LOOP('',(#73899,#73900,#73901,#73902));
#29109=EDGE_LOOP('',(#73903,#73904,#73905,#73906));
#29110=EDGE_LOOP('',(#73907,#73908,#73909,#73910));
#29111=EDGE_LOOP('',(#73911,#73912,#73913,#73914));
#29112=EDGE_LOOP('',(#73915,#73916,#73917,#73918));
#29113=EDGE_LOOP('',(#73919,#73920,#73921,#73922));
#29114=EDGE_LOOP('',(#73923,#73924,#73925,#73926));
#29115=EDGE_LOOP('',(#73927,#73928,#73929,#73930));
#29116=EDGE_LOOP('',(#73931,#73932,#73933,#73934));
#29117=EDGE_LOOP('',(#73935,#73936,#73937,#73938));
#29118=EDGE_LOOP('',(#73939,#73940,#73941,#73942));
#29119=EDGE_LOOP('',(#73943,#73944,#73945,#73946));
#29120=EDGE_LOOP('',(#73947,#73948,#73949,#73950));
#29121=EDGE_LOOP('',(#73951,#73952,#73953,#73954));
#29122=EDGE_LOOP('',(#73955,#73956,#73957,#73958));
#29123=EDGE_LOOP('',(#73959,#73960,#73961,#73962));
#29124=EDGE_LOOP('',(#73963,#73964,#73965,#73966));
#29125=EDGE_LOOP('',(#73967,#73968,#73969,#73970));
#29126=EDGE_LOOP('',(#73971,#73972,#73973,#73974));
#29127=EDGE_LOOP('',(#73975,#73976,#73977,#73978));
#29128=EDGE_LOOP('',(#73979,#73980,#73981,#73982));
#29129=EDGE_LOOP('',(#73983,#73984,#73985,#73986));
#29130=EDGE_LOOP('',(#73987,#73988,#73989,#73990));
#29131=EDGE_LOOP('',(#73991,#73992,#73993,#73994));
#29132=EDGE_LOOP('',(#73995,#73996,#73997,#73998));
#29133=EDGE_LOOP('',(#73999,#74000,#74001,#74002));
#29134=EDGE_LOOP('',(#74003,#74004,#74005,#74006));
#29135=EDGE_LOOP('',(#74007,#74008,#74009,#74010));
#29136=EDGE_LOOP('',(#74011,#74012,#74013,#74014));
#29137=EDGE_LOOP('',(#74015,#74016,#74017,#74018));
#29138=EDGE_LOOP('',(#74019,#74020,#74021,#74022));
#29139=EDGE_LOOP('',(#74023,#74024,#74025,#74026));
#29140=EDGE_LOOP('',(#74027,#74028,#74029,#74030));
#29141=EDGE_LOOP('',(#74031,#74032,#74033,#74034));
#29142=EDGE_LOOP('',(#74035,#74036,#74037,#74038));
#29143=EDGE_LOOP('',(#74039,#74040,#74041,#74042));
#29144=EDGE_LOOP('',(#74043,#74044,#74045,#74046));
#29145=EDGE_LOOP('',(#74047,#74048,#74049,#74050));
#29146=EDGE_LOOP('',(#74051,#74052,#74053,#74054));
#29147=EDGE_LOOP('',(#74055,#74056,#74057,#74058));
#29148=EDGE_LOOP('',(#74059,#74060,#74061,#74062));
#29149=EDGE_LOOP('',(#74063,#74064,#74065,#74066));
#29150=EDGE_LOOP('',(#74067,#74068,#74069,#74070));
#29151=EDGE_LOOP('',(#74071,#74072,#74073,#74074));
#29152=EDGE_LOOP('',(#74075,#74076,#74077,#74078));
#29153=EDGE_LOOP('',(#74079,#74080,#74081,#74082));
#29154=EDGE_LOOP('',(#74083,#74084,#74085,#74086));
#29155=EDGE_LOOP('',(#74087,#74088,#74089,#74090));
#29156=EDGE_LOOP('',(#74091,#74092,#74093,#74094));
#29157=EDGE_LOOP('',(#74095,#74096,#74097,#74098));
#29158=EDGE_LOOP('',(#74099,#74100,#74101,#74102));
#29159=EDGE_LOOP('',(#74103,#74104,#74105,#74106));
#29160=EDGE_LOOP('',(#74107,#74108,#74109,#74110));
#29161=EDGE_LOOP('',(#74111,#74112,#74113,#74114));
#29162=EDGE_LOOP('',(#74115,#74116,#74117,#74118));
#29163=EDGE_LOOP('',(#74119,#74120,#74121,#74122));
#29164=EDGE_LOOP('',(#74123,#74124,#74125,#74126));
#29165=EDGE_LOOP('',(#74127,#74128,#74129,#74130));
#29166=EDGE_LOOP('',(#74131,#74132,#74133,#74134));
#29167=EDGE_LOOP('',(#74135,#74136,#74137,#74138));
#29168=EDGE_LOOP('',(#74139,#74140,#74141,#74142));
#29169=EDGE_LOOP('',(#74143,#74144,#74145,#74146));
#29170=EDGE_LOOP('',(#74147,#74148,#74149,#74150));
#29171=EDGE_LOOP('',(#74151,#74152,#74153,#74154));
#29172=EDGE_LOOP('',(#74155,#74156,#74157,#74158));
#29173=EDGE_LOOP('',(#74159,#74160,#74161,#74162));
#29174=EDGE_LOOP('',(#74163,#74164,#74165,#74166));
#29175=EDGE_LOOP('',(#74167,#74168,#74169,#74170));
#29176=EDGE_LOOP('',(#74171,#74172,#74173,#74174));
#29177=EDGE_LOOP('',(#74175,#74176,#74177,#74178));
#29178=EDGE_LOOP('',(#74179,#74180,#74181,#74182));
#29179=EDGE_LOOP('',(#74183,#74184,#74185,#74186));
#29180=EDGE_LOOP('',(#74187,#74188,#74189,#74190));
#29181=EDGE_LOOP('',(#74191,#74192,#74193,#74194));
#29182=EDGE_LOOP('',(#74195,#74196,#74197,#74198));
#29183=EDGE_LOOP('',(#74199,#74200,#74201,#74202));
#29184=EDGE_LOOP('',(#74203,#74204,#74205,#74206));
#29185=EDGE_LOOP('',(#74207,#74208,#74209,#74210));
#29186=EDGE_LOOP('',(#74211,#74212,#74213,#74214));
#29187=EDGE_LOOP('',(#74215,#74216,#74217,#74218));
#29188=EDGE_LOOP('',(#74219,#74220,#74221,#74222));
#29189=EDGE_LOOP('',(#74223,#74224,#74225,#74226));
#29190=EDGE_LOOP('',(#74227,#74228,#74229,#74230));
#29191=EDGE_LOOP('',(#74231,#74232,#74233,#74234));
#29192=EDGE_LOOP('',(#74235,#74236,#74237,#74238));
#29193=EDGE_LOOP('',(#74239,#74240,#74241,#74242));
#29194=EDGE_LOOP('',(#74243,#74244,#74245,#74246));
#29195=EDGE_LOOP('',(#74247,#74248,#74249,#74250));
#29196=EDGE_LOOP('',(#74251,#74252,#74253,#74254));
#29197=EDGE_LOOP('',(#74255,#74256,#74257,#74258));
#29198=EDGE_LOOP('',(#74259,#74260,#74261,#74262));
#29199=EDGE_LOOP('',(#74263,#74264,#74265,#74266));
#29200=EDGE_LOOP('',(#74267,#74268,#74269,#74270));
#29201=EDGE_LOOP('',(#74271,#74272,#74273,#74274));
#29202=EDGE_LOOP('',(#74275,#74276,#74277,#74278));
#29203=EDGE_LOOP('',(#74279,#74280,#74281,#74282));
#29204=EDGE_LOOP('',(#74283,#74284,#74285,#74286));
#29205=EDGE_LOOP('',(#74287,#74288,#74289,#74290));
#29206=EDGE_LOOP('',(#74291,#74292,#74293,#74294));
#29207=EDGE_LOOP('',(#74295,#74296,#74297,#74298));
#29208=EDGE_LOOP('',(#74299,#74300,#74301,#74302));
#29209=EDGE_LOOP('',(#74303,#74304,#74305,#74306));
#29210=EDGE_LOOP('',(#74307,#74308,#74309,#74310));
#29211=EDGE_LOOP('',(#74311,#74312,#74313,#74314));
#29212=EDGE_LOOP('',(#74315,#74316,#74317,#74318));
#29213=EDGE_LOOP('',(#74319,#74320,#74321,#74322));
#29214=EDGE_LOOP('',(#74323,#74324,#74325,#74326));
#29215=EDGE_LOOP('',(#74327,#74328,#74329,#74330));
#29216=EDGE_LOOP('',(#74331,#74332,#74333,#74334));
#29217=EDGE_LOOP('',(#74335));
#29218=EDGE_LOOP('',(#74336));
#30298=B_SPLINE_CURVE_WITH_KNOTS('',3,(#183813,#183814,#183815,#183816,
#183817,#183818,#183819,#183820),.UNSPECIFIED.,.F.,.F.,(4,2,2,4),(1.98093781570329E-5,
0.435125302348886,0.651412660622268,0.869568218310475),.UNSPECIFIED.);
#30299=B_SPLINE_CURVE_WITH_KNOTS('',3,(#183826,#183827,#183828,#183829,
#183830,#183831,#183832,#183833,#183834,#183835,#183836,#183837,#183838,
#183839,#183840,#183841,#183842,#183843,#183844,#183845,#183846,#183847,
#183848,#183849,#183850,#183851,#183852,#183853,#183854,#183855,#183856,
#183857,#183858,#183859,#183860,#183861,#183862,#183863,#183864,#183865,
#183866,#183867,#183868,#183869,#183870,#183871,#183872,#183873,#183874,
#183875,#183876,#183877,#183878,#183879,#183880,#183881,#183882,#183883,
#183884,#183885,#183886,#183887,#183888,#183889,#183890,#183891,#183892,
#183893,#183894,#183895,#183896,#183897,#183898,#183899,#183900,#183901,
#183902,#183903,#183904,#183905,#183906,#183907),.UNSPECIFIED.,.F.,.F.,
(4,2,2,2,2,2,2,2,2,2,2,2,2,2,2,2,2,2,2,2,2,2,2,2,2,2,2,2,2,2,2,2,2,2,2,
2,2,2,2,2,4),(-25.3488773908543,-25.2117579765738,-25.0765301219692,-24.8121844159216,
-24.6100474871139,-24.4348153226359,-24.1591117730323,-23.9801715480672,
-23.7098723062826,-23.3436886097765,-23.124093349834,-22.9301004485503,
-22.713789244769,-22.5178484117983,-22.3445885926295,-22.1365517072343,
-21.9617467722256,-21.6860606757945,-21.5039208682341,-21.3209414773744,
-21.1435380906266,-20.8678762695796,-20.6933425591195,-20.4219590279459,
-20.0473764685859,-19.8294686500964,-19.6344958137531,-19.4185809489582,
-19.2224066058403,-19.0491319032085,-18.841195416967,-18.6663874275954,
-18.3907086523902,-18.2086415850464,-18.0255307566173,-17.8481495826963,
-17.5724951826215,-17.39794550316,-17.1265746270368,-16.7520562837938,-16.6093578201488),
 .UNSPECIFIED.);
#30300=B_SPLINE_CURVE_WITH_KNOTS('',3,(#183910,#183911,#183912,#183913,
#183914,#183915,#183916,#183917,#183918,#183919,#183920,#183921,#183922,
#183923,#183924,#183925,#183926,#183927,#183928,#183929,#183930,#183931,
#183932,#183933,#183934,#183935,#183936,#183937,#183938,#183939,#183940,
#183941,#183942,#183943,#183944,#183945,#183946,#183947,#183948,#183949,
#183950,#183951,#183952,#183953,#183954,#183955,#183956,#183957,#183958,
#183959,#183960,#183961,#183962,#183963),.UNSPECIFIED.,.F.,.F.,(4,2,2,2,
2,2,2,2,2,2,2,2,2,2,2,2,2,2,2,2,2,2,2,2,2,2,4),(6.63472946974546E-5,0.119852469453836,
0.240332488052986,0.471018335111722,0.81956291339417,1.09565454106518,1.45232143744692,
1.76752908522675,2.11369209864303,2.3742079135105,2.92100550850285,3.10718760089758,
3.45781086818677,3.68161712065895,4.03562600471986,4.40380054033367,4.58503323789667,
5.13378113052651,5.39299395323343,5.73656971192001,6.01538708479495,6.35675532647042,
6.57106600077119,7.02865050751105,7.31409315488209,7.65074778062276,8.07357000628427),
 .UNSPECIFIED.);
#30301=B_SPLINE_CURVE_WITH_KNOTS('',3,(#183968,#183969,#183970,#183971,
#183972,#183973,#183974,#183975,#183976,#183977,#183978,#183979,#183980,
#183981,#183982,#183983,#183984,#183985,#183986,#183987,#183988,#183989,
#183990,#183991,#183992,#183993,#183994,#183995,#183996,#183997,#183998,
#183999,#184000,#184001,#184002,#184003,#184004,#184005,#184006,#184007,
#184008,#184009,#184010,#184011,#184012,#184013,#184014,#184015,#184016,
#184017,#184018,#184019,#184020,#184021,#184022,#184023,#184024,#184025,
#184026,#184027,#184028,#184029,#184030,#184031,#184032,#184033,#184034,
#184035,#184036,#184037,#184038,#184039,#184040,#184041,#184042,#184043,
#184044,#184045,#184046,#184047,#184048,#184049,#184050,#184051,#184052,
#184053),.UNSPECIFIED.,.F.,.F.,(4,2,2,2,2,2,2,2,2,2,2,2,2,2,2,2,2,2,2,2,
2,2,2,2,2,2,2,2,2,2,2,2,2,2,2,2,2,2,2,2,2,2,4),(-16.6093578201488,-16.5792653081084,
-16.3688617948715,-16.1942583158352,-15.9185937912375,-15.7341679467037,
-15.510329013096,-15.3337592978338,-15.1376405428431,-14.9617442945232,
-14.6860653778253,-14.5088808638798,-14.2381796190777,-13.8692442892602,
-13.6966458427509,-13.4851560245841,-13.3106424775729,-13.0349964870432,
-12.8479009746796,-12.6740346954215,-12.5002332859473,-12.3138240226037,
-12.0381735405829,-11.8636493211966,-11.6522937409599,-11.4796727640309,
-11.110050570064,-10.8392528782752,-10.6624476167363,-10.4372172998725,
-10.2537939564926,-9.97812630303468,-9.80345503736936,-9.59390281924938,
-9.42095531055332,-9.22887410887228,-9.00592036679354,-8.73026742422095,
-8.5488309202539,-8.38217370714925,-8.1948770877202,-7.91922350740144,-7.87061597992456),
 .UNSPECIFIED.);
#30302=B_SPLINE_CURVE_WITH_KNOTS('',3,(#184054,#184055,#184056,#184057,
#184058,#184059,#184060,#184061,#184062,#184063,#184064,#184065,#184066,
#184067,#184068,#184069,#184070,#184071,#184072,#184073,#184074,#184075,
#184076,#184077,#184078,#184079,#184080,#184081,#184082,#184083,#184084,
#184085,#184086,#184087,#184088,#184089,#184090,#184091,#184092,#184093,
#184094,#184095,#184096,#184097,#184098,#184099,#184100,#184101,#184102,
#184103,#184104,#184105,#184106,#184107,#184108,#184109,#184110,#184111,
#184112,#184113,#184114,#184115,#184116,#184117,#184118,#184119,#184120,
#184121,#184122,#184123,#184124,#184125,#184126,#184127,#184128,#184129,
#184130,#184131,#184132,#184133,#184134,#184135,#184136,#184137,#184138,
#184139,#184140,#184141,#184142,#184143,#184144,#184145,#184146,#184147,
#184148,#184149,#184150,#184151,#184152,#184153,#184154,#184155,#184156,
#184157,#184158,#184159,#184160,#184161),.UNSPECIFIED.,.F.,.F.,(4,2,2,2,
2,2,2,2,2,2,2,2,2,2,2,2,2,2,2,2,2,2,2,2,2,2,2,2,2,2,2,2,2,2,2,2,2,2,2,2,
2,2,2,2,2,2,2,2,2,2,2,2,2,4),(-8.73899861150267,-8.69914480337356,-8.54464421100673,
-8.39572763166509,-8.23116510095003,-8.04330833686929,-7.89530357788577,
-7.71444490512931,-7.63218540045482,-7.34190189330136,-7.18731818512391,
-7.03875298532148,-6.87440872067566,-6.68634926779794,-6.53835803539044,
-6.3574461866764,-6.27519062631498,-5.98491286681858,-5.83033369014256,
-5.68177659125073,-5.51744048167933,-5.32938533228556,-5.18139964121957,
-5.00049251951509,-4.91823952559342,-4.627971678843,-4.47339685583356,-4.32484684565646,
-4.16051662597844,-3.9724686670833,-3.82448853460015,-3.64358883675198,
-3.56134283666075,-3.27107437284463,-3.11651405924174,-2.96793565491532,
-2.80344671651332,-2.6155305073513,-2.46749047947249,-2.28682286631188,
-2.20469916989341,-1.91428724602398,-1.76006360631775,-1.61059279284905,
-1.52984381579783,-1.23251915858275,-1.07535085998026,-0.928129335387397,
-0.845106454401542,-0.561534774960734,-0.41156192518634,-0.314806053587988,
-0.213628494228944,-4.30320540010522E-5),.UNSPECIFIED.);
#30303=B_SPLINE_CURVE_WITH_KNOTS('',3,(#184168,#184169,#184170,#184171,
#184172,#184173,#184174,#184175,#184176,#184177,#184178,#184179,#184180,
#184181,#184182,#184183,#184184,#184185,#184186,#184187,#184188,#184189,
#184190,#184191,#184192,#184193,#184194,#184195,#184196,#184197,#184198,
#184199,#184200,#184201,#184202,#184203,#184204,#184205,#184206,#184207,
#184208,#184209,#184210,#184211,#184212,#184213,#184214,#184215,#184216,
#184217,#184218,#184219,#184220,#184221,#184222,#184223,#184224,#184225,
#184226,#184227,#184228,#184229,#184230,#184231,#184232,#184233,#184234,
#184235,#184236,#184237,#184238,#184239,#184240,#184241),.UNSPECIFIED.,
 .F.,.F.,(4,2,2,2,2,2,2,2,2,2,2,2,2,2,2,2,2,2,2,2,2,2,2,2,2,2,2,2,2,2,2,
2,2,2,2,2,4),(-7.87061597992456,-7.74470628455937,-7.53319093454486,-7.36059066540921,
-6.99174256274364,-6.72104629906109,-6.54380121348743,-6.26811290449752,
-6.0922320395682,-5.8959050199953,-5.719400421899,-5.49597956919839,-5.31123334622609,
-5.03556141350746,-4.86096963377401,-4.65034766871294,-4.47758950715269,
-4.10414504573837,-3.83287387892188,-3.65788145499446,-3.44503513096825,
-3.25094276997586,-2.97525557236685,-2.80045632747259,-2.59234243153645,
-2.41909859753841,-2.22334257313634,-2.00672459368894,-1.81352307443079,
-1.59254980365457,-1.23297515385466,-0.963874962372695,-0.779853288355305,
-0.585014064424859,-0.293134115374441,-0.147808546265094,-9.31271228427911E-6),
 .UNSPECIFIED.);
#30304=B_SPLINE_CURVE_WITH_KNOTS('',3,(#184242,#184243,#184244,#184245,
#184246,#184247,#184248,#184249,#184250,#184251,#184252,#184253,#184254,
#184255,#184256,#184257,#184258,#184259,#184260,#184261,#184262,#184263,
#184264,#184265,#184266,#184267,#184268,#184269,#184270,#184271,#184272,
#184273,#184274,#184275,#184276,#184277,#184278,#184279,#184280,#184281,
#184282,#184283,#184284,#184285,#184286,#184287,#184288,#184289,#184290,
#184291,#184292,#184293,#184294,#184295,#184296,#184297,#184298,#184299,
#184300,#184301,#184302,#184303,#184304,#184305,#184306,#184307,#184308,
#184309,#184310,#184311,#184312,#184313,#184314,#184315,#184316,#184317,
#184318,#184319,#184320,#184321,#184322,#184323,#184324,#184325,#184326,
#184327,#184328,#184329,#184330,#184331,#184332,#184333,#184334,#184335,
#184336,#184337,#184338,#184339,#184340,#184341,#184342,#184343,#184344,
#184345,#184346,#184347),.UNSPECIFIED.,.F.,.F.,(4,2,2,2,2,2,2,2,2,2,2,2,
2,2,2,2,2,2,2,2,2,2,2,2,2,2,2,2,2,2,2,2,2,2,2,2,2,2,2,2,2,2,2,2,2,2,2,2,
2,2,2,2,4),(-17.4782773446469,-17.3145507638988,-17.2323097895944,-17.0514231256051,
-16.9034535217882,-16.7154162229866,-16.5510957447174,-16.4025567378387,
-16.2479928964372,-15.9577428595964,-15.8754948526675,-15.6946006751635,
-15.5466254429558,-15.3585808507769,-15.1942544180056,-15.045708273596,
-14.8911399994233,-14.6008798764381,-14.5186292733015,-14.3377298054029,
-14.1897490289545,-14.0016983511229,-13.8373654025521,-13.6888138885248,
-13.5342402921702,-13.2439697088235,-13.1617163401424,-12.9808071777748,
-12.8328216847827,-12.6447522100799,-12.4804258903256,-12.3318894677204,
-12.1773052701961,-11.886991386448,-11.8047439638111,-11.62342288253,-11.4754890658908,
-11.2859093990368,-11.1230831642647,-10.9770480843857,-10.8218072863131,
-10.5274988371903,-10.4462882197963,-10.2870405659291,-10.1350158954007,
-9.86489557230041,-9.77667896000119,-9.58326202343803,-9.43586173011933,
-9.22167535505261,-9.0712847440584,-8.98887090232673,-8.73899861150267),
 .UNSPECIFIED.);
#30305=B_SPLINE_CURVE_WITH_KNOTS('',3,(#184367,#184368,#184369,#184370,
#184371,#184372,#184373,#184374,#184375,#184376,#184377,#184378,#184379,
#184380,#184381,#184382,#184383,#184384),.UNSPECIFIED.,.F.,.F.,(4,2,2,2,
2,2,2,2,4),(0.118255944796295,0.150196749040088,0.182137553283882,0.210325561008924,
0.238513568733966,0.266701576459009,0.294889584184051,0.326830388427845,
0.358771192671638),.UNSPECIFIED.);
#30306=B_SPLINE_CURVE_WITH_KNOTS('',3,(#184388,#184389,#184390,#184391,
#184392,#184393,#184394,#184395,#184396,#184397,#184398,#184399,#184400,
#184401,#184402,#184403,#184404,#184405),.UNSPECIFIED.,.F.,.F.,(4,2,2,2,
2,2,2,2,4),(-0.357545008588623,-0.325833280361292,-0.294121552133961,-0.265932611678201,
-0.237743671222442,-0.209554730766682,-0.181365790310923,-0.149654062083592,
-0.117942333856262),.UNSPECIFIED.);
#30307=B_SPLINE_CURVE_WITH_KNOTS('',3,(#184410,#184411,#184412,#184413,
#184414,#184415,#184416,#184417,#184418,#184419,#184420,#184421,#184422,
#184423,#184424,#184425,#184426,#184427),.UNSPECIFIED.,.F.,.F.,(4,2,2,2,
2,2,2,2,4),(-0.357545008588621,-0.325833280361291,-0.29412155213396,-0.265932611678201,
-0.237743671222441,-0.209554730766681,-0.181365790310922,-0.149654062083591,
-0.117942333856259),.UNSPECIFIED.);
#30308=B_SPLINE_CURVE_WITH_KNOTS('',3,(#184431,#184432,#184433,#184434,
#184435,#184436,#184437,#184438,#184439,#184440,#184441,#184442,#184443,
#184444,#184445,#184446,#184447,#184448),.UNSPECIFIED.,.F.,.F.,(4,2,2,2,
2,2,2,2,4),(-0.358783917084611,-0.327792365271302,-0.296800813457993,-0.26765719109598,
-0.238513568733966,-0.210325561008924,-0.182137553283882,-0.150196749040089,
-0.118255944796295),.UNSPECIFIED.);
#30309=B_SPLINE_CURVE_WITH_KNOTS('',3,(#184456,#184457,#184458,#184459,
#184460,#184461,#184462,#184463,#184464,#184465,#184466,#184467,#184468,
#184469,#184470,#184471,#184472,#184473,#184474),.UNSPECIFIED.,.F.,.F.,
(4,2,2,2,3,2,2,2,4),(-0.120257623937773,-0.0883168196939601,-0.0563760154501472,
-0.0281880077250899,-3.25711679849405E-14,0.0281880077250248,0.0563760154500821,
0.0883168196938949,0.120257623937708),.UNSPECIFIED.);
#30310=B_SPLINE_CURVE_WITH_KNOTS('',3,(#184486,#184487,#184488,#184489,
#184490,#184491,#184492,#184493,#184494,#184495,#184496,#184497,#184498,
#184499,#184500,#184501,#184502,#184503),.UNSPECIFIED.,.F.,.F.,(4,2,2,2,
2,2,2,2,4),(-0.358786911659494,-0.3268461074157,-0.294905303171906,-0.266717295446863,
-0.238529287721821,-0.209385665359807,-0.180242042997794,-0.149250491184484,
-0.118258939371175),.UNSPECIFIED.);
#30311=B_SPLINE_CURVE_WITH_KNOTS('',3,(#184506,#184507,#184508,#184509,
#184510,#184511,#184512,#184513,#184514,#184515,#184516,#184517,#184518,
#184519,#184520,#184521,#184522,#184523,#184524),.UNSPECIFIED.,.F.,.F.,
(4,2,2,2,3,2,2,2,4),(-0.120257623937686,-0.0883168196938895,-0.0563760154500934,
-0.0281880077250492,-5.10702591327572E-15,0.0281880077250392,0.0563760154500835,
0.0883168196938795,0.120257623937675),.UNSPECIFIED.);
#30312=B_SPLINE_CURVE_WITH_KNOTS('',3,(#184529,#184530,#184531,#184532,
#184533,#184534,#184535,#184536,#184537,#184538,#184539,#184540,#184541,
#184542,#184543,#184544,#184545,#184546),.UNSPECIFIED.,.F.,.F.,(4,2,2,2,
2,2,2,2,4),(-0.358783917084615,-0.327792365271305,-0.296800813457996,-0.267657191095982,
-0.238513568733968,-0.210325561008926,-0.182137553283884,-0.150196749040089,
-0.118255944796295),.UNSPECIFIED.);
#30313=B_SPLINE_CURVE_WITH_KNOTS('',3,(#184549,#184550,#184551,#184552,
#184553,#184554,#184555,#184556,#184557,#184558,#184559,#184560,#184561,
#184562,#184563,#184564,#184565,#184566,#184567),.UNSPECIFIED.,.F.,.F.,
(4,2,2,2,3,2,2,2,4),(0.356772508105138,0.388713312348931,0.420654116592725,
0.448842124317767,0.477030132042809,0.505218139767852,0.533406147492894,
0.565346951736688,0.597287755980482),.UNSPECIFIED.);
#30314=B_SPLINE_CURVE_WITH_KNOTS('',3,(#184571,#184572,#184573,#184574,
#184575,#184576,#184577,#184578,#184579,#184580,#184581,#184582,#184583,
#184584,#184585,#184586,#184587,#184588,#184589),.UNSPECIFIED.,.F.,.F.,
(4,2,2,2,3,2,2,2,4),(0.35677250810512,0.388713312348932,0.420654116592744,
0.448842124317802,0.477030132042859,0.505218139767916,0.533406147492973,
0.565346951736786,0.597287755980598),.UNSPECIFIED.);
#30315=B_SPLINE_CURVE_WITH_KNOTS('',3,(#184594,#184595,#184596,#184597,
#184598,#184599,#184600,#184601,#184602,#184603,#184604,#184605,#184606,
#184607,#184608,#184609,#184610,#184611),.UNSPECIFIED.,.F.,.F.,(4,2,2,2,
2,2,2,2,4),(-0.357556076431055,-0.326734510063867,-0.29591294369668,-0.266828307459561,
-0.237743671222443,-0.209554730766684,-0.181365790310925,-0.149654062083593,
-0.117942333856261),.UNSPECIFIED.);
#30316=B_SPLINE_CURVE_WITH_KNOTS('',3,(#184618,#184619,#184620,#184621,
#184622,#184623,#184624,#184625,#184626,#184627,#184628,#184629,#184630,
#184631,#184632,#184633,#184634,#184635),.UNSPECIFIED.,.F.,.F.,(4,2,2,2,
2,2,2,2,4),(-0.357558765732128,-0.325847037504796,-0.294135309277465,-0.265946368821705,
-0.237757428365946,-0.208672792128828,-0.17958815589171,-0.148766589524522,
-0.117945023157334),.UNSPECIFIED.);
#30317=B_SPLINE_CURVE_WITH_KNOTS('',3,(#184645,#184646,#184647,#184648,
#184649,#184650,#184651,#184652,#184653,#184654,#184655,#184656,#184657,
#184658,#184659,#184660,#184661,#184662,#184663),.UNSPECIFIED.,.F.,.F.,
(4,2,2,2,3,2,2,2,4),(-0.119801337366205,-0.0880896091388694,-0.0563778809115339,
-0.0281889404557727,-1.15601972439094E-14,0.02818894045575,0.0563778809115115,
0.0880896091388471,0.119801337366183),.UNSPECIFIED.);
#30318=B_SPLINE_CURVE_WITH_KNOTS('',3,(#184675,#184676,#184677,#184678,
#184679,#184680,#184681,#184682,#184683,#184684,#184685,#184686,#184687,
#184688,#184689,#184690,#184691,#184692,#184693),.UNSPECIFIED.,.F.,.F.,
(4,2,2,2,3,2,2,2,4),(-0.119812405208569,-0.0889908388413916,-0.0581692724742138,
-0.0290846362371043,5.25968157916168E-15,0.0281889404557555,0.0563778809115058,
0.0880896091388275,0.119801337366149),.UNSPECIFIED.);
#30319=B_SPLINE_CURVE_WITH_KNOTS('',3,(#184698,#184699,#184700,#184701,
#184702,#184703,#184704,#184705,#184706,#184707,#184708,#184709,#184710,
#184711,#184712,#184713,#184714,#184715,#184716),.UNSPECIFIED.,.F.,.F.,
(4,2,2,2,3,2,2,2,4),(-0.119801337366148,-0.0880896091388235,-0.0563778809114992,
-0.028188940455747,5.14865927669916E-15,0.0290846362371171,0.0581692724742291,
0.0889908388414093,0.11981240520859),.UNSPECIFIED.);
#30320=B_SPLINE_CURVE_WITH_KNOTS('',3,(#184721,#184722,#184723,#184724,
#184725,#184726,#184727,#184728,#184729,#184730,#184731,#184732,#184733,
#184734,#184735,#184736,#184737,#184738,#184739),.UNSPECIFIED.,.F.,.F.,
(4,2,2,2,3,2,2,2,4),(-0.119801337366183,-0.0880896091388476,-0.0563778809115119,
-0.0281889404557501,1.15879528195251E-14,0.0281889404557729,0.0563778809115343,
0.08808960913887,0.119801337366206),.UNSPECIFIED.);
#30321=B_SPLINE_CURVE_WITH_KNOTS('',3,(#184812,#184813,#184814,#184815,
#184816,#184817,#184818,#184819,#184820,#184821,#184822,#184823,#184824,
#184825,#184826,#184827,#184828,#184829,#184830,#184831,#184832,#184833,
#184834,#184835,#184836,#184837,#184838,#184839,#184840,#184841,#184842,
#184843,#184844,#184845,#184846,#184847,#184848,#184849,#184850,#184851,
#184852,#184853,#184854,#184855,#184856,#184857,#184858,#184859,#184860,
#184861,#184862,#184863,#184864,#184865,#184866,#184867),.UNSPECIFIED.,
 .F.,.F.,(4,2,2,2,2,2,2,2,2,2,2,2,2,2,2,2,2,2,2,2,2,2,2,2,2,2,2,4),(1.00000000824441E-6,
0.275071439947967,0.543589949820334,0.726708281005337,0.964982097293981,
1.23327523189536,1.50260089643556,1.77224618743942,2.03912144009645,2.30999928062765,
2.57411052670835,2.84582268677525,3.10783768543331,3.37967001978092,3.6453167716663,
3.9093743140936,4.17506210086737,4.43697141321252,4.70280662599637,4.96284365192071,
5.09444162419176,5.36127414381699,5.62123954982782,5.88473753210837,6.10516180647631,
6.44201482456383,6.60698025662302,6.77613368119588),.UNSPECIFIED.);
#30322=B_SPLINE_CURVE_WITH_KNOTS('',3,(#184871,#184872,#184873,#184874,
#184875,#184876,#184877,#184878,#184879,#184880,#184881,#184882,#184883,
#184884,#184885,#184886,#184887,#184888,#184889,#184890,#184891,#184892,
#184893,#184894,#184895,#184896,#184897,#184898,#184899,#184900,#184901),
 .UNSPECIFIED.,.F.,.F.,(4,3,3,3,3,3,3,3,3,3,4),(0.,0.0699423398648104,0.139991703689476,
0.15887188919288,0.241543521732975,0.317743778385759,0.397179722982199,
0.476615667578639,0.551702197147984,0.590430876649392,0.635487556771519),
 .UNSPECIFIED.);
#30323=B_SPLINE_CURVE_WITH_KNOTS('',3,(#184902,#184903,#184904,#184905,
#184906,#184907),.UNSPECIFIED.,.F.,.F.,(4,2,4),(0.635487559214341,0.817743778385759,
1.),.UNSPECIFIED.);
#30324=B_SPLINE_CURVE_WITH_KNOTS('',3,(#185056,#185057,#185058,#185059,
#185060,#185061,#185062,#185063,#185064,#185065,#185066,#185067,#185068,
#185069,#185070,#185071,#185072,#185073,#185074,#185075,#185076,#185077,
#185078,#185079,#185080,#185081,#185082,#185083,#185084,#185085,#185086,
#185087,#185088,#185089,#185090,#185091,#185092,#185093,#185094,#185095,
#185096,#185097,#185098,#185099,#185100,#185101,#185102,#185103,#185104,
#185105,#185106,#185107,#185108,#185109,#185110,#185111,#185112,#185113,
#185114,#185115,#185116,#185117,#185118,#185119,#185120,#185121,#185122,
#185123,#185124,#185125,#185126,#185127,#185128,#185129,#185130,#185131,
#185132,#185133,#185134,#185135,#185136,#185137,#185138,#185139,#185140,
#185141,#185142,#185143,#185144,#185145,#185146,#185147,#185148,#185149,
#185150,#185151,#185152,#185153,#185154,#185155,#185156,#185157,#185158,
#185159,#185160,#185161,#185162,#185163,#185164,#185165,#185166,#185167,
#185168,#185169,#185170,#185171,#185172,#185173,#185174,#185175,#185176,
#185177,#185178,#185179,#185180,#185181,#185182,#185183,#185184,#185185,
#185186,#185187,#185188,#185189,#185190,#185191,#185192,#185193,#185194,
#185195,#185196,#185197,#185198,#185199,#185200,#185201,#185202,#185203,
#185204,#185205,#185206,#185207,#185208,#185209,#185210,#185211,#185212,
#185213,#185214,#185215,#185216,#185217,#185218,#185219,#185220,#185221,
#185222,#185223,#185224,#185225,#185226,#185227,#185228,#185229,#185230,
#185231,#185232,#185233,#185234,#185235,#185236,#185237,#185238,#185239,
#185240,#185241,#185242,#185243,#185244,#185245,#185246,#185247,#185248,
#185249,#185250,#185251,#185252,#185253,#185254,#185255,#185256,#185257,
#185258,#185259,#185260,#185261,#185262,#185263,#185264,#185265,#185266,
#185267,#185268,#185269,#185270,#185271,#185272,#185273,#185274,#185275,
#185276,#185277,#185278,#185279,#185280,#185281,#185282,#185283,#185284,
#185285,#185286,#185287,#185288,#185289,#185290,#185291,#185292,#185293,
#185294,#185295,#185296,#185297,#185298,#185299,#185300,#185301,#185302,
#185303,#185304,#185305,#185306,#185307,#185308,#185309,#185310,#185311,
#185312,#185313,#185314,#185315,#185316,#185317,#185318,#185319,#185320,
#185321,#185322,#185323,#185324,#185325,#185326,#185327,#185328,#185329,
#185330,#185331,#185332,#185333,#185334,#185335,#185336,#185337,#185338,
#185339,#185340,#185341,#185342,#185343,#185344,#185345,#185346,#185347,
#185348,#185349,#185350,#185351,#185352,#185353,#185354,#185355,#185356,
#185357,#185358,#185359,#185360,#185361,#185362,#185363,#185364,#185365,
#185366,#185367,#185368,#185369,#185370,#185371,#185372,#185373,#185374,
#185375,#185376,#185377,#185378,#185379,#185380,#185381,#185382,#185383,
#185384,#185385,#185386,#185387,#185388,#185389,#185390,#185391,#185392,
#185393,#185394,#185395,#185396,#185397,#185398,#185399,#185400,#185401,
#185402,#185403,#185404,#185405,#185406,#185407,#185408,#185409,#185410,
#185411,#185412,#185413,#185414,#185415,#185416,#185417,#185418,#185419,
#185420,#185421,#185422,#185423,#185424,#185425,#185426,#185427,#185428,
#185429,#185430,#185431,#185432,#185433,#185434,#185435,#185436,#185437,
#185438,#185439,#185440,#185441,#185442,#185443,#185444,#185445,#185446,
#185447,#185448,#185449,#185450,#185451,#185452,#185453,#185454,#185455,
#185456,#185457,#185458,#185459,#185460,#185461,#185462,#185463,#185464,
#185465,#185466,#185467,#185468,#185469,#185470,#185471,#185472,#185473,
#185474,#185475,#185476,#185477,#185478,#185479),.UNSPECIFIED.,.F.,.F.,
(4,2,2,2,2,2,2,2,2,2,2,2,2,2,2,2,2,2,2,2,2,2,2,2,2,2,2,2,2,2,2,2,2,2,2,
2,2,2,2,2,2,2,2,2,2,2,2,2,2,2,2,2,2,2,2,2,2,2,2,2,2,2,2,2,2,2,2,2,2,2,2,
2,2,2,2,2,2,2,2,2,2,2,2,2,2,2,2,2,2,2,2,2,2,2,2,2,2,2,2,2,2,2,2,2,2,2,2,
2,2,2,2,2,2,2,2,2,2,2,2,2,2,2,2,2,2,2,2,2,2,2,2,2,2,2,2,2,2,2,2,2,2,2,2,
2,2,2,2,2,2,2,2,2,2,2,2,2,2,2,2,2,2,2,2,2,2,2,2,2,2,2,2,2,2,2,2,2,2,2,2,
2,2,2,2,2,2,2,2,2,2,2,2,2,2,2,2,2,2,2,2,2,2,2,2,2,2,2,2,2,2,2,2,4),(0.000164533515203592,
0.15574788143604,0.300311425412708,0.569373761758525,0.79618657880448,0.922541857226,
0.988904254887107,1.0653692971268,1.25210389344582,1.42535492735896,1.50265916110143,
1.58851742855532,1.66019897681292,1.7154790824507,1.77355589777661,1.95475787098224,
2.04862650077206,2.12027287069596,2.17286295576569,2.2595637445942,2.34255832444489,
2.38071228733387,2.42149276767208,2.47124766457881,2.6150539169351,2.75087412291449,
2.80056720175112,2.84167674733784,2.98305280903366,3.07138278232828,3.10632890237946,
3.14629868941928,3.22861226113931,3.36258398098612,3.43849932049605,3.47714516706065,
3.51392785473813,3.6117878053805,3.70836592068353,3.76794458464598,3.79962609632322,
3.83743317455229,3.94227692301846,4.04709614636816,4.11179326352921,4.14572233491239,
4.18359857780085,4.2847010418534,4.38923781641045,4.45343794502814,4.48682377962691,
4.52149832706062,4.59643350613506,4.71314948116913,4.76039791117649,4.79937613171105,
4.83531193373953,4.89766444205739,5.05424405055733,5.13467567943698,5.173180257863,
5.20800344399481,5.34491460624367,5.43934749892766,5.47878821833075,5.52559040811516,
5.69013077490027,5.77544264138173,5.8379652638945,5.87889902859667,5.92624035708248,
6.04473759572682,6.09274842224217,6.14285502964907,6.19964912006544,6.36932165795769,
6.46449491795829,6.53568224943887,6.58612340023522,6.68154754770684,6.78172409066983,
6.85266260775808,7.08411900047799,7.18340018586257,7.26475716566072,7.34592524358762,
7.44742089527027,7.57757375930111,7.75796056009403,7.97929905302474,8.09228581444125,
8.61092620220196,8.74282270043409,8.99753184305009,9.23459888874445,9.36815206661486,
9.43329508924799,9.50767505195354,9.73032389966636,9.8365758432595,9.92238613205742,
9.99555986248376,10.0676642998935,10.1467995025813,10.198486501858,10.2778943711568,
10.3930873678413,10.5270230683069,10.5865851703363,10.6386106779327,10.6882622302918,
10.8052544371083,10.851675060425,10.8938848923791,10.9627076822763,11.1735165890948,
11.2332315816838,11.274511843921,11.3258318815358,11.4433870595462,11.5176797599669,
11.5528679247441,11.5915777257815,11.6720238231879,11.8279526244865,11.8919536687505,
11.9287288660531,11.9675433985747,12.014254075755,12.1301965112121,12.2053125480792,
12.2394501915855,12.273327920918,12.3405513281499,12.4550836863104,12.5460185108539,
12.5832819421439,12.6173385791642,12.6864705035049,12.8086815512044,12.8894377209578,
12.9260334996992,12.9579593879317,13.0214163878057,13.1308924188965,13.2132216960653,
13.2493968551011,13.2873945418515,13.3639203976739,13.5033029393173,13.5807831965947,
13.619109048039,13.6543434044654,13.7602592767141,13.8745338706366,13.9152694853788,
13.9596948201189,14.0508765813697,14.2367980478715,14.2906477020263,14.3309772172887,
14.3914972781408,14.5048023767773,14.56371883741,14.6153600973738,14.6966447505308,
14.818385443839,14.9499347785817,15.0060265353982,15.05981889999,15.127586751363,
15.2245099254412,15.2973100920515,15.4691547722829,15.6527398494129,15.7273552713701,
15.7908427662886,15.9217598306892,16.0990554913762,16.4443175652378,16.5617592512692,
17.0838742715074,17.1932159661468,17.3259554357176,17.6060135285824,17.7357461921405,
17.8427816548078,17.9152772018098,18.0124495522896,18.1509017133738,18.296623164564,
18.3725042626396,18.4559825970312,18.5838321615931,18.6358492486316,18.7210910207846,
18.8555132024386,18.9686220505528,19.024120219767,19.0762897095534,19.1802134193937,
19.2520770089242,19.2932612111306,19.3373941271067,19.4249263100775,19.5932635977254,
19.6592373098822,19.7004586930598,19.7463549783324,19.9232344224063,19.9501361012415,
19.9622891784342),.UNSPECIFIED.);
#30325=B_SPLINE_CURVE_WITH_KNOTS('',3,(#185481,#185482,#185483,#185484,
#185485,#185486,#185487,#185488,#185489,#185490,#185491,#185492,#185493,
#185494),.UNSPECIFIED.,.F.,.F.,(4,2,2,2,2,2,4),(2.32621539683198E-5,0.400098729001259,
0.799101480288672,1.34105949117882,1.70265074241555,1.91405386469819,2.12102518490325),
 .UNSPECIFIED.);
#30326=B_SPLINE_CURVE_WITH_KNOTS('',3,(#185496,#185497,#185498,#185499),
 .UNSPECIFIED.,.F.,.F.,(4,4),(0.,0.00660405994458262),.UNSPECIFIED.);
#30327=B_SPLINE_CURVE_WITH_KNOTS('',3,(#185500,#185501,#185502,#185503,
#185504,#185505,#185506,#185507,#185508,#185509,#185510,#185511),
 .UNSPECIFIED.,.F.,.F.,(4,2,2,2,2,4),(-18.1421165145352,-17.9925634623113,
-17.9105025327825,-17.7593505375724,-17.6048012785571,-17.4782773446469),
 .UNSPECIFIED.);
#30328=B_SPLINE_CURVE_WITH_KNOTS('',3,(#185592,#185593,#185594,#185595,
#185596,#185597,#185598,#185599,#185600,#185601,#185602,#185603,#185604,
#185605,#185606,#185607,#185608,#185609,#185610,#185611,#185612,#185613,
#185614,#185615,#185616,#185617,#185618,#185619,#185620,#185621,#185622,
#185623,#185624,#185625,#185626,#185627,#185628,#185629,#185630,#185631,
#185632,#185633,#185634,#185635,#185636,#185637,#185638,#185639,#185640,
#185641,#185642,#185643,#185644,#185645,#185646,#185647,#185648,#185649,
#185650,#185651,#185652,#185653,#185654,#185655,#185656,#185657,#185658,
#185659,#185660,#185661,#185662,#185663,#185664,#185665,#185666,#185667),
 .UNSPECIFIED.,.F.,.F.,(4,2,2,2,2,2,2,2,2,2,2,2,2,2,2,2,2,2,2,2,2,2,2,2,
2,2,2,2,2,2,2,2,2,2,2,2,2,4),(9.5121277628468E-5,0.249595276786102,0.402925412314556,
0.521282340890639,0.751084079383089,1.01658038578886,1.25339646377788,1.50485759578655,
1.610531239197,1.88100328567676,2.1163995971987,2.29305069595439,2.53046871405044,
2.69847868939906,2.96099769965047,3.18389439258267,3.71587281309874,3.92336136867365,
4.12173585205318,4.37630183981309,4.57630326379367,4.67864799639467,4.89141453502725,
5.14664142545471,5.37623130030702,5.71415099752245,5.97637698865336,6.23695400971814,
6.75820129659731,7.01668233427012,7.20065892246672,7.45676982547489,7.98061722365381,
8.24162856837933,8.36890312771966,8.8427719861429,9.08125032492622,9.32032447711697),
 .UNSPECIFIED.);
#30329=B_SPLINE_CURVE_WITH_KNOTS('',3,(#185669,#185670,#185671,#185672,
#185673,#185674,#185675,#185676,#185677,#185678,#185679,#185680,#185681,
#185682,#185683,#185684,#185685,#185686,#185687,#185688,#185689,#185690,
#185691,#185692,#185693,#185694,#185695,#185696,#185697,#185698,#185699,
#185700,#185701,#185702,#185703,#185704,#185705,#185706,#185707,#185708,
#185709,#185710,#185711,#185712,#185713,#185714,#185715,#185716,#185717,
#185718,#185719,#185720,#185721,#185722,#185723,#185724,#185725,#185726,
#185727,#185728,#185729,#185730,#185731,#185732,#185733,#185734,#185735,
#185736,#185737,#185738,#185739,#185740,#185741,#185742,#185743,#185744,
#185745,#185746,#185747,#185748,#185749,#185750,#185751,#185752,#185753,
#185754,#185755,#185756,#185757,#185758,#185759,#185760,#185761,#185762,
#185763,#185764,#185765,#185766,#185767,#185768,#185769,#185770,#185771,
#185772,#185773,#185774,#185775,#185776,#185777,#185778,#185779,#185780,
#185781,#185782,#185783,#185784,#185785,#185786,#185787,#185788,#185789,
#185790,#185791,#185792),.UNSPECIFIED.,.F.,.F.,(4,3,3,3,3,3,3,3,3,3,3,3,
3,3,3,3,3,3,3,3,3,3,3,3,3,3,3,3,3,3,3,3,3,3,3,3,3,3,3,3,3,4),(0.,0.0276914053910685,
0.0664920742418303,0.106600634168667,0.145179304224856,0.175451960403814,
0.183883838061466,0.190699425235669,0.218730858025732,0.239809569979581,
0.247513314271047,0.252696050322163,0.292154019225632,0.331863658139455,
0.371731219090931,0.387360553656524,0.427049658799308,0.467428988434914,
0.485094945150492,0.49455817189996,0.499129004833813,0.502646411513384,
0.541484936161962,0.580472912016988,0.619451931615742,0.658127145790832,
0.681122858545679,0.686905028775457,0.692898726594125,0.719841435153799,
0.734962865518979,0.742523580701569,0.746492661689958,0.74924581130424,
0.750084295884158,0.788114818739895,0.826614366988998,0.86547301495562,
0.90460707319013,0.943746161219805,0.982674727452436,1.),.UNSPECIFIED.);
#30330=B_SPLINE_CURVE_WITH_KNOTS('',3,(#185794,#185795,#185796,#185797),
 .UNSPECIFIED.,.F.,.F.,(4,4),(-0.000360640939376314,0.),.UNSPECIFIED.);
#30331=B_SPLINE_CURVE_WITH_KNOTS('',3,(#185798,#185799,#185800,#185801,
#185802,#185803,#185804,#185805,#185806,#185807,#185808,#185809,#185810,
#185811,#185812,#185813,#185814,#185815,#185816,#185817,#185818,#185819,
#185820,#185821,#185822,#185823,#185824,#185825,#185826,#185827,#185828,
#185829,#185830,#185831,#185832,#185833,#185834,#185835,#185836,#185837,
#185838,#185839,#185840,#185841,#185842,#185843,#185844,#185845,#185846,
#185847,#185848,#185849,#185850,#185851,#185852,#185853,#185854,#185855,
#185856,#185857,#185858,#185859,#185860,#185861,#185862,#185863,#185864,
#185865,#185866,#185867),.UNSPECIFIED.,.F.,.F.,(4,2,2,2,2,2,2,2,2,2,2,2,
2,2,2,2,2,2,2,2,2,2,2,2,2,2,2,2,2,2,2,2,2,2,4),(-6.70530344949381,-6.3523661180227,
-6.21616553242361,-6.05570076631061,-5.86324644351769,-5.75752630293958,
-5.57746835957856,-5.32503153778005,-5.11610470936969,-4.90230388945836,
-4.79773619952221,-4.58648071047068,-4.39330135932084,-4.2188712833661,
-4.11297408472852,-3.97677726421539,-3.84549117665225,-3.71129611429485,
-3.58847537704995,-3.462789093206,-3.26206199633315,-3.11034685614292,-2.83007851493899,
-2.35622475827822,-2.16802485780617,-1.93367740396821,-1.80677119945566,
-1.61140432188186,-1.47961053146882,-1.23439747229975,-1.04314403571828,
-0.901677225570379,-0.45467837226067,-0.229205497357456,-0.00019735943205006),
 .UNSPECIFIED.);
#30332=B_SPLINE_CURVE_WITH_KNOTS('',3,(#186009,#186010,#186011,#186012,
#186013,#186014,#186015,#186016,#186017,#186018,#186019,#186020,#186021,
#186022,#186023,#186024,#186025,#186026,#186027,#186028,#186029,#186030,
#186031,#186032,#186033,#186034,#186035,#186036,#186037,#186038,#186039,
#186040,#186041,#186042,#186043,#186044,#186045,#186046,#186047,#186048,
#186049,#186050,#186051,#186052,#186053,#186054,#186055,#186056,#186057,
#186058,#186059,#186060,#186061,#186062,#186063,#186064,#186065,#186066,
#186067,#186068,#186069,#186070,#186071,#186072,#186073,#186074,#186075,
#186076,#186077,#186078,#186079,#186080,#186081,#186082,#186083,#186084,
#186085,#186086,#186087,#186088,#186089,#186090,#186091,#186092,#186093,
#186094,#186095,#186096,#186097,#186098,#186099,#186100,#186101,#186102,
#186103,#186104,#186105,#186106,#186107,#186108,#186109,#186110,#186111,
#186112,#186113,#186114,#186115,#186116,#186117,#186118,#186119,#186120,
#186121,#186122,#186123,#186124,#186125,#186126,#186127,#186128,#186129,
#186130,#186131,#186132,#186133,#186134,#186135,#186136,#186137,#186138,
#186139,#186140,#186141,#186142,#186143,#186144,#186145,#186146,#186147,
#186148,#186149,#186150,#186151,#186152,#186153,#186154,#186155,#186156,
#186157,#186158,#186159,#186160,#186161,#186162,#186163,#186164,#186165,
#186166,#186167,#186168,#186169,#186170,#186171,#186172,#186173,#186174,
#186175,#186176,#186177,#186178,#186179,#186180,#186181,#186182,#186183,
#186184,#186185,#186186,#186187,#186188,#186189,#186190,#186191,#186192,
#186193,#186194,#186195,#186196,#186197,#186198,#186199,#186200,#186201,
#186202,#186203,#186204,#186205,#186206,#186207,#186208,#186209,#186210,
#186211,#186212,#186213,#186214,#186215,#186216,#186217,#186218,#186219,
#186220,#186221,#186222,#186223,#186224,#186225,#186226,#186227,#186228,
#186229,#186230,#186231,#186232,#186233,#186234,#186235,#186236,#186237,
#186238,#186239,#186240,#186241,#186242,#186243,#186244,#186245,#186246,
#186247,#186248,#186249,#186250,#186251,#186252,#186253,#186254,#186255,
#186256,#186257,#186258,#186259,#186260,#186261,#186262,#186263,#186264,
#186265,#186266,#186267,#186268,#186269,#186270,#186271,#186272,#186273,
#186274,#186275,#186276,#186277,#186278,#186279,#186280,#186281,#186282,
#186283,#186284,#186285,#186286,#186287,#186288,#186289,#186290,#186291,
#186292,#186293,#186294,#186295,#186296,#186297,#186298,#186299,#186300,
#186301,#186302,#186303,#186304,#186305,#186306,#186307,#186308,#186309,
#186310,#186311,#186312,#186313,#186314,#186315,#186316,#186317,#186318,
#186319,#186320,#186321,#186322,#186323,#186324,#186325,#186326,#186327,
#186328,#186329,#186330,#186331,#186332,#186333,#186334,#186335,#186336,
#186337,#186338,#186339,#186340,#186341,#186342,#186343,#186344,#186345,
#186346,#186347,#186348,#186349,#186350,#186351,#186352,#186353,#186354,
#186355,#186356,#186357,#186358,#186359,#186360,#186361,#186362,#186363,
#186364,#186365,#186366,#186367,#186368,#186369,#186370,#186371,#186372,
#186373,#186374,#186375,#186376,#186377,#186378,#186379,#186380,#186381,
#186382,#186383,#186384,#186385,#186386,#186387,#186388,#186389,#186390,
#186391,#186392,#186393,#186394,#186395,#186396,#186397,#186398,#186399,
#186400,#186401,#186402,#186403,#186404,#186405,#186406,#186407,#186408,
#186409,#186410,#186411,#186412,#186413,#186414,#186415,#186416,#186417,
#186418,#186419,#186420,#186421,#186422,#186423,#186424,#186425,#186426,
#186427,#186428),.UNSPECIFIED.,.F.,.F.,(4,2,2,2,2,2,2,2,2,2,2,2,2,2,2,2,
2,2,2,2,2,2,2,2,2,2,2,2,2,2,2,2,2,2,2,2,2,2,2,2,2,2,2,2,2,2,2,2,2,2,2,2,
2,2,2,2,2,2,2,2,2,2,2,2,2,2,2,2,2,2,2,2,2,2,2,2,2,2,2,2,2,2,2,2,2,2,2,2,
2,2,2,2,2,2,2,2,2,2,2,2,2,2,2,2,2,2,2,2,2,2,2,2,2,2,2,2,2,2,2,2,2,2,2,2,
2,2,2,2,2,2,2,2,2,2,2,2,2,2,2,2,2,2,2,2,2,2,2,2,2,2,2,2,2,2,2,2,2,2,2,2,
2,2,2,2,2,2,2,2,2,2,2,2,2,2,2,2,2,2,2,2,2,2,2,2,2,2,2,2,2,2,2,2,2,2,2,2,
2,2,2,2,2,2,2,2,2,2,2,2,2,4),(-21.8329251448155,-21.6443827645098,-21.5732407549653,
-21.4937793564471,-21.3036935948802,-21.1950255432799,-21.1302502295424,
-21.0062043365996,-20.8956464117004,-20.8495843915274,-20.7926915242238,
-20.6645775558975,-20.586408714092,-20.461637530838,-20.3595427854041,-20.1985602066991,
-20.1453544408803,-20.1043960712606,-19.9756229159482,-19.88814467434,-19.7911012649131,
-19.6507351841967,-19.5093899344014,-19.453489464351,-19.4080492880456,
-19.3489994344965,-19.2040163537948,-19.1434388099925,-19.0805936762193,
-18.979017836747,-18.8094306948228,-18.7128296685487,-18.6460413514842,
-18.4771673378652,-18.3721213587991,-18.3156755479724,-18.178125879852,
-18.0491151473622,-17.9981253909182,-17.8584086914978,-17.6688254349913,
-17.5859758529825,-17.499684076209,-17.3848610015013,-17.3166647400089,
-17.2760782035752,-17.1634007314228,-16.9970020382501,-16.8804829120801,
-16.7477798300899,-16.6501523196607,-16.5908288232001,-16.5497170959436,
-16.4140180509483,-16.3021699235238,-16.2150863070732,-16.0601667092189,
-15.9286097189282,-15.8821907279592,-15.8348094666183,-15.6531777111572,
-15.5555277630453,-15.4953667835224,-15.3410430155883,-15.2004015569117,
-15.1344094696977,-14.9371678957363,-14.8106943984559,-14.7503347499441,
-14.5949231760321,-14.4884550179283,-14.4425584435066,-14.3184945675219,
-14.1167954208962,-14.0221544659323,-13.9217386657594,-13.8199513853057,
-13.7569930854452,-13.7172190677987,-13.5899115647471,-13.4860952228305,
-13.3750486109775,-13.2342883034089,-13.1168722215261,-13.0613073120677,
-13.0168955754192,-12.9641889276144,-12.8257016274758,-12.7630104237111,
-12.6931293473043,-12.5847956599781,-12.3954142745935,-12.3361766735367,
-12.2835030511139,-12.0937418228578,-11.989663675477,-11.9333618005977,
-11.7821776465091,-11.650065948291,-11.5942783726521,-11.4372704510442,
-11.2704115699778,-11.1981389409495,-11.1116287657827,-10.9954416907346,
-10.943180460361,-10.8982455627616,-10.8381247965561,-10.7311394039421,
-10.5639880855157,-10.4583057422459,-10.3283572843291,-10.2186298399277,
-10.1786771935202,-10.1232450305456,-10.0430232151756,-9.92337233040851,
-9.82627804394939,-9.65433544558044,-9.51106261477267,-9.46485794953245,
-9.40667614441514,-9.18485385318469,-9.12078871442883,-8.96331818580267,
-8.79330185738388,-8.7314749974436,-8.60391771326453,-8.45958860209339,
-8.39713249969306,-8.32340459424354,-8.2095325045695,-8.12349454627661,
-8.06899666183474,-7.97971801445844,-7.75403315050388,-7.66186828080559,
-7.5850840797206,-7.49406962693947,-7.39953238386288,-7.35521010723848,
-7.30425096509559,-7.07833953163658,-6.96035821501014,-6.83011103593677,
-6.68586967100914,-6.64055674783179,-6.59308766991904,-6.53375843097421,
-6.35873389077308,-6.27162098010247,-6.07877227115871,-5.94418030597099,
-5.89639674667542,-5.78250149271391,-5.63100810747453,-5.57357436413799,
-5.46781284842467,-5.29426621008378,-5.22427614936901,-5.13033477719018,
-4.97823105212994,-4.87430784643472,-4.81377783645382,-4.75822182974962,
-4.6332498800261,-4.55442529116533,-4.50942665398307,-4.42683325193232,
-4.1847708687164,-4.08929937501717,-3.98367052808113,-3.8364247733426,-3.79671297631128,
-3.73331902314079,-3.62334590164148,-3.50865127727065,-3.39372167724177,
-3.22019220688821,-3.11571682197365,-3.07415734032848,-3.00045509449745,
-2.86858467446023,-2.79450504880198,-2.71346183938156,-2.61417115195599,
-2.3937657849274,-2.33641916099488,-2.2671746271922,-2.10622552046567,-2.04086190697162,
-1.97500729742979,-1.88805238173785,-1.7243916329033,-1.66967464879849,
-1.50861406559062,-1.34057573516499,-1.26894107176565,-1.16016163255503,
-1.02030806014582,-0.976593745862524,-0.915928188220698,-0.8064189356607,
-0.646691593117389,-0.542287460916897,-0.401621152798373,-0.299052515077757,
-0.258763143589947,-0.203698819625743,-0.0115231415835987),
 .UNSPECIFIED.);
#30333=B_SPLINE_CURVE_WITH_KNOTS('',3,(#186430,#186431,#186432,#186433,
#186434,#186435,#186436,#186437,#186438,#186439,#186440,#186441,#186442,
#186443,#186444,#186445,#186446,#186447,#186448,#186449,#186450,#186451,
#186452,#186453,#186454,#186455,#186456,#186457,#186458,#186459,#186460,
#186461,#186462,#186463,#186464,#186465,#186466,#186467,#186468,#186469,
#186470,#186471,#186472,#186473,#186474,#186475,#186476,#186477,#186478,
#186479,#186480,#186481,#186482,#186483,#186484,#186485,#186486,#186487,
#186488,#186489,#186490,#186491,#186492,#186493,#186494,#186495,#186496,
#186497,#186498,#186499,#186500,#186501,#186502,#186503,#186504,#186505,
#186506,#186507,#186508,#186509,#186510,#186511,#186512,#186513,#186514,
#186515,#186516,#186517,#186518,#186519,#186520,#186521,#186522,#186523,
#186524,#186525,#186526,#186527,#186528,#186529,#186530,#186531,#186532,
#186533,#186534,#186535,#186536,#186537,#186538,#186539,#186540,#186541,
#186542,#186543,#186544,#186545,#186546,#186547,#186548,#186549,#186550,
#186551,#186552,#186553,#186554,#186555,#186556,#186557,#186558,#186559,
#186560,#186561,#186562,#186563,#186564,#186565,#186566,#186567,#186568,
#186569,#186570,#186571,#186572,#186573,#186574,#186575,#186576,#186577,
#186578,#186579,#186580),.UNSPECIFIED.,.F.,.F.,(4,3,3,3,3,3,3,3,3,3,3,3,
3,3,3,3,3,3,3,3,3,3,3,3,3,3,3,3,3,3,3,3,3,3,3,3,3,3,3,3,3,3,3,3,3,3,3,3,
3,3,4),(0.,0.0392866652558998,0.0785456651531797,0.0880372583011311,0.0920278542607797,
0.0956231269293492,0.112912484515642,0.122437251525716,0.124969665134475,
0.127473761529773,0.164063235736105,0.200668571059852,0.227798128282118,
0.24236056777765,0.248093420263772,0.252685719858583,0.297930728075632,
0.343215831814716,0.365856436119722,0.383101361047376,0.417705028837983,
0.443984982286002,0.46862243864352,0.471549913649985,0.488617603051972,
0.499949749118747,0.502163791399289,0.545535599660173,0.588876763877804,
0.620040203893865,0.624334132892357,0.628034909772857,0.667089344334197,
0.677782778063702,0.685552586199097,0.690858618578248,0.716899516151074,
0.74283750634619,0.747597535630855,0.750418042766665,0.789527071692462,
0.801691374770918,0.81061815205851,0.816126459479278,0.838184284006286,
0.85757334010825,0.874944966513778,0.879852174093526,0.919450746518562,
0.959062655278241,0.993296732821997),.UNSPECIFIED.);
#30334=B_SPLINE_CURVE_WITH_KNOTS('',3,(#186581,#186582,#186583,#186584),
 .UNSPECIFIED.,.F.,.F.,(4,4),(0.,0.00140322528949482),.UNSPECIFIED.);
#30335=B_SPLINE_CURVE_WITH_KNOTS('',3,(#186616,#186617,#186618,#186619),
 .UNSPECIFIED.,.F.,.F.,(4,4),(0.,0.00269304460844964),.UNSPECIFIED.);
#30336=B_SPLINE_CURVE_WITH_KNOTS('',3,(#186620,#186621,#186622,#186623,
#186624,#186625,#186626,#186627,#186628,#186629,#186630,#186631,#186632,
#186633),.UNSPECIFIED.,.F.,.F.,(4,2,2,2,2,2,4),(0.000161979881089482,0.400873717312025,
0.801763578870112,1.29477100198553,1.7630975899284,2.11375019375441,2.46863362347642),
 .UNSPECIFIED.);
#30337=B_SPLINE_CURVE_WITH_KNOTS('',3,(#186981,#186982,#186983,#186984,
#186985,#186986),.UNSPECIFIED.,.F.,.F.,(4,2,4),(-0.194208713167773,-0.0971361853452758,
-3.86117433745282E-5),.UNSPECIFIED.);
#30338=B_SPLINE_CURVE_WITH_KNOTS('',3,(#187064,#187065,#187066,#187067,
#187068,#187069),.UNSPECIFIED.,.F.,.F.,(4,2,4),(-0.194199485947135,-0.0971172181367527,
-0.00177501603400677),.UNSPECIFIED.);
#30339=B_SPLINE_CURVE_WITH_KNOTS('',3,(#187070,#187071,#187072,#187073),
 .UNSPECIFIED.,.F.,.F.,(4,4),(-0.00170970345529554,0.),.UNSPECIFIED.);
#31407=CIRCLE('',#80983,13.9);
#31408=CIRCLE('',#80985,13.9);
#31409=CIRCLE('',#80988,13.9);
#31410=CIRCLE('',#80990,11.58843628952);
#31411=CIRCLE('',#80991,11.69981713671);
#31412=CIRCLE('',#80992,11.58843628952);
#31413=CIRCLE('',#80994,0.7);
#31414=CIRCLE('',#80995,11.40026076189);
#31415=CIRCLE('',#80997,1.3);
#31416=CIRCLE('',#80998,11.05);
#31417=CIRCLE('',#81002,11.05);
#31418=CIRCLE('',#81003,11.05);
#31419=CIRCLE('',#81004,11.05);
#31420=CIRCLE('',#81005,11.05);
#31421=CIRCLE('',#81006,11.05);
#31422=CIRCLE('',#81007,11.05);
#31423=CIRCLE('',#81008,11.05);
#31424=CIRCLE('',#81009,11.05);
#31425=CIRCLE('',#81010,11.05);
#31426=CIRCLE('',#81011,11.05);
#31427=CIRCLE('',#81012,11.05);
#31428=CIRCLE('',#81016,11.35);
#31429=CIRCLE('',#81017,11.35);
#31430=CIRCLE('',#81018,11.35);
#31431=CIRCLE('',#81019,11.35);
#31432=CIRCLE('',#81020,11.35);
#31433=CIRCLE('',#81021,11.35);
#31434=CIRCLE('',#81022,11.35);
#31435=CIRCLE('',#81023,11.35);
#31436=CIRCLE('',#81024,11.35);
#31437=CIRCLE('',#81025,11.35);
#31438=CIRCLE('',#81026,11.35);
#31439=CIRCLE('',#81027,11.35);
#31440=CIRCLE('',#81029,10.84999988564);
#31441=CIRCLE('',#81030,0.5);
#31442=CIRCLE('',#81032,9.84999999999999);
#31443=CIRCLE('',#81033,9.84999999999999);
#31444=CIRCLE('',#81035,10.15);
#31445=CIRCLE('',#81036,10.15);
#31446=CIRCLE('',#81038,1.);
#31447=CIRCLE('',#81039,11.6194313553);
#31448=CIRCLE('',#81041,1.);
#31449=CIRCLE('',#81042,11.88825353763);
#31450=CIRCLE('',#81043,11.88825353763);
#31451=CIRCLE('',#81045,12.);
#31452=CIRCLE('',#81047,12.25);
#31453=CIRCLE('',#81048,12.25);
#31454=CIRCLE('',#81050,12.75);
#31455=CIRCLE('',#81051,12.75);
#31456=CIRCLE('',#81053,13.1);
#31457=CIRCLE('',#81054,13.1);
#31458=CIRCLE('',#81056,13.7);
#31459=CIRCLE('',#81057,13.7);
#31460=CIRCLE('',#81058,13.7);
#31461=CIRCLE('',#81059,13.7);
#31462=CIRCLE('',#81060,13.7);
#31463=CIRCLE('',#81061,13.7);
#31464=CIRCLE('',#81063,13.4);
#31465=CIRCLE('',#81065,12.75);
#31466=CIRCLE('',#81066,12.75);
#31467=CIRCLE('',#81069,13.2);
#31468=CIRCLE('',#81071,13.2);
#31469=CIRCLE('',#81077,13.9);
#31470=CIRCLE('',#81083,13.07481294348);
#31471=CIRCLE('',#81085,15.44456161589);
#31472=CIRCLE('',#81086,15.74486371827);
#31473=CIRCLE('',#81088,13.39778838118);
#31474=CIRCLE('',#81089,13.04356099794);
#31475=CIRCLE('',#81091,15.75914761359);
#31476=CIRCLE('',#81092,15.45912298634);
#31477=CIRCLE('',#81094,8.729046339664);
#31478=CIRCLE('',#81096,13.07481294348);
#31479=CIRCLE('',#81098,15.36666793768);
#31480=CIRCLE('',#81099,15.66846302312);
#31481=CIRCLE('',#81101,13.39778838118);
#31482=CIRCLE('',#81102,13.04356099794);
#31483=CIRCLE('',#81104,15.71466619139);
#31484=CIRCLE('',#81105,15.41377577062);
#31485=CIRCLE('',#81107,8.729046339664);
#31486=CIRCLE('',#81109,13.04356099794);
#31487=CIRCLE('',#81110,13.39778838118);
#31488=CIRCLE('',#81112,15.52741876511);
#31489=CIRCLE('',#81114,13.07481294348);
#31490=CIRCLE('',#81116,15.3030873848);
#31491=CIRCLE('',#81117,15.60611205608);
#31492=CIRCLE('',#81119,8.72904633966399);
#31493=CIRCLE('',#81121,15.45912298634);
#31494=CIRCLE('',#81122,15.75914761359);
#31495=CIRCLE('',#81124,13.62844391363);
#31496=CIRCLE('',#81125,13.96784641621);
#31497=CIRCLE('',#81127,15.44456161589);
#31498=CIRCLE('',#81128,15.74486371827);
#31499=CIRCLE('',#81130,13.34857608537);
#31500=CIRCLE('',#81131,13.69491633808);
#31501=CIRCLE('',#81133,15.41377577062);
#31502=CIRCLE('',#81134,15.71466619139);
#31503=CIRCLE('',#81136,13.62844391363);
#31504=CIRCLE('',#81137,13.96784641621);
#31505=CIRCLE('',#81139,15.36666793768);
#31506=CIRCLE('',#81140,15.66846302312);
#31507=CIRCLE('',#81142,13.34857608537);
#31508=CIRCLE('',#81143,13.69491633808);
#31509=CIRCLE('',#81145,15.3030873848);
#31510=CIRCLE('',#81146,15.60611205608);
#31511=CIRCLE('',#81148,13.62844391363);
#31512=CIRCLE('',#81149,13.96784641621);
#31513=CIRCLE('',#81151,15.22282771061);
#31514=CIRCLE('',#81152,15.52741876511);
#31515=CIRCLE('',#81154,13.34857608537);
#31516=CIRCLE('',#81155,13.69491633808);
#31517=CIRCLE('',#81157,13.62844391363);
#31518=CIRCLE('',#81158,13.96784641621);
#31519=CIRCLE('',#81160,15.01114530963);
#31520=CIRCLE('',#81161,15.31994561044);
#31521=CIRCLE('',#81163,13.34857608537);
#31522=CIRCLE('',#81164,13.69491633808);
#31523=CIRCLE('',#81166,15.12562340887);
#31524=CIRCLE('',#81167,15.4321331483);
#31525=CIRCLE('',#81169,13.69491633808);
#31526=CIRCLE('',#81171,14.72869592011);
#31527=CIRCLE('',#81172,15.0432953008);
#31528=CIRCLE('',#81174,13.96784641621);
#31529=CIRCLE('',#81175,13.62844391363);
#31530=CIRCLE('',#81177,15.19048167462);
#31531=CIRCLE('',#81178,14.87899470754);
#31532=CIRCLE('',#81180,8.729046339664);
#31533=CIRCLE('',#81182,13.1066579839);
#31534=CIRCLE('',#81183,13.45922484792);
#31535=CIRCLE('',#81185,15.28837739941);
#31536=CIRCLE('',#81186,15.59168796208);
#31537=CIRCLE('',#81188,13.14156510873);
#31538=CIRCLE('',#81190,15.20475200412);
#31539=CIRCLE('',#81191,15.50969804693);
#31540=CIRCLE('',#81193,8.729046339664);
#31541=CIRCLE('',#81195,13.1066579839);
#31542=CIRCLE('',#81196,13.45922484792);
#31543=CIRCLE('',#81198,15.40566400734);
#31544=CIRCLE('',#81199,15.70670982437);
#31545=CIRCLE('',#81201,13.14156510873);
#31546=CIRCLE('',#81203,15.35527542921);
#31547=CIRCLE('',#81204,15.65729010739);
#31548=CIRCLE('',#81206,8.729046339664);
#31549=CIRCLE('',#81208,13.1066579839);
#31550=CIRCLE('',#81209,13.45922484792);
#31551=CIRCLE('',#81211,15.45750573369);
#31552=CIRCLE('',#81212,15.75756115352);
#31553=CIRCLE('',#81214,12.78023800666);
#31554=CIRCLE('',#81215,13.14156510873);
#31555=CIRCLE('',#81217,15.43970477396);
#31556=CIRCLE('',#81218,15.7400995393);
#31557=CIRCLE('',#81220,8.729046339664);
#31558=CIRCLE('',#81222,13.1066579839);
#31559=CIRCLE('',#81223,13.45922484792);
#31560=CIRCLE('',#81225,15.44456161589);
#31561=CIRCLE('',#81226,15.74486371827);
#31562=CIRCLE('',#81228,12.78023800666);
#31563=CIRCLE('',#81229,13.14156510873);
#31564=CIRCLE('',#81231,15.45912298634);
#31565=CIRCLE('',#81232,15.75914761359);
#31566=CIRCLE('',#81234,13.1066579839);
#31567=CIRCLE('',#81235,13.45922484792);
#31568=CIRCLE('',#81237,15.36666793768);
#31569=CIRCLE('',#81238,15.66846302312);
#31570=CIRCLE('',#81240,13.14156510873);
#31571=CIRCLE('',#81242,15.41377577062);
#31572=CIRCLE('',#81243,15.71466619139);
#31573=CIRCLE('',#81245,8.72904633966401);
#31574=CIRCLE('',#81247,13.1066579839);
#31575=CIRCLE('',#81248,13.45922484792);
#31576=CIRCLE('',#81250,15.22282771061);
#31577=CIRCLE('',#81251,15.52741876511);
#31578=CIRCLE('',#81253,13.14156510873);
#31579=CIRCLE('',#81255,15.3030873848);
#31580=CIRCLE('',#81256,15.60611205608);
#31581=CIRCLE('',#81258,8.729046339664);
#31582=CIRCLE('',#81260,13.1066579839);
#31583=CIRCLE('',#81261,13.45922484792);
#31584=CIRCLE('',#81263,15.3030873848);
#31585=CIRCLE('',#81264,15.60611205608);
#31586=CIRCLE('',#81266,13.14156510873);
#31587=CIRCLE('',#81268,15.22282771061);
#31588=CIRCLE('',#81269,15.52741876511);
#31589=CIRCLE('',#81271,8.729046339664);
#31590=CIRCLE('',#81273,13.1066579839);
#31591=CIRCLE('',#81274,13.45922484792);
#31592=CIRCLE('',#81276,15.41377577062);
#31593=CIRCLE('',#81277,15.71466619139);
#31594=CIRCLE('',#81279,13.14156510873);
#31595=CIRCLE('',#81281,15.36666793768);
#31596=CIRCLE('',#81282,15.66846302312);
#31597=CIRCLE('',#81284,8.729046339664);
#31598=CIRCLE('',#81286,15.45912298634);
#31599=CIRCLE('',#81287,15.75914761359);
#31600=CIRCLE('',#81289,12.78023800666);
#31601=CIRCLE('',#81290,13.14156510873);
#31602=CIRCLE('',#81292,15.44456161589);
#31603=CIRCLE('',#81293,15.74486371827);
#31604=CIRCLE('',#81295,13.1066579839);
#31605=CIRCLE('',#81296,13.45922484792);
#31606=CIRCLE('',#81298,15.45912298634);
#31607=CIRCLE('',#81299,15.75914761359);
#31608=CIRCLE('',#81301,14.1185864557);
#31609=CIRCLE('',#81302,14.4464782389);
#31610=CIRCLE('',#81304,15.44456161589);
#31611=CIRCLE('',#81305,15.74486371827);
#31612=CIRCLE('',#81307,13.88468521454);
#31613=CIRCLE('',#81308,14.21797220095);
#31614=CIRCLE('',#81310,15.41377577062);
#31615=CIRCLE('',#81311,15.71466619139);
#31616=CIRCLE('',#81313,14.1185864557);
#31617=CIRCLE('',#81314,14.4464782389);
#31618=CIRCLE('',#81316,15.36666793768);
#31619=CIRCLE('',#81317,15.66846302312);
#31620=CIRCLE('',#81319,13.88468521454);
#31621=CIRCLE('',#81320,14.21797220095);
#31622=CIRCLE('',#81322,15.3030873848);
#31623=CIRCLE('',#81323,15.60611205608);
#31624=CIRCLE('',#81325,14.1185864557);
#31625=CIRCLE('',#81326,14.4464782389);
#31626=CIRCLE('',#81328,15.22282771061);
#31627=CIRCLE('',#81329,15.52741876511);
#31628=CIRCLE('',#81331,13.88468521454);
#31629=CIRCLE('',#81332,14.21797220095);
#31630=CIRCLE('',#81334,15.12562340887);
#31631=CIRCLE('',#81335,15.4321331483);
#31632=CIRCLE('',#81337,14.1185864557);
#31633=CIRCLE('',#81338,14.4464782389);
#31634=CIRCLE('',#81340,15.01114530963);
#31635=CIRCLE('',#81341,15.31994561044);
#31636=CIRCLE('',#81343,13.88468521454);
#31637=CIRCLE('',#81344,14.21797220095);
#31638=CIRCLE('',#81346,14.87899470754);
#31639=CIRCLE('',#81347,15.19048167462);
#31640=CIRCLE('',#81349,14.1185864557);
#31641=CIRCLE('',#81350,14.4464782389);
#31642=CIRCLE('',#81352,14.72869592011);
#31643=CIRCLE('',#81353,15.0432953008);
#31644=CIRCLE('',#81355,13.88468521454);
#31645=CIRCLE('',#81356,14.21797220095);
#31646=CIRCLE('',#81358,14.87786051511);
#31647=CIRCLE('',#81359,14.55968693025);
#31648=CIRCLE('',#81361,14.4464782389);
#31649=CIRCLE('',#81362,14.1185864557);
#31650=CIRCLE('',#81364,14.37130764777);
#31651=CIRCLE('',#81365,14.69356095393);
#31652=CIRCLE('',#81367,14.21797220095);
#31653=CIRCLE('',#81368,13.88468521454);
#31654=CIRCLE('',#81370,8.72904633966401);
#31655=CIRCLE('',#81372,13.68153805341);
#31656=CIRCLE('',#81373,14.01965525635);
#31657=CIRCLE('',#81375,14.8504034796);
#31658=CIRCLE('',#81376,15.16247781555);
#31659=CIRCLE('',#81378,13.75139023906);
#31660=CIRCLE('',#81380,14.6964105654);
#31661=CIRCLE('',#81381,15.01168656437);
#31662=CIRCLE('',#81383,8.729046339664);
#31663=CIRCLE('',#81385,13.68153805341);
#31664=CIRCLE('',#81386,14.01965525635);
#31665=CIRCLE('',#81388,15.10412140798);
#31666=CIRCLE('',#81389,15.41105880551);
#31667=CIRCLE('',#81391,13.40650899776);
#31668=CIRCLE('',#81392,13.75139023906);
#31669=CIRCLE('',#81394,14.98614304973);
#31670=CIRCLE('',#81395,15.29544813031);
#31671=CIRCLE('',#81397,13.68153805341);
#31672=CIRCLE('',#81398,14.01965525635);
#31673=CIRCLE('',#81400,15.28837739941);
#31674=CIRCLE('',#81401,15.59168796208);
#31675=CIRCLE('',#81403,13.40650899776);
#31676=CIRCLE('',#81404,13.75139023906);
#31677=CIRCLE('',#81406,15.20475200412);
#31678=CIRCLE('',#81407,15.50969804693);
#31679=CIRCLE('',#81409,13.68153805341);
#31680=CIRCLE('',#81410,14.01965525635);
#31681=CIRCLE('',#81412,15.40566400734);
#31682=CIRCLE('',#81413,15.70670982437);
#31683=CIRCLE('',#81415,13.40650899776);
#31684=CIRCLE('',#81416,13.75139023906);
#31685=CIRCLE('',#81418,15.35527542921);
#31686=CIRCLE('',#81419,15.65729010739);
#31687=CIRCLE('',#81421,13.68153805341);
#31688=CIRCLE('',#81422,14.01965525635);
#31689=CIRCLE('',#81424,15.45750573369);
#31690=CIRCLE('',#81425,15.75756115352);
#31691=CIRCLE('',#81427,13.40650899776);
#31692=CIRCLE('',#81428,13.75139023906);
#31693=CIRCLE('',#81430,15.43970477396);
#31694=CIRCLE('',#81431,15.7400995393);
#31695=CIRCLE('',#81433,13.68153805341);
#31696=CIRCLE('',#81434,14.01965525635);
#31697=CIRCLE('',#81436,15.44456161589);
#31698=CIRCLE('',#81437,15.74486371827);
#31699=CIRCLE('',#81439,13.40650899776);
#31700=CIRCLE('',#81440,13.75139023906);
#31701=CIRCLE('',#81442,15.45912298634);
#31702=CIRCLE('',#81443,15.75914761359);
#31703=CIRCLE('',#81445,13.68153805341);
#31704=CIRCLE('',#81446,14.01965525635);
#31705=CIRCLE('',#81448,15.36666793768);
#31706=CIRCLE('',#81449,15.66846302312);
#31707=CIRCLE('',#81451,13.40650899776);
#31708=CIRCLE('',#81452,13.75139023906);
#31709=CIRCLE('',#81454,15.41377577062);
#31710=CIRCLE('',#81455,15.71466619139);
#31711=CIRCLE('',#81457,13.68153805341);
#31712=CIRCLE('',#81458,14.01965525635);
#31713=CIRCLE('',#81460,15.22282771061);
#31714=CIRCLE('',#81461,15.52741876511);
#31715=CIRCLE('',#81463,13.40650899776);
#31716=CIRCLE('',#81464,13.75139023906);
#31717=CIRCLE('',#81466,15.3030873848);
#31718=CIRCLE('',#81467,15.60611205608);
#31719=CIRCLE('',#81469,13.68153805341);
#31720=CIRCLE('',#81470,14.01965525635);
#31721=CIRCLE('',#81472,15.01114530963);
#31722=CIRCLE('',#81473,15.31994561044);
#31723=CIRCLE('',#81475,13.40650899776);
#31724=CIRCLE('',#81476,13.75139023906);
#31725=CIRCLE('',#81478,15.12562340887);
#31726=CIRCLE('',#81479,15.4321331483);
#31727=CIRCLE('',#81481,13.68153805341);
#31728=CIRCLE('',#81482,14.01965525635);
#31729=CIRCLE('',#81484,14.72869592011);
#31730=CIRCLE('',#81485,15.0432953008);
#31731=CIRCLE('',#81487,13.75139023906);
#31732=CIRCLE('',#81489,14.87899470754);
#31733=CIRCLE('',#81490,15.19048167462);
#31734=CIRCLE('',#81492,8.729046339664);
#31735=CIRCLE('',#81494,13.68153805341);
#31736=CIRCLE('',#81495,14.01965525635);
#31737=CIRCLE('',#81497,14.87899470754);
#31738=CIRCLE('',#81498,15.19048167462);
#31739=CIRCLE('',#81500,13.75139023906);
#31740=CIRCLE('',#81502,14.72869592011);
#31741=CIRCLE('',#81503,15.0432953008);
#31742=CIRCLE('',#81505,8.72904633966401);
#31743=CIRCLE('',#81507,15.12562340887);
#31744=CIRCLE('',#81508,15.4321331483);
#31745=CIRCLE('',#81510,13.40650899776);
#31746=CIRCLE('',#81511,13.75139023906);
#31747=CIRCLE('',#81513,15.01114530963);
#31748=CIRCLE('',#81514,15.31994561044);
#31749=CIRCLE('',#81516,13.68153805341);
#31750=CIRCLE('',#81517,14.01965525635);
#31751=CIRCLE('',#81519,15.3030873848);
#31752=CIRCLE('',#81520,15.60611205608);
#31753=CIRCLE('',#81522,13.40650899776);
#31754=CIRCLE('',#81523,13.75139023906);
#31755=CIRCLE('',#81525,15.22282771061);
#31756=CIRCLE('',#81526,15.52741876511);
#31757=CIRCLE('',#81528,13.68153805341);
#31758=CIRCLE('',#81529,14.01965525635);
#31759=CIRCLE('',#81531,15.41377577062);
#31760=CIRCLE('',#81532,15.71466619139);
#31761=CIRCLE('',#81534,13.40650899776);
#31762=CIRCLE('',#81535,13.75139023906);
#31763=CIRCLE('',#81537,15.36666793768);
#31764=CIRCLE('',#81538,15.66846302312);
#31765=CIRCLE('',#81540,13.68153805341);
#31766=CIRCLE('',#81541,14.01965525635);
#31767=CIRCLE('',#81543,15.45912298634);
#31768=CIRCLE('',#81544,15.75914761359);
#31769=CIRCLE('',#81546,13.40650899776);
#31770=CIRCLE('',#81547,13.75139023906);
#31771=CIRCLE('',#81549,15.44456161589);
#31772=CIRCLE('',#81550,15.74486371827);
#31773=CIRCLE('',#81552,13.68153805341);
#31774=CIRCLE('',#81553,14.01965525635);
#31775=CIRCLE('',#81555,15.45912298634);
#31776=CIRCLE('',#81556,15.75914761359);
#31777=CIRCLE('',#81558,14.52358370055);
#31778=CIRCLE('',#81559,14.84253123652);
#31779=CIRCLE('',#81561,15.44456161589);
#31780=CIRCLE('',#81562,15.74486371827);
#31781=CIRCLE('',#81564,14.33124152008);
#31782=CIRCLE('',#81565,14.65437591667);
#31783=CIRCLE('',#81567,15.41377577062);
#31784=CIRCLE('',#81568,15.71466619139);
#31785=CIRCLE('',#81570,14.52358370055);
#31786=CIRCLE('',#81571,14.84253123652);
#31787=CIRCLE('',#81573,15.36666793768);
#31788=CIRCLE('',#81574,15.66846302312);
#31789=CIRCLE('',#81576,14.33124152008);
#31790=CIRCLE('',#81577,14.65437591667);
#31791=CIRCLE('',#81579,15.3030873848);
#31792=CIRCLE('',#81580,15.60611205608);
#31793=CIRCLE('',#81582,14.52358370055);
#31794=CIRCLE('',#81583,14.84253123652);
#31795=CIRCLE('',#81585,15.22282771061);
#31796=CIRCLE('',#81586,15.52741876511);
#31797=CIRCLE('',#81588,14.33124152008);
#31798=CIRCLE('',#81589,14.65437591667);
#31799=CIRCLE('',#81591,15.12562340887);
#31800=CIRCLE('',#81592,15.4321331483);
#31801=CIRCLE('',#81594,14.52358370055);
#31802=CIRCLE('',#81595,14.84253123652);
#31803=CIRCLE('',#81597,15.01114530963);
#31804=CIRCLE('',#81598,15.31994561044);
#31805=CIRCLE('',#81600,14.33124152008);
#31806=CIRCLE('',#81601,14.65437591667);
#31807=CIRCLE('',#81603,14.87899470754);
#31808=CIRCLE('',#81604,15.19048167462);
#31809=CIRCLE('',#81606,14.52358370055);
#31810=CIRCLE('',#81607,14.84253123652);
#31811=CIRCLE('',#81609,14.72869592011);
#31812=CIRCLE('',#81610,15.0432953008);
#31813=CIRCLE('',#81612,14.33124152008);
#31814=CIRCLE('',#81613,14.65437591667);
#31815=CIRCLE('',#81615,14.55968693025);
#31816=CIRCLE('',#81616,14.87786051511);
#31817=CIRCLE('',#81618,14.52358370055);
#31818=CIRCLE('',#81619,14.84253123652);
#31819=CIRCLE('',#81621,14.37130764777);
#31820=CIRCLE('',#81622,14.69356095393);
#31821=CIRCLE('',#81624,14.33124152008);
#31822=CIRCLE('',#81625,14.65437591667);
#31823=CIRCLE('',#81627,8.729046339664);
#31824=CIRCLE('',#81629,14.16278516066);
#31825=CIRCLE('',#81630,14.48967679098);
#31826=CIRCLE('',#81632,14.52358370055);
#31827=CIRCLE('',#81633,14.84253123652);
#31828=CIRCLE('',#81635,13.93321511737);
#31829=CIRCLE('',#81636,14.26536832707);
#31830=CIRCLE('',#81638,14.33124152008);
#31831=CIRCLE('',#81639,14.65437591667);
#31832=CIRCLE('',#81641,14.16278516066);
#31833=CIRCLE('',#81642,14.48967679098);
#31834=CIRCLE('',#81644,14.8504034796);
#31835=CIRCLE('',#81645,15.16247781555);
#31836=CIRCLE('',#81647,13.93321511737);
#31837=CIRCLE('',#81648,14.26536832707);
#31838=CIRCLE('',#81650,14.6964105654);
#31839=CIRCLE('',#81651,15.01168656437);
#31840=CIRCLE('',#81653,14.16278516066);
#31841=CIRCLE('',#81654,14.48967679098);
#31842=CIRCLE('',#81656,15.10412140798);
#31843=CIRCLE('',#81657,15.41105880551);
#31844=CIRCLE('',#81659,13.93321511737);
#31845=CIRCLE('',#81660,14.26536832707);
#31846=CIRCLE('',#81662,14.98614304973);
#31847=CIRCLE('',#81663,15.29544813031);
#31848=CIRCLE('',#81665,14.16278516066);
#31849=CIRCLE('',#81666,14.48967679098);
#31850=CIRCLE('',#81668,15.28837739941);
#31851=CIRCLE('',#81669,15.59168796208);
#31852=CIRCLE('',#81671,13.93321511737);
#31853=CIRCLE('',#81672,14.26536832707);
#31854=CIRCLE('',#81674,15.20475200412);
#31855=CIRCLE('',#81675,15.50969804693);
#31856=CIRCLE('',#81677,14.16278516066);
#31857=CIRCLE('',#81678,14.48967679098);
#31858=CIRCLE('',#81680,15.40566400734);
#31859=CIRCLE('',#81681,15.70670982437);
#31860=CIRCLE('',#81683,13.93321511737);
#31861=CIRCLE('',#81684,14.26536832707);
#31862=CIRCLE('',#81686,15.35527542921);
#31863=CIRCLE('',#81687,15.65729010739);
#31864=CIRCLE('',#81689,14.16278516066);
#31865=CIRCLE('',#81690,14.48967679098);
#31866=CIRCLE('',#81692,15.45750573369);
#31867=CIRCLE('',#81693,15.75756115352);
#31868=CIRCLE('',#81695,13.93321511737);
#31869=CIRCLE('',#81696,14.26536832707);
#31870=CIRCLE('',#81698,15.43970477396);
#31871=CIRCLE('',#81699,15.7400995393);
#31872=CIRCLE('',#81701,14.16278516066);
#31873=CIRCLE('',#81702,14.48967679098);
#31874=CIRCLE('',#81704,15.44456161589);
#31875=CIRCLE('',#81705,15.74486371827);
#31876=CIRCLE('',#81707,13.93321511737);
#31877=CIRCLE('',#81708,14.26536832707);
#31878=CIRCLE('',#81710,15.45912298634);
#31879=CIRCLE('',#81711,15.75914761359);
#31880=CIRCLE('',#81713,14.16278516066);
#31881=CIRCLE('',#81714,14.48967679098);
#31882=CIRCLE('',#81716,15.36666793768);
#31883=CIRCLE('',#81717,15.66846302312);
#31884=CIRCLE('',#81719,13.93321511737);
#31885=CIRCLE('',#81720,14.26536832707);
#31886=CIRCLE('',#81722,15.41377577062);
#31887=CIRCLE('',#81723,15.71466619139);
#31888=CIRCLE('',#81725,14.16278516066);
#31889=CIRCLE('',#81726,14.48967679098);
#31890=CIRCLE('',#81728,15.22282771061);
#31891=CIRCLE('',#81729,15.52741876511);
#31892=CIRCLE('',#81731,13.93321511737);
#31893=CIRCLE('',#81732,14.26536832707);
#31894=CIRCLE('',#81734,15.3030873848);
#31895=CIRCLE('',#81735,15.60611205608);
#31896=CIRCLE('',#81737,14.16278516066);
#31897=CIRCLE('',#81738,14.48967679098);
#31898=CIRCLE('',#81740,15.01114530963);
#31899=CIRCLE('',#81741,15.31994561044);
#31900=CIRCLE('',#81743,13.93321511737);
#31901=CIRCLE('',#81744,14.26536832707);
#31902=CIRCLE('',#81746,15.12562340887);
#31903=CIRCLE('',#81747,15.4321331483);
#31904=CIRCLE('',#81749,14.16278516066);
#31905=CIRCLE('',#81750,14.48967679098);
#31906=CIRCLE('',#81752,14.72869592011);
#31907=CIRCLE('',#81753,15.0432953008);
#31908=CIRCLE('',#81755,13.93321511737);
#31909=CIRCLE('',#81756,14.26536832707);
#31910=CIRCLE('',#81758,14.87899470754);
#31911=CIRCLE('',#81759,15.19048167462);
#31912=CIRCLE('',#81761,14.55968693025);
#31913=CIRCLE('',#81762,14.87786051511);
#31914=CIRCLE('',#81764,14.16278516066);
#31915=CIRCLE('',#81765,14.48967679098);
#31916=CIRCLE('',#81767,14.37130764777);
#31917=CIRCLE('',#81768,14.69356095393);
#31918=CIRCLE('',#81770,13.93321511737);
#31919=CIRCLE('',#81771,14.26536832707);
#31920=CIRCLE('',#81773,8.72904633966401);
#31921=CIRCLE('',#81775,14.16278516066);
#31922=CIRCLE('',#81776,14.48967679098);
#31923=CIRCLE('',#81778,14.55968693025);
#31924=CIRCLE('',#81779,14.87786051511);
#31925=CIRCLE('',#81781,13.93321511737);
#31926=CIRCLE('',#81782,14.26536832707);
#31927=CIRCLE('',#81784,14.37130764777);
#31928=CIRCLE('',#81785,14.69356095393);
#31929=CIRCLE('',#81787,8.72904633966401);
#31930=CIRCLE('',#81789,14.87899470754);
#31931=CIRCLE('',#81790,15.19048167462);
#31932=CIRCLE('',#81792,13.93321511737);
#31933=CIRCLE('',#81793,14.26536832707);
#31934=CIRCLE('',#81795,14.72869592011);
#31935=CIRCLE('',#81796,15.0432953008);
#31936=CIRCLE('',#81798,14.16278516066);
#31937=CIRCLE('',#81799,14.48967679098);
#31938=CIRCLE('',#81801,15.12562340887);
#31939=CIRCLE('',#81802,15.4321331483);
#31940=CIRCLE('',#81804,13.93321511737);
#31941=CIRCLE('',#81805,14.26536832707);
#31942=CIRCLE('',#81807,15.01114530963);
#31943=CIRCLE('',#81808,15.31994561044);
#31944=CIRCLE('',#81810,14.16278516066);
#31945=CIRCLE('',#81811,14.48967679098);
#31946=CIRCLE('',#81813,15.3030873848);
#31947=CIRCLE('',#81814,15.60611205608);
#31948=CIRCLE('',#81816,13.93321511737);
#31949=CIRCLE('',#81817,14.26536832707);
#31950=CIRCLE('',#81819,15.22282771061);
#31951=CIRCLE('',#81820,15.52741876511);
#31952=CIRCLE('',#81822,14.16278516066);
#31953=CIRCLE('',#81823,14.48967679098);
#31954=CIRCLE('',#81825,15.41377577062);
#31955=CIRCLE('',#81826,15.71466619139);
#31956=CIRCLE('',#81828,13.93321511737);
#31957=CIRCLE('',#81829,14.26536832707);
#31958=CIRCLE('',#81831,15.36666793768);
#31959=CIRCLE('',#81832,15.66846302312);
#31960=CIRCLE('',#81834,14.16278516066);
#31961=CIRCLE('',#81835,14.48967679098);
#31962=CIRCLE('',#81837,15.45912298634);
#31963=CIRCLE('',#81838,15.75914761359);
#31964=CIRCLE('',#81840,13.93321511737);
#31965=CIRCLE('',#81841,14.26536832707);
#31966=CIRCLE('',#81843,15.44456161589);
#31967=CIRCLE('',#81844,15.74486371827);
#31968=CIRCLE('',#81846,14.16278516066);
#31969=CIRCLE('',#81847,14.48967679098);
#31970=CIRCLE('',#81849,15.45912298634);
#31971=CIRCLE('',#81850,15.75914761359);
#31972=CIRCLE('',#81852,14.8504034796);
#31973=CIRCLE('',#81853,15.16247781555);
#31974=CIRCLE('',#81855,15.44456161589);
#31975=CIRCLE('',#81856,15.74486371827);
#31976=CIRCLE('',#81858,14.6964105654);
#31977=CIRCLE('',#81859,15.01168656437);
#31978=CIRCLE('',#81861,15.41377577062);
#31979=CIRCLE('',#81862,15.71466619139);
#31980=CIRCLE('',#81864,14.8504034796);
#31981=CIRCLE('',#81865,15.16247781555);
#31982=CIRCLE('',#81867,15.36666793768);
#31983=CIRCLE('',#81868,15.66846302312);
#31984=CIRCLE('',#81870,14.6964105654);
#31985=CIRCLE('',#81871,15.01168656437);
#31986=CIRCLE('',#81873,15.3030873848);
#31987=CIRCLE('',#81874,15.60611205608);
#31988=CIRCLE('',#81876,14.8504034796);
#31989=CIRCLE('',#81877,15.16247781555);
#31990=CIRCLE('',#81879,15.22282771061);
#31991=CIRCLE('',#81880,15.52741876511);
#31992=CIRCLE('',#81882,14.6964105654);
#31993=CIRCLE('',#81883,15.01168656437);
#31994=CIRCLE('',#81885,15.12562340887);
#31995=CIRCLE('',#81886,15.4321331483);
#31996=CIRCLE('',#81888,14.8504034796);
#31997=CIRCLE('',#81889,15.16247781555);
#31998=CIRCLE('',#81891,15.01114530963);
#31999=CIRCLE('',#81892,15.31994561044);
#32000=CIRCLE('',#81894,14.6964105654);
#32001=CIRCLE('',#81895,15.01168656437);
#32002=CIRCLE('',#81897,14.87899470754);
#32003=CIRCLE('',#81898,15.19048167462);
#32004=CIRCLE('',#81900,14.8504034796);
#32005=CIRCLE('',#81901,15.16247781555);
#32006=CIRCLE('',#81903,14.72869592011);
#32007=CIRCLE('',#81904,15.0432953008);
#32008=CIRCLE('',#81906,14.6964105654);
#32009=CIRCLE('',#81907,15.01168656437);
#32010=CIRCLE('',#81909,14.55968693025);
#32011=CIRCLE('',#81910,14.87786051511);
#32012=CIRCLE('',#81912,14.8504034796);
#32013=CIRCLE('',#81913,15.16247781555);
#32014=CIRCLE('',#81915,14.37130764777);
#32015=CIRCLE('',#81916,14.69356095393);
#32016=CIRCLE('',#81918,14.6964105654);
#32017=CIRCLE('',#81919,15.01168656437);
#32018=CIRCLE('',#81921,14.55968693025);
#32019=CIRCLE('',#81922,14.87786051511);
#32020=CIRCLE('',#81924,15.10412140798);
#32021=CIRCLE('',#81925,15.41105880551);
#32022=CIRCLE('',#81927,14.37130764777);
#32023=CIRCLE('',#81928,14.69356095393);
#32024=CIRCLE('',#81930,14.98614304973);
#32025=CIRCLE('',#81931,15.29544813031);
#32026=CIRCLE('',#81933,14.55968693025);
#32027=CIRCLE('',#81934,14.87786051511);
#32028=CIRCLE('',#81936,15.28837739941);
#32029=CIRCLE('',#81937,15.59168796208);
#32030=CIRCLE('',#81939,14.37130764777);
#32031=CIRCLE('',#81940,14.69356095393);
#32032=CIRCLE('',#81942,15.20475200412);
#32033=CIRCLE('',#81943,15.50969804693);
#32034=CIRCLE('',#81945,14.55968693025);
#32035=CIRCLE('',#81946,14.87786051511);
#32036=CIRCLE('',#81948,15.40566400734);
#32037=CIRCLE('',#81949,15.70670982437);
#32038=CIRCLE('',#81951,14.37130764777);
#32039=CIRCLE('',#81952,14.69356095393);
#32040=CIRCLE('',#81954,15.35527542921);
#32041=CIRCLE('',#81955,15.65729010739);
#32042=CIRCLE('',#81957,14.55968693025);
#32043=CIRCLE('',#81958,14.87786051511);
#32044=CIRCLE('',#81960,15.45750573369);
#32045=CIRCLE('',#81961,15.75756115352);
#32046=CIRCLE('',#81963,14.37130764777);
#32047=CIRCLE('',#81964,14.69356095393);
#32048=CIRCLE('',#81966,15.43970477396);
#32049=CIRCLE('',#81967,15.7400995393);
#32050=CIRCLE('',#81969,14.55968693025);
#32051=CIRCLE('',#81970,14.87786051511);
#32052=CIRCLE('',#81972,15.44456161589);
#32053=CIRCLE('',#81973,15.74486371827);
#32054=CIRCLE('',#81975,14.37130764777);
#32055=CIRCLE('',#81976,14.69356095393);
#32056=CIRCLE('',#81978,15.45912298634);
#32057=CIRCLE('',#81979,15.75914761359);
#32058=CIRCLE('',#81981,14.55968693025);
#32059=CIRCLE('',#81982,14.87786051511);
#32060=CIRCLE('',#81984,15.36666793768);
#32061=CIRCLE('',#81985,15.66846302312);
#32062=CIRCLE('',#81987,14.37130764777);
#32063=CIRCLE('',#81988,14.69356095393);
#32064=CIRCLE('',#81990,15.41377577062);
#32065=CIRCLE('',#81991,15.71466619139);
#32066=CIRCLE('',#81993,14.55968693025);
#32067=CIRCLE('',#81994,14.87786051511);
#32068=CIRCLE('',#81996,15.22282771061);
#32069=CIRCLE('',#81997,15.52741876511);
#32070=CIRCLE('',#81999,14.37130764777);
#32071=CIRCLE('',#82000,14.69356095393);
#32072=CIRCLE('',#82002,15.3030873848);
#32073=CIRCLE('',#82003,15.60611205608);
#32074=CIRCLE('',#82005,14.55968693025);
#32075=CIRCLE('',#82006,14.87786051511);
#32076=CIRCLE('',#82008,15.01114530963);
#32077=CIRCLE('',#82009,15.31994561044);
#32078=CIRCLE('',#82011,14.37130764777);
#32079=CIRCLE('',#82012,14.69356095393);
#32080=CIRCLE('',#82014,15.12562340887);
#32081=CIRCLE('',#82015,15.4321331483);
#32082=CIRCLE('',#82017,14.55968693025);
#32083=CIRCLE('',#82018,14.87786051511);
#32084=CIRCLE('',#82020,14.72869592011);
#32085=CIRCLE('',#82021,15.0432953008);
#32086=CIRCLE('',#82023,14.37130764777);
#32087=CIRCLE('',#82024,14.69356095393);
#32088=CIRCLE('',#82026,14.87899470754);
#32089=CIRCLE('',#82027,15.19048167462);
#32090=CIRCLE('',#82029,14.55968693025);
#32091=CIRCLE('',#82030,14.87786051511);
#32092=CIRCLE('',#82032,14.37130764777);
#32093=CIRCLE('',#82033,14.69356095393);
#32094=CIRCLE('',#82035,14.37130764777);
#32095=CIRCLE('',#82036,14.69356095393);
#32096=CIRCLE('',#82038,14.55968693025);
#32097=CIRCLE('',#82039,14.87786051511);
#32098=CIRCLE('',#82041,14.87899470754);
#32099=CIRCLE('',#82042,15.19048167462);
#32100=CIRCLE('',#82044,14.37130764777);
#32101=CIRCLE('',#82045,14.69356095393);
#32102=CIRCLE('',#82047,14.72869592011);
#32103=CIRCLE('',#82048,15.0432953008);
#32104=CIRCLE('',#82050,14.55968693025);
#32105=CIRCLE('',#82051,14.87786051511);
#32106=CIRCLE('',#82053,15.12562340887);
#32107=CIRCLE('',#82054,15.4321331483);
#32108=CIRCLE('',#82056,14.37130764777);
#32109=CIRCLE('',#82057,14.69356095393);
#32110=CIRCLE('',#82059,15.01114530963);
#32111=CIRCLE('',#82060,15.31994561044);
#32112=CIRCLE('',#82062,14.55968693025);
#32113=CIRCLE('',#82063,14.87786051511);
#32114=CIRCLE('',#82065,15.3030873848);
#32115=CIRCLE('',#82066,15.60611205608);
#32116=CIRCLE('',#82068,14.37130764777);
#32117=CIRCLE('',#82069,14.69356095393);
#32118=CIRCLE('',#82071,15.22282771061);
#32119=CIRCLE('',#82072,15.52741876511);
#32120=CIRCLE('',#82074,14.55968693025);
#32121=CIRCLE('',#82075,14.87786051511);
#32122=CIRCLE('',#82077,15.41377577062);
#32123=CIRCLE('',#82078,15.71466619139);
#32124=CIRCLE('',#82080,14.37130764777);
#32125=CIRCLE('',#82081,14.69356095393);
#32126=CIRCLE('',#82083,15.36666793768);
#32127=CIRCLE('',#82084,15.66846302312);
#32128=CIRCLE('',#82086,14.55968693025);
#32129=CIRCLE('',#82087,14.87786051511);
#32130=CIRCLE('',#82089,15.45912298634);
#32131=CIRCLE('',#82090,15.75914761359);
#32132=CIRCLE('',#82092,14.37130764777);
#32133=CIRCLE('',#82093,14.69356095393);
#32134=CIRCLE('',#82095,15.44456161589);
#32135=CIRCLE('',#82096,15.74486371827);
#32136=CIRCLE('',#82098,14.55968693025);
#32137=CIRCLE('',#82099,14.87786051511);
#32138=CIRCLE('',#82101,15.10412140798);
#32139=CIRCLE('',#82102,15.41105880551);
#32140=CIRCLE('',#82104,15.44456161589);
#32141=CIRCLE('',#82105,15.74486371827);
#32142=CIRCLE('',#82107,14.98614304973);
#32143=CIRCLE('',#82108,15.29544813031);
#32144=CIRCLE('',#82110,15.45912298634);
#32145=CIRCLE('',#82111,15.75914761359);
#32146=CIRCLE('',#82113,15.41377577062);
#32147=CIRCLE('',#82114,15.71466619139);
#32148=CIRCLE('',#82116,15.10412140798);
#32149=CIRCLE('',#82117,15.41105880551);
#32150=CIRCLE('',#82119,15.36666793768);
#32151=CIRCLE('',#82120,15.66846302312);
#32152=CIRCLE('',#82122,14.98614304973);
#32153=CIRCLE('',#82123,15.29544813031);
#32154=CIRCLE('',#82125,15.3030873848);
#32155=CIRCLE('',#82126,15.60611205608);
#32156=CIRCLE('',#82128,15.10412140798);
#32157=CIRCLE('',#82129,15.41105880551);
#32158=CIRCLE('',#82131,15.22282771061);
#32159=CIRCLE('',#82132,15.52741876511);
#32160=CIRCLE('',#82134,14.98614304973);
#32161=CIRCLE('',#82135,15.29544813031);
#32162=CIRCLE('',#82137,15.12562340887);
#32163=CIRCLE('',#82138,15.4321331483);
#32164=CIRCLE('',#82140,15.10412140798);
#32165=CIRCLE('',#82141,15.41105880551);
#32166=CIRCLE('',#82143,15.01114530963);
#32167=CIRCLE('',#82144,15.31994561044);
#32168=CIRCLE('',#82146,14.98614304973);
#32169=CIRCLE('',#82147,15.29544813031);
#32170=CIRCLE('',#82149,14.87899470754);
#32171=CIRCLE('',#82150,15.19048167462);
#32172=CIRCLE('',#82152,15.10412140798);
#32173=CIRCLE('',#82153,15.41105880551);
#32174=CIRCLE('',#82155,14.72869592011);
#32175=CIRCLE('',#82156,15.0432953008);
#32176=CIRCLE('',#82158,14.98614304973);
#32177=CIRCLE('',#82159,15.29544813031);
#32178=CIRCLE('',#82161,14.87899470754);
#32179=CIRCLE('',#82162,15.19048167462);
#32180=CIRCLE('',#82164,15.28837739941);
#32181=CIRCLE('',#82165,15.59168796208);
#32182=CIRCLE('',#82167,14.72869592011);
#32183=CIRCLE('',#82168,15.0432953008);
#32184=CIRCLE('',#82170,15.20475200412);
#32185=CIRCLE('',#82171,15.50969804693);
#32186=CIRCLE('',#82173,14.87899470754);
#32187=CIRCLE('',#82174,15.19048167462);
#32188=CIRCLE('',#82176,15.40566400734);
#32189=CIRCLE('',#82177,15.70670982437);
#32190=CIRCLE('',#82179,14.72869592011);
#32191=CIRCLE('',#82180,15.0432953008);
#32192=CIRCLE('',#82182,15.35527542921);
#32193=CIRCLE('',#82183,15.65729010739);
#32194=CIRCLE('',#82185,14.87899470754);
#32195=CIRCLE('',#82186,15.19048167462);
#32196=CIRCLE('',#82188,15.45750573369);
#32197=CIRCLE('',#82189,15.75756115352);
#32198=CIRCLE('',#82191,14.72869592011);
#32199=CIRCLE('',#82192,15.0432953008);
#32200=CIRCLE('',#82194,15.43970477396);
#32201=CIRCLE('',#82195,15.7400995393);
#32202=CIRCLE('',#82197,14.87899470754);
#32203=CIRCLE('',#82198,15.19048167462);
#32204=CIRCLE('',#82200,15.44456161589);
#32205=CIRCLE('',#82201,15.74486371827);
#32206=CIRCLE('',#82203,14.72869592011);
#32207=CIRCLE('',#82204,15.0432953008);
#32208=CIRCLE('',#82206,15.45912298634);
#32209=CIRCLE('',#82207,15.75914761359);
#32210=CIRCLE('',#82209,14.87899470754);
#32211=CIRCLE('',#82210,15.19048167462);
#32212=CIRCLE('',#82212,15.36666793768);
#32213=CIRCLE('',#82213,15.66846302312);
#32214=CIRCLE('',#82215,14.72869592011);
#32215=CIRCLE('',#82216,15.0432953008);
#32216=CIRCLE('',#82218,15.41377577062);
#32217=CIRCLE('',#82219,15.71466619139);
#32218=CIRCLE('',#82221,14.87899470754);
#32219=CIRCLE('',#82222,15.19048167462);
#32220=CIRCLE('',#82224,15.22282771061);
#32221=CIRCLE('',#82225,15.52741876511);
#32222=CIRCLE('',#82227,14.72869592011);
#32223=CIRCLE('',#82228,15.0432953008);
#32224=CIRCLE('',#82230,15.3030873848);
#32225=CIRCLE('',#82231,15.60611205608);
#32226=CIRCLE('',#82233,14.87899470754);
#32227=CIRCLE('',#82234,15.19048167462);
#32228=CIRCLE('',#82236,15.01114530963);
#32229=CIRCLE('',#82237,15.31994561044);
#32230=CIRCLE('',#82239,14.72869592011);
#32231=CIRCLE('',#82240,15.0432953008);
#32232=CIRCLE('',#82242,15.12562340887);
#32233=CIRCLE('',#82243,15.4321331483);
#32234=CIRCLE('',#82245,14.87899470754);
#32235=CIRCLE('',#82246,15.19048167462);
#32236=CIRCLE('',#82248,14.72869592011);
#32237=CIRCLE('',#82249,15.0432953008);
#32238=CIRCLE('',#82251,14.72869592011);
#32239=CIRCLE('',#82252,15.0432953008);
#32240=CIRCLE('',#82254,14.87899470754);
#32241=CIRCLE('',#82255,15.19048167462);
#32242=CIRCLE('',#82257,15.12562340887);
#32243=CIRCLE('',#82258,15.4321331483);
#32244=CIRCLE('',#82260,14.72869592011);
#32245=CIRCLE('',#82261,15.0432953008);
#32246=CIRCLE('',#82263,15.01114530963);
#32247=CIRCLE('',#82264,15.31994561044);
#32248=CIRCLE('',#82266,14.87899470754);
#32249=CIRCLE('',#82267,15.19048167462);
#32250=CIRCLE('',#82269,15.3030873848);
#32251=CIRCLE('',#82270,15.60611205608);
#32252=CIRCLE('',#82272,14.72869592011);
#32253=CIRCLE('',#82273,15.0432953008);
#32254=CIRCLE('',#82275,15.22282771061);
#32255=CIRCLE('',#82276,15.52741876511);
#32256=CIRCLE('',#82278,14.87899470754);
#32257=CIRCLE('',#82279,15.19048167462);
#32258=CIRCLE('',#82281,15.41377577062);
#32259=CIRCLE('',#82282,15.71466619139);
#32260=CIRCLE('',#82284,14.72869592011);
#32261=CIRCLE('',#82285,15.0432953008);
#32262=CIRCLE('',#82287,15.36666793768);
#32263=CIRCLE('',#82288,15.66846302312);
#32264=CIRCLE('',#82290,14.87899470754);
#32265=CIRCLE('',#82291,15.19048167462);
#32266=CIRCLE('',#82293,15.45912298634);
#32267=CIRCLE('',#82294,15.75914761359);
#32268=CIRCLE('',#82296,14.72869592011);
#32269=CIRCLE('',#82297,15.0432953008);
#32270=CIRCLE('',#82299,15.44456161589);
#32271=CIRCLE('',#82300,15.74486371827);
#32272=CIRCLE('',#82302,14.87899470754);
#32273=CIRCLE('',#82303,15.19048167462);
#32274=CIRCLE('',#82305,15.45912298634);
#32275=CIRCLE('',#82306,15.75914761359);
#32276=CIRCLE('',#82308,15.28837739941);
#32277=CIRCLE('',#82309,15.59168796208);
#32278=CIRCLE('',#82311,15.44456161589);
#32279=CIRCLE('',#82312,15.74486371827);
#32280=CIRCLE('',#82314,15.20475200412);
#32281=CIRCLE('',#82315,15.50969804693);
#32282=CIRCLE('',#82317,15.41377577062);
#32283=CIRCLE('',#82318,15.71466619139);
#32284=CIRCLE('',#82320,15.28837739941);
#32285=CIRCLE('',#82321,15.59168796208);
#32286=CIRCLE('',#82323,15.36666793768);
#32287=CIRCLE('',#82324,15.66846302312);
#32288=CIRCLE('',#82326,15.20475200412);
#32289=CIRCLE('',#82327,15.50969804693);
#32290=CIRCLE('',#82329,15.3030873848);
#32291=CIRCLE('',#82330,15.60611205608);
#32292=CIRCLE('',#82332,15.28837739941);
#32293=CIRCLE('',#82333,15.59168796208);
#32294=CIRCLE('',#82335,15.22282771061);
#32295=CIRCLE('',#82336,15.52741876511);
#32296=CIRCLE('',#82338,15.20475200412);
#32297=CIRCLE('',#82339,15.50969804693);
#32298=CIRCLE('',#82341,15.12562340887);
#32299=CIRCLE('',#82342,15.4321331483);
#32300=CIRCLE('',#82344,15.28837739941);
#32301=CIRCLE('',#82345,15.59168796208);
#32302=CIRCLE('',#82347,15.01114530963);
#32303=CIRCLE('',#82348,15.31994561044);
#32304=CIRCLE('',#82350,15.20475200412);
#32305=CIRCLE('',#82351,15.50969804693);
#32306=CIRCLE('',#82353,15.12562340887);
#32307=CIRCLE('',#82354,15.4321331483);
#32308=CIRCLE('',#82356,15.40566400734);
#32309=CIRCLE('',#82357,15.70670982437);
#32310=CIRCLE('',#82359,15.01114530963);
#32311=CIRCLE('',#82360,15.31994561044);
#32312=CIRCLE('',#82362,15.35527542921);
#32313=CIRCLE('',#82363,15.65729010739);
#32314=CIRCLE('',#82365,15.12562340887);
#32315=CIRCLE('',#82366,15.4321331483);
#32316=CIRCLE('',#82368,15.45750573369);
#32317=CIRCLE('',#82369,15.75756115352);
#32318=CIRCLE('',#82371,15.01114530963);
#32319=CIRCLE('',#82372,15.31994561044);
#32320=CIRCLE('',#82374,15.43970477396);
#32321=CIRCLE('',#82375,15.7400995393);
#32322=CIRCLE('',#82377,15.12562340887);
#32323=CIRCLE('',#82378,15.4321331483);
#32324=CIRCLE('',#82380,15.44456161589);
#32325=CIRCLE('',#82381,15.74486371827);
#32326=CIRCLE('',#82383,15.01114530963);
#32327=CIRCLE('',#82384,15.31994561044);
#32328=CIRCLE('',#82386,15.45912298634);
#32329=CIRCLE('',#82387,15.75914761359);
#32330=CIRCLE('',#82389,15.12562340887);
#32331=CIRCLE('',#82390,15.4321331483);
#32332=CIRCLE('',#82392,15.36666793768);
#32333=CIRCLE('',#82393,15.66846302312);
#32334=CIRCLE('',#82395,15.01114530963);
#32335=CIRCLE('',#82396,15.31994561044);
#32336=CIRCLE('',#82398,15.41377577062);
#32337=CIRCLE('',#82399,15.71466619139);
#32338=CIRCLE('',#82401,15.12562340887);
#32339=CIRCLE('',#82402,15.4321331483);
#32340=CIRCLE('',#82404,15.22282771061);
#32341=CIRCLE('',#82405,15.52741876511);
#32342=CIRCLE('',#82407,15.01114530963);
#32343=CIRCLE('',#82408,15.31994561044);
#32344=CIRCLE('',#82410,15.3030873848);
#32345=CIRCLE('',#82411,15.60611205608);
#32346=CIRCLE('',#82413,15.12562340887);
#32347=CIRCLE('',#82414,15.4321331483);
#32348=CIRCLE('',#82416,15.01114530963);
#32349=CIRCLE('',#82417,15.31994561044);
#32350=CIRCLE('',#82419,15.01114530963);
#32351=CIRCLE('',#82420,15.31994561044);
#32352=CIRCLE('',#82422,15.12562340887);
#32353=CIRCLE('',#82423,15.4321331483);
#32354=CIRCLE('',#82425,15.3030873848);
#32355=CIRCLE('',#82426,15.60611205608);
#32356=CIRCLE('',#82428,15.01114530963);
#32357=CIRCLE('',#82429,15.31994561044);
#32358=CIRCLE('',#82431,15.22282771061);
#32359=CIRCLE('',#82432,15.52741876511);
#32360=CIRCLE('',#82434,15.12562340887);
#32361=CIRCLE('',#82435,15.4321331483);
#32362=CIRCLE('',#82437,15.41377577062);
#32363=CIRCLE('',#82438,15.71466619139);
#32364=CIRCLE('',#82440,15.01114530963);
#32365=CIRCLE('',#82441,15.31994561044);
#32366=CIRCLE('',#82443,15.36666793768);
#32367=CIRCLE('',#82444,15.66846302312);
#32368=CIRCLE('',#82446,15.12562340887);
#32369=CIRCLE('',#82447,15.4321331483);
#32370=CIRCLE('',#82449,15.45912298634);
#32371=CIRCLE('',#82450,15.75914761359);
#32372=CIRCLE('',#82452,15.01114530963);
#32373=CIRCLE('',#82453,15.31994561044);
#32374=CIRCLE('',#82455,15.44456161589);
#32375=CIRCLE('',#82456,15.74486371827);
#32376=CIRCLE('',#82458,15.12562340887);
#32377=CIRCLE('',#82459,15.4321331483);
#32378=CIRCLE('',#82461,15.45912298634);
#32379=CIRCLE('',#82462,15.75914761359);
#32380=CIRCLE('',#82464,15.40566400734);
#32381=CIRCLE('',#82465,15.70670982437);
#32382=CIRCLE('',#82467,15.44456161589);
#32383=CIRCLE('',#82468,15.74486371827);
#32384=CIRCLE('',#82470,15.35527542921);
#32385=CIRCLE('',#82471,15.65729010739);
#32386=CIRCLE('',#82473,15.41377577062);
#32387=CIRCLE('',#82474,15.71466619139);
#32388=CIRCLE('',#82476,15.40566400734);
#32389=CIRCLE('',#82477,15.70670982437);
#32390=CIRCLE('',#82479,15.36666793768);
#32391=CIRCLE('',#82480,15.66846302312);
#32392=CIRCLE('',#82482,15.35527542921);
#32393=CIRCLE('',#82483,15.65729010739);
#32394=CIRCLE('',#82485,15.3030873848);
#32395=CIRCLE('',#82486,15.60611205608);
#32396=CIRCLE('',#82488,15.40566400734);
#32397=CIRCLE('',#82489,15.70670982437);
#32398=CIRCLE('',#82491,15.22282771061);
#32399=CIRCLE('',#82492,15.52741876511);
#32400=CIRCLE('',#82494,15.35527542921);
#32401=CIRCLE('',#82495,15.65729010739);
#32402=CIRCLE('',#82497,15.3030873848);
#32403=CIRCLE('',#82498,15.60611205608);
#32404=CIRCLE('',#82500,15.45750573369);
#32405=CIRCLE('',#82501,15.75756115352);
#32406=CIRCLE('',#82503,15.22282771061);
#32407=CIRCLE('',#82504,15.52741876511);
#32408=CIRCLE('',#82506,15.43970477396);
#32409=CIRCLE('',#82507,15.7400995393);
#32410=CIRCLE('',#82509,15.3030873848);
#32411=CIRCLE('',#82510,15.60611205608);
#32412=CIRCLE('',#82512,15.44456161589);
#32413=CIRCLE('',#82513,15.74486371827);
#32414=CIRCLE('',#82515,15.22282771061);
#32415=CIRCLE('',#82516,15.52741876511);
#32416=CIRCLE('',#82518,15.45912298634);
#32417=CIRCLE('',#82519,15.75914761359);
#32418=CIRCLE('',#82521,15.3030873848);
#32419=CIRCLE('',#82522,15.60611205608);
#32420=CIRCLE('',#82524,15.36666793768);
#32421=CIRCLE('',#82525,15.66846302312);
#32422=CIRCLE('',#82527,15.22282771061);
#32423=CIRCLE('',#82528,15.52741876511);
#32424=CIRCLE('',#82530,15.41377577062);
#32425=CIRCLE('',#82531,15.71466619139);
#32426=CIRCLE('',#82533,15.3030873848);
#32427=CIRCLE('',#82534,15.60611205608);
#32428=CIRCLE('',#82536,15.22282771061);
#32429=CIRCLE('',#82537,15.52741876511);
#32430=CIRCLE('',#82539,15.22282771061);
#32431=CIRCLE('',#82540,15.52741876511);
#32432=CIRCLE('',#82542,15.3030873848);
#32433=CIRCLE('',#82543,15.60611205608);
#32434=CIRCLE('',#82545,15.41377577062);
#32435=CIRCLE('',#82546,15.71466619139);
#32436=CIRCLE('',#82548,15.22282771061);
#32437=CIRCLE('',#82549,15.52741876511);
#32438=CIRCLE('',#82551,15.36666793768);
#32439=CIRCLE('',#82552,15.66846302312);
#32440=CIRCLE('',#82554,15.3030873848);
#32441=CIRCLE('',#82555,15.60611205608);
#32442=CIRCLE('',#82557,15.45912298634);
#32443=CIRCLE('',#82558,15.75914761359);
#32444=CIRCLE('',#82560,15.22282771061);
#32445=CIRCLE('',#82561,15.52741876511);
#32446=CIRCLE('',#82563,15.44456161589);
#32447=CIRCLE('',#82564,15.74486371827);
#32448=CIRCLE('',#82566,15.3030873848);
#32449=CIRCLE('',#82567,15.60611205608);
#32450=CIRCLE('',#82569,15.45912298634);
#32451=CIRCLE('',#82570,15.75914761359);
#32452=CIRCLE('',#82572,15.45750573369);
#32453=CIRCLE('',#82573,15.75756115352);
#32454=CIRCLE('',#82575,15.44456161589);
#32455=CIRCLE('',#82576,15.74486371827);
#32456=CIRCLE('',#82578,15.43970477396);
#32457=CIRCLE('',#82579,15.7400995393);
#32458=CIRCLE('',#82581,15.41377577062);
#32459=CIRCLE('',#82582,15.71466619139);
#32460=CIRCLE('',#82584,15.45750573369);
#32461=CIRCLE('',#82585,15.75756115352);
#32462=CIRCLE('',#82587,15.36666793768);
#32463=CIRCLE('',#82588,15.66846302312);
#32464=CIRCLE('',#82590,15.43970477396);
#32465=CIRCLE('',#82591,15.7400995393);
#32466=CIRCLE('',#82593,15.41377577062);
#32467=CIRCLE('',#82594,15.71466619139);
#32468=CIRCLE('',#82596,15.44456161589);
#32469=CIRCLE('',#82597,15.74486371827);
#32470=CIRCLE('',#82599,15.36666793768);
#32471=CIRCLE('',#82600,15.66846302312);
#32472=CIRCLE('',#82602,15.45912298634);
#32473=CIRCLE('',#82603,15.75914761359);
#32474=CIRCLE('',#82605,15.41377577062);
#32475=CIRCLE('',#82606,15.71466619139);
#32476=CIRCLE('',#82608,15.36666793768);
#32477=CIRCLE('',#82609,15.66846302312);
#32478=CIRCLE('',#82611,15.36666793768);
#32479=CIRCLE('',#82612,15.66846302312);
#32480=CIRCLE('',#82614,15.41377577062);
#32481=CIRCLE('',#82615,15.71466619139);
#32482=CIRCLE('',#82617,15.45912298634);
#32483=CIRCLE('',#82618,15.75914761359);
#32484=CIRCLE('',#82620,15.36666793768);
#32485=CIRCLE('',#82621,15.66846302312);
#32486=CIRCLE('',#82623,15.44456161589);
#32487=CIRCLE('',#82624,15.74486371827);
#32488=CIRCLE('',#82626,15.41377577062);
#32489=CIRCLE('',#82627,15.71466619139);
#32490=CIRCLE('',#82629,13.04356099794);
#32491=CIRCLE('',#82630,13.39778838118);
#32492=CIRCLE('',#82632,15.3030873848);
#32493=CIRCLE('',#82633,15.60611205608);
#32494=CIRCLE('',#82635,13.07481294348);
#32495=CIRCLE('',#82637,15.52741876511);
#32496=CIRCLE('',#82639,8.729046339664);
#32497=CIRCLE('',#82641,13.04356099794);
#32498=CIRCLE('',#82642,13.39778838118);
#32499=CIRCLE('',#82644,15.41377577062);
#32500=CIRCLE('',#82645,15.71466619139);
#32501=CIRCLE('',#82647,13.07481294348);
#32502=CIRCLE('',#82649,15.36666793768);
#32503=CIRCLE('',#82650,15.66846302312);
#32504=CIRCLE('',#82652,8.72904633966401);
#32505=CIRCLE('',#82654,13.04356099794);
#32506=CIRCLE('',#82655,13.39778838118);
#32507=CIRCLE('',#82657,15.45912298634);
#32508=CIRCLE('',#82658,15.75914761359);
#32509=CIRCLE('',#82660,13.07481294348);
#32510=CIRCLE('',#82662,15.44456161589);
#32511=CIRCLE('',#82663,15.74486371827);
#32512=CIRCLE('',#82665,8.729046339664);
#32513=CIRCLE('',#82667,13.04356099794);
#32514=CIRCLE('',#82668,13.39778838118);
#32515=CIRCLE('',#82670,15.43970477396);
#32516=CIRCLE('',#82671,15.7400995393);
#32517=CIRCLE('',#82673,13.07481294348);
#32518=CIRCLE('',#82675,15.45750573369);
#32519=CIRCLE('',#82676,15.75756115352);
#32520=CIRCLE('',#82678,8.729046339664);
#32521=CIRCLE('',#82680,13.04356099794);
#32522=CIRCLE('',#82681,13.39778838118);
#32523=CIRCLE('',#82683,15.35527542921);
#32524=CIRCLE('',#82684,15.65729010739);
#32525=CIRCLE('',#82686,13.07481294348);
#32526=CIRCLE('',#82688,15.40566400734);
#32527=CIRCLE('',#82689,15.70670982437);
#32528=CIRCLE('',#82691,8.729046339664);
#32529=CIRCLE('',#82693,13.04356099794);
#32530=CIRCLE('',#82694,13.39778838118);
#32531=CIRCLE('',#82696,15.50969804693);
#32532=CIRCLE('',#82698,13.07481294348);
#32533=CIRCLE('',#82700,15.28837739941);
#32534=CIRCLE('',#82701,15.59168796208);
#32535=CIRCLE('',#82703,8.729046339664);
#32536=CIRCLE('',#82705,15.28837739941);
#32537=CIRCLE('',#82706,15.59168796208);
#32538=CIRCLE('',#82708,13.07481294348);
#32539=CIRCLE('',#82710,15.50969804693);
#32540=CIRCLE('',#82712,13.04356099794);
#32541=CIRCLE('',#82713,13.39778838118);
#32542=CIRCLE('',#82715,8.729046339664);
#32543=CIRCLE('',#82717,13.04356099794);
#32544=CIRCLE('',#82718,13.39778838118);
#32545=CIRCLE('',#82720,15.40566400734);
#32546=CIRCLE('',#82721,15.70670982437);
#32547=CIRCLE('',#82723,13.07481294348);
#32548=CIRCLE('',#82725,15.35527542921);
#32549=CIRCLE('',#82726,15.65729010739);
#32550=CIRCLE('',#82728,8.729046339664);
#32551=CIRCLE('',#82730,13.04356099794);
#32552=CIRCLE('',#82731,13.39778838118);
#32553=CIRCLE('',#82733,15.45750573369);
#32554=CIRCLE('',#82734,15.75756115352);
#32555=CIRCLE('',#82736,13.07481294348);
#32556=CIRCLE('',#82738,15.43970477396);
#32557=CIRCLE('',#82739,15.7400995393);
#32558=CIRCLE('',#82741,8.729046339664);
#32559=CIRCLE('',#82743,13.62844391363);
#32560=CIRCLE('',#82744,13.96784641621);
#32561=CIRCLE('',#82746,14.87899470754);
#32562=CIRCLE('',#82747,15.19048167462);
#32563=CIRCLE('',#82749,13.69491633808);
#32564=CIRCLE('',#82751,14.72869592011);
#32565=CIRCLE('',#82752,15.0432953008);
#32566=CIRCLE('',#82754,8.729046339664);
#32567=CIRCLE('',#82756,13.34857608537);
#32568=CIRCLE('',#82757,13.69491633808);
#32569=CIRCLE('',#82759,15.01114530963);
#32570=CIRCLE('',#82760,15.31994561044);
#32571=CIRCLE('',#82762,13.62844391363);
#32572=CIRCLE('',#82763,13.96784641621);
#32573=CIRCLE('',#82765,15.12562340887);
#32574=CIRCLE('',#82766,15.4321331483);
#32575=CIRCLE('',#82768,13.34857608537);
#32576=CIRCLE('',#82769,13.69491633808);
#32577=CIRCLE('',#82771,15.22282771061);
#32578=CIRCLE('',#82772,15.52741876511);
#32579=CIRCLE('',#82774,13.62844391363);
#32580=CIRCLE('',#82775,13.96784641621);
#32581=CIRCLE('',#82777,15.3030873848);
#32582=CIRCLE('',#82778,15.60611205608);
#32583=CIRCLE('',#82780,13.34857608537);
#32584=CIRCLE('',#82781,13.69491633808);
#32585=CIRCLE('',#82783,15.36666793768);
#32586=CIRCLE('',#82784,15.66846302312);
#32587=CIRCLE('',#82786,13.62844391363);
#32588=CIRCLE('',#82787,13.96784641621);
#32589=CIRCLE('',#82789,15.41377577062);
#32590=CIRCLE('',#82790,15.71466619139);
#32591=CIRCLE('',#82792,13.34857608537);
#32592=CIRCLE('',#82793,13.69491633808);
#32593=CIRCLE('',#82795,15.44456161589);
#32594=CIRCLE('',#82796,15.74486371827);
#32595=CIRCLE('',#82798,13.62844391363);
#32596=CIRCLE('',#82799,13.96784641621);
#32597=CIRCLE('',#82801,15.45912298634);
#32598=CIRCLE('',#82802,15.75914761359);
#32599=CIRCLE('',#82804,13.34857608537);
#32600=CIRCLE('',#82805,13.69491633808);
#32601=CIRCLE('',#82807,15.45750573369);
#32602=CIRCLE('',#82808,15.75756115352);
#32603=CIRCLE('',#82810,13.62844391363);
#32604=CIRCLE('',#82811,13.96784641621);
#32605=CIRCLE('',#82813,15.43970477396);
#32606=CIRCLE('',#82814,15.7400995393);
#32607=CIRCLE('',#82816,13.34857608537);
#32608=CIRCLE('',#82817,13.69491633808);
#32609=CIRCLE('',#82819,15.40566400734);
#32610=CIRCLE('',#82820,15.70670982437);
#32611=CIRCLE('',#82822,13.62844391363);
#32612=CIRCLE('',#82823,13.96784641621);
#32613=CIRCLE('',#82825,15.35527542921);
#32614=CIRCLE('',#82826,15.65729010739);
#32615=CIRCLE('',#82828,13.34857608537);
#32616=CIRCLE('',#82829,13.69491633808);
#32617=CIRCLE('',#82831,15.28837739941);
#32618=CIRCLE('',#82832,15.59168796208);
#32619=CIRCLE('',#82834,13.62844391363);
#32620=CIRCLE('',#82835,13.96784641621);
#32621=CIRCLE('',#82837,15.20475200412);
#32622=CIRCLE('',#82838,15.50969804693);
#32623=CIRCLE('',#82840,13.34857608537);
#32624=CIRCLE('',#82841,13.69491633808);
#32625=CIRCLE('',#82843,15.10412140798);
#32626=CIRCLE('',#82844,15.41105880551);
#32627=CIRCLE('',#82846,13.62844391363);
#32628=CIRCLE('',#82847,13.96784641621);
#32629=CIRCLE('',#82849,14.98614304973);
#32630=CIRCLE('',#82850,15.29544813031);
#32631=CIRCLE('',#82852,13.62844391363);
#32632=CIRCLE('',#82853,13.96784641621);
#32633=CIRCLE('',#82855,15.01168656437);
#32634=CIRCLE('',#82857,13.69491633808);
#32635=CIRCLE('',#82859,14.8504034796);
#32636=CIRCLE('',#82860,15.16247781555);
#32637=CIRCLE('',#82862,8.729046339664);
#32638=CIRCLE('',#82864,14.8504034796);
#32639=CIRCLE('',#82865,15.16247781555);
#32640=CIRCLE('',#82867,13.69491633808);
#32641=CIRCLE('',#82869,15.01168656437);
#32642=CIRCLE('',#82871,13.62844391363);
#32643=CIRCLE('',#82872,13.96784641621);
#32644=CIRCLE('',#82874,8.729046339664);
#32645=CIRCLE('',#82876,13.62844391363);
#32646=CIRCLE('',#82877,13.96784641621);
#32647=CIRCLE('',#82879,15.10412140798);
#32648=CIRCLE('',#82880,15.41105880551);
#32649=CIRCLE('',#82882,13.34857608537);
#32650=CIRCLE('',#82883,13.69491633808);
#32651=CIRCLE('',#82885,14.98614304973);
#32652=CIRCLE('',#82886,15.29544813031);
#32653=CIRCLE('',#82888,15.20475200412);
#32654=CIRCLE('',#82889,15.50969804693);
#32655=CIRCLE('',#82891,13.62844391363);
#32656=CIRCLE('',#82892,13.96784641621);
#32657=CIRCLE('',#82894,15.28837739941);
#32658=CIRCLE('',#82895,15.59168796208);
#32659=CIRCLE('',#82897,13.34857608537);
#32660=CIRCLE('',#82898,13.69491633808);
#32661=CIRCLE('',#82900,15.35527542921);
#32662=CIRCLE('',#82901,15.65729010739);
#32663=CIRCLE('',#82903,13.62844391363);
#32664=CIRCLE('',#82904,13.96784641621);
#32665=CIRCLE('',#82906,15.40566400734);
#32666=CIRCLE('',#82907,15.70670982437);
#32667=CIRCLE('',#82909,13.34857608537);
#32668=CIRCLE('',#82910,13.69491633808);
#32669=CIRCLE('',#82912,15.43970477396);
#32670=CIRCLE('',#82913,15.7400995393);
#32671=CIRCLE('',#82915,13.62844391363);
#32672=CIRCLE('',#82916,13.96784641621);
#32673=CIRCLE('',#82918,15.45750573369);
#32674=CIRCLE('',#82919,15.75756115352);
#32675=CIRCLE('',#82921,13.34857608537);
#32676=CIRCLE('',#82922,13.69491633808);
#32677=CIRCLE('',#82924,15.45750573369);
#32678=CIRCLE('',#82925,15.75756115352);
#32679=CIRCLE('',#82927,13.1066579839);
#32680=CIRCLE('',#82928,13.45922484792);
#32681=CIRCLE('',#82930,15.43970477396);
#32682=CIRCLE('',#82931,15.7400995393);
#32683=CIRCLE('',#82933,12.78023800666);
#32684=CIRCLE('',#82934,13.14156510873);
#32685=CIRCLE('',#82936,8.729046339664);
#32686=CIRCLE('',#82938,13.1066579839);
#32687=CIRCLE('',#82939,13.45922484792);
#32688=CIRCLE('',#82941,15.35527542921);
#32689=CIRCLE('',#82942,15.65729010739);
#32690=CIRCLE('',#82944,13.14156510873);
#32691=CIRCLE('',#82946,15.40566400734);
#32692=CIRCLE('',#82947,15.70670982437);
#32693=CIRCLE('',#82949,8.729046339664);
#32694=CIRCLE('',#82951,13.1066579839);
#32695=CIRCLE('',#82952,13.45922484792);
#32696=CIRCLE('',#82954,15.20475200412);
#32697=CIRCLE('',#82955,15.50969804693);
#32698=CIRCLE('',#82957,13.14156510873);
#32699=CIRCLE('',#82959,15.28837739941);
#32700=CIRCLE('',#82960,15.59168796208);
#32701=CIRCLE('',#82962,8.729046339664);
#32702=CIRCLE('',#82964,14.1185864557);
#32703=CIRCLE('',#82965,14.4464782389);
#32704=CIRCLE('',#82967,14.55968693025);
#32705=CIRCLE('',#82968,14.87786051511);
#32706=CIRCLE('',#82970,13.88468521454);
#32707=CIRCLE('',#82971,14.21797220095);
#32708=CIRCLE('',#82973,14.37130764777);
#32709=CIRCLE('',#82974,14.69356095393);
#32710=CIRCLE('',#82976,8.72904633966401);
#32711=CIRCLE('',#82978,13.88468521454);
#32712=CIRCLE('',#82979,14.21797220095);
#32713=CIRCLE('',#82981,14.72869592011);
#32714=CIRCLE('',#82982,15.0432953008);
#32715=CIRCLE('',#82984,14.1185864557);
#32716=CIRCLE('',#82985,14.4464782389);
#32717=CIRCLE('',#82987,14.87899470754);
#32718=CIRCLE('',#82988,15.19048167462);
#32719=CIRCLE('',#82990,13.88468521454);
#32720=CIRCLE('',#82991,14.21797220095);
#32721=CIRCLE('',#82993,15.01114530963);
#32722=CIRCLE('',#82994,15.31994561044);
#32723=CIRCLE('',#82996,14.1185864557);
#32724=CIRCLE('',#82997,14.4464782389);
#32725=CIRCLE('',#82999,15.12562340887);
#32726=CIRCLE('',#83000,15.4321331483);
#32727=CIRCLE('',#83002,13.88468521454);
#32728=CIRCLE('',#83003,14.21797220095);
#32729=CIRCLE('',#83005,15.22282771061);
#32730=CIRCLE('',#83006,15.52741876511);
#32731=CIRCLE('',#83008,14.1185864557);
#32732=CIRCLE('',#83009,14.4464782389);
#32733=CIRCLE('',#83011,15.3030873848);
#32734=CIRCLE('',#83012,15.60611205608);
#32735=CIRCLE('',#83014,13.88468521454);
#32736=CIRCLE('',#83015,14.21797220095);
#32737=CIRCLE('',#83017,15.36666793768);
#32738=CIRCLE('',#83018,15.66846302312);
#32739=CIRCLE('',#83020,14.1185864557);
#32740=CIRCLE('',#83021,14.4464782389);
#32741=CIRCLE('',#83023,15.41377577062);
#32742=CIRCLE('',#83024,15.71466619139);
#32743=CIRCLE('',#83026,13.88468521454);
#32744=CIRCLE('',#83027,14.21797220095);
#32745=CIRCLE('',#83029,15.44456161589);
#32746=CIRCLE('',#83030,15.74486371827);
#32747=CIRCLE('',#83032,14.1185864557);
#32748=CIRCLE('',#83033,14.4464782389);
#32749=CIRCLE('',#83035,15.45912298634);
#32750=CIRCLE('',#83036,15.75914761359);
#32751=CIRCLE('',#83038,13.88468521454);
#32752=CIRCLE('',#83039,14.21797220095);
#32753=CIRCLE('',#83041,15.45750573369);
#32754=CIRCLE('',#83042,15.75756115352);
#32755=CIRCLE('',#83044,14.1185864557);
#32756=CIRCLE('',#83045,14.4464782389);
#32757=CIRCLE('',#83047,15.43970477396);
#32758=CIRCLE('',#83048,15.7400995393);
#32759=CIRCLE('',#83050,13.88468521454);
#32760=CIRCLE('',#83051,14.21797220095);
#32761=CIRCLE('',#83053,15.40566400734);
#32762=CIRCLE('',#83054,15.70670982437);
#32763=CIRCLE('',#83056,14.1185864557);
#32764=CIRCLE('',#83057,14.4464782389);
#32765=CIRCLE('',#83059,15.35527542921);
#32766=CIRCLE('',#83060,15.65729010739);
#32767=CIRCLE('',#83062,13.88468521454);
#32768=CIRCLE('',#83063,14.21797220095);
#32769=CIRCLE('',#83065,15.28837739941);
#32770=CIRCLE('',#83066,15.59168796208);
#32771=CIRCLE('',#83068,14.1185864557);
#32772=CIRCLE('',#83069,14.4464782389);
#32773=CIRCLE('',#83071,15.20475200412);
#32774=CIRCLE('',#83072,15.50969804693);
#32775=CIRCLE('',#83074,13.88468521454);
#32776=CIRCLE('',#83075,14.21797220095);
#32777=CIRCLE('',#83077,15.10412140798);
#32778=CIRCLE('',#83078,15.41105880551);
#32779=CIRCLE('',#83080,14.1185864557);
#32780=CIRCLE('',#83081,14.4464782389);
#32781=CIRCLE('',#83083,14.98614304973);
#32782=CIRCLE('',#83084,15.29544813031);
#32783=CIRCLE('',#83086,13.88468521454);
#32784=CIRCLE('',#83087,14.21797220095);
#32785=CIRCLE('',#83089,14.8504034796);
#32786=CIRCLE('',#83090,15.16247781555);
#32787=CIRCLE('',#83092,14.1185864557);
#32788=CIRCLE('',#83093,14.4464782389);
#32789=CIRCLE('',#83095,14.6964105654);
#32790=CIRCLE('',#83096,15.01168656437);
#32791=CIRCLE('',#83098,14.52358370055);
#32792=CIRCLE('',#83099,14.84253123652);
#32793=CIRCLE('',#83101,14.1185864557);
#32794=CIRCLE('',#83102,14.4464782389);
#32795=CIRCLE('',#83104,14.33124152008);
#32796=CIRCLE('',#83105,14.65437591667);
#32797=CIRCLE('',#83107,13.88468521454);
#32798=CIRCLE('',#83108,14.21797220095);
#32799=CIRCLE('',#83110,8.729046339664);
#32800=CIRCLE('',#83112,14.1185864557);
#32801=CIRCLE('',#83113,14.4464782389);
#32802=CIRCLE('',#83115,14.52358370055);
#32803=CIRCLE('',#83116,14.84253123652);
#32804=CIRCLE('',#83118,13.88468521454);
#32805=CIRCLE('',#83119,14.21797220095);
#32806=CIRCLE('',#83121,14.33124152008);
#32807=CIRCLE('',#83122,14.65437591667);
#32808=CIRCLE('',#83124,8.729046339664);
#32809=CIRCLE('',#83126,14.6964105654);
#32810=CIRCLE('',#83127,15.01168656437);
#32811=CIRCLE('',#83129,14.1185864557);
#32812=CIRCLE('',#83130,14.4464782389);
#32813=CIRCLE('',#83132,14.8504034796);
#32814=CIRCLE('',#83133,15.16247781555);
#32815=CIRCLE('',#83135,13.88468521454);
#32816=CIRCLE('',#83136,14.21797220095);
#32817=CIRCLE('',#83138,14.98614304973);
#32818=CIRCLE('',#83139,15.29544813031);
#32819=CIRCLE('',#83141,14.1185864557);
#32820=CIRCLE('',#83142,14.4464782389);
#32821=CIRCLE('',#83144,15.10412140798);
#32822=CIRCLE('',#83145,15.41105880551);
#32823=CIRCLE('',#83147,13.88468521454);
#32824=CIRCLE('',#83148,14.21797220095);
#32825=CIRCLE('',#83150,15.20475200412);
#32826=CIRCLE('',#83151,15.50969804693);
#32827=CIRCLE('',#83153,14.1185864557);
#32828=CIRCLE('',#83154,14.4464782389);
#32829=CIRCLE('',#83156,15.28837739941);
#32830=CIRCLE('',#83157,15.59168796208);
#32831=CIRCLE('',#83159,13.88468521454);
#32832=CIRCLE('',#83160,14.21797220095);
#32833=CIRCLE('',#83162,15.35527542921);
#32834=CIRCLE('',#83163,15.65729010739);
#32835=CIRCLE('',#83165,14.1185864557);
#32836=CIRCLE('',#83166,14.4464782389);
#32837=CIRCLE('',#83168,15.40566400734);
#32838=CIRCLE('',#83169,15.70670982437);
#32839=CIRCLE('',#83171,13.88468521454);
#32840=CIRCLE('',#83172,14.21797220095);
#32841=CIRCLE('',#83174,15.43970477396);
#32842=CIRCLE('',#83175,15.7400995393);
#32843=CIRCLE('',#83177,14.1185864557);
#32844=CIRCLE('',#83178,14.4464782389);
#32845=CIRCLE('',#83180,15.45750573369);
#32846=CIRCLE('',#83181,15.75756115352);
#32847=CIRCLE('',#83183,13.88468521454);
#32848=CIRCLE('',#83184,14.21797220095);
#32849=CIRCLE('',#83186,15.43970477396);
#32850=CIRCLE('',#83187,15.7400995393);
#32851=CIRCLE('',#83189,13.40650899776);
#32852=CIRCLE('',#83190,13.75139023906);
#32853=CIRCLE('',#83192,15.45750573369);
#32854=CIRCLE('',#83193,15.75756115352);
#32855=CIRCLE('',#83195,13.68153805341);
#32856=CIRCLE('',#83196,14.01965525635);
#32857=CIRCLE('',#83198,15.35527542921);
#32858=CIRCLE('',#83199,15.65729010739);
#32859=CIRCLE('',#83201,13.40650899776);
#32860=CIRCLE('',#83202,13.75139023906);
#32861=CIRCLE('',#83204,15.40566400734);
#32862=CIRCLE('',#83205,15.70670982437);
#32863=CIRCLE('',#83207,13.68153805341);
#32864=CIRCLE('',#83208,14.01965525635);
#32865=CIRCLE('',#83210,15.20475200412);
#32866=CIRCLE('',#83211,15.50969804693);
#32867=CIRCLE('',#83213,13.40650899776);
#32868=CIRCLE('',#83214,13.75139023906);
#32869=CIRCLE('',#83216,15.28837739941);
#32870=CIRCLE('',#83217,15.59168796208);
#32871=CIRCLE('',#83219,13.68153805341);
#32872=CIRCLE('',#83220,14.01965525635);
#32873=CIRCLE('',#83222,14.98614304973);
#32874=CIRCLE('',#83223,15.29544813031);
#32875=CIRCLE('',#83225,13.40650899776);
#32876=CIRCLE('',#83226,13.75139023906);
#32877=CIRCLE('',#83228,15.10412140798);
#32878=CIRCLE('',#83229,15.41105880551);
#32879=CIRCLE('',#83231,13.68153805341);
#32880=CIRCLE('',#83232,14.01965525635);
#32881=CIRCLE('',#83234,13.68153805341);
#32882=CIRCLE('',#83235,14.01965525635);
#32883=CIRCLE('',#83237,14.6964105654);
#32884=CIRCLE('',#83238,15.01168656437);
#32885=CIRCLE('',#83240,13.75139023906);
#32886=CIRCLE('',#83242,14.8504034796);
#32887=CIRCLE('',#83243,15.16247781555);
#32888=CIRCLE('',#83245,8.729046339664);
#32889=CIRCLE('',#83247,14.52358370055);
#32890=CIRCLE('',#83248,14.84253123652);
#32891=CIRCLE('',#83250,14.16278516066);
#32892=CIRCLE('',#83251,14.48967679098);
#32893=CIRCLE('',#83253,14.33124152008);
#32894=CIRCLE('',#83254,14.65437591667);
#32895=CIRCLE('',#83256,13.93321511737);
#32896=CIRCLE('',#83257,14.26536832707);
#32897=CIRCLE('',#83259,8.72904633966401);
#32898=CIRCLE('',#83261,14.33124152008);
#32899=CIRCLE('',#83262,14.65437591667);
#32900=CIRCLE('',#83264,14.37130764777);
#32901=CIRCLE('',#83265,14.69356095393);
#32902=CIRCLE('',#83267,14.52358370055);
#32903=CIRCLE('',#83268,14.84253123652);
#32904=CIRCLE('',#83270,14.55968693025);
#32905=CIRCLE('',#83271,14.87786051511);
#32906=CIRCLE('',#83273,14.33124152008);
#32907=CIRCLE('',#83274,14.65437591667);
#32908=CIRCLE('',#83276,14.72869592011);
#32909=CIRCLE('',#83277,15.0432953008);
#32910=CIRCLE('',#83279,14.52358370055);
#32911=CIRCLE('',#83280,14.84253123652);
#32912=CIRCLE('',#83282,14.87899470754);
#32913=CIRCLE('',#83283,15.19048167462);
#32914=CIRCLE('',#83285,14.33124152008);
#32915=CIRCLE('',#83286,14.65437591667);
#32916=CIRCLE('',#83288,15.01114530963);
#32917=CIRCLE('',#83289,15.31994561044);
#32918=CIRCLE('',#83291,14.52358370055);
#32919=CIRCLE('',#83292,14.84253123652);
#32920=CIRCLE('',#83294,15.12562340887);
#32921=CIRCLE('',#83295,15.4321331483);
#32922=CIRCLE('',#83297,14.33124152008);
#32923=CIRCLE('',#83298,14.65437591667);
#32924=CIRCLE('',#83300,15.22282771061);
#32925=CIRCLE('',#83301,15.52741876511);
#32926=CIRCLE('',#83303,14.52358370055);
#32927=CIRCLE('',#83304,14.84253123652);
#32928=CIRCLE('',#83306,15.3030873848);
#32929=CIRCLE('',#83307,15.60611205608);
#32930=CIRCLE('',#83309,14.33124152008);
#32931=CIRCLE('',#83310,14.65437591667);
#32932=CIRCLE('',#83312,15.36666793768);
#32933=CIRCLE('',#83313,15.66846302312);
#32934=CIRCLE('',#83315,14.52358370055);
#32935=CIRCLE('',#83316,14.84253123652);
#32936=CIRCLE('',#83318,15.41377577062);
#32937=CIRCLE('',#83319,15.71466619139);
#32938=CIRCLE('',#83321,14.33124152008);
#32939=CIRCLE('',#83322,14.65437591667);
#32940=CIRCLE('',#83324,15.44456161589);
#32941=CIRCLE('',#83325,15.74486371827);
#32942=CIRCLE('',#83327,14.52358370055);
#32943=CIRCLE('',#83328,14.84253123652);
#32944=CIRCLE('',#83330,15.45912298634);
#32945=CIRCLE('',#83331,15.75914761359);
#32946=CIRCLE('',#83333,14.33124152008);
#32947=CIRCLE('',#83334,14.65437591667);
#32948=CIRCLE('',#83336,15.45750573369);
#32949=CIRCLE('',#83337,15.75756115352);
#32950=CIRCLE('',#83339,14.52358370055);
#32951=CIRCLE('',#83340,14.84253123652);
#32952=CIRCLE('',#83342,15.43970477396);
#32953=CIRCLE('',#83343,15.7400995393);
#32954=CIRCLE('',#83345,14.33124152008);
#32955=CIRCLE('',#83346,14.65437591667);
#32956=CIRCLE('',#83348,15.40566400734);
#32957=CIRCLE('',#83349,15.70670982437);
#32958=CIRCLE('',#83351,14.52358370055);
#32959=CIRCLE('',#83352,14.84253123652);
#32960=CIRCLE('',#83354,15.35527542921);
#32961=CIRCLE('',#83355,15.65729010739);
#32962=CIRCLE('',#83357,14.33124152008);
#32963=CIRCLE('',#83358,14.65437591667);
#32964=CIRCLE('',#83360,15.28837739941);
#32965=CIRCLE('',#83361,15.59168796208);
#32966=CIRCLE('',#83363,14.52358370055);
#32967=CIRCLE('',#83364,14.84253123652);
#32968=CIRCLE('',#83366,15.20475200412);
#32969=CIRCLE('',#83367,15.50969804693);
#32970=CIRCLE('',#83369,14.33124152008);
#32971=CIRCLE('',#83370,14.65437591667);
#32972=CIRCLE('',#83372,15.10412140798);
#32973=CIRCLE('',#83373,15.41105880551);
#32974=CIRCLE('',#83375,14.52358370055);
#32975=CIRCLE('',#83376,14.84253123652);
#32976=CIRCLE('',#83378,14.98614304973);
#32977=CIRCLE('',#83379,15.29544813031);
#32978=CIRCLE('',#83381,14.33124152008);
#32979=CIRCLE('',#83382,14.65437591667);
#32980=CIRCLE('',#83384,14.8504034796);
#32981=CIRCLE('',#83385,15.16247781555);
#32982=CIRCLE('',#83387,14.52358370055);
#32983=CIRCLE('',#83388,14.84253123652);
#32984=CIRCLE('',#83390,14.6964105654);
#32985=CIRCLE('',#83391,15.01168656437);
#32986=CIRCLE('',#83393,14.33124152008);
#32987=CIRCLE('',#83394,14.65437591667);
#32988=CIRCLE('',#83396,14.52358370055);
#32989=CIRCLE('',#83397,14.84253123652);
#32990=CIRCLE('',#83399,14.52358370055);
#32991=CIRCLE('',#83400,14.84253123652);
#32992=CIRCLE('',#83402,14.33124152008);
#32993=CIRCLE('',#83403,14.65437591667);
#32994=CIRCLE('',#83405,14.6964105654);
#32995=CIRCLE('',#83406,15.01168656437);
#32996=CIRCLE('',#83408,14.52358370055);
#32997=CIRCLE('',#83409,14.84253123652);
#32998=CIRCLE('',#83411,14.8504034796);
#32999=CIRCLE('',#83412,15.16247781555);
#33000=CIRCLE('',#83414,14.33124152008);
#33001=CIRCLE('',#83415,14.65437591667);
#33002=CIRCLE('',#83417,14.98614304973);
#33003=CIRCLE('',#83418,15.29544813031);
#33004=CIRCLE('',#83420,14.52358370055);
#33005=CIRCLE('',#83421,14.84253123652);
#33006=CIRCLE('',#83423,15.10412140798);
#33007=CIRCLE('',#83424,15.41105880551);
#33008=CIRCLE('',#83426,14.33124152008);
#33009=CIRCLE('',#83427,14.65437591667);
#33010=CIRCLE('',#83429,15.20475200412);
#33011=CIRCLE('',#83430,15.50969804693);
#33012=CIRCLE('',#83432,14.52358370055);
#33013=CIRCLE('',#83433,14.84253123652);
#33014=CIRCLE('',#83435,15.28837739941);
#33015=CIRCLE('',#83436,15.59168796208);
#33016=CIRCLE('',#83438,14.33124152008);
#33017=CIRCLE('',#83439,14.65437591667);
#33018=CIRCLE('',#83441,15.35527542921);
#33019=CIRCLE('',#83442,15.65729010739);
#33020=CIRCLE('',#83444,14.52358370055);
#33021=CIRCLE('',#83445,14.84253123652);
#33022=CIRCLE('',#83447,15.40566400734);
#33023=CIRCLE('',#83448,15.70670982437);
#33024=CIRCLE('',#83450,14.33124152008);
#33025=CIRCLE('',#83451,14.65437591667);
#33026=CIRCLE('',#83453,15.43970477396);
#33027=CIRCLE('',#83454,15.7400995393);
#33028=CIRCLE('',#83456,14.52358370055);
#33029=CIRCLE('',#83457,14.84253123652);
#33030=CIRCLE('',#83459,15.45750573369);
#33031=CIRCLE('',#83460,15.75756115352);
#33032=CIRCLE('',#83462,14.33124152008);
#33033=CIRCLE('',#83463,14.65437591667);
#33034=CIRCLE('',#83465,15.43970477396);
#33035=CIRCLE('',#83466,15.7400995393);
#33036=CIRCLE('',#83468,13.93321511737);
#33037=CIRCLE('',#83469,14.26536832707);
#33038=CIRCLE('',#83471,15.45750573369);
#33039=CIRCLE('',#83472,15.75756115352);
#33040=CIRCLE('',#83474,14.16278516066);
#33041=CIRCLE('',#83475,14.48967679098);
#33042=CIRCLE('',#83477,15.35527542921);
#33043=CIRCLE('',#83478,15.65729010739);
#33044=CIRCLE('',#83480,13.93321511737);
#33045=CIRCLE('',#83481,14.26536832707);
#33046=CIRCLE('',#83483,15.40566400734);
#33047=CIRCLE('',#83484,15.70670982437);
#33048=CIRCLE('',#83486,14.16278516066);
#33049=CIRCLE('',#83487,14.48967679098);
#33050=CIRCLE('',#83489,15.20475200412);
#33051=CIRCLE('',#83490,15.50969804693);
#33052=CIRCLE('',#83492,13.93321511737);
#33053=CIRCLE('',#83493,14.26536832707);
#33054=CIRCLE('',#83495,15.28837739941);
#33055=CIRCLE('',#83496,15.59168796208);
#33056=CIRCLE('',#83498,14.16278516066);
#33057=CIRCLE('',#83499,14.48967679098);
#33058=CIRCLE('',#83501,14.98614304973);
#33059=CIRCLE('',#83502,15.29544813031);
#33060=CIRCLE('',#83504,13.93321511737);
#33061=CIRCLE('',#83505,14.26536832707);
#33062=CIRCLE('',#83507,15.10412140798);
#33063=CIRCLE('',#83508,15.41105880551);
#33064=CIRCLE('',#83510,14.16278516066);
#33065=CIRCLE('',#83511,14.48967679098);
#33066=CIRCLE('',#83513,14.6964105654);
#33067=CIRCLE('',#83514,15.01168656437);
#33068=CIRCLE('',#83516,13.93321511737);
#33069=CIRCLE('',#83517,14.26536832707);
#33070=CIRCLE('',#83519,14.8504034796);
#33071=CIRCLE('',#83520,15.16247781555);
#33072=CIRCLE('',#83522,14.16278516066);
#33073=CIRCLE('',#83523,14.48967679098);
#33074=CIRCLE('',#83525,14.6964105654);
#33075=CIRCLE('',#83526,15.01168656437);
#33076=CIRCLE('',#83528,14.37130764777);
#33077=CIRCLE('',#83529,14.69356095393);
#33078=CIRCLE('',#83531,14.8504034796);
#33079=CIRCLE('',#83532,15.16247781555);
#33080=CIRCLE('',#83534,14.55968693025);
#33081=CIRCLE('',#83535,14.87786051511);
#33082=CIRCLE('',#83537,14.6964105654);
#33083=CIRCLE('',#83538,15.01168656437);
#33084=CIRCLE('',#83540,14.72869592011);
#33085=CIRCLE('',#83541,15.0432953008);
#33086=CIRCLE('',#83543,14.8504034796);
#33087=CIRCLE('',#83544,15.16247781555);
#33088=CIRCLE('',#83546,14.87899470754);
#33089=CIRCLE('',#83547,15.19048167462);
#33090=CIRCLE('',#83549,14.6964105654);
#33091=CIRCLE('',#83550,15.01168656437);
#33092=CIRCLE('',#83552,15.01114530963);
#33093=CIRCLE('',#83553,15.31994561044);
#33094=CIRCLE('',#83555,14.8504034796);
#33095=CIRCLE('',#83556,15.16247781555);
#33096=CIRCLE('',#83558,15.12562340887);
#33097=CIRCLE('',#83559,15.4321331483);
#33098=CIRCLE('',#83561,14.6964105654);
#33099=CIRCLE('',#83562,15.01168656437);
#33100=CIRCLE('',#83564,15.22282771061);
#33101=CIRCLE('',#83565,15.52741876511);
#33102=CIRCLE('',#83567,14.8504034796);
#33103=CIRCLE('',#83568,15.16247781555);
#33104=CIRCLE('',#83570,15.3030873848);
#33105=CIRCLE('',#83571,15.60611205608);
#33106=CIRCLE('',#83573,14.6964105654);
#33107=CIRCLE('',#83574,15.01168656437);
#33108=CIRCLE('',#83576,15.36666793768);
#33109=CIRCLE('',#83577,15.66846302312);
#33110=CIRCLE('',#83579,14.8504034796);
#33111=CIRCLE('',#83580,15.16247781555);
#33112=CIRCLE('',#83582,15.41377577062);
#33113=CIRCLE('',#83583,15.71466619139);
#33114=CIRCLE('',#83585,14.6964105654);
#33115=CIRCLE('',#83586,15.01168656437);
#33116=CIRCLE('',#83588,15.44456161589);
#33117=CIRCLE('',#83589,15.74486371827);
#33118=CIRCLE('',#83591,14.8504034796);
#33119=CIRCLE('',#83592,15.16247781555);
#33120=CIRCLE('',#83594,15.45912298634);
#33121=CIRCLE('',#83595,15.75914761359);
#33122=CIRCLE('',#83597,14.6964105654);
#33123=CIRCLE('',#83598,15.01168656437);
#33124=CIRCLE('',#83600,15.45750573369);
#33125=CIRCLE('',#83601,15.75756115352);
#33126=CIRCLE('',#83603,14.8504034796);
#33127=CIRCLE('',#83604,15.16247781555);
#33128=CIRCLE('',#83606,15.43970477396);
#33129=CIRCLE('',#83607,15.7400995393);
#33130=CIRCLE('',#83609,14.6964105654);
#33131=CIRCLE('',#83610,15.01168656437);
#33132=CIRCLE('',#83612,15.40566400734);
#33133=CIRCLE('',#83613,15.70670982437);
#33134=CIRCLE('',#83615,14.8504034796);
#33135=CIRCLE('',#83616,15.16247781555);
#33136=CIRCLE('',#83618,15.35527542921);
#33137=CIRCLE('',#83619,15.65729010739);
#33138=CIRCLE('',#83621,14.6964105654);
#33139=CIRCLE('',#83622,15.01168656437);
#33140=CIRCLE('',#83624,15.28837739941);
#33141=CIRCLE('',#83625,15.59168796208);
#33142=CIRCLE('',#83627,14.8504034796);
#33143=CIRCLE('',#83628,15.16247781555);
#33144=CIRCLE('',#83630,15.20475200412);
#33145=CIRCLE('',#83631,15.50969804693);
#33146=CIRCLE('',#83633,14.6964105654);
#33147=CIRCLE('',#83634,15.01168656437);
#33148=CIRCLE('',#83636,15.10412140798);
#33149=CIRCLE('',#83637,15.41105880551);
#33150=CIRCLE('',#83639,14.8504034796);
#33151=CIRCLE('',#83640,15.16247781555);
#33152=CIRCLE('',#83642,14.98614304973);
#33153=CIRCLE('',#83643,15.29544813031);
#33154=CIRCLE('',#83645,14.6964105654);
#33155=CIRCLE('',#83646,15.01168656437);
#33156=CIRCLE('',#83648,14.8504034796);
#33157=CIRCLE('',#83649,15.16247781555);
#33158=CIRCLE('',#83651,14.8504034796);
#33159=CIRCLE('',#83652,15.16247781555);
#33160=CIRCLE('',#83654,14.6964105654);
#33161=CIRCLE('',#83655,15.01168656437);
#33162=CIRCLE('',#83657,14.98614304973);
#33163=CIRCLE('',#83658,15.29544813031);
#33164=CIRCLE('',#83660,14.8504034796);
#33165=CIRCLE('',#83661,15.16247781555);
#33166=CIRCLE('',#83663,15.10412140798);
#33167=CIRCLE('',#83664,15.41105880551);
#33168=CIRCLE('',#83666,14.6964105654);
#33169=CIRCLE('',#83667,15.01168656437);
#33170=CIRCLE('',#83669,15.20475200412);
#33171=CIRCLE('',#83670,15.50969804693);
#33172=CIRCLE('',#83672,14.8504034796);
#33173=CIRCLE('',#83673,15.16247781555);
#33174=CIRCLE('',#83675,15.28837739941);
#33175=CIRCLE('',#83676,15.59168796208);
#33176=CIRCLE('',#83678,14.6964105654);
#33177=CIRCLE('',#83679,15.01168656437);
#33178=CIRCLE('',#83681,15.35527542921);
#33179=CIRCLE('',#83682,15.65729010739);
#33180=CIRCLE('',#83684,14.8504034796);
#33181=CIRCLE('',#83685,15.16247781555);
#33182=CIRCLE('',#83687,15.40566400734);
#33183=CIRCLE('',#83688,15.70670982437);
#33184=CIRCLE('',#83690,14.6964105654);
#33185=CIRCLE('',#83691,15.01168656437);
#33186=CIRCLE('',#83693,15.43970477396);
#33187=CIRCLE('',#83694,15.7400995393);
#33188=CIRCLE('',#83696,14.8504034796);
#33189=CIRCLE('',#83697,15.16247781555);
#33190=CIRCLE('',#83699,15.45750573369);
#33191=CIRCLE('',#83700,15.75756115352);
#33192=CIRCLE('',#83702,14.6964105654);
#33193=CIRCLE('',#83703,15.01168656437);
#33194=CIRCLE('',#83705,15.43970477396);
#33195=CIRCLE('',#83706,15.7400995393);
#33196=CIRCLE('',#83708,14.37130764777);
#33197=CIRCLE('',#83709,14.69356095393);
#33198=CIRCLE('',#83711,15.45750573369);
#33199=CIRCLE('',#83712,15.75756115352);
#33200=CIRCLE('',#83714,14.55968693025);
#33201=CIRCLE('',#83715,14.87786051511);
#33202=CIRCLE('',#83717,15.35527542921);
#33203=CIRCLE('',#83718,15.65729010739);
#33204=CIRCLE('',#83720,14.37130764777);
#33205=CIRCLE('',#83721,14.69356095393);
#33206=CIRCLE('',#83723,15.40566400734);
#33207=CIRCLE('',#83724,15.70670982437);
#33208=CIRCLE('',#83726,14.55968693025);
#33209=CIRCLE('',#83727,14.87786051511);
#33210=CIRCLE('',#83729,15.20475200412);
#33211=CIRCLE('',#83730,15.50969804693);
#33212=CIRCLE('',#83732,14.37130764777);
#33213=CIRCLE('',#83733,14.69356095393);
#33214=CIRCLE('',#83735,15.28837739941);
#33215=CIRCLE('',#83736,15.59168796208);
#33216=CIRCLE('',#83738,14.55968693025);
#33217=CIRCLE('',#83739,14.87786051511);
#33218=CIRCLE('',#83741,14.98614304973);
#33219=CIRCLE('',#83742,15.29544813031);
#33220=CIRCLE('',#83744,14.37130764777);
#33221=CIRCLE('',#83745,14.69356095393);
#33222=CIRCLE('',#83747,15.10412140798);
#33223=CIRCLE('',#83748,15.41105880551);
#33224=CIRCLE('',#83750,14.55968693025);
#33225=CIRCLE('',#83751,14.87786051511);
#33226=CIRCLE('',#83753,14.98614304973);
#33227=CIRCLE('',#83754,15.29544813031);
#33228=CIRCLE('',#83756,14.72869592011);
#33229=CIRCLE('',#83757,15.0432953008);
#33230=CIRCLE('',#83759,15.10412140798);
#33231=CIRCLE('',#83760,15.41105880551);
#33232=CIRCLE('',#83762,14.87899470754);
#33233=CIRCLE('',#83763,15.19048167462);
#33234=CIRCLE('',#83765,14.98614304973);
#33235=CIRCLE('',#83766,15.29544813031);
#33236=CIRCLE('',#83768,15.01114530963);
#33237=CIRCLE('',#83769,15.31994561044);
#33238=CIRCLE('',#83771,15.10412140798);
#33239=CIRCLE('',#83772,15.41105880551);
#33240=CIRCLE('',#83774,15.12562340887);
#33241=CIRCLE('',#83775,15.4321331483);
#33242=CIRCLE('',#83777,14.98614304973);
#33243=CIRCLE('',#83778,15.29544813031);
#33244=CIRCLE('',#83780,15.22282771061);
#33245=CIRCLE('',#83781,15.52741876511);
#33246=CIRCLE('',#83783,15.10412140798);
#33247=CIRCLE('',#83784,15.41105880551);
#33248=CIRCLE('',#83786,15.3030873848);
#33249=CIRCLE('',#83787,15.60611205608);
#33250=CIRCLE('',#83789,14.98614304973);
#33251=CIRCLE('',#83790,15.29544813031);
#33252=CIRCLE('',#83792,15.36666793768);
#33253=CIRCLE('',#83793,15.66846302312);
#33254=CIRCLE('',#83795,15.10412140798);
#33255=CIRCLE('',#83796,15.41105880551);
#33256=CIRCLE('',#83798,15.41377577062);
#33257=CIRCLE('',#83799,15.71466619139);
#33258=CIRCLE('',#83801,14.98614304973);
#33259=CIRCLE('',#83802,15.29544813031);
#33260=CIRCLE('',#83804,15.44456161589);
#33261=CIRCLE('',#83805,15.74486371827);
#33262=CIRCLE('',#83807,15.10412140798);
#33263=CIRCLE('',#83808,15.41105880551);
#33264=CIRCLE('',#83810,15.45912298634);
#33265=CIRCLE('',#83811,15.75914761359);
#33266=CIRCLE('',#83813,14.98614304973);
#33267=CIRCLE('',#83814,15.29544813031);
#33268=CIRCLE('',#83816,15.45750573369);
#33269=CIRCLE('',#83817,15.75756115352);
#33270=CIRCLE('',#83819,15.10412140798);
#33271=CIRCLE('',#83820,15.41105880551);
#33272=CIRCLE('',#83822,15.43970477396);
#33273=CIRCLE('',#83823,15.7400995393);
#33274=CIRCLE('',#83825,14.98614304973);
#33275=CIRCLE('',#83826,15.29544813031);
#33276=CIRCLE('',#83828,15.40566400734);
#33277=CIRCLE('',#83829,15.70670982437);
#33278=CIRCLE('',#83831,15.10412140798);
#33279=CIRCLE('',#83832,15.41105880551);
#33280=CIRCLE('',#83834,15.35527542921);
#33281=CIRCLE('',#83835,15.65729010739);
#33282=CIRCLE('',#83837,14.98614304973);
#33283=CIRCLE('',#83838,15.29544813031);
#33284=CIRCLE('',#83840,15.28837739941);
#33285=CIRCLE('',#83841,15.59168796208);
#33286=CIRCLE('',#83843,15.10412140798);
#33287=CIRCLE('',#83844,15.41105880551);
#33288=CIRCLE('',#83846,15.20475200412);
#33289=CIRCLE('',#83847,15.50969804693);
#33290=CIRCLE('',#83849,14.98614304973);
#33291=CIRCLE('',#83850,15.29544813031);
#33292=CIRCLE('',#83852,15.10412140798);
#33293=CIRCLE('',#83853,15.41105880551);
#33294=CIRCLE('',#83855,15.10412140798);
#33295=CIRCLE('',#83856,15.41105880551);
#33296=CIRCLE('',#83858,14.98614304973);
#33297=CIRCLE('',#83859,15.29544813031);
#33298=CIRCLE('',#83861,15.20475200412);
#33299=CIRCLE('',#83862,15.50969804693);
#33300=CIRCLE('',#83864,15.10412140798);
#33301=CIRCLE('',#83865,15.41105880551);
#33302=CIRCLE('',#83867,15.28837739941);
#33303=CIRCLE('',#83868,15.59168796208);
#33304=CIRCLE('',#83870,14.98614304973);
#33305=CIRCLE('',#83871,15.29544813031);
#33306=CIRCLE('',#83873,15.35527542921);
#33307=CIRCLE('',#83874,15.65729010739);
#33308=CIRCLE('',#83876,15.10412140798);
#33309=CIRCLE('',#83877,15.41105880551);
#33310=CIRCLE('',#83879,15.40566400734);
#33311=CIRCLE('',#83880,15.70670982437);
#33312=CIRCLE('',#83882,14.98614304973);
#33313=CIRCLE('',#83883,15.29544813031);
#33314=CIRCLE('',#83885,15.10412140798);
#33315=CIRCLE('',#83886,15.41105880551);
#33316=CIRCLE('',#83888,15.45750573369);
#33317=CIRCLE('',#83889,15.75756115352);
#33318=CIRCLE('',#83891,14.98614304973);
#33319=CIRCLE('',#83892,15.29544813031);
#33320=CIRCLE('',#83894,15.43970477396);
#33321=CIRCLE('',#83895,15.7400995393);
#33322=CIRCLE('',#83897,15.43970477396);
#33323=CIRCLE('',#83898,15.7400995393);
#33324=CIRCLE('',#83900,14.72869592011);
#33325=CIRCLE('',#83901,15.0432953008);
#33326=CIRCLE('',#83903,15.45750573369);
#33327=CIRCLE('',#83904,15.75756115352);
#33328=CIRCLE('',#83906,14.87899470754);
#33329=CIRCLE('',#83907,15.19048167462);
#33330=CIRCLE('',#83909,15.35527542921);
#33331=CIRCLE('',#83910,15.65729010739);
#33332=CIRCLE('',#83912,14.72869592011);
#33333=CIRCLE('',#83913,15.0432953008);
#33334=CIRCLE('',#83915,15.40566400734);
#33335=CIRCLE('',#83916,15.70670982437);
#33336=CIRCLE('',#83918,14.87899470754);
#33337=CIRCLE('',#83919,15.19048167462);
#33338=CIRCLE('',#83921,15.20475200412);
#33339=CIRCLE('',#83922,15.50969804693);
#33340=CIRCLE('',#83924,14.72869592011);
#33341=CIRCLE('',#83925,15.0432953008);
#33342=CIRCLE('',#83927,15.28837739941);
#33343=CIRCLE('',#83928,15.59168796208);
#33344=CIRCLE('',#83930,14.87899470754);
#33345=CIRCLE('',#83931,15.19048167462);
#33346=CIRCLE('',#83933,15.20475200412);
#33347=CIRCLE('',#83934,15.50969804693);
#33348=CIRCLE('',#83936,15.01114530963);
#33349=CIRCLE('',#83937,15.31994561044);
#33350=CIRCLE('',#83939,15.28837739941);
#33351=CIRCLE('',#83940,15.59168796208);
#33352=CIRCLE('',#83942,15.12562340887);
#33353=CIRCLE('',#83943,15.4321331483);
#33354=CIRCLE('',#83945,15.20475200412);
#33355=CIRCLE('',#83946,15.50969804693);
#33356=CIRCLE('',#83948,15.22282771061);
#33357=CIRCLE('',#83949,15.52741876511);
#33358=CIRCLE('',#83951,15.28837739941);
#33359=CIRCLE('',#83952,15.59168796208);
#33360=CIRCLE('',#83954,15.3030873848);
#33361=CIRCLE('',#83955,15.60611205608);
#33362=CIRCLE('',#83957,15.20475200412);
#33363=CIRCLE('',#83958,15.50969804693);
#33364=CIRCLE('',#83960,15.36666793768);
#33365=CIRCLE('',#83961,15.66846302312);
#33366=CIRCLE('',#83963,15.28837739941);
#33367=CIRCLE('',#83964,15.59168796208);
#33368=CIRCLE('',#83966,15.41377577062);
#33369=CIRCLE('',#83967,15.71466619139);
#33370=CIRCLE('',#83969,15.20475200412);
#33371=CIRCLE('',#83970,15.50969804693);
#33372=CIRCLE('',#83972,15.44456161589);
#33373=CIRCLE('',#83973,15.74486371827);
#33374=CIRCLE('',#83975,15.28837739941);
#33375=CIRCLE('',#83976,15.59168796208);
#33376=CIRCLE('',#83978,15.45912298634);
#33377=CIRCLE('',#83979,15.75914761359);
#33378=CIRCLE('',#83981,15.20475200412);
#33379=CIRCLE('',#83982,15.50969804693);
#33380=CIRCLE('',#83984,15.45750573369);
#33381=CIRCLE('',#83985,15.75756115352);
#33382=CIRCLE('',#83987,15.28837739941);
#33383=CIRCLE('',#83988,15.59168796208);
#33384=CIRCLE('',#83990,15.43970477396);
#33385=CIRCLE('',#83991,15.7400995393);
#33386=CIRCLE('',#83993,15.20475200412);
#33387=CIRCLE('',#83994,15.50969804693);
#33388=CIRCLE('',#83996,15.40566400734);
#33389=CIRCLE('',#83997,15.70670982437);
#33390=CIRCLE('',#83999,15.28837739941);
#33391=CIRCLE('',#84000,15.59168796208);
#33392=CIRCLE('',#84002,15.35527542921);
#33393=CIRCLE('',#84003,15.65729010739);
#33394=CIRCLE('',#84005,15.20475200412);
#33395=CIRCLE('',#84006,15.50969804693);
#33396=CIRCLE('',#84008,15.28837739941);
#33397=CIRCLE('',#84009,15.59168796208);
#33398=CIRCLE('',#84011,15.28837739941);
#33399=CIRCLE('',#84012,15.59168796208);
#33400=CIRCLE('',#84014,15.20475200412);
#33401=CIRCLE('',#84015,15.50969804693);
#33402=CIRCLE('',#84017,15.35527542921);
#33403=CIRCLE('',#84018,15.65729010739);
#33404=CIRCLE('',#84020,15.28837739941);
#33405=CIRCLE('',#84021,15.59168796208);
#33406=CIRCLE('',#84023,15.40566400734);
#33407=CIRCLE('',#84024,15.70670982437);
#33408=CIRCLE('',#84026,15.20475200412);
#33409=CIRCLE('',#84027,15.50969804693);
#33410=CIRCLE('',#84029,15.43970477396);
#33411=CIRCLE('',#84030,15.7400995393);
#33412=CIRCLE('',#84032,15.28837739941);
#33413=CIRCLE('',#84033,15.59168796208);
#33414=CIRCLE('',#84035,15.45750573369);
#33415=CIRCLE('',#84036,15.75756115352);
#33416=CIRCLE('',#84038,15.20475200412);
#33417=CIRCLE('',#84039,15.50969804693);
#33418=CIRCLE('',#84041,15.43970477396);
#33419=CIRCLE('',#84042,15.7400995393);
#33420=CIRCLE('',#84044,15.01114530963);
#33421=CIRCLE('',#84045,15.31994561044);
#33422=CIRCLE('',#84047,15.45750573369);
#33423=CIRCLE('',#84048,15.75756115352);
#33424=CIRCLE('',#84050,15.12562340887);
#33425=CIRCLE('',#84051,15.4321331483);
#33426=CIRCLE('',#84053,15.35527542921);
#33427=CIRCLE('',#84054,15.65729010739);
#33428=CIRCLE('',#84056,15.01114530963);
#33429=CIRCLE('',#84057,15.31994561044);
#33430=CIRCLE('',#84059,15.40566400734);
#33431=CIRCLE('',#84060,15.70670982437);
#33432=CIRCLE('',#84062,15.12562340887);
#33433=CIRCLE('',#84063,15.4321331483);
#33434=CIRCLE('',#84065,15.35527542921);
#33435=CIRCLE('',#84066,15.65729010739);
#33436=CIRCLE('',#84068,15.22282771061);
#33437=CIRCLE('',#84069,15.52741876511);
#33438=CIRCLE('',#84071,15.40566400734);
#33439=CIRCLE('',#84072,15.70670982437);
#33440=CIRCLE('',#84074,15.3030873848);
#33441=CIRCLE('',#84075,15.60611205608);
#33442=CIRCLE('',#84077,15.35527542921);
#33443=CIRCLE('',#84078,15.65729010739);
#33444=CIRCLE('',#84080,15.36666793768);
#33445=CIRCLE('',#84081,15.66846302312);
#33446=CIRCLE('',#84083,15.40566400734);
#33447=CIRCLE('',#84084,15.70670982437);
#33448=CIRCLE('',#84086,15.41377577062);
#33449=CIRCLE('',#84087,15.71466619139);
#33450=CIRCLE('',#84089,15.35527542921);
#33451=CIRCLE('',#84090,15.65729010739);
#33452=CIRCLE('',#84092,15.44456161589);
#33453=CIRCLE('',#84093,15.74486371827);
#33454=CIRCLE('',#84095,15.40566400734);
#33455=CIRCLE('',#84096,15.70670982437);
#33456=CIRCLE('',#84098,15.45912298634);
#33457=CIRCLE('',#84099,15.75914761359);
#33458=CIRCLE('',#84101,15.35527542921);
#33459=CIRCLE('',#84102,15.65729010739);
#33460=CIRCLE('',#84104,15.45750573369);
#33461=CIRCLE('',#84105,15.75756115352);
#33462=CIRCLE('',#84107,15.40566400734);
#33463=CIRCLE('',#84108,15.70670982437);
#33464=CIRCLE('',#84110,15.43970477396);
#33465=CIRCLE('',#84111,15.7400995393);
#33466=CIRCLE('',#84113,15.35527542921);
#33467=CIRCLE('',#84114,15.65729010739);
#33468=CIRCLE('',#84116,15.40566400734);
#33469=CIRCLE('',#84117,15.70670982437);
#33470=CIRCLE('',#84119,15.40566400734);
#33471=CIRCLE('',#84120,15.70670982437);
#33472=CIRCLE('',#84122,15.35527542921);
#33473=CIRCLE('',#84123,15.65729010739);
#33474=CIRCLE('',#84125,15.43970477396);
#33475=CIRCLE('',#84126,15.7400995393);
#33476=CIRCLE('',#84128,15.40566400734);
#33477=CIRCLE('',#84129,15.70670982437);
#33478=CIRCLE('',#84131,15.45750573369);
#33479=CIRCLE('',#84132,15.75756115352);
#33480=CIRCLE('',#84134,15.35527542921);
#33481=CIRCLE('',#84135,15.65729010739);
#33482=CIRCLE('',#84137,15.43970477396);
#33483=CIRCLE('',#84138,15.7400995393);
#33484=CIRCLE('',#84140,15.22282771061);
#33485=CIRCLE('',#84141,15.52741876511);
#33486=CIRCLE('',#84143,15.45750573369);
#33487=CIRCLE('',#84144,15.75756115352);
#33488=CIRCLE('',#84146,15.3030873848);
#33489=CIRCLE('',#84147,15.60611205608);
#33490=CIRCLE('',#84149,15.43970477396);
#33491=CIRCLE('',#84150,15.7400995393);
#33492=CIRCLE('',#84152,15.36666793768);
#33493=CIRCLE('',#84153,15.66846302312);
#33494=CIRCLE('',#84155,15.45750573369);
#33495=CIRCLE('',#84156,15.75756115352);
#33496=CIRCLE('',#84158,15.41377577062);
#33497=CIRCLE('',#84159,15.71466619139);
#33498=CIRCLE('',#84161,15.43970477396);
#33499=CIRCLE('',#84162,15.7400995393);
#33500=CIRCLE('',#84164,15.44456161589);
#33501=CIRCLE('',#84165,15.74486371827);
#33502=CIRCLE('',#84167,15.45750573369);
#33503=CIRCLE('',#84168,15.75756115352);
#33504=CIRCLE('',#84170,15.45912298634);
#33505=CIRCLE('',#84171,15.75914761359);
#33506=CIRCLE('',#84173,15.43970477396);
#33507=CIRCLE('',#84174,15.7400995393);
#33508=CIRCLE('',#84176,15.45750573369);
#33509=CIRCLE('',#84177,15.75756115352);
#33510=CIRCLE('',#84179,15.45750573369);
#33511=CIRCLE('',#84180,15.75756115352);
#33512=CIRCLE('',#84182,15.43970477396);
#33513=CIRCLE('',#84183,15.7400995393);
#33514=CIRCLE('',#85950,9.152185531336);
#33515=CIRCLE('',#85952,15.45912298634);
#33516=CIRCLE('',#85953,15.44456161589);
#33517=CIRCLE('',#85954,15.44456161589);
#33518=CIRCLE('',#85955,15.45912298634);
#33519=CIRCLE('',#85957,15.75914761359);
#33520=CIRCLE('',#85959,15.74486371827);
#33521=CIRCLE('',#85961,15.74486371827);
#33522=CIRCLE('',#85963,15.75914761359);
#33523=CIRCLE('',#85965,9.25);
#35028=VERTEX_POINT('',#183809);
#35029=VERTEX_POINT('',#183810);
#35030=VERTEX_POINT('',#183812);
#35031=VERTEX_POINT('',#183823);
#35032=VERTEX_POINT('',#183824);
#35033=VERTEX_POINT('',#183908);
#35034=VERTEX_POINT('',#183965);
#35035=VERTEX_POINT('',#183966);
#35036=VERTEX_POINT('',#184163);
#35037=VERTEX_POINT('',#184164);
#35038=VERTEX_POINT('',#184166);
#35039=VERTEX_POINT('',#184349);
#35040=VERTEX_POINT('',#184350);
#35041=VERTEX_POINT('',#184352);
#35042=VERTEX_POINT('',#184357);
#35043=VERTEX_POINT('',#184361);
#35044=VERTEX_POINT('',#184365);
#35045=VERTEX_POINT('',#184366);
#35046=VERTEX_POINT('',#184385);
#35047=VERTEX_POINT('',#184387);
#35048=VERTEX_POINT('',#184408);
#35049=VERTEX_POINT('',#184409);
#35050=VERTEX_POINT('',#184428);
#35051=VERTEX_POINT('',#184430);
#35052=VERTEX_POINT('',#184451);
#35053=VERTEX_POINT('',#184453);
#35054=VERTEX_POINT('',#184455);
#35055=VERTEX_POINT('',#184475);
#35056=VERTEX_POINT('',#184477);
#35057=VERTEX_POINT('',#184482);
#35058=VERTEX_POINT('',#184483);
#35059=VERTEX_POINT('',#184485);
#35060=VERTEX_POINT('',#184504);
#35061=VERTEX_POINT('',#184525);
#35062=VERTEX_POINT('',#184526);
#35063=VERTEX_POINT('',#184528);
#35064=VERTEX_POINT('',#184547);
#35065=VERTEX_POINT('',#184568);
#35066=VERTEX_POINT('',#184570);
#35067=VERTEX_POINT('',#184592);
#35068=VERTEX_POINT('',#184593);
#35069=VERTEX_POINT('',#184615);
#35070=VERTEX_POINT('',#184617);
#35071=VERTEX_POINT('',#184638);
#35072=VERTEX_POINT('',#184640);
#35073=VERTEX_POINT('',#184642);
#35074=VERTEX_POINT('',#184644);
#35075=VERTEX_POINT('',#184664);
#35076=VERTEX_POINT('',#184666);
#35077=VERTEX_POINT('',#184671);
#35078=VERTEX_POINT('',#184673);
#35079=VERTEX_POINT('',#184694);
#35080=VERTEX_POINT('',#184696);
#35081=VERTEX_POINT('',#184717);
#35082=VERTEX_POINT('',#184719);
#35083=VERTEX_POINT('',#184741);
#35084=VERTEX_POINT('',#184745);
#35085=VERTEX_POINT('',#184747);
#35086=VERTEX_POINT('',#184751);
#35087=VERTEX_POINT('',#184753);
#35088=VERTEX_POINT('',#184757);
#35089=VERTEX_POINT('',#184761);
#35090=VERTEX_POINT('',#184763);
#35091=VERTEX_POINT('',#184767);
#35092=VERTEX_POINT('',#184771);
#35093=VERTEX_POINT('',#184773);
#35094=VERTEX_POINT('',#184777);
#35095=VERTEX_POINT('',#184779);
#35096=VERTEX_POINT('',#184783);
#35097=VERTEX_POINT('',#184785);
#35098=VERTEX_POINT('',#184789);
#35099=VERTEX_POINT('',#184790);
#35100=VERTEX_POINT('',#184792);
#35101=VERTEX_POINT('',#184794);
#35102=VERTEX_POINT('',#184796);
#35103=VERTEX_POINT('',#184798);
#35104=VERTEX_POINT('',#184800);
#35105=VERTEX_POINT('',#184802);
#35106=VERTEX_POINT('',#184804);
#35107=VERTEX_POINT('',#184807);
#35108=VERTEX_POINT('',#184811);
#35109=VERTEX_POINT('',#184868);
#35110=VERTEX_POINT('',#184870);
#35111=VERTEX_POINT('',#184909);
#35112=VERTEX_POINT('',#184911);
#35113=VERTEX_POINT('',#185054);
#35114=VERTEX_POINT('',#185055);
#35115=VERTEX_POINT('',#185480);
#35116=VERTEX_POINT('',#185495);
#35117=VERTEX_POINT('',#185589);
#35118=VERTEX_POINT('',#185591);
#35119=VERTEX_POINT('',#185668);
#35120=VERTEX_POINT('',#185793);
#35121=VERTEX_POINT('',#186008);
#35122=VERTEX_POINT('',#186429);
#35123=VERTEX_POINT('',#186586);
#35124=VERTEX_POINT('',#186591);
#35125=VERTEX_POINT('',#186597);
#35126=VERTEX_POINT('',#186603);
#35127=VERTEX_POINT('',#186615);
#35128=VERTEX_POINT('',#187063);
#35129=VERTEX_POINT('',#187078);
#35130=VERTEX_POINT('',#187079);
#35131=VERTEX_POINT('',#187081);
#35132=VERTEX_POINT('',#187083);
#35133=VERTEX_POINT('',#187087);
#35134=VERTEX_POINT('',#187089);
#35135=VERTEX_POINT('',#187091);
#35136=VERTEX_POINT('',#187095);
#35137=VERTEX_POINT('',#187097);
#35138=VERTEX_POINT('',#187102);
#35139=VERTEX_POINT('',#187108);
#35140=VERTEX_POINT('',#187109);
#35141=VERTEX_POINT('',#187111);
#35142=VERTEX_POINT('',#187113);
#35143=VERTEX_POINT('',#187117);
#35144=VERTEX_POINT('',#187118);
#35145=VERTEX_POINT('',#187120);
#35146=VERTEX_POINT('',#187125);
#35147=VERTEX_POINT('',#187127);
#35148=VERTEX_POINT('',#187132);
#35149=VERTEX_POINT('',#187138);
#35150=VERTEX_POINT('',#187139);
#35151=VERTEX_POINT('',#187141);
#35152=VERTEX_POINT('',#187143);
#35153=VERTEX_POINT('',#187147);
#35154=VERTEX_POINT('',#187148);
#35155=VERTEX_POINT('',#187153);
#35156=VERTEX_POINT('',#187154);
#35157=VERTEX_POINT('',#187159);
#35158=VERTEX_POINT('',#187166);
#35159=VERTEX_POINT('',#187167);
#35160=VERTEX_POINT('',#187169);
#35161=VERTEX_POINT('',#187171);
#35162=VERTEX_POINT('',#187175);
#35163=VERTEX_POINT('',#187176);
#35164=VERTEX_POINT('',#187181);
#35165=VERTEX_POINT('',#187182);
#35166=VERTEX_POINT('',#187190);
#35167=VERTEX_POINT('',#187191);
#35168=VERTEX_POINT('',#187193);
#35169=VERTEX_POINT('',#187195);
#35170=VERTEX_POINT('',#187199);
#35171=VERTEX_POINT('',#187200);
#35172=VERTEX_POINT('',#187205);
#35173=VERTEX_POINT('',#187206);
#35174=VERTEX_POINT('',#187214);
#35175=VERTEX_POINT('',#187215);
#35176=VERTEX_POINT('',#187217);
#35177=VERTEX_POINT('',#187219);
#35178=VERTEX_POINT('',#187223);
#35179=VERTEX_POINT('',#187224);
#35180=VERTEX_POINT('',#187229);
#35181=VERTEX_POINT('',#187230);
#35182=VERTEX_POINT('',#187238);
#35183=VERTEX_POINT('',#187239);
#35184=VERTEX_POINT('',#187241);
#35185=VERTEX_POINT('',#187243);
#35186=VERTEX_POINT('',#187247);
#35187=VERTEX_POINT('',#187248);
#35188=VERTEX_POINT('',#187253);
#35189=VERTEX_POINT('',#187254);
#35190=VERTEX_POINT('',#187262);
#35191=VERTEX_POINT('',#187263);
#35192=VERTEX_POINT('',#187265);
#35193=VERTEX_POINT('',#187267);
#35194=VERTEX_POINT('',#187271);
#35195=VERTEX_POINT('',#187272);
#35196=VERTEX_POINT('',#187274);
#35197=VERTEX_POINT('',#187279);
#35198=VERTEX_POINT('',#187281);
#35199=VERTEX_POINT('',#187286);
#35200=VERTEX_POINT('',#187292);
#35201=VERTEX_POINT('',#187293);
#35202=VERTEX_POINT('',#187295);
#35203=VERTEX_POINT('',#187297);
#35204=VERTEX_POINT('',#187301);
#35205=VERTEX_POINT('',#187302);
#35206=VERTEX_POINT('',#187304);
#35207=VERTEX_POINT('',#187309);
#35208=VERTEX_POINT('',#187310);
#35209=VERTEX_POINT('',#187315);
#35210=VERTEX_POINT('',#187322);
#35211=VERTEX_POINT('',#187323);
#35212=VERTEX_POINT('',#187325);
#35213=VERTEX_POINT('',#187327);
#35214=VERTEX_POINT('',#187331);
#35215=VERTEX_POINT('',#187332);
#35216=VERTEX_POINT('',#187334);
#35217=VERTEX_POINT('',#187339);
#35218=VERTEX_POINT('',#187340);
#35219=VERTEX_POINT('',#187345);
#35220=VERTEX_POINT('',#187352);
#35221=VERTEX_POINT('',#187353);
#35222=VERTEX_POINT('',#187355);
#35223=VERTEX_POINT('',#187357);
#35224=VERTEX_POINT('',#187361);
#35225=VERTEX_POINT('',#187362);
#35226=VERTEX_POINT('',#187367);
#35227=VERTEX_POINT('',#187368);
#35228=VERTEX_POINT('',#187370);
#35229=VERTEX_POINT('',#187375);
#35230=VERTEX_POINT('',#187382);
#35231=VERTEX_POINT('',#187383);
#35232=VERTEX_POINT('',#187385);
#35233=VERTEX_POINT('',#187387);
#35234=VERTEX_POINT('',#187391);
#35235=VERTEX_POINT('',#187392);
#35236=VERTEX_POINT('',#187397);
#35237=VERTEX_POINT('',#187398);
#35238=VERTEX_POINT('',#187406);
#35239=VERTEX_POINT('',#187407);
#35240=VERTEX_POINT('',#187409);
#35241=VERTEX_POINT('',#187411);
#35242=VERTEX_POINT('',#187415);
#35243=VERTEX_POINT('',#187416);
#35244=VERTEX_POINT('',#187418);
#35245=VERTEX_POINT('',#187423);
#35246=VERTEX_POINT('',#187424);
#35247=VERTEX_POINT('',#187429);
#35248=VERTEX_POINT('',#187436);
#35249=VERTEX_POINT('',#187437);
#35250=VERTEX_POINT('',#187439);
#35251=VERTEX_POINT('',#187441);
#35252=VERTEX_POINT('',#187445);
#35253=VERTEX_POINT('',#187446);
#35254=VERTEX_POINT('',#187448);
#35255=VERTEX_POINT('',#187453);
#35256=VERTEX_POINT('',#187454);
#35257=VERTEX_POINT('',#187459);
#35258=VERTEX_POINT('',#187466);
#35259=VERTEX_POINT('',#187467);
#35260=VERTEX_POINT('',#187469);
#35261=VERTEX_POINT('',#187471);
#35262=VERTEX_POINT('',#187475);
#35263=VERTEX_POINT('',#187476);
#35264=VERTEX_POINT('',#187478);
#35265=VERTEX_POINT('',#187483);
#35266=VERTEX_POINT('',#187484);
#35267=VERTEX_POINT('',#187489);
#35268=VERTEX_POINT('',#187496);
#35269=VERTEX_POINT('',#187497);
#35270=VERTEX_POINT('',#187499);
#35271=VERTEX_POINT('',#187501);
#35272=VERTEX_POINT('',#187505);
#35273=VERTEX_POINT('',#187506);
#35274=VERTEX_POINT('',#187508);
#35275=VERTEX_POINT('',#187513);
#35276=VERTEX_POINT('',#187514);
#35277=VERTEX_POINT('',#187519);
#35278=VERTEX_POINT('',#187526);
#35279=VERTEX_POINT('',#187527);
#35280=VERTEX_POINT('',#187529);
#35281=VERTEX_POINT('',#187531);
#35282=VERTEX_POINT('',#187535);
#35283=VERTEX_POINT('',#187536);
#35284=VERTEX_POINT('',#187541);
#35285=VERTEX_POINT('',#187542);
#35286=VERTEX_POINT('',#187550);
#35287=VERTEX_POINT('',#187551);
#35288=VERTEX_POINT('',#187553);
#35289=VERTEX_POINT('',#187555);
#35290=VERTEX_POINT('',#187559);
#35291=VERTEX_POINT('',#187560);
#35292=VERTEX_POINT('',#187565);
#35293=VERTEX_POINT('',#187566);
#35294=VERTEX_POINT('',#187574);
#35295=VERTEX_POINT('',#187575);
#35296=VERTEX_POINT('',#187577);
#35297=VERTEX_POINT('',#187579);
#35298=VERTEX_POINT('',#187583);
#35299=VERTEX_POINT('',#187584);
#35300=VERTEX_POINT('',#187589);
#35301=VERTEX_POINT('',#187590);
#35302=VERTEX_POINT('',#187598);
#35303=VERTEX_POINT('',#187599);
#35304=VERTEX_POINT('',#187601);
#35305=VERTEX_POINT('',#187603);
#35306=VERTEX_POINT('',#187607);
#35307=VERTEX_POINT('',#187608);
#35308=VERTEX_POINT('',#187613);
#35309=VERTEX_POINT('',#187614);
#35310=VERTEX_POINT('',#187622);
#35311=VERTEX_POINT('',#187623);
#35312=VERTEX_POINT('',#187625);
#35313=VERTEX_POINT('',#187627);
#35314=VERTEX_POINT('',#187631);
#35315=VERTEX_POINT('',#187632);
#35316=VERTEX_POINT('',#187637);
#35317=VERTEX_POINT('',#187638);
#35318=VERTEX_POINT('',#187646);
#35319=VERTEX_POINT('',#187647);
#35320=VERTEX_POINT('',#187649);
#35321=VERTEX_POINT('',#187651);
#35322=VERTEX_POINT('',#187655);
#35323=VERTEX_POINT('',#187656);
#35324=VERTEX_POINT('',#187661);
#35325=VERTEX_POINT('',#187662);
#35326=VERTEX_POINT('',#187670);
#35327=VERTEX_POINT('',#187671);
#35328=VERTEX_POINT('',#187673);
#35329=VERTEX_POINT('',#187675);
#35330=VERTEX_POINT('',#187679);
#35331=VERTEX_POINT('',#187681);
#35332=VERTEX_POINT('',#187685);
#35333=VERTEX_POINT('',#187686);
#35334=VERTEX_POINT('',#187689);
#35335=VERTEX_POINT('',#187694);
#35336=VERTEX_POINT('',#187700);
#35337=VERTEX_POINT('',#187701);
#35338=VERTEX_POINT('',#187703);
#35339=VERTEX_POINT('',#187705);
#35340=VERTEX_POINT('',#187709);
#35341=VERTEX_POINT('',#187710);
#35342=VERTEX_POINT('',#187712);
#35343=VERTEX_POINT('',#187717);
#35344=VERTEX_POINT('',#187718);
#35345=VERTEX_POINT('',#187723);
#35346=VERTEX_POINT('',#187730);
#35347=VERTEX_POINT('',#187731);
#35348=VERTEX_POINT('',#187733);
#35349=VERTEX_POINT('',#187735);
#35350=VERTEX_POINT('',#187739);
#35351=VERTEX_POINT('',#187740);
#35352=VERTEX_POINT('',#187745);
#35353=VERTEX_POINT('',#187746);
#35354=VERTEX_POINT('',#187754);
#35355=VERTEX_POINT('',#187755);
#35356=VERTEX_POINT('',#187757);
#35357=VERTEX_POINT('',#187759);
#35358=VERTEX_POINT('',#187763);
#35359=VERTEX_POINT('',#187764);
#35360=VERTEX_POINT('',#187769);
#35361=VERTEX_POINT('',#187770);
#35362=VERTEX_POINT('',#187778);
#35363=VERTEX_POINT('',#187779);
#35364=VERTEX_POINT('',#187781);
#35365=VERTEX_POINT('',#187783);
#35366=VERTEX_POINT('',#187787);
#35367=VERTEX_POINT('',#187788);
#35368=VERTEX_POINT('',#187793);
#35369=VERTEX_POINT('',#187794);
#35370=VERTEX_POINT('',#187802);
#35371=VERTEX_POINT('',#187803);
#35372=VERTEX_POINT('',#187805);
#35373=VERTEX_POINT('',#187807);
#35374=VERTEX_POINT('',#187811);
#35375=VERTEX_POINT('',#187812);
#35376=VERTEX_POINT('',#187817);
#35377=VERTEX_POINT('',#187818);
#35378=VERTEX_POINT('',#187826);
#35379=VERTEX_POINT('',#187827);
#35380=VERTEX_POINT('',#187829);
#35381=VERTEX_POINT('',#187831);
#35382=VERTEX_POINT('',#187835);
#35383=VERTEX_POINT('',#187836);
#35384=VERTEX_POINT('',#187841);
#35385=VERTEX_POINT('',#187842);
#35386=VERTEX_POINT('',#187850);
#35387=VERTEX_POINT('',#187851);
#35388=VERTEX_POINT('',#187853);
#35389=VERTEX_POINT('',#187855);
#35390=VERTEX_POINT('',#187859);
#35391=VERTEX_POINT('',#187860);
#35392=VERTEX_POINT('',#187865);
#35393=VERTEX_POINT('',#187866);
#35394=VERTEX_POINT('',#187874);
#35395=VERTEX_POINT('',#187875);
#35396=VERTEX_POINT('',#187877);
#35397=VERTEX_POINT('',#187879);
#35398=VERTEX_POINT('',#187883);
#35399=VERTEX_POINT('',#187884);
#35400=VERTEX_POINT('',#187889);
#35401=VERTEX_POINT('',#187890);
#35402=VERTEX_POINT('',#187898);
#35403=VERTEX_POINT('',#187899);
#35404=VERTEX_POINT('',#187901);
#35405=VERTEX_POINT('',#187903);
#35406=VERTEX_POINT('',#187907);
#35407=VERTEX_POINT('',#187908);
#35408=VERTEX_POINT('',#187913);
#35409=VERTEX_POINT('',#187914);
#35410=VERTEX_POINT('',#187922);
#35411=VERTEX_POINT('',#187923);
#35412=VERTEX_POINT('',#187925);
#35413=VERTEX_POINT('',#187927);
#35414=VERTEX_POINT('',#187931);
#35415=VERTEX_POINT('',#187932);
#35416=VERTEX_POINT('',#187934);
#35417=VERTEX_POINT('',#187939);
#35418=VERTEX_POINT('',#187940);
#35419=VERTEX_POINT('',#187945);
#35420=VERTEX_POINT('',#187952);
#35421=VERTEX_POINT('',#187953);
#35422=VERTEX_POINT('',#187955);
#35423=VERTEX_POINT('',#187957);
#35424=VERTEX_POINT('',#187961);
#35425=VERTEX_POINT('',#187962);
#35426=VERTEX_POINT('',#187964);
#35427=VERTEX_POINT('',#187969);
#35428=VERTEX_POINT('',#187970);
#35429=VERTEX_POINT('',#187975);
#35430=VERTEX_POINT('',#187982);
#35431=VERTEX_POINT('',#187983);
#35432=VERTEX_POINT('',#187985);
#35433=VERTEX_POINT('',#187987);
#35434=VERTEX_POINT('',#187991);
#35435=VERTEX_POINT('',#187992);
#35436=VERTEX_POINT('',#187997);
#35437=VERTEX_POINT('',#187998);
#35438=VERTEX_POINT('',#188006);
#35439=VERTEX_POINT('',#188007);
#35440=VERTEX_POINT('',#188009);
#35441=VERTEX_POINT('',#188011);
#35442=VERTEX_POINT('',#188015);
#35443=VERTEX_POINT('',#188016);
#35444=VERTEX_POINT('',#188021);
#35445=VERTEX_POINT('',#188022);
#35446=VERTEX_POINT('',#188030);
#35447=VERTEX_POINT('',#188031);
#35448=VERTEX_POINT('',#188033);
#35449=VERTEX_POINT('',#188035);
#35450=VERTEX_POINT('',#188039);
#35451=VERTEX_POINT('',#188040);
#35452=VERTEX_POINT('',#188045);
#35453=VERTEX_POINT('',#188046);
#35454=VERTEX_POINT('',#188054);
#35455=VERTEX_POINT('',#188055);
#35456=VERTEX_POINT('',#188057);
#35457=VERTEX_POINT('',#188059);
#35458=VERTEX_POINT('',#188063);
#35459=VERTEX_POINT('',#188064);
#35460=VERTEX_POINT('',#188069);
#35461=VERTEX_POINT('',#188070);
#35462=VERTEX_POINT('',#188078);
#35463=VERTEX_POINT('',#188079);
#35464=VERTEX_POINT('',#188081);
#35465=VERTEX_POINT('',#188083);
#35466=VERTEX_POINT('',#188087);
#35467=VERTEX_POINT('',#188088);
#35468=VERTEX_POINT('',#188093);
#35469=VERTEX_POINT('',#188094);
#35470=VERTEX_POINT('',#188102);
#35471=VERTEX_POINT('',#188103);
#35472=VERTEX_POINT('',#188105);
#35473=VERTEX_POINT('',#188107);
#35474=VERTEX_POINT('',#188111);
#35475=VERTEX_POINT('',#188112);
#35476=VERTEX_POINT('',#188117);
#35477=VERTEX_POINT('',#188118);
#35478=VERTEX_POINT('',#188126);
#35479=VERTEX_POINT('',#188127);
#35480=VERTEX_POINT('',#188129);
#35481=VERTEX_POINT('',#188131);
#35482=VERTEX_POINT('',#188135);
#35483=VERTEX_POINT('',#188136);
#35484=VERTEX_POINT('',#188141);
#35485=VERTEX_POINT('',#188142);
#35486=VERTEX_POINT('',#188150);
#35487=VERTEX_POINT('',#188151);
#35488=VERTEX_POINT('',#188153);
#35489=VERTEX_POINT('',#188155);
#35490=VERTEX_POINT('',#188159);
#35491=VERTEX_POINT('',#188160);
#35492=VERTEX_POINT('',#188165);
#35493=VERTEX_POINT('',#188166);
#35494=VERTEX_POINT('',#188174);
#35495=VERTEX_POINT('',#188175);
#35496=VERTEX_POINT('',#188177);
#35497=VERTEX_POINT('',#188179);
#35498=VERTEX_POINT('',#188183);
#35499=VERTEX_POINT('',#188184);
#35500=VERTEX_POINT('',#188189);
#35501=VERTEX_POINT('',#188190);
#35502=VERTEX_POINT('',#188198);
#35503=VERTEX_POINT('',#188199);
#35504=VERTEX_POINT('',#188201);
#35505=VERTEX_POINT('',#188203);
#35506=VERTEX_POINT('',#188207);
#35507=VERTEX_POINT('',#188208);
#35508=VERTEX_POINT('',#188213);
#35509=VERTEX_POINT('',#188214);
#35510=VERTEX_POINT('',#188222);
#35511=VERTEX_POINT('',#188223);
#35512=VERTEX_POINT('',#188225);
#35513=VERTEX_POINT('',#188229);
#35514=VERTEX_POINT('',#188230);
#35515=VERTEX_POINT('',#188232);
#35516=VERTEX_POINT('',#188234);
#35517=VERTEX_POINT('',#188238);
#35518=VERTEX_POINT('',#188239);
#35519=VERTEX_POINT('',#188244);
#35520=VERTEX_POINT('',#188252);
#35521=VERTEX_POINT('',#188253);
#35522=VERTEX_POINT('',#188255);
#35523=VERTEX_POINT('',#188257);
#35524=VERTEX_POINT('',#188261);
#35525=VERTEX_POINT('',#188262);
#35526=VERTEX_POINT('',#188267);
#35527=VERTEX_POINT('',#188268);
#35528=VERTEX_POINT('',#188276);
#35529=VERTEX_POINT('',#188277);
#35530=VERTEX_POINT('',#188279);
#35531=VERTEX_POINT('',#188281);
#35532=VERTEX_POINT('',#188285);
#35533=VERTEX_POINT('',#188286);
#35534=VERTEX_POINT('',#188291);
#35535=VERTEX_POINT('',#188292);
#35536=VERTEX_POINT('',#188300);
#35537=VERTEX_POINT('',#188301);
#35538=VERTEX_POINT('',#188303);
#35539=VERTEX_POINT('',#188305);
#35540=VERTEX_POINT('',#188309);
#35541=VERTEX_POINT('',#188310);
#35542=VERTEX_POINT('',#188315);
#35543=VERTEX_POINT('',#188316);
#35544=VERTEX_POINT('',#188324);
#35545=VERTEX_POINT('',#188325);
#35546=VERTEX_POINT('',#188327);
#35547=VERTEX_POINT('',#188329);
#35548=VERTEX_POINT('',#188333);
#35549=VERTEX_POINT('',#188334);
#35550=VERTEX_POINT('',#188339);
#35551=VERTEX_POINT('',#188340);
#35552=VERTEX_POINT('',#188348);
#35553=VERTEX_POINT('',#188349);
#35554=VERTEX_POINT('',#188351);
#35555=VERTEX_POINT('',#188353);
#35556=VERTEX_POINT('',#188357);
#35557=VERTEX_POINT('',#188358);
#35558=VERTEX_POINT('',#188363);
#35559=VERTEX_POINT('',#188364);
#35560=VERTEX_POINT('',#188372);
#35561=VERTEX_POINT('',#188373);
#35562=VERTEX_POINT('',#188375);
#35563=VERTEX_POINT('',#188377);
#35564=VERTEX_POINT('',#188381);
#35565=VERTEX_POINT('',#188382);
#35566=VERTEX_POINT('',#188387);
#35567=VERTEX_POINT('',#188388);
#35568=VERTEX_POINT('',#188396);
#35569=VERTEX_POINT('',#188397);
#35570=VERTEX_POINT('',#188399);
#35571=VERTEX_POINT('',#188401);
#35572=VERTEX_POINT('',#188405);
#35573=VERTEX_POINT('',#188406);
#35574=VERTEX_POINT('',#188411);
#35575=VERTEX_POINT('',#188412);
#35576=VERTEX_POINT('',#188420);
#35577=VERTEX_POINT('',#188421);
#35578=VERTEX_POINT('',#188423);
#35579=VERTEX_POINT('',#188425);
#35580=VERTEX_POINT('',#188429);
#35581=VERTEX_POINT('',#188430);
#35582=VERTEX_POINT('',#188435);
#35583=VERTEX_POINT('',#188436);
#35584=VERTEX_POINT('',#188444);
#35585=VERTEX_POINT('',#188445);
#35586=VERTEX_POINT('',#188447);
#35587=VERTEX_POINT('',#188449);
#35588=VERTEX_POINT('',#188453);
#35589=VERTEX_POINT('',#188454);
#35590=VERTEX_POINT('',#188459);
#35591=VERTEX_POINT('',#188460);
#35592=VERTEX_POINT('',#188468);
#35593=VERTEX_POINT('',#188469);
#35594=VERTEX_POINT('',#188471);
#35595=VERTEX_POINT('',#188473);
#35596=VERTEX_POINT('',#188477);
#35597=VERTEX_POINT('',#188478);
#35598=VERTEX_POINT('',#188483);
#35599=VERTEX_POINT('',#188484);
#35600=VERTEX_POINT('',#188492);
#35601=VERTEX_POINT('',#188493);
#35602=VERTEX_POINT('',#188495);
#35603=VERTEX_POINT('',#188497);
#35604=VERTEX_POINT('',#188501);
#35605=VERTEX_POINT('',#188502);
#35606=VERTEX_POINT('',#188507);
#35607=VERTEX_POINT('',#188508);
#35608=VERTEX_POINT('',#188510);
#35609=VERTEX_POINT('',#188515);
#35610=VERTEX_POINT('',#188522);
#35611=VERTEX_POINT('',#188523);
#35612=VERTEX_POINT('',#188525);
#35613=VERTEX_POINT('',#188527);
#35614=VERTEX_POINT('',#188531);
#35615=VERTEX_POINT('',#188532);
#35616=VERTEX_POINT('',#188537);
#35617=VERTEX_POINT('',#188538);
#35618=VERTEX_POINT('',#188540);
#35619=VERTEX_POINT('',#188545);
#35620=VERTEX_POINT('',#188552);
#35621=VERTEX_POINT('',#188553);
#35622=VERTEX_POINT('',#188555);
#35623=VERTEX_POINT('',#188557);
#35624=VERTEX_POINT('',#188561);
#35625=VERTEX_POINT('',#188562);
#35626=VERTEX_POINT('',#188567);
#35627=VERTEX_POINT('',#188568);
#35628=VERTEX_POINT('',#188576);
#35629=VERTEX_POINT('',#188577);
#35630=VERTEX_POINT('',#188579);
#35631=VERTEX_POINT('',#188581);
#35632=VERTEX_POINT('',#188585);
#35633=VERTEX_POINT('',#188586);
#35634=VERTEX_POINT('',#188591);
#35635=VERTEX_POINT('',#188592);
#35636=VERTEX_POINT('',#188600);
#35637=VERTEX_POINT('',#188601);
#35638=VERTEX_POINT('',#188603);
#35639=VERTEX_POINT('',#188605);
#35640=VERTEX_POINT('',#188609);
#35641=VERTEX_POINT('',#188610);
#35642=VERTEX_POINT('',#188615);
#35643=VERTEX_POINT('',#188616);
#35644=VERTEX_POINT('',#188624);
#35645=VERTEX_POINT('',#188625);
#35646=VERTEX_POINT('',#188627);
#35647=VERTEX_POINT('',#188629);
#35648=VERTEX_POINT('',#188633);
#35649=VERTEX_POINT('',#188634);
#35650=VERTEX_POINT('',#188639);
#35651=VERTEX_POINT('',#188640);
#35652=VERTEX_POINT('',#188648);
#35653=VERTEX_POINT('',#188649);
#35654=VERTEX_POINT('',#188651);
#35655=VERTEX_POINT('',#188653);
#35656=VERTEX_POINT('',#188657);
#35657=VERTEX_POINT('',#188658);
#35658=VERTEX_POINT('',#188663);
#35659=VERTEX_POINT('',#188664);
#35660=VERTEX_POINT('',#188672);
#35661=VERTEX_POINT('',#188673);
#35662=VERTEX_POINT('',#188675);
#35663=VERTEX_POINT('',#188677);
#35664=VERTEX_POINT('',#188681);
#35665=VERTEX_POINT('',#188682);
#35666=VERTEX_POINT('',#188687);
#35667=VERTEX_POINT('',#188688);
#35668=VERTEX_POINT('',#188696);
#35669=VERTEX_POINT('',#188697);
#35670=VERTEX_POINT('',#188699);
#35671=VERTEX_POINT('',#188701);
#35672=VERTEX_POINT('',#188705);
#35673=VERTEX_POINT('',#188706);
#35674=VERTEX_POINT('',#188711);
#35675=VERTEX_POINT('',#188712);
#35676=VERTEX_POINT('',#188720);
#35677=VERTEX_POINT('',#188721);
#35678=VERTEX_POINT('',#188723);
#35679=VERTEX_POINT('',#188725);
#35680=VERTEX_POINT('',#188729);
#35681=VERTEX_POINT('',#188730);
#35682=VERTEX_POINT('',#188735);
#35683=VERTEX_POINT('',#188736);
#35684=VERTEX_POINT('',#188744);
#35685=VERTEX_POINT('',#188745);
#35686=VERTEX_POINT('',#188747);
#35687=VERTEX_POINT('',#188749);
#35688=VERTEX_POINT('',#188753);
#35689=VERTEX_POINT('',#188754);
#35690=VERTEX_POINT('',#188759);
#35691=VERTEX_POINT('',#188760);
#35692=VERTEX_POINT('',#188768);
#35693=VERTEX_POINT('',#188769);
#35694=VERTEX_POINT('',#188771);
#35695=VERTEX_POINT('',#188773);
#35696=VERTEX_POINT('',#188777);
#35697=VERTEX_POINT('',#188778);
#35698=VERTEX_POINT('',#188783);
#35699=VERTEX_POINT('',#188784);
#35700=VERTEX_POINT('',#188792);
#35701=VERTEX_POINT('',#188793);
#35702=VERTEX_POINT('',#188795);
#35703=VERTEX_POINT('',#188797);
#35704=VERTEX_POINT('',#188801);
#35705=VERTEX_POINT('',#188802);
#35706=VERTEX_POINT('',#188807);
#35707=VERTEX_POINT('',#188808);
#35708=VERTEX_POINT('',#188816);
#35709=VERTEX_POINT('',#188817);
#35710=VERTEX_POINT('',#188819);
#35711=VERTEX_POINT('',#188821);
#35712=VERTEX_POINT('',#188825);
#35713=VERTEX_POINT('',#188826);
#35714=VERTEX_POINT('',#188831);
#35715=VERTEX_POINT('',#188832);
#35716=VERTEX_POINT('',#188840);
#35717=VERTEX_POINT('',#188841);
#35718=VERTEX_POINT('',#188843);
#35719=VERTEX_POINT('',#188845);
#35720=VERTEX_POINT('',#188849);
#35721=VERTEX_POINT('',#188850);
#35722=VERTEX_POINT('',#188855);
#35723=VERTEX_POINT('',#188856);
#35724=VERTEX_POINT('',#188864);
#35725=VERTEX_POINT('',#188865);
#35726=VERTEX_POINT('',#188867);
#35727=VERTEX_POINT('',#188869);
#35728=VERTEX_POINT('',#188873);
#35729=VERTEX_POINT('',#188874);
#35730=VERTEX_POINT('',#188879);
#35731=VERTEX_POINT('',#188880);
#35732=VERTEX_POINT('',#188888);
#35733=VERTEX_POINT('',#188889);
#35734=VERTEX_POINT('',#188891);
#35735=VERTEX_POINT('',#188893);
#35736=VERTEX_POINT('',#188897);
#35737=VERTEX_POINT('',#188898);
#35738=VERTEX_POINT('',#188903);
#35739=VERTEX_POINT('',#188904);
#35740=VERTEX_POINT('',#188912);
#35741=VERTEX_POINT('',#188913);
#35742=VERTEX_POINT('',#188915);
#35743=VERTEX_POINT('',#188917);
#35744=VERTEX_POINT('',#188921);
#35745=VERTEX_POINT('',#188922);
#35746=VERTEX_POINT('',#188927);
#35747=VERTEX_POINT('',#188928);
#35748=VERTEX_POINT('',#188936);
#35749=VERTEX_POINT('',#188937);
#35750=VERTEX_POINT('',#188939);
#35751=VERTEX_POINT('',#188941);
#35752=VERTEX_POINT('',#188945);
#35753=VERTEX_POINT('',#188946);
#35754=VERTEX_POINT('',#188951);
#35755=VERTEX_POINT('',#188952);
#35756=VERTEX_POINT('',#188960);
#35757=VERTEX_POINT('',#188961);
#35758=VERTEX_POINT('',#188963);
#35759=VERTEX_POINT('',#188965);
#35760=VERTEX_POINT('',#188969);
#35761=VERTEX_POINT('',#188970);
#35762=VERTEX_POINT('',#188975);
#35763=VERTEX_POINT('',#188976);
#35764=VERTEX_POINT('',#188984);
#35765=VERTEX_POINT('',#188985);
#35766=VERTEX_POINT('',#188987);
#35767=VERTEX_POINT('',#188989);
#35768=VERTEX_POINT('',#188993);
#35769=VERTEX_POINT('',#188994);
#35770=VERTEX_POINT('',#188999);
#35771=VERTEX_POINT('',#189000);
#35772=VERTEX_POINT('',#189008);
#35773=VERTEX_POINT('',#189009);
#35774=VERTEX_POINT('',#189011);
#35775=VERTEX_POINT('',#189013);
#35776=VERTEX_POINT('',#189017);
#35777=VERTEX_POINT('',#189018);
#35778=VERTEX_POINT('',#189023);
#35779=VERTEX_POINT('',#189024);
#35780=VERTEX_POINT('',#189032);
#35781=VERTEX_POINT('',#189033);
#35782=VERTEX_POINT('',#189035);
#35783=VERTEX_POINT('',#189037);
#35784=VERTEX_POINT('',#189041);
#35785=VERTEX_POINT('',#189042);
#35786=VERTEX_POINT('',#189047);
#35787=VERTEX_POINT('',#189048);
#35788=VERTEX_POINT('',#189056);
#35789=VERTEX_POINT('',#189057);
#35790=VERTEX_POINT('',#189059);
#35791=VERTEX_POINT('',#189061);
#35792=VERTEX_POINT('',#189065);
#35793=VERTEX_POINT('',#189066);
#35794=VERTEX_POINT('',#189071);
#35795=VERTEX_POINT('',#189072);
#35796=VERTEX_POINT('',#189080);
#35797=VERTEX_POINT('',#189081);
#35798=VERTEX_POINT('',#189083);
#35799=VERTEX_POINT('',#189085);
#35800=VERTEX_POINT('',#189089);
#35801=VERTEX_POINT('',#189090);
#35802=VERTEX_POINT('',#189095);
#35803=VERTEX_POINT('',#189096);
#35804=VERTEX_POINT('',#189104);
#35805=VERTEX_POINT('',#189105);
#35806=VERTEX_POINT('',#189107);
#35807=VERTEX_POINT('',#189109);
#35808=VERTEX_POINT('',#189113);
#35809=VERTEX_POINT('',#189114);
#35810=VERTEX_POINT('',#189119);
#35811=VERTEX_POINT('',#189120);
#35812=VERTEX_POINT('',#189128);
#35813=VERTEX_POINT('',#189129);
#35814=VERTEX_POINT('',#189131);
#35815=VERTEX_POINT('',#189133);
#35816=VERTEX_POINT('',#189137);
#35817=VERTEX_POINT('',#189138);
#35818=VERTEX_POINT('',#189143);
#35819=VERTEX_POINT('',#189144);
#35820=VERTEX_POINT('',#189152);
#35821=VERTEX_POINT('',#189153);
#35822=VERTEX_POINT('',#189155);
#35823=VERTEX_POINT('',#189157);
#35824=VERTEX_POINT('',#189161);
#35825=VERTEX_POINT('',#189162);
#35826=VERTEX_POINT('',#189167);
#35827=VERTEX_POINT('',#189168);
#35828=VERTEX_POINT('',#189176);
#35829=VERTEX_POINT('',#189177);
#35830=VERTEX_POINT('',#189179);
#35831=VERTEX_POINT('',#189181);
#35832=VERTEX_POINT('',#189185);
#35833=VERTEX_POINT('',#189186);
#35834=VERTEX_POINT('',#189191);
#35835=VERTEX_POINT('',#189192);
#35836=VERTEX_POINT('',#189200);
#35837=VERTEX_POINT('',#189201);
#35838=VERTEX_POINT('',#189203);
#35839=VERTEX_POINT('',#189205);
#35840=VERTEX_POINT('',#189209);
#35841=VERTEX_POINT('',#189210);
#35842=VERTEX_POINT('',#189215);
#35843=VERTEX_POINT('',#189216);
#35844=VERTEX_POINT('',#189224);
#35845=VERTEX_POINT('',#189225);
#35846=VERTEX_POINT('',#189227);
#35847=VERTEX_POINT('',#189229);
#35848=VERTEX_POINT('',#189233);
#35849=VERTEX_POINT('',#189234);
#35850=VERTEX_POINT('',#189239);
#35851=VERTEX_POINT('',#189240);
#35852=VERTEX_POINT('',#189248);
#35853=VERTEX_POINT('',#189249);
#35854=VERTEX_POINT('',#189251);
#35855=VERTEX_POINT('',#189253);
#35856=VERTEX_POINT('',#189257);
#35857=VERTEX_POINT('',#189258);
#35858=VERTEX_POINT('',#189263);
#35859=VERTEX_POINT('',#189264);
#35860=VERTEX_POINT('',#189272);
#35861=VERTEX_POINT('',#189273);
#35862=VERTEX_POINT('',#189275);
#35863=VERTEX_POINT('',#189277);
#35864=VERTEX_POINT('',#189281);
#35865=VERTEX_POINT('',#189282);
#35866=VERTEX_POINT('',#189287);
#35867=VERTEX_POINT('',#189288);
#35868=VERTEX_POINT('',#189296);
#35869=VERTEX_POINT('',#189297);
#35870=VERTEX_POINT('',#189299);
#35871=VERTEX_POINT('',#189301);
#35872=VERTEX_POINT('',#189305);
#35873=VERTEX_POINT('',#189306);
#35874=VERTEX_POINT('',#189311);
#35875=VERTEX_POINT('',#189312);
#35876=VERTEX_POINT('',#189320);
#35877=VERTEX_POINT('',#189321);
#35878=VERTEX_POINT('',#189323);
#35879=VERTEX_POINT('',#189325);
#35880=VERTEX_POINT('',#189329);
#35881=VERTEX_POINT('',#189330);
#35882=VERTEX_POINT('',#189335);
#35883=VERTEX_POINT('',#189336);
#35884=VERTEX_POINT('',#189344);
#35885=VERTEX_POINT('',#189345);
#35886=VERTEX_POINT('',#189347);
#35887=VERTEX_POINT('',#189349);
#35888=VERTEX_POINT('',#189353);
#35889=VERTEX_POINT('',#189354);
#35890=VERTEX_POINT('',#189359);
#35891=VERTEX_POINT('',#189360);
#35892=VERTEX_POINT('',#189368);
#35893=VERTEX_POINT('',#189369);
#35894=VERTEX_POINT('',#189371);
#35895=VERTEX_POINT('',#189373);
#35896=VERTEX_POINT('',#189377);
#35897=VERTEX_POINT('',#189378);
#35898=VERTEX_POINT('',#189383);
#35899=VERTEX_POINT('',#189384);
#35900=VERTEX_POINT('',#189392);
#35901=VERTEX_POINT('',#189393);
#35902=VERTEX_POINT('',#189395);
#35903=VERTEX_POINT('',#189397);
#35904=VERTEX_POINT('',#189401);
#35905=VERTEX_POINT('',#189402);
#35906=VERTEX_POINT('',#189407);
#35907=VERTEX_POINT('',#189408);
#35908=VERTEX_POINT('',#189416);
#35909=VERTEX_POINT('',#189417);
#35910=VERTEX_POINT('',#189419);
#35911=VERTEX_POINT('',#189421);
#35912=VERTEX_POINT('',#189425);
#35913=VERTEX_POINT('',#189426);
#35914=VERTEX_POINT('',#189431);
#35915=VERTEX_POINT('',#189432);
#35916=VERTEX_POINT('',#189440);
#35917=VERTEX_POINT('',#189441);
#35918=VERTEX_POINT('',#189443);
#35919=VERTEX_POINT('',#189445);
#35920=VERTEX_POINT('',#189449);
#35921=VERTEX_POINT('',#189450);
#35922=VERTEX_POINT('',#189455);
#35923=VERTEX_POINT('',#189456);
#35924=VERTEX_POINT('',#189464);
#35925=VERTEX_POINT('',#189465);
#35926=VERTEX_POINT('',#189467);
#35927=VERTEX_POINT('',#189469);
#35928=VERTEX_POINT('',#189473);
#35929=VERTEX_POINT('',#189474);
#35930=VERTEX_POINT('',#189479);
#35931=VERTEX_POINT('',#189480);
#35932=VERTEX_POINT('',#189488);
#35933=VERTEX_POINT('',#189489);
#35934=VERTEX_POINT('',#189491);
#35935=VERTEX_POINT('',#189493);
#35936=VERTEX_POINT('',#189497);
#35937=VERTEX_POINT('',#189498);
#35938=VERTEX_POINT('',#189503);
#35939=VERTEX_POINT('',#189504);
#35940=VERTEX_POINT('',#189512);
#35941=VERTEX_POINT('',#189513);
#35942=VERTEX_POINT('',#189515);
#35943=VERTEX_POINT('',#189517);
#35944=VERTEX_POINT('',#189521);
#35945=VERTEX_POINT('',#189522);
#35946=VERTEX_POINT('',#189527);
#35947=VERTEX_POINT('',#189528);
#35948=VERTEX_POINT('',#189536);
#35949=VERTEX_POINT('',#189537);
#35950=VERTEX_POINT('',#189539);
#35951=VERTEX_POINT('',#189541);
#35952=VERTEX_POINT('',#189545);
#35953=VERTEX_POINT('',#189546);
#35954=VERTEX_POINT('',#189551);
#35955=VERTEX_POINT('',#189552);
#35956=VERTEX_POINT('',#189560);
#35957=VERTEX_POINT('',#189561);
#35958=VERTEX_POINT('',#189563);
#35959=VERTEX_POINT('',#189565);
#35960=VERTEX_POINT('',#189569);
#35961=VERTEX_POINT('',#189570);
#35962=VERTEX_POINT('',#189575);
#35963=VERTEX_POINT('',#189576);
#35964=VERTEX_POINT('',#189584);
#35965=VERTEX_POINT('',#189585);
#35966=VERTEX_POINT('',#189587);
#35967=VERTEX_POINT('',#189589);
#35968=VERTEX_POINT('',#189593);
#35969=VERTEX_POINT('',#189594);
#35970=VERTEX_POINT('',#189599);
#35971=VERTEX_POINT('',#189600);
#35972=VERTEX_POINT('',#189608);
#35973=VERTEX_POINT('',#189609);
#35974=VERTEX_POINT('',#189611);
#35975=VERTEX_POINT('',#189613);
#35976=VERTEX_POINT('',#189617);
#35977=VERTEX_POINT('',#189618);
#35978=VERTEX_POINT('',#189623);
#35979=VERTEX_POINT('',#189624);
#35980=VERTEX_POINT('',#189632);
#35981=VERTEX_POINT('',#189633);
#35982=VERTEX_POINT('',#189635);
#35983=VERTEX_POINT('',#189637);
#35984=VERTEX_POINT('',#189641);
#35985=VERTEX_POINT('',#189642);
#35986=VERTEX_POINT('',#189647);
#35987=VERTEX_POINT('',#189648);
#35988=VERTEX_POINT('',#189656);
#35989=VERTEX_POINT('',#189657);
#35990=VERTEX_POINT('',#189659);
#35991=VERTEX_POINT('',#189661);
#35992=VERTEX_POINT('',#189665);
#35993=VERTEX_POINT('',#189666);
#35994=VERTEX_POINT('',#189671);
#35995=VERTEX_POINT('',#189672);
#35996=VERTEX_POINT('',#189680);
#35997=VERTEX_POINT('',#189681);
#35998=VERTEX_POINT('',#189683);
#35999=VERTEX_POINT('',#189685);
#36000=VERTEX_POINT('',#189689);
#36001=VERTEX_POINT('',#189690);
#36002=VERTEX_POINT('',#189695);
#36003=VERTEX_POINT('',#189696);
#36004=VERTEX_POINT('',#189704);
#36005=VERTEX_POINT('',#189705);
#36006=VERTEX_POINT('',#189707);
#36007=VERTEX_POINT('',#189709);
#36008=VERTEX_POINT('',#189713);
#36009=VERTEX_POINT('',#189714);
#36010=VERTEX_POINT('',#189719);
#36011=VERTEX_POINT('',#189720);
#36012=VERTEX_POINT('',#189728);
#36013=VERTEX_POINT('',#189729);
#36014=VERTEX_POINT('',#189731);
#36015=VERTEX_POINT('',#189733);
#36016=VERTEX_POINT('',#189737);
#36017=VERTEX_POINT('',#189738);
#36018=VERTEX_POINT('',#189743);
#36019=VERTEX_POINT('',#189744);
#36020=VERTEX_POINT('',#189752);
#36021=VERTEX_POINT('',#189753);
#36022=VERTEX_POINT('',#189755);
#36023=VERTEX_POINT('',#189757);
#36024=VERTEX_POINT('',#189761);
#36025=VERTEX_POINT('',#189762);
#36026=VERTEX_POINT('',#189767);
#36027=VERTEX_POINT('',#189768);
#36028=VERTEX_POINT('',#189776);
#36029=VERTEX_POINT('',#189777);
#36030=VERTEX_POINT('',#189779);
#36031=VERTEX_POINT('',#189781);
#36032=VERTEX_POINT('',#189785);
#36033=VERTEX_POINT('',#189786);
#36034=VERTEX_POINT('',#189791);
#36035=VERTEX_POINT('',#189792);
#36036=VERTEX_POINT('',#189800);
#36037=VERTEX_POINT('',#189801);
#36038=VERTEX_POINT('',#189803);
#36039=VERTEX_POINT('',#189805);
#36040=VERTEX_POINT('',#189809);
#36041=VERTEX_POINT('',#189810);
#36042=VERTEX_POINT('',#189815);
#36043=VERTEX_POINT('',#189816);
#36044=VERTEX_POINT('',#189824);
#36045=VERTEX_POINT('',#189825);
#36046=VERTEX_POINT('',#189827);
#36047=VERTEX_POINT('',#189829);
#36048=VERTEX_POINT('',#189833);
#36049=VERTEX_POINT('',#189834);
#36050=VERTEX_POINT('',#189839);
#36051=VERTEX_POINT('',#189840);
#36052=VERTEX_POINT('',#189848);
#36053=VERTEX_POINT('',#189849);
#36054=VERTEX_POINT('',#189851);
#36055=VERTEX_POINT('',#189853);
#36056=VERTEX_POINT('',#189857);
#36057=VERTEX_POINT('',#189858);
#36058=VERTEX_POINT('',#189863);
#36059=VERTEX_POINT('',#189864);
#36060=VERTEX_POINT('',#189872);
#36061=VERTEX_POINT('',#189873);
#36062=VERTEX_POINT('',#189875);
#36063=VERTEX_POINT('',#189877);
#36064=VERTEX_POINT('',#189881);
#36065=VERTEX_POINT('',#189882);
#36066=VERTEX_POINT('',#189887);
#36067=VERTEX_POINT('',#189888);
#36068=VERTEX_POINT('',#189896);
#36069=VERTEX_POINT('',#189897);
#36070=VERTEX_POINT('',#189899);
#36071=VERTEX_POINT('',#189901);
#36072=VERTEX_POINT('',#189905);
#36073=VERTEX_POINT('',#189906);
#36074=VERTEX_POINT('',#189911);
#36075=VERTEX_POINT('',#189912);
#36076=VERTEX_POINT('',#189920);
#36077=VERTEX_POINT('',#189921);
#36078=VERTEX_POINT('',#189923);
#36079=VERTEX_POINT('',#189925);
#36080=VERTEX_POINT('',#189929);
#36081=VERTEX_POINT('',#189930);
#36082=VERTEX_POINT('',#189935);
#36083=VERTEX_POINT('',#189936);
#36084=VERTEX_POINT('',#189944);
#36085=VERTEX_POINT('',#189945);
#36086=VERTEX_POINT('',#189947);
#36087=VERTEX_POINT('',#189949);
#36088=VERTEX_POINT('',#189953);
#36089=VERTEX_POINT('',#189954);
#36090=VERTEX_POINT('',#189959);
#36091=VERTEX_POINT('',#189960);
#36092=VERTEX_POINT('',#189968);
#36093=VERTEX_POINT('',#189969);
#36094=VERTEX_POINT('',#189971);
#36095=VERTEX_POINT('',#189973);
#36096=VERTEX_POINT('',#189977);
#36097=VERTEX_POINT('',#189978);
#36098=VERTEX_POINT('',#189983);
#36099=VERTEX_POINT('',#189984);
#36100=VERTEX_POINT('',#189992);
#36101=VERTEX_POINT('',#189993);
#36102=VERTEX_POINT('',#189995);
#36103=VERTEX_POINT('',#189997);
#36104=VERTEX_POINT('',#190001);
#36105=VERTEX_POINT('',#190002);
#36106=VERTEX_POINT('',#190007);
#36107=VERTEX_POINT('',#190008);
#36108=VERTEX_POINT('',#190016);
#36109=VERTEX_POINT('',#190017);
#36110=VERTEX_POINT('',#190019);
#36111=VERTEX_POINT('',#190021);
#36112=VERTEX_POINT('',#190025);
#36113=VERTEX_POINT('',#190026);
#36114=VERTEX_POINT('',#190031);
#36115=VERTEX_POINT('',#190032);
#36116=VERTEX_POINT('',#190040);
#36117=VERTEX_POINT('',#190041);
#36118=VERTEX_POINT('',#190043);
#36119=VERTEX_POINT('',#190045);
#36120=VERTEX_POINT('',#190049);
#36121=VERTEX_POINT('',#190050);
#36122=VERTEX_POINT('',#190055);
#36123=VERTEX_POINT('',#190056);
#36124=VERTEX_POINT('',#190064);
#36125=VERTEX_POINT('',#190065);
#36126=VERTEX_POINT('',#190067);
#36127=VERTEX_POINT('',#190069);
#36128=VERTEX_POINT('',#190073);
#36129=VERTEX_POINT('',#190074);
#36130=VERTEX_POINT('',#190079);
#36131=VERTEX_POINT('',#190080);
#36132=VERTEX_POINT('',#190088);
#36133=VERTEX_POINT('',#190089);
#36134=VERTEX_POINT('',#190091);
#36135=VERTEX_POINT('',#190093);
#36136=VERTEX_POINT('',#190097);
#36137=VERTEX_POINT('',#190098);
#36138=VERTEX_POINT('',#190103);
#36139=VERTEX_POINT('',#190104);
#36140=VERTEX_POINT('',#190112);
#36141=VERTEX_POINT('',#190113);
#36142=VERTEX_POINT('',#190115);
#36143=VERTEX_POINT('',#190117);
#36144=VERTEX_POINT('',#190121);
#36145=VERTEX_POINT('',#190122);
#36146=VERTEX_POINT('',#190127);
#36147=VERTEX_POINT('',#190128);
#36148=VERTEX_POINT('',#190136);
#36149=VERTEX_POINT('',#190137);
#36150=VERTEX_POINT('',#190139);
#36151=VERTEX_POINT('',#190141);
#36152=VERTEX_POINT('',#190145);
#36153=VERTEX_POINT('',#190146);
#36154=VERTEX_POINT('',#190151);
#36155=VERTEX_POINT('',#190152);
#36156=VERTEX_POINT('',#190160);
#36157=VERTEX_POINT('',#190161);
#36158=VERTEX_POINT('',#190163);
#36159=VERTEX_POINT('',#190165);
#36160=VERTEX_POINT('',#190169);
#36161=VERTEX_POINT('',#190170);
#36162=VERTEX_POINT('',#190175);
#36163=VERTEX_POINT('',#190176);
#36164=VERTEX_POINT('',#190184);
#36165=VERTEX_POINT('',#190185);
#36166=VERTEX_POINT('',#190187);
#36167=VERTEX_POINT('',#190189);
#36168=VERTEX_POINT('',#190193);
#36169=VERTEX_POINT('',#190194);
#36170=VERTEX_POINT('',#190199);
#36171=VERTEX_POINT('',#190200);
#36172=VERTEX_POINT('',#190208);
#36173=VERTEX_POINT('',#190209);
#36174=VERTEX_POINT('',#190211);
#36175=VERTEX_POINT('',#190213);
#36176=VERTEX_POINT('',#190217);
#36177=VERTEX_POINT('',#190218);
#36178=VERTEX_POINT('',#190223);
#36179=VERTEX_POINT('',#190224);
#36180=VERTEX_POINT('',#190232);
#36181=VERTEX_POINT('',#190233);
#36182=VERTEX_POINT('',#190235);
#36183=VERTEX_POINT('',#190237);
#36184=VERTEX_POINT('',#190241);
#36185=VERTEX_POINT('',#190242);
#36186=VERTEX_POINT('',#190244);
#36187=VERTEX_POINT('',#190249);
#36188=VERTEX_POINT('',#190250);
#36189=VERTEX_POINT('',#190260);
#36190=VERTEX_POINT('',#190261);
#36191=VERTEX_POINT('',#190263);
#36192=VERTEX_POINT('',#190265);
#36193=VERTEX_POINT('',#190269);
#36194=VERTEX_POINT('',#190270);
#36195=VERTEX_POINT('',#190272);
#36196=VERTEX_POINT('',#190277);
#36197=VERTEX_POINT('',#190278);
#36198=VERTEX_POINT('',#190283);
#36199=VERTEX_POINT('',#190290);
#36200=VERTEX_POINT('',#190291);
#36201=VERTEX_POINT('',#190293);
#36202=VERTEX_POINT('',#190295);
#36203=VERTEX_POINT('',#190299);
#36204=VERTEX_POINT('',#190300);
#36205=VERTEX_POINT('',#190302);
#36206=VERTEX_POINT('',#190307);
#36207=VERTEX_POINT('',#190308);
#36208=VERTEX_POINT('',#190313);
#36209=VERTEX_POINT('',#190320);
#36210=VERTEX_POINT('',#190321);
#36211=VERTEX_POINT('',#190323);
#36212=VERTEX_POINT('',#190325);
#36213=VERTEX_POINT('',#190329);
#36214=VERTEX_POINT('',#190330);
#36215=VERTEX_POINT('',#190332);
#36216=VERTEX_POINT('',#190337);
#36217=VERTEX_POINT('',#190338);
#36218=VERTEX_POINT('',#190343);
#36219=VERTEX_POINT('',#190350);
#36220=VERTEX_POINT('',#190351);
#36221=VERTEX_POINT('',#190353);
#36222=VERTEX_POINT('',#190355);
#36223=VERTEX_POINT('',#190359);
#36224=VERTEX_POINT('',#190360);
#36225=VERTEX_POINT('',#190362);
#36226=VERTEX_POINT('',#190367);
#36227=VERTEX_POINT('',#190368);
#36228=VERTEX_POINT('',#190373);
#36229=VERTEX_POINT('',#190380);
#36230=VERTEX_POINT('',#190381);
#36231=VERTEX_POINT('',#190383);
#36232=VERTEX_POINT('',#190385);
#36233=VERTEX_POINT('',#190387);
#36234=VERTEX_POINT('',#190391);
#36235=VERTEX_POINT('',#190392);
#36236=VERTEX_POINT('',#190397);
#36237=VERTEX_POINT('',#190398);
#36238=VERTEX_POINT('',#190403);
#36239=VERTEX_POINT('',#190410);
#36240=VERTEX_POINT('',#190411);
#36241=VERTEX_POINT('',#190413);
#36242=VERTEX_POINT('',#190415);
#36243=VERTEX_POINT('',#190417);
#36244=VERTEX_POINT('',#190421);
#36245=VERTEX_POINT('',#190422);
#36246=VERTEX_POINT('',#190427);
#36247=VERTEX_POINT('',#190428);
#36248=VERTEX_POINT('',#190433);
#36249=VERTEX_POINT('',#190440);
#36250=VERTEX_POINT('',#190441);
#36251=VERTEX_POINT('',#190443);
#36252=VERTEX_POINT('',#190445);
#36253=VERTEX_POINT('',#190449);
#36254=VERTEX_POINT('',#190450);
#36255=VERTEX_POINT('',#190452);
#36256=VERTEX_POINT('',#190457);
#36257=VERTEX_POINT('',#190458);
#36258=VERTEX_POINT('',#190463);
#36259=VERTEX_POINT('',#190470);
#36260=VERTEX_POINT('',#190471);
#36261=VERTEX_POINT('',#190473);
#36262=VERTEX_POINT('',#190475);
#36263=VERTEX_POINT('',#190479);
#36264=VERTEX_POINT('',#190480);
#36265=VERTEX_POINT('',#190482);
#36266=VERTEX_POINT('',#190487);
#36267=VERTEX_POINT('',#190488);
#36268=VERTEX_POINT('',#190493);
#36269=VERTEX_POINT('',#190500);
#36270=VERTEX_POINT('',#190501);
#36271=VERTEX_POINT('',#190503);
#36272=VERTEX_POINT('',#190505);
#36273=VERTEX_POINT('',#190509);
#36274=VERTEX_POINT('',#190510);
#36275=VERTEX_POINT('',#190512);
#36276=VERTEX_POINT('',#190517);
#36277=VERTEX_POINT('',#190518);
#36278=VERTEX_POINT('',#190523);
#36279=VERTEX_POINT('',#190530);
#36280=VERTEX_POINT('',#190531);
#36281=VERTEX_POINT('',#190533);
#36282=VERTEX_POINT('',#190535);
#36283=VERTEX_POINT('',#190539);
#36284=VERTEX_POINT('',#190540);
#36285=VERTEX_POINT('',#190545);
#36286=VERTEX_POINT('',#190546);
#36287=VERTEX_POINT('',#190554);
#36288=VERTEX_POINT('',#190555);
#36289=VERTEX_POINT('',#190557);
#36290=VERTEX_POINT('',#190559);
#36291=VERTEX_POINT('',#190563);
#36292=VERTEX_POINT('',#190564);
#36293=VERTEX_POINT('',#190569);
#36294=VERTEX_POINT('',#190570);
#36295=VERTEX_POINT('',#190578);
#36296=VERTEX_POINT('',#190579);
#36297=VERTEX_POINT('',#190581);
#36298=VERTEX_POINT('',#190583);
#36299=VERTEX_POINT('',#190587);
#36300=VERTEX_POINT('',#190588);
#36301=VERTEX_POINT('',#190593);
#36302=VERTEX_POINT('',#190594);
#36303=VERTEX_POINT('',#190602);
#36304=VERTEX_POINT('',#190603);
#36305=VERTEX_POINT('',#190605);
#36306=VERTEX_POINT('',#190607);
#36307=VERTEX_POINT('',#190611);
#36308=VERTEX_POINT('',#190612);
#36309=VERTEX_POINT('',#190617);
#36310=VERTEX_POINT('',#190618);
#36311=VERTEX_POINT('',#190626);
#36312=VERTEX_POINT('',#190627);
#36313=VERTEX_POINT('',#190629);
#36314=VERTEX_POINT('',#190631);
#36315=VERTEX_POINT('',#190635);
#36316=VERTEX_POINT('',#190636);
#36317=VERTEX_POINT('',#190641);
#36318=VERTEX_POINT('',#190642);
#36319=VERTEX_POINT('',#190650);
#36320=VERTEX_POINT('',#190651);
#36321=VERTEX_POINT('',#190653);
#36322=VERTEX_POINT('',#190655);
#36323=VERTEX_POINT('',#190659);
#36324=VERTEX_POINT('',#190660);
#36325=VERTEX_POINT('',#190665);
#36326=VERTEX_POINT('',#190666);
#36327=VERTEX_POINT('',#190674);
#36328=VERTEX_POINT('',#190675);
#36329=VERTEX_POINT('',#190677);
#36330=VERTEX_POINT('',#190679);
#36331=VERTEX_POINT('',#190683);
#36332=VERTEX_POINT('',#190684);
#36333=VERTEX_POINT('',#190689);
#36334=VERTEX_POINT('',#190690);
#36335=VERTEX_POINT('',#190698);
#36336=VERTEX_POINT('',#190699);
#36337=VERTEX_POINT('',#190701);
#36338=VERTEX_POINT('',#190703);
#36339=VERTEX_POINT('',#190707);
#36340=VERTEX_POINT('',#190708);
#36341=VERTEX_POINT('',#190713);
#36342=VERTEX_POINT('',#190714);
#36343=VERTEX_POINT('',#190722);
#36344=VERTEX_POINT('',#190723);
#36345=VERTEX_POINT('',#190725);
#36346=VERTEX_POINT('',#190727);
#36347=VERTEX_POINT('',#190729);
#36348=VERTEX_POINT('',#190733);
#36349=VERTEX_POINT('',#190734);
#36350=VERTEX_POINT('',#190739);
#36351=VERTEX_POINT('',#190740);
#36352=VERTEX_POINT('',#190745);
#36353=VERTEX_POINT('',#190752);
#36354=VERTEX_POINT('',#190753);
#36355=VERTEX_POINT('',#190755);
#36356=VERTEX_POINT('',#190757);
#36357=VERTEX_POINT('',#190759);
#36358=VERTEX_POINT('',#190763);
#36359=VERTEX_POINT('',#190764);
#36360=VERTEX_POINT('',#190769);
#36361=VERTEX_POINT('',#190770);
#36362=VERTEX_POINT('',#190775);
#36363=VERTEX_POINT('',#190782);
#36364=VERTEX_POINT('',#190783);
#36365=VERTEX_POINT('',#190785);
#36366=VERTEX_POINT('',#190787);
#36367=VERTEX_POINT('',#190791);
#36368=VERTEX_POINT('',#190792);
#36369=VERTEX_POINT('',#190797);
#36370=VERTEX_POINT('',#190798);
#36371=VERTEX_POINT('',#190806);
#36372=VERTEX_POINT('',#190807);
#36373=VERTEX_POINT('',#190809);
#36374=VERTEX_POINT('',#190811);
#36375=VERTEX_POINT('',#190815);
#36376=VERTEX_POINT('',#190816);
#36377=VERTEX_POINT('',#190821);
#36378=VERTEX_POINT('',#190822);
#36379=VERTEX_POINT('',#190830);
#36380=VERTEX_POINT('',#190831);
#36381=VERTEX_POINT('',#190833);
#36382=VERTEX_POINT('',#190835);
#36383=VERTEX_POINT('',#190839);
#36384=VERTEX_POINT('',#190840);
#36385=VERTEX_POINT('',#190845);
#36386=VERTEX_POINT('',#190846);
#36387=VERTEX_POINT('',#190854);
#36388=VERTEX_POINT('',#190855);
#36389=VERTEX_POINT('',#190857);
#36390=VERTEX_POINT('',#190859);
#36391=VERTEX_POINT('',#190863);
#36392=VERTEX_POINT('',#190864);
#36393=VERTEX_POINT('',#190869);
#36394=VERTEX_POINT('',#190870);
#36395=VERTEX_POINT('',#190878);
#36396=VERTEX_POINT('',#190879);
#36397=VERTEX_POINT('',#190881);
#36398=VERTEX_POINT('',#190883);
#36399=VERTEX_POINT('',#190887);
#36400=VERTEX_POINT('',#190888);
#36401=VERTEX_POINT('',#190893);
#36402=VERTEX_POINT('',#190894);
#36403=VERTEX_POINT('',#190896);
#36404=VERTEX_POINT('',#190901);
#36405=VERTEX_POINT('',#190908);
#36406=VERTEX_POINT('',#190909);
#36407=VERTEX_POINT('',#190911);
#36408=VERTEX_POINT('',#190913);
#36409=VERTEX_POINT('',#190917);
#36410=VERTEX_POINT('',#190918);
#36411=VERTEX_POINT('',#190920);
#36412=VERTEX_POINT('',#190925);
#36413=VERTEX_POINT('',#190926);
#36414=VERTEX_POINT('',#190931);
#36415=VERTEX_POINT('',#190938);
#36416=VERTEX_POINT('',#190939);
#36417=VERTEX_POINT('',#190941);
#36418=VERTEX_POINT('',#190943);
#36419=VERTEX_POINT('',#190947);
#36420=VERTEX_POINT('',#190948);
#36421=VERTEX_POINT('',#190950);
#36422=VERTEX_POINT('',#190955);
#36423=VERTEX_POINT('',#190956);
#36424=VERTEX_POINT('',#190961);
#36425=VERTEX_POINT('',#190968);
#36426=VERTEX_POINT('',#190969);
#36427=VERTEX_POINT('',#190971);
#36428=VERTEX_POINT('',#190973);
#36429=VERTEX_POINT('',#190977);
#36430=VERTEX_POINT('',#190978);
#36431=VERTEX_POINT('',#190983);
#36432=VERTEX_POINT('',#190984);
#36433=VERTEX_POINT('',#190986);
#36434=VERTEX_POINT('',#190991);
#36435=VERTEX_POINT('',#190998);
#36436=VERTEX_POINT('',#190999);
#36437=VERTEX_POINT('',#191001);
#36438=VERTEX_POINT('',#191003);
#36439=VERTEX_POINT('',#191007);
#36440=VERTEX_POINT('',#191008);
#36441=VERTEX_POINT('',#191013);
#36442=VERTEX_POINT('',#191014);
#36443=VERTEX_POINT('',#191022);
#36444=VERTEX_POINT('',#191023);
#36445=VERTEX_POINT('',#191025);
#36446=VERTEX_POINT('',#191027);
#36447=VERTEX_POINT('',#191031);
#36448=VERTEX_POINT('',#191032);
#36449=VERTEX_POINT('',#191037);
#36450=VERTEX_POINT('',#191038);
#36451=VERTEX_POINT('',#191046);
#36452=VERTEX_POINT('',#191047);
#36453=VERTEX_POINT('',#191049);
#36454=VERTEX_POINT('',#191051);
#36455=VERTEX_POINT('',#191055);
#36456=VERTEX_POINT('',#191056);
#36457=VERTEX_POINT('',#191061);
#36458=VERTEX_POINT('',#191062);
#36459=VERTEX_POINT('',#191070);
#36460=VERTEX_POINT('',#191071);
#36461=VERTEX_POINT('',#191073);
#36462=VERTEX_POINT('',#191075);
#36463=VERTEX_POINT('',#191079);
#36464=VERTEX_POINT('',#191080);
#36465=VERTEX_POINT('',#191085);
#36466=VERTEX_POINT('',#191086);
#36467=VERTEX_POINT('',#191094);
#36468=VERTEX_POINT('',#191095);
#36469=VERTEX_POINT('',#191097);
#36470=VERTEX_POINT('',#191099);
#36471=VERTEX_POINT('',#191103);
#36472=VERTEX_POINT('',#191104);
#36473=VERTEX_POINT('',#191109);
#36474=VERTEX_POINT('',#191110);
#36475=VERTEX_POINT('',#191118);
#36476=VERTEX_POINT('',#191119);
#36477=VERTEX_POINT('',#191121);
#36478=VERTEX_POINT('',#191123);
#36479=VERTEX_POINT('',#191127);
#36480=VERTEX_POINT('',#191128);
#36481=VERTEX_POINT('',#191133);
#36482=VERTEX_POINT('',#191134);
#36483=VERTEX_POINT('',#191142);
#36484=VERTEX_POINT('',#191143);
#36485=VERTEX_POINT('',#191145);
#36486=VERTEX_POINT('',#191147);
#36487=VERTEX_POINT('',#191151);
#36488=VERTEX_POINT('',#191152);
#36489=VERTEX_POINT('',#191157);
#36490=VERTEX_POINT('',#191158);
#36491=VERTEX_POINT('',#191166);
#36492=VERTEX_POINT('',#191167);
#36493=VERTEX_POINT('',#191169);
#36494=VERTEX_POINT('',#191171);
#36495=VERTEX_POINT('',#191175);
#36496=VERTEX_POINT('',#191176);
#36497=VERTEX_POINT('',#191181);
#36498=VERTEX_POINT('',#191182);
#36499=VERTEX_POINT('',#191190);
#36500=VERTEX_POINT('',#191191);
#36501=VERTEX_POINT('',#191193);
#36502=VERTEX_POINT('',#191195);
#36503=VERTEX_POINT('',#191199);
#36504=VERTEX_POINT('',#191200);
#36505=VERTEX_POINT('',#191205);
#36506=VERTEX_POINT('',#191206);
#36507=VERTEX_POINT('',#191214);
#36508=VERTEX_POINT('',#191215);
#36509=VERTEX_POINT('',#191217);
#36510=VERTEX_POINT('',#191219);
#36511=VERTEX_POINT('',#191223);
#36512=VERTEX_POINT('',#191224);
#36513=VERTEX_POINT('',#191229);
#36514=VERTEX_POINT('',#191230);
#36515=VERTEX_POINT('',#191238);
#36516=VERTEX_POINT('',#191239);
#36517=VERTEX_POINT('',#191241);
#36518=VERTEX_POINT('',#191243);
#36519=VERTEX_POINT('',#191247);
#36520=VERTEX_POINT('',#191248);
#36521=VERTEX_POINT('',#191253);
#36522=VERTEX_POINT('',#191254);
#36523=VERTEX_POINT('',#191256);
#36524=VERTEX_POINT('',#191261);
#36525=VERTEX_POINT('',#191268);
#36526=VERTEX_POINT('',#191269);
#36527=VERTEX_POINT('',#191271);
#36528=VERTEX_POINT('',#191273);
#36529=VERTEX_POINT('',#191277);
#36530=VERTEX_POINT('',#191278);
#36531=VERTEX_POINT('',#191283);
#36532=VERTEX_POINT('',#191284);
#36533=VERTEX_POINT('',#191286);
#36534=VERTEX_POINT('',#191291);
#36535=VERTEX_POINT('',#191298);
#36536=VERTEX_POINT('',#191299);
#36537=VERTEX_POINT('',#191301);
#36538=VERTEX_POINT('',#191303);
#36539=VERTEX_POINT('',#191307);
#36540=VERTEX_POINT('',#191308);
#36541=VERTEX_POINT('',#191313);
#36542=VERTEX_POINT('',#191314);
#36543=VERTEX_POINT('',#191322);
#36544=VERTEX_POINT('',#191323);
#36545=VERTEX_POINT('',#191325);
#36546=VERTEX_POINT('',#191327);
#36547=VERTEX_POINT('',#191331);
#36548=VERTEX_POINT('',#191332);
#36549=VERTEX_POINT('',#191337);
#36550=VERTEX_POINT('',#191338);
#36551=VERTEX_POINT('',#191346);
#36552=VERTEX_POINT('',#191347);
#36553=VERTEX_POINT('',#191349);
#36554=VERTEX_POINT('',#191351);
#36555=VERTEX_POINT('',#191355);
#36556=VERTEX_POINT('',#191356);
#36557=VERTEX_POINT('',#191361);
#36558=VERTEX_POINT('',#191362);
#36559=VERTEX_POINT('',#191370);
#36560=VERTEX_POINT('',#191371);
#36561=VERTEX_POINT('',#191373);
#36562=VERTEX_POINT('',#191375);
#36563=VERTEX_POINT('',#191379);
#36564=VERTEX_POINT('',#191380);
#36565=VERTEX_POINT('',#191385);
#36566=VERTEX_POINT('',#191386);
#36567=VERTEX_POINT('',#191394);
#36568=VERTEX_POINT('',#191395);
#36569=VERTEX_POINT('',#191397);
#36570=VERTEX_POINT('',#191399);
#36571=VERTEX_POINT('',#191403);
#36572=VERTEX_POINT('',#191404);
#36573=VERTEX_POINT('',#191409);
#36574=VERTEX_POINT('',#191410);
#36575=VERTEX_POINT('',#191418);
#36576=VERTEX_POINT('',#191419);
#36577=VERTEX_POINT('',#191421);
#36578=VERTEX_POINT('',#191423);
#36579=VERTEX_POINT('',#191427);
#36580=VERTEX_POINT('',#191428);
#36581=VERTEX_POINT('',#191433);
#36582=VERTEX_POINT('',#191434);
#36583=VERTEX_POINT('',#191442);
#36584=VERTEX_POINT('',#191443);
#36585=VERTEX_POINT('',#191445);
#36586=VERTEX_POINT('',#191447);
#36587=VERTEX_POINT('',#191451);
#36588=VERTEX_POINT('',#191452);
#36589=VERTEX_POINT('',#191457);
#36590=VERTEX_POINT('',#191458);
#36591=VERTEX_POINT('',#191466);
#36592=VERTEX_POINT('',#191467);
#36593=VERTEX_POINT('',#191469);
#36594=VERTEX_POINT('',#191471);
#36595=VERTEX_POINT('',#191475);
#36596=VERTEX_POINT('',#191476);
#36597=VERTEX_POINT('',#191481);
#36598=VERTEX_POINT('',#191482);
#36599=VERTEX_POINT('',#191490);
#36600=VERTEX_POINT('',#191491);
#36601=VERTEX_POINT('',#191493);
#36602=VERTEX_POINT('',#191495);
#36603=VERTEX_POINT('',#191499);
#36604=VERTEX_POINT('',#191500);
#36605=VERTEX_POINT('',#191505);
#36606=VERTEX_POINT('',#191506);
#36607=VERTEX_POINT('',#191514);
#36608=VERTEX_POINT('',#191515);
#36609=VERTEX_POINT('',#191517);
#36610=VERTEX_POINT('',#191519);
#36611=VERTEX_POINT('',#191523);
#36612=VERTEX_POINT('',#191524);
#36613=VERTEX_POINT('',#191526);
#36614=VERTEX_POINT('',#191531);
#36615=VERTEX_POINT('',#191532);
#36616=VERTEX_POINT('',#191537);
#36617=VERTEX_POINT('',#191544);
#36618=VERTEX_POINT('',#191545);
#36619=VERTEX_POINT('',#191547);
#36620=VERTEX_POINT('',#191549);
#36621=VERTEX_POINT('',#191553);
#36622=VERTEX_POINT('',#191554);
#36623=VERTEX_POINT('',#191559);
#36624=VERTEX_POINT('',#191560);
#36625=VERTEX_POINT('',#191562);
#36626=VERTEX_POINT('',#191567);
#36627=VERTEX_POINT('',#191574);
#36628=VERTEX_POINT('',#191575);
#36629=VERTEX_POINT('',#191577);
#36630=VERTEX_POINT('',#191579);
#36631=VERTEX_POINT('',#191583);
#36632=VERTEX_POINT('',#191584);
#36633=VERTEX_POINT('',#191589);
#36634=VERTEX_POINT('',#191590);
#36635=VERTEX_POINT('',#191598);
#36636=VERTEX_POINT('',#191599);
#36637=VERTEX_POINT('',#191601);
#36638=VERTEX_POINT('',#191603);
#36639=VERTEX_POINT('',#191607);
#36640=VERTEX_POINT('',#191608);
#36641=VERTEX_POINT('',#191613);
#36642=VERTEX_POINT('',#191614);
#36643=VERTEX_POINT('',#191622);
#36644=VERTEX_POINT('',#191623);
#36645=VERTEX_POINT('',#191625);
#36646=VERTEX_POINT('',#191627);
#36647=VERTEX_POINT('',#191631);
#36648=VERTEX_POINT('',#191632);
#36649=VERTEX_POINT('',#191637);
#36650=VERTEX_POINT('',#191638);
#36651=VERTEX_POINT('',#191646);
#36652=VERTEX_POINT('',#191647);
#36653=VERTEX_POINT('',#191649);
#36654=VERTEX_POINT('',#191651);
#36655=VERTEX_POINT('',#191655);
#36656=VERTEX_POINT('',#191656);
#36657=VERTEX_POINT('',#191661);
#36658=VERTEX_POINT('',#191662);
#36659=VERTEX_POINT('',#191670);
#36660=VERTEX_POINT('',#191671);
#36661=VERTEX_POINT('',#191673);
#36662=VERTEX_POINT('',#191675);
#36663=VERTEX_POINT('',#191679);
#36664=VERTEX_POINT('',#191680);
#36665=VERTEX_POINT('',#191685);
#36666=VERTEX_POINT('',#191686);
#36667=VERTEX_POINT('',#191694);
#36668=VERTEX_POINT('',#191695);
#36669=VERTEX_POINT('',#191697);
#36670=VERTEX_POINT('',#191699);
#36671=VERTEX_POINT('',#191703);
#36672=VERTEX_POINT('',#191704);
#36673=VERTEX_POINT('',#191709);
#36674=VERTEX_POINT('',#191710);
#36675=VERTEX_POINT('',#191718);
#36676=VERTEX_POINT('',#191719);
#36677=VERTEX_POINT('',#191721);
#36678=VERTEX_POINT('',#191723);
#36679=VERTEX_POINT('',#191727);
#36680=VERTEX_POINT('',#191728);
#36681=VERTEX_POINT('',#191733);
#36682=VERTEX_POINT('',#191734);
#36683=VERTEX_POINT('',#191742);
#36684=VERTEX_POINT('',#191743);
#36685=VERTEX_POINT('',#191745);
#36686=VERTEX_POINT('',#191747);
#36687=VERTEX_POINT('',#191751);
#36688=VERTEX_POINT('',#191752);
#36689=VERTEX_POINT('',#191757);
#36690=VERTEX_POINT('',#191758);
#36691=VERTEX_POINT('',#191766);
#36692=VERTEX_POINT('',#191767);
#36693=VERTEX_POINT('',#191769);
#36694=VERTEX_POINT('',#191771);
#36695=VERTEX_POINT('',#191775);
#36696=VERTEX_POINT('',#191776);
#36697=VERTEX_POINT('',#191781);
#36698=VERTEX_POINT('',#191782);
#36699=VERTEX_POINT('',#191790);
#36700=VERTEX_POINT('',#191791);
#36701=VERTEX_POINT('',#191793);
#36702=VERTEX_POINT('',#191795);
#36703=VERTEX_POINT('',#191799);
#36704=VERTEX_POINT('',#191800);
#36705=VERTEX_POINT('',#191805);
#36706=VERTEX_POINT('',#191806);
#36707=VERTEX_POINT('',#191814);
#36708=VERTEX_POINT('',#191815);
#36709=VERTEX_POINT('',#191817);
#36710=VERTEX_POINT('',#191819);
#36711=VERTEX_POINT('',#191823);
#36712=VERTEX_POINT('',#191824);
#36713=VERTEX_POINT('',#191829);
#36714=VERTEX_POINT('',#191830);
#36715=VERTEX_POINT('',#191838);
#36716=VERTEX_POINT('',#191839);
#36717=VERTEX_POINT('',#191841);
#36718=VERTEX_POINT('',#191843);
#36719=VERTEX_POINT('',#191847);
#36720=VERTEX_POINT('',#191848);
#36721=VERTEX_POINT('',#191853);
#36722=VERTEX_POINT('',#191854);
#36723=VERTEX_POINT('',#191862);
#36724=VERTEX_POINT('',#191863);
#36725=VERTEX_POINT('',#191865);
#36726=VERTEX_POINT('',#191867);
#36727=VERTEX_POINT('',#191871);
#36728=VERTEX_POINT('',#191872);
#36729=VERTEX_POINT('',#191877);
#36730=VERTEX_POINT('',#191878);
#36731=VERTEX_POINT('',#191886);
#36732=VERTEX_POINT('',#191887);
#36733=VERTEX_POINT('',#191889);
#36734=VERTEX_POINT('',#191891);
#36735=VERTEX_POINT('',#191895);
#36736=VERTEX_POINT('',#191896);
#36737=VERTEX_POINT('',#191901);
#36738=VERTEX_POINT('',#191902);
#36739=VERTEX_POINT('',#191910);
#36740=VERTEX_POINT('',#191911);
#36741=VERTEX_POINT('',#191913);
#36742=VERTEX_POINT('',#191915);
#36743=VERTEX_POINT('',#191919);
#36744=VERTEX_POINT('',#191920);
#36745=VERTEX_POINT('',#191925);
#36746=VERTEX_POINT('',#191926);
#36747=VERTEX_POINT('',#191934);
#36748=VERTEX_POINT('',#191935);
#36749=VERTEX_POINT('',#191937);
#36750=VERTEX_POINT('',#191939);
#36751=VERTEX_POINT('',#191943);
#36752=VERTEX_POINT('',#191944);
#36753=VERTEX_POINT('',#191949);
#36754=VERTEX_POINT('',#191950);
#36755=VERTEX_POINT('',#191958);
#36756=VERTEX_POINT('',#191959);
#36757=VERTEX_POINT('',#191961);
#36758=VERTEX_POINT('',#191963);
#36759=VERTEX_POINT('',#191967);
#36760=VERTEX_POINT('',#191968);
#36761=VERTEX_POINT('',#191973);
#36762=VERTEX_POINT('',#191974);
#36763=VERTEX_POINT('',#191982);
#36764=VERTEX_POINT('',#191983);
#36765=VERTEX_POINT('',#191985);
#36766=VERTEX_POINT('',#191987);
#36767=VERTEX_POINT('',#191991);
#36768=VERTEX_POINT('',#191992);
#36769=VERTEX_POINT('',#191997);
#36770=VERTEX_POINT('',#191998);
#36771=VERTEX_POINT('',#192006);
#36772=VERTEX_POINT('',#192007);
#36773=VERTEX_POINT('',#192009);
#36774=VERTEX_POINT('',#192011);
#36775=VERTEX_POINT('',#192015);
#36776=VERTEX_POINT('',#192016);
#36777=VERTEX_POINT('',#192021);
#36778=VERTEX_POINT('',#192022);
#36779=VERTEX_POINT('',#192030);
#36780=VERTEX_POINT('',#192031);
#36781=VERTEX_POINT('',#192033);
#36782=VERTEX_POINT('',#192035);
#36783=VERTEX_POINT('',#192039);
#36784=VERTEX_POINT('',#192040);
#36785=VERTEX_POINT('',#192045);
#36786=VERTEX_POINT('',#192046);
#36787=VERTEX_POINT('',#192054);
#36788=VERTEX_POINT('',#192055);
#36789=VERTEX_POINT('',#192057);
#36790=VERTEX_POINT('',#192059);
#36791=VERTEX_POINT('',#192063);
#36792=VERTEX_POINT('',#192064);
#36793=VERTEX_POINT('',#192069);
#36794=VERTEX_POINT('',#192070);
#36795=VERTEX_POINT('',#192078);
#36796=VERTEX_POINT('',#192079);
#36797=VERTEX_POINT('',#192081);
#36798=VERTEX_POINT('',#192083);
#36799=VERTEX_POINT('',#192087);
#36800=VERTEX_POINT('',#192088);
#36801=VERTEX_POINT('',#192093);
#36802=VERTEX_POINT('',#192094);
#36803=VERTEX_POINT('',#192102);
#36804=VERTEX_POINT('',#192103);
#36805=VERTEX_POINT('',#192105);
#36806=VERTEX_POINT('',#192107);
#36807=VERTEX_POINT('',#192111);
#36808=VERTEX_POINT('',#192112);
#36809=VERTEX_POINT('',#192117);
#36810=VERTEX_POINT('',#192118);
#36811=VERTEX_POINT('',#192126);
#36812=VERTEX_POINT('',#192127);
#36813=VERTEX_POINT('',#192129);
#36814=VERTEX_POINT('',#192131);
#36815=VERTEX_POINT('',#192135);
#36816=VERTEX_POINT('',#192136);
#36817=VERTEX_POINT('',#192141);
#36818=VERTEX_POINT('',#192142);
#36819=VERTEX_POINT('',#192150);
#36820=VERTEX_POINT('',#192151);
#36821=VERTEX_POINT('',#192153);
#36822=VERTEX_POINT('',#192155);
#36823=VERTEX_POINT('',#192159);
#36824=VERTEX_POINT('',#192160);
#36825=VERTEX_POINT('',#192165);
#36826=VERTEX_POINT('',#192166);
#36827=VERTEX_POINT('',#192174);
#36828=VERTEX_POINT('',#192175);
#36829=VERTEX_POINT('',#192177);
#36830=VERTEX_POINT('',#192179);
#36831=VERTEX_POINT('',#192183);
#36832=VERTEX_POINT('',#192184);
#36833=VERTEX_POINT('',#192189);
#36834=VERTEX_POINT('',#192190);
#36835=VERTEX_POINT('',#192198);
#36836=VERTEX_POINT('',#192199);
#36837=VERTEX_POINT('',#192201);
#36838=VERTEX_POINT('',#192203);
#36839=VERTEX_POINT('',#192207);
#36840=VERTEX_POINT('',#192208);
#36841=VERTEX_POINT('',#192213);
#36842=VERTEX_POINT('',#192214);
#36843=VERTEX_POINT('',#192222);
#36844=VERTEX_POINT('',#192223);
#36845=VERTEX_POINT('',#192225);
#36846=VERTEX_POINT('',#192227);
#36847=VERTEX_POINT('',#192231);
#36848=VERTEX_POINT('',#192232);
#36849=VERTEX_POINT('',#192237);
#36850=VERTEX_POINT('',#192238);
#36851=VERTEX_POINT('',#192246);
#36852=VERTEX_POINT('',#192247);
#36853=VERTEX_POINT('',#192249);
#36854=VERTEX_POINT('',#192251);
#36855=VERTEX_POINT('',#192255);
#36856=VERTEX_POINT('',#192256);
#36857=VERTEX_POINT('',#192261);
#36858=VERTEX_POINT('',#192262);
#36859=VERTEX_POINT('',#192270);
#36860=VERTEX_POINT('',#192271);
#36861=VERTEX_POINT('',#192273);
#36862=VERTEX_POINT('',#192275);
#36863=VERTEX_POINT('',#192279);
#36864=VERTEX_POINT('',#192280);
#36865=VERTEX_POINT('',#192285);
#36866=VERTEX_POINT('',#192286);
#36867=VERTEX_POINT('',#192294);
#36868=VERTEX_POINT('',#192295);
#36869=VERTEX_POINT('',#192297);
#36870=VERTEX_POINT('',#192299);
#36871=VERTEX_POINT('',#192303);
#36872=VERTEX_POINT('',#192304);
#36873=VERTEX_POINT('',#192309);
#36874=VERTEX_POINT('',#192310);
#36875=VERTEX_POINT('',#192318);
#36876=VERTEX_POINT('',#192319);
#36877=VERTEX_POINT('',#192321);
#36878=VERTEX_POINT('',#192323);
#36879=VERTEX_POINT('',#192327);
#36880=VERTEX_POINT('',#192328);
#36881=VERTEX_POINT('',#192333);
#36882=VERTEX_POINT('',#192334);
#36883=VERTEX_POINT('',#192342);
#36884=VERTEX_POINT('',#192343);
#36885=VERTEX_POINT('',#192345);
#36886=VERTEX_POINT('',#192347);
#36887=VERTEX_POINT('',#192351);
#36888=VERTEX_POINT('',#192352);
#36889=VERTEX_POINT('',#192357);
#36890=VERTEX_POINT('',#192358);
#36891=VERTEX_POINT('',#192366);
#36892=VERTEX_POINT('',#192367);
#36893=VERTEX_POINT('',#192369);
#36894=VERTEX_POINT('',#192371);
#36895=VERTEX_POINT('',#192375);
#36896=VERTEX_POINT('',#192376);
#36897=VERTEX_POINT('',#192381);
#36898=VERTEX_POINT('',#192382);
#36899=VERTEX_POINT('',#192390);
#36900=VERTEX_POINT('',#192391);
#36901=VERTEX_POINT('',#192393);
#36902=VERTEX_POINT('',#192395);
#36903=VERTEX_POINT('',#192399);
#36904=VERTEX_POINT('',#192400);
#36905=VERTEX_POINT('',#192405);
#36906=VERTEX_POINT('',#192406);
#36907=VERTEX_POINT('',#192414);
#36908=VERTEX_POINT('',#192415);
#36909=VERTEX_POINT('',#192417);
#36910=VERTEX_POINT('',#192419);
#36911=VERTEX_POINT('',#192423);
#36912=VERTEX_POINT('',#192424);
#36913=VERTEX_POINT('',#192429);
#36914=VERTEX_POINT('',#192430);
#36915=VERTEX_POINT('',#192438);
#36916=VERTEX_POINT('',#192439);
#36917=VERTEX_POINT('',#192441);
#36918=VERTEX_POINT('',#192443);
#36919=VERTEX_POINT('',#192447);
#36920=VERTEX_POINT('',#192448);
#36921=VERTEX_POINT('',#192453);
#36922=VERTEX_POINT('',#192454);
#36923=VERTEX_POINT('',#192462);
#36924=VERTEX_POINT('',#192463);
#36925=VERTEX_POINT('',#192465);
#36926=VERTEX_POINT('',#192467);
#36927=VERTEX_POINT('',#192471);
#36928=VERTEX_POINT('',#192472);
#36929=VERTEX_POINT('',#192477);
#36930=VERTEX_POINT('',#192478);
#36931=VERTEX_POINT('',#192486);
#36932=VERTEX_POINT('',#192487);
#36933=VERTEX_POINT('',#192489);
#36934=VERTEX_POINT('',#192491);
#36935=VERTEX_POINT('',#192495);
#36936=VERTEX_POINT('',#192496);
#36937=VERTEX_POINT('',#192501);
#36938=VERTEX_POINT('',#192502);
#36939=VERTEX_POINT('',#192510);
#36940=VERTEX_POINT('',#192511);
#36941=VERTEX_POINT('',#192513);
#36942=VERTEX_POINT('',#192515);
#36943=VERTEX_POINT('',#192519);
#36944=VERTEX_POINT('',#192520);
#36945=VERTEX_POINT('',#192525);
#36946=VERTEX_POINT('',#192526);
#36947=VERTEX_POINT('',#192534);
#36948=VERTEX_POINT('',#192535);
#36949=VERTEX_POINT('',#192537);
#36950=VERTEX_POINT('',#192539);
#36951=VERTEX_POINT('',#192543);
#36952=VERTEX_POINT('',#192544);
#36953=VERTEX_POINT('',#192549);
#36954=VERTEX_POINT('',#192550);
#36955=VERTEX_POINT('',#192558);
#36956=VERTEX_POINT('',#192559);
#36957=VERTEX_POINT('',#192561);
#36958=VERTEX_POINT('',#192563);
#36959=VERTEX_POINT('',#192567);
#36960=VERTEX_POINT('',#192568);
#36961=VERTEX_POINT('',#192573);
#36962=VERTEX_POINT('',#192574);
#36963=VERTEX_POINT('',#192582);
#36964=VERTEX_POINT('',#192583);
#36965=VERTEX_POINT('',#192585);
#36966=VERTEX_POINT('',#192587);
#36967=VERTEX_POINT('',#192591);
#36968=VERTEX_POINT('',#192592);
#36969=VERTEX_POINT('',#192597);
#36970=VERTEX_POINT('',#192598);
#36971=VERTEX_POINT('',#192606);
#36972=VERTEX_POINT('',#192607);
#36973=VERTEX_POINT('',#192609);
#36974=VERTEX_POINT('',#192611);
#36975=VERTEX_POINT('',#192615);
#36976=VERTEX_POINT('',#192616);
#36977=VERTEX_POINT('',#192621);
#36978=VERTEX_POINT('',#192622);
#36979=VERTEX_POINT('',#192630);
#36980=VERTEX_POINT('',#192631);
#36981=VERTEX_POINT('',#192633);
#36982=VERTEX_POINT('',#192635);
#36983=VERTEX_POINT('',#192639);
#36984=VERTEX_POINT('',#192640);
#36985=VERTEX_POINT('',#192645);
#36986=VERTEX_POINT('',#192646);
#36987=VERTEX_POINT('',#192654);
#36988=VERTEX_POINT('',#192655);
#36989=VERTEX_POINT('',#192657);
#36990=VERTEX_POINT('',#192659);
#36991=VERTEX_POINT('',#192663);
#36992=VERTEX_POINT('',#192664);
#36993=VERTEX_POINT('',#192669);
#36994=VERTEX_POINT('',#192670);
#36995=VERTEX_POINT('',#192678);
#36996=VERTEX_POINT('',#192679);
#36997=VERTEX_POINT('',#192681);
#36998=VERTEX_POINT('',#192683);
#36999=VERTEX_POINT('',#192687);
#37000=VERTEX_POINT('',#192688);
#37001=VERTEX_POINT('',#192693);
#37002=VERTEX_POINT('',#192694);
#37003=VERTEX_POINT('',#192702);
#37004=VERTEX_POINT('',#192703);
#37005=VERTEX_POINT('',#192705);
#37006=VERTEX_POINT('',#192707);
#37007=VERTEX_POINT('',#192711);
#37008=VERTEX_POINT('',#192712);
#37009=VERTEX_POINT('',#192717);
#37010=VERTEX_POINT('',#192718);
#37011=VERTEX_POINT('',#192726);
#37012=VERTEX_POINT('',#192727);
#37013=VERTEX_POINT('',#192729);
#37014=VERTEX_POINT('',#192731);
#37015=VERTEX_POINT('',#192735);
#37016=VERTEX_POINT('',#192736);
#37017=VERTEX_POINT('',#192741);
#37018=VERTEX_POINT('',#192742);
#37019=VERTEX_POINT('',#192750);
#37020=VERTEX_POINT('',#192751);
#37021=VERTEX_POINT('',#192753);
#37022=VERTEX_POINT('',#192755);
#37023=VERTEX_POINT('',#192759);
#37024=VERTEX_POINT('',#192760);
#37025=VERTEX_POINT('',#192765);
#37026=VERTEX_POINT('',#192766);
#37027=VERTEX_POINT('',#192774);
#37028=VERTEX_POINT('',#192775);
#37029=VERTEX_POINT('',#192777);
#37030=VERTEX_POINT('',#192779);
#37031=VERTEX_POINT('',#192783);
#37032=VERTEX_POINT('',#192784);
#37033=VERTEX_POINT('',#192789);
#37034=VERTEX_POINT('',#192790);
#37035=VERTEX_POINT('',#192798);
#37036=VERTEX_POINT('',#192799);
#37037=VERTEX_POINT('',#192801);
#37038=VERTEX_POINT('',#192803);
#37039=VERTEX_POINT('',#192807);
#37040=VERTEX_POINT('',#192808);
#37041=VERTEX_POINT('',#192813);
#37042=VERTEX_POINT('',#192814);
#37043=VERTEX_POINT('',#192822);
#37044=VERTEX_POINT('',#192823);
#37045=VERTEX_POINT('',#192825);
#37046=VERTEX_POINT('',#192827);
#37047=VERTEX_POINT('',#192831);
#37048=VERTEX_POINT('',#192832);
#37049=VERTEX_POINT('',#192837);
#37050=VERTEX_POINT('',#192838);
#37051=VERTEX_POINT('',#192846);
#37052=VERTEX_POINT('',#192847);
#37053=VERTEX_POINT('',#192849);
#37054=VERTEX_POINT('',#192851);
#37055=VERTEX_POINT('',#192855);
#37056=VERTEX_POINT('',#192856);
#37057=VERTEX_POINT('',#192861);
#37058=VERTEX_POINT('',#192862);
#37059=VERTEX_POINT('',#192870);
#37060=VERTEX_POINT('',#192871);
#37061=VERTEX_POINT('',#192873);
#37062=VERTEX_POINT('',#192875);
#37063=VERTEX_POINT('',#192879);
#37064=VERTEX_POINT('',#192880);
#37065=VERTEX_POINT('',#192885);
#37066=VERTEX_POINT('',#192886);
#37067=VERTEX_POINT('',#192894);
#37068=VERTEX_POINT('',#192895);
#37069=VERTEX_POINT('',#192897);
#37070=VERTEX_POINT('',#192899);
#37071=VERTEX_POINT('',#192903);
#37072=VERTEX_POINT('',#192904);
#37073=VERTEX_POINT('',#192909);
#37074=VERTEX_POINT('',#192910);
#37075=VERTEX_POINT('',#192918);
#37076=VERTEX_POINT('',#192919);
#37077=VERTEX_POINT('',#192921);
#37078=VERTEX_POINT('',#192923);
#37079=VERTEX_POINT('',#192927);
#37080=VERTEX_POINT('',#192928);
#37081=VERTEX_POINT('',#192933);
#37082=VERTEX_POINT('',#192934);
#37083=VERTEX_POINT('',#192942);
#37084=VERTEX_POINT('',#192943);
#37085=VERTEX_POINT('',#192945);
#37086=VERTEX_POINT('',#192947);
#37087=VERTEX_POINT('',#192951);
#37088=VERTEX_POINT('',#192952);
#37089=VERTEX_POINT('',#192957);
#37090=VERTEX_POINT('',#192958);
#37091=VERTEX_POINT('',#192966);
#37092=VERTEX_POINT('',#192967);
#37093=VERTEX_POINT('',#192969);
#37094=VERTEX_POINT('',#192971);
#37095=VERTEX_POINT('',#192975);
#37096=VERTEX_POINT('',#192976);
#37097=VERTEX_POINT('',#192981);
#37098=VERTEX_POINT('',#192982);
#37099=VERTEX_POINT('',#192990);
#37100=VERTEX_POINT('',#192991);
#37101=VERTEX_POINT('',#192993);
#37102=VERTEX_POINT('',#192995);
#37103=VERTEX_POINT('',#192999);
#37104=VERTEX_POINT('',#193000);
#37105=VERTEX_POINT('',#193005);
#37106=VERTEX_POINT('',#193006);
#37107=VERTEX_POINT('',#193014);
#37108=VERTEX_POINT('',#193015);
#37109=VERTEX_POINT('',#193017);
#37110=VERTEX_POINT('',#193019);
#37111=VERTEX_POINT('',#193023);
#37112=VERTEX_POINT('',#193024);
#37113=VERTEX_POINT('',#193029);
#37114=VERTEX_POINT('',#193030);
#37115=VERTEX_POINT('',#193038);
#37116=VERTEX_POINT('',#193039);
#37117=VERTEX_POINT('',#193041);
#37118=VERTEX_POINT('',#193043);
#37119=VERTEX_POINT('',#193047);
#37120=VERTEX_POINT('',#193048);
#37121=VERTEX_POINT('',#193053);
#37122=VERTEX_POINT('',#193054);
#37123=VERTEX_POINT('',#193062);
#37124=VERTEX_POINT('',#193063);
#37125=VERTEX_POINT('',#193065);
#37126=VERTEX_POINT('',#193067);
#37127=VERTEX_POINT('',#193071);
#37128=VERTEX_POINT('',#193072);
#37129=VERTEX_POINT('',#193077);
#37130=VERTEX_POINT('',#193078);
#37131=VERTEX_POINT('',#193086);
#37132=VERTEX_POINT('',#193087);
#37133=VERTEX_POINT('',#193089);
#37134=VERTEX_POINT('',#193091);
#37135=VERTEX_POINT('',#193095);
#37136=VERTEX_POINT('',#193096);
#37137=VERTEX_POINT('',#193101);
#37138=VERTEX_POINT('',#193102);
#37139=VERTEX_POINT('',#193110);
#37140=VERTEX_POINT('',#193111);
#37141=VERTEX_POINT('',#193113);
#37142=VERTEX_POINT('',#193115);
#37143=VERTEX_POINT('',#193119);
#37144=VERTEX_POINT('',#193120);
#37145=VERTEX_POINT('',#193125);
#37146=VERTEX_POINT('',#193126);
#37147=VERTEX_POINT('',#193134);
#37148=VERTEX_POINT('',#193135);
#37149=VERTEX_POINT('',#193137);
#37150=VERTEX_POINT('',#193139);
#37151=VERTEX_POINT('',#193143);
#37152=VERTEX_POINT('',#193144);
#37153=VERTEX_POINT('',#193149);
#37154=VERTEX_POINT('',#193150);
#37155=VERTEX_POINT('',#193158);
#37156=VERTEX_POINT('',#193159);
#37157=VERTEX_POINT('',#193161);
#37158=VERTEX_POINT('',#193163);
#37159=VERTEX_POINT('',#193167);
#37160=VERTEX_POINT('',#193168);
#37161=VERTEX_POINT('',#193173);
#37162=VERTEX_POINT('',#193174);
#37163=VERTEX_POINT('',#193182);
#37164=VERTEX_POINT('',#193183);
#37165=VERTEX_POINT('',#193185);
#37166=VERTEX_POINT('',#193187);
#37167=VERTEX_POINT('',#193191);
#37168=VERTEX_POINT('',#193192);
#37169=VERTEX_POINT('',#193197);
#37170=VERTEX_POINT('',#193198);
#37171=VERTEX_POINT('',#193206);
#37172=VERTEX_POINT('',#193207);
#37173=VERTEX_POINT('',#193209);
#37174=VERTEX_POINT('',#193211);
#37175=VERTEX_POINT('',#193215);
#37176=VERTEX_POINT('',#193216);
#37177=VERTEX_POINT('',#193221);
#37178=VERTEX_POINT('',#193222);
#37179=VERTEX_POINT('',#193230);
#37180=VERTEX_POINT('',#193231);
#37181=VERTEX_POINT('',#193233);
#37182=VERTEX_POINT('',#193235);
#37183=VERTEX_POINT('',#193239);
#37184=VERTEX_POINT('',#193240);
#37185=VERTEX_POINT('',#193245);
#37186=VERTEX_POINT('',#193246);
#37187=VERTEX_POINT('',#193254);
#37188=VERTEX_POINT('',#193255);
#37189=VERTEX_POINT('',#193257);
#37190=VERTEX_POINT('',#193259);
#37191=VERTEX_POINT('',#193263);
#37192=VERTEX_POINT('',#193264);
#37193=VERTEX_POINT('',#193269);
#37194=VERTEX_POINT('',#193270);
#37195=VERTEX_POINT('',#193278);
#37196=VERTEX_POINT('',#193279);
#37197=VERTEX_POINT('',#193281);
#37198=VERTEX_POINT('',#193283);
#37199=VERTEX_POINT('',#193287);
#37200=VERTEX_POINT('',#193288);
#37201=VERTEX_POINT('',#193293);
#37202=VERTEX_POINT('',#193294);
#37203=VERTEX_POINT('',#193302);
#37204=VERTEX_POINT('',#193303);
#37205=VERTEX_POINT('',#193305);
#37206=VERTEX_POINT('',#193307);
#37207=VERTEX_POINT('',#193311);
#37208=VERTEX_POINT('',#193312);
#37209=VERTEX_POINT('',#193317);
#37210=VERTEX_POINT('',#193318);
#37211=VERTEX_POINT('',#193326);
#37212=VERTEX_POINT('',#193327);
#37213=VERTEX_POINT('',#193329);
#37214=VERTEX_POINT('',#193331);
#37215=VERTEX_POINT('',#193335);
#37216=VERTEX_POINT('',#193336);
#37217=VERTEX_POINT('',#193341);
#37218=VERTEX_POINT('',#193342);
#37219=VERTEX_POINT('',#193350);
#37220=VERTEX_POINT('',#193351);
#37221=VERTEX_POINT('',#193353);
#37222=VERTEX_POINT('',#193355);
#37223=VERTEX_POINT('',#193359);
#37224=VERTEX_POINT('',#193360);
#37225=VERTEX_POINT('',#193365);
#37226=VERTEX_POINT('',#193366);
#37227=VERTEX_POINT('',#193374);
#37228=VERTEX_POINT('',#193375);
#37229=VERTEX_POINT('',#193377);
#37230=VERTEX_POINT('',#193379);
#37231=VERTEX_POINT('',#193383);
#37232=VERTEX_POINT('',#193384);
#37233=VERTEX_POINT('',#193389);
#37234=VERTEX_POINT('',#193390);
#37235=VERTEX_POINT('',#193398);
#37236=VERTEX_POINT('',#193399);
#37237=VERTEX_POINT('',#193401);
#37238=VERTEX_POINT('',#193403);
#37239=VERTEX_POINT('',#193407);
#37240=VERTEX_POINT('',#193408);
#37241=VERTEX_POINT('',#193413);
#37242=VERTEX_POINT('',#193414);
#37243=VERTEX_POINT('',#193423);
#37244=VERTEX_POINT('',#193424);
#37245=VERTEX_POINT('',#193426);
#37246=VERTEX_POINT('',#193428);
#37247=VERTEX_POINT('',#193432);
#37248=VERTEX_POINT('',#193433);
#37249=VERTEX_POINT('',#193438);
#37250=VERTEX_POINT('',#193439);
#37251=VERTEX_POINT('',#193447);
#37252=VERTEX_POINT('',#193448);
#37253=VERTEX_POINT('',#193450);
#37254=VERTEX_POINT('',#193452);
#37255=VERTEX_POINT('',#193456);
#37256=VERTEX_POINT('',#193457);
#37257=VERTEX_POINT('',#193462);
#37258=VERTEX_POINT('',#193463);
#37259=VERTEX_POINT('',#193471);
#37260=VERTEX_POINT('',#193472);
#37261=VERTEX_POINT('',#193474);
#37262=VERTEX_POINT('',#193476);
#37263=VERTEX_POINT('',#193480);
#37264=VERTEX_POINT('',#193481);
#37265=VERTEX_POINT('',#193486);
#37266=VERTEX_POINT('',#193487);
#37267=VERTEX_POINT('',#193495);
#37268=VERTEX_POINT('',#193496);
#37269=VERTEX_POINT('',#193498);
#37270=VERTEX_POINT('',#193500);
#37271=VERTEX_POINT('',#193504);
#37272=VERTEX_POINT('',#193505);
#37273=VERTEX_POINT('',#193510);
#37274=VERTEX_POINT('',#193511);
#37275=VERTEX_POINT('',#193519);
#37276=VERTEX_POINT('',#193520);
#37277=VERTEX_POINT('',#193522);
#37278=VERTEX_POINT('',#193524);
#37279=VERTEX_POINT('',#193528);
#37280=VERTEX_POINT('',#193529);
#37281=VERTEX_POINT('',#193534);
#37282=VERTEX_POINT('',#193535);
#37283=VERTEX_POINT('',#193543);
#37284=VERTEX_POINT('',#193544);
#37285=VERTEX_POINT('',#193546);
#37286=VERTEX_POINT('',#193548);
#37287=VERTEX_POINT('',#193552);
#37288=VERTEX_POINT('',#193553);
#37289=VERTEX_POINT('',#193558);
#37290=VERTEX_POINT('',#193559);
#37291=VERTEX_POINT('',#193567);
#37292=VERTEX_POINT('',#193568);
#37293=VERTEX_POINT('',#193570);
#37294=VERTEX_POINT('',#193572);
#37295=VERTEX_POINT('',#193576);
#37296=VERTEX_POINT('',#193577);
#37297=VERTEX_POINT('',#193582);
#37298=VERTEX_POINT('',#193583);
#37299=VERTEX_POINT('',#193591);
#37300=VERTEX_POINT('',#193592);
#37301=VERTEX_POINT('',#193594);
#37302=VERTEX_POINT('',#193596);
#37303=VERTEX_POINT('',#193600);
#37304=VERTEX_POINT('',#193601);
#37305=VERTEX_POINT('',#193606);
#37306=VERTEX_POINT('',#193607);
#37307=VERTEX_POINT('',#193615);
#37308=VERTEX_POINT('',#193616);
#37309=VERTEX_POINT('',#193618);
#37310=VERTEX_POINT('',#193620);
#37311=VERTEX_POINT('',#193624);
#37312=VERTEX_POINT('',#193625);
#37313=VERTEX_POINT('',#193630);
#37314=VERTEX_POINT('',#193631);
#37315=VERTEX_POINT('',#193639);
#37316=VERTEX_POINT('',#193640);
#37317=VERTEX_POINT('',#193642);
#37318=VERTEX_POINT('',#193644);
#37319=VERTEX_POINT('',#193648);
#37320=VERTEX_POINT('',#193649);
#37321=VERTEX_POINT('',#193654);
#37322=VERTEX_POINT('',#193655);
#37323=VERTEX_POINT('',#193663);
#37324=VERTEX_POINT('',#193664);
#37325=VERTEX_POINT('',#193666);
#37326=VERTEX_POINT('',#193668);
#37327=VERTEX_POINT('',#193672);
#37328=VERTEX_POINT('',#193673);
#37329=VERTEX_POINT('',#193678);
#37330=VERTEX_POINT('',#193679);
#37331=VERTEX_POINT('',#193687);
#37332=VERTEX_POINT('',#193688);
#37333=VERTEX_POINT('',#193690);
#37334=VERTEX_POINT('',#193692);
#37335=VERTEX_POINT('',#193696);
#37336=VERTEX_POINT('',#193697);
#37337=VERTEX_POINT('',#193702);
#37338=VERTEX_POINT('',#193703);
#37339=VERTEX_POINT('',#193711);
#37340=VERTEX_POINT('',#193712);
#37341=VERTEX_POINT('',#193714);
#37342=VERTEX_POINT('',#193716);
#37343=VERTEX_POINT('',#193720);
#37344=VERTEX_POINT('',#193721);
#37345=VERTEX_POINT('',#193726);
#37346=VERTEX_POINT('',#193727);
#37347=VERTEX_POINT('',#193735);
#37348=VERTEX_POINT('',#193736);
#37349=VERTEX_POINT('',#193738);
#37350=VERTEX_POINT('',#193740);
#37351=VERTEX_POINT('',#193744);
#37352=VERTEX_POINT('',#193745);
#37353=VERTEX_POINT('',#193750);
#37354=VERTEX_POINT('',#193751);
#37355=VERTEX_POINT('',#193759);
#37356=VERTEX_POINT('',#193760);
#37357=VERTEX_POINT('',#193762);
#37358=VERTEX_POINT('',#193764);
#37359=VERTEX_POINT('',#193768);
#37360=VERTEX_POINT('',#193769);
#37361=VERTEX_POINT('',#193774);
#37362=VERTEX_POINT('',#193775);
#37363=VERTEX_POINT('',#193783);
#37364=VERTEX_POINT('',#193784);
#37365=VERTEX_POINT('',#193786);
#37366=VERTEX_POINT('',#193788);
#37367=VERTEX_POINT('',#193792);
#37368=VERTEX_POINT('',#193793);
#37369=VERTEX_POINT('',#193798);
#37370=VERTEX_POINT('',#193799);
#37371=VERTEX_POINT('',#193807);
#37372=VERTEX_POINT('',#193808);
#37373=VERTEX_POINT('',#193810);
#37374=VERTEX_POINT('',#193812);
#37375=VERTEX_POINT('',#193816);
#37376=VERTEX_POINT('',#193817);
#37377=VERTEX_POINT('',#193822);
#37378=VERTEX_POINT('',#193823);
#37379=VERTEX_POINT('',#193831);
#37380=VERTEX_POINT('',#193832);
#37381=VERTEX_POINT('',#193834);
#37382=VERTEX_POINT('',#193836);
#37383=VERTEX_POINT('',#193840);
#37384=VERTEX_POINT('',#193841);
#37385=VERTEX_POINT('',#193846);
#37386=VERTEX_POINT('',#193847);
#37387=VERTEX_POINT('',#193855);
#37388=VERTEX_POINT('',#193856);
#37389=VERTEX_POINT('',#193858);
#37390=VERTEX_POINT('',#193860);
#37391=VERTEX_POINT('',#193864);
#37392=VERTEX_POINT('',#193865);
#37393=VERTEX_POINT('',#193870);
#37394=VERTEX_POINT('',#193871);
#37395=VERTEX_POINT('',#193879);
#37396=VERTEX_POINT('',#193880);
#37397=VERTEX_POINT('',#193882);
#37398=VERTEX_POINT('',#193884);
#37399=VERTEX_POINT('',#193888);
#37400=VERTEX_POINT('',#193889);
#37401=VERTEX_POINT('',#193894);
#37402=VERTEX_POINT('',#193895);
#37403=VERTEX_POINT('',#193903);
#37404=VERTEX_POINT('',#193904);
#37405=VERTEX_POINT('',#193906);
#37406=VERTEX_POINT('',#193908);
#37407=VERTEX_POINT('',#193912);
#37408=VERTEX_POINT('',#193913);
#37409=VERTEX_POINT('',#193918);
#37410=VERTEX_POINT('',#193919);
#37411=VERTEX_POINT('',#193927);
#37412=VERTEX_POINT('',#193928);
#37413=VERTEX_POINT('',#193930);
#37414=VERTEX_POINT('',#193932);
#37415=VERTEX_POINT('',#193936);
#37416=VERTEX_POINT('',#193937);
#37417=VERTEX_POINT('',#193942);
#37418=VERTEX_POINT('',#193943);
#37419=VERTEX_POINT('',#193951);
#37420=VERTEX_POINT('',#193952);
#37421=VERTEX_POINT('',#193954);
#37422=VERTEX_POINT('',#193956);
#37423=VERTEX_POINT('',#193960);
#37424=VERTEX_POINT('',#193961);
#37425=VERTEX_POINT('',#193966);
#37426=VERTEX_POINT('',#193967);
#37427=VERTEX_POINT('',#193975);
#37428=VERTEX_POINT('',#193976);
#37429=VERTEX_POINT('',#193978);
#37430=VERTEX_POINT('',#193980);
#37431=VERTEX_POINT('',#193984);
#37432=VERTEX_POINT('',#193985);
#37433=VERTEX_POINT('',#193990);
#37434=VERTEX_POINT('',#193991);
#37435=VERTEX_POINT('',#193999);
#37436=VERTEX_POINT('',#194000);
#37437=VERTEX_POINT('',#194002);
#37438=VERTEX_POINT('',#194004);
#37439=VERTEX_POINT('',#194008);
#37440=VERTEX_POINT('',#194009);
#37441=VERTEX_POINT('',#194014);
#37442=VERTEX_POINT('',#194015);
#37443=VERTEX_POINT('',#194023);
#37444=VERTEX_POINT('',#194024);
#37445=VERTEX_POINT('',#194026);
#37446=VERTEX_POINT('',#194028);
#37447=VERTEX_POINT('',#194032);
#37448=VERTEX_POINT('',#194033);
#37449=VERTEX_POINT('',#194038);
#37450=VERTEX_POINT('',#194039);
#37451=VERTEX_POINT('',#194047);
#37452=VERTEX_POINT('',#194048);
#37453=VERTEX_POINT('',#194050);
#37454=VERTEX_POINT('',#194052);
#37455=VERTEX_POINT('',#194056);
#37456=VERTEX_POINT('',#194057);
#37457=VERTEX_POINT('',#194062);
#37458=VERTEX_POINT('',#194063);
#37459=VERTEX_POINT('',#194071);
#37460=VERTEX_POINT('',#194072);
#37461=VERTEX_POINT('',#194074);
#37462=VERTEX_POINT('',#194076);
#37463=VERTEX_POINT('',#194080);
#37464=VERTEX_POINT('',#194081);
#37465=VERTEX_POINT('',#194086);
#37466=VERTEX_POINT('',#194087);
#37467=VERTEX_POINT('',#194095);
#37468=VERTEX_POINT('',#194096);
#37469=VERTEX_POINT('',#194098);
#37470=VERTEX_POINT('',#194100);
#37471=VERTEX_POINT('',#194104);
#37472=VERTEX_POINT('',#194105);
#37473=VERTEX_POINT('',#194110);
#37474=VERTEX_POINT('',#194111);
#37475=VERTEX_POINT('',#194119);
#37476=VERTEX_POINT('',#194120);
#37477=VERTEX_POINT('',#194122);
#37478=VERTEX_POINT('',#194124);
#37479=VERTEX_POINT('',#194128);
#37480=VERTEX_POINT('',#194129);
#37481=VERTEX_POINT('',#194134);
#37482=VERTEX_POINT('',#194135);
#37483=VERTEX_POINT('',#194143);
#37484=VERTEX_POINT('',#194144);
#37485=VERTEX_POINT('',#194146);
#37486=VERTEX_POINT('',#194148);
#37487=VERTEX_POINT('',#194152);
#37488=VERTEX_POINT('',#194153);
#37489=VERTEX_POINT('',#194158);
#37490=VERTEX_POINT('',#194159);
#37491=VERTEX_POINT('',#194167);
#37492=VERTEX_POINT('',#194168);
#37493=VERTEX_POINT('',#194170);
#37494=VERTEX_POINT('',#194172);
#37495=VERTEX_POINT('',#194176);
#37496=VERTEX_POINT('',#194177);
#37497=VERTEX_POINT('',#194182);
#37498=VERTEX_POINT('',#194183);
#37499=VERTEX_POINT('',#194191);
#37500=VERTEX_POINT('',#194192);
#37501=VERTEX_POINT('',#194194);
#37502=VERTEX_POINT('',#194196);
#37503=VERTEX_POINT('',#194200);
#37504=VERTEX_POINT('',#194201);
#37505=VERTEX_POINT('',#194206);
#37506=VERTEX_POINT('',#194207);
#37507=VERTEX_POINT('',#194215);
#37508=VERTEX_POINT('',#194216);
#37509=VERTEX_POINT('',#194218);
#37510=VERTEX_POINT('',#194220);
#37511=VERTEX_POINT('',#194224);
#37512=VERTEX_POINT('',#194225);
#37513=VERTEX_POINT('',#194230);
#37514=VERTEX_POINT('',#194231);
#37515=VERTEX_POINT('',#194239);
#37516=VERTEX_POINT('',#194240);
#37517=VERTEX_POINT('',#194242);
#37518=VERTEX_POINT('',#194244);
#37519=VERTEX_POINT('',#194248);
#37520=VERTEX_POINT('',#194249);
#37521=VERTEX_POINT('',#194254);
#37522=VERTEX_POINT('',#194255);
#37523=VERTEX_POINT('',#194263);
#37524=VERTEX_POINT('',#194264);
#37525=VERTEX_POINT('',#194266);
#37526=VERTEX_POINT('',#194268);
#37527=VERTEX_POINT('',#194272);
#37528=VERTEX_POINT('',#194273);
#37529=VERTEX_POINT('',#194278);
#37530=VERTEX_POINT('',#194279);
#37531=VERTEX_POINT('',#194287);
#37532=VERTEX_POINT('',#194288);
#37533=VERTEX_POINT('',#194290);
#37534=VERTEX_POINT('',#194292);
#37535=VERTEX_POINT('',#194296);
#37536=VERTEX_POINT('',#194297);
#37537=VERTEX_POINT('',#194302);
#37538=VERTEX_POINT('',#194303);
#37539=VERTEX_POINT('',#194311);
#37540=VERTEX_POINT('',#194312);
#37541=VERTEX_POINT('',#194314);
#37542=VERTEX_POINT('',#194316);
#37543=VERTEX_POINT('',#194320);
#37544=VERTEX_POINT('',#194321);
#37545=VERTEX_POINT('',#194326);
#37546=VERTEX_POINT('',#194327);
#37547=VERTEX_POINT('',#194335);
#37548=VERTEX_POINT('',#194336);
#37549=VERTEX_POINT('',#194338);
#37550=VERTEX_POINT('',#194340);
#37551=VERTEX_POINT('',#194344);
#37552=VERTEX_POINT('',#194345);
#37553=VERTEX_POINT('',#194350);
#37554=VERTEX_POINT('',#194351);
#37555=VERTEX_POINT('',#194359);
#37556=VERTEX_POINT('',#194360);
#37557=VERTEX_POINT('',#194362);
#37558=VERTEX_POINT('',#194364);
#37559=VERTEX_POINT('',#194368);
#37560=VERTEX_POINT('',#194369);
#37561=VERTEX_POINT('',#194374);
#37562=VERTEX_POINT('',#194375);
#37563=VERTEX_POINT('',#194383);
#37564=VERTEX_POINT('',#194384);
#37565=VERTEX_POINT('',#194386);
#37566=VERTEX_POINT('',#194388);
#37567=VERTEX_POINT('',#194392);
#37568=VERTEX_POINT('',#194393);
#37569=VERTEX_POINT('',#194398);
#37570=VERTEX_POINT('',#194399);
#37571=VERTEX_POINT('',#194407);
#37572=VERTEX_POINT('',#194408);
#37573=VERTEX_POINT('',#194410);
#37574=VERTEX_POINT('',#194412);
#37575=VERTEX_POINT('',#194416);
#37576=VERTEX_POINT('',#194417);
#37577=VERTEX_POINT('',#194422);
#37578=VERTEX_POINT('',#194423);
#37579=VERTEX_POINT('',#194431);
#37580=VERTEX_POINT('',#194432);
#37581=VERTEX_POINT('',#194434);
#37582=VERTEX_POINT('',#194436);
#37583=VERTEX_POINT('',#194440);
#37584=VERTEX_POINT('',#194441);
#37585=VERTEX_POINT('',#194446);
#37586=VERTEX_POINT('',#194447);
#37587=VERTEX_POINT('',#194455);
#37588=VERTEX_POINT('',#194456);
#37589=VERTEX_POINT('',#194458);
#37590=VERTEX_POINT('',#194460);
#37591=VERTEX_POINT('',#194464);
#37592=VERTEX_POINT('',#194465);
#37593=VERTEX_POINT('',#194470);
#37594=VERTEX_POINT('',#194471);
#37595=VERTEX_POINT('',#194479);
#37596=VERTEX_POINT('',#194480);
#37597=VERTEX_POINT('',#194482);
#37598=VERTEX_POINT('',#194484);
#37599=VERTEX_POINT('',#194488);
#37600=VERTEX_POINT('',#194489);
#37601=VERTEX_POINT('',#194494);
#37602=VERTEX_POINT('',#194495);
#37603=VERTEX_POINT('',#194503);
#37604=VERTEX_POINT('',#194504);
#37605=VERTEX_POINT('',#194506);
#37606=VERTEX_POINT('',#194508);
#37607=VERTEX_POINT('',#194512);
#37608=VERTEX_POINT('',#194513);
#37609=VERTEX_POINT('',#194518);
#37610=VERTEX_POINT('',#194519);
#37611=VERTEX_POINT('',#194527);
#37612=VERTEX_POINT('',#194528);
#37613=VERTEX_POINT('',#194530);
#37614=VERTEX_POINT('',#194532);
#37615=VERTEX_POINT('',#194536);
#37616=VERTEX_POINT('',#194537);
#37617=VERTEX_POINT('',#194542);
#37618=VERTEX_POINT('',#194543);
#37619=VERTEX_POINT('',#194551);
#37620=VERTEX_POINT('',#194552);
#37621=VERTEX_POINT('',#194554);
#37622=VERTEX_POINT('',#194556);
#37623=VERTEX_POINT('',#194560);
#37624=VERTEX_POINT('',#194561);
#37625=VERTEX_POINT('',#194566);
#37626=VERTEX_POINT('',#194567);
#37627=VERTEX_POINT('',#194575);
#37628=VERTEX_POINT('',#194576);
#37629=VERTEX_POINT('',#194578);
#37630=VERTEX_POINT('',#194580);
#37631=VERTEX_POINT('',#194584);
#37632=VERTEX_POINT('',#194585);
#37633=VERTEX_POINT('',#194590);
#37634=VERTEX_POINT('',#194591);
#37635=VERTEX_POINT('',#194599);
#37636=VERTEX_POINT('',#194600);
#37637=VERTEX_POINT('',#194602);
#37638=VERTEX_POINT('',#194604);
#37639=VERTEX_POINT('',#194608);
#37640=VERTEX_POINT('',#194609);
#37641=VERTEX_POINT('',#194614);
#37642=VERTEX_POINT('',#194615);
#37643=VERTEX_POINT('',#194623);
#37644=VERTEX_POINT('',#194624);
#37645=VERTEX_POINT('',#194626);
#37646=VERTEX_POINT('',#194628);
#37647=VERTEX_POINT('',#194632);
#37648=VERTEX_POINT('',#194633);
#37649=VERTEX_POINT('',#194638);
#37650=VERTEX_POINT('',#194639);
#37651=VERTEX_POINT('',#194647);
#37652=VERTEX_POINT('',#194648);
#37653=VERTEX_POINT('',#194650);
#37654=VERTEX_POINT('',#194652);
#37655=VERTEX_POINT('',#194656);
#37656=VERTEX_POINT('',#194657);
#37657=VERTEX_POINT('',#194662);
#37658=VERTEX_POINT('',#194663);
#37659=VERTEX_POINT('',#194671);
#37660=VERTEX_POINT('',#194672);
#37661=VERTEX_POINT('',#194674);
#37662=VERTEX_POINT('',#194676);
#37663=VERTEX_POINT('',#194680);
#37664=VERTEX_POINT('',#194681);
#37665=VERTEX_POINT('',#194686);
#37666=VERTEX_POINT('',#194687);
#37667=VERTEX_POINT('',#194695);
#37668=VERTEX_POINT('',#194696);
#37669=VERTEX_POINT('',#194698);
#37670=VERTEX_POINT('',#194700);
#37671=VERTEX_POINT('',#194704);
#37672=VERTEX_POINT('',#194705);
#37673=VERTEX_POINT('',#194710);
#37674=VERTEX_POINT('',#194711);
#37675=VERTEX_POINT('',#194719);
#37676=VERTEX_POINT('',#194720);
#37677=VERTEX_POINT('',#194722);
#37678=VERTEX_POINT('',#194724);
#37679=VERTEX_POINT('',#194728);
#37680=VERTEX_POINT('',#194729);
#37681=VERTEX_POINT('',#194734);
#37682=VERTEX_POINT('',#194735);
#37683=VERTEX_POINT('',#194743);
#37684=VERTEX_POINT('',#194744);
#37685=VERTEX_POINT('',#194746);
#37686=VERTEX_POINT('',#194748);
#37687=VERTEX_POINT('',#194752);
#37688=VERTEX_POINT('',#194753);
#37689=VERTEX_POINT('',#194758);
#37690=VERTEX_POINT('',#194759);
#37691=VERTEX_POINT('',#194767);
#37692=VERTEX_POINT('',#194768);
#37693=VERTEX_POINT('',#194770);
#37694=VERTEX_POINT('',#194772);
#37695=VERTEX_POINT('',#194776);
#37696=VERTEX_POINT('',#194777);
#37697=VERTEX_POINT('',#194782);
#37698=VERTEX_POINT('',#194783);
#37699=VERTEX_POINT('',#194791);
#37700=VERTEX_POINT('',#194792);
#37701=VERTEX_POINT('',#194794);
#37702=VERTEX_POINT('',#194796);
#37703=VERTEX_POINT('',#194800);
#37704=VERTEX_POINT('',#194801);
#37705=VERTEX_POINT('',#194806);
#37706=VERTEX_POINT('',#194807);
#37707=VERTEX_POINT('',#194815);
#37708=VERTEX_POINT('',#194816);
#37709=VERTEX_POINT('',#194818);
#37710=VERTEX_POINT('',#194820);
#37711=VERTEX_POINT('',#194824);
#37712=VERTEX_POINT('',#194825);
#37713=VERTEX_POINT('',#194830);
#37714=VERTEX_POINT('',#194831);
#37715=VERTEX_POINT('',#194839);
#37716=VERTEX_POINT('',#194840);
#37717=VERTEX_POINT('',#194842);
#37718=VERTEX_POINT('',#194844);
#37719=VERTEX_POINT('',#194848);
#37720=VERTEX_POINT('',#194849);
#37721=VERTEX_POINT('',#194854);
#37722=VERTEX_POINT('',#194855);
#37723=VERTEX_POINT('',#194863);
#37724=VERTEX_POINT('',#194864);
#37725=VERTEX_POINT('',#194866);
#37726=VERTEX_POINT('',#194868);
#37727=VERTEX_POINT('',#194872);
#37728=VERTEX_POINT('',#194873);
#37729=VERTEX_POINT('',#194878);
#37730=VERTEX_POINT('',#194879);
#37731=VERTEX_POINT('',#194887);
#37732=VERTEX_POINT('',#194888);
#37733=VERTEX_POINT('',#194890);
#37734=VERTEX_POINT('',#194892);
#37735=VERTEX_POINT('',#194896);
#37736=VERTEX_POINT('',#194897);
#37737=VERTEX_POINT('',#194902);
#37738=VERTEX_POINT('',#194903);
#37739=VERTEX_POINT('',#194911);
#37740=VERTEX_POINT('',#194912);
#37741=VERTEX_POINT('',#194914);
#37742=VERTEX_POINT('',#194916);
#37743=VERTEX_POINT('',#194920);
#37744=VERTEX_POINT('',#194921);
#37745=VERTEX_POINT('',#194926);
#37746=VERTEX_POINT('',#194927);
#37747=VERTEX_POINT('',#194935);
#37748=VERTEX_POINT('',#194936);
#37749=VERTEX_POINT('',#194938);
#37750=VERTEX_POINT('',#194940);
#37751=VERTEX_POINT('',#194944);
#37752=VERTEX_POINT('',#194945);
#37753=VERTEX_POINT('',#194950);
#37754=VERTEX_POINT('',#194951);
#37755=VERTEX_POINT('',#194959);
#37756=VERTEX_POINT('',#194960);
#37757=VERTEX_POINT('',#194962);
#37758=VERTEX_POINT('',#194964);
#37759=VERTEX_POINT('',#194968);
#37760=VERTEX_POINT('',#194969);
#37761=VERTEX_POINT('',#194974);
#37762=VERTEX_POINT('',#194975);
#37763=VERTEX_POINT('',#194983);
#37764=VERTEX_POINT('',#194984);
#37765=VERTEX_POINT('',#194986);
#37766=VERTEX_POINT('',#194988);
#37767=VERTEX_POINT('',#194992);
#37768=VERTEX_POINT('',#194993);
#37769=VERTEX_POINT('',#194998);
#37770=VERTEX_POINT('',#194999);
#37771=VERTEX_POINT('',#195007);
#37772=VERTEX_POINT('',#195008);
#37773=VERTEX_POINT('',#195010);
#37774=VERTEX_POINT('',#195012);
#37775=VERTEX_POINT('',#195016);
#37776=VERTEX_POINT('',#195017);
#37777=VERTEX_POINT('',#195022);
#37778=VERTEX_POINT('',#195023);
#37779=VERTEX_POINT('',#195031);
#37780=VERTEX_POINT('',#195032);
#37781=VERTEX_POINT('',#195034);
#37782=VERTEX_POINT('',#195036);
#37783=VERTEX_POINT('',#195040);
#37784=VERTEX_POINT('',#195041);
#37785=VERTEX_POINT('',#195046);
#37786=VERTEX_POINT('',#195047);
#37787=VERTEX_POINT('',#195055);
#37788=VERTEX_POINT('',#195056);
#37789=VERTEX_POINT('',#195058);
#37790=VERTEX_POINT('',#195060);
#37791=VERTEX_POINT('',#195064);
#37792=VERTEX_POINT('',#195065);
#37793=VERTEX_POINT('',#195070);
#37794=VERTEX_POINT('',#195071);
#37795=VERTEX_POINT('',#195079);
#37796=VERTEX_POINT('',#195080);
#37797=VERTEX_POINT('',#195082);
#37798=VERTEX_POINT('',#195084);
#37799=VERTEX_POINT('',#195088);
#37800=VERTEX_POINT('',#195089);
#37801=VERTEX_POINT('',#195094);
#37802=VERTEX_POINT('',#195095);
#37803=VERTEX_POINT('',#195103);
#37804=VERTEX_POINT('',#195104);
#37805=VERTEX_POINT('',#195106);
#37806=VERTEX_POINT('',#195108);
#37807=VERTEX_POINT('',#195112);
#37808=VERTEX_POINT('',#195113);
#37809=VERTEX_POINT('',#195118);
#37810=VERTEX_POINT('',#195119);
#37811=VERTEX_POINT('',#195127);
#37812=VERTEX_POINT('',#195128);
#37813=VERTEX_POINT('',#195130);
#37814=VERTEX_POINT('',#195132);
#37815=VERTEX_POINT('',#195136);
#37816=VERTEX_POINT('',#195137);
#37817=VERTEX_POINT('',#195142);
#37818=VERTEX_POINT('',#195143);
#37819=VERTEX_POINT('',#195151);
#37820=VERTEX_POINT('',#195152);
#37821=VERTEX_POINT('',#195154);
#37822=VERTEX_POINT('',#195156);
#37823=VERTEX_POINT('',#195160);
#37824=VERTEX_POINT('',#195161);
#37825=VERTEX_POINT('',#195166);
#37826=VERTEX_POINT('',#195167);
#37827=VERTEX_POINT('',#195175);
#37828=VERTEX_POINT('',#195176);
#37829=VERTEX_POINT('',#195178);
#37830=VERTEX_POINT('',#195180);
#37831=VERTEX_POINT('',#195184);
#37832=VERTEX_POINT('',#195185);
#37833=VERTEX_POINT('',#195190);
#37834=VERTEX_POINT('',#195191);
#37835=VERTEX_POINT('',#195199);
#37836=VERTEX_POINT('',#195200);
#37837=VERTEX_POINT('',#195202);
#37838=VERTEX_POINT('',#195204);
#37839=VERTEX_POINT('',#195208);
#37840=VERTEX_POINT('',#195209);
#37841=VERTEX_POINT('',#195214);
#37842=VERTEX_POINT('',#195215);
#37843=VERTEX_POINT('',#195223);
#37844=VERTEX_POINT('',#195224);
#37845=VERTEX_POINT('',#195226);
#37846=VERTEX_POINT('',#195228);
#37847=VERTEX_POINT('',#195232);
#37848=VERTEX_POINT('',#195233);
#37849=VERTEX_POINT('',#195238);
#37850=VERTEX_POINT('',#195239);
#37851=VERTEX_POINT('',#195247);
#37852=VERTEX_POINT('',#195248);
#37853=VERTEX_POINT('',#195250);
#37854=VERTEX_POINT('',#195252);
#37855=VERTEX_POINT('',#195256);
#37856=VERTEX_POINT('',#195257);
#37857=VERTEX_POINT('',#195262);
#37858=VERTEX_POINT('',#195263);
#37859=VERTEX_POINT('',#195271);
#37860=VERTEX_POINT('',#195272);
#37861=VERTEX_POINT('',#195274);
#37862=VERTEX_POINT('',#195276);
#37863=VERTEX_POINT('',#195280);
#37864=VERTEX_POINT('',#195281);
#37865=VERTEX_POINT('',#195286);
#37866=VERTEX_POINT('',#195287);
#37867=VERTEX_POINT('',#195295);
#37868=VERTEX_POINT('',#195296);
#37869=VERTEX_POINT('',#195298);
#37870=VERTEX_POINT('',#195300);
#37871=VERTEX_POINT('',#195304);
#37872=VERTEX_POINT('',#195305);
#37873=VERTEX_POINT('',#195310);
#37874=VERTEX_POINT('',#195311);
#37875=VERTEX_POINT('',#195319);
#37876=VERTEX_POINT('',#195320);
#37877=VERTEX_POINT('',#195322);
#37878=VERTEX_POINT('',#195324);
#37879=VERTEX_POINT('',#195328);
#37880=VERTEX_POINT('',#195329);
#37881=VERTEX_POINT('',#195334);
#37882=VERTEX_POINT('',#195335);
#37883=VERTEX_POINT('',#195343);
#37884=VERTEX_POINT('',#195344);
#37885=VERTEX_POINT('',#195346);
#37886=VERTEX_POINT('',#195348);
#37887=VERTEX_POINT('',#195352);
#37888=VERTEX_POINT('',#195353);
#37889=VERTEX_POINT('',#195358);
#37890=VERTEX_POINT('',#195359);
#37891=VERTEX_POINT('',#195367);
#37892=VERTEX_POINT('',#195368);
#37893=VERTEX_POINT('',#195370);
#37894=VERTEX_POINT('',#195372);
#37895=VERTEX_POINT('',#195376);
#37896=VERTEX_POINT('',#195377);
#37897=VERTEX_POINT('',#195382);
#37898=VERTEX_POINT('',#195383);
#37899=VERTEX_POINT('',#195391);
#37900=VERTEX_POINT('',#195392);
#37901=VERTEX_POINT('',#195394);
#37902=VERTEX_POINT('',#195396);
#37903=VERTEX_POINT('',#195400);
#37904=VERTEX_POINT('',#195401);
#37905=VERTEX_POINT('',#195406);
#37906=VERTEX_POINT('',#195407);
#37907=VERTEX_POINT('',#195415);
#37908=VERTEX_POINT('',#195416);
#37909=VERTEX_POINT('',#195418);
#37910=VERTEX_POINT('',#195420);
#37911=VERTEX_POINT('',#195424);
#37912=VERTEX_POINT('',#195425);
#37913=VERTEX_POINT('',#195430);
#37914=VERTEX_POINT('',#195431);
#37915=VERTEX_POINT('',#195439);
#37916=VERTEX_POINT('',#195440);
#37917=VERTEX_POINT('',#195442);
#37918=VERTEX_POINT('',#195444);
#37919=VERTEX_POINT('',#195448);
#37920=VERTEX_POINT('',#195449);
#37921=VERTEX_POINT('',#195454);
#37922=VERTEX_POINT('',#195455);
#37923=VERTEX_POINT('',#195463);
#37924=VERTEX_POINT('',#195464);
#37925=VERTEX_POINT('',#195466);
#37926=VERTEX_POINT('',#195468);
#37927=VERTEX_POINT('',#195472);
#37928=VERTEX_POINT('',#195473);
#37929=VERTEX_POINT('',#195478);
#37930=VERTEX_POINT('',#195479);
#37931=VERTEX_POINT('',#195487);
#37932=VERTEX_POINT('',#195488);
#37933=VERTEX_POINT('',#195490);
#37934=VERTEX_POINT('',#195492);
#37935=VERTEX_POINT('',#195496);
#37936=VERTEX_POINT('',#195497);
#37937=VERTEX_POINT('',#195502);
#37938=VERTEX_POINT('',#195503);
#37939=VERTEX_POINT('',#195511);
#37940=VERTEX_POINT('',#195512);
#37941=VERTEX_POINT('',#195514);
#37942=VERTEX_POINT('',#195516);
#37943=VERTEX_POINT('',#195520);
#37944=VERTEX_POINT('',#195521);
#37945=VERTEX_POINT('',#195526);
#37946=VERTEX_POINT('',#195527);
#37947=VERTEX_POINT('',#195535);
#37948=VERTEX_POINT('',#195536);
#37949=VERTEX_POINT('',#195538);
#37950=VERTEX_POINT('',#195540);
#37951=VERTEX_POINT('',#195544);
#37952=VERTEX_POINT('',#195545);
#37953=VERTEX_POINT('',#195550);
#37954=VERTEX_POINT('',#195551);
#37955=VERTEX_POINT('',#195559);
#37956=VERTEX_POINT('',#195560);
#37957=VERTEX_POINT('',#195562);
#37958=VERTEX_POINT('',#195564);
#37959=VERTEX_POINT('',#195568);
#37960=VERTEX_POINT('',#195569);
#37961=VERTEX_POINT('',#195574);
#37962=VERTEX_POINT('',#195575);
#37963=VERTEX_POINT('',#195583);
#37964=VERTEX_POINT('',#195584);
#37965=VERTEX_POINT('',#195586);
#37966=VERTEX_POINT('',#195588);
#37967=VERTEX_POINT('',#195592);
#37968=VERTEX_POINT('',#195593);
#37969=VERTEX_POINT('',#195598);
#37970=VERTEX_POINT('',#195599);
#37971=VERTEX_POINT('',#195607);
#37972=VERTEX_POINT('',#195608);
#37973=VERTEX_POINT('',#195610);
#37974=VERTEX_POINT('',#195612);
#37975=VERTEX_POINT('',#195616);
#37976=VERTEX_POINT('',#195617);
#37977=VERTEX_POINT('',#195622);
#37978=VERTEX_POINT('',#195623);
#37979=VERTEX_POINT('',#195631);
#37980=VERTEX_POINT('',#195632);
#37981=VERTEX_POINT('',#195634);
#37982=VERTEX_POINT('',#195636);
#37983=VERTEX_POINT('',#195640);
#37984=VERTEX_POINT('',#195641);
#37985=VERTEX_POINT('',#195646);
#37986=VERTEX_POINT('',#195647);
#37987=VERTEX_POINT('',#195655);
#37988=VERTEX_POINT('',#195656);
#37989=VERTEX_POINT('',#195658);
#37990=VERTEX_POINT('',#195660);
#37991=VERTEX_POINT('',#195664);
#37992=VERTEX_POINT('',#195665);
#37993=VERTEX_POINT('',#195670);
#37994=VERTEX_POINT('',#195671);
#37995=VERTEX_POINT('',#195679);
#37996=VERTEX_POINT('',#195680);
#37997=VERTEX_POINT('',#195682);
#37998=VERTEX_POINT('',#195684);
#37999=VERTEX_POINT('',#195688);
#38000=VERTEX_POINT('',#195689);
#38001=VERTEX_POINT('',#195694);
#38002=VERTEX_POINT('',#195695);
#38003=VERTEX_POINT('',#195703);
#38004=VERTEX_POINT('',#195704);
#38005=VERTEX_POINT('',#195706);
#38006=VERTEX_POINT('',#195708);
#38007=VERTEX_POINT('',#195712);
#38008=VERTEX_POINT('',#195713);
#38009=VERTEX_POINT('',#195718);
#38010=VERTEX_POINT('',#195719);
#38011=VERTEX_POINT('',#195727);
#38012=VERTEX_POINT('',#195728);
#38013=VERTEX_POINT('',#195730);
#38014=VERTEX_POINT('',#195732);
#38015=VERTEX_POINT('',#195736);
#38016=VERTEX_POINT('',#195737);
#38017=VERTEX_POINT('',#195742);
#38018=VERTEX_POINT('',#195743);
#38019=VERTEX_POINT('',#195751);
#38020=VERTEX_POINT('',#195752);
#38021=VERTEX_POINT('',#195754);
#38022=VERTEX_POINT('',#195756);
#38023=VERTEX_POINT('',#195760);
#38024=VERTEX_POINT('',#195761);
#38025=VERTEX_POINT('',#195766);
#38026=VERTEX_POINT('',#195767);
#38027=VERTEX_POINT('',#195775);
#38028=VERTEX_POINT('',#195776);
#38029=VERTEX_POINT('',#195778);
#38030=VERTEX_POINT('',#195780);
#38031=VERTEX_POINT('',#195784);
#38032=VERTEX_POINT('',#195785);
#38033=VERTEX_POINT('',#195790);
#38034=VERTEX_POINT('',#195791);
#38035=VERTEX_POINT('',#195799);
#38036=VERTEX_POINT('',#195800);
#38037=VERTEX_POINT('',#195802);
#38038=VERTEX_POINT('',#195804);
#38039=VERTEX_POINT('',#195808);
#38040=VERTEX_POINT('',#195809);
#38041=VERTEX_POINT('',#195814);
#38042=VERTEX_POINT('',#195815);
#38043=VERTEX_POINT('',#195823);
#38044=VERTEX_POINT('',#195824);
#38045=VERTEX_POINT('',#195826);
#38046=VERTEX_POINT('',#195828);
#38047=VERTEX_POINT('',#195832);
#38048=VERTEX_POINT('',#195833);
#38049=VERTEX_POINT('',#195838);
#38050=VERTEX_POINT('',#195839);
#38051=VERTEX_POINT('',#195847);
#38052=VERTEX_POINT('',#195848);
#38053=VERTEX_POINT('',#195850);
#38054=VERTEX_POINT('',#195852);
#38055=VERTEX_POINT('',#195856);
#38056=VERTEX_POINT('',#195857);
#38057=VERTEX_POINT('',#195862);
#38058=VERTEX_POINT('',#195863);
#38059=VERTEX_POINT('',#195871);
#38060=VERTEX_POINT('',#195872);
#38061=VERTEX_POINT('',#195874);
#38062=VERTEX_POINT('',#195876);
#38063=VERTEX_POINT('',#195880);
#38064=VERTEX_POINT('',#195881);
#38065=VERTEX_POINT('',#195886);
#38066=VERTEX_POINT('',#195887);
#38067=VERTEX_POINT('',#195895);
#38068=VERTEX_POINT('',#195896);
#38069=VERTEX_POINT('',#195898);
#38070=VERTEX_POINT('',#195900);
#38071=VERTEX_POINT('',#195904);
#38072=VERTEX_POINT('',#195905);
#38073=VERTEX_POINT('',#195910);
#38074=VERTEX_POINT('',#195911);
#38075=VERTEX_POINT('',#195919);
#38076=VERTEX_POINT('',#195920);
#38077=VERTEX_POINT('',#195922);
#38078=VERTEX_POINT('',#195924);
#38079=VERTEX_POINT('',#195928);
#38080=VERTEX_POINT('',#195929);
#38081=VERTEX_POINT('',#195934);
#38082=VERTEX_POINT('',#195935);
#38083=VERTEX_POINT('',#195943);
#38084=VERTEX_POINT('',#195944);
#38085=VERTEX_POINT('',#195946);
#38086=VERTEX_POINT('',#195948);
#38087=VERTEX_POINT('',#195952);
#38088=VERTEX_POINT('',#195953);
#38089=VERTEX_POINT('',#195958);
#38090=VERTEX_POINT('',#195959);
#38091=VERTEX_POINT('',#195967);
#38092=VERTEX_POINT('',#195968);
#38093=VERTEX_POINT('',#195970);
#38094=VERTEX_POINT('',#195972);
#38095=VERTEX_POINT('',#195976);
#38096=VERTEX_POINT('',#195977);
#38097=VERTEX_POINT('',#195982);
#38098=VERTEX_POINT('',#195983);
#38099=VERTEX_POINT('',#195991);
#38100=VERTEX_POINT('',#195992);
#38101=VERTEX_POINT('',#195994);
#38102=VERTEX_POINT('',#195996);
#38103=VERTEX_POINT('',#196000);
#38104=VERTEX_POINT('',#196001);
#38105=VERTEX_POINT('',#196006);
#38106=VERTEX_POINT('',#196007);
#38107=VERTEX_POINT('',#196015);
#38108=VERTEX_POINT('',#196016);
#38109=VERTEX_POINT('',#196018);
#38110=VERTEX_POINT('',#196020);
#38111=VERTEX_POINT('',#196024);
#38112=VERTEX_POINT('',#196025);
#38113=VERTEX_POINT('',#196030);
#38114=VERTEX_POINT('',#196031);
#38115=VERTEX_POINT('',#196039);
#38116=VERTEX_POINT('',#196040);
#38117=VERTEX_POINT('',#196042);
#38118=VERTEX_POINT('',#196044);
#38119=VERTEX_POINT('',#196048);
#38120=VERTEX_POINT('',#196049);
#38121=VERTEX_POINT('',#196054);
#38122=VERTEX_POINT('',#196055);
#38123=VERTEX_POINT('',#196063);
#38124=VERTEX_POINT('',#196064);
#38125=VERTEX_POINT('',#196066);
#38126=VERTEX_POINT('',#196068);
#38127=VERTEX_POINT('',#196072);
#38128=VERTEX_POINT('',#196073);
#38129=VERTEX_POINT('',#196078);
#38130=VERTEX_POINT('',#196079);
#38131=VERTEX_POINT('',#196087);
#38132=VERTEX_POINT('',#196088);
#38133=VERTEX_POINT('',#196090);
#38134=VERTEX_POINT('',#196092);
#38135=VERTEX_POINT('',#196096);
#38136=VERTEX_POINT('',#196097);
#38137=VERTEX_POINT('',#196102);
#38138=VERTEX_POINT('',#196103);
#38139=VERTEX_POINT('',#196111);
#38140=VERTEX_POINT('',#196112);
#38141=VERTEX_POINT('',#196114);
#38142=VERTEX_POINT('',#196116);
#38143=VERTEX_POINT('',#196120);
#38144=VERTEX_POINT('',#196121);
#38145=VERTEX_POINT('',#196126);
#38146=VERTEX_POINT('',#196127);
#38147=VERTEX_POINT('',#196135);
#38148=VERTEX_POINT('',#196136);
#38149=VERTEX_POINT('',#196138);
#38150=VERTEX_POINT('',#196140);
#38151=VERTEX_POINT('',#196144);
#38152=VERTEX_POINT('',#196145);
#38153=VERTEX_POINT('',#196150);
#38154=VERTEX_POINT('',#196151);
#38155=VERTEX_POINT('',#196159);
#38156=VERTEX_POINT('',#196160);
#38157=VERTEX_POINT('',#196162);
#38158=VERTEX_POINT('',#196164);
#38159=VERTEX_POINT('',#196168);
#38160=VERTEX_POINT('',#196169);
#38161=VERTEX_POINT('',#196174);
#38162=VERTEX_POINT('',#196175);
#38163=VERTEX_POINT('',#196183);
#38164=VERTEX_POINT('',#196184);
#38165=VERTEX_POINT('',#196186);
#38166=VERTEX_POINT('',#196188);
#38167=VERTEX_POINT('',#196192);
#38168=VERTEX_POINT('',#196193);
#38169=VERTEX_POINT('',#196198);
#38170=VERTEX_POINT('',#196199);
#38171=VERTEX_POINT('',#196207);
#38172=VERTEX_POINT('',#196208);
#38173=VERTEX_POINT('',#196210);
#38174=VERTEX_POINT('',#196212);
#38175=VERTEX_POINT('',#196216);
#38176=VERTEX_POINT('',#196217);
#38177=VERTEX_POINT('',#196222);
#38178=VERTEX_POINT('',#196223);
#38179=VERTEX_POINT('',#196231);
#38180=VERTEX_POINT('',#196232);
#38181=VERTEX_POINT('',#196234);
#38182=VERTEX_POINT('',#196236);
#38183=VERTEX_POINT('',#196240);
#38184=VERTEX_POINT('',#196241);
#38185=VERTEX_POINT('',#196246);
#38186=VERTEX_POINT('',#196247);
#38187=VERTEX_POINT('',#196255);
#38188=VERTEX_POINT('',#196256);
#38189=VERTEX_POINT('',#196258);
#38190=VERTEX_POINT('',#196260);
#38191=VERTEX_POINT('',#196264);
#38192=VERTEX_POINT('',#196265);
#38193=VERTEX_POINT('',#196270);
#38194=VERTEX_POINT('',#196271);
#38195=VERTEX_POINT('',#196279);
#38196=VERTEX_POINT('',#196280);
#38197=VERTEX_POINT('',#196282);
#38198=VERTEX_POINT('',#196284);
#38199=VERTEX_POINT('',#196288);
#38200=VERTEX_POINT('',#196289);
#38201=VERTEX_POINT('',#196294);
#38202=VERTEX_POINT('',#196295);
#38203=VERTEX_POINT('',#196303);
#38204=VERTEX_POINT('',#196304);
#38205=VERTEX_POINT('',#196306);
#38206=VERTEX_POINT('',#196308);
#38207=VERTEX_POINT('',#196312);
#38208=VERTEX_POINT('',#196313);
#38209=VERTEX_POINT('',#196318);
#38210=VERTEX_POINT('',#196319);
#38211=VERTEX_POINT('',#196327);
#38212=VERTEX_POINT('',#196328);
#38213=VERTEX_POINT('',#196330);
#38214=VERTEX_POINT('',#196332);
#38215=VERTEX_POINT('',#196336);
#38216=VERTEX_POINT('',#196337);
#38217=VERTEX_POINT('',#196342);
#38218=VERTEX_POINT('',#196343);
#38219=VERTEX_POINT('',#196351);
#38220=VERTEX_POINT('',#196352);
#38221=VERTEX_POINT('',#196354);
#38222=VERTEX_POINT('',#196356);
#38223=VERTEX_POINT('',#196360);
#38224=VERTEX_POINT('',#196361);
#38225=VERTEX_POINT('',#196366);
#38226=VERTEX_POINT('',#196367);
#38227=VERTEX_POINT('',#196375);
#38228=VERTEX_POINT('',#196376);
#38229=VERTEX_POINT('',#196378);
#38230=VERTEX_POINT('',#196380);
#38231=VERTEX_POINT('',#196384);
#38232=VERTEX_POINT('',#196385);
#38233=VERTEX_POINT('',#196390);
#38234=VERTEX_POINT('',#196391);
#38235=VERTEX_POINT('',#196399);
#38236=VERTEX_POINT('',#196400);
#38237=VERTEX_POINT('',#196402);
#38238=VERTEX_POINT('',#196404);
#38239=VERTEX_POINT('',#196408);
#38240=VERTEX_POINT('',#196409);
#38241=VERTEX_POINT('',#196414);
#38242=VERTEX_POINT('',#196415);
#38243=VERTEX_POINT('',#196423);
#38244=VERTEX_POINT('',#196424);
#38245=VERTEX_POINT('',#196426);
#38246=VERTEX_POINT('',#196428);
#38247=VERTEX_POINT('',#196432);
#38248=VERTEX_POINT('',#196433);
#38249=VERTEX_POINT('',#196438);
#38250=VERTEX_POINT('',#196439);
#38251=VERTEX_POINT('',#196447);
#38252=VERTEX_POINT('',#196448);
#38253=VERTEX_POINT('',#196450);
#38254=VERTEX_POINT('',#196452);
#38255=VERTEX_POINT('',#196456);
#38256=VERTEX_POINT('',#196457);
#38257=VERTEX_POINT('',#196462);
#38258=VERTEX_POINT('',#196463);
#38259=VERTEX_POINT('',#196471);
#38260=VERTEX_POINT('',#196472);
#38261=VERTEX_POINT('',#196474);
#38262=VERTEX_POINT('',#196476);
#38263=VERTEX_POINT('',#196480);
#38264=VERTEX_POINT('',#196481);
#38265=VERTEX_POINT('',#196486);
#38266=VERTEX_POINT('',#196487);
#38267=VERTEX_POINT('',#196495);
#38268=VERTEX_POINT('',#196496);
#38269=VERTEX_POINT('',#196498);
#38270=VERTEX_POINT('',#196500);
#38271=VERTEX_POINT('',#196504);
#38272=VERTEX_POINT('',#196505);
#38273=VERTEX_POINT('',#196510);
#38274=VERTEX_POINT('',#196511);
#38275=VERTEX_POINT('',#196519);
#38276=VERTEX_POINT('',#196520);
#38277=VERTEX_POINT('',#196522);
#38278=VERTEX_POINT('',#196524);
#38279=VERTEX_POINT('',#196528);
#38280=VERTEX_POINT('',#196529);
#38281=VERTEX_POINT('',#196534);
#38282=VERTEX_POINT('',#196535);
#38283=VERTEX_POINT('',#196543);
#38284=VERTEX_POINT('',#196544);
#38285=VERTEX_POINT('',#196546);
#38286=VERTEX_POINT('',#196548);
#38287=VERTEX_POINT('',#196552);
#38288=VERTEX_POINT('',#196553);
#38289=VERTEX_POINT('',#196558);
#38290=VERTEX_POINT('',#196559);
#38291=VERTEX_POINT('',#196567);
#38292=VERTEX_POINT('',#196568);
#38293=VERTEX_POINT('',#196570);
#38294=VERTEX_POINT('',#196572);
#38295=VERTEX_POINT('',#196576);
#38296=VERTEX_POINT('',#196577);
#38297=VERTEX_POINT('',#196582);
#38298=VERTEX_POINT('',#196583);
#38299=VERTEX_POINT('',#196591);
#38300=VERTEX_POINT('',#196592);
#38301=VERTEX_POINT('',#196594);
#38302=VERTEX_POINT('',#196596);
#38303=VERTEX_POINT('',#196600);
#38304=VERTEX_POINT('',#196601);
#38305=VERTEX_POINT('',#196606);
#38306=VERTEX_POINT('',#196607);
#38307=VERTEX_POINT('',#196615);
#38308=VERTEX_POINT('',#196616);
#38309=VERTEX_POINT('',#196618);
#38310=VERTEX_POINT('',#196620);
#38311=VERTEX_POINT('',#196624);
#38312=VERTEX_POINT('',#196625);
#38313=VERTEX_POINT('',#196630);
#38314=VERTEX_POINT('',#196631);
#38315=VERTEX_POINT('',#196639);
#38316=VERTEX_POINT('',#196640);
#38317=VERTEX_POINT('',#196642);
#38318=VERTEX_POINT('',#196644);
#38319=VERTEX_POINT('',#196648);
#38320=VERTEX_POINT('',#196649);
#38321=VERTEX_POINT('',#196654);
#38322=VERTEX_POINT('',#196655);
#38323=VERTEX_POINT('',#196663);
#38324=VERTEX_POINT('',#196664);
#38325=VERTEX_POINT('',#196666);
#38326=VERTEX_POINT('',#196668);
#38327=VERTEX_POINT('',#196672);
#38328=VERTEX_POINT('',#196673);
#38329=VERTEX_POINT('',#196678);
#38330=VERTEX_POINT('',#196679);
#38331=VERTEX_POINT('',#196687);
#38332=VERTEX_POINT('',#196688);
#38333=VERTEX_POINT('',#196690);
#38334=VERTEX_POINT('',#196692);
#38335=VERTEX_POINT('',#196696);
#38336=VERTEX_POINT('',#196697);
#38337=VERTEX_POINT('',#196702);
#38338=VERTEX_POINT('',#196703);
#38339=VERTEX_POINT('',#196711);
#38340=VERTEX_POINT('',#196712);
#38341=VERTEX_POINT('',#196714);
#38342=VERTEX_POINT('',#196716);
#38343=VERTEX_POINT('',#196720);
#38344=VERTEX_POINT('',#196721);
#38345=VERTEX_POINT('',#196726);
#38346=VERTEX_POINT('',#196727);
#38347=VERTEX_POINT('',#196735);
#38348=VERTEX_POINT('',#196736);
#38349=VERTEX_POINT('',#196738);
#38350=VERTEX_POINT('',#196740);
#38351=VERTEX_POINT('',#196744);
#38352=VERTEX_POINT('',#196745);
#38353=VERTEX_POINT('',#196750);
#38354=VERTEX_POINT('',#196751);
#38355=VERTEX_POINT('',#196759);
#38356=VERTEX_POINT('',#196760);
#38357=VERTEX_POINT('',#196762);
#38358=VERTEX_POINT('',#196764);
#38359=VERTEX_POINT('',#196768);
#38360=VERTEX_POINT('',#196769);
#38361=VERTEX_POINT('',#196774);
#38362=VERTEX_POINT('',#196775);
#38363=VERTEX_POINT('',#196783);
#38364=VERTEX_POINT('',#196784);
#38365=VERTEX_POINT('',#196786);
#38366=VERTEX_POINT('',#196788);
#38367=VERTEX_POINT('',#196792);
#38368=VERTEX_POINT('',#196793);
#38369=VERTEX_POINT('',#196798);
#38370=VERTEX_POINT('',#196799);
#38371=VERTEX_POINT('',#196807);
#38372=VERTEX_POINT('',#196808);
#38373=VERTEX_POINT('',#196810);
#38374=VERTEX_POINT('',#196812);
#38375=VERTEX_POINT('',#196816);
#38376=VERTEX_POINT('',#196817);
#38377=VERTEX_POINT('',#196822);
#38378=VERTEX_POINT('',#196823);
#38379=VERTEX_POINT('',#196831);
#38380=VERTEX_POINT('',#196832);
#38381=VERTEX_POINT('',#196834);
#38382=VERTEX_POINT('',#196836);
#38383=VERTEX_POINT('',#196840);
#38384=VERTEX_POINT('',#196841);
#38385=VERTEX_POINT('',#196846);
#38386=VERTEX_POINT('',#196847);
#38387=VERTEX_POINT('',#196855);
#38388=VERTEX_POINT('',#196856);
#38389=VERTEX_POINT('',#196858);
#38390=VERTEX_POINT('',#196860);
#38391=VERTEX_POINT('',#196864);
#38392=VERTEX_POINT('',#196865);
#38393=VERTEX_POINT('',#196870);
#38394=VERTEX_POINT('',#196871);
#38395=VERTEX_POINT('',#196879);
#38396=VERTEX_POINT('',#196880);
#38397=VERTEX_POINT('',#196882);
#38398=VERTEX_POINT('',#196884);
#38399=VERTEX_POINT('',#196888);
#38400=VERTEX_POINT('',#196889);
#38401=VERTEX_POINT('',#196894);
#38402=VERTEX_POINT('',#196895);
#38403=VERTEX_POINT('',#196903);
#38404=VERTEX_POINT('',#196904);
#38405=VERTEX_POINT('',#196906);
#38406=VERTEX_POINT('',#196908);
#38407=VERTEX_POINT('',#196912);
#38408=VERTEX_POINT('',#196913);
#38409=VERTEX_POINT('',#196918);
#38410=VERTEX_POINT('',#196919);
#38411=VERTEX_POINT('',#196927);
#38412=VERTEX_POINT('',#196928);
#38413=VERTEX_POINT('',#196930);
#38414=VERTEX_POINT('',#196932);
#38415=VERTEX_POINT('',#196936);
#38416=VERTEX_POINT('',#196937);
#38417=VERTEX_POINT('',#196942);
#38418=VERTEX_POINT('',#196943);
#38419=VERTEX_POINT('',#196951);
#38420=VERTEX_POINT('',#196952);
#38421=VERTEX_POINT('',#196954);
#38422=VERTEX_POINT('',#196956);
#38423=VERTEX_POINT('',#196960);
#38424=VERTEX_POINT('',#196961);
#38425=VERTEX_POINT('',#196966);
#38426=VERTEX_POINT('',#196967);
#38427=VERTEX_POINT('',#196975);
#38428=VERTEX_POINT('',#196976);
#38429=VERTEX_POINT('',#196978);
#38430=VERTEX_POINT('',#196980);
#38431=VERTEX_POINT('',#196984);
#38432=VERTEX_POINT('',#196985);
#38433=VERTEX_POINT('',#196990);
#38434=VERTEX_POINT('',#196991);
#38435=VERTEX_POINT('',#196999);
#38436=VERTEX_POINT('',#197000);
#38437=VERTEX_POINT('',#197002);
#38438=VERTEX_POINT('',#197004);
#38439=VERTEX_POINT('',#197008);
#38440=VERTEX_POINT('',#197009);
#38441=VERTEX_POINT('',#197014);
#38442=VERTEX_POINT('',#197015);
#38443=VERTEX_POINT('',#197023);
#38444=VERTEX_POINT('',#197024);
#38445=VERTEX_POINT('',#197026);
#38446=VERTEX_POINT('',#197028);
#38447=VERTEX_POINT('',#197032);
#38448=VERTEX_POINT('',#197033);
#38449=VERTEX_POINT('',#197038);
#38450=VERTEX_POINT('',#197039);
#38451=VERTEX_POINT('',#197047);
#38452=VERTEX_POINT('',#197048);
#38453=VERTEX_POINT('',#197050);
#38454=VERTEX_POINT('',#197052);
#38455=VERTEX_POINT('',#197056);
#38456=VERTEX_POINT('',#197057);
#38457=VERTEX_POINT('',#197062);
#38458=VERTEX_POINT('',#197063);
#38459=VERTEX_POINT('',#197071);
#38460=VERTEX_POINT('',#197072);
#38461=VERTEX_POINT('',#197074);
#38462=VERTEX_POINT('',#197076);
#38463=VERTEX_POINT('',#197080);
#38464=VERTEX_POINT('',#197081);
#38465=VERTEX_POINT('',#197086);
#38466=VERTEX_POINT('',#197087);
#38467=VERTEX_POINT('',#197095);
#38468=VERTEX_POINT('',#197096);
#38469=VERTEX_POINT('',#197098);
#38470=VERTEX_POINT('',#197100);
#38471=VERTEX_POINT('',#197104);
#38472=VERTEX_POINT('',#197105);
#38473=VERTEX_POINT('',#197110);
#38474=VERTEX_POINT('',#197111);
#38475=VERTEX_POINT('',#197119);
#38476=VERTEX_POINT('',#197120);
#38477=VERTEX_POINT('',#197122);
#38478=VERTEX_POINT('',#197124);
#38479=VERTEX_POINT('',#197128);
#38480=VERTEX_POINT('',#197129);
#38481=VERTEX_POINT('',#197134);
#38482=VERTEX_POINT('',#197135);
#38483=VERTEX_POINT('',#197143);
#38484=VERTEX_POINT('',#197144);
#38485=VERTEX_POINT('',#197146);
#38486=VERTEX_POINT('',#197148);
#38487=VERTEX_POINT('',#197152);
#38488=VERTEX_POINT('',#197153);
#38489=VERTEX_POINT('',#197158);
#38490=VERTEX_POINT('',#197159);
#38491=VERTEX_POINT('',#197167);
#38492=VERTEX_POINT('',#197168);
#38493=VERTEX_POINT('',#197170);
#38494=VERTEX_POINT('',#197172);
#38495=VERTEX_POINT('',#197176);
#38496=VERTEX_POINT('',#197177);
#38497=VERTEX_POINT('',#197182);
#38498=VERTEX_POINT('',#197183);
#38499=VERTEX_POINT('',#197191);
#38500=VERTEX_POINT('',#197192);
#38501=VERTEX_POINT('',#197194);
#38502=VERTEX_POINT('',#197196);
#38503=VERTEX_POINT('',#197200);
#38504=VERTEX_POINT('',#197201);
#38505=VERTEX_POINT('',#197206);
#38506=VERTEX_POINT('',#197207);
#38507=VERTEX_POINT('',#197215);
#38508=VERTEX_POINT('',#197216);
#38509=VERTEX_POINT('',#197218);
#38510=VERTEX_POINT('',#197220);
#38511=VERTEX_POINT('',#197224);
#38512=VERTEX_POINT('',#197225);
#38513=VERTEX_POINT('',#197230);
#38514=VERTEX_POINT('',#197231);
#38515=VERTEX_POINT('',#197239);
#38516=VERTEX_POINT('',#197240);
#38517=VERTEX_POINT('',#197242);
#38518=VERTEX_POINT('',#197244);
#38519=VERTEX_POINT('',#197248);
#38520=VERTEX_POINT('',#197249);
#38521=VERTEX_POINT('',#197254);
#38522=VERTEX_POINT('',#197255);
#38523=VERTEX_POINT('',#197263);
#38524=VERTEX_POINT('',#197264);
#38525=VERTEX_POINT('',#197266);
#38526=VERTEX_POINT('',#197268);
#38527=VERTEX_POINT('',#197272);
#38528=VERTEX_POINT('',#197273);
#38529=VERTEX_POINT('',#197278);
#38530=VERTEX_POINT('',#197279);
#38531=VERTEX_POINT('',#197287);
#38532=VERTEX_POINT('',#197288);
#38533=VERTEX_POINT('',#197290);
#38534=VERTEX_POINT('',#197292);
#38535=VERTEX_POINT('',#197296);
#38536=VERTEX_POINT('',#197297);
#38537=VERTEX_POINT('',#197302);
#38538=VERTEX_POINT('',#197303);
#38539=VERTEX_POINT('',#197311);
#38540=VERTEX_POINT('',#197312);
#38541=VERTEX_POINT('',#197314);
#38542=VERTEX_POINT('',#197316);
#38543=VERTEX_POINT('',#197320);
#38544=VERTEX_POINT('',#197321);
#38545=VERTEX_POINT('',#197326);
#38546=VERTEX_POINT('',#197327);
#38547=VERTEX_POINT('',#197335);
#38548=VERTEX_POINT('',#197336);
#38549=VERTEX_POINT('',#197338);
#38550=VERTEX_POINT('',#197340);
#38551=VERTEX_POINT('',#197344);
#38552=VERTEX_POINT('',#197345);
#38553=VERTEX_POINT('',#197350);
#38554=VERTEX_POINT('',#197351);
#38555=VERTEX_POINT('',#197359);
#38556=VERTEX_POINT('',#197360);
#38557=VERTEX_POINT('',#197362);
#38558=VERTEX_POINT('',#197364);
#38559=VERTEX_POINT('',#197368);
#38560=VERTEX_POINT('',#197369);
#38561=VERTEX_POINT('',#197374);
#38562=VERTEX_POINT('',#197375);
#38563=VERTEX_POINT('',#197383);
#38564=VERTEX_POINT('',#197384);
#38565=VERTEX_POINT('',#197386);
#38566=VERTEX_POINT('',#197388);
#38567=VERTEX_POINT('',#197392);
#38568=VERTEX_POINT('',#197393);
#38569=VERTEX_POINT('',#197398);
#38570=VERTEX_POINT('',#197399);
#38571=VERTEX_POINT('',#197407);
#38572=VERTEX_POINT('',#197408);
#38573=VERTEX_POINT('',#197410);
#38574=VERTEX_POINT('',#197412);
#38575=VERTEX_POINT('',#197416);
#38576=VERTEX_POINT('',#197417);
#38577=VERTEX_POINT('',#197422);
#38578=VERTEX_POINT('',#197423);
#38579=VERTEX_POINT('',#197431);
#38580=VERTEX_POINT('',#197432);
#38581=VERTEX_POINT('',#197434);
#38582=VERTEX_POINT('',#197436);
#38583=VERTEX_POINT('',#197440);
#38584=VERTEX_POINT('',#197441);
#38585=VERTEX_POINT('',#197446);
#38586=VERTEX_POINT('',#197447);
#38587=VERTEX_POINT('',#197455);
#38588=VERTEX_POINT('',#197456);
#38589=VERTEX_POINT('',#197458);
#38590=VERTEX_POINT('',#197460);
#38591=VERTEX_POINT('',#197464);
#38592=VERTEX_POINT('',#197465);
#38593=VERTEX_POINT('',#197470);
#38594=VERTEX_POINT('',#197471);
#38595=VERTEX_POINT('',#197479);
#38596=VERTEX_POINT('',#197480);
#38597=VERTEX_POINT('',#197482);
#38598=VERTEX_POINT('',#197484);
#38599=VERTEX_POINT('',#197488);
#38600=VERTEX_POINT('',#197489);
#38601=VERTEX_POINT('',#197494);
#38602=VERTEX_POINT('',#197495);
#38603=VERTEX_POINT('',#197503);
#38604=VERTEX_POINT('',#197504);
#38605=VERTEX_POINT('',#197506);
#38606=VERTEX_POINT('',#197508);
#38607=VERTEX_POINT('',#197512);
#38608=VERTEX_POINT('',#197513);
#38609=VERTEX_POINT('',#197518);
#38610=VERTEX_POINT('',#197519);
#38611=VERTEX_POINT('',#197527);
#38612=VERTEX_POINT('',#197528);
#38613=VERTEX_POINT('',#197530);
#38614=VERTEX_POINT('',#197532);
#38615=VERTEX_POINT('',#197536);
#38616=VERTEX_POINT('',#197537);
#38617=VERTEX_POINT('',#197542);
#38618=VERTEX_POINT('',#197543);
#38619=VERTEX_POINT('',#197551);
#38620=VERTEX_POINT('',#197552);
#38621=VERTEX_POINT('',#197554);
#38622=VERTEX_POINT('',#197556);
#38623=VERTEX_POINT('',#197560);
#38624=VERTEX_POINT('',#197561);
#38625=VERTEX_POINT('',#197566);
#38626=VERTEX_POINT('',#197567);
#38627=VERTEX_POINT('',#197575);
#38628=VERTEX_POINT('',#197576);
#38629=VERTEX_POINT('',#197578);
#38630=VERTEX_POINT('',#197580);
#38631=VERTEX_POINT('',#197584);
#38632=VERTEX_POINT('',#197585);
#38633=VERTEX_POINT('',#197590);
#38634=VERTEX_POINT('',#197591);
#38635=VERTEX_POINT('',#197599);
#38636=VERTEX_POINT('',#197600);
#38637=VERTEX_POINT('',#197602);
#38638=VERTEX_POINT('',#197604);
#38639=VERTEX_POINT('',#197608);
#38640=VERTEX_POINT('',#197609);
#38641=VERTEX_POINT('',#197614);
#38642=VERTEX_POINT('',#197615);
#38643=VERTEX_POINT('',#197623);
#38644=VERTEX_POINT('',#197624);
#38645=VERTEX_POINT('',#197626);
#38646=VERTEX_POINT('',#197628);
#38647=VERTEX_POINT('',#197632);
#38648=VERTEX_POINT('',#197633);
#38649=VERTEX_POINT('',#197638);
#38650=VERTEX_POINT('',#197639);
#38651=VERTEX_POINT('',#197647);
#38652=VERTEX_POINT('',#197648);
#38653=VERTEX_POINT('',#197650);
#38654=VERTEX_POINT('',#197652);
#38655=VERTEX_POINT('',#197656);
#38656=VERTEX_POINT('',#197657);
#38657=VERTEX_POINT('',#197662);
#38658=VERTEX_POINT('',#197663);
#38659=VERTEX_POINT('',#197671);
#38660=VERTEX_POINT('',#197672);
#38661=VERTEX_POINT('',#197674);
#38662=VERTEX_POINT('',#197676);
#38663=VERTEX_POINT('',#197680);
#38664=VERTEX_POINT('',#197681);
#38665=VERTEX_POINT('',#197686);
#38666=VERTEX_POINT('',#197687);
#38667=VERTEX_POINT('',#197695);
#38668=VERTEX_POINT('',#197696);
#38669=VERTEX_POINT('',#197698);
#38670=VERTEX_POINT('',#197700);
#38671=VERTEX_POINT('',#197704);
#38672=VERTEX_POINT('',#197705);
#38673=VERTEX_POINT('',#197710);
#38674=VERTEX_POINT('',#197711);
#38675=VERTEX_POINT('',#197719);
#38676=VERTEX_POINT('',#197720);
#38677=VERTEX_POINT('',#197722);
#38678=VERTEX_POINT('',#197724);
#38679=VERTEX_POINT('',#197728);
#38680=VERTEX_POINT('',#197729);
#38681=VERTEX_POINT('',#197734);
#38682=VERTEX_POINT('',#197735);
#38683=VERTEX_POINT('',#197743);
#38684=VERTEX_POINT('',#197744);
#38685=VERTEX_POINT('',#197746);
#38686=VERTEX_POINT('',#197748);
#38687=VERTEX_POINT('',#197752);
#38688=VERTEX_POINT('',#197753);
#38689=VERTEX_POINT('',#197758);
#38690=VERTEX_POINT('',#197759);
#38691=VERTEX_POINT('',#197767);
#38692=VERTEX_POINT('',#197768);
#38693=VERTEX_POINT('',#197770);
#38694=VERTEX_POINT('',#197772);
#38695=VERTEX_POINT('',#197776);
#38696=VERTEX_POINT('',#197777);
#38697=VERTEX_POINT('',#197782);
#38698=VERTEX_POINT('',#197783);
#38699=VERTEX_POINT('',#197791);
#38700=VERTEX_POINT('',#197792);
#38701=VERTEX_POINT('',#197794);
#38702=VERTEX_POINT('',#197796);
#38703=VERTEX_POINT('',#197800);
#38704=VERTEX_POINT('',#197801);
#38705=VERTEX_POINT('',#197806);
#38706=VERTEX_POINT('',#197807);
#38707=VERTEX_POINT('',#197815);
#38708=VERTEX_POINT('',#197816);
#38709=VERTEX_POINT('',#197818);
#38710=VERTEX_POINT('',#197820);
#38711=VERTEX_POINT('',#197824);
#38712=VERTEX_POINT('',#197825);
#38713=VERTEX_POINT('',#197830);
#38714=VERTEX_POINT('',#197831);
#38715=VERTEX_POINT('',#197839);
#38716=VERTEX_POINT('',#197840);
#38717=VERTEX_POINT('',#197842);
#38718=VERTEX_POINT('',#197844);
#38719=VERTEX_POINT('',#197848);
#38720=VERTEX_POINT('',#197849);
#38721=VERTEX_POINT('',#197854);
#38722=VERTEX_POINT('',#197855);
#38723=VERTEX_POINT('',#197863);
#38724=VERTEX_POINT('',#197864);
#38725=VERTEX_POINT('',#197866);
#38726=VERTEX_POINT('',#197868);
#38727=VERTEX_POINT('',#197872);
#38728=VERTEX_POINT('',#197873);
#38729=VERTEX_POINT('',#197878);
#38730=VERTEX_POINT('',#197879);
#38731=VERTEX_POINT('',#197887);
#38732=VERTEX_POINT('',#197888);
#38733=VERTEX_POINT('',#197890);
#38734=VERTEX_POINT('',#197892);
#38735=VERTEX_POINT('',#197896);
#38736=VERTEX_POINT('',#197897);
#38737=VERTEX_POINT('',#197902);
#38738=VERTEX_POINT('',#197903);
#38739=VERTEX_POINT('',#197911);
#38740=VERTEX_POINT('',#197912);
#38741=VERTEX_POINT('',#197914);
#38742=VERTEX_POINT('',#197916);
#38743=VERTEX_POINT('',#197920);
#38744=VERTEX_POINT('',#197921);
#38745=VERTEX_POINT('',#197926);
#38746=VERTEX_POINT('',#197927);
#38747=VERTEX_POINT('',#197935);
#38748=VERTEX_POINT('',#197936);
#38749=VERTEX_POINT('',#197938);
#38750=VERTEX_POINT('',#197940);
#38751=VERTEX_POINT('',#197944);
#38752=VERTEX_POINT('',#197945);
#38753=VERTEX_POINT('',#197950);
#38754=VERTEX_POINT('',#197951);
#38755=VERTEX_POINT('',#197959);
#38756=VERTEX_POINT('',#197960);
#38757=VERTEX_POINT('',#197962);
#38758=VERTEX_POINT('',#197964);
#38759=VERTEX_POINT('',#197968);
#38760=VERTEX_POINT('',#197969);
#38761=VERTEX_POINT('',#197974);
#38762=VERTEX_POINT('',#197975);
#38763=VERTEX_POINT('',#197983);
#38764=VERTEX_POINT('',#197984);
#38765=VERTEX_POINT('',#197986);
#38766=VERTEX_POINT('',#197988);
#38767=VERTEX_POINT('',#197992);
#38768=VERTEX_POINT('',#197993);
#38769=VERTEX_POINT('',#197998);
#38770=VERTEX_POINT('',#197999);
#38771=VERTEX_POINT('',#198007);
#38772=VERTEX_POINT('',#198008);
#38773=VERTEX_POINT('',#198010);
#38774=VERTEX_POINT('',#198012);
#38775=VERTEX_POINT('',#198016);
#38776=VERTEX_POINT('',#198017);
#38777=VERTEX_POINT('',#198022);
#38778=VERTEX_POINT('',#198023);
#38779=VERTEX_POINT('',#198031);
#38780=VERTEX_POINT('',#198032);
#38781=VERTEX_POINT('',#198034);
#38782=VERTEX_POINT('',#198036);
#38783=VERTEX_POINT('',#198040);
#38784=VERTEX_POINT('',#198041);
#38785=VERTEX_POINT('',#198046);
#38786=VERTEX_POINT('',#198047);
#38787=VERTEX_POINT('',#198055);
#38788=VERTEX_POINT('',#198056);
#38789=VERTEX_POINT('',#198058);
#38790=VERTEX_POINT('',#198060);
#38791=VERTEX_POINT('',#198064);
#38792=VERTEX_POINT('',#198065);
#38793=VERTEX_POINT('',#198070);
#38794=VERTEX_POINT('',#198071);
#38795=VERTEX_POINT('',#198079);
#38796=VERTEX_POINT('',#198080);
#38797=VERTEX_POINT('',#198082);
#38798=VERTEX_POINT('',#198084);
#38799=VERTEX_POINT('',#198088);
#38800=VERTEX_POINT('',#198089);
#38801=VERTEX_POINT('',#198094);
#38802=VERTEX_POINT('',#198095);
#38803=VERTEX_POINT('',#198103);
#38804=VERTEX_POINT('',#198104);
#38805=VERTEX_POINT('',#198106);
#38806=VERTEX_POINT('',#198108);
#38807=VERTEX_POINT('',#198112);
#38808=VERTEX_POINT('',#198113);
#38809=VERTEX_POINT('',#198118);
#38810=VERTEX_POINT('',#198119);
#38811=VERTEX_POINT('',#198127);
#38812=VERTEX_POINT('',#198128);
#38813=VERTEX_POINT('',#198130);
#38814=VERTEX_POINT('',#198132);
#38815=VERTEX_POINT('',#198136);
#38816=VERTEX_POINT('',#198137);
#38817=VERTEX_POINT('',#198142);
#38818=VERTEX_POINT('',#198143);
#38819=VERTEX_POINT('',#198151);
#38820=VERTEX_POINT('',#198152);
#38821=VERTEX_POINT('',#198154);
#38822=VERTEX_POINT('',#198156);
#38823=VERTEX_POINT('',#198160);
#38824=VERTEX_POINT('',#198161);
#38825=VERTEX_POINT('',#198166);
#38826=VERTEX_POINT('',#198167);
#38827=VERTEX_POINT('',#198175);
#38828=VERTEX_POINT('',#198176);
#38829=VERTEX_POINT('',#198178);
#38830=VERTEX_POINT('',#198180);
#38831=VERTEX_POINT('',#198184);
#38832=VERTEX_POINT('',#198185);
#38833=VERTEX_POINT('',#198190);
#38834=VERTEX_POINT('',#198191);
#38835=VERTEX_POINT('',#198199);
#38836=VERTEX_POINT('',#198200);
#38837=VERTEX_POINT('',#198202);
#38838=VERTEX_POINT('',#198204);
#38839=VERTEX_POINT('',#198208);
#38840=VERTEX_POINT('',#198209);
#38841=VERTEX_POINT('',#198214);
#38842=VERTEX_POINT('',#198215);
#38843=VERTEX_POINT('',#198223);
#38844=VERTEX_POINT('',#198224);
#38845=VERTEX_POINT('',#198226);
#38846=VERTEX_POINT('',#198228);
#38847=VERTEX_POINT('',#198232);
#38848=VERTEX_POINT('',#198233);
#38849=VERTEX_POINT('',#198238);
#38850=VERTEX_POINT('',#198239);
#38851=VERTEX_POINT('',#198247);
#38852=VERTEX_POINT('',#198248);
#38853=VERTEX_POINT('',#198250);
#38854=VERTEX_POINT('',#198252);
#38855=VERTEX_POINT('',#198256);
#38856=VERTEX_POINT('',#198257);
#38857=VERTEX_POINT('',#198262);
#38858=VERTEX_POINT('',#198263);
#38859=VERTEX_POINT('',#198271);
#38860=VERTEX_POINT('',#198272);
#38861=VERTEX_POINT('',#198274);
#38862=VERTEX_POINT('',#198276);
#38863=VERTEX_POINT('',#198280);
#38864=VERTEX_POINT('',#198281);
#38865=VERTEX_POINT('',#198286);
#38866=VERTEX_POINT('',#198287);
#38867=VERTEX_POINT('',#198295);
#38868=VERTEX_POINT('',#198296);
#38869=VERTEX_POINT('',#198298);
#38870=VERTEX_POINT('',#198300);
#38871=VERTEX_POINT('',#198304);
#38872=VERTEX_POINT('',#198305);
#38873=VERTEX_POINT('',#198310);
#38874=VERTEX_POINT('',#198311);
#38875=VERTEX_POINT('',#198319);
#38876=VERTEX_POINT('',#198320);
#38877=VERTEX_POINT('',#198322);
#38878=VERTEX_POINT('',#198324);
#38879=VERTEX_POINT('',#198328);
#38880=VERTEX_POINT('',#198329);
#38881=VERTEX_POINT('',#198334);
#38882=VERTEX_POINT('',#198335);
#38883=VERTEX_POINT('',#198343);
#38884=VERTEX_POINT('',#198344);
#38885=VERTEX_POINT('',#198346);
#38886=VERTEX_POINT('',#198348);
#38887=VERTEX_POINT('',#198352);
#38888=VERTEX_POINT('',#198353);
#38889=VERTEX_POINT('',#198358);
#38890=VERTEX_POINT('',#198359);
#38891=VERTEX_POINT('',#198367);
#38892=VERTEX_POINT('',#198368);
#38893=VERTEX_POINT('',#198370);
#38894=VERTEX_POINT('',#198372);
#38895=VERTEX_POINT('',#198376);
#38896=VERTEX_POINT('',#198377);
#38897=VERTEX_POINT('',#198382);
#38898=VERTEX_POINT('',#198383);
#38899=VERTEX_POINT('',#198391);
#38900=VERTEX_POINT('',#198392);
#38901=VERTEX_POINT('',#198394);
#38902=VERTEX_POINT('',#198396);
#38903=VERTEX_POINT('',#198400);
#38904=VERTEX_POINT('',#198401);
#38905=VERTEX_POINT('',#198406);
#38906=VERTEX_POINT('',#198407);
#38907=VERTEX_POINT('',#198415);
#38908=VERTEX_POINT('',#198416);
#38909=VERTEX_POINT('',#198418);
#38910=VERTEX_POINT('',#198420);
#38911=VERTEX_POINT('',#198424);
#38912=VERTEX_POINT('',#198425);
#38913=VERTEX_POINT('',#198430);
#38914=VERTEX_POINT('',#198431);
#38915=VERTEX_POINT('',#198439);
#38916=VERTEX_POINT('',#198440);
#38917=VERTEX_POINT('',#198442);
#38918=VERTEX_POINT('',#198444);
#38919=VERTEX_POINT('',#198448);
#38920=VERTEX_POINT('',#198449);
#38921=VERTEX_POINT('',#198454);
#38922=VERTEX_POINT('',#198455);
#38923=VERTEX_POINT('',#198463);
#38924=VERTEX_POINT('',#198464);
#38925=VERTEX_POINT('',#198466);
#38926=VERTEX_POINT('',#198468);
#38927=VERTEX_POINT('',#198472);
#38928=VERTEX_POINT('',#198473);
#38929=VERTEX_POINT('',#198478);
#38930=VERTEX_POINT('',#198479);
#38931=VERTEX_POINT('',#198487);
#38932=VERTEX_POINT('',#198488);
#38933=VERTEX_POINT('',#198490);
#38934=VERTEX_POINT('',#198492);
#38935=VERTEX_POINT('',#198496);
#38936=VERTEX_POINT('',#198497);
#38937=VERTEX_POINT('',#198502);
#38938=VERTEX_POINT('',#198503);
#38939=VERTEX_POINT('',#198511);
#38940=VERTEX_POINT('',#198512);
#38941=VERTEX_POINT('',#198514);
#38942=VERTEX_POINT('',#198516);
#38943=VERTEX_POINT('',#198520);
#38944=VERTEX_POINT('',#198521);
#38945=VERTEX_POINT('',#198526);
#38946=VERTEX_POINT('',#198527);
#38947=VERTEX_POINT('',#198535);
#38948=VERTEX_POINT('',#198536);
#38949=VERTEX_POINT('',#198538);
#38950=VERTEX_POINT('',#198540);
#38951=VERTEX_POINT('',#198544);
#38952=VERTEX_POINT('',#198545);
#38953=VERTEX_POINT('',#198550);
#38954=VERTEX_POINT('',#198551);
#38955=VERTEX_POINT('',#198559);
#38956=VERTEX_POINT('',#198560);
#38957=VERTEX_POINT('',#198562);
#38958=VERTEX_POINT('',#198564);
#38959=VERTEX_POINT('',#198568);
#38960=VERTEX_POINT('',#198569);
#38961=VERTEX_POINT('',#198574);
#38962=VERTEX_POINT('',#198575);
#38963=VERTEX_POINT('',#198583);
#38964=VERTEX_POINT('',#198584);
#38965=VERTEX_POINT('',#198586);
#38966=VERTEX_POINT('',#198588);
#38967=VERTEX_POINT('',#198592);
#38968=VERTEX_POINT('',#198593);
#38969=VERTEX_POINT('',#198598);
#38970=VERTEX_POINT('',#198599);
#38971=VERTEX_POINT('',#198607);
#38972=VERTEX_POINT('',#198608);
#38973=VERTEX_POINT('',#198610);
#38974=VERTEX_POINT('',#198612);
#38975=VERTEX_POINT('',#198616);
#38976=VERTEX_POINT('',#198617);
#38977=VERTEX_POINT('',#198622);
#38978=VERTEX_POINT('',#198623);
#38979=VERTEX_POINT('',#198631);
#38980=VERTEX_POINT('',#198632);
#38981=VERTEX_POINT('',#198634);
#38982=VERTEX_POINT('',#198636);
#38983=VERTEX_POINT('',#198640);
#38984=VERTEX_POINT('',#198641);
#38985=VERTEX_POINT('',#198646);
#38986=VERTEX_POINT('',#198647);
#38987=VERTEX_POINT('',#198655);
#38988=VERTEX_POINT('',#198656);
#38989=VERTEX_POINT('',#198658);
#38990=VERTEX_POINT('',#198660);
#38991=VERTEX_POINT('',#198664);
#38992=VERTEX_POINT('',#198665);
#38993=VERTEX_POINT('',#198670);
#38994=VERTEX_POINT('',#198671);
#38995=VERTEX_POINT('',#198679);
#38996=VERTEX_POINT('',#198680);
#38997=VERTEX_POINT('',#198682);
#38998=VERTEX_POINT('',#198684);
#38999=VERTEX_POINT('',#198688);
#39000=VERTEX_POINT('',#198689);
#39001=VERTEX_POINT('',#198694);
#39002=VERTEX_POINT('',#198695);
#39003=VERTEX_POINT('',#198703);
#39004=VERTEX_POINT('',#198704);
#39005=VERTEX_POINT('',#198706);
#39006=VERTEX_POINT('',#198708);
#39007=VERTEX_POINT('',#198712);
#39008=VERTEX_POINT('',#198713);
#39009=VERTEX_POINT('',#198718);
#39010=VERTEX_POINT('',#198719);
#39011=VERTEX_POINT('',#198727);
#39012=VERTEX_POINT('',#198728);
#39013=VERTEX_POINT('',#198730);
#39014=VERTEX_POINT('',#198732);
#39015=VERTEX_POINT('',#198736);
#39016=VERTEX_POINT('',#198737);
#39017=VERTEX_POINT('',#198742);
#39018=VERTEX_POINT('',#198743);
#39019=VERTEX_POINT('',#198751);
#39020=VERTEX_POINT('',#198752);
#39021=VERTEX_POINT('',#198754);
#39022=VERTEX_POINT('',#198756);
#39023=VERTEX_POINT('',#198760);
#39024=VERTEX_POINT('',#198761);
#39025=VERTEX_POINT('',#198766);
#39026=VERTEX_POINT('',#198767);
#39027=VERTEX_POINT('',#198775);
#39028=VERTEX_POINT('',#198776);
#39029=VERTEX_POINT('',#198778);
#39030=VERTEX_POINT('',#198780);
#39031=VERTEX_POINT('',#198784);
#39032=VERTEX_POINT('',#198785);
#39033=VERTEX_POINT('',#198790);
#39034=VERTEX_POINT('',#198791);
#39035=VERTEX_POINT('',#198799);
#39036=VERTEX_POINT('',#198800);
#39037=VERTEX_POINT('',#198802);
#39038=VERTEX_POINT('',#198804);
#39039=VERTEX_POINT('',#198808);
#39040=VERTEX_POINT('',#198809);
#39041=VERTEX_POINT('',#198814);
#39042=VERTEX_POINT('',#198815);
#39043=VERTEX_POINT('',#198823);
#39044=VERTEX_POINT('',#198824);
#39045=VERTEX_POINT('',#198826);
#39046=VERTEX_POINT('',#198828);
#39047=VERTEX_POINT('',#198832);
#39048=VERTEX_POINT('',#198833);
#39049=VERTEX_POINT('',#198838);
#39050=VERTEX_POINT('',#198839);
#39051=VERTEX_POINT('',#198847);
#39052=VERTEX_POINT('',#198848);
#39053=VERTEX_POINT('',#198850);
#39054=VERTEX_POINT('',#198852);
#39055=VERTEX_POINT('',#198856);
#39056=VERTEX_POINT('',#198857);
#39057=VERTEX_POINT('',#198862);
#39058=VERTEX_POINT('',#198863);
#39059=VERTEX_POINT('',#198871);
#39060=VERTEX_POINT('',#198872);
#39061=VERTEX_POINT('',#198874);
#39062=VERTEX_POINT('',#198876);
#39063=VERTEX_POINT('',#198880);
#39064=VERTEX_POINT('',#198881);
#39065=VERTEX_POINT('',#198886);
#39066=VERTEX_POINT('',#198887);
#39067=VERTEX_POINT('',#198895);
#39068=VERTEX_POINT('',#198896);
#39069=VERTEX_POINT('',#198898);
#39070=VERTEX_POINT('',#198900);
#39071=VERTEX_POINT('',#198904);
#39072=VERTEX_POINT('',#198905);
#39073=VERTEX_POINT('',#198910);
#39074=VERTEX_POINT('',#198911);
#39075=VERTEX_POINT('',#198919);
#39076=VERTEX_POINT('',#198920);
#39077=VERTEX_POINT('',#198922);
#39078=VERTEX_POINT('',#198924);
#39079=VERTEX_POINT('',#198928);
#39080=VERTEX_POINT('',#198929);
#39081=VERTEX_POINT('',#198934);
#39082=VERTEX_POINT('',#198935);
#39083=VERTEX_POINT('',#198943);
#39084=VERTEX_POINT('',#198944);
#39085=VERTEX_POINT('',#198946);
#39086=VERTEX_POINT('',#198948);
#39087=VERTEX_POINT('',#198952);
#39088=VERTEX_POINT('',#198953);
#39089=VERTEX_POINT('',#198958);
#39090=VERTEX_POINT('',#198959);
#39091=VERTEX_POINT('',#198967);
#39092=VERTEX_POINT('',#198968);
#39093=VERTEX_POINT('',#198970);
#39094=VERTEX_POINT('',#198972);
#39095=VERTEX_POINT('',#198976);
#39096=VERTEX_POINT('',#198977);
#39097=VERTEX_POINT('',#198982);
#39098=VERTEX_POINT('',#198983);
#39099=VERTEX_POINT('',#198991);
#39100=VERTEX_POINT('',#198992);
#39101=VERTEX_POINT('',#198994);
#39102=VERTEX_POINT('',#198996);
#39103=VERTEX_POINT('',#199000);
#39104=VERTEX_POINT('',#199001);
#39105=VERTEX_POINT('',#199006);
#39106=VERTEX_POINT('',#199007);
#39107=VERTEX_POINT('',#199015);
#39108=VERTEX_POINT('',#199016);
#39109=VERTEX_POINT('',#199018);
#39110=VERTEX_POINT('',#199020);
#39111=VERTEX_POINT('',#199024);
#39112=VERTEX_POINT('',#199025);
#39113=VERTEX_POINT('',#199030);
#39114=VERTEX_POINT('',#199031);
#39115=VERTEX_POINT('',#199039);
#39116=VERTEX_POINT('',#199040);
#39117=VERTEX_POINT('',#199042);
#39118=VERTEX_POINT('',#199044);
#39119=VERTEX_POINT('',#199048);
#39120=VERTEX_POINT('',#199049);
#39121=VERTEX_POINT('',#199054);
#39122=VERTEX_POINT('',#199055);
#39123=VERTEX_POINT('',#199063);
#39124=VERTEX_POINT('',#199064);
#39125=VERTEX_POINT('',#199066);
#39126=VERTEX_POINT('',#199068);
#39127=VERTEX_POINT('',#199072);
#39128=VERTEX_POINT('',#199073);
#39129=VERTEX_POINT('',#199078);
#39130=VERTEX_POINT('',#199079);
#39131=VERTEX_POINT('',#199087);
#39132=VERTEX_POINT('',#199088);
#39133=VERTEX_POINT('',#199090);
#39134=VERTEX_POINT('',#199092);
#39135=VERTEX_POINT('',#199096);
#39136=VERTEX_POINT('',#199097);
#39137=VERTEX_POINT('',#199102);
#39138=VERTEX_POINT('',#199103);
#39139=VERTEX_POINT('',#199111);
#39140=VERTEX_POINT('',#199112);
#39141=VERTEX_POINT('',#199114);
#39142=VERTEX_POINT('',#199116);
#39143=VERTEX_POINT('',#199120);
#39144=VERTEX_POINT('',#199121);
#39145=VERTEX_POINT('',#199126);
#39146=VERTEX_POINT('',#199127);
#39147=VERTEX_POINT('',#199135);
#39148=VERTEX_POINT('',#199136);
#39149=VERTEX_POINT('',#199138);
#39150=VERTEX_POINT('',#199140);
#39151=VERTEX_POINT('',#199144);
#39152=VERTEX_POINT('',#199145);
#39153=VERTEX_POINT('',#199150);
#39154=VERTEX_POINT('',#199151);
#39155=VERTEX_POINT('',#199159);
#39156=VERTEX_POINT('',#199160);
#39157=VERTEX_POINT('',#199162);
#39158=VERTEX_POINT('',#199164);
#39159=VERTEX_POINT('',#199168);
#39160=VERTEX_POINT('',#199169);
#39161=VERTEX_POINT('',#199174);
#39162=VERTEX_POINT('',#199175);
#39163=VERTEX_POINT('',#199183);
#39164=VERTEX_POINT('',#199184);
#39165=VERTEX_POINT('',#199186);
#39166=VERTEX_POINT('',#199188);
#39167=VERTEX_POINT('',#199192);
#39168=VERTEX_POINT('',#199193);
#39169=VERTEX_POINT('',#199198);
#39170=VERTEX_POINT('',#199199);
#39171=VERTEX_POINT('',#199207);
#39172=VERTEX_POINT('',#199208);
#39173=VERTEX_POINT('',#199210);
#39174=VERTEX_POINT('',#199212);
#39175=VERTEX_POINT('',#199216);
#39176=VERTEX_POINT('',#199217);
#39177=VERTEX_POINT('',#199222);
#39178=VERTEX_POINT('',#199223);
#39179=VERTEX_POINT('',#199231);
#39180=VERTEX_POINT('',#199232);
#39181=VERTEX_POINT('',#199234);
#39182=VERTEX_POINT('',#199236);
#39183=VERTEX_POINT('',#199240);
#39184=VERTEX_POINT('',#199241);
#39185=VERTEX_POINT('',#199246);
#39186=VERTEX_POINT('',#199247);
#39187=VERTEX_POINT('',#199255);
#39188=VERTEX_POINT('',#199256);
#39189=VERTEX_POINT('',#199258);
#39190=VERTEX_POINT('',#199260);
#39191=VERTEX_POINT('',#199264);
#39192=VERTEX_POINT('',#199265);
#39193=VERTEX_POINT('',#199270);
#39194=VERTEX_POINT('',#199271);
#39195=VERTEX_POINT('',#199279);
#39196=VERTEX_POINT('',#199280);
#39197=VERTEX_POINT('',#199282);
#39198=VERTEX_POINT('',#199284);
#39199=VERTEX_POINT('',#199288);
#39200=VERTEX_POINT('',#199289);
#39201=VERTEX_POINT('',#199294);
#39202=VERTEX_POINT('',#199295);
#39203=VERTEX_POINT('',#199303);
#39204=VERTEX_POINT('',#199304);
#39205=VERTEX_POINT('',#199306);
#39206=VERTEX_POINT('',#199308);
#39207=VERTEX_POINT('',#199312);
#39208=VERTEX_POINT('',#199313);
#39209=VERTEX_POINT('',#199318);
#39210=VERTEX_POINT('',#199319);
#39211=VERTEX_POINT('',#199327);
#39212=VERTEX_POINT('',#199328);
#39213=VERTEX_POINT('',#199330);
#39214=VERTEX_POINT('',#199332);
#39215=VERTEX_POINT('',#199336);
#39216=VERTEX_POINT('',#199337);
#39217=VERTEX_POINT('',#199342);
#39218=VERTEX_POINT('',#199343);
#39219=VERTEX_POINT('',#199351);
#39220=VERTEX_POINT('',#199352);
#39221=VERTEX_POINT('',#199354);
#39222=VERTEX_POINT('',#199356);
#39223=VERTEX_POINT('',#199360);
#39224=VERTEX_POINT('',#199361);
#39225=VERTEX_POINT('',#199366);
#39226=VERTEX_POINT('',#199367);
#39227=VERTEX_POINT('',#199375);
#39228=VERTEX_POINT('',#199376);
#39229=VERTEX_POINT('',#199378);
#39230=VERTEX_POINT('',#199380);
#39231=VERTEX_POINT('',#199384);
#39232=VERTEX_POINT('',#199385);
#39233=VERTEX_POINT('',#199390);
#39234=VERTEX_POINT('',#199391);
#39235=VERTEX_POINT('',#199399);
#39236=VERTEX_POINT('',#199400);
#39237=VERTEX_POINT('',#199402);
#39238=VERTEX_POINT('',#199404);
#39239=VERTEX_POINT('',#199408);
#39240=VERTEX_POINT('',#199409);
#39241=VERTEX_POINT('',#199414);
#39242=VERTEX_POINT('',#199415);
#39243=VERTEX_POINT('',#199423);
#39244=VERTEX_POINT('',#199424);
#39245=VERTEX_POINT('',#199426);
#39246=VERTEX_POINT('',#199428);
#39247=VERTEX_POINT('',#199432);
#39248=VERTEX_POINT('',#199433);
#39249=VERTEX_POINT('',#199438);
#39250=VERTEX_POINT('',#199439);
#39251=VERTEX_POINT('',#199447);
#39252=VERTEX_POINT('',#199448);
#39253=VERTEX_POINT('',#199450);
#39254=VERTEX_POINT('',#199452);
#39255=VERTEX_POINT('',#199456);
#39256=VERTEX_POINT('',#199457);
#39257=VERTEX_POINT('',#199462);
#39258=VERTEX_POINT('',#199463);
#39259=VERTEX_POINT('',#199471);
#39260=VERTEX_POINT('',#199472);
#39261=VERTEX_POINT('',#199474);
#39262=VERTEX_POINT('',#199476);
#39263=VERTEX_POINT('',#199480);
#39264=VERTEX_POINT('',#199481);
#39265=VERTEX_POINT('',#199486);
#39266=VERTEX_POINT('',#199487);
#39267=VERTEX_POINT('',#199495);
#39268=VERTEX_POINT('',#199496);
#39269=VERTEX_POINT('',#199498);
#39270=VERTEX_POINT('',#199500);
#39271=VERTEX_POINT('',#199504);
#39272=VERTEX_POINT('',#199505);
#39273=VERTEX_POINT('',#199510);
#39274=VERTEX_POINT('',#199511);
#39275=VERTEX_POINT('',#199519);
#39276=VERTEX_POINT('',#199520);
#39277=VERTEX_POINT('',#199522);
#39278=VERTEX_POINT('',#199524);
#39279=VERTEX_POINT('',#199528);
#39280=VERTEX_POINT('',#199529);
#39281=VERTEX_POINT('',#199534);
#39282=VERTEX_POINT('',#199535);
#39283=VERTEX_POINT('',#199543);
#39284=VERTEX_POINT('',#199544);
#39285=VERTEX_POINT('',#199546);
#39286=VERTEX_POINT('',#199548);
#39287=VERTEX_POINT('',#199552);
#39288=VERTEX_POINT('',#199553);
#39289=VERTEX_POINT('',#199558);
#39290=VERTEX_POINT('',#199559);
#39291=VERTEX_POINT('',#199567);
#39292=VERTEX_POINT('',#199568);
#39293=VERTEX_POINT('',#199570);
#39294=VERTEX_POINT('',#199572);
#39295=VERTEX_POINT('',#199576);
#39296=VERTEX_POINT('',#199577);
#39297=VERTEX_POINT('',#199582);
#39298=VERTEX_POINT('',#199583);
#39299=VERTEX_POINT('',#199591);
#39300=VERTEX_POINT('',#199592);
#39301=VERTEX_POINT('',#199594);
#39302=VERTEX_POINT('',#199596);
#39303=VERTEX_POINT('',#199600);
#39304=VERTEX_POINT('',#199601);
#39305=VERTEX_POINT('',#199606);
#39306=VERTEX_POINT('',#199607);
#39307=VERTEX_POINT('',#199615);
#39308=VERTEX_POINT('',#199616);
#39309=VERTEX_POINT('',#199618);
#39310=VERTEX_POINT('',#199620);
#39311=VERTEX_POINT('',#199624);
#39312=VERTEX_POINT('',#199625);
#39313=VERTEX_POINT('',#199630);
#39314=VERTEX_POINT('',#199631);
#39315=VERTEX_POINT('',#199639);
#39316=VERTEX_POINT('',#199640);
#39317=VERTEX_POINT('',#199642);
#39318=VERTEX_POINT('',#199644);
#39319=VERTEX_POINT('',#199648);
#39320=VERTEX_POINT('',#199649);
#39321=VERTEX_POINT('',#199654);
#39322=VERTEX_POINT('',#199655);
#39323=VERTEX_POINT('',#199663);
#39324=VERTEX_POINT('',#199664);
#39325=VERTEX_POINT('',#199666);
#39326=VERTEX_POINT('',#199668);
#39327=VERTEX_POINT('',#199672);
#39328=VERTEX_POINT('',#199673);
#39329=VERTEX_POINT('',#199678);
#39330=VERTEX_POINT('',#199679);
#39331=VERTEX_POINT('',#199687);
#39332=VERTEX_POINT('',#199688);
#39333=VERTEX_POINT('',#199690);
#39334=VERTEX_POINT('',#199692);
#39335=VERTEX_POINT('',#199696);
#39336=VERTEX_POINT('',#199697);
#39337=VERTEX_POINT('',#199702);
#39338=VERTEX_POINT('',#199703);
#39339=VERTEX_POINT('',#199711);
#39340=VERTEX_POINT('',#199712);
#39341=VERTEX_POINT('',#199714);
#39342=VERTEX_POINT('',#199716);
#39343=VERTEX_POINT('',#199720);
#39344=VERTEX_POINT('',#199721);
#39345=VERTEX_POINT('',#199726);
#39346=VERTEX_POINT('',#199727);
#39347=VERTEX_POINT('',#199735);
#39348=VERTEX_POINT('',#199736);
#39349=VERTEX_POINT('',#199738);
#39350=VERTEX_POINT('',#199740);
#39351=VERTEX_POINT('',#199744);
#39352=VERTEX_POINT('',#199745);
#39353=VERTEX_POINT('',#199750);
#39354=VERTEX_POINT('',#199751);
#39355=VERTEX_POINT('',#199759);
#39356=VERTEX_POINT('',#199760);
#39357=VERTEX_POINT('',#199762);
#39358=VERTEX_POINT('',#199764);
#39359=VERTEX_POINT('',#199768);
#39360=VERTEX_POINT('',#199769);
#39361=VERTEX_POINT('',#199774);
#39362=VERTEX_POINT('',#199775);
#39363=VERTEX_POINT('',#199783);
#39364=VERTEX_POINT('',#199784);
#39365=VERTEX_POINT('',#199786);
#39366=VERTEX_POINT('',#199788);
#39367=VERTEX_POINT('',#199792);
#39368=VERTEX_POINT('',#199793);
#39369=VERTEX_POINT('',#199798);
#39370=VERTEX_POINT('',#199799);
#39371=VERTEX_POINT('',#199807);
#39372=VERTEX_POINT('',#199808);
#39373=VERTEX_POINT('',#199810);
#39374=VERTEX_POINT('',#199812);
#39375=VERTEX_POINT('',#199816);
#39376=VERTEX_POINT('',#199817);
#39377=VERTEX_POINT('',#199822);
#39378=VERTEX_POINT('',#199823);
#39379=VERTEX_POINT('',#199831);
#39380=VERTEX_POINT('',#199832);
#39381=VERTEX_POINT('',#199834);
#39382=VERTEX_POINT('',#199836);
#39383=VERTEX_POINT('',#199840);
#39384=VERTEX_POINT('',#199841);
#39385=VERTEX_POINT('',#199846);
#39386=VERTEX_POINT('',#199847);
#39387=VERTEX_POINT('',#199855);
#39388=VERTEX_POINT('',#199856);
#39389=VERTEX_POINT('',#199858);
#39390=VERTEX_POINT('',#199860);
#39391=VERTEX_POINT('',#199864);
#39392=VERTEX_POINT('',#199865);
#39393=VERTEX_POINT('',#199870);
#39394=VERTEX_POINT('',#199871);
#39395=VERTEX_POINT('',#199879);
#39396=VERTEX_POINT('',#199880);
#39397=VERTEX_POINT('',#199882);
#39398=VERTEX_POINT('',#199884);
#39399=VERTEX_POINT('',#199888);
#39400=VERTEX_POINT('',#199889);
#39401=VERTEX_POINT('',#199894);
#39402=VERTEX_POINT('',#199895);
#39403=VERTEX_POINT('',#199903);
#39404=VERTEX_POINT('',#199904);
#39405=VERTEX_POINT('',#199906);
#39406=VERTEX_POINT('',#199908);
#39407=VERTEX_POINT('',#199912);
#39408=VERTEX_POINT('',#199913);
#39409=VERTEX_POINT('',#199918);
#39410=VERTEX_POINT('',#199919);
#39411=VERTEX_POINT('',#199927);
#39412=VERTEX_POINT('',#199928);
#39413=VERTEX_POINT('',#199930);
#39414=VERTEX_POINT('',#199932);
#39415=VERTEX_POINT('',#199936);
#39416=VERTEX_POINT('',#199937);
#39417=VERTEX_POINT('',#199942);
#39418=VERTEX_POINT('',#199943);
#39419=VERTEX_POINT('',#199951);
#39420=VERTEX_POINT('',#199952);
#39421=VERTEX_POINT('',#199954);
#39422=VERTEX_POINT('',#199956);
#39423=VERTEX_POINT('',#199960);
#39424=VERTEX_POINT('',#199961);
#39425=VERTEX_POINT('',#199966);
#39426=VERTEX_POINT('',#199967);
#39427=VERTEX_POINT('',#199975);
#39428=VERTEX_POINT('',#199976);
#39429=VERTEX_POINT('',#199978);
#39430=VERTEX_POINT('',#199980);
#39431=VERTEX_POINT('',#199984);
#39432=VERTEX_POINT('',#199985);
#39433=VERTEX_POINT('',#199990);
#39434=VERTEX_POINT('',#199991);
#39435=VERTEX_POINT('',#199999);
#39436=VERTEX_POINT('',#200000);
#39437=VERTEX_POINT('',#200002);
#39438=VERTEX_POINT('',#200004);
#39439=VERTEX_POINT('',#200008);
#39440=VERTEX_POINT('',#200009);
#39441=VERTEX_POINT('',#200014);
#39442=VERTEX_POINT('',#200015);
#39443=VERTEX_POINT('',#200023);
#39444=VERTEX_POINT('',#200024);
#39445=VERTEX_POINT('',#200026);
#39446=VERTEX_POINT('',#200028);
#39447=VERTEX_POINT('',#200032);
#39448=VERTEX_POINT('',#200033);
#39449=VERTEX_POINT('',#200038);
#39450=VERTEX_POINT('',#200039);
#39451=VERTEX_POINT('',#200047);
#39452=VERTEX_POINT('',#200048);
#39453=VERTEX_POINT('',#200050);
#39454=VERTEX_POINT('',#200052);
#39455=VERTEX_POINT('',#200056);
#39456=VERTEX_POINT('',#200057);
#39457=VERTEX_POINT('',#200062);
#39458=VERTEX_POINT('',#200063);
#39459=VERTEX_POINT('',#200071);
#39460=VERTEX_POINT('',#200072);
#39461=VERTEX_POINT('',#200074);
#39462=VERTEX_POINT('',#200076);
#39463=VERTEX_POINT('',#200080);
#39464=VERTEX_POINT('',#200081);
#39465=VERTEX_POINT('',#200086);
#39466=VERTEX_POINT('',#200087);
#39467=VERTEX_POINT('',#200095);
#39468=VERTEX_POINT('',#200096);
#39469=VERTEX_POINT('',#200098);
#39470=VERTEX_POINT('',#200100);
#39471=VERTEX_POINT('',#200104);
#39472=VERTEX_POINT('',#200105);
#39473=VERTEX_POINT('',#200110);
#39474=VERTEX_POINT('',#200111);
#39475=VERTEX_POINT('',#200119);
#39476=VERTEX_POINT('',#200120);
#39477=VERTEX_POINT('',#200122);
#39478=VERTEX_POINT('',#200124);
#39479=VERTEX_POINT('',#200128);
#39480=VERTEX_POINT('',#200129);
#39481=VERTEX_POINT('',#200134);
#39482=VERTEX_POINT('',#200135);
#39483=VERTEX_POINT('',#200143);
#39484=VERTEX_POINT('',#200144);
#39485=VERTEX_POINT('',#200146);
#39486=VERTEX_POINT('',#200148);
#39487=VERTEX_POINT('',#200152);
#39488=VERTEX_POINT('',#200153);
#39489=VERTEX_POINT('',#200158);
#39490=VERTEX_POINT('',#200159);
#39491=VERTEX_POINT('',#200167);
#39492=VERTEX_POINT('',#200168);
#39493=VERTEX_POINT('',#200170);
#39494=VERTEX_POINT('',#200172);
#39495=VERTEX_POINT('',#200176);
#39496=VERTEX_POINT('',#200177);
#39497=VERTEX_POINT('',#200182);
#39498=VERTEX_POINT('',#200183);
#39499=VERTEX_POINT('',#200191);
#39500=VERTEX_POINT('',#200192);
#39501=VERTEX_POINT('',#200194);
#39502=VERTEX_POINT('',#200196);
#39503=VERTEX_POINT('',#200200);
#39504=VERTEX_POINT('',#200201);
#39505=VERTEX_POINT('',#200206);
#39506=VERTEX_POINT('',#200207);
#39507=VERTEX_POINT('',#200215);
#39508=VERTEX_POINT('',#200216);
#39509=VERTEX_POINT('',#200218);
#39510=VERTEX_POINT('',#200220);
#39511=VERTEX_POINT('',#200224);
#39512=VERTEX_POINT('',#200225);
#39513=VERTEX_POINT('',#200230);
#39514=VERTEX_POINT('',#200231);
#39515=VERTEX_POINT('',#200239);
#39516=VERTEX_POINT('',#200240);
#39517=VERTEX_POINT('',#200242);
#39518=VERTEX_POINT('',#200244);
#39519=VERTEX_POINT('',#200248);
#39520=VERTEX_POINT('',#200249);
#39521=VERTEX_POINT('',#200254);
#39522=VERTEX_POINT('',#200255);
#39523=VERTEX_POINT('',#200263);
#39524=VERTEX_POINT('',#200264);
#39525=VERTEX_POINT('',#200266);
#39526=VERTEX_POINT('',#200268);
#39527=VERTEX_POINT('',#200272);
#39528=VERTEX_POINT('',#200273);
#39529=VERTEX_POINT('',#200278);
#39530=VERTEX_POINT('',#200279);
#39531=VERTEX_POINT('',#200287);
#39532=VERTEX_POINT('',#200288);
#39533=VERTEX_POINT('',#200290);
#39534=VERTEX_POINT('',#200292);
#39535=VERTEX_POINT('',#200296);
#39536=VERTEX_POINT('',#200297);
#39537=VERTEX_POINT('',#200302);
#39538=VERTEX_POINT('',#200303);
#39539=VERTEX_POINT('',#200311);
#39540=VERTEX_POINT('',#200312);
#39541=VERTEX_POINT('',#200314);
#39542=VERTEX_POINT('',#200316);
#39543=VERTEX_POINT('',#200320);
#39544=VERTEX_POINT('',#200321);
#39545=VERTEX_POINT('',#200326);
#39546=VERTEX_POINT('',#200327);
#39547=VERTEX_POINT('',#200335);
#39548=VERTEX_POINT('',#200336);
#39549=VERTEX_POINT('',#200338);
#39550=VERTEX_POINT('',#200340);
#39551=VERTEX_POINT('',#200344);
#39552=VERTEX_POINT('',#200345);
#39553=VERTEX_POINT('',#200350);
#39554=VERTEX_POINT('',#200351);
#39555=VERTEX_POINT('',#200359);
#39556=VERTEX_POINT('',#200360);
#39557=VERTEX_POINT('',#200362);
#39558=VERTEX_POINT('',#200364);
#39559=VERTEX_POINT('',#200368);
#39560=VERTEX_POINT('',#200369);
#39561=VERTEX_POINT('',#200374);
#39562=VERTEX_POINT('',#200375);
#39563=VERTEX_POINT('',#200383);
#39564=VERTEX_POINT('',#200384);
#39565=VERTEX_POINT('',#200386);
#39566=VERTEX_POINT('',#200388);
#39567=VERTEX_POINT('',#200392);
#39568=VERTEX_POINT('',#200393);
#39569=VERTEX_POINT('',#200398);
#39570=VERTEX_POINT('',#200399);
#39571=VERTEX_POINT('',#200407);
#39572=VERTEX_POINT('',#200408);
#39573=VERTEX_POINT('',#200410);
#39574=VERTEX_POINT('',#200412);
#39575=VERTEX_POINT('',#200416);
#39576=VERTEX_POINT('',#200417);
#39577=VERTEX_POINT('',#200422);
#39578=VERTEX_POINT('',#200423);
#39579=VERTEX_POINT('',#200431);
#39580=VERTEX_POINT('',#200432);
#39581=VERTEX_POINT('',#200434);
#39582=VERTEX_POINT('',#200436);
#39583=VERTEX_POINT('',#200440);
#39584=VERTEX_POINT('',#200441);
#39585=VERTEX_POINT('',#200446);
#39586=VERTEX_POINT('',#200447);
#39587=VERTEX_POINT('',#200455);
#39588=VERTEX_POINT('',#200456);
#39589=VERTEX_POINT('',#200458);
#39590=VERTEX_POINT('',#200460);
#39591=VERTEX_POINT('',#200464);
#39592=VERTEX_POINT('',#200465);
#39593=VERTEX_POINT('',#200470);
#39594=VERTEX_POINT('',#200471);
#39595=VERTEX_POINT('',#200479);
#39596=VERTEX_POINT('',#200480);
#39597=VERTEX_POINT('',#200482);
#39598=VERTEX_POINT('',#200484);
#39599=VERTEX_POINT('',#200488);
#39600=VERTEX_POINT('',#200489);
#39601=VERTEX_POINT('',#200494);
#39602=VERTEX_POINT('',#200495);
#39603=VERTEX_POINT('',#200503);
#39604=VERTEX_POINT('',#200504);
#39605=VERTEX_POINT('',#200506);
#39606=VERTEX_POINT('',#200508);
#39607=VERTEX_POINT('',#200512);
#39608=VERTEX_POINT('',#200513);
#39609=VERTEX_POINT('',#200518);
#39610=VERTEX_POINT('',#200519);
#39611=VERTEX_POINT('',#200527);
#39612=VERTEX_POINT('',#200528);
#39613=VERTEX_POINT('',#200530);
#39614=VERTEX_POINT('',#200532);
#39615=VERTEX_POINT('',#200536);
#39616=VERTEX_POINT('',#200537);
#39617=VERTEX_POINT('',#200542);
#39618=VERTEX_POINT('',#200543);
#39619=VERTEX_POINT('',#200551);
#39620=VERTEX_POINT('',#200552);
#39621=VERTEX_POINT('',#200554);
#39622=VERTEX_POINT('',#200556);
#39623=VERTEX_POINT('',#200560);
#39624=VERTEX_POINT('',#200561);
#39625=VERTEX_POINT('',#200566);
#39626=VERTEX_POINT('',#200567);
#39627=VERTEX_POINT('',#200575);
#39628=VERTEX_POINT('',#200576);
#39629=VERTEX_POINT('',#200578);
#39630=VERTEX_POINT('',#200580);
#39631=VERTEX_POINT('',#200584);
#39632=VERTEX_POINT('',#200585);
#39633=VERTEX_POINT('',#200590);
#39634=VERTEX_POINT('',#200591);
#39635=VERTEX_POINT('',#200599);
#39636=VERTEX_POINT('',#200600);
#39637=VERTEX_POINT('',#200602);
#39638=VERTEX_POINT('',#200604);
#39639=VERTEX_POINT('',#200608);
#39640=VERTEX_POINT('',#200609);
#39641=VERTEX_POINT('',#200614);
#39642=VERTEX_POINT('',#200615);
#39643=VERTEX_POINT('',#200623);
#39644=VERTEX_POINT('',#200624);
#39645=VERTEX_POINT('',#200626);
#39646=VERTEX_POINT('',#200628);
#39647=VERTEX_POINT('',#200632);
#39648=VERTEX_POINT('',#200633);
#39649=VERTEX_POINT('',#200638);
#39650=VERTEX_POINT('',#200639);
#39651=VERTEX_POINT('',#200647);
#39652=VERTEX_POINT('',#200648);
#39653=VERTEX_POINT('',#200650);
#39654=VERTEX_POINT('',#200652);
#39655=VERTEX_POINT('',#200656);
#39656=VERTEX_POINT('',#200657);
#39657=VERTEX_POINT('',#200662);
#39658=VERTEX_POINT('',#200663);
#39659=VERTEX_POINT('',#200671);
#39660=VERTEX_POINT('',#200672);
#39661=VERTEX_POINT('',#200674);
#39662=VERTEX_POINT('',#200676);
#39663=VERTEX_POINT('',#200680);
#39664=VERTEX_POINT('',#200681);
#39665=VERTEX_POINT('',#200686);
#39666=VERTEX_POINT('',#200687);
#39667=VERTEX_POINT('',#200695);
#39668=VERTEX_POINT('',#200696);
#39669=VERTEX_POINT('',#200698);
#39670=VERTEX_POINT('',#200700);
#39671=VERTEX_POINT('',#200704);
#39672=VERTEX_POINT('',#200705);
#39673=VERTEX_POINT('',#200710);
#39674=VERTEX_POINT('',#200711);
#39675=VERTEX_POINT('',#200719);
#39676=VERTEX_POINT('',#200720);
#39677=VERTEX_POINT('',#200722);
#39678=VERTEX_POINT('',#200724);
#39679=VERTEX_POINT('',#200728);
#39680=VERTEX_POINT('',#200729);
#39681=VERTEX_POINT('',#200734);
#39682=VERTEX_POINT('',#200735);
#39683=VERTEX_POINT('',#200743);
#39684=VERTEX_POINT('',#200744);
#39685=VERTEX_POINT('',#200746);
#39686=VERTEX_POINT('',#200748);
#39687=VERTEX_POINT('',#200752);
#39688=VERTEX_POINT('',#200753);
#39689=VERTEX_POINT('',#200758);
#39690=VERTEX_POINT('',#200759);
#39691=VERTEX_POINT('',#200767);
#39692=VERTEX_POINT('',#200768);
#39693=VERTEX_POINT('',#200770);
#39694=VERTEX_POINT('',#200772);
#39695=VERTEX_POINT('',#200776);
#39696=VERTEX_POINT('',#200777);
#39697=VERTEX_POINT('',#200782);
#39698=VERTEX_POINT('',#200783);
#39699=VERTEX_POINT('',#200791);
#39700=VERTEX_POINT('',#200792);
#39701=VERTEX_POINT('',#200794);
#39702=VERTEX_POINT('',#200796);
#39703=VERTEX_POINT('',#200800);
#39704=VERTEX_POINT('',#200801);
#39705=VERTEX_POINT('',#200806);
#39706=VERTEX_POINT('',#200807);
#39707=VERTEX_POINT('',#200815);
#39708=VERTEX_POINT('',#200816);
#39709=VERTEX_POINT('',#200818);
#39710=VERTEX_POINT('',#200820);
#39711=VERTEX_POINT('',#200824);
#39712=VERTEX_POINT('',#200825);
#39713=VERTEX_POINT('',#200830);
#39714=VERTEX_POINT('',#200831);
#39715=VERTEX_POINT('',#200839);
#39716=VERTEX_POINT('',#200840);
#39717=VERTEX_POINT('',#200842);
#39718=VERTEX_POINT('',#200844);
#39719=VERTEX_POINT('',#200848);
#39720=VERTEX_POINT('',#200849);
#39721=VERTEX_POINT('',#200854);
#39722=VERTEX_POINT('',#200855);
#39723=VERTEX_POINT('',#200863);
#39724=VERTEX_POINT('',#200864);
#39725=VERTEX_POINT('',#200866);
#39726=VERTEX_POINT('',#200868);
#39727=VERTEX_POINT('',#200872);
#39728=VERTEX_POINT('',#200873);
#39729=VERTEX_POINT('',#200878);
#39730=VERTEX_POINT('',#200879);
#39731=VERTEX_POINT('',#200887);
#39732=VERTEX_POINT('',#200888);
#39733=VERTEX_POINT('',#200890);
#39734=VERTEX_POINT('',#200892);
#39735=VERTEX_POINT('',#200896);
#39736=VERTEX_POINT('',#200897);
#39737=VERTEX_POINT('',#200902);
#39738=VERTEX_POINT('',#200903);
#39739=VERTEX_POINT('',#200911);
#39740=VERTEX_POINT('',#200912);
#39741=VERTEX_POINT('',#200914);
#39742=VERTEX_POINT('',#200916);
#39743=VERTEX_POINT('',#200920);
#39744=VERTEX_POINT('',#200921);
#39745=VERTEX_POINT('',#200926);
#39746=VERTEX_POINT('',#200927);
#39747=VERTEX_POINT('',#200935);
#39748=VERTEX_POINT('',#200936);
#39749=VERTEX_POINT('',#200938);
#39750=VERTEX_POINT('',#200940);
#39751=VERTEX_POINT('',#200944);
#39752=VERTEX_POINT('',#200945);
#39753=VERTEX_POINT('',#200950);
#39754=VERTEX_POINT('',#200951);
#39755=VERTEX_POINT('',#200959);
#39756=VERTEX_POINT('',#200960);
#39757=VERTEX_POINT('',#200962);
#39758=VERTEX_POINT('',#200964);
#39759=VERTEX_POINT('',#200968);
#39760=VERTEX_POINT('',#200969);
#39761=VERTEX_POINT('',#200974);
#39762=VERTEX_POINT('',#200975);
#39763=VERTEX_POINT('',#200983);
#39764=VERTEX_POINT('',#200984);
#39765=VERTEX_POINT('',#200986);
#39766=VERTEX_POINT('',#200988);
#39767=VERTEX_POINT('',#200992);
#39768=VERTEX_POINT('',#200993);
#39769=VERTEX_POINT('',#200998);
#39770=VERTEX_POINT('',#200999);
#39771=VERTEX_POINT('',#201007);
#39772=VERTEX_POINT('',#201008);
#39773=VERTEX_POINT('',#201010);
#39774=VERTEX_POINT('',#201012);
#39775=VERTEX_POINT('',#201016);
#39776=VERTEX_POINT('',#201017);
#39777=VERTEX_POINT('',#201022);
#39778=VERTEX_POINT('',#201023);
#39779=VERTEX_POINT('',#201031);
#39780=VERTEX_POINT('',#201032);
#39781=VERTEX_POINT('',#201034);
#39782=VERTEX_POINT('',#201036);
#39783=VERTEX_POINT('',#201040);
#39784=VERTEX_POINT('',#201041);
#39785=VERTEX_POINT('',#201046);
#39786=VERTEX_POINT('',#201047);
#39787=VERTEX_POINT('',#201055);
#39788=VERTEX_POINT('',#201056);
#39789=VERTEX_POINT('',#201058);
#39790=VERTEX_POINT('',#201060);
#39791=VERTEX_POINT('',#201064);
#39792=VERTEX_POINT('',#201065);
#39793=VERTEX_POINT('',#201070);
#39794=VERTEX_POINT('',#201071);
#39795=VERTEX_POINT('',#201079);
#39796=VERTEX_POINT('',#201080);
#39797=VERTEX_POINT('',#201082);
#39798=VERTEX_POINT('',#201084);
#39799=VERTEX_POINT('',#201088);
#39800=VERTEX_POINT('',#201089);
#39801=VERTEX_POINT('',#201094);
#39802=VERTEX_POINT('',#201095);
#39803=VERTEX_POINT('',#201103);
#39804=VERTEX_POINT('',#201104);
#39805=VERTEX_POINT('',#201106);
#39806=VERTEX_POINT('',#201108);
#39807=VERTEX_POINT('',#201112);
#39808=VERTEX_POINT('',#201113);
#39809=VERTEX_POINT('',#201118);
#39810=VERTEX_POINT('',#201119);
#39811=VERTEX_POINT('',#201127);
#39812=VERTEX_POINT('',#201128);
#39813=VERTEX_POINT('',#201130);
#39814=VERTEX_POINT('',#201132);
#39815=VERTEX_POINT('',#201136);
#39816=VERTEX_POINT('',#201137);
#39817=VERTEX_POINT('',#201142);
#39818=VERTEX_POINT('',#201143);
#39819=VERTEX_POINT('',#201151);
#39820=VERTEX_POINT('',#201152);
#39821=VERTEX_POINT('',#201154);
#39822=VERTEX_POINT('',#201156);
#39823=VERTEX_POINT('',#201160);
#39824=VERTEX_POINT('',#201161);
#39825=VERTEX_POINT('',#201166);
#39826=VERTEX_POINT('',#201167);
#39827=VERTEX_POINT('',#201175);
#39828=VERTEX_POINT('',#201176);
#39829=VERTEX_POINT('',#201178);
#39830=VERTEX_POINT('',#201180);
#39831=VERTEX_POINT('',#201184);
#39832=VERTEX_POINT('',#201185);
#39833=VERTEX_POINT('',#201190);
#39834=VERTEX_POINT('',#201191);
#39835=VERTEX_POINT('',#201199);
#39836=VERTEX_POINT('',#201200);
#39837=VERTEX_POINT('',#201202);
#39838=VERTEX_POINT('',#201204);
#39839=VERTEX_POINT('',#201208);
#39840=VERTEX_POINT('',#201209);
#39841=VERTEX_POINT('',#201214);
#39842=VERTEX_POINT('',#201215);
#39843=VERTEX_POINT('',#201223);
#39844=VERTEX_POINT('',#201224);
#39845=VERTEX_POINT('',#201226);
#39846=VERTEX_POINT('',#201228);
#39847=VERTEX_POINT('',#201232);
#39848=VERTEX_POINT('',#201233);
#39849=VERTEX_POINT('',#201238);
#39850=VERTEX_POINT('',#201239);
#39851=VERTEX_POINT('',#201247);
#39852=VERTEX_POINT('',#201248);
#39853=VERTEX_POINT('',#201250);
#39854=VERTEX_POINT('',#201252);
#39855=VERTEX_POINT('',#201256);
#39856=VERTEX_POINT('',#201257);
#39857=VERTEX_POINT('',#201262);
#39858=VERTEX_POINT('',#201263);
#39859=VERTEX_POINT('',#201271);
#39860=VERTEX_POINT('',#201272);
#39861=VERTEX_POINT('',#201274);
#39862=VERTEX_POINT('',#201276);
#39863=VERTEX_POINT('',#201280);
#39864=VERTEX_POINT('',#201281);
#39865=VERTEX_POINT('',#201286);
#39866=VERTEX_POINT('',#201287);
#39867=VERTEX_POINT('',#201295);
#39868=VERTEX_POINT('',#201296);
#39869=VERTEX_POINT('',#201298);
#39870=VERTEX_POINT('',#201300);
#39871=VERTEX_POINT('',#201304);
#39872=VERTEX_POINT('',#201305);
#39873=VERTEX_POINT('',#201310);
#39874=VERTEX_POINT('',#201311);
#39875=VERTEX_POINT('',#201319);
#39876=VERTEX_POINT('',#201320);
#39877=VERTEX_POINT('',#201322);
#39878=VERTEX_POINT('',#201324);
#39879=VERTEX_POINT('',#201328);
#39880=VERTEX_POINT('',#201329);
#39881=VERTEX_POINT('',#201334);
#39882=VERTEX_POINT('',#201335);
#39883=VERTEX_POINT('',#201343);
#39884=VERTEX_POINT('',#201344);
#39885=VERTEX_POINT('',#201346);
#39886=VERTEX_POINT('',#201348);
#39887=VERTEX_POINT('',#201352);
#39888=VERTEX_POINT('',#201353);
#39889=VERTEX_POINT('',#201358);
#39890=VERTEX_POINT('',#201359);
#39891=VERTEX_POINT('',#201367);
#39892=VERTEX_POINT('',#201368);
#39893=VERTEX_POINT('',#201370);
#39894=VERTEX_POINT('',#201372);
#39895=VERTEX_POINT('',#201376);
#39896=VERTEX_POINT('',#201377);
#39897=VERTEX_POINT('',#201382);
#39898=VERTEX_POINT('',#201383);
#39899=VERTEX_POINT('',#201391);
#39900=VERTEX_POINT('',#201392);
#39901=VERTEX_POINT('',#201394);
#39902=VERTEX_POINT('',#201396);
#39903=VERTEX_POINT('',#201400);
#39904=VERTEX_POINT('',#201401);
#39905=VERTEX_POINT('',#201406);
#39906=VERTEX_POINT('',#201407);
#39907=VERTEX_POINT('',#201415);
#39908=VERTEX_POINT('',#201416);
#39909=VERTEX_POINT('',#201418);
#39910=VERTEX_POINT('',#201420);
#39911=VERTEX_POINT('',#201424);
#39912=VERTEX_POINT('',#201425);
#39913=VERTEX_POINT('',#201430);
#39914=VERTEX_POINT('',#201431);
#39915=VERTEX_POINT('',#201439);
#39916=VERTEX_POINT('',#201440);
#39917=VERTEX_POINT('',#201442);
#39918=VERTEX_POINT('',#201444);
#39919=VERTEX_POINT('',#201448);
#39920=VERTEX_POINT('',#201449);
#39921=VERTEX_POINT('',#201454);
#39922=VERTEX_POINT('',#201455);
#39923=VERTEX_POINT('',#201463);
#39924=VERTEX_POINT('',#201464);
#39925=VERTEX_POINT('',#201466);
#39926=VERTEX_POINT('',#201468);
#39927=VERTEX_POINT('',#201472);
#39928=VERTEX_POINT('',#201473);
#39929=VERTEX_POINT('',#201478);
#39930=VERTEX_POINT('',#201479);
#39931=VERTEX_POINT('',#201487);
#39932=VERTEX_POINT('',#201488);
#39933=VERTEX_POINT('',#201490);
#39934=VERTEX_POINT('',#201492);
#39935=VERTEX_POINT('',#201496);
#39936=VERTEX_POINT('',#201497);
#39937=VERTEX_POINT('',#201502);
#39938=VERTEX_POINT('',#201503);
#39939=VERTEX_POINT('',#201511);
#39940=VERTEX_POINT('',#201512);
#39941=VERTEX_POINT('',#201514);
#39942=VERTEX_POINT('',#201516);
#39943=VERTEX_POINT('',#201520);
#39944=VERTEX_POINT('',#201521);
#39945=VERTEX_POINT('',#201526);
#39946=VERTEX_POINT('',#201527);
#39947=VERTEX_POINT('',#201535);
#39948=VERTEX_POINT('',#201536);
#39949=VERTEX_POINT('',#201538);
#39950=VERTEX_POINT('',#201540);
#39951=VERTEX_POINT('',#201544);
#39952=VERTEX_POINT('',#201545);
#39953=VERTEX_POINT('',#201550);
#39954=VERTEX_POINT('',#201551);
#39955=VERTEX_POINT('',#201559);
#39956=VERTEX_POINT('',#201560);
#39957=VERTEX_POINT('',#201562);
#39958=VERTEX_POINT('',#201564);
#39959=VERTEX_POINT('',#201568);
#39960=VERTEX_POINT('',#201569);
#39961=VERTEX_POINT('',#201574);
#39962=VERTEX_POINT('',#201575);
#39963=VERTEX_POINT('',#201583);
#39964=VERTEX_POINT('',#201584);
#39965=VERTEX_POINT('',#201586);
#39966=VERTEX_POINT('',#201588);
#39967=VERTEX_POINT('',#201592);
#39968=VERTEX_POINT('',#201593);
#39969=VERTEX_POINT('',#201598);
#39970=VERTEX_POINT('',#201599);
#39971=VERTEX_POINT('',#201607);
#39972=VERTEX_POINT('',#201608);
#39973=VERTEX_POINT('',#201610);
#39974=VERTEX_POINT('',#201612);
#39975=VERTEX_POINT('',#201616);
#39976=VERTEX_POINT('',#201617);
#39977=VERTEX_POINT('',#201622);
#39978=VERTEX_POINT('',#201623);
#39979=VERTEX_POINT('',#201631);
#39980=VERTEX_POINT('',#201632);
#39981=VERTEX_POINT('',#201634);
#39982=VERTEX_POINT('',#201636);
#39983=VERTEX_POINT('',#201640);
#39984=VERTEX_POINT('',#201641);
#39985=VERTEX_POINT('',#201646);
#39986=VERTEX_POINT('',#201647);
#39987=VERTEX_POINT('',#201655);
#39988=VERTEX_POINT('',#201656);
#39989=VERTEX_POINT('',#201658);
#39990=VERTEX_POINT('',#201660);
#39991=VERTEX_POINT('',#201664);
#39992=VERTEX_POINT('',#201665);
#39993=VERTEX_POINT('',#201670);
#39994=VERTEX_POINT('',#201671);
#39995=VERTEX_POINT('',#201679);
#39996=VERTEX_POINT('',#201680);
#39997=VERTEX_POINT('',#201682);
#39998=VERTEX_POINT('',#201684);
#39999=VERTEX_POINT('',#201688);
#40000=VERTEX_POINT('',#201689);
#40001=VERTEX_POINT('',#201694);
#40002=VERTEX_POINT('',#201695);
#40003=VERTEX_POINT('',#201703);
#40004=VERTEX_POINT('',#201704);
#40005=VERTEX_POINT('',#201706);
#40006=VERTEX_POINT('',#201708);
#40007=VERTEX_POINT('',#201712);
#40008=VERTEX_POINT('',#201713);
#40009=VERTEX_POINT('',#201718);
#40010=VERTEX_POINT('',#201719);
#40011=VERTEX_POINT('',#201727);
#40012=VERTEX_POINT('',#201728);
#40013=VERTEX_POINT('',#201730);
#40014=VERTEX_POINT('',#201732);
#40015=VERTEX_POINT('',#201736);
#40016=VERTEX_POINT('',#201737);
#40017=VERTEX_POINT('',#201742);
#40018=VERTEX_POINT('',#201743);
#40019=VERTEX_POINT('',#201751);
#40020=VERTEX_POINT('',#201752);
#40021=VERTEX_POINT('',#201754);
#40022=VERTEX_POINT('',#201756);
#40023=VERTEX_POINT('',#201760);
#40024=VERTEX_POINT('',#201761);
#40025=VERTEX_POINT('',#201766);
#40026=VERTEX_POINT('',#201767);
#40027=VERTEX_POINT('',#201775);
#40028=VERTEX_POINT('',#201776);
#40029=VERTEX_POINT('',#201778);
#40030=VERTEX_POINT('',#201780);
#40031=VERTEX_POINT('',#201784);
#40032=VERTEX_POINT('',#201785);
#40033=VERTEX_POINT('',#201790);
#40034=VERTEX_POINT('',#201791);
#40035=VERTEX_POINT('',#201799);
#40036=VERTEX_POINT('',#201800);
#40037=VERTEX_POINT('',#201802);
#40038=VERTEX_POINT('',#201804);
#40039=VERTEX_POINT('',#201808);
#40040=VERTEX_POINT('',#201809);
#40041=VERTEX_POINT('',#201814);
#40042=VERTEX_POINT('',#201815);
#40043=VERTEX_POINT('',#201823);
#40044=VERTEX_POINT('',#201824);
#40045=VERTEX_POINT('',#201826);
#40046=VERTEX_POINT('',#201828);
#40047=VERTEX_POINT('',#201832);
#40048=VERTEX_POINT('',#201833);
#40049=VERTEX_POINT('',#201838);
#40050=VERTEX_POINT('',#201839);
#40051=VERTEX_POINT('',#201847);
#40052=VERTEX_POINT('',#201848);
#40053=VERTEX_POINT('',#201850);
#40054=VERTEX_POINT('',#201852);
#40055=VERTEX_POINT('',#201856);
#40056=VERTEX_POINT('',#201857);
#40057=VERTEX_POINT('',#201862);
#40058=VERTEX_POINT('',#201863);
#40059=VERTEX_POINT('',#201871);
#40060=VERTEX_POINT('',#201872);
#40061=VERTEX_POINT('',#201874);
#40062=VERTEX_POINT('',#201876);
#40063=VERTEX_POINT('',#201880);
#40064=VERTEX_POINT('',#201881);
#40065=VERTEX_POINT('',#201886);
#40066=VERTEX_POINT('',#201887);
#40067=VERTEX_POINT('',#201895);
#40068=VERTEX_POINT('',#201896);
#40069=VERTEX_POINT('',#201898);
#40070=VERTEX_POINT('',#201900);
#40071=VERTEX_POINT('',#201904);
#40072=VERTEX_POINT('',#201905);
#40073=VERTEX_POINT('',#201910);
#40074=VERTEX_POINT('',#201911);
#40075=VERTEX_POINT('',#201919);
#40076=VERTEX_POINT('',#201920);
#40077=VERTEX_POINT('',#201922);
#40078=VERTEX_POINT('',#201924);
#40079=VERTEX_POINT('',#201928);
#40080=VERTEX_POINT('',#201929);
#40081=VERTEX_POINT('',#201934);
#40082=VERTEX_POINT('',#201935);
#40083=VERTEX_POINT('',#201943);
#40084=VERTEX_POINT('',#201944);
#40085=VERTEX_POINT('',#201946);
#40086=VERTEX_POINT('',#201948);
#40087=VERTEX_POINT('',#201952);
#40088=VERTEX_POINT('',#201953);
#40089=VERTEX_POINT('',#201958);
#40090=VERTEX_POINT('',#201959);
#40091=VERTEX_POINT('',#201967);
#40092=VERTEX_POINT('',#201968);
#40093=VERTEX_POINT('',#201970);
#40094=VERTEX_POINT('',#201972);
#40095=VERTEX_POINT('',#201976);
#40096=VERTEX_POINT('',#201977);
#40097=VERTEX_POINT('',#201982);
#40098=VERTEX_POINT('',#201983);
#40099=VERTEX_POINT('',#201991);
#40100=VERTEX_POINT('',#201992);
#40101=VERTEX_POINT('',#201994);
#40102=VERTEX_POINT('',#201996);
#40103=VERTEX_POINT('',#202000);
#40104=VERTEX_POINT('',#202001);
#40105=VERTEX_POINT('',#202006);
#40106=VERTEX_POINT('',#202007);
#40107=VERTEX_POINT('',#202015);
#40108=VERTEX_POINT('',#202016);
#40109=VERTEX_POINT('',#202018);
#40110=VERTEX_POINT('',#202020);
#40111=VERTEX_POINT('',#202024);
#40112=VERTEX_POINT('',#202025);
#40113=VERTEX_POINT('',#202030);
#40114=VERTEX_POINT('',#202031);
#40115=VERTEX_POINT('',#202039);
#40116=VERTEX_POINT('',#202040);
#40117=VERTEX_POINT('',#202042);
#40118=VERTEX_POINT('',#202044);
#40119=VERTEX_POINT('',#202048);
#40120=VERTEX_POINT('',#202049);
#40121=VERTEX_POINT('',#202054);
#40122=VERTEX_POINT('',#202055);
#40123=VERTEX_POINT('',#202063);
#40124=VERTEX_POINT('',#202064);
#40125=VERTEX_POINT('',#202066);
#40126=VERTEX_POINT('',#202068);
#40127=VERTEX_POINT('',#202072);
#40128=VERTEX_POINT('',#202073);
#40129=VERTEX_POINT('',#202078);
#40130=VERTEX_POINT('',#202079);
#40131=VERTEX_POINT('',#202087);
#40132=VERTEX_POINT('',#202088);
#40133=VERTEX_POINT('',#202090);
#40134=VERTEX_POINT('',#202092);
#40135=VERTEX_POINT('',#202096);
#40136=VERTEX_POINT('',#202097);
#40137=VERTEX_POINT('',#202102);
#40138=VERTEX_POINT('',#202103);
#40139=VERTEX_POINT('',#202111);
#40140=VERTEX_POINT('',#202112);
#40141=VERTEX_POINT('',#202114);
#40142=VERTEX_POINT('',#202116);
#40143=VERTEX_POINT('',#202120);
#40144=VERTEX_POINT('',#202121);
#40145=VERTEX_POINT('',#202126);
#40146=VERTEX_POINT('',#202127);
#40147=VERTEX_POINT('',#202135);
#40148=VERTEX_POINT('',#202136);
#40149=VERTEX_POINT('',#202138);
#40150=VERTEX_POINT('',#202140);
#40151=VERTEX_POINT('',#202144);
#40152=VERTEX_POINT('',#202145);
#40153=VERTEX_POINT('',#202150);
#40154=VERTEX_POINT('',#202151);
#40155=VERTEX_POINT('',#202159);
#40156=VERTEX_POINT('',#202160);
#40157=VERTEX_POINT('',#202162);
#40158=VERTEX_POINT('',#202164);
#40159=VERTEX_POINT('',#202168);
#40160=VERTEX_POINT('',#202169);
#40161=VERTEX_POINT('',#202174);
#40162=VERTEX_POINT('',#202175);
#40163=VERTEX_POINT('',#202183);
#40164=VERTEX_POINT('',#202184);
#40165=VERTEX_POINT('',#202186);
#40166=VERTEX_POINT('',#202188);
#40167=VERTEX_POINT('',#202192);
#40168=VERTEX_POINT('',#202193);
#40169=VERTEX_POINT('',#202198);
#40170=VERTEX_POINT('',#202199);
#40171=VERTEX_POINT('',#202207);
#40172=VERTEX_POINT('',#202208);
#40173=VERTEX_POINT('',#202210);
#40174=VERTEX_POINT('',#202212);
#40175=VERTEX_POINT('',#202216);
#40176=VERTEX_POINT('',#202217);
#40177=VERTEX_POINT('',#202222);
#40178=VERTEX_POINT('',#202223);
#40179=VERTEX_POINT('',#202231);
#40180=VERTEX_POINT('',#202232);
#40181=VERTEX_POINT('',#202234);
#40182=VERTEX_POINT('',#202236);
#40183=VERTEX_POINT('',#202240);
#40184=VERTEX_POINT('',#202241);
#40185=VERTEX_POINT('',#202246);
#40186=VERTEX_POINT('',#202247);
#40187=VERTEX_POINT('',#202255);
#40188=VERTEX_POINT('',#202256);
#40189=VERTEX_POINT('',#202258);
#40190=VERTEX_POINT('',#202260);
#40191=VERTEX_POINT('',#202264);
#40192=VERTEX_POINT('',#202265);
#40193=VERTEX_POINT('',#202270);
#40194=VERTEX_POINT('',#202271);
#40195=VERTEX_POINT('',#202279);
#40196=VERTEX_POINT('',#202280);
#40197=VERTEX_POINT('',#202282);
#40198=VERTEX_POINT('',#202284);
#40199=VERTEX_POINT('',#202288);
#40200=VERTEX_POINT('',#202289);
#40201=VERTEX_POINT('',#202294);
#40202=VERTEX_POINT('',#202295);
#40203=VERTEX_POINT('',#202303);
#40204=VERTEX_POINT('',#202304);
#40205=VERTEX_POINT('',#202306);
#40206=VERTEX_POINT('',#202308);
#40207=VERTEX_POINT('',#202312);
#40208=VERTEX_POINT('',#202313);
#40209=VERTEX_POINT('',#202318);
#40210=VERTEX_POINT('',#202319);
#40211=VERTEX_POINT('',#202327);
#40212=VERTEX_POINT('',#202328);
#40213=VERTEX_POINT('',#202330);
#40214=VERTEX_POINT('',#202332);
#40215=VERTEX_POINT('',#202336);
#40216=VERTEX_POINT('',#202337);
#40217=VERTEX_POINT('',#202342);
#40218=VERTEX_POINT('',#202343);
#40219=VERTEX_POINT('',#202351);
#40220=VERTEX_POINT('',#202352);
#40221=VERTEX_POINT('',#202354);
#40222=VERTEX_POINT('',#202356);
#40223=VERTEX_POINT('',#202360);
#40224=VERTEX_POINT('',#202361);
#40225=VERTEX_POINT('',#202366);
#40226=VERTEX_POINT('',#202367);
#40227=VERTEX_POINT('',#202375);
#40228=VERTEX_POINT('',#202376);
#40229=VERTEX_POINT('',#202378);
#40230=VERTEX_POINT('',#202380);
#40231=VERTEX_POINT('',#202384);
#40232=VERTEX_POINT('',#202385);
#40233=VERTEX_POINT('',#202390);
#40234=VERTEX_POINT('',#202391);
#40235=VERTEX_POINT('',#202399);
#40236=VERTEX_POINT('',#202400);
#40237=VERTEX_POINT('',#202402);
#40238=VERTEX_POINT('',#202404);
#40239=VERTEX_POINT('',#202408);
#40240=VERTEX_POINT('',#202409);
#40241=VERTEX_POINT('',#202414);
#40242=VERTEX_POINT('',#202415);
#40243=VERTEX_POINT('',#202423);
#40244=VERTEX_POINT('',#202424);
#40245=VERTEX_POINT('',#202426);
#40246=VERTEX_POINT('',#202428);
#40247=VERTEX_POINT('',#202432);
#40248=VERTEX_POINT('',#202433);
#40249=VERTEX_POINT('',#202438);
#40250=VERTEX_POINT('',#202439);
#40251=VERTEX_POINT('',#202447);
#40252=VERTEX_POINT('',#202448);
#40253=VERTEX_POINT('',#202450);
#40254=VERTEX_POINT('',#202452);
#40255=VERTEX_POINT('',#202456);
#40256=VERTEX_POINT('',#202457);
#40257=VERTEX_POINT('',#202462);
#40258=VERTEX_POINT('',#202463);
#40259=VERTEX_POINT('',#202471);
#40260=VERTEX_POINT('',#202472);
#40261=VERTEX_POINT('',#202474);
#40262=VERTEX_POINT('',#202476);
#40263=VERTEX_POINT('',#202480);
#40264=VERTEX_POINT('',#202481);
#40265=VERTEX_POINT('',#202486);
#40266=VERTEX_POINT('',#202487);
#40267=VERTEX_POINT('',#202495);
#40268=VERTEX_POINT('',#202496);
#40269=VERTEX_POINT('',#202498);
#40270=VERTEX_POINT('',#202500);
#40271=VERTEX_POINT('',#202504);
#40272=VERTEX_POINT('',#202505);
#40273=VERTEX_POINT('',#202510);
#40274=VERTEX_POINT('',#202511);
#40275=VERTEX_POINT('',#202519);
#40276=VERTEX_POINT('',#202520);
#40277=VERTEX_POINT('',#202522);
#40278=VERTEX_POINT('',#202524);
#40279=VERTEX_POINT('',#202528);
#40280=VERTEX_POINT('',#202529);
#40281=VERTEX_POINT('',#202534);
#40282=VERTEX_POINT('',#202535);
#40283=VERTEX_POINT('',#202543);
#40284=VERTEX_POINT('',#202544);
#40285=VERTEX_POINT('',#202546);
#40286=VERTEX_POINT('',#202548);
#40287=VERTEX_POINT('',#202552);
#40288=VERTEX_POINT('',#202553);
#40289=VERTEX_POINT('',#202558);
#40290=VERTEX_POINT('',#202559);
#40291=VERTEX_POINT('',#202567);
#40292=VERTEX_POINT('',#202568);
#40293=VERTEX_POINT('',#202570);
#40294=VERTEX_POINT('',#202572);
#40295=VERTEX_POINT('',#202576);
#40296=VERTEX_POINT('',#202577);
#40297=VERTEX_POINT('',#202582);
#40298=VERTEX_POINT('',#202583);
#40299=VERTEX_POINT('',#202591);
#40300=VERTEX_POINT('',#202592);
#40301=VERTEX_POINT('',#202594);
#40302=VERTEX_POINT('',#202596);
#40303=VERTEX_POINT('',#202600);
#40304=VERTEX_POINT('',#202601);
#40305=VERTEX_POINT('',#202606);
#40306=VERTEX_POINT('',#202607);
#40307=VERTEX_POINT('',#202615);
#40308=VERTEX_POINT('',#202616);
#40309=VERTEX_POINT('',#202618);
#40310=VERTEX_POINT('',#202620);
#40311=VERTEX_POINT('',#202624);
#40312=VERTEX_POINT('',#202625);
#40313=VERTEX_POINT('',#202630);
#40314=VERTEX_POINT('',#202631);
#40315=VERTEX_POINT('',#202639);
#40316=VERTEX_POINT('',#202640);
#40317=VERTEX_POINT('',#202642);
#40318=VERTEX_POINT('',#202644);
#40319=VERTEX_POINT('',#202648);
#40320=VERTEX_POINT('',#202649);
#40321=VERTEX_POINT('',#202654);
#40322=VERTEX_POINT('',#202655);
#40323=VERTEX_POINT('',#202663);
#40324=VERTEX_POINT('',#202664);
#40325=VERTEX_POINT('',#202666);
#40326=VERTEX_POINT('',#202668);
#40327=VERTEX_POINT('',#202672);
#40328=VERTEX_POINT('',#202673);
#40329=VERTEX_POINT('',#202678);
#40330=VERTEX_POINT('',#202679);
#40331=VERTEX_POINT('',#202687);
#40332=VERTEX_POINT('',#202688);
#40333=VERTEX_POINT('',#202690);
#40334=VERTEX_POINT('',#202692);
#40335=VERTEX_POINT('',#202696);
#40336=VERTEX_POINT('',#202697);
#40337=VERTEX_POINT('',#202702);
#40338=VERTEX_POINT('',#202703);
#40339=VERTEX_POINT('',#202711);
#40340=VERTEX_POINT('',#202712);
#40341=VERTEX_POINT('',#202714);
#40342=VERTEX_POINT('',#202716);
#40343=VERTEX_POINT('',#202720);
#40344=VERTEX_POINT('',#202721);
#40345=VERTEX_POINT('',#202726);
#40346=VERTEX_POINT('',#202727);
#40347=VERTEX_POINT('',#202735);
#40348=VERTEX_POINT('',#202736);
#40349=VERTEX_POINT('',#202738);
#40350=VERTEX_POINT('',#202740);
#40351=VERTEX_POINT('',#202744);
#40352=VERTEX_POINT('',#202745);
#40353=VERTEX_POINT('',#202750);
#40354=VERTEX_POINT('',#202751);
#40355=VERTEX_POINT('',#202759);
#40356=VERTEX_POINT('',#202760);
#40357=VERTEX_POINT('',#202762);
#40358=VERTEX_POINT('',#202764);
#40359=VERTEX_POINT('',#202768);
#40360=VERTEX_POINT('',#202769);
#40361=VERTEX_POINT('',#202774);
#40362=VERTEX_POINT('',#202775);
#40363=VERTEX_POINT('',#202783);
#40364=VERTEX_POINT('',#202784);
#40365=VERTEX_POINT('',#202786);
#40366=VERTEX_POINT('',#202788);
#40367=VERTEX_POINT('',#202792);
#40368=VERTEX_POINT('',#202793);
#40369=VERTEX_POINT('',#202798);
#40370=VERTEX_POINT('',#202799);
#40371=VERTEX_POINT('',#202807);
#40372=VERTEX_POINT('',#202808);
#40373=VERTEX_POINT('',#202810);
#40374=VERTEX_POINT('',#202812);
#40375=VERTEX_POINT('',#202816);
#40376=VERTEX_POINT('',#202817);
#40377=VERTEX_POINT('',#202822);
#40378=VERTEX_POINT('',#202823);
#40379=VERTEX_POINT('',#202831);
#40380=VERTEX_POINT('',#202832);
#40381=VERTEX_POINT('',#202834);
#40382=VERTEX_POINT('',#202836);
#40383=VERTEX_POINT('',#202840);
#40384=VERTEX_POINT('',#202841);
#40385=VERTEX_POINT('',#202846);
#40386=VERTEX_POINT('',#202847);
#40387=VERTEX_POINT('',#202855);
#40388=VERTEX_POINT('',#202856);
#40389=VERTEX_POINT('',#202858);
#40390=VERTEX_POINT('',#202860);
#40391=VERTEX_POINT('',#202864);
#40392=VERTEX_POINT('',#202865);
#40393=VERTEX_POINT('',#202870);
#40394=VERTEX_POINT('',#202871);
#40395=VERTEX_POINT('',#202879);
#40396=VERTEX_POINT('',#202880);
#40397=VERTEX_POINT('',#202882);
#40398=VERTEX_POINT('',#202884);
#40399=VERTEX_POINT('',#202888);
#40400=VERTEX_POINT('',#202889);
#40401=VERTEX_POINT('',#202894);
#40402=VERTEX_POINT('',#202895);
#40403=VERTEX_POINT('',#202903);
#40404=VERTEX_POINT('',#202904);
#40405=VERTEX_POINT('',#202906);
#40406=VERTEX_POINT('',#202908);
#40407=VERTEX_POINT('',#202912);
#40408=VERTEX_POINT('',#202913);
#40409=VERTEX_POINT('',#202918);
#40410=VERTEX_POINT('',#202919);
#40411=VERTEX_POINT('',#202927);
#40412=VERTEX_POINT('',#202928);
#40413=VERTEX_POINT('',#202930);
#40414=VERTEX_POINT('',#202932);
#40415=VERTEX_POINT('',#202936);
#40416=VERTEX_POINT('',#202937);
#40417=VERTEX_POINT('',#202942);
#40418=VERTEX_POINT('',#202943);
#40419=VERTEX_POINT('',#202951);
#40420=VERTEX_POINT('',#202952);
#40421=VERTEX_POINT('',#202954);
#40422=VERTEX_POINT('',#202956);
#40423=VERTEX_POINT('',#202960);
#40424=VERTEX_POINT('',#202961);
#40425=VERTEX_POINT('',#202966);
#40426=VERTEX_POINT('',#202967);
#40427=VERTEX_POINT('',#202975);
#40428=VERTEX_POINT('',#202976);
#40429=VERTEX_POINT('',#202978);
#40430=VERTEX_POINT('',#202980);
#40431=VERTEX_POINT('',#202984);
#40432=VERTEX_POINT('',#202985);
#40433=VERTEX_POINT('',#202990);
#40434=VERTEX_POINT('',#202991);
#40435=VERTEX_POINT('',#202999);
#40436=VERTEX_POINT('',#203000);
#40437=VERTEX_POINT('',#203002);
#40438=VERTEX_POINT('',#203004);
#40439=VERTEX_POINT('',#203008);
#40440=VERTEX_POINT('',#203009);
#40441=VERTEX_POINT('',#203014);
#40442=VERTEX_POINT('',#203015);
#40443=VERTEX_POINT('',#203023);
#40444=VERTEX_POINT('',#203024);
#40445=VERTEX_POINT('',#203026);
#40446=VERTEX_POINT('',#203028);
#40447=VERTEX_POINT('',#203032);
#40448=VERTEX_POINT('',#203033);
#40449=VERTEX_POINT('',#203038);
#40450=VERTEX_POINT('',#203039);
#40451=VERTEX_POINT('',#203047);
#40452=VERTEX_POINT('',#203048);
#40453=VERTEX_POINT('',#203050);
#40454=VERTEX_POINT('',#203052);
#40455=VERTEX_POINT('',#203056);
#40456=VERTEX_POINT('',#203057);
#40457=VERTEX_POINT('',#203062);
#40458=VERTEX_POINT('',#203063);
#40459=VERTEX_POINT('',#203071);
#40460=VERTEX_POINT('',#203072);
#40461=VERTEX_POINT('',#203074);
#40462=VERTEX_POINT('',#203076);
#40463=VERTEX_POINT('',#203080);
#40464=VERTEX_POINT('',#203081);
#40465=VERTEX_POINT('',#203086);
#40466=VERTEX_POINT('',#203087);
#40467=VERTEX_POINT('',#203095);
#40468=VERTEX_POINT('',#203096);
#40469=VERTEX_POINT('',#203098);
#40470=VERTEX_POINT('',#203100);
#40471=VERTEX_POINT('',#203104);
#40472=VERTEX_POINT('',#203105);
#40473=VERTEX_POINT('',#203110);
#40474=VERTEX_POINT('',#203111);
#40475=VERTEX_POINT('',#203119);
#40476=VERTEX_POINT('',#203120);
#40477=VERTEX_POINT('',#203122);
#40478=VERTEX_POINT('',#203124);
#40479=VERTEX_POINT('',#203128);
#40480=VERTEX_POINT('',#203129);
#40481=VERTEX_POINT('',#203134);
#40482=VERTEX_POINT('',#203135);
#40483=VERTEX_POINT('',#203143);
#40484=VERTEX_POINT('',#203144);
#40485=VERTEX_POINT('',#203146);
#40486=VERTEX_POINT('',#203148);
#40487=VERTEX_POINT('',#203152);
#40488=VERTEX_POINT('',#203153);
#40489=VERTEX_POINT('',#203158);
#40490=VERTEX_POINT('',#203159);
#40491=VERTEX_POINT('',#203167);
#40492=VERTEX_POINT('',#203168);
#40493=VERTEX_POINT('',#203170);
#40494=VERTEX_POINT('',#203172);
#40495=VERTEX_POINT('',#203176);
#40496=VERTEX_POINT('',#203177);
#40497=VERTEX_POINT('',#203182);
#40498=VERTEX_POINT('',#203183);
#40499=VERTEX_POINT('',#203191);
#40500=VERTEX_POINT('',#203192);
#40501=VERTEX_POINT('',#203194);
#40502=VERTEX_POINT('',#203196);
#40503=VERTEX_POINT('',#203200);
#40504=VERTEX_POINT('',#203201);
#40505=VERTEX_POINT('',#203206);
#40506=VERTEX_POINT('',#203207);
#40507=VERTEX_POINT('',#203215);
#40508=VERTEX_POINT('',#203216);
#40509=VERTEX_POINT('',#203218);
#40510=VERTEX_POINT('',#203220);
#40511=VERTEX_POINT('',#203224);
#40512=VERTEX_POINT('',#203225);
#40513=VERTEX_POINT('',#203230);
#40514=VERTEX_POINT('',#203231);
#40515=VERTEX_POINT('',#203239);
#40516=VERTEX_POINT('',#203240);
#40517=VERTEX_POINT('',#203242);
#40518=VERTEX_POINT('',#203244);
#40519=VERTEX_POINT('',#203248);
#40520=VERTEX_POINT('',#203249);
#40521=VERTEX_POINT('',#203254);
#40522=VERTEX_POINT('',#203255);
#40523=VERTEX_POINT('',#203263);
#40524=VERTEX_POINT('',#203264);
#40525=VERTEX_POINT('',#203266);
#40526=VERTEX_POINT('',#203268);
#40527=VERTEX_POINT('',#203272);
#40528=VERTEX_POINT('',#203273);
#40529=VERTEX_POINT('',#203278);
#40530=VERTEX_POINT('',#203279);
#40531=VERTEX_POINT('',#203287);
#40532=VERTEX_POINT('',#203288);
#40533=VERTEX_POINT('',#203290);
#40534=VERTEX_POINT('',#203292);
#40535=VERTEX_POINT('',#203296);
#40536=VERTEX_POINT('',#203297);
#40537=VERTEX_POINT('',#203302);
#40538=VERTEX_POINT('',#203303);
#40539=VERTEX_POINT('',#203311);
#40540=VERTEX_POINT('',#203312);
#40541=VERTEX_POINT('',#203314);
#40542=VERTEX_POINT('',#203316);
#40543=VERTEX_POINT('',#203320);
#40544=VERTEX_POINT('',#203321);
#40545=VERTEX_POINT('',#203326);
#40546=VERTEX_POINT('',#203327);
#40547=VERTEX_POINT('',#203335);
#40548=VERTEX_POINT('',#203336);
#40549=VERTEX_POINT('',#203338);
#40550=VERTEX_POINT('',#203340);
#40551=VERTEX_POINT('',#203344);
#40552=VERTEX_POINT('',#203345);
#40553=VERTEX_POINT('',#203350);
#40554=VERTEX_POINT('',#203351);
#40555=VERTEX_POINT('',#203359);
#40556=VERTEX_POINT('',#203360);
#40557=VERTEX_POINT('',#203362);
#40558=VERTEX_POINT('',#203364);
#40559=VERTEX_POINT('',#203368);
#40560=VERTEX_POINT('',#203369);
#40561=VERTEX_POINT('',#203374);
#40562=VERTEX_POINT('',#203375);
#40563=VERTEX_POINT('',#203383);
#40564=VERTEX_POINT('',#203384);
#40565=VERTEX_POINT('',#203386);
#40566=VERTEX_POINT('',#203388);
#40567=VERTEX_POINT('',#203392);
#40568=VERTEX_POINT('',#203393);
#40569=VERTEX_POINT('',#203398);
#40570=VERTEX_POINT('',#203399);
#40571=VERTEX_POINT('',#203407);
#40572=VERTEX_POINT('',#203408);
#40573=VERTEX_POINT('',#203410);
#40574=VERTEX_POINT('',#203412);
#40575=VERTEX_POINT('',#203416);
#40576=VERTEX_POINT('',#203417);
#40577=VERTEX_POINT('',#203422);
#40578=VERTEX_POINT('',#203423);
#40579=VERTEX_POINT('',#203431);
#40580=VERTEX_POINT('',#203432);
#40581=VERTEX_POINT('',#203434);
#40582=VERTEX_POINT('',#203436);
#40583=VERTEX_POINT('',#203440);
#40584=VERTEX_POINT('',#203441);
#40585=VERTEX_POINT('',#203446);
#40586=VERTEX_POINT('',#203447);
#40587=VERTEX_POINT('',#203455);
#40588=VERTEX_POINT('',#203456);
#40589=VERTEX_POINT('',#203458);
#40590=VERTEX_POINT('',#203460);
#40591=VERTEX_POINT('',#203464);
#40592=VERTEX_POINT('',#203465);
#40593=VERTEX_POINT('',#203470);
#40594=VERTEX_POINT('',#203471);
#40595=VERTEX_POINT('',#203479);
#40596=VERTEX_POINT('',#203480);
#40597=VERTEX_POINT('',#203482);
#40598=VERTEX_POINT('',#203484);
#40599=VERTEX_POINT('',#203488);
#40600=VERTEX_POINT('',#203489);
#40601=VERTEX_POINT('',#203494);
#40602=VERTEX_POINT('',#203495);
#40603=VERTEX_POINT('',#203503);
#40604=VERTEX_POINT('',#203504);
#40605=VERTEX_POINT('',#203506);
#40606=VERTEX_POINT('',#203508);
#40607=VERTEX_POINT('',#203512);
#40608=VERTEX_POINT('',#203513);
#40609=VERTEX_POINT('',#203518);
#40610=VERTEX_POINT('',#203519);
#40611=VERTEX_POINT('',#203527);
#40612=VERTEX_POINT('',#203528);
#40613=VERTEX_POINT('',#203530);
#40614=VERTEX_POINT('',#203532);
#40615=VERTEX_POINT('',#203536);
#40616=VERTEX_POINT('',#203537);
#40617=VERTEX_POINT('',#203542);
#40618=VERTEX_POINT('',#203543);
#40619=VERTEX_POINT('',#203551);
#40620=VERTEX_POINT('',#203552);
#40621=VERTEX_POINT('',#203554);
#40622=VERTEX_POINT('',#203556);
#40623=VERTEX_POINT('',#203560);
#40624=VERTEX_POINT('',#203561);
#40625=VERTEX_POINT('',#203566);
#40626=VERTEX_POINT('',#203567);
#40627=VERTEX_POINT('',#203575);
#40628=VERTEX_POINT('',#203576);
#40629=VERTEX_POINT('',#203578);
#40630=VERTEX_POINT('',#203580);
#40631=VERTEX_POINT('',#203584);
#40632=VERTEX_POINT('',#203585);
#40633=VERTEX_POINT('',#203590);
#40634=VERTEX_POINT('',#203591);
#40635=VERTEX_POINT('',#203599);
#40636=VERTEX_POINT('',#203600);
#40637=VERTEX_POINT('',#203602);
#40638=VERTEX_POINT('',#203604);
#40639=VERTEX_POINT('',#203608);
#40640=VERTEX_POINT('',#203609);
#40641=VERTEX_POINT('',#203614);
#40642=VERTEX_POINT('',#203615);
#40643=VERTEX_POINT('',#203623);
#40644=VERTEX_POINT('',#203624);
#40645=VERTEX_POINT('',#203626);
#40646=VERTEX_POINT('',#203628);
#40647=VERTEX_POINT('',#203632);
#40648=VERTEX_POINT('',#203633);
#40649=VERTEX_POINT('',#203638);
#40650=VERTEX_POINT('',#203639);
#40651=VERTEX_POINT('',#203647);
#40652=VERTEX_POINT('',#203648);
#40653=VERTEX_POINT('',#203650);
#40654=VERTEX_POINT('',#203652);
#40655=VERTEX_POINT('',#203656);
#40656=VERTEX_POINT('',#203657);
#40657=VERTEX_POINT('',#203662);
#40658=VERTEX_POINT('',#203663);
#40659=VERTEX_POINT('',#203671);
#40660=VERTEX_POINT('',#203672);
#40661=VERTEX_POINT('',#203674);
#40662=VERTEX_POINT('',#203676);
#40663=VERTEX_POINT('',#203680);
#40664=VERTEX_POINT('',#203681);
#40665=VERTEX_POINT('',#203686);
#40666=VERTEX_POINT('',#203687);
#40667=VERTEX_POINT('',#203695);
#40668=VERTEX_POINT('',#203696);
#40669=VERTEX_POINT('',#203698);
#40670=VERTEX_POINT('',#203700);
#40671=VERTEX_POINT('',#203704);
#40672=VERTEX_POINT('',#203705);
#40673=VERTEX_POINT('',#203710);
#40674=VERTEX_POINT('',#203711);
#40675=VERTEX_POINT('',#203719);
#40676=VERTEX_POINT('',#203720);
#40677=VERTEX_POINT('',#203722);
#40678=VERTEX_POINT('',#203724);
#40679=VERTEX_POINT('',#203728);
#40680=VERTEX_POINT('',#203729);
#40681=VERTEX_POINT('',#203734);
#40682=VERTEX_POINT('',#203735);
#40683=VERTEX_POINT('',#203743);
#40684=VERTEX_POINT('',#203744);
#40685=VERTEX_POINT('',#203746);
#40686=VERTEX_POINT('',#203748);
#40687=VERTEX_POINT('',#203752);
#40688=VERTEX_POINT('',#203753);
#40689=VERTEX_POINT('',#203758);
#40690=VERTEX_POINT('',#203759);
#40691=VERTEX_POINT('',#203767);
#40692=VERTEX_POINT('',#203768);
#40693=VERTEX_POINT('',#203770);
#40694=VERTEX_POINT('',#203772);
#40695=VERTEX_POINT('',#203776);
#40696=VERTEX_POINT('',#203777);
#40697=VERTEX_POINT('',#203782);
#40698=VERTEX_POINT('',#203783);
#40699=VERTEX_POINT('',#203791);
#40700=VERTEX_POINT('',#203792);
#40701=VERTEX_POINT('',#203794);
#40702=VERTEX_POINT('',#203796);
#40703=VERTEX_POINT('',#203800);
#40704=VERTEX_POINT('',#203801);
#40705=VERTEX_POINT('',#203806);
#40706=VERTEX_POINT('',#203807);
#40707=VERTEX_POINT('',#203815);
#40708=VERTEX_POINT('',#203816);
#40709=VERTEX_POINT('',#203818);
#40710=VERTEX_POINT('',#203820);
#40711=VERTEX_POINT('',#203824);
#40712=VERTEX_POINT('',#203825);
#40713=VERTEX_POINT('',#203830);
#40714=VERTEX_POINT('',#203831);
#40715=VERTEX_POINT('',#203839);
#40716=VERTEX_POINT('',#203840);
#40717=VERTEX_POINT('',#203842);
#40718=VERTEX_POINT('',#203844);
#40719=VERTEX_POINT('',#203848);
#40720=VERTEX_POINT('',#203849);
#40721=VERTEX_POINT('',#203854);
#40722=VERTEX_POINT('',#203855);
#40723=VERTEX_POINT('',#203863);
#40724=VERTEX_POINT('',#203864);
#40725=VERTEX_POINT('',#203866);
#40726=VERTEX_POINT('',#203868);
#40727=VERTEX_POINT('',#203872);
#40728=VERTEX_POINT('',#203873);
#40729=VERTEX_POINT('',#203878);
#40730=VERTEX_POINT('',#203879);
#40731=VERTEX_POINT('',#203888);
#40732=VERTEX_POINT('',#203889);
#40733=VERTEX_POINT('',#203891);
#40734=VERTEX_POINT('',#203893);
#40735=VERTEX_POINT('',#203897);
#40736=VERTEX_POINT('',#203899);
#40737=VERTEX_POINT('',#203903);
#40738=VERTEX_POINT('',#203907);
#40739=VERTEX_POINT('',#203935);
#40740=VERTEX_POINT('',#203938);
#40741=VERTEX_POINT('',#203939);
#40742=VERTEX_POINT('',#203941);
#40743=VERTEX_POINT('',#203943);
#40744=VERTEX_POINT('',#203947);
#40745=VERTEX_POINT('',#203949);
#40746=VERTEX_POINT('',#203953);
#40747=VERTEX_POINT('',#203957);
#40748=VERTEX_POINT('',#203963);
#43418=EDGE_CURVE('',#35028,#35029,#3226,.T.);
#43419=EDGE_CURVE('',#35028,#35030,#30298,.T.);
#43420=EDGE_CURVE('',#35030,#35029,#31407,.T.);
#43421=EDGE_CURVE('',#35031,#35032,#3227,.T.);
#43422=EDGE_CURVE('',#35028,#35031,#30299,.T.);
#43423=EDGE_CURVE('',#35029,#35033,#31408,.T.);
#43424=EDGE_CURVE('',#35032,#35033,#30300,.F.);
#43425=EDGE_CURVE('',#35034,#35035,#3228,.T.);
#43426=EDGE_CURVE('',#35031,#35034,#30301,.T.);
#43427=EDGE_CURVE('',#35032,#35035,#30302,.F.);
#43428=EDGE_CURVE('',#35036,#35037,#3229,.T.);
#43429=EDGE_CURVE('',#35038,#35036,#31409,.T.);
#43430=EDGE_CURVE('',#35034,#35038,#30303,.T.);
#43431=EDGE_CURVE('',#35035,#35037,#30304,.F.);
#43432=EDGE_CURVE('',#35039,#35040,#31410,.T.);
#43433=EDGE_CURVE('',#35040,#35041,#3230,.T.);
#43434=EDGE_CURVE('',#35041,#35041,#31411,.T.);
#43435=EDGE_CURVE('',#35040,#35039,#31412,.T.);
#43436=EDGE_CURVE('',#35039,#35042,#31413,.T.);
#43437=EDGE_CURVE('',#35042,#35042,#31414,.T.);
#43438=EDGE_CURVE('',#35042,#35043,#31415,.T.);
#43439=EDGE_CURVE('',#35043,#35043,#31416,.T.);
#43440=EDGE_CURVE('',#35044,#35045,#30305,.F.);
#43441=EDGE_CURVE('',#35044,#35046,#3231,.T.);
#43442=EDGE_CURVE('',#35047,#35046,#30306,.F.);
#43443=EDGE_CURVE('',#35045,#35047,#3232,.T.);
#43444=EDGE_CURVE('',#35048,#35049,#30307,.F.);
#43445=EDGE_CURVE('',#35048,#35050,#3233,.T.);
#43446=EDGE_CURVE('',#35051,#35050,#30308,.F.);
#43447=EDGE_CURVE('',#35049,#35051,#3234,.T.);
#43448=EDGE_CURVE('',#35043,#35052,#3235,.T.);
#43449=EDGE_CURVE('',#35052,#35053,#31417,.T.);
#43450=EDGE_CURVE('',#35053,#35054,#30309,.T.);
#43451=EDGE_CURVE('',#35055,#35054,#31418,.T.);
#43452=EDGE_CURVE('',#35055,#35056,#3236,.T.);
#43453=EDGE_CURVE('',#35056,#35056,#31419,.T.);
#43454=EDGE_CURVE('',#35044,#35055,#31420,.T.);
#43455=EDGE_CURVE('',#35045,#35052,#31421,.T.);
#43456=EDGE_CURVE('',#35057,#35058,#31422,.T.);
#43457=EDGE_CURVE('',#35057,#35059,#30310,.T.);
#43458=EDGE_CURVE('',#35059,#35060,#31423,.T.);
#43459=EDGE_CURVE('',#35060,#35058,#30311,.T.);
#43460=EDGE_CURVE('',#35061,#35062,#31424,.T.);
#43461=EDGE_CURVE('',#35062,#35063,#30312,.T.);
#43462=EDGE_CURVE('',#35064,#35063,#31425,.T.);
#43463=EDGE_CURVE('',#35064,#35061,#30313,.T.);
#43464=EDGE_CURVE('',#35065,#35050,#31426,.T.);
#43465=EDGE_CURVE('',#35065,#35066,#30314,.T.);
#43466=EDGE_CURVE('',#35066,#35051,#31427,.T.);
#43467=EDGE_CURVE('',#35067,#35068,#30315,.F.);
#43468=EDGE_CURVE('',#35067,#35063,#3237,.T.);
#43469=EDGE_CURVE('',#35068,#35062,#3238,.T.);
#43470=EDGE_CURVE('',#35057,#35069,#3239,.T.);
#43471=EDGE_CURVE('',#35070,#35069,#30316,.F.);
#43472=EDGE_CURVE('',#35059,#35070,#3240,.T.);
#43473=EDGE_CURVE('',#35071,#35071,#31428,.T.);
#43474=EDGE_CURVE('',#35071,#35072,#3241,.T.);
#43475=EDGE_CURVE('',#35072,#35073,#31429,.T.);
#43476=EDGE_CURVE('',#35073,#35074,#30317,.T.);
#43477=EDGE_CURVE('',#35075,#35074,#31430,.T.);
#43478=EDGE_CURVE('',#35075,#35076,#3242,.T.);
#43479=EDGE_CURVE('',#35076,#35076,#31431,.T.);
#43480=EDGE_CURVE('',#35047,#35075,#31432,.T.);
#43481=EDGE_CURVE('',#35046,#35072,#31433,.T.);
#43482=EDGE_CURVE('',#35077,#35067,#31434,.T.);
#43483=EDGE_CURVE('',#35078,#35068,#31435,.T.);
#43484=EDGE_CURVE('',#35078,#35077,#30318,.T.);
#43485=EDGE_CURVE('',#35070,#35079,#31436,.T.);
#43486=EDGE_CURVE('',#35069,#35080,#31437,.T.);
#43487=EDGE_CURVE('',#35080,#35079,#30319,.T.);
#43488=EDGE_CURVE('',#35081,#35048,#31438,.T.);
#43489=EDGE_CURVE('',#35082,#35049,#31439,.T.);
#43490=EDGE_CURVE('',#35082,#35081,#30320,.T.);
#43491=EDGE_CURVE('',#35083,#35083,#31440,.T.);
#43492=EDGE_CURVE('',#35083,#35071,#31441,.T.);
#43493=EDGE_CURVE('',#35084,#35084,#31442,.T.);
#43494=EDGE_CURVE('',#35084,#35085,#3243,.T.);
#43495=EDGE_CURVE('',#35085,#35085,#31443,.T.);
#43496=EDGE_CURVE('',#35086,#35086,#31444,.T.);
#43497=EDGE_CURVE('',#35086,#35087,#3244,.T.);
#43498=EDGE_CURVE('',#35087,#35087,#31445,.T.);
#43499=EDGE_CURVE('',#35076,#35088,#31446,.T.);
#43500=EDGE_CURVE('',#35088,#35088,#31447,.T.);
#43501=EDGE_CURVE('',#35088,#35089,#31448,.T.);
#43502=EDGE_CURVE('',#35090,#35089,#31449,.T.);
#43503=EDGE_CURVE('',#35089,#35090,#31450,.T.);
#43504=EDGE_CURVE('',#35091,#35091,#31451,.T.);
#43505=EDGE_CURVE('',#35091,#35090,#3245,.T.);
#43506=EDGE_CURVE('',#35092,#35092,#31452,.T.);
#43507=EDGE_CURVE('',#35092,#35093,#3246,.T.);
#43508=EDGE_CURVE('',#35093,#35093,#31453,.T.);
#43509=EDGE_CURVE('',#35094,#35094,#31454,.T.);
#43510=EDGE_CURVE('',#35094,#35095,#3247,.T.);
#43511=EDGE_CURVE('',#35095,#35095,#31455,.T.);
#43512=EDGE_CURVE('',#35096,#35096,#31456,.T.);
#43513=EDGE_CURVE('',#35096,#35097,#3248,.T.);
#43514=EDGE_CURVE('',#35097,#35097,#31457,.T.);
#43515=EDGE_CURVE('',#35098,#35099,#31458,.T.);
#43516=EDGE_CURVE('',#35100,#35099,#3249,.T.);
#43517=EDGE_CURVE('',#35101,#35100,#31459,.T.);
#43518=EDGE_CURVE('',#35101,#35102,#3250,.T.);
#43519=EDGE_CURVE('',#35102,#35103,#31460,.T.);
#43520=EDGE_CURVE('',#35103,#35104,#3251,.T.);
#43521=EDGE_CURVE('',#35105,#35104,#31461,.T.);
#43522=EDGE_CURVE('',#35105,#35106,#3252,.T.);
#43523=EDGE_CURVE('',#35106,#35106,#31462,.T.);
#43524=EDGE_CURVE('',#35107,#35105,#31463,.T.);
#43525=EDGE_CURVE('',#35098,#35107,#3253,.T.);
#43526=EDGE_CURVE('',#35108,#35030,#30321,.F.);
#43527=EDGE_CURVE('',#35109,#35108,#31464,.T.);
#43528=EDGE_CURVE('',#35109,#35110,#30322,.T.);
#43529=EDGE_CURVE('',#35110,#35033,#30323,.T.);
#43530=EDGE_CURVE('',#35111,#35111,#31465,.T.);
#43531=EDGE_CURVE('',#35111,#35112,#3254,.T.);
#43532=EDGE_CURVE('',#35112,#35112,#31466,.T.);
#43533=EDGE_CURVE('',#35113,#35114,#30324,.T.);
#43534=EDGE_CURVE('',#35115,#35114,#30325,.T.);
#43535=EDGE_CURVE('',#35116,#35115,#30326,.T.);
#43536=EDGE_CURVE('',#35037,#35116,#30327,.F.);
#43537=EDGE_CURVE('',#35113,#35032,#3255,.T.);
#43538=EDGE_CURVE('',#35117,#35113,#3256,.T.);
#43539=EDGE_CURVE('',#35118,#35113,#30328,.T.);
#43540=EDGE_CURVE('',#35119,#35118,#30329,.T.);
#43541=EDGE_CURVE('',#35119,#35120,#30330,.T.);
#43542=EDGE_CURVE('',#35120,#35117,#30331,.T.);
#43543=EDGE_CURVE('',#35117,#35121,#30332,.T.);
#43544=EDGE_CURVE('',#35122,#35121,#30333,.T.);
#43545=EDGE_CURVE('',#35114,#35122,#30334,.T.);
#43546=EDGE_CURVE('',#35102,#35123,#1802,.T.);
#43547=EDGE_CURVE('',#35100,#35101,#3257,.T.);
#43548=EDGE_CURVE('',#35124,#35099,#1803,.T.);
#43549=EDGE_CURVE('',#35124,#35123,#3258,.T.);
#43550=EDGE_CURVE('',#35125,#35103,#1804,.T.);
#43551=EDGE_CURVE('',#35125,#35123,#31467,.T.);
#43552=EDGE_CURVE('',#35098,#35126,#1805,.T.);
#43553=EDGE_CURVE('',#35124,#35126,#31468,.T.);
#43554=EDGE_CURVE('',#35104,#35107,#3259,.T.);
#43555=EDGE_CURVE('',#35125,#35126,#3260,.T.);
#43556=EDGE_CURVE('',#35121,#35127,#30335,.T.);
#43557=EDGE_CURVE('',#35127,#35038,#30336,.T.);
#43558=EDGE_CURVE('',#35036,#35116,#31469,.T.);
#43559=EDGE_CURVE('',#35028,#35117,#3261,.T.);
#43560=EDGE_CURVE('',#35118,#35109,#30337,.T.);
#43561=EDGE_CURVE('',#35128,#35120,#30338,.T.);
#43562=EDGE_CURVE('',#35128,#35108,#30339,.T.);
#43563=EDGE_CURVE('',#35129,#35130,#31470,.T.);
#43564=EDGE_CURVE('',#35131,#35129,#3262,.T.);
#43565=EDGE_CURVE('',#35132,#35131,#3263,.T.);
#43566=EDGE_CURVE('',#35132,#35130,#3264,.T.);
#43567=EDGE_CURVE('',#35133,#35132,#3265,.T.);
#43568=EDGE_CURVE('',#35133,#35134,#31471,.T.);
#43569=EDGE_CURVE('',#35134,#35135,#3266,.T.);
#43570=EDGE_CURVE('',#35130,#35135,#31472,.T.);
#43571=EDGE_CURVE('',#35135,#35136,#31473,.T.);
#43572=EDGE_CURVE('',#35134,#35137,#31474,.T.);
#43573=EDGE_CURVE('',#35137,#35136,#3267,.T.);
#43574=EDGE_CURVE('',#35136,#35129,#31475,.T.);
#43575=EDGE_CURVE('',#35137,#35138,#31476,.T.);
#43576=EDGE_CURVE('',#35131,#35138,#3268,.T.);
#43577=EDGE_CURVE('',#35138,#35133,#31477,.T.);
#43578=EDGE_CURVE('',#35139,#35140,#31478,.T.);
#43579=EDGE_CURVE('',#35141,#35139,#3269,.T.);
#43580=EDGE_CURVE('',#35142,#35141,#3270,.T.);
#43581=EDGE_CURVE('',#35142,#35140,#3271,.T.);
#43582=EDGE_CURVE('',#35143,#35144,#31479,.T.);
#43583=EDGE_CURVE('',#35144,#35145,#3272,.T.);
#43584=EDGE_CURVE('',#35140,#35145,#31480,.T.);
#43585=EDGE_CURVE('',#35143,#35142,#3273,.T.);
#43586=EDGE_CURVE('',#35145,#35146,#31481,.T.);
#43587=EDGE_CURVE('',#35144,#35147,#31482,.T.);
#43588=EDGE_CURVE('',#35147,#35146,#3274,.T.);
#43589=EDGE_CURVE('',#35146,#35139,#31483,.T.);
#43590=EDGE_CURVE('',#35147,#35148,#31484,.T.);
#43591=EDGE_CURVE('',#35141,#35148,#3275,.T.);
#43592=EDGE_CURVE('',#35148,#35143,#31485,.T.);
#43593=EDGE_CURVE('',#35149,#35150,#3276,.T.);
#43594=EDGE_CURVE('',#35149,#35151,#31486,.T.);
#43595=EDGE_CURVE('',#35151,#35152,#3277,.T.);
#43596=EDGE_CURVE('',#35150,#35152,#31487,.T.);
#43597=EDGE_CURVE('',#35153,#35154,#3278,.T.);
#43598=EDGE_CURVE('',#35149,#35153,#3279,.T.);
#43599=EDGE_CURVE('',#35154,#35150,#31488,.T.);
#43600=EDGE_CURVE('',#35155,#35156,#3280,.T.);
#43601=EDGE_CURVE('',#35153,#35155,#3281,.T.);
#43602=EDGE_CURVE('',#35156,#35154,#31489,.T.);
#43603=EDGE_CURVE('',#35151,#35157,#31490,.T.);
#43604=EDGE_CURVE('',#35155,#35157,#3282,.T.);
#43605=EDGE_CURVE('',#35152,#35156,#31491,.T.);
#43606=EDGE_CURVE('',#35157,#35149,#31492,.T.);
#43607=EDGE_CURVE('',#35158,#35159,#3283,.T.);
#43608=EDGE_CURVE('',#35158,#35160,#31493,.T.);
#43609=EDGE_CURVE('',#35160,#35161,#3284,.T.);
#43610=EDGE_CURVE('',#35159,#35161,#31494,.T.);
#43611=EDGE_CURVE('',#35162,#35163,#3285,.T.);
#43612=EDGE_CURVE('',#35162,#35158,#31495,.T.);
#43613=EDGE_CURVE('',#35163,#35159,#31496,.T.);
#43614=EDGE_CURVE('',#35164,#35165,#3286,.T.);
#43615=EDGE_CURVE('',#35164,#35162,#31497,.T.);
#43616=EDGE_CURVE('',#35165,#35163,#31498,.T.);
#43617=EDGE_CURVE('',#35160,#35164,#31499,.T.);
#43618=EDGE_CURVE('',#35161,#35165,#31500,.T.);
#43619=EDGE_CURVE('',#35166,#35167,#3287,.T.);
#43620=EDGE_CURVE('',#35166,#35168,#31501,.T.);
#43621=EDGE_CURVE('',#35168,#35169,#3288,.T.);
#43622=EDGE_CURVE('',#35167,#35169,#31502,.T.);
#43623=EDGE_CURVE('',#35170,#35171,#3289,.T.);
#43624=EDGE_CURVE('',#35170,#35166,#31503,.T.);
#43625=EDGE_CURVE('',#35171,#35167,#31504,.T.);
#43626=EDGE_CURVE('',#35172,#35173,#3290,.T.);
#43627=EDGE_CURVE('',#35172,#35170,#31505,.T.);
#43628=EDGE_CURVE('',#35173,#35171,#31506,.T.);
#43629=EDGE_CURVE('',#35168,#35172,#31507,.T.);
#43630=EDGE_CURVE('',#35169,#35173,#31508,.T.);
#43631=EDGE_CURVE('',#35174,#35175,#3291,.T.);
#43632=EDGE_CURVE('',#35174,#35176,#31509,.T.);
#43633=EDGE_CURVE('',#35176,#35177,#3292,.T.);
#43634=EDGE_CURVE('',#35175,#35177,#31510,.T.);
#43635=EDGE_CURVE('',#35178,#35179,#3293,.T.);
#43636=EDGE_CURVE('',#35178,#35174,#31511,.T.);
#43637=EDGE_CURVE('',#35179,#35175,#31512,.T.);
#43638=EDGE_CURVE('',#35180,#35181,#3294,.T.);
#43639=EDGE_CURVE('',#35180,#35178,#31513,.T.);
#43640=EDGE_CURVE('',#35181,#35179,#31514,.T.);
#43641=EDGE_CURVE('',#35176,#35180,#31515,.T.);
#43642=EDGE_CURVE('',#35177,#35181,#31516,.T.);
#43643=EDGE_CURVE('',#35182,#35183,#3295,.T.);
#43644=EDGE_CURVE('',#35182,#35184,#31517,.T.);
#43645=EDGE_CURVE('',#35184,#35185,#3296,.T.);
#43646=EDGE_CURVE('',#35183,#35185,#31518,.T.);
#43647=EDGE_CURVE('',#35186,#35187,#3297,.T.);
#43648=EDGE_CURVE('',#35186,#35182,#31519,.T.);
#43649=EDGE_CURVE('',#35187,#35183,#31520,.T.);
#43650=EDGE_CURVE('',#35188,#35189,#3298,.T.);
#43651=EDGE_CURVE('',#35188,#35186,#31521,.T.);
#43652=EDGE_CURVE('',#35189,#35187,#31522,.T.);
#43653=EDGE_CURVE('',#35184,#35188,#31523,.T.);
#43654=EDGE_CURVE('',#35185,#35189,#31524,.T.);
#43655=EDGE_CURVE('',#35190,#35191,#31525,.T.);
#43656=EDGE_CURVE('',#35192,#35190,#3299,.T.);
#43657=EDGE_CURVE('',#35193,#35192,#3300,.T.);
#43658=EDGE_CURVE('',#35193,#35191,#3301,.T.);
#43659=EDGE_CURVE('',#35194,#35195,#31526,.T.);
#43660=EDGE_CURVE('',#35195,#35196,#3302,.T.);
#43661=EDGE_CURVE('',#35191,#35196,#31527,.T.);
#43662=EDGE_CURVE('',#35194,#35193,#3303,.T.);
#43663=EDGE_CURVE('',#35196,#35197,#31528,.T.);
#43664=EDGE_CURVE('',#35195,#35198,#31529,.T.);
#43665=EDGE_CURVE('',#35198,#35197,#3304,.T.);
#43666=EDGE_CURVE('',#35197,#35190,#31530,.T.);
#43667=EDGE_CURVE('',#35198,#35199,#31531,.T.);
#43668=EDGE_CURVE('',#35192,#35199,#3305,.T.);
#43669=EDGE_CURVE('',#35199,#35194,#31532,.T.);
#43670=EDGE_CURVE('',#35200,#35201,#3306,.T.);
#43671=EDGE_CURVE('',#35200,#35202,#31533,.T.);
#43672=EDGE_CURVE('',#35202,#35203,#3307,.T.);
#43673=EDGE_CURVE('',#35201,#35203,#31534,.T.);
#43674=EDGE_CURVE('',#35204,#35205,#3308,.T.);
#43675=EDGE_CURVE('',#35206,#35204,#3309,.T.);
#43676=EDGE_CURVE('',#35206,#35200,#31535,.T.);
#43677=EDGE_CURVE('',#35205,#35201,#31536,.T.);
#43678=EDGE_CURVE('',#35207,#35208,#3310,.T.);
#43679=EDGE_CURVE('',#35204,#35207,#3311,.T.);
#43680=EDGE_CURVE('',#35208,#35205,#31537,.T.);
#43681=EDGE_CURVE('',#35202,#35209,#31538,.T.);
#43682=EDGE_CURVE('',#35207,#35209,#3312,.T.);
#43683=EDGE_CURVE('',#35203,#35208,#31539,.T.);
#43684=EDGE_CURVE('',#35209,#35206,#31540,.T.);
#43685=EDGE_CURVE('',#35210,#35211,#3313,.T.);
#43686=EDGE_CURVE('',#35210,#35212,#31541,.T.);
#43687=EDGE_CURVE('',#35212,#35213,#3314,.T.);
#43688=EDGE_CURVE('',#35211,#35213,#31542,.T.);
#43689=EDGE_CURVE('',#35214,#35215,#3315,.T.);
#43690=EDGE_CURVE('',#35216,#35214,#3316,.T.);
#43691=EDGE_CURVE('',#35216,#35210,#31543,.T.);
#43692=EDGE_CURVE('',#35215,#35211,#31544,.T.);
#43693=EDGE_CURVE('',#35217,#35218,#3317,.T.);
#43694=EDGE_CURVE('',#35214,#35217,#3318,.T.);
#43695=EDGE_CURVE('',#35218,#35215,#31545,.T.);
#43696=EDGE_CURVE('',#35212,#35219,#31546,.T.);
#43697=EDGE_CURVE('',#35217,#35219,#3319,.T.);
#43698=EDGE_CURVE('',#35213,#35218,#31547,.T.);
#43699=EDGE_CURVE('',#35219,#35216,#31548,.T.);
#43700=EDGE_CURVE('',#35220,#35221,#3320,.T.);
#43701=EDGE_CURVE('',#35220,#35222,#31549,.T.);
#43702=EDGE_CURVE('',#35222,#35223,#3321,.T.);
#43703=EDGE_CURVE('',#35221,#35223,#31550,.T.);
#43704=EDGE_CURVE('',#35224,#35225,#3322,.T.);
#43705=EDGE_CURVE('',#35224,#35220,#31551,.T.);
#43706=EDGE_CURVE('',#35225,#35221,#31552,.T.);
#43707=EDGE_CURVE('',#35226,#35227,#3323,.T.);
#43708=EDGE_CURVE('',#35228,#35226,#3324,.T.);
#43709=EDGE_CURVE('',#35228,#35224,#31553,.T.);
#43710=EDGE_CURVE('',#35227,#35225,#31554,.T.);
#43711=EDGE_CURVE('',#35222,#35229,#31555,.T.);
#43712=EDGE_CURVE('',#35226,#35229,#3325,.T.);
#43713=EDGE_CURVE('',#35223,#35227,#31556,.T.);
#43714=EDGE_CURVE('',#35229,#35228,#31557,.T.);
#43715=EDGE_CURVE('',#35230,#35231,#3326,.T.);
#43716=EDGE_CURVE('',#35230,#35232,#31558,.T.);
#43717=EDGE_CURVE('',#35232,#35233,#3327,.T.);
#43718=EDGE_CURVE('',#35231,#35233,#31559,.T.);
#43719=EDGE_CURVE('',#35234,#35235,#3328,.T.);
#43720=EDGE_CURVE('',#35234,#35230,#31560,.T.);
#43721=EDGE_CURVE('',#35235,#35231,#31561,.T.);
#43722=EDGE_CURVE('',#35236,#35237,#3329,.T.);
#43723=EDGE_CURVE('',#35236,#35234,#31562,.T.);
#43724=EDGE_CURVE('',#35237,#35235,#31563,.T.);
#43725=EDGE_CURVE('',#35232,#35236,#31564,.T.);
#43726=EDGE_CURVE('',#35233,#35237,#31565,.T.);
#43727=EDGE_CURVE('',#35238,#35239,#3330,.T.);
#43728=EDGE_CURVE('',#35238,#35240,#31566,.T.);
#43729=EDGE_CURVE('',#35240,#35241,#3331,.T.);
#43730=EDGE_CURVE('',#35239,#35241,#31567,.T.);
#43731=EDGE_CURVE('',#35242,#35243,#3332,.T.);
#43732=EDGE_CURVE('',#35244,#35242,#3333,.T.);
#43733=EDGE_CURVE('',#35244,#35238,#31568,.T.);
#43734=EDGE_CURVE('',#35243,#35239,#31569,.T.);
#43735=EDGE_CURVE('',#35245,#35246,#3334,.T.);
#43736=EDGE_CURVE('',#35242,#35245,#3335,.T.);
#43737=EDGE_CURVE('',#35246,#35243,#31570,.T.);
#43738=EDGE_CURVE('',#35240,#35247,#31571,.T.);
#43739=EDGE_CURVE('',#35245,#35247,#3336,.T.);
#43740=EDGE_CURVE('',#35241,#35246,#31572,.T.);
#43741=EDGE_CURVE('',#35247,#35244,#31573,.T.);
#43742=EDGE_CURVE('',#35248,#35249,#3337,.T.);
#43743=EDGE_CURVE('',#35248,#35250,#31574,.T.);
#43744=EDGE_CURVE('',#35250,#35251,#3338,.T.);
#43745=EDGE_CURVE('',#35249,#35251,#31575,.T.);
#43746=EDGE_CURVE('',#35252,#35253,#3339,.T.);
#43747=EDGE_CURVE('',#35254,#35252,#3340,.T.);
#43748=EDGE_CURVE('',#35254,#35248,#31576,.T.);
#43749=EDGE_CURVE('',#35253,#35249,#31577,.T.);
#43750=EDGE_CURVE('',#35255,#35256,#3341,.T.);
#43751=EDGE_CURVE('',#35252,#35255,#3342,.T.);
#43752=EDGE_CURVE('',#35256,#35253,#31578,.T.);
#43753=EDGE_CURVE('',#35250,#35257,#31579,.T.);
#43754=EDGE_CURVE('',#35255,#35257,#3343,.T.);
#43755=EDGE_CURVE('',#35251,#35256,#31580,.T.);
#43756=EDGE_CURVE('',#35257,#35254,#31581,.T.);
#43757=EDGE_CURVE('',#35258,#35259,#3344,.T.);
#43758=EDGE_CURVE('',#35258,#35260,#31582,.T.);
#43759=EDGE_CURVE('',#35260,#35261,#3345,.T.);
#43760=EDGE_CURVE('',#35259,#35261,#31583,.T.);
#43761=EDGE_CURVE('',#35262,#35263,#3346,.T.);
#43762=EDGE_CURVE('',#35264,#35262,#3347,.T.);
#43763=EDGE_CURVE('',#35264,#35258,#31584,.T.);
#43764=EDGE_CURVE('',#35263,#35259,#31585,.T.);
#43765=EDGE_CURVE('',#35265,#35266,#3348,.T.);
#43766=EDGE_CURVE('',#35262,#35265,#3349,.T.);
#43767=EDGE_CURVE('',#35266,#35263,#31586,.T.);
#43768=EDGE_CURVE('',#35260,#35267,#31587,.T.);
#43769=EDGE_CURVE('',#35265,#35267,#3350,.T.);
#43770=EDGE_CURVE('',#35261,#35266,#31588,.T.);
#43771=EDGE_CURVE('',#35267,#35264,#31589,.T.);
#43772=EDGE_CURVE('',#35268,#35269,#3351,.T.);
#43773=EDGE_CURVE('',#35268,#35270,#31590,.T.);
#43774=EDGE_CURVE('',#35270,#35271,#3352,.T.);
#43775=EDGE_CURVE('',#35269,#35271,#31591,.T.);
#43776=EDGE_CURVE('',#35272,#35273,#3353,.T.);
#43777=EDGE_CURVE('',#35274,#35272,#3354,.T.);
#43778=EDGE_CURVE('',#35274,#35268,#31592,.T.);
#43779=EDGE_CURVE('',#35273,#35269,#31593,.T.);
#43780=EDGE_CURVE('',#35275,#35276,#3355,.T.);
#43781=EDGE_CURVE('',#35272,#35275,#3356,.T.);
#43782=EDGE_CURVE('',#35276,#35273,#31594,.T.);
#43783=EDGE_CURVE('',#35270,#35277,#31595,.T.);
#43784=EDGE_CURVE('',#35275,#35277,#3357,.T.);
#43785=EDGE_CURVE('',#35271,#35276,#31596,.T.);
#43786=EDGE_CURVE('',#35277,#35274,#31597,.T.);
#43787=EDGE_CURVE('',#35278,#35279,#3358,.T.);
#43788=EDGE_CURVE('',#35278,#35280,#31598,.T.);
#43789=EDGE_CURVE('',#35280,#35281,#3359,.T.);
#43790=EDGE_CURVE('',#35279,#35281,#31599,.T.);
#43791=EDGE_CURVE('',#35282,#35283,#3360,.T.);
#43792=EDGE_CURVE('',#35282,#35278,#31600,.T.);
#43793=EDGE_CURVE('',#35283,#35279,#31601,.T.);
#43794=EDGE_CURVE('',#35284,#35285,#3361,.T.);
#43795=EDGE_CURVE('',#35284,#35282,#31602,.T.);
#43796=EDGE_CURVE('',#35285,#35283,#31603,.T.);
#43797=EDGE_CURVE('',#35280,#35284,#31604,.T.);
#43798=EDGE_CURVE('',#35281,#35285,#31605,.T.);
#43799=EDGE_CURVE('',#35286,#35287,#3362,.T.);
#43800=EDGE_CURVE('',#35286,#35288,#31606,.T.);
#43801=EDGE_CURVE('',#35288,#35289,#3363,.T.);
#43802=EDGE_CURVE('',#35287,#35289,#31607,.T.);
#43803=EDGE_CURVE('',#35290,#35291,#3364,.T.);
#43804=EDGE_CURVE('',#35290,#35286,#31608,.T.);
#43805=EDGE_CURVE('',#35291,#35287,#31609,.T.);
#43806=EDGE_CURVE('',#35292,#35293,#3365,.T.);
#43807=EDGE_CURVE('',#35292,#35290,#31610,.T.);
#43808=EDGE_CURVE('',#35293,#35291,#31611,.T.);
#43809=EDGE_CURVE('',#35288,#35292,#31612,.T.);
#43810=EDGE_CURVE('',#35289,#35293,#31613,.T.);
#43811=EDGE_CURVE('',#35294,#35295,#3366,.T.);
#43812=EDGE_CURVE('',#35294,#35296,#31614,.T.);
#43813=EDGE_CURVE('',#35296,#35297,#3367,.T.);
#43814=EDGE_CURVE('',#35295,#35297,#31615,.T.);
#43815=EDGE_CURVE('',#35298,#35299,#3368,.T.);
#43816=EDGE_CURVE('',#35298,#35294,#31616,.T.);
#43817=EDGE_CURVE('',#35299,#35295,#31617,.T.);
#43818=EDGE_CURVE('',#35300,#35301,#3369,.T.);
#43819=EDGE_CURVE('',#35300,#35298,#31618,.T.);
#43820=EDGE_CURVE('',#35301,#35299,#31619,.T.);
#43821=EDGE_CURVE('',#35296,#35300,#31620,.T.);
#43822=EDGE_CURVE('',#35297,#35301,#31621,.T.);
#43823=EDGE_CURVE('',#35302,#35303,#3370,.T.);
#43824=EDGE_CURVE('',#35302,#35304,#31622,.T.);
#43825=EDGE_CURVE('',#35304,#35305,#3371,.T.);
#43826=EDGE_CURVE('',#35303,#35305,#31623,.T.);
#43827=EDGE_CURVE('',#35306,#35307,#3372,.T.);
#43828=EDGE_CURVE('',#35306,#35302,#31624,.T.);
#43829=EDGE_CURVE('',#35307,#35303,#31625,.T.);
#43830=EDGE_CURVE('',#35308,#35309,#3373,.T.);
#43831=EDGE_CURVE('',#35308,#35306,#31626,.T.);
#43832=EDGE_CURVE('',#35309,#35307,#31627,.T.);
#43833=EDGE_CURVE('',#35304,#35308,#31628,.T.);
#43834=EDGE_CURVE('',#35305,#35309,#31629,.T.);
#43835=EDGE_CURVE('',#35310,#35311,#3374,.T.);
#43836=EDGE_CURVE('',#35310,#35312,#31630,.T.);
#43837=EDGE_CURVE('',#35312,#35313,#3375,.T.);
#43838=EDGE_CURVE('',#35311,#35313,#31631,.T.);
#43839=EDGE_CURVE('',#35314,#35315,#3376,.T.);
#43840=EDGE_CURVE('',#35314,#35310,#31632,.T.);
#43841=EDGE_CURVE('',#35315,#35311,#31633,.T.);
#43842=EDGE_CURVE('',#35316,#35317,#3377,.T.);
#43843=EDGE_CURVE('',#35316,#35314,#31634,.T.);
#43844=EDGE_CURVE('',#35317,#35315,#31635,.T.);
#43845=EDGE_CURVE('',#35312,#35316,#31636,.T.);
#43846=EDGE_CURVE('',#35313,#35317,#31637,.T.);
#43847=EDGE_CURVE('',#35318,#35319,#3378,.T.);
#43848=EDGE_CURVE('',#35318,#35320,#31638,.T.);
#43849=EDGE_CURVE('',#35320,#35321,#3379,.T.);
#43850=EDGE_CURVE('',#35319,#35321,#31639,.T.);
#43851=EDGE_CURVE('',#35322,#35323,#3380,.T.);
#43852=EDGE_CURVE('',#35322,#35318,#31640,.T.);
#43853=EDGE_CURVE('',#35323,#35319,#31641,.T.);
#43854=EDGE_CURVE('',#35324,#35325,#3381,.T.);
#43855=EDGE_CURVE('',#35324,#35322,#31642,.T.);
#43856=EDGE_CURVE('',#35325,#35323,#31643,.T.);
#43857=EDGE_CURVE('',#35320,#35324,#31644,.T.);
#43858=EDGE_CURVE('',#35321,#35325,#31645,.T.);
#43859=EDGE_CURVE('',#35326,#35327,#31646,.T.);
#43860=EDGE_CURVE('',#35328,#35326,#3382,.T.);
#43861=EDGE_CURVE('',#35328,#35329,#31647,.T.);
#43862=EDGE_CURVE('',#35329,#35327,#3383,.T.);
#43863=EDGE_CURVE('',#35330,#35326,#31648,.T.);
#43864=EDGE_CURVE('',#35331,#35330,#3384,.T.);
#43865=EDGE_CURVE('',#35331,#35328,#31649,.T.);
#43866=EDGE_CURVE('',#35332,#35333,#3385,.T.);
#43867=EDGE_CURVE('',#35332,#35331,#31650,.T.);
#43868=EDGE_CURVE('',#35334,#35330,#31651,.T.);
#43869=EDGE_CURVE('',#35333,#35334,#3386,.T.);
#43870=EDGE_CURVE('',#35327,#35334,#31652,.T.);
#43871=EDGE_CURVE('',#35329,#35335,#31653,.T.);
#43872=EDGE_CURVE('',#35333,#35335,#3387,.T.);
#43873=EDGE_CURVE('',#35335,#35332,#31654,.T.);
#43874=EDGE_CURVE('',#35336,#35337,#3388,.T.);
#43875=EDGE_CURVE('',#35336,#35338,#31655,.T.);
#43876=EDGE_CURVE('',#35338,#35339,#3389,.T.);
#43877=EDGE_CURVE('',#35337,#35339,#31656,.T.);
#43878=EDGE_CURVE('',#35340,#35341,#3390,.T.);
#43879=EDGE_CURVE('',#35342,#35340,#3391,.T.);
#43880=EDGE_CURVE('',#35342,#35336,#31657,.T.);
#43881=EDGE_CURVE('',#35341,#35337,#31658,.T.);
#43882=EDGE_CURVE('',#35343,#35344,#3392,.T.);
#43883=EDGE_CURVE('',#35340,#35343,#3393,.T.);
#43884=EDGE_CURVE('',#35344,#35341,#31659,.T.);
#43885=EDGE_CURVE('',#35338,#35345,#31660,.T.);
#43886=EDGE_CURVE('',#35343,#35345,#3394,.T.);
#43887=EDGE_CURVE('',#35339,#35344,#31661,.T.);
#43888=EDGE_CURVE('',#35345,#35342,#31662,.T.);
#43889=EDGE_CURVE('',#35346,#35347,#3395,.T.);
#43890=EDGE_CURVE('',#35346,#35348,#31663,.T.);
#43891=EDGE_CURVE('',#35348,#35349,#3396,.T.);
#43892=EDGE_CURVE('',#35347,#35349,#31664,.T.);
#43893=EDGE_CURVE('',#35350,#35351,#3397,.T.);
#43894=EDGE_CURVE('',#35350,#35346,#31665,.T.);
#43895=EDGE_CURVE('',#35351,#35347,#31666,.T.);
#43896=EDGE_CURVE('',#35352,#35353,#3398,.T.);
#43897=EDGE_CURVE('',#35352,#35350,#31667,.T.);
#43898=EDGE_CURVE('',#35353,#35351,#31668,.T.);
#43899=EDGE_CURVE('',#35348,#35352,#31669,.T.);
#43900=EDGE_CURVE('',#35349,#35353,#31670,.T.);
#43901=EDGE_CURVE('',#35354,#35355,#3399,.T.);
#43902=EDGE_CURVE('',#35354,#35356,#31671,.T.);
#43903=EDGE_CURVE('',#35356,#35357,#3400,.T.);
#43904=EDGE_CURVE('',#35355,#35357,#31672,.T.);
#43905=EDGE_CURVE('',#35358,#35359,#3401,.T.);
#43906=EDGE_CURVE('',#35358,#35354,#31673,.T.);
#43907=EDGE_CURVE('',#35359,#35355,#31674,.T.);
#43908=EDGE_CURVE('',#35360,#35361,#3402,.T.);
#43909=EDGE_CURVE('',#35360,#35358,#31675,.T.);
#43910=EDGE_CURVE('',#35361,#35359,#31676,.T.);
#43911=EDGE_CURVE('',#35356,#35360,#31677,.T.);
#43912=EDGE_CURVE('',#35357,#35361,#31678,.T.);
#43913=EDGE_CURVE('',#35362,#35363,#3403,.T.);
#43914=EDGE_CURVE('',#35362,#35364,#31679,.T.);
#43915=EDGE_CURVE('',#35364,#35365,#3404,.T.);
#43916=EDGE_CURVE('',#35363,#35365,#31680,.T.);
#43917=EDGE_CURVE('',#35366,#35367,#3405,.T.);
#43918=EDGE_CURVE('',#35366,#35362,#31681,.T.);
#43919=EDGE_CURVE('',#35367,#35363,#31682,.T.);
#43920=EDGE_CURVE('',#35368,#35369,#3406,.T.);
#43921=EDGE_CURVE('',#35368,#35366,#31683,.T.);
#43922=EDGE_CURVE('',#35369,#35367,#31684,.T.);
#43923=EDGE_CURVE('',#35364,#35368,#31685,.T.);
#43924=EDGE_CURVE('',#35365,#35369,#31686,.T.);
#43925=EDGE_CURVE('',#35370,#35371,#3407,.T.);
#43926=EDGE_CURVE('',#35370,#35372,#31687,.T.);
#43927=EDGE_CURVE('',#35372,#35373,#3408,.T.);
#43928=EDGE_CURVE('',#35371,#35373,#31688,.T.);
#43929=EDGE_CURVE('',#35374,#35375,#3409,.T.);
#43930=EDGE_CURVE('',#35374,#35370,#31689,.T.);
#43931=EDGE_CURVE('',#35375,#35371,#31690,.T.);
#43932=EDGE_CURVE('',#35376,#35377,#3410,.T.);
#43933=EDGE_CURVE('',#35376,#35374,#31691,.T.);
#43934=EDGE_CURVE('',#35377,#35375,#31692,.T.);
#43935=EDGE_CURVE('',#35372,#35376,#31693,.T.);
#43936=EDGE_CURVE('',#35373,#35377,#31694,.T.);
#43937=EDGE_CURVE('',#35378,#35379,#3411,.T.);
#43938=EDGE_CURVE('',#35378,#35380,#31695,.T.);
#43939=EDGE_CURVE('',#35380,#35381,#3412,.T.);
#43940=EDGE_CURVE('',#35379,#35381,#31696,.T.);
#43941=EDGE_CURVE('',#35382,#35383,#3413,.T.);
#43942=EDGE_CURVE('',#35382,#35378,#31697,.T.);
#43943=EDGE_CURVE('',#35383,#35379,#31698,.T.);
#43944=EDGE_CURVE('',#35384,#35385,#3414,.T.);
#43945=EDGE_CURVE('',#35384,#35382,#31699,.T.);
#43946=EDGE_CURVE('',#35385,#35383,#31700,.T.);
#43947=EDGE_CURVE('',#35380,#35384,#31701,.T.);
#43948=EDGE_CURVE('',#35381,#35385,#31702,.T.);
#43949=EDGE_CURVE('',#35386,#35387,#3415,.T.);
#43950=EDGE_CURVE('',#35386,#35388,#31703,.T.);
#43951=EDGE_CURVE('',#35388,#35389,#3416,.T.);
#43952=EDGE_CURVE('',#35387,#35389,#31704,.T.);
#43953=EDGE_CURVE('',#35390,#35391,#3417,.T.);
#43954=EDGE_CURVE('',#35390,#35386,#31705,.T.);
#43955=EDGE_CURVE('',#35391,#35387,#31706,.T.);
#43956=EDGE_CURVE('',#35392,#35393,#3418,.T.);
#43957=EDGE_CURVE('',#35392,#35390,#31707,.T.);
#43958=EDGE_CURVE('',#35393,#35391,#31708,.T.);
#43959=EDGE_CURVE('',#35388,#35392,#31709,.T.);
#43960=EDGE_CURVE('',#35389,#35393,#31710,.T.);
#43961=EDGE_CURVE('',#35394,#35395,#3419,.T.);
#43962=EDGE_CURVE('',#35394,#35396,#31711,.T.);
#43963=EDGE_CURVE('',#35396,#35397,#3420,.T.);
#43964=EDGE_CURVE('',#35395,#35397,#31712,.T.);
#43965=EDGE_CURVE('',#35398,#35399,#3421,.T.);
#43966=EDGE_CURVE('',#35398,#35394,#31713,.T.);
#43967=EDGE_CURVE('',#35399,#35395,#31714,.T.);
#43968=EDGE_CURVE('',#35400,#35401,#3422,.T.);
#43969=EDGE_CURVE('',#35400,#35398,#31715,.T.);
#43970=EDGE_CURVE('',#35401,#35399,#31716,.T.);
#43971=EDGE_CURVE('',#35396,#35400,#31717,.T.);
#43972=EDGE_CURVE('',#35397,#35401,#31718,.T.);
#43973=EDGE_CURVE('',#35402,#35403,#3423,.T.);
#43974=EDGE_CURVE('',#35402,#35404,#31719,.T.);
#43975=EDGE_CURVE('',#35404,#35405,#3424,.T.);
#43976=EDGE_CURVE('',#35403,#35405,#31720,.T.);
#43977=EDGE_CURVE('',#35406,#35407,#3425,.T.);
#43978=EDGE_CURVE('',#35406,#35402,#31721,.T.);
#43979=EDGE_CURVE('',#35407,#35403,#31722,.T.);
#43980=EDGE_CURVE('',#35408,#35409,#3426,.T.);
#43981=EDGE_CURVE('',#35408,#35406,#31723,.T.);
#43982=EDGE_CURVE('',#35409,#35407,#31724,.T.);
#43983=EDGE_CURVE('',#35404,#35408,#31725,.T.);
#43984=EDGE_CURVE('',#35405,#35409,#31726,.T.);
#43985=EDGE_CURVE('',#35410,#35411,#3427,.T.);
#43986=EDGE_CURVE('',#35410,#35412,#31727,.T.);
#43987=EDGE_CURVE('',#35412,#35413,#3428,.T.);
#43988=EDGE_CURVE('',#35411,#35413,#31728,.T.);
#43989=EDGE_CURVE('',#35414,#35415,#3429,.T.);
#43990=EDGE_CURVE('',#35416,#35414,#3430,.T.);
#43991=EDGE_CURVE('',#35416,#35410,#31729,.T.);
#43992=EDGE_CURVE('',#35415,#35411,#31730,.T.);
#43993=EDGE_CURVE('',#35417,#35418,#3431,.T.);
#43994=EDGE_CURVE('',#35414,#35417,#3432,.T.);
#43995=EDGE_CURVE('',#35418,#35415,#31731,.T.);
#43996=EDGE_CURVE('',#35412,#35419,#31732,.T.);
#43997=EDGE_CURVE('',#35417,#35419,#3433,.T.);
#43998=EDGE_CURVE('',#35413,#35418,#31733,.T.);
#43999=EDGE_CURVE('',#35419,#35416,#31734,.T.);
#44000=EDGE_CURVE('',#35420,#35421,#3434,.T.);
#44001=EDGE_CURVE('',#35420,#35422,#31735,.T.);
#44002=EDGE_CURVE('',#35422,#35423,#3435,.T.);
#44003=EDGE_CURVE('',#35421,#35423,#31736,.T.);
#44004=EDGE_CURVE('',#35424,#35425,#3436,.T.);
#44005=EDGE_CURVE('',#35426,#35424,#3437,.T.);
#44006=EDGE_CURVE('',#35426,#35420,#31737,.T.);
#44007=EDGE_CURVE('',#35425,#35421,#31738,.T.);
#44008=EDGE_CURVE('',#35427,#35428,#3438,.T.);
#44009=EDGE_CURVE('',#35424,#35427,#3439,.T.);
#44010=EDGE_CURVE('',#35428,#35425,#31739,.T.);
#44011=EDGE_CURVE('',#35422,#35429,#31740,.T.);
#44012=EDGE_CURVE('',#35427,#35429,#3440,.T.);
#44013=EDGE_CURVE('',#35423,#35428,#31741,.T.);
#44014=EDGE_CURVE('',#35429,#35426,#31742,.T.);
#44015=EDGE_CURVE('',#35430,#35431,#3441,.T.);
#44016=EDGE_CURVE('',#35430,#35432,#31743,.T.);
#44017=EDGE_CURVE('',#35432,#35433,#3442,.T.);
#44018=EDGE_CURVE('',#35431,#35433,#31744,.T.);
#44019=EDGE_CURVE('',#35434,#35435,#3443,.T.);
#44020=EDGE_CURVE('',#35434,#35430,#31745,.T.);
#44021=EDGE_CURVE('',#35435,#35431,#31746,.T.);
#44022=EDGE_CURVE('',#35436,#35437,#3444,.T.);
#44023=EDGE_CURVE('',#35436,#35434,#31747,.T.);
#44024=EDGE_CURVE('',#35437,#35435,#31748,.T.);
#44025=EDGE_CURVE('',#35432,#35436,#31749,.T.);
#44026=EDGE_CURVE('',#35433,#35437,#31750,.T.);
#44027=EDGE_CURVE('',#35438,#35439,#3445,.T.);
#44028=EDGE_CURVE('',#35438,#35440,#31751,.T.);
#44029=EDGE_CURVE('',#35440,#35441,#3446,.T.);
#44030=EDGE_CURVE('',#35439,#35441,#31752,.T.);
#44031=EDGE_CURVE('',#35442,#35443,#3447,.T.);
#44032=EDGE_CURVE('',#35442,#35438,#31753,.T.);
#44033=EDGE_CURVE('',#35443,#35439,#31754,.T.);
#44034=EDGE_CURVE('',#35444,#35445,#3448,.T.);
#44035=EDGE_CURVE('',#35444,#35442,#31755,.T.);
#44036=EDGE_CURVE('',#35445,#35443,#31756,.T.);
#44037=EDGE_CURVE('',#35440,#35444,#31757,.T.);
#44038=EDGE_CURVE('',#35441,#35445,#31758,.T.);
#44039=EDGE_CURVE('',#35446,#35447,#3449,.T.);
#44040=EDGE_CURVE('',#35446,#35448,#31759,.T.);
#44041=EDGE_CURVE('',#35448,#35449,#3450,.T.);
#44042=EDGE_CURVE('',#35447,#35449,#31760,.T.);
#44043=EDGE_CURVE('',#35450,#35451,#3451,.T.);
#44044=EDGE_CURVE('',#35450,#35446,#31761,.T.);
#44045=EDGE_CURVE('',#35451,#35447,#31762,.T.);
#44046=EDGE_CURVE('',#35452,#35453,#3452,.T.);
#44047=EDGE_CURVE('',#35452,#35450,#31763,.T.);
#44048=EDGE_CURVE('',#35453,#35451,#31764,.T.);
#44049=EDGE_CURVE('',#35448,#35452,#31765,.T.);
#44050=EDGE_CURVE('',#35449,#35453,#31766,.T.);
#44051=EDGE_CURVE('',#35454,#35455,#3453,.T.);
#44052=EDGE_CURVE('',#35454,#35456,#31767,.T.);
#44053=EDGE_CURVE('',#35456,#35457,#3454,.T.);
#44054=EDGE_CURVE('',#35455,#35457,#31768,.T.);
#44055=EDGE_CURVE('',#35458,#35459,#3455,.T.);
#44056=EDGE_CURVE('',#35458,#35454,#31769,.T.);
#44057=EDGE_CURVE('',#35459,#35455,#31770,.T.);
#44058=EDGE_CURVE('',#35460,#35461,#3456,.T.);
#44059=EDGE_CURVE('',#35460,#35458,#31771,.T.);
#44060=EDGE_CURVE('',#35461,#35459,#31772,.T.);
#44061=EDGE_CURVE('',#35456,#35460,#31773,.T.);
#44062=EDGE_CURVE('',#35457,#35461,#31774,.T.);
#44063=EDGE_CURVE('',#35462,#35463,#3457,.T.);
#44064=EDGE_CURVE('',#35462,#35464,#31775,.T.);
#44065=EDGE_CURVE('',#35464,#35465,#3458,.T.);
#44066=EDGE_CURVE('',#35463,#35465,#31776,.T.);
#44067=EDGE_CURVE('',#35466,#35467,#3459,.T.);
#44068=EDGE_CURVE('',#35466,#35462,#31777,.T.);
#44069=EDGE_CURVE('',#35467,#35463,#31778,.T.);
#44070=EDGE_CURVE('',#35468,#35469,#3460,.T.);
#44071=EDGE_CURVE('',#35468,#35466,#31779,.T.);
#44072=EDGE_CURVE('',#35469,#35467,#31780,.T.);
#44073=EDGE_CURVE('',#35464,#35468,#31781,.T.);
#44074=EDGE_CURVE('',#35465,#35469,#31782,.T.);
#44075=EDGE_CURVE('',#35470,#35471,#3461,.T.);
#44076=EDGE_CURVE('',#35470,#35472,#31783,.T.);
#44077=EDGE_CURVE('',#35472,#35473,#3462,.T.);
#44078=EDGE_CURVE('',#35471,#35473,#31784,.T.);
#44079=EDGE_CURVE('',#35474,#35475,#3463,.T.);
#44080=EDGE_CURVE('',#35474,#35470,#31785,.T.);
#44081=EDGE_CURVE('',#35475,#35471,#31786,.T.);
#44082=EDGE_CURVE('',#35476,#35477,#3464,.T.);
#44083=EDGE_CURVE('',#35476,#35474,#31787,.T.);
#44084=EDGE_CURVE('',#35477,#35475,#31788,.T.);
#44085=EDGE_CURVE('',#35472,#35476,#31789,.T.);
#44086=EDGE_CURVE('',#35473,#35477,#31790,.T.);
#44087=EDGE_CURVE('',#35478,#35479,#3465,.T.);
#44088=EDGE_CURVE('',#35478,#35480,#31791,.T.);
#44089=EDGE_CURVE('',#35480,#35481,#3466,.T.);
#44090=EDGE_CURVE('',#35479,#35481,#31792,.T.);
#44091=EDGE_CURVE('',#35482,#35483,#3467,.T.);
#44092=EDGE_CURVE('',#35482,#35478,#31793,.T.);
#44093=EDGE_CURVE('',#35483,#35479,#31794,.T.);
#44094=EDGE_CURVE('',#35484,#35485,#3468,.T.);
#44095=EDGE_CURVE('',#35484,#35482,#31795,.T.);
#44096=EDGE_CURVE('',#35485,#35483,#31796,.T.);
#44097=EDGE_CURVE('',#35480,#35484,#31797,.T.);
#44098=EDGE_CURVE('',#35481,#35485,#31798,.T.);
#44099=EDGE_CURVE('',#35486,#35487,#3469,.T.);
#44100=EDGE_CURVE('',#35486,#35488,#31799,.T.);
#44101=EDGE_CURVE('',#35488,#35489,#3470,.T.);
#44102=EDGE_CURVE('',#35487,#35489,#31800,.T.);
#44103=EDGE_CURVE('',#35490,#35491,#3471,.T.);
#44104=EDGE_CURVE('',#35490,#35486,#31801,.T.);
#44105=EDGE_CURVE('',#35491,#35487,#31802,.T.);
#44106=EDGE_CURVE('',#35492,#35493,#3472,.T.);
#44107=EDGE_CURVE('',#35492,#35490,#31803,.T.);
#44108=EDGE_CURVE('',#35493,#35491,#31804,.T.);
#44109=EDGE_CURVE('',#35488,#35492,#31805,.T.);
#44110=EDGE_CURVE('',#35489,#35493,#31806,.T.);
#44111=EDGE_CURVE('',#35494,#35495,#3473,.T.);
#44112=EDGE_CURVE('',#35494,#35496,#31807,.T.);
#44113=EDGE_CURVE('',#35496,#35497,#3474,.T.);
#44114=EDGE_CURVE('',#35495,#35497,#31808,.T.);
#44115=EDGE_CURVE('',#35498,#35499,#3475,.T.);
#44116=EDGE_CURVE('',#35498,#35494,#31809,.T.);
#44117=EDGE_CURVE('',#35499,#35495,#31810,.T.);
#44118=EDGE_CURVE('',#35500,#35501,#3476,.T.);
#44119=EDGE_CURVE('',#35500,#35498,#31811,.T.);
#44120=EDGE_CURVE('',#35501,#35499,#31812,.T.);
#44121=EDGE_CURVE('',#35496,#35500,#31813,.T.);
#44122=EDGE_CURVE('',#35497,#35501,#31814,.T.);
#44123=EDGE_CURVE('',#35502,#35503,#3477,.T.);
#44124=EDGE_CURVE('',#35502,#35504,#31815,.T.);
#44125=EDGE_CURVE('',#35504,#35505,#3478,.T.);
#44126=EDGE_CURVE('',#35503,#35505,#31816,.T.);
#44127=EDGE_CURVE('',#35506,#35507,#3479,.T.);
#44128=EDGE_CURVE('',#35506,#35502,#31817,.T.);
#44129=EDGE_CURVE('',#35507,#35503,#31818,.T.);
#44130=EDGE_CURVE('',#35508,#35509,#3480,.T.);
#44131=EDGE_CURVE('',#35508,#35506,#31819,.T.);
#44132=EDGE_CURVE('',#35509,#35507,#31820,.T.);
#44133=EDGE_CURVE('',#35504,#35508,#31821,.T.);
#44134=EDGE_CURVE('',#35505,#35509,#31822,.T.);
#44135=EDGE_CURVE('',#35510,#35511,#3481,.T.);
#44136=EDGE_CURVE('',#35511,#35512,#3482,.T.);
#44137=EDGE_CURVE('',#35512,#35510,#31823,.T.);
#44138=EDGE_CURVE('',#35513,#35514,#3483,.T.);
#44139=EDGE_CURVE('',#35513,#35515,#31824,.T.);
#44140=EDGE_CURVE('',#35515,#35516,#3484,.T.);
#44141=EDGE_CURVE('',#35514,#35516,#31825,.T.);
#44142=EDGE_CURVE('',#35517,#35518,#3485,.T.);
#44143=EDGE_CURVE('',#35517,#35513,#31826,.T.);
#44144=EDGE_CURVE('',#35518,#35514,#31827,.T.);
#44145=EDGE_CURVE('',#35511,#35519,#3486,.T.);
#44146=EDGE_CURVE('',#35510,#35517,#31828,.T.);
#44147=EDGE_CURVE('',#35519,#35518,#31829,.T.);
#44148=EDGE_CURVE('',#35515,#35512,#31830,.T.);
#44149=EDGE_CURVE('',#35516,#35519,#31831,.T.);
#44150=EDGE_CURVE('',#35520,#35521,#3487,.T.);
#44151=EDGE_CURVE('',#35520,#35522,#31832,.T.);
#44152=EDGE_CURVE('',#35522,#35523,#3488,.T.);
#44153=EDGE_CURVE('',#35521,#35523,#31833,.T.);
#44154=EDGE_CURVE('',#35524,#35525,#3489,.T.);
#44155=EDGE_CURVE('',#35524,#35520,#31834,.T.);
#44156=EDGE_CURVE('',#35525,#35521,#31835,.T.);
#44157=EDGE_CURVE('',#35526,#35527,#3490,.T.);
#44158=EDGE_CURVE('',#35526,#35524,#31836,.T.);
#44159=EDGE_CURVE('',#35527,#35525,#31837,.T.);
#44160=EDGE_CURVE('',#35522,#35526,#31838,.T.);
#44161=EDGE_CURVE('',#35523,#35527,#31839,.T.);
#44162=EDGE_CURVE('',#35528,#35529,#3491,.T.);
#44163=EDGE_CURVE('',#35528,#35530,#31840,.T.);
#44164=EDGE_CURVE('',#35530,#35531,#3492,.T.);
#44165=EDGE_CURVE('',#35529,#35531,#31841,.T.);
#44166=EDGE_CURVE('',#35532,#35533,#3493,.T.);
#44167=EDGE_CURVE('',#35532,#35528,#31842,.T.);
#44168=EDGE_CURVE('',#35533,#35529,#31843,.T.);
#44169=EDGE_CURVE('',#35534,#35535,#3494,.T.);
#44170=EDGE_CURVE('',#35534,#35532,#31844,.T.);
#44171=EDGE_CURVE('',#35535,#35533,#31845,.T.);
#44172=EDGE_CURVE('',#35530,#35534,#31846,.T.);
#44173=EDGE_CURVE('',#35531,#35535,#31847,.T.);
#44174=EDGE_CURVE('',#35536,#35537,#3495,.T.);
#44175=EDGE_CURVE('',#35536,#35538,#31848,.T.);
#44176=EDGE_CURVE('',#35538,#35539,#3496,.T.);
#44177=EDGE_CURVE('',#35537,#35539,#31849,.T.);
#44178=EDGE_CURVE('',#35540,#35541,#3497,.T.);
#44179=EDGE_CURVE('',#35540,#35536,#31850,.T.);
#44180=EDGE_CURVE('',#35541,#35537,#31851,.T.);
#44181=EDGE_CURVE('',#35542,#35543,#3498,.T.);
#44182=EDGE_CURVE('',#35542,#35540,#31852,.T.);
#44183=EDGE_CURVE('',#35543,#35541,#31853,.T.);
#44184=EDGE_CURVE('',#35538,#35542,#31854,.T.);
#44185=EDGE_CURVE('',#35539,#35543,#31855,.T.);
#44186=EDGE_CURVE('',#35544,#35545,#3499,.T.);
#44187=EDGE_CURVE('',#35544,#35546,#31856,.T.);
#44188=EDGE_CURVE('',#35546,#35547,#3500,.T.);
#44189=EDGE_CURVE('',#35545,#35547,#31857,.T.);
#44190=EDGE_CURVE('',#35548,#35549,#3501,.T.);
#44191=EDGE_CURVE('',#35548,#35544,#31858,.T.);
#44192=EDGE_CURVE('',#35549,#35545,#31859,.T.);
#44193=EDGE_CURVE('',#35550,#35551,#3502,.T.);
#44194=EDGE_CURVE('',#35550,#35548,#31860,.T.);
#44195=EDGE_CURVE('',#35551,#35549,#31861,.T.);
#44196=EDGE_CURVE('',#35546,#35550,#31862,.T.);
#44197=EDGE_CURVE('',#35547,#35551,#31863,.T.);
#44198=EDGE_CURVE('',#35552,#35553,#3503,.T.);
#44199=EDGE_CURVE('',#35552,#35554,#31864,.T.);
#44200=EDGE_CURVE('',#35554,#35555,#3504,.T.);
#44201=EDGE_CURVE('',#35553,#35555,#31865,.T.);
#44202=EDGE_CURVE('',#35556,#35557,#3505,.T.);
#44203=EDGE_CURVE('',#35556,#35552,#31866,.T.);
#44204=EDGE_CURVE('',#35557,#35553,#31867,.T.);
#44205=EDGE_CURVE('',#35558,#35559,#3506,.T.);
#44206=EDGE_CURVE('',#35558,#35556,#31868,.T.);
#44207=EDGE_CURVE('',#35559,#35557,#31869,.T.);
#44208=EDGE_CURVE('',#35554,#35558,#31870,.T.);
#44209=EDGE_CURVE('',#35555,#35559,#31871,.T.);
#44210=EDGE_CURVE('',#35560,#35561,#3507,.T.);
#44211=EDGE_CURVE('',#35560,#35562,#31872,.T.);
#44212=EDGE_CURVE('',#35562,#35563,#3508,.T.);
#44213=EDGE_CURVE('',#35561,#35563,#31873,.T.);
#44214=EDGE_CURVE('',#35564,#35565,#3509,.T.);
#44215=EDGE_CURVE('',#35564,#35560,#31874,.T.);
#44216=EDGE_CURVE('',#35565,#35561,#31875,.T.);
#44217=EDGE_CURVE('',#35566,#35567,#3510,.T.);
#44218=EDGE_CURVE('',#35566,#35564,#31876,.T.);
#44219=EDGE_CURVE('',#35567,#35565,#31877,.T.);
#44220=EDGE_CURVE('',#35562,#35566,#31878,.T.);
#44221=EDGE_CURVE('',#35563,#35567,#31879,.T.);
#44222=EDGE_CURVE('',#35568,#35569,#3511,.T.);
#44223=EDGE_CURVE('',#35568,#35570,#31880,.T.);
#44224=EDGE_CURVE('',#35570,#35571,#3512,.T.);
#44225=EDGE_CURVE('',#35569,#35571,#31881,.T.);
#44226=EDGE_CURVE('',#35572,#35573,#3513,.T.);
#44227=EDGE_CURVE('',#35572,#35568,#31882,.T.);
#44228=EDGE_CURVE('',#35573,#35569,#31883,.T.);
#44229=EDGE_CURVE('',#35574,#35575,#3514,.T.);
#44230=EDGE_CURVE('',#35574,#35572,#31884,.T.);
#44231=EDGE_CURVE('',#35575,#35573,#31885,.T.);
#44232=EDGE_CURVE('',#35570,#35574,#31886,.T.);
#44233=EDGE_CURVE('',#35571,#35575,#31887,.T.);
#44234=EDGE_CURVE('',#35576,#35577,#3515,.T.);
#44235=EDGE_CURVE('',#35576,#35578,#31888,.T.);
#44236=EDGE_CURVE('',#35578,#35579,#3516,.T.);
#44237=EDGE_CURVE('',#35577,#35579,#31889,.T.);
#44238=EDGE_CURVE('',#35580,#35581,#3517,.T.);
#44239=EDGE_CURVE('',#35580,#35576,#31890,.T.);
#44240=EDGE_CURVE('',#35581,#35577,#31891,.T.);
#44241=EDGE_CURVE('',#35582,#35583,#3518,.T.);
#44242=EDGE_CURVE('',#35582,#35580,#31892,.T.);
#44243=EDGE_CURVE('',#35583,#35581,#31893,.T.);
#44244=EDGE_CURVE('',#35578,#35582,#31894,.T.);
#44245=EDGE_CURVE('',#35579,#35583,#31895,.T.);
#44246=EDGE_CURVE('',#35584,#35585,#3519,.T.);
#44247=EDGE_CURVE('',#35584,#35586,#31896,.T.);
#44248=EDGE_CURVE('',#35586,#35587,#3520,.T.);
#44249=EDGE_CURVE('',#35585,#35587,#31897,.T.);
#44250=EDGE_CURVE('',#35588,#35589,#3521,.T.);
#44251=EDGE_CURVE('',#35588,#35584,#31898,.T.);
#44252=EDGE_CURVE('',#35589,#35585,#31899,.T.);
#44253=EDGE_CURVE('',#35590,#35591,#3522,.T.);
#44254=EDGE_CURVE('',#35590,#35588,#31900,.T.);
#44255=EDGE_CURVE('',#35591,#35589,#31901,.T.);
#44256=EDGE_CURVE('',#35586,#35590,#31902,.T.);
#44257=EDGE_CURVE('',#35587,#35591,#31903,.T.);
#44258=EDGE_CURVE('',#35592,#35593,#3523,.T.);
#44259=EDGE_CURVE('',#35592,#35594,#31904,.T.);
#44260=EDGE_CURVE('',#35594,#35595,#3524,.T.);
#44261=EDGE_CURVE('',#35593,#35595,#31905,.T.);
#44262=EDGE_CURVE('',#35596,#35597,#3525,.T.);
#44263=EDGE_CURVE('',#35596,#35592,#31906,.T.);
#44264=EDGE_CURVE('',#35597,#35593,#31907,.T.);
#44265=EDGE_CURVE('',#35598,#35599,#3526,.T.);
#44266=EDGE_CURVE('',#35598,#35596,#31908,.T.);
#44267=EDGE_CURVE('',#35599,#35597,#31909,.T.);
#44268=EDGE_CURVE('',#35594,#35598,#31910,.T.);
#44269=EDGE_CURVE('',#35595,#35599,#31911,.T.);
#44270=EDGE_CURVE('',#35600,#35601,#3527,.T.);
#44271=EDGE_CURVE('',#35600,#35602,#31912,.T.);
#44272=EDGE_CURVE('',#35602,#35603,#3528,.T.);
#44273=EDGE_CURVE('',#35601,#35603,#31913,.T.);
#44274=EDGE_CURVE('',#35604,#35605,#3529,.T.);
#44275=EDGE_CURVE('',#35604,#35600,#31914,.T.);
#44276=EDGE_CURVE('',#35605,#35601,#31915,.T.);
#44277=EDGE_CURVE('',#35606,#35607,#3530,.T.);
#44278=EDGE_CURVE('',#35608,#35606,#3531,.T.);
#44279=EDGE_CURVE('',#35608,#35604,#31916,.T.);
#44280=EDGE_CURVE('',#35607,#35605,#31917,.T.);
#44281=EDGE_CURVE('',#35602,#35609,#31918,.T.);
#44282=EDGE_CURVE('',#35606,#35609,#3532,.T.);
#44283=EDGE_CURVE('',#35603,#35607,#31919,.T.);
#44284=EDGE_CURVE('',#35609,#35608,#31920,.T.);
#44285=EDGE_CURVE('',#35610,#35611,#3533,.T.);
#44286=EDGE_CURVE('',#35610,#35612,#31921,.T.);
#44287=EDGE_CURVE('',#35612,#35613,#3534,.T.);
#44288=EDGE_CURVE('',#35611,#35613,#31922,.T.);
#44289=EDGE_CURVE('',#35614,#35615,#3535,.T.);
#44290=EDGE_CURVE('',#35614,#35610,#31923,.T.);
#44291=EDGE_CURVE('',#35615,#35611,#31924,.T.);
#44292=EDGE_CURVE('',#35616,#35617,#3536,.T.);
#44293=EDGE_CURVE('',#35618,#35616,#3537,.T.);
#44294=EDGE_CURVE('',#35618,#35614,#31925,.T.);
#44295=EDGE_CURVE('',#35617,#35615,#31926,.T.);
#44296=EDGE_CURVE('',#35612,#35619,#31927,.T.);
#44297=EDGE_CURVE('',#35616,#35619,#3538,.T.);
#44298=EDGE_CURVE('',#35613,#35617,#31928,.T.);
#44299=EDGE_CURVE('',#35619,#35618,#31929,.T.);
#44300=EDGE_CURVE('',#35620,#35621,#3539,.T.);
#44301=EDGE_CURVE('',#35620,#35622,#31930,.T.);
#44302=EDGE_CURVE('',#35622,#35623,#3540,.T.);
#44303=EDGE_CURVE('',#35621,#35623,#31931,.T.);
#44304=EDGE_CURVE('',#35624,#35625,#3541,.T.);
#44305=EDGE_CURVE('',#35624,#35620,#31932,.T.);
#44306=EDGE_CURVE('',#35625,#35621,#31933,.T.);
#44307=EDGE_CURVE('',#35626,#35627,#3542,.T.);
#44308=EDGE_CURVE('',#35626,#35624,#31934,.T.);
#44309=EDGE_CURVE('',#35627,#35625,#31935,.T.);
#44310=EDGE_CURVE('',#35622,#35626,#31936,.T.);
#44311=EDGE_CURVE('',#35623,#35627,#31937,.T.);
#44312=EDGE_CURVE('',#35628,#35629,#3543,.T.);
#44313=EDGE_CURVE('',#35628,#35630,#31938,.T.);
#44314=EDGE_CURVE('',#35630,#35631,#3544,.T.);
#44315=EDGE_CURVE('',#35629,#35631,#31939,.T.);
#44316=EDGE_CURVE('',#35632,#35633,#3545,.T.);
#44317=EDGE_CURVE('',#35632,#35628,#31940,.T.);
#44318=EDGE_CURVE('',#35633,#35629,#31941,.T.);
#44319=EDGE_CURVE('',#35634,#35635,#3546,.T.);
#44320=EDGE_CURVE('',#35634,#35632,#31942,.T.);
#44321=EDGE_CURVE('',#35635,#35633,#31943,.T.);
#44322=EDGE_CURVE('',#35630,#35634,#31944,.T.);
#44323=EDGE_CURVE('',#35631,#35635,#31945,.T.);
#44324=EDGE_CURVE('',#35636,#35637,#3547,.T.);
#44325=EDGE_CURVE('',#35636,#35638,#31946,.T.);
#44326=EDGE_CURVE('',#35638,#35639,#3548,.T.);
#44327=EDGE_CURVE('',#35637,#35639,#31947,.T.);
#44328=EDGE_CURVE('',#35640,#35641,#3549,.T.);
#44329=EDGE_CURVE('',#35640,#35636,#31948,.T.);
#44330=EDGE_CURVE('',#35641,#35637,#31949,.T.);
#44331=EDGE_CURVE('',#35642,#35643,#3550,.T.);
#44332=EDGE_CURVE('',#35642,#35640,#31950,.T.);
#44333=EDGE_CURVE('',#35643,#35641,#31951,.T.);
#44334=EDGE_CURVE('',#35638,#35642,#31952,.T.);
#44335=EDGE_CURVE('',#35639,#35643,#31953,.T.);
#44336=EDGE_CURVE('',#35644,#35645,#3551,.T.);
#44337=EDGE_CURVE('',#35644,#35646,#31954,.T.);
#44338=EDGE_CURVE('',#35646,#35647,#3552,.T.);
#44339=EDGE_CURVE('',#35645,#35647,#31955,.T.);
#44340=EDGE_CURVE('',#35648,#35649,#3553,.T.);
#44341=EDGE_CURVE('',#35648,#35644,#31956,.T.);
#44342=EDGE_CURVE('',#35649,#35645,#31957,.T.);
#44343=EDGE_CURVE('',#35650,#35651,#3554,.T.);
#44344=EDGE_CURVE('',#35650,#35648,#31958,.T.);
#44345=EDGE_CURVE('',#35651,#35649,#31959,.T.);
#44346=EDGE_CURVE('',#35646,#35650,#31960,.T.);
#44347=EDGE_CURVE('',#35647,#35651,#31961,.T.);
#44348=EDGE_CURVE('',#35652,#35653,#3555,.T.);
#44349=EDGE_CURVE('',#35652,#35654,#31962,.T.);
#44350=EDGE_CURVE('',#35654,#35655,#3556,.T.);
#44351=EDGE_CURVE('',#35653,#35655,#31963,.T.);
#44352=EDGE_CURVE('',#35656,#35657,#3557,.T.);
#44353=EDGE_CURVE('',#35656,#35652,#31964,.T.);
#44354=EDGE_CURVE('',#35657,#35653,#31965,.T.);
#44355=EDGE_CURVE('',#35658,#35659,#3558,.T.);
#44356=EDGE_CURVE('',#35658,#35656,#31966,.T.);
#44357=EDGE_CURVE('',#35659,#35657,#31967,.T.);
#44358=EDGE_CURVE('',#35654,#35658,#31968,.T.);
#44359=EDGE_CURVE('',#35655,#35659,#31969,.T.);
#44360=EDGE_CURVE('',#35660,#35661,#3559,.T.);
#44361=EDGE_CURVE('',#35660,#35662,#31970,.T.);
#44362=EDGE_CURVE('',#35662,#35663,#3560,.T.);
#44363=EDGE_CURVE('',#35661,#35663,#31971,.T.);
#44364=EDGE_CURVE('',#35664,#35665,#3561,.T.);
#44365=EDGE_CURVE('',#35664,#35660,#31972,.T.);
#44366=EDGE_CURVE('',#35665,#35661,#31973,.T.);
#44367=EDGE_CURVE('',#35666,#35667,#3562,.T.);
#44368=EDGE_CURVE('',#35666,#35664,#31974,.T.);
#44369=EDGE_CURVE('',#35667,#35665,#31975,.T.);
#44370=EDGE_CURVE('',#35662,#35666,#31976,.T.);
#44371=EDGE_CURVE('',#35663,#35667,#31977,.T.);
#44372=EDGE_CURVE('',#35668,#35669,#3563,.T.);
#44373=EDGE_CURVE('',#35668,#35670,#31978,.T.);
#44374=EDGE_CURVE('',#35670,#35671,#3564,.T.);
#44375=EDGE_CURVE('',#35669,#35671,#31979,.T.);
#44376=EDGE_CURVE('',#35672,#35673,#3565,.T.);
#44377=EDGE_CURVE('',#35672,#35668,#31980,.T.);
#44378=EDGE_CURVE('',#35673,#35669,#31981,.T.);
#44379=EDGE_CURVE('',#35674,#35675,#3566,.T.);
#44380=EDGE_CURVE('',#35674,#35672,#31982,.T.);
#44381=EDGE_CURVE('',#35675,#35673,#31983,.T.);
#44382=EDGE_CURVE('',#35670,#35674,#31984,.T.);
#44383=EDGE_CURVE('',#35671,#35675,#31985,.T.);
#44384=EDGE_CURVE('',#35676,#35677,#3567,.T.);
#44385=EDGE_CURVE('',#35676,#35678,#31986,.T.);
#44386=EDGE_CURVE('',#35678,#35679,#3568,.T.);
#44387=EDGE_CURVE('',#35677,#35679,#31987,.T.);
#44388=EDGE_CURVE('',#35680,#35681,#3569,.T.);
#44389=EDGE_CURVE('',#35680,#35676,#31988,.T.);
#44390=EDGE_CURVE('',#35681,#35677,#31989,.T.);
#44391=EDGE_CURVE('',#35682,#35683,#3570,.T.);
#44392=EDGE_CURVE('',#35682,#35680,#31990,.T.);
#44393=EDGE_CURVE('',#35683,#35681,#31991,.T.);
#44394=EDGE_CURVE('',#35678,#35682,#31992,.T.);
#44395=EDGE_CURVE('',#35679,#35683,#31993,.T.);
#44396=EDGE_CURVE('',#35684,#35685,#3571,.T.);
#44397=EDGE_CURVE('',#35684,#35686,#31994,.T.);
#44398=EDGE_CURVE('',#35686,#35687,#3572,.T.);
#44399=EDGE_CURVE('',#35685,#35687,#31995,.T.);
#44400=EDGE_CURVE('',#35688,#35689,#3573,.T.);
#44401=EDGE_CURVE('',#35688,#35684,#31996,.T.);
#44402=EDGE_CURVE('',#35689,#35685,#31997,.T.);
#44403=EDGE_CURVE('',#35690,#35691,#3574,.T.);
#44404=EDGE_CURVE('',#35690,#35688,#31998,.T.);
#44405=EDGE_CURVE('',#35691,#35689,#31999,.T.);
#44406=EDGE_CURVE('',#35686,#35690,#32000,.T.);
#44407=EDGE_CURVE('',#35687,#35691,#32001,.T.);
#44408=EDGE_CURVE('',#35692,#35693,#3575,.T.);
#44409=EDGE_CURVE('',#35692,#35694,#32002,.T.);
#44410=EDGE_CURVE('',#35694,#35695,#3576,.T.);
#44411=EDGE_CURVE('',#35693,#35695,#32003,.T.);
#44412=EDGE_CURVE('',#35696,#35697,#3577,.T.);
#44413=EDGE_CURVE('',#35696,#35692,#32004,.T.);
#44414=EDGE_CURVE('',#35697,#35693,#32005,.T.);
#44415=EDGE_CURVE('',#35698,#35699,#3578,.T.);
#44416=EDGE_CURVE('',#35698,#35696,#32006,.T.);
#44417=EDGE_CURVE('',#35699,#35697,#32007,.T.);
#44418=EDGE_CURVE('',#35694,#35698,#32008,.T.);
#44419=EDGE_CURVE('',#35695,#35699,#32009,.T.);
#44420=EDGE_CURVE('',#35700,#35701,#3579,.T.);
#44421=EDGE_CURVE('',#35700,#35702,#32010,.T.);
#44422=EDGE_CURVE('',#35702,#35703,#3580,.T.);
#44423=EDGE_CURVE('',#35701,#35703,#32011,.T.);
#44424=EDGE_CURVE('',#35704,#35705,#3581,.T.);
#44425=EDGE_CURVE('',#35704,#35700,#32012,.T.);
#44426=EDGE_CURVE('',#35705,#35701,#32013,.T.);
#44427=EDGE_CURVE('',#35706,#35707,#3582,.T.);
#44428=EDGE_CURVE('',#35706,#35704,#32014,.T.);
#44429=EDGE_CURVE('',#35707,#35705,#32015,.T.);
#44430=EDGE_CURVE('',#35702,#35706,#32016,.T.);
#44431=EDGE_CURVE('',#35703,#35707,#32017,.T.);
#44432=EDGE_CURVE('',#35708,#35709,#3583,.T.);
#44433=EDGE_CURVE('',#35708,#35710,#32018,.T.);
#44434=EDGE_CURVE('',#35710,#35711,#3584,.T.);
#44435=EDGE_CURVE('',#35709,#35711,#32019,.T.);
#44436=EDGE_CURVE('',#35712,#35713,#3585,.T.);
#44437=EDGE_CURVE('',#35712,#35708,#32020,.T.);
#44438=EDGE_CURVE('',#35713,#35709,#32021,.T.);
#44439=EDGE_CURVE('',#35714,#35715,#3586,.T.);
#44440=EDGE_CURVE('',#35714,#35712,#32022,.T.);
#44441=EDGE_CURVE('',#35715,#35713,#32023,.T.);
#44442=EDGE_CURVE('',#35710,#35714,#32024,.T.);
#44443=EDGE_CURVE('',#35711,#35715,#32025,.T.);
#44444=EDGE_CURVE('',#35716,#35717,#3587,.T.);
#44445=EDGE_CURVE('',#35716,#35718,#32026,.T.);
#44446=EDGE_CURVE('',#35718,#35719,#3588,.T.);
#44447=EDGE_CURVE('',#35717,#35719,#32027,.T.);
#44448=EDGE_CURVE('',#35720,#35721,#3589,.T.);
#44449=EDGE_CURVE('',#35720,#35716,#32028,.T.);
#44450=EDGE_CURVE('',#35721,#35717,#32029,.T.);
#44451=EDGE_CURVE('',#35722,#35723,#3590,.T.);
#44452=EDGE_CURVE('',#35722,#35720,#32030,.T.);
#44453=EDGE_CURVE('',#35723,#35721,#32031,.T.);
#44454=EDGE_CURVE('',#35718,#35722,#32032,.T.);
#44455=EDGE_CURVE('',#35719,#35723,#32033,.T.);
#44456=EDGE_CURVE('',#35724,#35725,#3591,.T.);
#44457=EDGE_CURVE('',#35724,#35726,#32034,.T.);
#44458=EDGE_CURVE('',#35726,#35727,#3592,.T.);
#44459=EDGE_CURVE('',#35725,#35727,#32035,.T.);
#44460=EDGE_CURVE('',#35728,#35729,#3593,.T.);
#44461=EDGE_CURVE('',#35728,#35724,#32036,.T.);
#44462=EDGE_CURVE('',#35729,#35725,#32037,.T.);
#44463=EDGE_CURVE('',#35730,#35731,#3594,.T.);
#44464=EDGE_CURVE('',#35730,#35728,#32038,.T.);
#44465=EDGE_CURVE('',#35731,#35729,#32039,.T.);
#44466=EDGE_CURVE('',#35726,#35730,#32040,.T.);
#44467=EDGE_CURVE('',#35727,#35731,#32041,.T.);
#44468=EDGE_CURVE('',#35732,#35733,#3595,.T.);
#44469=EDGE_CURVE('',#35732,#35734,#32042,.T.);
#44470=EDGE_CURVE('',#35734,#35735,#3596,.T.);
#44471=EDGE_CURVE('',#35733,#35735,#32043,.T.);
#44472=EDGE_CURVE('',#35736,#35737,#3597,.T.);
#44473=EDGE_CURVE('',#35736,#35732,#32044,.T.);
#44474=EDGE_CURVE('',#35737,#35733,#32045,.T.);
#44475=EDGE_CURVE('',#35738,#35739,#3598,.T.);
#44476=EDGE_CURVE('',#35738,#35736,#32046,.T.);
#44477=EDGE_CURVE('',#35739,#35737,#32047,.T.);
#44478=EDGE_CURVE('',#35734,#35738,#32048,.T.);
#44479=EDGE_CURVE('',#35735,#35739,#32049,.T.);
#44480=EDGE_CURVE('',#35740,#35741,#3599,.T.);
#44481=EDGE_CURVE('',#35740,#35742,#32050,.T.);
#44482=EDGE_CURVE('',#35742,#35743,#3600,.T.);
#44483=EDGE_CURVE('',#35741,#35743,#32051,.T.);
#44484=EDGE_CURVE('',#35744,#35745,#3601,.T.);
#44485=EDGE_CURVE('',#35744,#35740,#32052,.T.);
#44486=EDGE_CURVE('',#35745,#35741,#32053,.T.);
#44487=EDGE_CURVE('',#35746,#35747,#3602,.T.);
#44488=EDGE_CURVE('',#35746,#35744,#32054,.T.);
#44489=EDGE_CURVE('',#35747,#35745,#32055,.T.);
#44490=EDGE_CURVE('',#35742,#35746,#32056,.T.);
#44491=EDGE_CURVE('',#35743,#35747,#32057,.T.);
#44492=EDGE_CURVE('',#35748,#35749,#3603,.T.);
#44493=EDGE_CURVE('',#35748,#35750,#32058,.T.);
#44494=EDGE_CURVE('',#35750,#35751,#3604,.T.);
#44495=EDGE_CURVE('',#35749,#35751,#32059,.T.);
#44496=EDGE_CURVE('',#35752,#35753,#3605,.T.);
#44497=EDGE_CURVE('',#35752,#35748,#32060,.T.);
#44498=EDGE_CURVE('',#35753,#35749,#32061,.T.);
#44499=EDGE_CURVE('',#35754,#35755,#3606,.T.);
#44500=EDGE_CURVE('',#35754,#35752,#32062,.T.);
#44501=EDGE_CURVE('',#35755,#35753,#32063,.T.);
#44502=EDGE_CURVE('',#35750,#35754,#32064,.T.);
#44503=EDGE_CURVE('',#35751,#35755,#32065,.T.);
#44504=EDGE_CURVE('',#35756,#35757,#3607,.T.);
#44505=EDGE_CURVE('',#35756,#35758,#32066,.T.);
#44506=EDGE_CURVE('',#35758,#35759,#3608,.T.);
#44507=EDGE_CURVE('',#35757,#35759,#32067,.T.);
#44508=EDGE_CURVE('',#35760,#35761,#3609,.T.);
#44509=EDGE_CURVE('',#35760,#35756,#32068,.T.);
#44510=EDGE_CURVE('',#35761,#35757,#32069,.T.);
#44511=EDGE_CURVE('',#35762,#35763,#3610,.T.);
#44512=EDGE_CURVE('',#35762,#35760,#32070,.T.);
#44513=EDGE_CURVE('',#35763,#35761,#32071,.T.);
#44514=EDGE_CURVE('',#35758,#35762,#32072,.T.);
#44515=EDGE_CURVE('',#35759,#35763,#32073,.T.);
#44516=EDGE_CURVE('',#35764,#35765,#3611,.T.);
#44517=EDGE_CURVE('',#35764,#35766,#32074,.T.);
#44518=EDGE_CURVE('',#35766,#35767,#3612,.T.);
#44519=EDGE_CURVE('',#35765,#35767,#32075,.T.);
#44520=EDGE_CURVE('',#35768,#35769,#3613,.T.);
#44521=EDGE_CURVE('',#35768,#35764,#32076,.T.);
#44522=EDGE_CURVE('',#35769,#35765,#32077,.T.);
#44523=EDGE_CURVE('',#35770,#35771,#3614,.T.);
#44524=EDGE_CURVE('',#35770,#35768,#32078,.T.);
#44525=EDGE_CURVE('',#35771,#35769,#32079,.T.);
#44526=EDGE_CURVE('',#35766,#35770,#32080,.T.);
#44527=EDGE_CURVE('',#35767,#35771,#32081,.T.);
#44528=EDGE_CURVE('',#35772,#35773,#3615,.T.);
#44529=EDGE_CURVE('',#35772,#35774,#32082,.T.);
#44530=EDGE_CURVE('',#35774,#35775,#3616,.T.);
#44531=EDGE_CURVE('',#35773,#35775,#32083,.T.);
#44532=EDGE_CURVE('',#35776,#35777,#3617,.T.);
#44533=EDGE_CURVE('',#35776,#35772,#32084,.T.);
#44534=EDGE_CURVE('',#35777,#35773,#32085,.T.);
#44535=EDGE_CURVE('',#35778,#35779,#3618,.T.);
#44536=EDGE_CURVE('',#35778,#35776,#32086,.T.);
#44537=EDGE_CURVE('',#35779,#35777,#32087,.T.);
#44538=EDGE_CURVE('',#35774,#35778,#32088,.T.);
#44539=EDGE_CURVE('',#35775,#35779,#32089,.T.);
#44540=EDGE_CURVE('',#35780,#35781,#3619,.T.);
#44541=EDGE_CURVE('',#35780,#35782,#32090,.T.);
#44542=EDGE_CURVE('',#35782,#35783,#3620,.T.);
#44543=EDGE_CURVE('',#35781,#35783,#32091,.T.);
#44544=EDGE_CURVE('',#35784,#35785,#3621,.T.);
#44545=EDGE_CURVE('',#35784,#35780,#32092,.T.);
#44546=EDGE_CURVE('',#35785,#35781,#32093,.T.);
#44547=EDGE_CURVE('',#35786,#35787,#3622,.T.);
#44548=EDGE_CURVE('',#35786,#35784,#32094,.T.);
#44549=EDGE_CURVE('',#35787,#35785,#32095,.T.);
#44550=EDGE_CURVE('',#35782,#35786,#32096,.T.);
#44551=EDGE_CURVE('',#35783,#35787,#32097,.T.);
#44552=EDGE_CURVE('',#35788,#35789,#3623,.T.);
#44553=EDGE_CURVE('',#35788,#35790,#32098,.T.);
#44554=EDGE_CURVE('',#35790,#35791,#3624,.T.);
#44555=EDGE_CURVE('',#35789,#35791,#32099,.T.);
#44556=EDGE_CURVE('',#35792,#35793,#3625,.T.);
#44557=EDGE_CURVE('',#35792,#35788,#32100,.T.);
#44558=EDGE_CURVE('',#35793,#35789,#32101,.T.);
#44559=EDGE_CURVE('',#35794,#35795,#3626,.T.);
#44560=EDGE_CURVE('',#35794,#35792,#32102,.T.);
#44561=EDGE_CURVE('',#35795,#35793,#32103,.T.);
#44562=EDGE_CURVE('',#35790,#35794,#32104,.T.);
#44563=EDGE_CURVE('',#35791,#35795,#32105,.T.);
#44564=EDGE_CURVE('',#35796,#35797,#3627,.T.);
#44565=EDGE_CURVE('',#35796,#35798,#32106,.T.);
#44566=EDGE_CURVE('',#35798,#35799,#3628,.T.);
#44567=EDGE_CURVE('',#35797,#35799,#32107,.T.);
#44568=EDGE_CURVE('',#35800,#35801,#3629,.T.);
#44569=EDGE_CURVE('',#35800,#35796,#32108,.T.);
#44570=EDGE_CURVE('',#35801,#35797,#32109,.T.);
#44571=EDGE_CURVE('',#35802,#35803,#3630,.T.);
#44572=EDGE_CURVE('',#35802,#35800,#32110,.T.);
#44573=EDGE_CURVE('',#35803,#35801,#32111,.T.);
#44574=EDGE_CURVE('',#35798,#35802,#32112,.T.);
#44575=EDGE_CURVE('',#35799,#35803,#32113,.T.);
#44576=EDGE_CURVE('',#35804,#35805,#3631,.T.);
#44577=EDGE_CURVE('',#35804,#35806,#32114,.T.);
#44578=EDGE_CURVE('',#35806,#35807,#3632,.T.);
#44579=EDGE_CURVE('',#35805,#35807,#32115,.T.);
#44580=EDGE_CURVE('',#35808,#35809,#3633,.T.);
#44581=EDGE_CURVE('',#35808,#35804,#32116,.T.);
#44582=EDGE_CURVE('',#35809,#35805,#32117,.T.);
#44583=EDGE_CURVE('',#35810,#35811,#3634,.T.);
#44584=EDGE_CURVE('',#35810,#35808,#32118,.T.);
#44585=EDGE_CURVE('',#35811,#35809,#32119,.T.);
#44586=EDGE_CURVE('',#35806,#35810,#32120,.T.);
#44587=EDGE_CURVE('',#35807,#35811,#32121,.T.);
#44588=EDGE_CURVE('',#35812,#35813,#3635,.T.);
#44589=EDGE_CURVE('',#35812,#35814,#32122,.T.);
#44590=EDGE_CURVE('',#35814,#35815,#3636,.T.);
#44591=EDGE_CURVE('',#35813,#35815,#32123,.T.);
#44592=EDGE_CURVE('',#35816,#35817,#3637,.T.);
#44593=EDGE_CURVE('',#35816,#35812,#32124,.T.);
#44594=EDGE_CURVE('',#35817,#35813,#32125,.T.);
#44595=EDGE_CURVE('',#35818,#35819,#3638,.T.);
#44596=EDGE_CURVE('',#35818,#35816,#32126,.T.);
#44597=EDGE_CURVE('',#35819,#35817,#32127,.T.);
#44598=EDGE_CURVE('',#35814,#35818,#32128,.T.);
#44599=EDGE_CURVE('',#35815,#35819,#32129,.T.);
#44600=EDGE_CURVE('',#35820,#35821,#3639,.T.);
#44601=EDGE_CURVE('',#35820,#35822,#32130,.T.);
#44602=EDGE_CURVE('',#35822,#35823,#3640,.T.);
#44603=EDGE_CURVE('',#35821,#35823,#32131,.T.);
#44604=EDGE_CURVE('',#35824,#35825,#3641,.T.);
#44605=EDGE_CURVE('',#35824,#35820,#32132,.T.);
#44606=EDGE_CURVE('',#35825,#35821,#32133,.T.);
#44607=EDGE_CURVE('',#35826,#35827,#3642,.T.);
#44608=EDGE_CURVE('',#35826,#35824,#32134,.T.);
#44609=EDGE_CURVE('',#35827,#35825,#32135,.T.);
#44610=EDGE_CURVE('',#35822,#35826,#32136,.T.);
#44611=EDGE_CURVE('',#35823,#35827,#32137,.T.);
#44612=EDGE_CURVE('',#35828,#35829,#3643,.T.);
#44613=EDGE_CURVE('',#35828,#35830,#32138,.T.);
#44614=EDGE_CURVE('',#35830,#35831,#3644,.T.);
#44615=EDGE_CURVE('',#35829,#35831,#32139,.T.);
#44616=EDGE_CURVE('',#35832,#35833,#3645,.T.);
#44617=EDGE_CURVE('',#35832,#35828,#32140,.T.);
#44618=EDGE_CURVE('',#35833,#35829,#32141,.T.);
#44619=EDGE_CURVE('',#35834,#35835,#3646,.T.);
#44620=EDGE_CURVE('',#35834,#35832,#32142,.T.);
#44621=EDGE_CURVE('',#35835,#35833,#32143,.T.);
#44622=EDGE_CURVE('',#35830,#35834,#32144,.T.);
#44623=EDGE_CURVE('',#35831,#35835,#32145,.T.);
#44624=EDGE_CURVE('',#35836,#35837,#3647,.T.);
#44625=EDGE_CURVE('',#35836,#35838,#32146,.T.);
#44626=EDGE_CURVE('',#35838,#35839,#3648,.T.);
#44627=EDGE_CURVE('',#35837,#35839,#32147,.T.);
#44628=EDGE_CURVE('',#35840,#35841,#3649,.T.);
#44629=EDGE_CURVE('',#35840,#35836,#32148,.T.);
#44630=EDGE_CURVE('',#35841,#35837,#32149,.T.);
#44631=EDGE_CURVE('',#35842,#35843,#3650,.T.);
#44632=EDGE_CURVE('',#35842,#35840,#32150,.T.);
#44633=EDGE_CURVE('',#35843,#35841,#32151,.T.);
#44634=EDGE_CURVE('',#35838,#35842,#32152,.T.);
#44635=EDGE_CURVE('',#35839,#35843,#32153,.T.);
#44636=EDGE_CURVE('',#35844,#35845,#3651,.T.);
#44637=EDGE_CURVE('',#35844,#35846,#32154,.T.);
#44638=EDGE_CURVE('',#35846,#35847,#3652,.T.);
#44639=EDGE_CURVE('',#35845,#35847,#32155,.T.);
#44640=EDGE_CURVE('',#35848,#35849,#3653,.T.);
#44641=EDGE_CURVE('',#35848,#35844,#32156,.T.);
#44642=EDGE_CURVE('',#35849,#35845,#32157,.T.);
#44643=EDGE_CURVE('',#35850,#35851,#3654,.T.);
#44644=EDGE_CURVE('',#35850,#35848,#32158,.T.);
#44645=EDGE_CURVE('',#35851,#35849,#32159,.T.);
#44646=EDGE_CURVE('',#35846,#35850,#32160,.T.);
#44647=EDGE_CURVE('',#35847,#35851,#32161,.T.);
#44648=EDGE_CURVE('',#35852,#35853,#3655,.T.);
#44649=EDGE_CURVE('',#35852,#35854,#32162,.T.);
#44650=EDGE_CURVE('',#35854,#35855,#3656,.T.);
#44651=EDGE_CURVE('',#35853,#35855,#32163,.T.);
#44652=EDGE_CURVE('',#35856,#35857,#3657,.T.);
#44653=EDGE_CURVE('',#35856,#35852,#32164,.T.);
#44654=EDGE_CURVE('',#35857,#35853,#32165,.T.);
#44655=EDGE_CURVE('',#35858,#35859,#3658,.T.);
#44656=EDGE_CURVE('',#35858,#35856,#32166,.T.);
#44657=EDGE_CURVE('',#35859,#35857,#32167,.T.);
#44658=EDGE_CURVE('',#35854,#35858,#32168,.T.);
#44659=EDGE_CURVE('',#35855,#35859,#32169,.T.);
#44660=EDGE_CURVE('',#35860,#35861,#3659,.T.);
#44661=EDGE_CURVE('',#35860,#35862,#32170,.T.);
#44662=EDGE_CURVE('',#35862,#35863,#3660,.T.);
#44663=EDGE_CURVE('',#35861,#35863,#32171,.T.);
#44664=EDGE_CURVE('',#35864,#35865,#3661,.T.);
#44665=EDGE_CURVE('',#35864,#35860,#32172,.T.);
#44666=EDGE_CURVE('',#35865,#35861,#32173,.T.);
#44667=EDGE_CURVE('',#35866,#35867,#3662,.T.);
#44668=EDGE_CURVE('',#35866,#35864,#32174,.T.);
#44669=EDGE_CURVE('',#35867,#35865,#32175,.T.);
#44670=EDGE_CURVE('',#35862,#35866,#32176,.T.);
#44671=EDGE_CURVE('',#35863,#35867,#32177,.T.);
#44672=EDGE_CURVE('',#35868,#35869,#3663,.T.);
#44673=EDGE_CURVE('',#35868,#35870,#32178,.T.);
#44674=EDGE_CURVE('',#35870,#35871,#3664,.T.);
#44675=EDGE_CURVE('',#35869,#35871,#32179,.T.);
#44676=EDGE_CURVE('',#35872,#35873,#3665,.T.);
#44677=EDGE_CURVE('',#35872,#35868,#32180,.T.);
#44678=EDGE_CURVE('',#35873,#35869,#32181,.T.);
#44679=EDGE_CURVE('',#35874,#35875,#3666,.T.);
#44680=EDGE_CURVE('',#35874,#35872,#32182,.T.);
#44681=EDGE_CURVE('',#35875,#35873,#32183,.T.);
#44682=EDGE_CURVE('',#35870,#35874,#32184,.T.);
#44683=EDGE_CURVE('',#35871,#35875,#32185,.T.);
#44684=EDGE_CURVE('',#35876,#35877,#3667,.T.);
#44685=EDGE_CURVE('',#35876,#35878,#32186,.T.);
#44686=EDGE_CURVE('',#35878,#35879,#3668,.T.);
#44687=EDGE_CURVE('',#35877,#35879,#32187,.T.);
#44688=EDGE_CURVE('',#35880,#35881,#3669,.T.);
#44689=EDGE_CURVE('',#35880,#35876,#32188,.T.);
#44690=EDGE_CURVE('',#35881,#35877,#32189,.T.);
#44691=EDGE_CURVE('',#35882,#35883,#3670,.T.);
#44692=EDGE_CURVE('',#35882,#35880,#32190,.T.);
#44693=EDGE_CURVE('',#35883,#35881,#32191,.T.);
#44694=EDGE_CURVE('',#35878,#35882,#32192,.T.);
#44695=EDGE_CURVE('',#35879,#35883,#32193,.T.);
#44696=EDGE_CURVE('',#35884,#35885,#3671,.T.);
#44697=EDGE_CURVE('',#35884,#35886,#32194,.T.);
#44698=EDGE_CURVE('',#35886,#35887,#3672,.T.);
#44699=EDGE_CURVE('',#35885,#35887,#32195,.T.);
#44700=EDGE_CURVE('',#35888,#35889,#3673,.T.);
#44701=EDGE_CURVE('',#35888,#35884,#32196,.T.);
#44702=EDGE_CURVE('',#35889,#35885,#32197,.T.);
#44703=EDGE_CURVE('',#35890,#35891,#3674,.T.);
#44704=EDGE_CURVE('',#35890,#35888,#32198,.T.);
#44705=EDGE_CURVE('',#35891,#35889,#32199,.T.);
#44706=EDGE_CURVE('',#35886,#35890,#32200,.T.);
#44707=EDGE_CURVE('',#35887,#35891,#32201,.T.);
#44708=EDGE_CURVE('',#35892,#35893,#3675,.T.);
#44709=EDGE_CURVE('',#35892,#35894,#32202,.T.);
#44710=EDGE_CURVE('',#35894,#35895,#3676,.T.);
#44711=EDGE_CURVE('',#35893,#35895,#32203,.T.);
#44712=EDGE_CURVE('',#35896,#35897,#3677,.T.);
#44713=EDGE_CURVE('',#35896,#35892,#32204,.T.);
#44714=EDGE_CURVE('',#35897,#35893,#32205,.T.);
#44715=EDGE_CURVE('',#35898,#35899,#3678,.T.);
#44716=EDGE_CURVE('',#35898,#35896,#32206,.T.);
#44717=EDGE_CURVE('',#35899,#35897,#32207,.T.);
#44718=EDGE_CURVE('',#35894,#35898,#32208,.T.);
#44719=EDGE_CURVE('',#35895,#35899,#32209,.T.);
#44720=EDGE_CURVE('',#35900,#35901,#3679,.T.);
#44721=EDGE_CURVE('',#35900,#35902,#32210,.T.);
#44722=EDGE_CURVE('',#35902,#35903,#3680,.T.);
#44723=EDGE_CURVE('',#35901,#35903,#32211,.T.);
#44724=EDGE_CURVE('',#35904,#35905,#3681,.T.);
#44725=EDGE_CURVE('',#35904,#35900,#32212,.T.);
#44726=EDGE_CURVE('',#35905,#35901,#32213,.T.);
#44727=EDGE_CURVE('',#35906,#35907,#3682,.T.);
#44728=EDGE_CURVE('',#35906,#35904,#32214,.T.);
#44729=EDGE_CURVE('',#35907,#35905,#32215,.T.);
#44730=EDGE_CURVE('',#35902,#35906,#32216,.T.);
#44731=EDGE_CURVE('',#35903,#35907,#32217,.T.);
#44732=EDGE_CURVE('',#35908,#35909,#3683,.T.);
#44733=EDGE_CURVE('',#35908,#35910,#32218,.T.);
#44734=EDGE_CURVE('',#35910,#35911,#3684,.T.);
#44735=EDGE_CURVE('',#35909,#35911,#32219,.T.);
#44736=EDGE_CURVE('',#35912,#35913,#3685,.T.);
#44737=EDGE_CURVE('',#35912,#35908,#32220,.T.);
#44738=EDGE_CURVE('',#35913,#35909,#32221,.T.);
#44739=EDGE_CURVE('',#35914,#35915,#3686,.T.);
#44740=EDGE_CURVE('',#35914,#35912,#32222,.T.);
#44741=EDGE_CURVE('',#35915,#35913,#32223,.T.);
#44742=EDGE_CURVE('',#35910,#35914,#32224,.T.);
#44743=EDGE_CURVE('',#35911,#35915,#32225,.T.);
#44744=EDGE_CURVE('',#35916,#35917,#3687,.T.);
#44745=EDGE_CURVE('',#35916,#35918,#32226,.T.);
#44746=EDGE_CURVE('',#35918,#35919,#3688,.T.);
#44747=EDGE_CURVE('',#35917,#35919,#32227,.T.);
#44748=EDGE_CURVE('',#35920,#35921,#3689,.T.);
#44749=EDGE_CURVE('',#35920,#35916,#32228,.T.);
#44750=EDGE_CURVE('',#35921,#35917,#32229,.T.);
#44751=EDGE_CURVE('',#35922,#35923,#3690,.T.);
#44752=EDGE_CURVE('',#35922,#35920,#32230,.T.);
#44753=EDGE_CURVE('',#35923,#35921,#32231,.T.);
#44754=EDGE_CURVE('',#35918,#35922,#32232,.T.);
#44755=EDGE_CURVE('',#35919,#35923,#32233,.T.);
#44756=EDGE_CURVE('',#35924,#35925,#3691,.T.);
#44757=EDGE_CURVE('',#35924,#35926,#32234,.T.);
#44758=EDGE_CURVE('',#35926,#35927,#3692,.T.);
#44759=EDGE_CURVE('',#35925,#35927,#32235,.T.);
#44760=EDGE_CURVE('',#35928,#35929,#3693,.T.);
#44761=EDGE_CURVE('',#35928,#35924,#32236,.T.);
#44762=EDGE_CURVE('',#35929,#35925,#32237,.T.);
#44763=EDGE_CURVE('',#35930,#35931,#3694,.T.);
#44764=EDGE_CURVE('',#35930,#35928,#32238,.T.);
#44765=EDGE_CURVE('',#35931,#35929,#32239,.T.);
#44766=EDGE_CURVE('',#35926,#35930,#32240,.T.);
#44767=EDGE_CURVE('',#35927,#35931,#32241,.T.);
#44768=EDGE_CURVE('',#35932,#35933,#3695,.T.);
#44769=EDGE_CURVE('',#35932,#35934,#32242,.T.);
#44770=EDGE_CURVE('',#35934,#35935,#3696,.T.);
#44771=EDGE_CURVE('',#35933,#35935,#32243,.T.);
#44772=EDGE_CURVE('',#35936,#35937,#3697,.T.);
#44773=EDGE_CURVE('',#35936,#35932,#32244,.T.);
#44774=EDGE_CURVE('',#35937,#35933,#32245,.T.);
#44775=EDGE_CURVE('',#35938,#35939,#3698,.T.);
#44776=EDGE_CURVE('',#35938,#35936,#32246,.T.);
#44777=EDGE_CURVE('',#35939,#35937,#32247,.T.);
#44778=EDGE_CURVE('',#35934,#35938,#32248,.T.);
#44779=EDGE_CURVE('',#35935,#35939,#32249,.T.);
#44780=EDGE_CURVE('',#35940,#35941,#3699,.T.);
#44781=EDGE_CURVE('',#35940,#35942,#32250,.T.);
#44782=EDGE_CURVE('',#35942,#35943,#3700,.T.);
#44783=EDGE_CURVE('',#35941,#35943,#32251,.T.);
#44784=EDGE_CURVE('',#35944,#35945,#3701,.T.);
#44785=EDGE_CURVE('',#35944,#35940,#32252,.T.);
#44786=EDGE_CURVE('',#35945,#35941,#32253,.T.);
#44787=EDGE_CURVE('',#35946,#35947,#3702,.T.);
#44788=EDGE_CURVE('',#35946,#35944,#32254,.T.);
#44789=EDGE_CURVE('',#35947,#35945,#32255,.T.);
#44790=EDGE_CURVE('',#35942,#35946,#32256,.T.);
#44791=EDGE_CURVE('',#35943,#35947,#32257,.T.);
#44792=EDGE_CURVE('',#35948,#35949,#3703,.T.);
#44793=EDGE_CURVE('',#35948,#35950,#32258,.T.);
#44794=EDGE_CURVE('',#35950,#35951,#3704,.T.);
#44795=EDGE_CURVE('',#35949,#35951,#32259,.T.);
#44796=EDGE_CURVE('',#35952,#35953,#3705,.T.);
#44797=EDGE_CURVE('',#35952,#35948,#32260,.T.);
#44798=EDGE_CURVE('',#35953,#35949,#32261,.T.);
#44799=EDGE_CURVE('',#35954,#35955,#3706,.T.);
#44800=EDGE_CURVE('',#35954,#35952,#32262,.T.);
#44801=EDGE_CURVE('',#35955,#35953,#32263,.T.);
#44802=EDGE_CURVE('',#35950,#35954,#32264,.T.);
#44803=EDGE_CURVE('',#35951,#35955,#32265,.T.);
#44804=EDGE_CURVE('',#35956,#35957,#3707,.T.);
#44805=EDGE_CURVE('',#35956,#35958,#32266,.T.);
#44806=EDGE_CURVE('',#35958,#35959,#3708,.T.);
#44807=EDGE_CURVE('',#35957,#35959,#32267,.T.);
#44808=EDGE_CURVE('',#35960,#35961,#3709,.T.);
#44809=EDGE_CURVE('',#35960,#35956,#32268,.T.);
#44810=EDGE_CURVE('',#35961,#35957,#32269,.T.);
#44811=EDGE_CURVE('',#35962,#35963,#3710,.T.);
#44812=EDGE_CURVE('',#35962,#35960,#32270,.T.);
#44813=EDGE_CURVE('',#35963,#35961,#32271,.T.);
#44814=EDGE_CURVE('',#35958,#35962,#32272,.T.);
#44815=EDGE_CURVE('',#35959,#35963,#32273,.T.);
#44816=EDGE_CURVE('',#35964,#35965,#3711,.T.);
#44817=EDGE_CURVE('',#35964,#35966,#32274,.T.);
#44818=EDGE_CURVE('',#35966,#35967,#3712,.T.);
#44819=EDGE_CURVE('',#35965,#35967,#32275,.T.);
#44820=EDGE_CURVE('',#35968,#35969,#3713,.T.);
#44821=EDGE_CURVE('',#35968,#35964,#32276,.T.);
#44822=EDGE_CURVE('',#35969,#35965,#32277,.T.);
#44823=EDGE_CURVE('',#35970,#35971,#3714,.T.);
#44824=EDGE_CURVE('',#35970,#35968,#32278,.T.);
#44825=EDGE_CURVE('',#35971,#35969,#32279,.T.);
#44826=EDGE_CURVE('',#35966,#35970,#32280,.T.);
#44827=EDGE_CURVE('',#35967,#35971,#32281,.T.);
#44828=EDGE_CURVE('',#35972,#35973,#3715,.T.);
#44829=EDGE_CURVE('',#35972,#35974,#32282,.T.);
#44830=EDGE_CURVE('',#35974,#35975,#3716,.T.);
#44831=EDGE_CURVE('',#35973,#35975,#32283,.T.);
#44832=EDGE_CURVE('',#35976,#35977,#3717,.T.);
#44833=EDGE_CURVE('',#35976,#35972,#32284,.T.);
#44834=EDGE_CURVE('',#35977,#35973,#32285,.T.);
#44835=EDGE_CURVE('',#35978,#35979,#3718,.T.);
#44836=EDGE_CURVE('',#35978,#35976,#32286,.T.);
#44837=EDGE_CURVE('',#35979,#35977,#32287,.T.);
#44838=EDGE_CURVE('',#35974,#35978,#32288,.T.);
#44839=EDGE_CURVE('',#35975,#35979,#32289,.T.);
#44840=EDGE_CURVE('',#35980,#35981,#3719,.T.);
#44841=EDGE_CURVE('',#35980,#35982,#32290,.T.);
#44842=EDGE_CURVE('',#35982,#35983,#3720,.T.);
#44843=EDGE_CURVE('',#35981,#35983,#32291,.T.);
#44844=EDGE_CURVE('',#35984,#35985,#3721,.T.);
#44845=EDGE_CURVE('',#35984,#35980,#32292,.T.);
#44846=EDGE_CURVE('',#35985,#35981,#32293,.T.);
#44847=EDGE_CURVE('',#35986,#35987,#3722,.T.);
#44848=EDGE_CURVE('',#35986,#35984,#32294,.T.);
#44849=EDGE_CURVE('',#35987,#35985,#32295,.T.);
#44850=EDGE_CURVE('',#35982,#35986,#32296,.T.);
#44851=EDGE_CURVE('',#35983,#35987,#32297,.T.);
#44852=EDGE_CURVE('',#35988,#35989,#3723,.T.);
#44853=EDGE_CURVE('',#35988,#35990,#32298,.T.);
#44854=EDGE_CURVE('',#35990,#35991,#3724,.T.);
#44855=EDGE_CURVE('',#35989,#35991,#32299,.T.);
#44856=EDGE_CURVE('',#35992,#35993,#3725,.T.);
#44857=EDGE_CURVE('',#35992,#35988,#32300,.T.);
#44858=EDGE_CURVE('',#35993,#35989,#32301,.T.);
#44859=EDGE_CURVE('',#35994,#35995,#3726,.T.);
#44860=EDGE_CURVE('',#35994,#35992,#32302,.T.);
#44861=EDGE_CURVE('',#35995,#35993,#32303,.T.);
#44862=EDGE_CURVE('',#35990,#35994,#32304,.T.);
#44863=EDGE_CURVE('',#35991,#35995,#32305,.T.);
#44864=EDGE_CURVE('',#35996,#35997,#3727,.T.);
#44865=EDGE_CURVE('',#35996,#35998,#32306,.T.);
#44866=EDGE_CURVE('',#35998,#35999,#3728,.T.);
#44867=EDGE_CURVE('',#35997,#35999,#32307,.T.);
#44868=EDGE_CURVE('',#36000,#36001,#3729,.T.);
#44869=EDGE_CURVE('',#36000,#35996,#32308,.T.);
#44870=EDGE_CURVE('',#36001,#35997,#32309,.T.);
#44871=EDGE_CURVE('',#36002,#36003,#3730,.T.);
#44872=EDGE_CURVE('',#36002,#36000,#32310,.T.);
#44873=EDGE_CURVE('',#36003,#36001,#32311,.T.);
#44874=EDGE_CURVE('',#35998,#36002,#32312,.T.);
#44875=EDGE_CURVE('',#35999,#36003,#32313,.T.);
#44876=EDGE_CURVE('',#36004,#36005,#3731,.T.);
#44877=EDGE_CURVE('',#36004,#36006,#32314,.T.);
#44878=EDGE_CURVE('',#36006,#36007,#3732,.T.);
#44879=EDGE_CURVE('',#36005,#36007,#32315,.T.);
#44880=EDGE_CURVE('',#36008,#36009,#3733,.T.);
#44881=EDGE_CURVE('',#36008,#36004,#32316,.T.);
#44882=EDGE_CURVE('',#36009,#36005,#32317,.T.);
#44883=EDGE_CURVE('',#36010,#36011,#3734,.T.);
#44884=EDGE_CURVE('',#36010,#36008,#32318,.T.);
#44885=EDGE_CURVE('',#36011,#36009,#32319,.T.);
#44886=EDGE_CURVE('',#36006,#36010,#32320,.T.);
#44887=EDGE_CURVE('',#36007,#36011,#32321,.T.);
#44888=EDGE_CURVE('',#36012,#36013,#3735,.T.);
#44889=EDGE_CURVE('',#36012,#36014,#32322,.T.);
#44890=EDGE_CURVE('',#36014,#36015,#3736,.T.);
#44891=EDGE_CURVE('',#36013,#36015,#32323,.T.);
#44892=EDGE_CURVE('',#36016,#36017,#3737,.T.);
#44893=EDGE_CURVE('',#36016,#36012,#32324,.T.);
#44894=EDGE_CURVE('',#36017,#36013,#32325,.T.);
#44895=EDGE_CURVE('',#36018,#36019,#3738,.T.);
#44896=EDGE_CURVE('',#36018,#36016,#32326,.T.);
#44897=EDGE_CURVE('',#36019,#36017,#32327,.T.);
#44898=EDGE_CURVE('',#36014,#36018,#32328,.T.);
#44899=EDGE_CURVE('',#36015,#36019,#32329,.T.);
#44900=EDGE_CURVE('',#36020,#36021,#3739,.T.);
#44901=EDGE_CURVE('',#36020,#36022,#32330,.T.);
#44902=EDGE_CURVE('',#36022,#36023,#3740,.T.);
#44903=EDGE_CURVE('',#36021,#36023,#32331,.T.);
#44904=EDGE_CURVE('',#36024,#36025,#3741,.T.);
#44905=EDGE_CURVE('',#36024,#36020,#32332,.T.);
#44906=EDGE_CURVE('',#36025,#36021,#32333,.T.);
#44907=EDGE_CURVE('',#36026,#36027,#3742,.T.);
#44908=EDGE_CURVE('',#36026,#36024,#32334,.T.);
#44909=EDGE_CURVE('',#36027,#36025,#32335,.T.);
#44910=EDGE_CURVE('',#36022,#36026,#32336,.T.);
#44911=EDGE_CURVE('',#36023,#36027,#32337,.T.);
#44912=EDGE_CURVE('',#36028,#36029,#3743,.T.);
#44913=EDGE_CURVE('',#36028,#36030,#32338,.T.);
#44914=EDGE_CURVE('',#36030,#36031,#3744,.T.);
#44915=EDGE_CURVE('',#36029,#36031,#32339,.T.);
#44916=EDGE_CURVE('',#36032,#36033,#3745,.T.);
#44917=EDGE_CURVE('',#36032,#36028,#32340,.T.);
#44918=EDGE_CURVE('',#36033,#36029,#32341,.T.);
#44919=EDGE_CURVE('',#36034,#36035,#3746,.T.);
#44920=EDGE_CURVE('',#36034,#36032,#32342,.T.);
#44921=EDGE_CURVE('',#36035,#36033,#32343,.T.);
#44922=EDGE_CURVE('',#36030,#36034,#32344,.T.);
#44923=EDGE_CURVE('',#36031,#36035,#32345,.T.);
#44924=EDGE_CURVE('',#36036,#36037,#3747,.T.);
#44925=EDGE_CURVE('',#36036,#36038,#32346,.T.);
#44926=EDGE_CURVE('',#36038,#36039,#3748,.T.);
#44927=EDGE_CURVE('',#36037,#36039,#32347,.T.);
#44928=EDGE_CURVE('',#36040,#36041,#3749,.T.);
#44929=EDGE_CURVE('',#36040,#36036,#32348,.T.);
#44930=EDGE_CURVE('',#36041,#36037,#32349,.T.);
#44931=EDGE_CURVE('',#36042,#36043,#3750,.T.);
#44932=EDGE_CURVE('',#36042,#36040,#32350,.T.);
#44933=EDGE_CURVE('',#36043,#36041,#32351,.T.);
#44934=EDGE_CURVE('',#36038,#36042,#32352,.T.);
#44935=EDGE_CURVE('',#36039,#36043,#32353,.T.);
#44936=EDGE_CURVE('',#36044,#36045,#3751,.T.);
#44937=EDGE_CURVE('',#36044,#36046,#32354,.T.);
#44938=EDGE_CURVE('',#36046,#36047,#3752,.T.);
#44939=EDGE_CURVE('',#36045,#36047,#32355,.T.);
#44940=EDGE_CURVE('',#36048,#36049,#3753,.T.);
#44941=EDGE_CURVE('',#36048,#36044,#32356,.T.);
#44942=EDGE_CURVE('',#36049,#36045,#32357,.T.);
#44943=EDGE_CURVE('',#36050,#36051,#3754,.T.);
#44944=EDGE_CURVE('',#36050,#36048,#32358,.T.);
#44945=EDGE_CURVE('',#36051,#36049,#32359,.T.);
#44946=EDGE_CURVE('',#36046,#36050,#32360,.T.);
#44947=EDGE_CURVE('',#36047,#36051,#32361,.T.);
#44948=EDGE_CURVE('',#36052,#36053,#3755,.T.);
#44949=EDGE_CURVE('',#36052,#36054,#32362,.T.);
#44950=EDGE_CURVE('',#36054,#36055,#3756,.T.);
#44951=EDGE_CURVE('',#36053,#36055,#32363,.T.);
#44952=EDGE_CURVE('',#36056,#36057,#3757,.T.);
#44953=EDGE_CURVE('',#36056,#36052,#32364,.T.);
#44954=EDGE_CURVE('',#36057,#36053,#32365,.T.);
#44955=EDGE_CURVE('',#36058,#36059,#3758,.T.);
#44956=EDGE_CURVE('',#36058,#36056,#32366,.T.);
#44957=EDGE_CURVE('',#36059,#36057,#32367,.T.);
#44958=EDGE_CURVE('',#36054,#36058,#32368,.T.);
#44959=EDGE_CURVE('',#36055,#36059,#32369,.T.);
#44960=EDGE_CURVE('',#36060,#36061,#3759,.T.);
#44961=EDGE_CURVE('',#36060,#36062,#32370,.T.);
#44962=EDGE_CURVE('',#36062,#36063,#3760,.T.);
#44963=EDGE_CURVE('',#36061,#36063,#32371,.T.);
#44964=EDGE_CURVE('',#36064,#36065,#3761,.T.);
#44965=EDGE_CURVE('',#36064,#36060,#32372,.T.);
#44966=EDGE_CURVE('',#36065,#36061,#32373,.T.);
#44967=EDGE_CURVE('',#36066,#36067,#3762,.T.);
#44968=EDGE_CURVE('',#36066,#36064,#32374,.T.);
#44969=EDGE_CURVE('',#36067,#36065,#32375,.T.);
#44970=EDGE_CURVE('',#36062,#36066,#32376,.T.);
#44971=EDGE_CURVE('',#36063,#36067,#32377,.T.);
#44972=EDGE_CURVE('',#36068,#36069,#3763,.T.);
#44973=EDGE_CURVE('',#36068,#36070,#32378,.T.);
#44974=EDGE_CURVE('',#36070,#36071,#3764,.T.);
#44975=EDGE_CURVE('',#36069,#36071,#32379,.T.);
#44976=EDGE_CURVE('',#36072,#36073,#3765,.T.);
#44977=EDGE_CURVE('',#36072,#36068,#32380,.T.);
#44978=EDGE_CURVE('',#36073,#36069,#32381,.T.);
#44979=EDGE_CURVE('',#36074,#36075,#3766,.T.);
#44980=EDGE_CURVE('',#36074,#36072,#32382,.T.);
#44981=EDGE_CURVE('',#36075,#36073,#32383,.T.);
#44982=EDGE_CURVE('',#36070,#36074,#32384,.T.);
#44983=EDGE_CURVE('',#36071,#36075,#32385,.T.);
#44984=EDGE_CURVE('',#36076,#36077,#3767,.T.);
#44985=EDGE_CURVE('',#36076,#36078,#32386,.T.);
#44986=EDGE_CURVE('',#36078,#36079,#3768,.T.);
#44987=EDGE_CURVE('',#36077,#36079,#32387,.T.);
#44988=EDGE_CURVE('',#36080,#36081,#3769,.T.);
#44989=EDGE_CURVE('',#36080,#36076,#32388,.T.);
#44990=EDGE_CURVE('',#36081,#36077,#32389,.T.);
#44991=EDGE_CURVE('',#36082,#36083,#3770,.T.);
#44992=EDGE_CURVE('',#36082,#36080,#32390,.T.);
#44993=EDGE_CURVE('',#36083,#36081,#32391,.T.);
#44994=EDGE_CURVE('',#36078,#36082,#32392,.T.);
#44995=EDGE_CURVE('',#36079,#36083,#32393,.T.);
#44996=EDGE_CURVE('',#36084,#36085,#3771,.T.);
#44997=EDGE_CURVE('',#36084,#36086,#32394,.T.);
#44998=EDGE_CURVE('',#36086,#36087,#3772,.T.);
#44999=EDGE_CURVE('',#36085,#36087,#32395,.T.);
#45000=EDGE_CURVE('',#36088,#36089,#3773,.T.);
#45001=EDGE_CURVE('',#36088,#36084,#32396,.T.);
#45002=EDGE_CURVE('',#36089,#36085,#32397,.T.);
#45003=EDGE_CURVE('',#36090,#36091,#3774,.T.);
#45004=EDGE_CURVE('',#36090,#36088,#32398,.T.);
#45005=EDGE_CURVE('',#36091,#36089,#32399,.T.);
#45006=EDGE_CURVE('',#36086,#36090,#32400,.T.);
#45007=EDGE_CURVE('',#36087,#36091,#32401,.T.);
#45008=EDGE_CURVE('',#36092,#36093,#3775,.T.);
#45009=EDGE_CURVE('',#36092,#36094,#32402,.T.);
#45010=EDGE_CURVE('',#36094,#36095,#3776,.T.);
#45011=EDGE_CURVE('',#36093,#36095,#32403,.T.);
#45012=EDGE_CURVE('',#36096,#36097,#3777,.T.);
#45013=EDGE_CURVE('',#36096,#36092,#32404,.T.);
#45014=EDGE_CURVE('',#36097,#36093,#32405,.T.);
#45015=EDGE_CURVE('',#36098,#36099,#3778,.T.);
#45016=EDGE_CURVE('',#36098,#36096,#32406,.T.);
#45017=EDGE_CURVE('',#36099,#36097,#32407,.T.);
#45018=EDGE_CURVE('',#36094,#36098,#32408,.T.);
#45019=EDGE_CURVE('',#36095,#36099,#32409,.T.);
#45020=EDGE_CURVE('',#36100,#36101,#3779,.T.);
#45021=EDGE_CURVE('',#36100,#36102,#32410,.T.);
#45022=EDGE_CURVE('',#36102,#36103,#3780,.T.);
#45023=EDGE_CURVE('',#36101,#36103,#32411,.T.);
#45024=EDGE_CURVE('',#36104,#36105,#3781,.T.);
#45025=EDGE_CURVE('',#36104,#36100,#32412,.T.);
#45026=EDGE_CURVE('',#36105,#36101,#32413,.T.);
#45027=EDGE_CURVE('',#36106,#36107,#3782,.T.);
#45028=EDGE_CURVE('',#36106,#36104,#32414,.T.);
#45029=EDGE_CURVE('',#36107,#36105,#32415,.T.);
#45030=EDGE_CURVE('',#36102,#36106,#32416,.T.);
#45031=EDGE_CURVE('',#36103,#36107,#32417,.T.);
#45032=EDGE_CURVE('',#36108,#36109,#3783,.T.);
#45033=EDGE_CURVE('',#36108,#36110,#32418,.T.);
#45034=EDGE_CURVE('',#36110,#36111,#3784,.T.);
#45035=EDGE_CURVE('',#36109,#36111,#32419,.T.);
#45036=EDGE_CURVE('',#36112,#36113,#3785,.T.);
#45037=EDGE_CURVE('',#36112,#36108,#32420,.T.);
#45038=EDGE_CURVE('',#36113,#36109,#32421,.T.);
#45039=EDGE_CURVE('',#36114,#36115,#3786,.T.);
#45040=EDGE_CURVE('',#36114,#36112,#32422,.T.);
#45041=EDGE_CURVE('',#36115,#36113,#32423,.T.);
#45042=EDGE_CURVE('',#36110,#36114,#32424,.T.);
#45043=EDGE_CURVE('',#36111,#36115,#32425,.T.);
#45044=EDGE_CURVE('',#36116,#36117,#3787,.T.);
#45045=EDGE_CURVE('',#36116,#36118,#32426,.T.);
#45046=EDGE_CURVE('',#36118,#36119,#3788,.T.);
#45047=EDGE_CURVE('',#36117,#36119,#32427,.T.);
#45048=EDGE_CURVE('',#36120,#36121,#3789,.T.);
#45049=EDGE_CURVE('',#36120,#36116,#32428,.T.);
#45050=EDGE_CURVE('',#36121,#36117,#32429,.T.);
#45051=EDGE_CURVE('',#36122,#36123,#3790,.T.);
#45052=EDGE_CURVE('',#36122,#36120,#32430,.T.);
#45053=EDGE_CURVE('',#36123,#36121,#32431,.T.);
#45054=EDGE_CURVE('',#36118,#36122,#32432,.T.);
#45055=EDGE_CURVE('',#36119,#36123,#32433,.T.);
#45056=EDGE_CURVE('',#36124,#36125,#3791,.T.);
#45057=EDGE_CURVE('',#36124,#36126,#32434,.T.);
#45058=EDGE_CURVE('',#36126,#36127,#3792,.T.);
#45059=EDGE_CURVE('',#36125,#36127,#32435,.T.);
#45060=EDGE_CURVE('',#36128,#36129,#3793,.T.);
#45061=EDGE_CURVE('',#36128,#36124,#32436,.T.);
#45062=EDGE_CURVE('',#36129,#36125,#32437,.T.);
#45063=EDGE_CURVE('',#36130,#36131,#3794,.T.);
#45064=EDGE_CURVE('',#36130,#36128,#32438,.T.);
#45065=EDGE_CURVE('',#36131,#36129,#32439,.T.);
#45066=EDGE_CURVE('',#36126,#36130,#32440,.T.);
#45067=EDGE_CURVE('',#36127,#36131,#32441,.T.);
#45068=EDGE_CURVE('',#36132,#36133,#3795,.T.);
#45069=EDGE_CURVE('',#36132,#36134,#32442,.T.);
#45070=EDGE_CURVE('',#36134,#36135,#3796,.T.);
#45071=EDGE_CURVE('',#36133,#36135,#32443,.T.);
#45072=EDGE_CURVE('',#36136,#36137,#3797,.T.);
#45073=EDGE_CURVE('',#36136,#36132,#32444,.T.);
#45074=EDGE_CURVE('',#36137,#36133,#32445,.T.);
#45075=EDGE_CURVE('',#36138,#36139,#3798,.T.);
#45076=EDGE_CURVE('',#36138,#36136,#32446,.T.);
#45077=EDGE_CURVE('',#36139,#36137,#32447,.T.);
#45078=EDGE_CURVE('',#36134,#36138,#32448,.T.);
#45079=EDGE_CURVE('',#36135,#36139,#32449,.T.);
#45080=EDGE_CURVE('',#36140,#36141,#3799,.T.);
#45081=EDGE_CURVE('',#36140,#36142,#32450,.T.);
#45082=EDGE_CURVE('',#36142,#36143,#3800,.T.);
#45083=EDGE_CURVE('',#36141,#36143,#32451,.T.);
#45084=EDGE_CURVE('',#36144,#36145,#3801,.T.);
#45085=EDGE_CURVE('',#36144,#36140,#32452,.T.);
#45086=EDGE_CURVE('',#36145,#36141,#32453,.T.);
#45087=EDGE_CURVE('',#36146,#36147,#3802,.T.);
#45088=EDGE_CURVE('',#36146,#36144,#32454,.T.);
#45089=EDGE_CURVE('',#36147,#36145,#32455,.T.);
#45090=EDGE_CURVE('',#36142,#36146,#32456,.T.);
#45091=EDGE_CURVE('',#36143,#36147,#32457,.T.);
#45092=EDGE_CURVE('',#36148,#36149,#3803,.T.);
#45093=EDGE_CURVE('',#36148,#36150,#32458,.T.);
#45094=EDGE_CURVE('',#36150,#36151,#3804,.T.);
#45095=EDGE_CURVE('',#36149,#36151,#32459,.T.);
#45096=EDGE_CURVE('',#36152,#36153,#3805,.T.);
#45097=EDGE_CURVE('',#36152,#36148,#32460,.T.);
#45098=EDGE_CURVE('',#36153,#36149,#32461,.T.);
#45099=EDGE_CURVE('',#36154,#36155,#3806,.T.);
#45100=EDGE_CURVE('',#36154,#36152,#32462,.T.);
#45101=EDGE_CURVE('',#36155,#36153,#32463,.T.);
#45102=EDGE_CURVE('',#36150,#36154,#32464,.T.);
#45103=EDGE_CURVE('',#36151,#36155,#32465,.T.);
#45104=EDGE_CURVE('',#36156,#36157,#3807,.T.);
#45105=EDGE_CURVE('',#36156,#36158,#32466,.T.);
#45106=EDGE_CURVE('',#36158,#36159,#3808,.T.);
#45107=EDGE_CURVE('',#36157,#36159,#32467,.T.);
#45108=EDGE_CURVE('',#36160,#36161,#3809,.T.);
#45109=EDGE_CURVE('',#36160,#36156,#32468,.T.);
#45110=EDGE_CURVE('',#36161,#36157,#32469,.T.);
#45111=EDGE_CURVE('',#36162,#36163,#3810,.T.);
#45112=EDGE_CURVE('',#36162,#36160,#32470,.T.);
#45113=EDGE_CURVE('',#36163,#36161,#32471,.T.);
#45114=EDGE_CURVE('',#36158,#36162,#32472,.T.);
#45115=EDGE_CURVE('',#36159,#36163,#32473,.T.);
#45116=EDGE_CURVE('',#36164,#36165,#3811,.T.);
#45117=EDGE_CURVE('',#36164,#36166,#32474,.T.);
#45118=EDGE_CURVE('',#36166,#36167,#3812,.T.);
#45119=EDGE_CURVE('',#36165,#36167,#32475,.T.);
#45120=EDGE_CURVE('',#36168,#36169,#3813,.T.);
#45121=EDGE_CURVE('',#36168,#36164,#32476,.T.);
#45122=EDGE_CURVE('',#36169,#36165,#32477,.T.);
#45123=EDGE_CURVE('',#36170,#36171,#3814,.T.);
#45124=EDGE_CURVE('',#36170,#36168,#32478,.T.);
#45125=EDGE_CURVE('',#36171,#36169,#32479,.T.);
#45126=EDGE_CURVE('',#36166,#36170,#32480,.T.);
#45127=EDGE_CURVE('',#36167,#36171,#32481,.T.);
#45128=EDGE_CURVE('',#36172,#36173,#3815,.T.);
#45129=EDGE_CURVE('',#36172,#36174,#32482,.T.);
#45130=EDGE_CURVE('',#36174,#36175,#3816,.T.);
#45131=EDGE_CURVE('',#36173,#36175,#32483,.T.);
#45132=EDGE_CURVE('',#36176,#36177,#3817,.T.);
#45133=EDGE_CURVE('',#36176,#36172,#32484,.T.);
#45134=EDGE_CURVE('',#36177,#36173,#32485,.T.);
#45135=EDGE_CURVE('',#36178,#36179,#3818,.T.);
#45136=EDGE_CURVE('',#36178,#36176,#32486,.T.);
#45137=EDGE_CURVE('',#36179,#36177,#32487,.T.);
#45138=EDGE_CURVE('',#36174,#36178,#32488,.T.);
#45139=EDGE_CURVE('',#36175,#36179,#32489,.T.);
#45140=EDGE_CURVE('',#36180,#36181,#3819,.T.);
#45141=EDGE_CURVE('',#36180,#36182,#32490,.T.);
#45142=EDGE_CURVE('',#36182,#36183,#3820,.T.);
#45143=EDGE_CURVE('',#36181,#36183,#32491,.T.);
#45144=EDGE_CURVE('',#36184,#36185,#3821,.T.);
#45145=EDGE_CURVE('',#36186,#36184,#3822,.T.);
#45146=EDGE_CURVE('',#36186,#36180,#32492,.T.);
#45147=EDGE_CURVE('',#36185,#36181,#32493,.T.);
#45148=EDGE_CURVE('',#36187,#36188,#3823,.T.);
#45149=EDGE_CURVE('',#36184,#36187,#3824,.T.);
#45150=EDGE_CURVE('',#36188,#36185,#32494,.T.);
#45151=EDGE_CURVE('',#36187,#36182,#3825,.T.);
#45152=EDGE_CURVE('',#36183,#36188,#32495,.T.);
#45153=EDGE_CURVE('',#36182,#36186,#32496,.T.);
#45154=EDGE_CURVE('',#36189,#36190,#3826,.T.);
#45155=EDGE_CURVE('',#36189,#36191,#32497,.T.);
#45156=EDGE_CURVE('',#36191,#36192,#3827,.T.);
#45157=EDGE_CURVE('',#36190,#36192,#32498,.T.);
#45158=EDGE_CURVE('',#36193,#36194,#3828,.T.);
#45159=EDGE_CURVE('',#36195,#36193,#3829,.T.);
#45160=EDGE_CURVE('',#36195,#36189,#32499,.T.);
#45161=EDGE_CURVE('',#36194,#36190,#32500,.T.);
#45162=EDGE_CURVE('',#36196,#36197,#3830,.T.);
#45163=EDGE_CURVE('',#36193,#36196,#3831,.T.);
#45164=EDGE_CURVE('',#36197,#36194,#32501,.T.);
#45165=EDGE_CURVE('',#36191,#36198,#32502,.T.);
#45166=EDGE_CURVE('',#36196,#36198,#3832,.T.);
#45167=EDGE_CURVE('',#36192,#36197,#32503,.T.);
#45168=EDGE_CURVE('',#36198,#36195,#32504,.T.);
#45169=EDGE_CURVE('',#36199,#36200,#3833,.T.);
#45170=EDGE_CURVE('',#36199,#36201,#32505,.T.);
#45171=EDGE_CURVE('',#36201,#36202,#3834,.T.);
#45172=EDGE_CURVE('',#36200,#36202,#32506,.T.);
#45173=EDGE_CURVE('',#36203,#36204,#3835,.T.);
#45174=EDGE_CURVE('',#36205,#36203,#3836,.T.);
#45175=EDGE_CURVE('',#36205,#36199,#32507,.T.);
#45176=EDGE_CURVE('',#36204,#36200,#32508,.T.);
#45177=EDGE_CURVE('',#36206,#36207,#3837,.T.);
#45178=EDGE_CURVE('',#36203,#36206,#3838,.T.);
#45179=EDGE_CURVE('',#36207,#36204,#32509,.T.);
#45180=EDGE_CURVE('',#36201,#36208,#32510,.T.);
#45181=EDGE_CURVE('',#36206,#36208,#3839,.T.);
#45182=EDGE_CURVE('',#36202,#36207,#32511,.T.);
#45183=EDGE_CURVE('',#36208,#36205,#32512,.T.);
#45184=EDGE_CURVE('',#36209,#36210,#3840,.T.);
#45185=EDGE_CURVE('',#36209,#36211,#32513,.T.);
#45186=EDGE_CURVE('',#36211,#36212,#3841,.T.);
#45187=EDGE_CURVE('',#36210,#36212,#32514,.T.);
#45188=EDGE_CURVE('',#36213,#36214,#3842,.T.);
#45189=EDGE_CURVE('',#36215,#36213,#3843,.T.);
#45190=EDGE_CURVE('',#36215,#36209,#32515,.T.);
#45191=EDGE_CURVE('',#36214,#36210,#32516,.T.);
#45192=EDGE_CURVE('',#36216,#36217,#3844,.T.);
#45193=EDGE_CURVE('',#36213,#36216,#3845,.T.);
#45194=EDGE_CURVE('',#36217,#36214,#32517,.T.);
#45195=EDGE_CURVE('',#36211,#36218,#32518,.T.);
#45196=EDGE_CURVE('',#36216,#36218,#3846,.T.);
#45197=EDGE_CURVE('',#36212,#36217,#32519,.T.);
#45198=EDGE_CURVE('',#36218,#36215,#32520,.T.);
#45199=EDGE_CURVE('',#36219,#36220,#3847,.T.);
#45200=EDGE_CURVE('',#36219,#36221,#32521,.T.);
#45201=EDGE_CURVE('',#36221,#36222,#3848,.T.);
#45202=EDGE_CURVE('',#36220,#36222,#32522,.T.);
#45203=EDGE_CURVE('',#36223,#36224,#3849,.T.);
#45204=EDGE_CURVE('',#36225,#36223,#3850,.T.);
#45205=EDGE_CURVE('',#36225,#36219,#32523,.T.);
#45206=EDGE_CURVE('',#36224,#36220,#32524,.T.);
#45207=EDGE_CURVE('',#36226,#36227,#3851,.T.);
#45208=EDGE_CURVE('',#36223,#36226,#3852,.T.);
#45209=EDGE_CURVE('',#36227,#36224,#32525,.T.);
#45210=EDGE_CURVE('',#36221,#36228,#32526,.T.);
#45211=EDGE_CURVE('',#36226,#36228,#3853,.T.);
#45212=EDGE_CURVE('',#36222,#36227,#32527,.T.);
#45213=EDGE_CURVE('',#36228,#36225,#32528,.T.);
#45214=EDGE_CURVE('',#36229,#36230,#3854,.T.);
#45215=EDGE_CURVE('',#36231,#36229,#3855,.T.);
#45216=EDGE_CURVE('',#36231,#36232,#32529,.T.);
#45217=EDGE_CURVE('',#36232,#36233,#3856,.T.);
#45218=EDGE_CURVE('',#36230,#36233,#32530,.T.);
#45219=EDGE_CURVE('',#36234,#36235,#3857,.T.);
#45220=EDGE_CURVE('',#36229,#36234,#3858,.T.);
#45221=EDGE_CURVE('',#36235,#36230,#32531,.T.);
#45222=EDGE_CURVE('',#36236,#36237,#3859,.T.);
#45223=EDGE_CURVE('',#36234,#36236,#3860,.T.);
#45224=EDGE_CURVE('',#36237,#36235,#32532,.T.);
#45225=EDGE_CURVE('',#36232,#36238,#32533,.T.);
#45226=EDGE_CURVE('',#36236,#36238,#3861,.T.);
#45227=EDGE_CURVE('',#36233,#36237,#32534,.T.);
#45228=EDGE_CURVE('',#36238,#36231,#32535,.T.);
#45229=EDGE_CURVE('',#36239,#36240,#3862,.T.);
#45230=EDGE_CURVE('',#36241,#36239,#3863,.T.);
#45231=EDGE_CURVE('',#36241,#36242,#32536,.T.);
#45232=EDGE_CURVE('',#36242,#36243,#3864,.T.);
#45233=EDGE_CURVE('',#36240,#36243,#32537,.T.);
#45234=EDGE_CURVE('',#36244,#36245,#3865,.T.);
#45235=EDGE_CURVE('',#36239,#36244,#3866,.T.);
#45236=EDGE_CURVE('',#36245,#36240,#32538,.T.);
#45237=EDGE_CURVE('',#36246,#36247,#3867,.T.);
#45238=EDGE_CURVE('',#36244,#36246,#3868,.T.);
#45239=EDGE_CURVE('',#36247,#36245,#32539,.T.);
#45240=EDGE_CURVE('',#36242,#36248,#32540,.T.);
#45241=EDGE_CURVE('',#36246,#36248,#3869,.T.);
#45242=EDGE_CURVE('',#36243,#36247,#32541,.T.);
#45243=EDGE_CURVE('',#36248,#36241,#32542,.T.);
#45244=EDGE_CURVE('',#36249,#36250,#3870,.T.);
#45245=EDGE_CURVE('',#36249,#36251,#32543,.T.);
#45246=EDGE_CURVE('',#36251,#36252,#3871,.T.);
#45247=EDGE_CURVE('',#36250,#36252,#32544,.T.);
#45248=EDGE_CURVE('',#36253,#36254,#3872,.T.);
#45249=EDGE_CURVE('',#36255,#36253,#3873,.T.);
#45250=EDGE_CURVE('',#36255,#36249,#32545,.T.);
#45251=EDGE_CURVE('',#36254,#36250,#32546,.T.);
#45252=EDGE_CURVE('',#36256,#36257,#3874,.T.);
#45253=EDGE_CURVE('',#36253,#36256,#3875,.T.);
#45254=EDGE_CURVE('',#36257,#36254,#32547,.T.);
#45255=EDGE_CURVE('',#36251,#36258,#32548,.T.);
#45256=EDGE_CURVE('',#36256,#36258,#3876,.T.);
#45257=EDGE_CURVE('',#36252,#36257,#32549,.T.);
#45258=EDGE_CURVE('',#36258,#36255,#32550,.T.);
#45259=EDGE_CURVE('',#36259,#36260,#3877,.T.);
#45260=EDGE_CURVE('',#36259,#36261,#32551,.T.);
#45261=EDGE_CURVE('',#36261,#36262,#3878,.T.);
#45262=EDGE_CURVE('',#36260,#36262,#32552,.T.);
#45263=EDGE_CURVE('',#36263,#36264,#3879,.T.);
#45264=EDGE_CURVE('',#36265,#36263,#3880,.T.);
#45265=EDGE_CURVE('',#36265,#36259,#32553,.T.);
#45266=EDGE_CURVE('',#36264,#36260,#32554,.T.);
#45267=EDGE_CURVE('',#36266,#36267,#3881,.T.);
#45268=EDGE_CURVE('',#36263,#36266,#3882,.T.);
#45269=EDGE_CURVE('',#36267,#36264,#32555,.T.);
#45270=EDGE_CURVE('',#36261,#36268,#32556,.T.);
#45271=EDGE_CURVE('',#36266,#36268,#3883,.T.);
#45272=EDGE_CURVE('',#36262,#36267,#32557,.T.);
#45273=EDGE_CURVE('',#36268,#36265,#32558,.T.);
#45274=EDGE_CURVE('',#36269,#36270,#3884,.T.);
#45275=EDGE_CURVE('',#36269,#36271,#32559,.T.);
#45276=EDGE_CURVE('',#36271,#36272,#3885,.T.);
#45277=EDGE_CURVE('',#36270,#36272,#32560,.T.);
#45278=EDGE_CURVE('',#36273,#36274,#3886,.T.);
#45279=EDGE_CURVE('',#36275,#36273,#3887,.T.);
#45280=EDGE_CURVE('',#36275,#36269,#32561,.T.);
#45281=EDGE_CURVE('',#36274,#36270,#32562,.T.);
#45282=EDGE_CURVE('',#36276,#36277,#3888,.T.);
#45283=EDGE_CURVE('',#36273,#36276,#3889,.T.);
#45284=EDGE_CURVE('',#36277,#36274,#32563,.T.);
#45285=EDGE_CURVE('',#36271,#36278,#32564,.T.);
#45286=EDGE_CURVE('',#36276,#36278,#3890,.T.);
#45287=EDGE_CURVE('',#36272,#36277,#32565,.T.);
#45288=EDGE_CURVE('',#36278,#36275,#32566,.T.);
#45289=EDGE_CURVE('',#36279,#36280,#3891,.T.);
#45290=EDGE_CURVE('',#36279,#36281,#32567,.T.);
#45291=EDGE_CURVE('',#36281,#36282,#3892,.T.);
#45292=EDGE_CURVE('',#36280,#36282,#32568,.T.);
#45293=EDGE_CURVE('',#36283,#36284,#3893,.T.);
#45294=EDGE_CURVE('',#36283,#36279,#32569,.T.);
#45295=EDGE_CURVE('',#36284,#36280,#32570,.T.);
#45296=EDGE_CURVE('',#36285,#36286,#3894,.T.);
#45297=EDGE_CURVE('',#36285,#36283,#32571,.T.);
#45298=EDGE_CURVE('',#36286,#36284,#32572,.T.);
#45299=EDGE_CURVE('',#36281,#36285,#32573,.T.);
#45300=EDGE_CURVE('',#36282,#36286,#32574,.T.);
#45301=EDGE_CURVE('',#36287,#36288,#3895,.T.);
#45302=EDGE_CURVE('',#36287,#36289,#32575,.T.);
#45303=EDGE_CURVE('',#36289,#36290,#3896,.T.);
#45304=EDGE_CURVE('',#36288,#36290,#32576,.T.);
#45305=EDGE_CURVE('',#36291,#36292,#3897,.T.);
#45306=EDGE_CURVE('',#36291,#36287,#32577,.T.);
#45307=EDGE_CURVE('',#36292,#36288,#32578,.T.);
#45308=EDGE_CURVE('',#36293,#36294,#3898,.T.);
#45309=EDGE_CURVE('',#36293,#36291,#32579,.T.);
#45310=EDGE_CURVE('',#36294,#36292,#32580,.T.);
#45311=EDGE_CURVE('',#36289,#36293,#32581,.T.);
#45312=EDGE_CURVE('',#36290,#36294,#32582,.T.);
#45313=EDGE_CURVE('',#36295,#36296,#3899,.T.);
#45314=EDGE_CURVE('',#36295,#36297,#32583,.T.);
#45315=EDGE_CURVE('',#36297,#36298,#3900,.T.);
#45316=EDGE_CURVE('',#36296,#36298,#32584,.T.);
#45317=EDGE_CURVE('',#36299,#36300,#3901,.T.);
#45318=EDGE_CURVE('',#36299,#36295,#32585,.T.);
#45319=EDGE_CURVE('',#36300,#36296,#32586,.T.);
#45320=EDGE_CURVE('',#36301,#36302,#3902,.T.);
#45321=EDGE_CURVE('',#36301,#36299,#32587,.T.);
#45322=EDGE_CURVE('',#36302,#36300,#32588,.T.);
#45323=EDGE_CURVE('',#36297,#36301,#32589,.T.);
#45324=EDGE_CURVE('',#36298,#36302,#32590,.T.);
#45325=EDGE_CURVE('',#36303,#36304,#3903,.T.);
#45326=EDGE_CURVE('',#36303,#36305,#32591,.T.);
#45327=EDGE_CURVE('',#36305,#36306,#3904,.T.);
#45328=EDGE_CURVE('',#36304,#36306,#32592,.T.);
#45329=EDGE_CURVE('',#36307,#36308,#3905,.T.);
#45330=EDGE_CURVE('',#36307,#36303,#32593,.T.);
#45331=EDGE_CURVE('',#36308,#36304,#32594,.T.);
#45332=EDGE_CURVE('',#36309,#36310,#3906,.T.);
#45333=EDGE_CURVE('',#36309,#36307,#32595,.T.);
#45334=EDGE_CURVE('',#36310,#36308,#32596,.T.);
#45335=EDGE_CURVE('',#36305,#36309,#32597,.T.);
#45336=EDGE_CURVE('',#36306,#36310,#32598,.T.);
#45337=EDGE_CURVE('',#36311,#36312,#3907,.T.);
#45338=EDGE_CURVE('',#36311,#36313,#32599,.T.);
#45339=EDGE_CURVE('',#36313,#36314,#3908,.T.);
#45340=EDGE_CURVE('',#36312,#36314,#32600,.T.);
#45341=EDGE_CURVE('',#36315,#36316,#3909,.T.);
#45342=EDGE_CURVE('',#36315,#36311,#32601,.T.);
#45343=EDGE_CURVE('',#36316,#36312,#32602,.T.);
#45344=EDGE_CURVE('',#36317,#36318,#3910,.T.);
#45345=EDGE_CURVE('',#36317,#36315,#32603,.T.);
#45346=EDGE_CURVE('',#36318,#36316,#32604,.T.);
#45347=EDGE_CURVE('',#36313,#36317,#32605,.T.);
#45348=EDGE_CURVE('',#36314,#36318,#32606,.T.);
#45349=EDGE_CURVE('',#36319,#36320,#3911,.T.);
#45350=EDGE_CURVE('',#36319,#36321,#32607,.T.);
#45351=EDGE_CURVE('',#36321,#36322,#3912,.T.);
#45352=EDGE_CURVE('',#36320,#36322,#32608,.T.);
#45353=EDGE_CURVE('',#36323,#36324,#3913,.T.);
#45354=EDGE_CURVE('',#36323,#36319,#32609,.T.);
#45355=EDGE_CURVE('',#36324,#36320,#32610,.T.);
#45356=EDGE_CURVE('',#36325,#36326,#3914,.T.);
#45357=EDGE_CURVE('',#36325,#36323,#32611,.T.);
#45358=EDGE_CURVE('',#36326,#36324,#32612,.T.);
#45359=EDGE_CURVE('',#36321,#36325,#32613,.T.);
#45360=EDGE_CURVE('',#36322,#36326,#32614,.T.);
#45361=EDGE_CURVE('',#36327,#36328,#3915,.T.);
#45362=EDGE_CURVE('',#36327,#36329,#32615,.T.);
#45363=EDGE_CURVE('',#36329,#36330,#3916,.T.);
#45364=EDGE_CURVE('',#36328,#36330,#32616,.T.);
#45365=EDGE_CURVE('',#36331,#36332,#3917,.T.);
#45366=EDGE_CURVE('',#36331,#36327,#32617,.T.);
#45367=EDGE_CURVE('',#36332,#36328,#32618,.T.);
#45368=EDGE_CURVE('',#36333,#36334,#3918,.T.);
#45369=EDGE_CURVE('',#36333,#36331,#32619,.T.);
#45370=EDGE_CURVE('',#36334,#36332,#32620,.T.);
#45371=EDGE_CURVE('',#36329,#36333,#32621,.T.);
#45372=EDGE_CURVE('',#36330,#36334,#32622,.T.);
#45373=EDGE_CURVE('',#36335,#36336,#3919,.T.);
#45374=EDGE_CURVE('',#36335,#36337,#32623,.T.);
#45375=EDGE_CURVE('',#36337,#36338,#3920,.T.);
#45376=EDGE_CURVE('',#36336,#36338,#32624,.T.);
#45377=EDGE_CURVE('',#36339,#36340,#3921,.T.);
#45378=EDGE_CURVE('',#36339,#36335,#32625,.T.);
#45379=EDGE_CURVE('',#36340,#36336,#32626,.T.);
#45380=EDGE_CURVE('',#36341,#36342,#3922,.T.);
#45381=EDGE_CURVE('',#36341,#36339,#32627,.T.);
#45382=EDGE_CURVE('',#36342,#36340,#32628,.T.);
#45383=EDGE_CURVE('',#36337,#36341,#32629,.T.);
#45384=EDGE_CURVE('',#36338,#36342,#32630,.T.);
#45385=EDGE_CURVE('',#36343,#36344,#3923,.T.);
#45386=EDGE_CURVE('',#36345,#36343,#3924,.T.);
#45387=EDGE_CURVE('',#36345,#36346,#32631,.T.);
#45388=EDGE_CURVE('',#36346,#36347,#3925,.T.);
#45389=EDGE_CURVE('',#36344,#36347,#32632,.T.);
#45390=EDGE_CURVE('',#36348,#36349,#3926,.T.);
#45391=EDGE_CURVE('',#36343,#36348,#3927,.T.);
#45392=EDGE_CURVE('',#36349,#36344,#32633,.T.);
#45393=EDGE_CURVE('',#36350,#36351,#3928,.T.);
#45394=EDGE_CURVE('',#36348,#36350,#3929,.T.);
#45395=EDGE_CURVE('',#36351,#36349,#32634,.T.);
#45396=EDGE_CURVE('',#36346,#36352,#32635,.T.);
#45397=EDGE_CURVE('',#36350,#36352,#3930,.T.);
#45398=EDGE_CURVE('',#36347,#36351,#32636,.T.);
#45399=EDGE_CURVE('',#36352,#36345,#32637,.T.);
#45400=EDGE_CURVE('',#36353,#36354,#3931,.T.);
#45401=EDGE_CURVE('',#36355,#36353,#3932,.T.);
#45402=EDGE_CURVE('',#36355,#36356,#32638,.T.);
#45403=EDGE_CURVE('',#36356,#36357,#3933,.T.);
#45404=EDGE_CURVE('',#36354,#36357,#32639,.T.);
#45405=EDGE_CURVE('',#36358,#36359,#3934,.T.);
#45406=EDGE_CURVE('',#36353,#36358,#3935,.T.);
#45407=EDGE_CURVE('',#36359,#36354,#32640,.T.);
#45408=EDGE_CURVE('',#36360,#36361,#3936,.T.);
#45409=EDGE_CURVE('',#36358,#36360,#3937,.T.);
#45410=EDGE_CURVE('',#36361,#36359,#32641,.T.);
#45411=EDGE_CURVE('',#36356,#36362,#32642,.T.);
#45412=EDGE_CURVE('',#36360,#36362,#3938,.T.);
#45413=EDGE_CURVE('',#36357,#36361,#32643,.T.);
#45414=EDGE_CURVE('',#36362,#36355,#32644,.T.);
#45415=EDGE_CURVE('',#36363,#36364,#3939,.T.);
#45416=EDGE_CURVE('',#36363,#36365,#32645,.T.);
#45417=EDGE_CURVE('',#36365,#36366,#3940,.T.);
#45418=EDGE_CURVE('',#36364,#36366,#32646,.T.);
#45419=EDGE_CURVE('',#36367,#36368,#3941,.T.);
#45420=EDGE_CURVE('',#36367,#36363,#32647,.T.);
#45421=EDGE_CURVE('',#36368,#36364,#32648,.T.);
#45422=EDGE_CURVE('',#36369,#36370,#3942,.T.);
#45423=EDGE_CURVE('',#36369,#36367,#32649,.T.);
#45424=EDGE_CURVE('',#36370,#36368,#32650,.T.);
#45425=EDGE_CURVE('',#36365,#36369,#32651,.T.);
#45426=EDGE_CURVE('',#36366,#36370,#32652,.T.);
#45427=EDGE_CURVE('',#36371,#36372,#3943,.T.);
#45428=EDGE_CURVE('',#36371,#36373,#32653,.T.);
#45429=EDGE_CURVE('',#36373,#36374,#3944,.T.);
#45430=EDGE_CURVE('',#36372,#36374,#32654,.T.);
#45431=EDGE_CURVE('',#36375,#36376,#3945,.T.);
#45432=EDGE_CURVE('',#36375,#36371,#32655,.T.);
#45433=EDGE_CURVE('',#36376,#36372,#32656,.T.);
#45434=EDGE_CURVE('',#36377,#36378,#3946,.T.);
#45435=EDGE_CURVE('',#36377,#36375,#32657,.T.);
#45436=EDGE_CURVE('',#36378,#36376,#32658,.T.);
#45437=EDGE_CURVE('',#36373,#36377,#32659,.T.);
#45438=EDGE_CURVE('',#36374,#36378,#32660,.T.);
#45439=EDGE_CURVE('',#36379,#36380,#3947,.T.);
#45440=EDGE_CURVE('',#36379,#36381,#32661,.T.);
#45441=EDGE_CURVE('',#36381,#36382,#3948,.T.);
#45442=EDGE_CURVE('',#36380,#36382,#32662,.T.);
#45443=EDGE_CURVE('',#36383,#36384,#3949,.T.);
#45444=EDGE_CURVE('',#36383,#36379,#32663,.T.);
#45445=EDGE_CURVE('',#36384,#36380,#32664,.T.);
#45446=EDGE_CURVE('',#36385,#36386,#3950,.T.);
#45447=EDGE_CURVE('',#36385,#36383,#32665,.T.);
#45448=EDGE_CURVE('',#36386,#36384,#32666,.T.);
#45449=EDGE_CURVE('',#36381,#36385,#32667,.T.);
#45450=EDGE_CURVE('',#36382,#36386,#32668,.T.);
#45451=EDGE_CURVE('',#36387,#36388,#3951,.T.);
#45452=EDGE_CURVE('',#36387,#36389,#32669,.T.);
#45453=EDGE_CURVE('',#36389,#36390,#3952,.T.);
#45454=EDGE_CURVE('',#36388,#36390,#32670,.T.);
#45455=EDGE_CURVE('',#36391,#36392,#3953,.T.);
#45456=EDGE_CURVE('',#36391,#36387,#32671,.T.);
#45457=EDGE_CURVE('',#36392,#36388,#32672,.T.);
#45458=EDGE_CURVE('',#36393,#36394,#3954,.T.);
#45459=EDGE_CURVE('',#36393,#36391,#32673,.T.);
#45460=EDGE_CURVE('',#36394,#36392,#32674,.T.);
#45461=EDGE_CURVE('',#36389,#36393,#32675,.T.);
#45462=EDGE_CURVE('',#36390,#36394,#32676,.T.);
#45463=EDGE_CURVE('',#36395,#36396,#3955,.T.);
#45464=EDGE_CURVE('',#36395,#36397,#32677,.T.);
#45465=EDGE_CURVE('',#36397,#36398,#3956,.T.);
#45466=EDGE_CURVE('',#36396,#36398,#32678,.T.);
#45467=EDGE_CURVE('',#36399,#36400,#3957,.T.);
#45468=EDGE_CURVE('',#36399,#36395,#32679,.T.);
#45469=EDGE_CURVE('',#36400,#36396,#32680,.T.);
#45470=EDGE_CURVE('',#36401,#36402,#3958,.T.);
#45471=EDGE_CURVE('',#36403,#36401,#3959,.T.);
#45472=EDGE_CURVE('',#36403,#36399,#32681,.T.);
#45473=EDGE_CURVE('',#36402,#36400,#32682,.T.);
#45474=EDGE_CURVE('',#36397,#36404,#32683,.T.);
#45475=EDGE_CURVE('',#36401,#36404,#3960,.T.);
#45476=EDGE_CURVE('',#36398,#36402,#32684,.T.);
#45477=EDGE_CURVE('',#36404,#36403,#32685,.T.);
#45478=EDGE_CURVE('',#36405,#36406,#3961,.T.);
#45479=EDGE_CURVE('',#36405,#36407,#32686,.T.);
#45480=EDGE_CURVE('',#36407,#36408,#3962,.T.);
#45481=EDGE_CURVE('',#36406,#36408,#32687,.T.);
#45482=EDGE_CURVE('',#36409,#36410,#3963,.T.);
#45483=EDGE_CURVE('',#36411,#36409,#3964,.T.);
#45484=EDGE_CURVE('',#36411,#36405,#32688,.T.);
#45485=EDGE_CURVE('',#36410,#36406,#32689,.T.);
#45486=EDGE_CURVE('',#36412,#36413,#3965,.T.);
#45487=EDGE_CURVE('',#36409,#36412,#3966,.T.);
#45488=EDGE_CURVE('',#36413,#36410,#32690,.T.);
#45489=EDGE_CURVE('',#36407,#36414,#32691,.T.);
#45490=EDGE_CURVE('',#36412,#36414,#3967,.T.);
#45491=EDGE_CURVE('',#36408,#36413,#32692,.T.);
#45492=EDGE_CURVE('',#36414,#36411,#32693,.T.);
#45493=EDGE_CURVE('',#36415,#36416,#3968,.T.);
#45494=EDGE_CURVE('',#36415,#36417,#32694,.T.);
#45495=EDGE_CURVE('',#36417,#36418,#3969,.T.);
#45496=EDGE_CURVE('',#36416,#36418,#32695,.T.);
#45497=EDGE_CURVE('',#36419,#36420,#3970,.T.);
#45498=EDGE_CURVE('',#36421,#36419,#3971,.T.);
#45499=EDGE_CURVE('',#36421,#36415,#32696,.T.);
#45500=EDGE_CURVE('',#36420,#36416,#32697,.T.);
#45501=EDGE_CURVE('',#36422,#36423,#3972,.T.);
#45502=EDGE_CURVE('',#36419,#36422,#3973,.T.);
#45503=EDGE_CURVE('',#36423,#36420,#32698,.T.);
#45504=EDGE_CURVE('',#36417,#36424,#32699,.T.);
#45505=EDGE_CURVE('',#36422,#36424,#3974,.T.);
#45506=EDGE_CURVE('',#36418,#36423,#32700,.T.);
#45507=EDGE_CURVE('',#36424,#36421,#32701,.T.);
#45508=EDGE_CURVE('',#36425,#36426,#3975,.T.);
#45509=EDGE_CURVE('',#36425,#36427,#32702,.T.);
#45510=EDGE_CURVE('',#36427,#36428,#3976,.T.);
#45511=EDGE_CURVE('',#36426,#36428,#32703,.T.);
#45512=EDGE_CURVE('',#36429,#36430,#3977,.T.);
#45513=EDGE_CURVE('',#36429,#36425,#32704,.T.);
#45514=EDGE_CURVE('',#36430,#36426,#32705,.T.);
#45515=EDGE_CURVE('',#36431,#36432,#3978,.T.);
#45516=EDGE_CURVE('',#36433,#36431,#3979,.T.);
#45517=EDGE_CURVE('',#36433,#36429,#32706,.T.);
#45518=EDGE_CURVE('',#36432,#36430,#32707,.T.);
#45519=EDGE_CURVE('',#36427,#36434,#32708,.T.);
#45520=EDGE_CURVE('',#36431,#36434,#3980,.T.);
#45521=EDGE_CURVE('',#36428,#36432,#32709,.T.);
#45522=EDGE_CURVE('',#36434,#36433,#32710,.T.);
#45523=EDGE_CURVE('',#36435,#36436,#3981,.T.);
#45524=EDGE_CURVE('',#36435,#36437,#32711,.T.);
#45525=EDGE_CURVE('',#36437,#36438,#3982,.T.);
#45526=EDGE_CURVE('',#36436,#36438,#32712,.T.);
#45527=EDGE_CURVE('',#36439,#36440,#3983,.T.);
#45528=EDGE_CURVE('',#36439,#36435,#32713,.T.);
#45529=EDGE_CURVE('',#36440,#36436,#32714,.T.);
#45530=EDGE_CURVE('',#36441,#36442,#3984,.T.);
#45531=EDGE_CURVE('',#36441,#36439,#32715,.T.);
#45532=EDGE_CURVE('',#36442,#36440,#32716,.T.);
#45533=EDGE_CURVE('',#36437,#36441,#32717,.T.);
#45534=EDGE_CURVE('',#36438,#36442,#32718,.T.);
#45535=EDGE_CURVE('',#36443,#36444,#3985,.T.);
#45536=EDGE_CURVE('',#36443,#36445,#32719,.T.);
#45537=EDGE_CURVE('',#36445,#36446,#3986,.T.);
#45538=EDGE_CURVE('',#36444,#36446,#32720,.T.);
#45539=EDGE_CURVE('',#36447,#36448,#3987,.T.);
#45540=EDGE_CURVE('',#36447,#36443,#32721,.T.);
#45541=EDGE_CURVE('',#36448,#36444,#32722,.T.);
#45542=EDGE_CURVE('',#36449,#36450,#3988,.T.);
#45543=EDGE_CURVE('',#36449,#36447,#32723,.T.);
#45544=EDGE_CURVE('',#36450,#36448,#32724,.T.);
#45545=EDGE_CURVE('',#36445,#36449,#32725,.T.);
#45546=EDGE_CURVE('',#36446,#36450,#32726,.T.);
#45547=EDGE_CURVE('',#36451,#36452,#3989,.T.);
#45548=EDGE_CURVE('',#36451,#36453,#32727,.T.);
#45549=EDGE_CURVE('',#36453,#36454,#3990,.T.);
#45550=EDGE_CURVE('',#36452,#36454,#32728,.T.);
#45551=EDGE_CURVE('',#36455,#36456,#3991,.T.);
#45552=EDGE_CURVE('',#36455,#36451,#32729,.T.);
#45553=EDGE_CURVE('',#36456,#36452,#32730,.T.);
#45554=EDGE_CURVE('',#36457,#36458,#3992,.T.);
#45555=EDGE_CURVE('',#36457,#36455,#32731,.T.);
#45556=EDGE_CURVE('',#36458,#36456,#32732,.T.);
#45557=EDGE_CURVE('',#36453,#36457,#32733,.T.);
#45558=EDGE_CURVE('',#36454,#36458,#32734,.T.);
#45559=EDGE_CURVE('',#36459,#36460,#3993,.T.);
#45560=EDGE_CURVE('',#36459,#36461,#32735,.T.);
#45561=EDGE_CURVE('',#36461,#36462,#3994,.T.);
#45562=EDGE_CURVE('',#36460,#36462,#32736,.T.);
#45563=EDGE_CURVE('',#36463,#36464,#3995,.T.);
#45564=EDGE_CURVE('',#36463,#36459,#32737,.T.);
#45565=EDGE_CURVE('',#36464,#36460,#32738,.T.);
#45566=EDGE_CURVE('',#36465,#36466,#3996,.T.);
#45567=EDGE_CURVE('',#36465,#36463,#32739,.T.);
#45568=EDGE_CURVE('',#36466,#36464,#32740,.T.);
#45569=EDGE_CURVE('',#36461,#36465,#32741,.T.);
#45570=EDGE_CURVE('',#36462,#36466,#32742,.T.);
#45571=EDGE_CURVE('',#36467,#36468,#3997,.T.);
#45572=EDGE_CURVE('',#36467,#36469,#32743,.T.);
#45573=EDGE_CURVE('',#36469,#36470,#3998,.T.);
#45574=EDGE_CURVE('',#36468,#36470,#32744,.T.);
#45575=EDGE_CURVE('',#36471,#36472,#3999,.T.);
#45576=EDGE_CURVE('',#36471,#36467,#32745,.T.);
#45577=EDGE_CURVE('',#36472,#36468,#32746,.T.);
#45578=EDGE_CURVE('',#36473,#36474,#4000,.T.);
#45579=EDGE_CURVE('',#36473,#36471,#32747,.T.);
#45580=EDGE_CURVE('',#36474,#36472,#32748,.T.);
#45581=EDGE_CURVE('',#36469,#36473,#32749,.T.);
#45582=EDGE_CURVE('',#36470,#36474,#32750,.T.);
#45583=EDGE_CURVE('',#36475,#36476,#4001,.T.);
#45584=EDGE_CURVE('',#36475,#36477,#32751,.T.);
#45585=EDGE_CURVE('',#36477,#36478,#4002,.T.);
#45586=EDGE_CURVE('',#36476,#36478,#32752,.T.);
#45587=EDGE_CURVE('',#36479,#36480,#4003,.T.);
#45588=EDGE_CURVE('',#36479,#36475,#32753,.T.);
#45589=EDGE_CURVE('',#36480,#36476,#32754,.T.);
#45590=EDGE_CURVE('',#36481,#36482,#4004,.T.);
#45591=EDGE_CURVE('',#36481,#36479,#32755,.T.);
#45592=EDGE_CURVE('',#36482,#36480,#32756,.T.);
#45593=EDGE_CURVE('',#36477,#36481,#32757,.T.);
#45594=EDGE_CURVE('',#36478,#36482,#32758,.T.);
#45595=EDGE_CURVE('',#36483,#36484,#4005,.T.);
#45596=EDGE_CURVE('',#36483,#36485,#32759,.T.);
#45597=EDGE_CURVE('',#36485,#36486,#4006,.T.);
#45598=EDGE_CURVE('',#36484,#36486,#32760,.T.);
#45599=EDGE_CURVE('',#36487,#36488,#4007,.T.);
#45600=EDGE_CURVE('',#36487,#36483,#32761,.T.);
#45601=EDGE_CURVE('',#36488,#36484,#32762,.T.);
#45602=EDGE_CURVE('',#36489,#36490,#4008,.T.);
#45603=EDGE_CURVE('',#36489,#36487,#32763,.T.);
#45604=EDGE_CURVE('',#36490,#36488,#32764,.T.);
#45605=EDGE_CURVE('',#36485,#36489,#32765,.T.);
#45606=EDGE_CURVE('',#36486,#36490,#32766,.T.);
#45607=EDGE_CURVE('',#36491,#36492,#4009,.T.);
#45608=EDGE_CURVE('',#36491,#36493,#32767,.T.);
#45609=EDGE_CURVE('',#36493,#36494,#4010,.T.);
#45610=EDGE_CURVE('',#36492,#36494,#32768,.T.);
#45611=EDGE_CURVE('',#36495,#36496,#4011,.T.);
#45612=EDGE_CURVE('',#36495,#36491,#32769,.T.);
#45613=EDGE_CURVE('',#36496,#36492,#32770,.T.);
#45614=EDGE_CURVE('',#36497,#36498,#4012,.T.);
#45615=EDGE_CURVE('',#36497,#36495,#32771,.T.);
#45616=EDGE_CURVE('',#36498,#36496,#32772,.T.);
#45617=EDGE_CURVE('',#36493,#36497,#32773,.T.);
#45618=EDGE_CURVE('',#36494,#36498,#32774,.T.);
#45619=EDGE_CURVE('',#36499,#36500,#4013,.T.);
#45620=EDGE_CURVE('',#36499,#36501,#32775,.T.);
#45621=EDGE_CURVE('',#36501,#36502,#4014,.T.);
#45622=EDGE_CURVE('',#36500,#36502,#32776,.T.);
#45623=EDGE_CURVE('',#36503,#36504,#4015,.T.);
#45624=EDGE_CURVE('',#36503,#36499,#32777,.T.);
#45625=EDGE_CURVE('',#36504,#36500,#32778,.T.);
#45626=EDGE_CURVE('',#36505,#36506,#4016,.T.);
#45627=EDGE_CURVE('',#36505,#36503,#32779,.T.);
#45628=EDGE_CURVE('',#36506,#36504,#32780,.T.);
#45629=EDGE_CURVE('',#36501,#36505,#32781,.T.);
#45630=EDGE_CURVE('',#36502,#36506,#32782,.T.);
#45631=EDGE_CURVE('',#36507,#36508,#4017,.T.);
#45632=EDGE_CURVE('',#36507,#36509,#32783,.T.);
#45633=EDGE_CURVE('',#36509,#36510,#4018,.T.);
#45634=EDGE_CURVE('',#36508,#36510,#32784,.T.);
#45635=EDGE_CURVE('',#36511,#36512,#4019,.T.);
#45636=EDGE_CURVE('',#36511,#36507,#32785,.T.);
#45637=EDGE_CURVE('',#36512,#36508,#32786,.T.);
#45638=EDGE_CURVE('',#36513,#36514,#4020,.T.);
#45639=EDGE_CURVE('',#36513,#36511,#32787,.T.);
#45640=EDGE_CURVE('',#36514,#36512,#32788,.T.);
#45641=EDGE_CURVE('',#36509,#36513,#32789,.T.);
#45642=EDGE_CURVE('',#36510,#36514,#32790,.T.);
#45643=EDGE_CURVE('',#36515,#36516,#4021,.T.);
#45644=EDGE_CURVE('',#36515,#36517,#32791,.T.);
#45645=EDGE_CURVE('',#36517,#36518,#4022,.T.);
#45646=EDGE_CURVE('',#36516,#36518,#32792,.T.);
#45647=EDGE_CURVE('',#36519,#36520,#4023,.T.);
#45648=EDGE_CURVE('',#36519,#36515,#32793,.T.);
#45649=EDGE_CURVE('',#36520,#36516,#32794,.T.);
#45650=EDGE_CURVE('',#36521,#36522,#4024,.T.);
#45651=EDGE_CURVE('',#36523,#36521,#4025,.T.);
#45652=EDGE_CURVE('',#36523,#36519,#32795,.T.);
#45653=EDGE_CURVE('',#36522,#36520,#32796,.T.);
#45654=EDGE_CURVE('',#36517,#36524,#32797,.T.);
#45655=EDGE_CURVE('',#36521,#36524,#4026,.T.);
#45656=EDGE_CURVE('',#36518,#36522,#32798,.T.);
#45657=EDGE_CURVE('',#36524,#36523,#32799,.T.);
#45658=EDGE_CURVE('',#36525,#36526,#4027,.T.);
#45659=EDGE_CURVE('',#36525,#36527,#32800,.T.);
#45660=EDGE_CURVE('',#36527,#36528,#4028,.T.);
#45661=EDGE_CURVE('',#36526,#36528,#32801,.T.);
#45662=EDGE_CURVE('',#36529,#36530,#4029,.T.);
#45663=EDGE_CURVE('',#36529,#36525,#32802,.T.);
#45664=EDGE_CURVE('',#36530,#36526,#32803,.T.);
#45665=EDGE_CURVE('',#36531,#36532,#4030,.T.);
#45666=EDGE_CURVE('',#36533,#36531,#4031,.T.);
#45667=EDGE_CURVE('',#36533,#36529,#32804,.T.);
#45668=EDGE_CURVE('',#36532,#36530,#32805,.T.);
#45669=EDGE_CURVE('',#36527,#36534,#32806,.T.);
#45670=EDGE_CURVE('',#36531,#36534,#4032,.T.);
#45671=EDGE_CURVE('',#36528,#36532,#32807,.T.);
#45672=EDGE_CURVE('',#36534,#36533,#32808,.T.);
#45673=EDGE_CURVE('',#36535,#36536,#4033,.T.);
#45674=EDGE_CURVE('',#36535,#36537,#32809,.T.);
#45675=EDGE_CURVE('',#36537,#36538,#4034,.T.);
#45676=EDGE_CURVE('',#36536,#36538,#32810,.T.);
#45677=EDGE_CURVE('',#36539,#36540,#4035,.T.);
#45678=EDGE_CURVE('',#36539,#36535,#32811,.T.);
#45679=EDGE_CURVE('',#36540,#36536,#32812,.T.);
#45680=EDGE_CURVE('',#36541,#36542,#4036,.T.);
#45681=EDGE_CURVE('',#36541,#36539,#32813,.T.);
#45682=EDGE_CURVE('',#36542,#36540,#32814,.T.);
#45683=EDGE_CURVE('',#36537,#36541,#32815,.T.);
#45684=EDGE_CURVE('',#36538,#36542,#32816,.T.);
#45685=EDGE_CURVE('',#36543,#36544,#4037,.T.);
#45686=EDGE_CURVE('',#36543,#36545,#32817,.T.);
#45687=EDGE_CURVE('',#36545,#36546,#4038,.T.);
#45688=EDGE_CURVE('',#36544,#36546,#32818,.T.);
#45689=EDGE_CURVE('',#36547,#36548,#4039,.T.);
#45690=EDGE_CURVE('',#36547,#36543,#32819,.T.);
#45691=EDGE_CURVE('',#36548,#36544,#32820,.T.);
#45692=EDGE_CURVE('',#36549,#36550,#4040,.T.);
#45693=EDGE_CURVE('',#36549,#36547,#32821,.T.);
#45694=EDGE_CURVE('',#36550,#36548,#32822,.T.);
#45695=EDGE_CURVE('',#36545,#36549,#32823,.T.);
#45696=EDGE_CURVE('',#36546,#36550,#32824,.T.);
#45697=EDGE_CURVE('',#36551,#36552,#4041,.T.);
#45698=EDGE_CURVE('',#36551,#36553,#32825,.T.);
#45699=EDGE_CURVE('',#36553,#36554,#4042,.T.);
#45700=EDGE_CURVE('',#36552,#36554,#32826,.T.);
#45701=EDGE_CURVE('',#36555,#36556,#4043,.T.);
#45702=EDGE_CURVE('',#36555,#36551,#32827,.T.);
#45703=EDGE_CURVE('',#36556,#36552,#32828,.T.);
#45704=EDGE_CURVE('',#36557,#36558,#4044,.T.);
#45705=EDGE_CURVE('',#36557,#36555,#32829,.T.);
#45706=EDGE_CURVE('',#36558,#36556,#32830,.T.);
#45707=EDGE_CURVE('',#36553,#36557,#32831,.T.);
#45708=EDGE_CURVE('',#36554,#36558,#32832,.T.);
#45709=EDGE_CURVE('',#36559,#36560,#4045,.T.);
#45710=EDGE_CURVE('',#36559,#36561,#32833,.T.);
#45711=EDGE_CURVE('',#36561,#36562,#4046,.T.);
#45712=EDGE_CURVE('',#36560,#36562,#32834,.T.);
#45713=EDGE_CURVE('',#36563,#36564,#4047,.T.);
#45714=EDGE_CURVE('',#36563,#36559,#32835,.T.);
#45715=EDGE_CURVE('',#36564,#36560,#32836,.T.);
#45716=EDGE_CURVE('',#36565,#36566,#4048,.T.);
#45717=EDGE_CURVE('',#36565,#36563,#32837,.T.);
#45718=EDGE_CURVE('',#36566,#36564,#32838,.T.);
#45719=EDGE_CURVE('',#36561,#36565,#32839,.T.);
#45720=EDGE_CURVE('',#36562,#36566,#32840,.T.);
#45721=EDGE_CURVE('',#36567,#36568,#4049,.T.);
#45722=EDGE_CURVE('',#36567,#36569,#32841,.T.);
#45723=EDGE_CURVE('',#36569,#36570,#4050,.T.);
#45724=EDGE_CURVE('',#36568,#36570,#32842,.T.);
#45725=EDGE_CURVE('',#36571,#36572,#4051,.T.);
#45726=EDGE_CURVE('',#36571,#36567,#32843,.T.);
#45727=EDGE_CURVE('',#36572,#36568,#32844,.T.);
#45728=EDGE_CURVE('',#36573,#36574,#4052,.T.);
#45729=EDGE_CURVE('',#36573,#36571,#32845,.T.);
#45730=EDGE_CURVE('',#36574,#36572,#32846,.T.);
#45731=EDGE_CURVE('',#36569,#36573,#32847,.T.);
#45732=EDGE_CURVE('',#36570,#36574,#32848,.T.);
#45733=EDGE_CURVE('',#36575,#36576,#4053,.T.);
#45734=EDGE_CURVE('',#36575,#36577,#32849,.T.);
#45735=EDGE_CURVE('',#36577,#36578,#4054,.T.);
#45736=EDGE_CURVE('',#36576,#36578,#32850,.T.);
#45737=EDGE_CURVE('',#36579,#36580,#4055,.T.);
#45738=EDGE_CURVE('',#36579,#36575,#32851,.T.);
#45739=EDGE_CURVE('',#36580,#36576,#32852,.T.);
#45740=EDGE_CURVE('',#36581,#36582,#4056,.T.);
#45741=EDGE_CURVE('',#36581,#36579,#32853,.T.);
#45742=EDGE_CURVE('',#36582,#36580,#32854,.T.);
#45743=EDGE_CURVE('',#36577,#36581,#32855,.T.);
#45744=EDGE_CURVE('',#36578,#36582,#32856,.T.);
#45745=EDGE_CURVE('',#36583,#36584,#4057,.T.);
#45746=EDGE_CURVE('',#36583,#36585,#32857,.T.);
#45747=EDGE_CURVE('',#36585,#36586,#4058,.T.);
#45748=EDGE_CURVE('',#36584,#36586,#32858,.T.);
#45749=EDGE_CURVE('',#36587,#36588,#4059,.T.);
#45750=EDGE_CURVE('',#36587,#36583,#32859,.T.);
#45751=EDGE_CURVE('',#36588,#36584,#32860,.T.);
#45752=EDGE_CURVE('',#36589,#36590,#4060,.T.);
#45753=EDGE_CURVE('',#36589,#36587,#32861,.T.);
#45754=EDGE_CURVE('',#36590,#36588,#32862,.T.);
#45755=EDGE_CURVE('',#36585,#36589,#32863,.T.);
#45756=EDGE_CURVE('',#36586,#36590,#32864,.T.);
#45757=EDGE_CURVE('',#36591,#36592,#4061,.T.);
#45758=EDGE_CURVE('',#36591,#36593,#32865,.T.);
#45759=EDGE_CURVE('',#36593,#36594,#4062,.T.);
#45760=EDGE_CURVE('',#36592,#36594,#32866,.T.);
#45761=EDGE_CURVE('',#36595,#36596,#4063,.T.);
#45762=EDGE_CURVE('',#36595,#36591,#32867,.T.);
#45763=EDGE_CURVE('',#36596,#36592,#32868,.T.);
#45764=EDGE_CURVE('',#36597,#36598,#4064,.T.);
#45765=EDGE_CURVE('',#36597,#36595,#32869,.T.);
#45766=EDGE_CURVE('',#36598,#36596,#32870,.T.);
#45767=EDGE_CURVE('',#36593,#36597,#32871,.T.);
#45768=EDGE_CURVE('',#36594,#36598,#32872,.T.);
#45769=EDGE_CURVE('',#36599,#36600,#4065,.T.);
#45770=EDGE_CURVE('',#36599,#36601,#32873,.T.);
#45771=EDGE_CURVE('',#36601,#36602,#4066,.T.);
#45772=EDGE_CURVE('',#36600,#36602,#32874,.T.);
#45773=EDGE_CURVE('',#36603,#36604,#4067,.T.);
#45774=EDGE_CURVE('',#36603,#36599,#32875,.T.);
#45775=EDGE_CURVE('',#36604,#36600,#32876,.T.);
#45776=EDGE_CURVE('',#36605,#36606,#4068,.T.);
#45777=EDGE_CURVE('',#36605,#36603,#32877,.T.);
#45778=EDGE_CURVE('',#36606,#36604,#32878,.T.);
#45779=EDGE_CURVE('',#36601,#36605,#32879,.T.);
#45780=EDGE_CURVE('',#36602,#36606,#32880,.T.);
#45781=EDGE_CURVE('',#36607,#36608,#4069,.T.);
#45782=EDGE_CURVE('',#36607,#36609,#32881,.T.);
#45783=EDGE_CURVE('',#36609,#36610,#4070,.T.);
#45784=EDGE_CURVE('',#36608,#36610,#32882,.T.);
#45785=EDGE_CURVE('',#36611,#36612,#4071,.T.);
#45786=EDGE_CURVE('',#36613,#36611,#4072,.T.);
#45787=EDGE_CURVE('',#36613,#36607,#32883,.T.);
#45788=EDGE_CURVE('',#36612,#36608,#32884,.T.);
#45789=EDGE_CURVE('',#36614,#36615,#4073,.T.);
#45790=EDGE_CURVE('',#36611,#36614,#4074,.T.);
#45791=EDGE_CURVE('',#36615,#36612,#32885,.T.);
#45792=EDGE_CURVE('',#36609,#36616,#32886,.T.);
#45793=EDGE_CURVE('',#36614,#36616,#4075,.T.);
#45794=EDGE_CURVE('',#36610,#36615,#32887,.T.);
#45795=EDGE_CURVE('',#36616,#36613,#32888,.T.);
#45796=EDGE_CURVE('',#36617,#36618,#4076,.T.);
#45797=EDGE_CURVE('',#36617,#36619,#32889,.T.);
#45798=EDGE_CURVE('',#36619,#36620,#4077,.T.);
#45799=EDGE_CURVE('',#36618,#36620,#32890,.T.);
#45800=EDGE_CURVE('',#36621,#36622,#4078,.T.);
#45801=EDGE_CURVE('',#36621,#36617,#32891,.T.);
#45802=EDGE_CURVE('',#36622,#36618,#32892,.T.);
#45803=EDGE_CURVE('',#36623,#36624,#4079,.T.);
#45804=EDGE_CURVE('',#36625,#36623,#4080,.T.);
#45805=EDGE_CURVE('',#36625,#36621,#32893,.T.);
#45806=EDGE_CURVE('',#36624,#36622,#32894,.T.);
#45807=EDGE_CURVE('',#36619,#36626,#32895,.T.);
#45808=EDGE_CURVE('',#36623,#36626,#4081,.T.);
#45809=EDGE_CURVE('',#36620,#36624,#32896,.T.);
#45810=EDGE_CURVE('',#36626,#36625,#32897,.T.);
#45811=EDGE_CURVE('',#36627,#36628,#4082,.T.);
#45812=EDGE_CURVE('',#36627,#36629,#32898,.T.);
#45813=EDGE_CURVE('',#36629,#36630,#4083,.T.);
#45814=EDGE_CURVE('',#36628,#36630,#32899,.T.);
#45815=EDGE_CURVE('',#36631,#36632,#4084,.T.);
#45816=EDGE_CURVE('',#36631,#36627,#32900,.T.);
#45817=EDGE_CURVE('',#36632,#36628,#32901,.T.);
#45818=EDGE_CURVE('',#36633,#36634,#4085,.T.);
#45819=EDGE_CURVE('',#36633,#36631,#32902,.T.);
#45820=EDGE_CURVE('',#36634,#36632,#32903,.T.);
#45821=EDGE_CURVE('',#36629,#36633,#32904,.T.);
#45822=EDGE_CURVE('',#36630,#36634,#32905,.T.);
#45823=EDGE_CURVE('',#36635,#36636,#4086,.T.);
#45824=EDGE_CURVE('',#36635,#36637,#32906,.T.);
#45825=EDGE_CURVE('',#36637,#36638,#4087,.T.);
#45826=EDGE_CURVE('',#36636,#36638,#32907,.T.);
#45827=EDGE_CURVE('',#36639,#36640,#4088,.T.);
#45828=EDGE_CURVE('',#36639,#36635,#32908,.T.);
#45829=EDGE_CURVE('',#36640,#36636,#32909,.T.);
#45830=EDGE_CURVE('',#36641,#36642,#4089,.T.);
#45831=EDGE_CURVE('',#36641,#36639,#32910,.T.);
#45832=EDGE_CURVE('',#36642,#36640,#32911,.T.);
#45833=EDGE_CURVE('',#36637,#36641,#32912,.T.);
#45834=EDGE_CURVE('',#36638,#36642,#32913,.T.);
#45835=EDGE_CURVE('',#36643,#36644,#4090,.T.);
#45836=EDGE_CURVE('',#36643,#36645,#32914,.T.);
#45837=EDGE_CURVE('',#36645,#36646,#4091,.T.);
#45838=EDGE_CURVE('',#36644,#36646,#32915,.T.);
#45839=EDGE_CURVE('',#36647,#36648,#4092,.T.);
#45840=EDGE_CURVE('',#36647,#36643,#32916,.T.);
#45841=EDGE_CURVE('',#36648,#36644,#32917,.T.);
#45842=EDGE_CURVE('',#36649,#36650,#4093,.T.);
#45843=EDGE_CURVE('',#36649,#36647,#32918,.T.);
#45844=EDGE_CURVE('',#36650,#36648,#32919,.T.);
#45845=EDGE_CURVE('',#36645,#36649,#32920,.T.);
#45846=EDGE_CURVE('',#36646,#36650,#32921,.T.);
#45847=EDGE_CURVE('',#36651,#36652,#4094,.T.);
#45848=EDGE_CURVE('',#36651,#36653,#32922,.T.);
#45849=EDGE_CURVE('',#36653,#36654,#4095,.T.);
#45850=EDGE_CURVE('',#36652,#36654,#32923,.T.);
#45851=EDGE_CURVE('',#36655,#36656,#4096,.T.);
#45852=EDGE_CURVE('',#36655,#36651,#32924,.T.);
#45853=EDGE_CURVE('',#36656,#36652,#32925,.T.);
#45854=EDGE_CURVE('',#36657,#36658,#4097,.T.);
#45855=EDGE_CURVE('',#36657,#36655,#32926,.T.);
#45856=EDGE_CURVE('',#36658,#36656,#32927,.T.);
#45857=EDGE_CURVE('',#36653,#36657,#32928,.T.);
#45858=EDGE_CURVE('',#36654,#36658,#32929,.T.);
#45859=EDGE_CURVE('',#36659,#36660,#4098,.T.);
#45860=EDGE_CURVE('',#36659,#36661,#32930,.T.);
#45861=EDGE_CURVE('',#36661,#36662,#4099,.T.);
#45862=EDGE_CURVE('',#36660,#36662,#32931,.T.);
#45863=EDGE_CURVE('',#36663,#36664,#4100,.T.);
#45864=EDGE_CURVE('',#36663,#36659,#32932,.T.);
#45865=EDGE_CURVE('',#36664,#36660,#32933,.T.);
#45866=EDGE_CURVE('',#36665,#36666,#4101,.T.);
#45867=EDGE_CURVE('',#36665,#36663,#32934,.T.);
#45868=EDGE_CURVE('',#36666,#36664,#32935,.T.);
#45869=EDGE_CURVE('',#36661,#36665,#32936,.T.);
#45870=EDGE_CURVE('',#36662,#36666,#32937,.T.);
#45871=EDGE_CURVE('',#36667,#36668,#4102,.T.);
#45872=EDGE_CURVE('',#36667,#36669,#32938,.T.);
#45873=EDGE_CURVE('',#36669,#36670,#4103,.T.);
#45874=EDGE_CURVE('',#36668,#36670,#32939,.T.);
#45875=EDGE_CURVE('',#36671,#36672,#4104,.T.);
#45876=EDGE_CURVE('',#36671,#36667,#32940,.T.);
#45877=EDGE_CURVE('',#36672,#36668,#32941,.T.);
#45878=EDGE_CURVE('',#36673,#36674,#4105,.T.);
#45879=EDGE_CURVE('',#36673,#36671,#32942,.T.);
#45880=EDGE_CURVE('',#36674,#36672,#32943,.T.);
#45881=EDGE_CURVE('',#36669,#36673,#32944,.T.);
#45882=EDGE_CURVE('',#36670,#36674,#32945,.T.);
#45883=EDGE_CURVE('',#36675,#36676,#4106,.T.);
#45884=EDGE_CURVE('',#36675,#36677,#32946,.T.);
#45885=EDGE_CURVE('',#36677,#36678,#4107,.T.);
#45886=EDGE_CURVE('',#36676,#36678,#32947,.T.);
#45887=EDGE_CURVE('',#36679,#36680,#4108,.T.);
#45888=EDGE_CURVE('',#36679,#36675,#32948,.T.);
#45889=EDGE_CURVE('',#36680,#36676,#32949,.T.);
#45890=EDGE_CURVE('',#36681,#36682,#4109,.T.);
#45891=EDGE_CURVE('',#36681,#36679,#32950,.T.);
#45892=EDGE_CURVE('',#36682,#36680,#32951,.T.);
#45893=EDGE_CURVE('',#36677,#36681,#32952,.T.);
#45894=EDGE_CURVE('',#36678,#36682,#32953,.T.);
#45895=EDGE_CURVE('',#36683,#36684,#4110,.T.);
#45896=EDGE_CURVE('',#36683,#36685,#32954,.T.);
#45897=EDGE_CURVE('',#36685,#36686,#4111,.T.);
#45898=EDGE_CURVE('',#36684,#36686,#32955,.T.);
#45899=EDGE_CURVE('',#36687,#36688,#4112,.T.);
#45900=EDGE_CURVE('',#36687,#36683,#32956,.T.);
#45901=EDGE_CURVE('',#36688,#36684,#32957,.T.);
#45902=EDGE_CURVE('',#36689,#36690,#4113,.T.);
#45903=EDGE_CURVE('',#36689,#36687,#32958,.T.);
#45904=EDGE_CURVE('',#36690,#36688,#32959,.T.);
#45905=EDGE_CURVE('',#36685,#36689,#32960,.T.);
#45906=EDGE_CURVE('',#36686,#36690,#32961,.T.);
#45907=EDGE_CURVE('',#36691,#36692,#4114,.T.);
#45908=EDGE_CURVE('',#36691,#36693,#32962,.T.);
#45909=EDGE_CURVE('',#36693,#36694,#4115,.T.);
#45910=EDGE_CURVE('',#36692,#36694,#32963,.T.);
#45911=EDGE_CURVE('',#36695,#36696,#4116,.T.);
#45912=EDGE_CURVE('',#36695,#36691,#32964,.T.);
#45913=EDGE_CURVE('',#36696,#36692,#32965,.T.);
#45914=EDGE_CURVE('',#36697,#36698,#4117,.T.);
#45915=EDGE_CURVE('',#36697,#36695,#32966,.T.);
#45916=EDGE_CURVE('',#36698,#36696,#32967,.T.);
#45917=EDGE_CURVE('',#36693,#36697,#32968,.T.);
#45918=EDGE_CURVE('',#36694,#36698,#32969,.T.);
#45919=EDGE_CURVE('',#36699,#36700,#4118,.T.);
#45920=EDGE_CURVE('',#36699,#36701,#32970,.T.);
#45921=EDGE_CURVE('',#36701,#36702,#4119,.T.);
#45922=EDGE_CURVE('',#36700,#36702,#32971,.T.);
#45923=EDGE_CURVE('',#36703,#36704,#4120,.T.);
#45924=EDGE_CURVE('',#36703,#36699,#32972,.T.);
#45925=EDGE_CURVE('',#36704,#36700,#32973,.T.);
#45926=EDGE_CURVE('',#36705,#36706,#4121,.T.);
#45927=EDGE_CURVE('',#36705,#36703,#32974,.T.);
#45928=EDGE_CURVE('',#36706,#36704,#32975,.T.);
#45929=EDGE_CURVE('',#36701,#36705,#32976,.T.);
#45930=EDGE_CURVE('',#36702,#36706,#32977,.T.);
#45931=EDGE_CURVE('',#36707,#36708,#4122,.T.);
#45932=EDGE_CURVE('',#36707,#36709,#32978,.T.);
#45933=EDGE_CURVE('',#36709,#36710,#4123,.T.);
#45934=EDGE_CURVE('',#36708,#36710,#32979,.T.);
#45935=EDGE_CURVE('',#36711,#36712,#4124,.T.);
#45936=EDGE_CURVE('',#36711,#36707,#32980,.T.);
#45937=EDGE_CURVE('',#36712,#36708,#32981,.T.);
#45938=EDGE_CURVE('',#36713,#36714,#4125,.T.);
#45939=EDGE_CURVE('',#36713,#36711,#32982,.T.);
#45940=EDGE_CURVE('',#36714,#36712,#32983,.T.);
#45941=EDGE_CURVE('',#36709,#36713,#32984,.T.);
#45942=EDGE_CURVE('',#36710,#36714,#32985,.T.);
#45943=EDGE_CURVE('',#36715,#36716,#4126,.T.);
#45944=EDGE_CURVE('',#36715,#36717,#32986,.T.);
#45945=EDGE_CURVE('',#36717,#36718,#4127,.T.);
#45946=EDGE_CURVE('',#36716,#36718,#32987,.T.);
#45947=EDGE_CURVE('',#36719,#36720,#4128,.T.);
#45948=EDGE_CURVE('',#36719,#36715,#32988,.T.);
#45949=EDGE_CURVE('',#36720,#36716,#32989,.T.);
#45950=EDGE_CURVE('',#36721,#36722,#4129,.T.);
#45951=EDGE_CURVE('',#36721,#36719,#32990,.T.);
#45952=EDGE_CURVE('',#36722,#36720,#32991,.T.);
#45953=EDGE_CURVE('',#36717,#36721,#32992,.T.);
#45954=EDGE_CURVE('',#36718,#36722,#32993,.T.);
#45955=EDGE_CURVE('',#36723,#36724,#4130,.T.);
#45956=EDGE_CURVE('',#36723,#36725,#32994,.T.);
#45957=EDGE_CURVE('',#36725,#36726,#4131,.T.);
#45958=EDGE_CURVE('',#36724,#36726,#32995,.T.);
#45959=EDGE_CURVE('',#36727,#36728,#4132,.T.);
#45960=EDGE_CURVE('',#36727,#36723,#32996,.T.);
#45961=EDGE_CURVE('',#36728,#36724,#32997,.T.);
#45962=EDGE_CURVE('',#36729,#36730,#4133,.T.);
#45963=EDGE_CURVE('',#36729,#36727,#32998,.T.);
#45964=EDGE_CURVE('',#36730,#36728,#32999,.T.);
#45965=EDGE_CURVE('',#36725,#36729,#33000,.T.);
#45966=EDGE_CURVE('',#36726,#36730,#33001,.T.);
#45967=EDGE_CURVE('',#36731,#36732,#4134,.T.);
#45968=EDGE_CURVE('',#36731,#36733,#33002,.T.);
#45969=EDGE_CURVE('',#36733,#36734,#4135,.T.);
#45970=EDGE_CURVE('',#36732,#36734,#33003,.T.);
#45971=EDGE_CURVE('',#36735,#36736,#4136,.T.);
#45972=EDGE_CURVE('',#36735,#36731,#33004,.T.);
#45973=EDGE_CURVE('',#36736,#36732,#33005,.T.);
#45974=EDGE_CURVE('',#36737,#36738,#4137,.T.);
#45975=EDGE_CURVE('',#36737,#36735,#33006,.T.);
#45976=EDGE_CURVE('',#36738,#36736,#33007,.T.);
#45977=EDGE_CURVE('',#36733,#36737,#33008,.T.);
#45978=EDGE_CURVE('',#36734,#36738,#33009,.T.);
#45979=EDGE_CURVE('',#36739,#36740,#4138,.T.);
#45980=EDGE_CURVE('',#36739,#36741,#33010,.T.);
#45981=EDGE_CURVE('',#36741,#36742,#4139,.T.);
#45982=EDGE_CURVE('',#36740,#36742,#33011,.T.);
#45983=EDGE_CURVE('',#36743,#36744,#4140,.T.);
#45984=EDGE_CURVE('',#36743,#36739,#33012,.T.);
#45985=EDGE_CURVE('',#36744,#36740,#33013,.T.);
#45986=EDGE_CURVE('',#36745,#36746,#4141,.T.);
#45987=EDGE_CURVE('',#36745,#36743,#33014,.T.);
#45988=EDGE_CURVE('',#36746,#36744,#33015,.T.);
#45989=EDGE_CURVE('',#36741,#36745,#33016,.T.);
#45990=EDGE_CURVE('',#36742,#36746,#33017,.T.);
#45991=EDGE_CURVE('',#36747,#36748,#4142,.T.);
#45992=EDGE_CURVE('',#36747,#36749,#33018,.T.);
#45993=EDGE_CURVE('',#36749,#36750,#4143,.T.);
#45994=EDGE_CURVE('',#36748,#36750,#33019,.T.);
#45995=EDGE_CURVE('',#36751,#36752,#4144,.T.);
#45996=EDGE_CURVE('',#36751,#36747,#33020,.T.);
#45997=EDGE_CURVE('',#36752,#36748,#33021,.T.);
#45998=EDGE_CURVE('',#36753,#36754,#4145,.T.);
#45999=EDGE_CURVE('',#36753,#36751,#33022,.T.);
#46000=EDGE_CURVE('',#36754,#36752,#33023,.T.);
#46001=EDGE_CURVE('',#36749,#36753,#33024,.T.);
#46002=EDGE_CURVE('',#36750,#36754,#33025,.T.);
#46003=EDGE_CURVE('',#36755,#36756,#4146,.T.);
#46004=EDGE_CURVE('',#36755,#36757,#33026,.T.);
#46005=EDGE_CURVE('',#36757,#36758,#4147,.T.);
#46006=EDGE_CURVE('',#36756,#36758,#33027,.T.);
#46007=EDGE_CURVE('',#36759,#36760,#4148,.T.);
#46008=EDGE_CURVE('',#36759,#36755,#33028,.T.);
#46009=EDGE_CURVE('',#36760,#36756,#33029,.T.);
#46010=EDGE_CURVE('',#36761,#36762,#4149,.T.);
#46011=EDGE_CURVE('',#36761,#36759,#33030,.T.);
#46012=EDGE_CURVE('',#36762,#36760,#33031,.T.);
#46013=EDGE_CURVE('',#36757,#36761,#33032,.T.);
#46014=EDGE_CURVE('',#36758,#36762,#33033,.T.);
#46015=EDGE_CURVE('',#36763,#36764,#4150,.T.);
#46016=EDGE_CURVE('',#36763,#36765,#33034,.T.);
#46017=EDGE_CURVE('',#36765,#36766,#4151,.T.);
#46018=EDGE_CURVE('',#36764,#36766,#33035,.T.);
#46019=EDGE_CURVE('',#36767,#36768,#4152,.T.);
#46020=EDGE_CURVE('',#36767,#36763,#33036,.T.);
#46021=EDGE_CURVE('',#36768,#36764,#33037,.T.);
#46022=EDGE_CURVE('',#36769,#36770,#4153,.T.);
#46023=EDGE_CURVE('',#36769,#36767,#33038,.T.);
#46024=EDGE_CURVE('',#36770,#36768,#33039,.T.);
#46025=EDGE_CURVE('',#36765,#36769,#33040,.T.);
#46026=EDGE_CURVE('',#36766,#36770,#33041,.T.);
#46027=EDGE_CURVE('',#36771,#36772,#4154,.T.);
#46028=EDGE_CURVE('',#36771,#36773,#33042,.T.);
#46029=EDGE_CURVE('',#36773,#36774,#4155,.T.);
#46030=EDGE_CURVE('',#36772,#36774,#33043,.T.);
#46031=EDGE_CURVE('',#36775,#36776,#4156,.T.);
#46032=EDGE_CURVE('',#36775,#36771,#33044,.T.);
#46033=EDGE_CURVE('',#36776,#36772,#33045,.T.);
#46034=EDGE_CURVE('',#36777,#36778,#4157,.T.);
#46035=EDGE_CURVE('',#36777,#36775,#33046,.T.);
#46036=EDGE_CURVE('',#36778,#36776,#33047,.T.);
#46037=EDGE_CURVE('',#36773,#36777,#33048,.T.);
#46038=EDGE_CURVE('',#36774,#36778,#33049,.T.);
#46039=EDGE_CURVE('',#36779,#36780,#4158,.T.);
#46040=EDGE_CURVE('',#36779,#36781,#33050,.T.);
#46041=EDGE_CURVE('',#36781,#36782,#4159,.T.);
#46042=EDGE_CURVE('',#36780,#36782,#33051,.T.);
#46043=EDGE_CURVE('',#36783,#36784,#4160,.T.);
#46044=EDGE_CURVE('',#36783,#36779,#33052,.T.);
#46045=EDGE_CURVE('',#36784,#36780,#33053,.T.);
#46046=EDGE_CURVE('',#36785,#36786,#4161,.T.);
#46047=EDGE_CURVE('',#36785,#36783,#33054,.T.);
#46048=EDGE_CURVE('',#36786,#36784,#33055,.T.);
#46049=EDGE_CURVE('',#36781,#36785,#33056,.T.);
#46050=EDGE_CURVE('',#36782,#36786,#33057,.T.);
#46051=EDGE_CURVE('',#36787,#36788,#4162,.T.);
#46052=EDGE_CURVE('',#36787,#36789,#33058,.T.);
#46053=EDGE_CURVE('',#36789,#36790,#4163,.T.);
#46054=EDGE_CURVE('',#36788,#36790,#33059,.T.);
#46055=EDGE_CURVE('',#36791,#36792,#4164,.T.);
#46056=EDGE_CURVE('',#36791,#36787,#33060,.T.);
#46057=EDGE_CURVE('',#36792,#36788,#33061,.T.);
#46058=EDGE_CURVE('',#36793,#36794,#4165,.T.);
#46059=EDGE_CURVE('',#36793,#36791,#33062,.T.);
#46060=EDGE_CURVE('',#36794,#36792,#33063,.T.);
#46061=EDGE_CURVE('',#36789,#36793,#33064,.T.);
#46062=EDGE_CURVE('',#36790,#36794,#33065,.T.);
#46063=EDGE_CURVE('',#36795,#36796,#4166,.T.);
#46064=EDGE_CURVE('',#36795,#36797,#33066,.T.);
#46065=EDGE_CURVE('',#36797,#36798,#4167,.T.);
#46066=EDGE_CURVE('',#36796,#36798,#33067,.T.);
#46067=EDGE_CURVE('',#36799,#36800,#4168,.T.);
#46068=EDGE_CURVE('',#36799,#36795,#33068,.T.);
#46069=EDGE_CURVE('',#36800,#36796,#33069,.T.);
#46070=EDGE_CURVE('',#36801,#36802,#4169,.T.);
#46071=EDGE_CURVE('',#36801,#36799,#33070,.T.);
#46072=EDGE_CURVE('',#36802,#36800,#33071,.T.);
#46073=EDGE_CURVE('',#36797,#36801,#33072,.T.);
#46074=EDGE_CURVE('',#36798,#36802,#33073,.T.);
#46075=EDGE_CURVE('',#36803,#36804,#4170,.T.);
#46076=EDGE_CURVE('',#36803,#36805,#33074,.T.);
#46077=EDGE_CURVE('',#36805,#36806,#4171,.T.);
#46078=EDGE_CURVE('',#36804,#36806,#33075,.T.);
#46079=EDGE_CURVE('',#36807,#36808,#4172,.T.);
#46080=EDGE_CURVE('',#36807,#36803,#33076,.T.);
#46081=EDGE_CURVE('',#36808,#36804,#33077,.T.);
#46082=EDGE_CURVE('',#36809,#36810,#4173,.T.);
#46083=EDGE_CURVE('',#36809,#36807,#33078,.T.);
#46084=EDGE_CURVE('',#36810,#36808,#33079,.T.);
#46085=EDGE_CURVE('',#36805,#36809,#33080,.T.);
#46086=EDGE_CURVE('',#36806,#36810,#33081,.T.);
#46087=EDGE_CURVE('',#36811,#36812,#4174,.T.);
#46088=EDGE_CURVE('',#36811,#36813,#33082,.T.);
#46089=EDGE_CURVE('',#36813,#36814,#4175,.T.);
#46090=EDGE_CURVE('',#36812,#36814,#33083,.T.);
#46091=EDGE_CURVE('',#36815,#36816,#4176,.T.);
#46092=EDGE_CURVE('',#36815,#36811,#33084,.T.);
#46093=EDGE_CURVE('',#36816,#36812,#33085,.T.);
#46094=EDGE_CURVE('',#36817,#36818,#4177,.T.);
#46095=EDGE_CURVE('',#36817,#36815,#33086,.T.);
#46096=EDGE_CURVE('',#36818,#36816,#33087,.T.);
#46097=EDGE_CURVE('',#36813,#36817,#33088,.T.);
#46098=EDGE_CURVE('',#36814,#36818,#33089,.T.);
#46099=EDGE_CURVE('',#36819,#36820,#4178,.T.);
#46100=EDGE_CURVE('',#36819,#36821,#33090,.T.);
#46101=EDGE_CURVE('',#36821,#36822,#4179,.T.);
#46102=EDGE_CURVE('',#36820,#36822,#33091,.T.);
#46103=EDGE_CURVE('',#36823,#36824,#4180,.T.);
#46104=EDGE_CURVE('',#36823,#36819,#33092,.T.);
#46105=EDGE_CURVE('',#36824,#36820,#33093,.T.);
#46106=EDGE_CURVE('',#36825,#36826,#4181,.T.);
#46107=EDGE_CURVE('',#36825,#36823,#33094,.T.);
#46108=EDGE_CURVE('',#36826,#36824,#33095,.T.);
#46109=EDGE_CURVE('',#36821,#36825,#33096,.T.);
#46110=EDGE_CURVE('',#36822,#36826,#33097,.T.);
#46111=EDGE_CURVE('',#36827,#36828,#4182,.T.);
#46112=EDGE_CURVE('',#36827,#36829,#33098,.T.);
#46113=EDGE_CURVE('',#36829,#36830,#4183,.T.);
#46114=EDGE_CURVE('',#36828,#36830,#33099,.T.);
#46115=EDGE_CURVE('',#36831,#36832,#4184,.T.);
#46116=EDGE_CURVE('',#36831,#36827,#33100,.T.);
#46117=EDGE_CURVE('',#36832,#36828,#33101,.T.);
#46118=EDGE_CURVE('',#36833,#36834,#4185,.T.);
#46119=EDGE_CURVE('',#36833,#36831,#33102,.T.);
#46120=EDGE_CURVE('',#36834,#36832,#33103,.T.);
#46121=EDGE_CURVE('',#36829,#36833,#33104,.T.);
#46122=EDGE_CURVE('',#36830,#36834,#33105,.T.);
#46123=EDGE_CURVE('',#36835,#36836,#4186,.T.);
#46124=EDGE_CURVE('',#36835,#36837,#33106,.T.);
#46125=EDGE_CURVE('',#36837,#36838,#4187,.T.);
#46126=EDGE_CURVE('',#36836,#36838,#33107,.T.);
#46127=EDGE_CURVE('',#36839,#36840,#4188,.T.);
#46128=EDGE_CURVE('',#36839,#36835,#33108,.T.);
#46129=EDGE_CURVE('',#36840,#36836,#33109,.T.);
#46130=EDGE_CURVE('',#36841,#36842,#4189,.T.);
#46131=EDGE_CURVE('',#36841,#36839,#33110,.T.);
#46132=EDGE_CURVE('',#36842,#36840,#33111,.T.);
#46133=EDGE_CURVE('',#36837,#36841,#33112,.T.);
#46134=EDGE_CURVE('',#36838,#36842,#33113,.T.);
#46135=EDGE_CURVE('',#36843,#36844,#4190,.T.);
#46136=EDGE_CURVE('',#36843,#36845,#33114,.T.);
#46137=EDGE_CURVE('',#36845,#36846,#4191,.T.);
#46138=EDGE_CURVE('',#36844,#36846,#33115,.T.);
#46139=EDGE_CURVE('',#36847,#36848,#4192,.T.);
#46140=EDGE_CURVE('',#36847,#36843,#33116,.T.);
#46141=EDGE_CURVE('',#36848,#36844,#33117,.T.);
#46142=EDGE_CURVE('',#36849,#36850,#4193,.T.);
#46143=EDGE_CURVE('',#36849,#36847,#33118,.T.);
#46144=EDGE_CURVE('',#36850,#36848,#33119,.T.);
#46145=EDGE_CURVE('',#36845,#36849,#33120,.T.);
#46146=EDGE_CURVE('',#36846,#36850,#33121,.T.);
#46147=EDGE_CURVE('',#36851,#36852,#4194,.T.);
#46148=EDGE_CURVE('',#36851,#36853,#33122,.T.);
#46149=EDGE_CURVE('',#36853,#36854,#4195,.T.);
#46150=EDGE_CURVE('',#36852,#36854,#33123,.T.);
#46151=EDGE_CURVE('',#36855,#36856,#4196,.T.);
#46152=EDGE_CURVE('',#36855,#36851,#33124,.T.);
#46153=EDGE_CURVE('',#36856,#36852,#33125,.T.);
#46154=EDGE_CURVE('',#36857,#36858,#4197,.T.);
#46155=EDGE_CURVE('',#36857,#36855,#33126,.T.);
#46156=EDGE_CURVE('',#36858,#36856,#33127,.T.);
#46157=EDGE_CURVE('',#36853,#36857,#33128,.T.);
#46158=EDGE_CURVE('',#36854,#36858,#33129,.T.);
#46159=EDGE_CURVE('',#36859,#36860,#4198,.T.);
#46160=EDGE_CURVE('',#36859,#36861,#33130,.T.);
#46161=EDGE_CURVE('',#36861,#36862,#4199,.T.);
#46162=EDGE_CURVE('',#36860,#36862,#33131,.T.);
#46163=EDGE_CURVE('',#36863,#36864,#4200,.T.);
#46164=EDGE_CURVE('',#36863,#36859,#33132,.T.);
#46165=EDGE_CURVE('',#36864,#36860,#33133,.T.);
#46166=EDGE_CURVE('',#36865,#36866,#4201,.T.);
#46167=EDGE_CURVE('',#36865,#36863,#33134,.T.);
#46168=EDGE_CURVE('',#36866,#36864,#33135,.T.);
#46169=EDGE_CURVE('',#36861,#36865,#33136,.T.);
#46170=EDGE_CURVE('',#36862,#36866,#33137,.T.);
#46171=EDGE_CURVE('',#36867,#36868,#4202,.T.);
#46172=EDGE_CURVE('',#36867,#36869,#33138,.T.);
#46173=EDGE_CURVE('',#36869,#36870,#4203,.T.);
#46174=EDGE_CURVE('',#36868,#36870,#33139,.T.);
#46175=EDGE_CURVE('',#36871,#36872,#4204,.T.);
#46176=EDGE_CURVE('',#36871,#36867,#33140,.T.);
#46177=EDGE_CURVE('',#36872,#36868,#33141,.T.);
#46178=EDGE_CURVE('',#36873,#36874,#4205,.T.);
#46179=EDGE_CURVE('',#36873,#36871,#33142,.T.);
#46180=EDGE_CURVE('',#36874,#36872,#33143,.T.);
#46181=EDGE_CURVE('',#36869,#36873,#33144,.T.);
#46182=EDGE_CURVE('',#36870,#36874,#33145,.T.);
#46183=EDGE_CURVE('',#36875,#36876,#4206,.T.);
#46184=EDGE_CURVE('',#36875,#36877,#33146,.T.);
#46185=EDGE_CURVE('',#36877,#36878,#4207,.T.);
#46186=EDGE_CURVE('',#36876,#36878,#33147,.T.);
#46187=EDGE_CURVE('',#36879,#36880,#4208,.T.);
#46188=EDGE_CURVE('',#36879,#36875,#33148,.T.);
#46189=EDGE_CURVE('',#36880,#36876,#33149,.T.);
#46190=EDGE_CURVE('',#36881,#36882,#4209,.T.);
#46191=EDGE_CURVE('',#36881,#36879,#33150,.T.);
#46192=EDGE_CURVE('',#36882,#36880,#33151,.T.);
#46193=EDGE_CURVE('',#36877,#36881,#33152,.T.);
#46194=EDGE_CURVE('',#36878,#36882,#33153,.T.);
#46195=EDGE_CURVE('',#36883,#36884,#4210,.T.);
#46196=EDGE_CURVE('',#36883,#36885,#33154,.T.);
#46197=EDGE_CURVE('',#36885,#36886,#4211,.T.);
#46198=EDGE_CURVE('',#36884,#36886,#33155,.T.);
#46199=EDGE_CURVE('',#36887,#36888,#4212,.T.);
#46200=EDGE_CURVE('',#36887,#36883,#33156,.T.);
#46201=EDGE_CURVE('',#36888,#36884,#33157,.T.);
#46202=EDGE_CURVE('',#36889,#36890,#4213,.T.);
#46203=EDGE_CURVE('',#36889,#36887,#33158,.T.);
#46204=EDGE_CURVE('',#36890,#36888,#33159,.T.);
#46205=EDGE_CURVE('',#36885,#36889,#33160,.T.);
#46206=EDGE_CURVE('',#36886,#36890,#33161,.T.);
#46207=EDGE_CURVE('',#36891,#36892,#4214,.T.);
#46208=EDGE_CURVE('',#36891,#36893,#33162,.T.);
#46209=EDGE_CURVE('',#36893,#36894,#4215,.T.);
#46210=EDGE_CURVE('',#36892,#36894,#33163,.T.);
#46211=EDGE_CURVE('',#36895,#36896,#4216,.T.);
#46212=EDGE_CURVE('',#36895,#36891,#33164,.T.);
#46213=EDGE_CURVE('',#36896,#36892,#33165,.T.);
#46214=EDGE_CURVE('',#36897,#36898,#4217,.T.);
#46215=EDGE_CURVE('',#36897,#36895,#33166,.T.);
#46216=EDGE_CURVE('',#36898,#36896,#33167,.T.);
#46217=EDGE_CURVE('',#36893,#36897,#33168,.T.);
#46218=EDGE_CURVE('',#36894,#36898,#33169,.T.);
#46219=EDGE_CURVE('',#36899,#36900,#4218,.T.);
#46220=EDGE_CURVE('',#36899,#36901,#33170,.T.);
#46221=EDGE_CURVE('',#36901,#36902,#4219,.T.);
#46222=EDGE_CURVE('',#36900,#36902,#33171,.T.);
#46223=EDGE_CURVE('',#36903,#36904,#4220,.T.);
#46224=EDGE_CURVE('',#36903,#36899,#33172,.T.);
#46225=EDGE_CURVE('',#36904,#36900,#33173,.T.);
#46226=EDGE_CURVE('',#36905,#36906,#4221,.T.);
#46227=EDGE_CURVE('',#36905,#36903,#33174,.T.);
#46228=EDGE_CURVE('',#36906,#36904,#33175,.T.);
#46229=EDGE_CURVE('',#36901,#36905,#33176,.T.);
#46230=EDGE_CURVE('',#36902,#36906,#33177,.T.);
#46231=EDGE_CURVE('',#36907,#36908,#4222,.T.);
#46232=EDGE_CURVE('',#36907,#36909,#33178,.T.);
#46233=EDGE_CURVE('',#36909,#36910,#4223,.T.);
#46234=EDGE_CURVE('',#36908,#36910,#33179,.T.);
#46235=EDGE_CURVE('',#36911,#36912,#4224,.T.);
#46236=EDGE_CURVE('',#36911,#36907,#33180,.T.);
#46237=EDGE_CURVE('',#36912,#36908,#33181,.T.);
#46238=EDGE_CURVE('',#36913,#36914,#4225,.T.);
#46239=EDGE_CURVE('',#36913,#36911,#33182,.T.);
#46240=EDGE_CURVE('',#36914,#36912,#33183,.T.);
#46241=EDGE_CURVE('',#36909,#36913,#33184,.T.);
#46242=EDGE_CURVE('',#36910,#36914,#33185,.T.);
#46243=EDGE_CURVE('',#36915,#36916,#4226,.T.);
#46244=EDGE_CURVE('',#36915,#36917,#33186,.T.);
#46245=EDGE_CURVE('',#36917,#36918,#4227,.T.);
#46246=EDGE_CURVE('',#36916,#36918,#33187,.T.);
#46247=EDGE_CURVE('',#36919,#36920,#4228,.T.);
#46248=EDGE_CURVE('',#36919,#36915,#33188,.T.);
#46249=EDGE_CURVE('',#36920,#36916,#33189,.T.);
#46250=EDGE_CURVE('',#36921,#36922,#4229,.T.);
#46251=EDGE_CURVE('',#36921,#36919,#33190,.T.);
#46252=EDGE_CURVE('',#36922,#36920,#33191,.T.);
#46253=EDGE_CURVE('',#36917,#36921,#33192,.T.);
#46254=EDGE_CURVE('',#36918,#36922,#33193,.T.);
#46255=EDGE_CURVE('',#36923,#36924,#4230,.T.);
#46256=EDGE_CURVE('',#36923,#36925,#33194,.T.);
#46257=EDGE_CURVE('',#36925,#36926,#4231,.T.);
#46258=EDGE_CURVE('',#36924,#36926,#33195,.T.);
#46259=EDGE_CURVE('',#36927,#36928,#4232,.T.);
#46260=EDGE_CURVE('',#36927,#36923,#33196,.T.);
#46261=EDGE_CURVE('',#36928,#36924,#33197,.T.);
#46262=EDGE_CURVE('',#36929,#36930,#4233,.T.);
#46263=EDGE_CURVE('',#36929,#36927,#33198,.T.);
#46264=EDGE_CURVE('',#36930,#36928,#33199,.T.);
#46265=EDGE_CURVE('',#36925,#36929,#33200,.T.);
#46266=EDGE_CURVE('',#36926,#36930,#33201,.T.);
#46267=EDGE_CURVE('',#36931,#36932,#4234,.T.);
#46268=EDGE_CURVE('',#36931,#36933,#33202,.T.);
#46269=EDGE_CURVE('',#36933,#36934,#4235,.T.);
#46270=EDGE_CURVE('',#36932,#36934,#33203,.T.);
#46271=EDGE_CURVE('',#36935,#36936,#4236,.T.);
#46272=EDGE_CURVE('',#36935,#36931,#33204,.T.);
#46273=EDGE_CURVE('',#36936,#36932,#33205,.T.);
#46274=EDGE_CURVE('',#36937,#36938,#4237,.T.);
#46275=EDGE_CURVE('',#36937,#36935,#33206,.T.);
#46276=EDGE_CURVE('',#36938,#36936,#33207,.T.);
#46277=EDGE_CURVE('',#36933,#36937,#33208,.T.);
#46278=EDGE_CURVE('',#36934,#36938,#33209,.T.);
#46279=EDGE_CURVE('',#36939,#36940,#4238,.T.);
#46280=EDGE_CURVE('',#36939,#36941,#33210,.T.);
#46281=EDGE_CURVE('',#36941,#36942,#4239,.T.);
#46282=EDGE_CURVE('',#36940,#36942,#33211,.T.);
#46283=EDGE_CURVE('',#36943,#36944,#4240,.T.);
#46284=EDGE_CURVE('',#36943,#36939,#33212,.T.);
#46285=EDGE_CURVE('',#36944,#36940,#33213,.T.);
#46286=EDGE_CURVE('',#36945,#36946,#4241,.T.);
#46287=EDGE_CURVE('',#36945,#36943,#33214,.T.);
#46288=EDGE_CURVE('',#36946,#36944,#33215,.T.);
#46289=EDGE_CURVE('',#36941,#36945,#33216,.T.);
#46290=EDGE_CURVE('',#36942,#36946,#33217,.T.);
#46291=EDGE_CURVE('',#36947,#36948,#4242,.T.);
#46292=EDGE_CURVE('',#36947,#36949,#33218,.T.);
#46293=EDGE_CURVE('',#36949,#36950,#4243,.T.);
#46294=EDGE_CURVE('',#36948,#36950,#33219,.T.);
#46295=EDGE_CURVE('',#36951,#36952,#4244,.T.);
#46296=EDGE_CURVE('',#36951,#36947,#33220,.T.);
#46297=EDGE_CURVE('',#36952,#36948,#33221,.T.);
#46298=EDGE_CURVE('',#36953,#36954,#4245,.T.);
#46299=EDGE_CURVE('',#36953,#36951,#33222,.T.);
#46300=EDGE_CURVE('',#36954,#36952,#33223,.T.);
#46301=EDGE_CURVE('',#36949,#36953,#33224,.T.);
#46302=EDGE_CURVE('',#36950,#36954,#33225,.T.);
#46303=EDGE_CURVE('',#36955,#36956,#4246,.T.);
#46304=EDGE_CURVE('',#36955,#36957,#33226,.T.);
#46305=EDGE_CURVE('',#36957,#36958,#4247,.T.);
#46306=EDGE_CURVE('',#36956,#36958,#33227,.T.);
#46307=EDGE_CURVE('',#36959,#36960,#4248,.T.);
#46308=EDGE_CURVE('',#36959,#36955,#33228,.T.);
#46309=EDGE_CURVE('',#36960,#36956,#33229,.T.);
#46310=EDGE_CURVE('',#36961,#36962,#4249,.T.);
#46311=EDGE_CURVE('',#36961,#36959,#33230,.T.);
#46312=EDGE_CURVE('',#36962,#36960,#33231,.T.);
#46313=EDGE_CURVE('',#36957,#36961,#33232,.T.);
#46314=EDGE_CURVE('',#36958,#36962,#33233,.T.);
#46315=EDGE_CURVE('',#36963,#36964,#4250,.T.);
#46316=EDGE_CURVE('',#36963,#36965,#33234,.T.);
#46317=EDGE_CURVE('',#36965,#36966,#4251,.T.);
#46318=EDGE_CURVE('',#36964,#36966,#33235,.T.);
#46319=EDGE_CURVE('',#36967,#36968,#4252,.T.);
#46320=EDGE_CURVE('',#36967,#36963,#33236,.T.);
#46321=EDGE_CURVE('',#36968,#36964,#33237,.T.);
#46322=EDGE_CURVE('',#36969,#36970,#4253,.T.);
#46323=EDGE_CURVE('',#36969,#36967,#33238,.T.);
#46324=EDGE_CURVE('',#36970,#36968,#33239,.T.);
#46325=EDGE_CURVE('',#36965,#36969,#33240,.T.);
#46326=EDGE_CURVE('',#36966,#36970,#33241,.T.);
#46327=EDGE_CURVE('',#36971,#36972,#4254,.T.);
#46328=EDGE_CURVE('',#36971,#36973,#33242,.T.);
#46329=EDGE_CURVE('',#36973,#36974,#4255,.T.);
#46330=EDGE_CURVE('',#36972,#36974,#33243,.T.);
#46331=EDGE_CURVE('',#36975,#36976,#4256,.T.);
#46332=EDGE_CURVE('',#36975,#36971,#33244,.T.);
#46333=EDGE_CURVE('',#36976,#36972,#33245,.T.);
#46334=EDGE_CURVE('',#36977,#36978,#4257,.T.);
#46335=EDGE_CURVE('',#36977,#36975,#33246,.T.);
#46336=EDGE_CURVE('',#36978,#36976,#33247,.T.);
#46337=EDGE_CURVE('',#36973,#36977,#33248,.T.);
#46338=EDGE_CURVE('',#36974,#36978,#33249,.T.);
#46339=EDGE_CURVE('',#36979,#36980,#4258,.T.);
#46340=EDGE_CURVE('',#36979,#36981,#33250,.T.);
#46341=EDGE_CURVE('',#36981,#36982,#4259,.T.);
#46342=EDGE_CURVE('',#36980,#36982,#33251,.T.);
#46343=EDGE_CURVE('',#36983,#36984,#4260,.T.);
#46344=EDGE_CURVE('',#36983,#36979,#33252,.T.);
#46345=EDGE_CURVE('',#36984,#36980,#33253,.T.);
#46346=EDGE_CURVE('',#36985,#36986,#4261,.T.);
#46347=EDGE_CURVE('',#36985,#36983,#33254,.T.);
#46348=EDGE_CURVE('',#36986,#36984,#33255,.T.);
#46349=EDGE_CURVE('',#36981,#36985,#33256,.T.);
#46350=EDGE_CURVE('',#36982,#36986,#33257,.T.);
#46351=EDGE_CURVE('',#36987,#36988,#4262,.T.);
#46352=EDGE_CURVE('',#36987,#36989,#33258,.T.);
#46353=EDGE_CURVE('',#36989,#36990,#4263,.T.);
#46354=EDGE_CURVE('',#36988,#36990,#33259,.T.);
#46355=EDGE_CURVE('',#36991,#36992,#4264,.T.);
#46356=EDGE_CURVE('',#36991,#36987,#33260,.T.);
#46357=EDGE_CURVE('',#36992,#36988,#33261,.T.);
#46358=EDGE_CURVE('',#36993,#36994,#4265,.T.);
#46359=EDGE_CURVE('',#36993,#36991,#33262,.T.);
#46360=EDGE_CURVE('',#36994,#36992,#33263,.T.);
#46361=EDGE_CURVE('',#36989,#36993,#33264,.T.);
#46362=EDGE_CURVE('',#36990,#36994,#33265,.T.);
#46363=EDGE_CURVE('',#36995,#36996,#4266,.T.);
#46364=EDGE_CURVE('',#36995,#36997,#33266,.T.);
#46365=EDGE_CURVE('',#36997,#36998,#4267,.T.);
#46366=EDGE_CURVE('',#36996,#36998,#33267,.T.);
#46367=EDGE_CURVE('',#36999,#37000,#4268,.T.);
#46368=EDGE_CURVE('',#36999,#36995,#33268,.T.);
#46369=EDGE_CURVE('',#37000,#36996,#33269,.T.);
#46370=EDGE_CURVE('',#37001,#37002,#4269,.T.);
#46371=EDGE_CURVE('',#37001,#36999,#33270,.T.);
#46372=EDGE_CURVE('',#37002,#37000,#33271,.T.);
#46373=EDGE_CURVE('',#36997,#37001,#33272,.T.);
#46374=EDGE_CURVE('',#36998,#37002,#33273,.T.);
#46375=EDGE_CURVE('',#37003,#37004,#4270,.T.);
#46376=EDGE_CURVE('',#37003,#37005,#33274,.T.);
#46377=EDGE_CURVE('',#37005,#37006,#4271,.T.);
#46378=EDGE_CURVE('',#37004,#37006,#33275,.T.);
#46379=EDGE_CURVE('',#37007,#37008,#4272,.T.);
#46380=EDGE_CURVE('',#37007,#37003,#33276,.T.);
#46381=EDGE_CURVE('',#37008,#37004,#33277,.T.);
#46382=EDGE_CURVE('',#37009,#37010,#4273,.T.);
#46383=EDGE_CURVE('',#37009,#37007,#33278,.T.);
#46384=EDGE_CURVE('',#37010,#37008,#33279,.T.);
#46385=EDGE_CURVE('',#37005,#37009,#33280,.T.);
#46386=EDGE_CURVE('',#37006,#37010,#33281,.T.);
#46387=EDGE_CURVE('',#37011,#37012,#4274,.T.);
#46388=EDGE_CURVE('',#37011,#37013,#33282,.T.);
#46389=EDGE_CURVE('',#37013,#37014,#4275,.T.);
#46390=EDGE_CURVE('',#37012,#37014,#33283,.T.);
#46391=EDGE_CURVE('',#37015,#37016,#4276,.T.);
#46392=EDGE_CURVE('',#37015,#37011,#33284,.T.);
#46393=EDGE_CURVE('',#37016,#37012,#33285,.T.);
#46394=EDGE_CURVE('',#37017,#37018,#4277,.T.);
#46395=EDGE_CURVE('',#37017,#37015,#33286,.T.);
#46396=EDGE_CURVE('',#37018,#37016,#33287,.T.);
#46397=EDGE_CURVE('',#37013,#37017,#33288,.T.);
#46398=EDGE_CURVE('',#37014,#37018,#33289,.T.);
#46399=EDGE_CURVE('',#37019,#37020,#4278,.T.);
#46400=EDGE_CURVE('',#37019,#37021,#33290,.T.);
#46401=EDGE_CURVE('',#37021,#37022,#4279,.T.);
#46402=EDGE_CURVE('',#37020,#37022,#33291,.T.);
#46403=EDGE_CURVE('',#37023,#37024,#4280,.T.);
#46404=EDGE_CURVE('',#37023,#37019,#33292,.T.);
#46405=EDGE_CURVE('',#37024,#37020,#33293,.T.);
#46406=EDGE_CURVE('',#37025,#37026,#4281,.T.);
#46407=EDGE_CURVE('',#37025,#37023,#33294,.T.);
#46408=EDGE_CURVE('',#37026,#37024,#33295,.T.);
#46409=EDGE_CURVE('',#37021,#37025,#33296,.T.);
#46410=EDGE_CURVE('',#37022,#37026,#33297,.T.);
#46411=EDGE_CURVE('',#37027,#37028,#4282,.T.);
#46412=EDGE_CURVE('',#37027,#37029,#33298,.T.);
#46413=EDGE_CURVE('',#37029,#37030,#4283,.T.);
#46414=EDGE_CURVE('',#37028,#37030,#33299,.T.);
#46415=EDGE_CURVE('',#37031,#37032,#4284,.T.);
#46416=EDGE_CURVE('',#37031,#37027,#33300,.T.);
#46417=EDGE_CURVE('',#37032,#37028,#33301,.T.);
#46418=EDGE_CURVE('',#37033,#37034,#4285,.T.);
#46419=EDGE_CURVE('',#37033,#37031,#33302,.T.);
#46420=EDGE_CURVE('',#37034,#37032,#33303,.T.);
#46421=EDGE_CURVE('',#37029,#37033,#33304,.T.);
#46422=EDGE_CURVE('',#37030,#37034,#33305,.T.);
#46423=EDGE_CURVE('',#37035,#37036,#4286,.T.);
#46424=EDGE_CURVE('',#37035,#37037,#33306,.T.);
#46425=EDGE_CURVE('',#37037,#37038,#4287,.T.);
#46426=EDGE_CURVE('',#37036,#37038,#33307,.T.);
#46427=EDGE_CURVE('',#37039,#37040,#4288,.T.);
#46428=EDGE_CURVE('',#37039,#37035,#33308,.T.);
#46429=EDGE_CURVE('',#37040,#37036,#33309,.T.);
#46430=EDGE_CURVE('',#37041,#37042,#4289,.T.);
#46431=EDGE_CURVE('',#37041,#37039,#33310,.T.);
#46432=EDGE_CURVE('',#37042,#37040,#33311,.T.);
#46433=EDGE_CURVE('',#37037,#37041,#33312,.T.);
#46434=EDGE_CURVE('',#37038,#37042,#33313,.T.);
#46435=EDGE_CURVE('',#37043,#37044,#4290,.T.);
#46436=EDGE_CURVE('',#37043,#37045,#33314,.T.);
#46437=EDGE_CURVE('',#37045,#37046,#4291,.T.);
#46438=EDGE_CURVE('',#37044,#37046,#33315,.T.);
#46439=EDGE_CURVE('',#37047,#37048,#4292,.T.);
#46440=EDGE_CURVE('',#37047,#37043,#33316,.T.);
#46441=EDGE_CURVE('',#37048,#37044,#33317,.T.);
#46442=EDGE_CURVE('',#37049,#37050,#4293,.T.);
#46443=EDGE_CURVE('',#37049,#37047,#33318,.T.);
#46444=EDGE_CURVE('',#37050,#37048,#33319,.T.);
#46445=EDGE_CURVE('',#37045,#37049,#33320,.T.);
#46446=EDGE_CURVE('',#37046,#37050,#33321,.T.);
#46447=EDGE_CURVE('',#37051,#37052,#4294,.T.);
#46448=EDGE_CURVE('',#37051,#37053,#33322,.T.);
#46449=EDGE_CURVE('',#37053,#37054,#4295,.T.);
#46450=EDGE_CURVE('',#37052,#37054,#33323,.T.);
#46451=EDGE_CURVE('',#37055,#37056,#4296,.T.);
#46452=EDGE_CURVE('',#37055,#37051,#33324,.T.);
#46453=EDGE_CURVE('',#37056,#37052,#33325,.T.);
#46454=EDGE_CURVE('',#37057,#37058,#4297,.T.);
#46455=EDGE_CURVE('',#37057,#37055,#33326,.T.);
#46456=EDGE_CURVE('',#37058,#37056,#33327,.T.);
#46457=EDGE_CURVE('',#37053,#37057,#33328,.T.);
#46458=EDGE_CURVE('',#37054,#37058,#33329,.T.);
#46459=EDGE_CURVE('',#37059,#37060,#4298,.T.);
#46460=EDGE_CURVE('',#37059,#37061,#33330,.T.);
#46461=EDGE_CURVE('',#37061,#37062,#4299,.T.);
#46462=EDGE_CURVE('',#37060,#37062,#33331,.T.);
#46463=EDGE_CURVE('',#37063,#37064,#4300,.T.);
#46464=EDGE_CURVE('',#37063,#37059,#33332,.T.);
#46465=EDGE_CURVE('',#37064,#37060,#33333,.T.);
#46466=EDGE_CURVE('',#37065,#37066,#4301,.T.);
#46467=EDGE_CURVE('',#37065,#37063,#33334,.T.);
#46468=EDGE_CURVE('',#37066,#37064,#33335,.T.);
#46469=EDGE_CURVE('',#37061,#37065,#33336,.T.);
#46470=EDGE_CURVE('',#37062,#37066,#33337,.T.);
#46471=EDGE_CURVE('',#37067,#37068,#4302,.T.);
#46472=EDGE_CURVE('',#37067,#37069,#33338,.T.);
#46473=EDGE_CURVE('',#37069,#37070,#4303,.T.);
#46474=EDGE_CURVE('',#37068,#37070,#33339,.T.);
#46475=EDGE_CURVE('',#37071,#37072,#4304,.T.);
#46476=EDGE_CURVE('',#37071,#37067,#33340,.T.);
#46477=EDGE_CURVE('',#37072,#37068,#33341,.T.);
#46478=EDGE_CURVE('',#37073,#37074,#4305,.T.);
#46479=EDGE_CURVE('',#37073,#37071,#33342,.T.);
#46480=EDGE_CURVE('',#37074,#37072,#33343,.T.);
#46481=EDGE_CURVE('',#37069,#37073,#33344,.T.);
#46482=EDGE_CURVE('',#37070,#37074,#33345,.T.);
#46483=EDGE_CURVE('',#37075,#37076,#4306,.T.);
#46484=EDGE_CURVE('',#37075,#37077,#33346,.T.);
#46485=EDGE_CURVE('',#37077,#37078,#4307,.T.);
#46486=EDGE_CURVE('',#37076,#37078,#33347,.T.);
#46487=EDGE_CURVE('',#37079,#37080,#4308,.T.);
#46488=EDGE_CURVE('',#37079,#37075,#33348,.T.);
#46489=EDGE_CURVE('',#37080,#37076,#33349,.T.);
#46490=EDGE_CURVE('',#37081,#37082,#4309,.T.);
#46491=EDGE_CURVE('',#37081,#37079,#33350,.T.);
#46492=EDGE_CURVE('',#37082,#37080,#33351,.T.);
#46493=EDGE_CURVE('',#37077,#37081,#33352,.T.);
#46494=EDGE_CURVE('',#37078,#37082,#33353,.T.);
#46495=EDGE_CURVE('',#37083,#37084,#4310,.T.);
#46496=EDGE_CURVE('',#37083,#37085,#33354,.T.);
#46497=EDGE_CURVE('',#37085,#37086,#4311,.T.);
#46498=EDGE_CURVE('',#37084,#37086,#33355,.T.);
#46499=EDGE_CURVE('',#37087,#37088,#4312,.T.);
#46500=EDGE_CURVE('',#37087,#37083,#33356,.T.);
#46501=EDGE_CURVE('',#37088,#37084,#33357,.T.);
#46502=EDGE_CURVE('',#37089,#37090,#4313,.T.);
#46503=EDGE_CURVE('',#37089,#37087,#33358,.T.);
#46504=EDGE_CURVE('',#37090,#37088,#33359,.T.);
#46505=EDGE_CURVE('',#37085,#37089,#33360,.T.);
#46506=EDGE_CURVE('',#37086,#37090,#33361,.T.);
#46507=EDGE_CURVE('',#37091,#37092,#4314,.T.);
#46508=EDGE_CURVE('',#37091,#37093,#33362,.T.);
#46509=EDGE_CURVE('',#37093,#37094,#4315,.T.);
#46510=EDGE_CURVE('',#37092,#37094,#33363,.T.);
#46511=EDGE_CURVE('',#37095,#37096,#4316,.T.);
#46512=EDGE_CURVE('',#37095,#37091,#33364,.T.);
#46513=EDGE_CURVE('',#37096,#37092,#33365,.T.);
#46514=EDGE_CURVE('',#37097,#37098,#4317,.T.);
#46515=EDGE_CURVE('',#37097,#37095,#33366,.T.);
#46516=EDGE_CURVE('',#37098,#37096,#33367,.T.);
#46517=EDGE_CURVE('',#37093,#37097,#33368,.T.);
#46518=EDGE_CURVE('',#37094,#37098,#33369,.T.);
#46519=EDGE_CURVE('',#37099,#37100,#4318,.T.);
#46520=EDGE_CURVE('',#37099,#37101,#33370,.T.);
#46521=EDGE_CURVE('',#37101,#37102,#4319,.T.);
#46522=EDGE_CURVE('',#37100,#37102,#33371,.T.);
#46523=EDGE_CURVE('',#37103,#37104,#4320,.T.);
#46524=EDGE_CURVE('',#37103,#37099,#33372,.T.);
#46525=EDGE_CURVE('',#37104,#37100,#33373,.T.);
#46526=EDGE_CURVE('',#37105,#37106,#4321,.T.);
#46527=EDGE_CURVE('',#37105,#37103,#33374,.T.);
#46528=EDGE_CURVE('',#37106,#37104,#33375,.T.);
#46529=EDGE_CURVE('',#37101,#37105,#33376,.T.);
#46530=EDGE_CURVE('',#37102,#37106,#33377,.T.);
#46531=EDGE_CURVE('',#37107,#37108,#4322,.T.);
#46532=EDGE_CURVE('',#37107,#37109,#33378,.T.);
#46533=EDGE_CURVE('',#37109,#37110,#4323,.T.);
#46534=EDGE_CURVE('',#37108,#37110,#33379,.T.);
#46535=EDGE_CURVE('',#37111,#37112,#4324,.T.);
#46536=EDGE_CURVE('',#37111,#37107,#33380,.T.);
#46537=EDGE_CURVE('',#37112,#37108,#33381,.T.);
#46538=EDGE_CURVE('',#37113,#37114,#4325,.T.);
#46539=EDGE_CURVE('',#37113,#37111,#33382,.T.);
#46540=EDGE_CURVE('',#37114,#37112,#33383,.T.);
#46541=EDGE_CURVE('',#37109,#37113,#33384,.T.);
#46542=EDGE_CURVE('',#37110,#37114,#33385,.T.);
#46543=EDGE_CURVE('',#37115,#37116,#4326,.T.);
#46544=EDGE_CURVE('',#37115,#37117,#33386,.T.);
#46545=EDGE_CURVE('',#37117,#37118,#4327,.T.);
#46546=EDGE_CURVE('',#37116,#37118,#33387,.T.);
#46547=EDGE_CURVE('',#37119,#37120,#4328,.T.);
#46548=EDGE_CURVE('',#37119,#37115,#33388,.T.);
#46549=EDGE_CURVE('',#37120,#37116,#33389,.T.);
#46550=EDGE_CURVE('',#37121,#37122,#4329,.T.);
#46551=EDGE_CURVE('',#37121,#37119,#33390,.T.);
#46552=EDGE_CURVE('',#37122,#37120,#33391,.T.);
#46553=EDGE_CURVE('',#37117,#37121,#33392,.T.);
#46554=EDGE_CURVE('',#37118,#37122,#33393,.T.);
#46555=EDGE_CURVE('',#37123,#37124,#4330,.T.);
#46556=EDGE_CURVE('',#37123,#37125,#33394,.T.);
#46557=EDGE_CURVE('',#37125,#37126,#4331,.T.);
#46558=EDGE_CURVE('',#37124,#37126,#33395,.T.);
#46559=EDGE_CURVE('',#37127,#37128,#4332,.T.);
#46560=EDGE_CURVE('',#37127,#37123,#33396,.T.);
#46561=EDGE_CURVE('',#37128,#37124,#33397,.T.);
#46562=EDGE_CURVE('',#37129,#37130,#4333,.T.);
#46563=EDGE_CURVE('',#37129,#37127,#33398,.T.);
#46564=EDGE_CURVE('',#37130,#37128,#33399,.T.);
#46565=EDGE_CURVE('',#37125,#37129,#33400,.T.);
#46566=EDGE_CURVE('',#37126,#37130,#33401,.T.);
#46567=EDGE_CURVE('',#37131,#37132,#4334,.T.);
#46568=EDGE_CURVE('',#37131,#37133,#33402,.T.);
#46569=EDGE_CURVE('',#37133,#37134,#4335,.T.);
#46570=EDGE_CURVE('',#37132,#37134,#33403,.T.);
#46571=EDGE_CURVE('',#37135,#37136,#4336,.T.);
#46572=EDGE_CURVE('',#37135,#37131,#33404,.T.);
#46573=EDGE_CURVE('',#37136,#37132,#33405,.T.);
#46574=EDGE_CURVE('',#37137,#37138,#4337,.T.);
#46575=EDGE_CURVE('',#37137,#37135,#33406,.T.);
#46576=EDGE_CURVE('',#37138,#37136,#33407,.T.);
#46577=EDGE_CURVE('',#37133,#37137,#33408,.T.);
#46578=EDGE_CURVE('',#37134,#37138,#33409,.T.);
#46579=EDGE_CURVE('',#37139,#37140,#4338,.T.);
#46580=EDGE_CURVE('',#37139,#37141,#33410,.T.);
#46581=EDGE_CURVE('',#37141,#37142,#4339,.T.);
#46582=EDGE_CURVE('',#37140,#37142,#33411,.T.);
#46583=EDGE_CURVE('',#37143,#37144,#4340,.T.);
#46584=EDGE_CURVE('',#37143,#37139,#33412,.T.);
#46585=EDGE_CURVE('',#37144,#37140,#33413,.T.);
#46586=EDGE_CURVE('',#37145,#37146,#4341,.T.);
#46587=EDGE_CURVE('',#37145,#37143,#33414,.T.);
#46588=EDGE_CURVE('',#37146,#37144,#33415,.T.);
#46589=EDGE_CURVE('',#37141,#37145,#33416,.T.);
#46590=EDGE_CURVE('',#37142,#37146,#33417,.T.);
#46591=EDGE_CURVE('',#37147,#37148,#4342,.T.);
#46592=EDGE_CURVE('',#37147,#37149,#33418,.T.);
#46593=EDGE_CURVE('',#37149,#37150,#4343,.T.);
#46594=EDGE_CURVE('',#37148,#37150,#33419,.T.);
#46595=EDGE_CURVE('',#37151,#37152,#4344,.T.);
#46596=EDGE_CURVE('',#37151,#37147,#33420,.T.);
#46597=EDGE_CURVE('',#37152,#37148,#33421,.T.);
#46598=EDGE_CURVE('',#37153,#37154,#4345,.T.);
#46599=EDGE_CURVE('',#37153,#37151,#33422,.T.);
#46600=EDGE_CURVE('',#37154,#37152,#33423,.T.);
#46601=EDGE_CURVE('',#37149,#37153,#33424,.T.);
#46602=EDGE_CURVE('',#37150,#37154,#33425,.T.);
#46603=EDGE_CURVE('',#37155,#37156,#4346,.T.);
#46604=EDGE_CURVE('',#37155,#37157,#33426,.T.);
#46605=EDGE_CURVE('',#37157,#37158,#4347,.T.);
#46606=EDGE_CURVE('',#37156,#37158,#33427,.T.);
#46607=EDGE_CURVE('',#37159,#37160,#4348,.T.);
#46608=EDGE_CURVE('',#37159,#37155,#33428,.T.);
#46609=EDGE_CURVE('',#37160,#37156,#33429,.T.);
#46610=EDGE_CURVE('',#37161,#37162,#4349,.T.);
#46611=EDGE_CURVE('',#37161,#37159,#33430,.T.);
#46612=EDGE_CURVE('',#37162,#37160,#33431,.T.);
#46613=EDGE_CURVE('',#37157,#37161,#33432,.T.);
#46614=EDGE_CURVE('',#37158,#37162,#33433,.T.);
#46615=EDGE_CURVE('',#37163,#37164,#4350,.T.);
#46616=EDGE_CURVE('',#37163,#37165,#33434,.T.);
#46617=EDGE_CURVE('',#37165,#37166,#4351,.T.);
#46618=EDGE_CURVE('',#37164,#37166,#33435,.T.);
#46619=EDGE_CURVE('',#37167,#37168,#4352,.T.);
#46620=EDGE_CURVE('',#37167,#37163,#33436,.T.);
#46621=EDGE_CURVE('',#37168,#37164,#33437,.T.);
#46622=EDGE_CURVE('',#37169,#37170,#4353,.T.);
#46623=EDGE_CURVE('',#37169,#37167,#33438,.T.);
#46624=EDGE_CURVE('',#37170,#37168,#33439,.T.);
#46625=EDGE_CURVE('',#37165,#37169,#33440,.T.);
#46626=EDGE_CURVE('',#37166,#37170,#33441,.T.);
#46627=EDGE_CURVE('',#37171,#37172,#4354,.T.);
#46628=EDGE_CURVE('',#37171,#37173,#33442,.T.);
#46629=EDGE_CURVE('',#37173,#37174,#4355,.T.);
#46630=EDGE_CURVE('',#37172,#37174,#33443,.T.);
#46631=EDGE_CURVE('',#37175,#37176,#4356,.T.);
#46632=EDGE_CURVE('',#37175,#37171,#33444,.T.);
#46633=EDGE_CURVE('',#37176,#37172,#33445,.T.);
#46634=EDGE_CURVE('',#37177,#37178,#4357,.T.);
#46635=EDGE_CURVE('',#37177,#37175,#33446,.T.);
#46636=EDGE_CURVE('',#37178,#37176,#33447,.T.);
#46637=EDGE_CURVE('',#37173,#37177,#33448,.T.);
#46638=EDGE_CURVE('',#37174,#37178,#33449,.T.);
#46639=EDGE_CURVE('',#37179,#37180,#4358,.T.);
#46640=EDGE_CURVE('',#37179,#37181,#33450,.T.);
#46641=EDGE_CURVE('',#37181,#37182,#4359,.T.);
#46642=EDGE_CURVE('',#37180,#37182,#33451,.T.);
#46643=EDGE_CURVE('',#37183,#37184,#4360,.T.);
#46644=EDGE_CURVE('',#37183,#37179,#33452,.T.);
#46645=EDGE_CURVE('',#37184,#37180,#33453,.T.);
#46646=EDGE_CURVE('',#37185,#37186,#4361,.T.);
#46647=EDGE_CURVE('',#37185,#37183,#33454,.T.);
#46648=EDGE_CURVE('',#37186,#37184,#33455,.T.);
#46649=EDGE_CURVE('',#37181,#37185,#33456,.T.);
#46650=EDGE_CURVE('',#37182,#37186,#33457,.T.);
#46651=EDGE_CURVE('',#37187,#37188,#4362,.T.);
#46652=EDGE_CURVE('',#37187,#37189,#33458,.T.);
#46653=EDGE_CURVE('',#37189,#37190,#4363,.T.);
#46654=EDGE_CURVE('',#37188,#37190,#33459,.T.);
#46655=EDGE_CURVE('',#37191,#37192,#4364,.T.);
#46656=EDGE_CURVE('',#37191,#37187,#33460,.T.);
#46657=EDGE_CURVE('',#37192,#37188,#33461,.T.);
#46658=EDGE_CURVE('',#37193,#37194,#4365,.T.);
#46659=EDGE_CURVE('',#37193,#37191,#33462,.T.);
#46660=EDGE_CURVE('',#37194,#37192,#33463,.T.);
#46661=EDGE_CURVE('',#37189,#37193,#33464,.T.);
#46662=EDGE_CURVE('',#37190,#37194,#33465,.T.);
#46663=EDGE_CURVE('',#37195,#37196,#4366,.T.);
#46664=EDGE_CURVE('',#37195,#37197,#33466,.T.);
#46665=EDGE_CURVE('',#37197,#37198,#4367,.T.);
#46666=EDGE_CURVE('',#37196,#37198,#33467,.T.);
#46667=EDGE_CURVE('',#37199,#37200,#4368,.T.);
#46668=EDGE_CURVE('',#37199,#37195,#33468,.T.);
#46669=EDGE_CURVE('',#37200,#37196,#33469,.T.);
#46670=EDGE_CURVE('',#37201,#37202,#4369,.T.);
#46671=EDGE_CURVE('',#37201,#37199,#33470,.T.);
#46672=EDGE_CURVE('',#37202,#37200,#33471,.T.);
#46673=EDGE_CURVE('',#37197,#37201,#33472,.T.);
#46674=EDGE_CURVE('',#37198,#37202,#33473,.T.);
#46675=EDGE_CURVE('',#37203,#37204,#4370,.T.);
#46676=EDGE_CURVE('',#37203,#37205,#33474,.T.);
#46677=EDGE_CURVE('',#37205,#37206,#4371,.T.);
#46678=EDGE_CURVE('',#37204,#37206,#33475,.T.);
#46679=EDGE_CURVE('',#37207,#37208,#4372,.T.);
#46680=EDGE_CURVE('',#37207,#37203,#33476,.T.);
#46681=EDGE_CURVE('',#37208,#37204,#33477,.T.);
#46682=EDGE_CURVE('',#37209,#37210,#4373,.T.);
#46683=EDGE_CURVE('',#37209,#37207,#33478,.T.);
#46684=EDGE_CURVE('',#37210,#37208,#33479,.T.);
#46685=EDGE_CURVE('',#37205,#37209,#33480,.T.);
#46686=EDGE_CURVE('',#37206,#37210,#33481,.T.);
#46687=EDGE_CURVE('',#37211,#37212,#4374,.T.);
#46688=EDGE_CURVE('',#37211,#37213,#33482,.T.);
#46689=EDGE_CURVE('',#37213,#37214,#4375,.T.);
#46690=EDGE_CURVE('',#37212,#37214,#33483,.T.);
#46691=EDGE_CURVE('',#37215,#37216,#4376,.T.);
#46692=EDGE_CURVE('',#37215,#37211,#33484,.T.);
#46693=EDGE_CURVE('',#37216,#37212,#33485,.T.);
#46694=EDGE_CURVE('',#37217,#37218,#4377,.T.);
#46695=EDGE_CURVE('',#37217,#37215,#33486,.T.);
#46696=EDGE_CURVE('',#37218,#37216,#33487,.T.);
#46697=EDGE_CURVE('',#37213,#37217,#33488,.T.);
#46698=EDGE_CURVE('',#37214,#37218,#33489,.T.);
#46699=EDGE_CURVE('',#37219,#37220,#4378,.T.);
#46700=EDGE_CURVE('',#37219,#37221,#33490,.T.);
#46701=EDGE_CURVE('',#37221,#37222,#4379,.T.);
#46702=EDGE_CURVE('',#37220,#37222,#33491,.T.);
#46703=EDGE_CURVE('',#37223,#37224,#4380,.T.);
#46704=EDGE_CURVE('',#37223,#37219,#33492,.T.);
#46705=EDGE_CURVE('',#37224,#37220,#33493,.T.);
#46706=EDGE_CURVE('',#37225,#37226,#4381,.T.);
#46707=EDGE_CURVE('',#37225,#37223,#33494,.T.);
#46708=EDGE_CURVE('',#37226,#37224,#33495,.T.);
#46709=EDGE_CURVE('',#37221,#37225,#33496,.T.);
#46710=EDGE_CURVE('',#37222,#37226,#33497,.T.);
#46711=EDGE_CURVE('',#37227,#37228,#4382,.T.);
#46712=EDGE_CURVE('',#37227,#37229,#33498,.T.);
#46713=EDGE_CURVE('',#37229,#37230,#4383,.T.);
#46714=EDGE_CURVE('',#37228,#37230,#33499,.T.);
#46715=EDGE_CURVE('',#37231,#37232,#4384,.T.);
#46716=EDGE_CURVE('',#37231,#37227,#33500,.T.);
#46717=EDGE_CURVE('',#37232,#37228,#33501,.T.);
#46718=EDGE_CURVE('',#37233,#37234,#4385,.T.);
#46719=EDGE_CURVE('',#37233,#37231,#33502,.T.);
#46720=EDGE_CURVE('',#37234,#37232,#33503,.T.);
#46721=EDGE_CURVE('',#37229,#37233,#33504,.T.);
#46722=EDGE_CURVE('',#37230,#37234,#33505,.T.);
#46723=EDGE_CURVE('',#37235,#37236,#4386,.T.);
#46724=EDGE_CURVE('',#37235,#37237,#33506,.T.);
#46725=EDGE_CURVE('',#37237,#37238,#4387,.T.);
#46726=EDGE_CURVE('',#37236,#37238,#33507,.T.);
#46727=EDGE_CURVE('',#37239,#37240,#4388,.T.);
#46728=EDGE_CURVE('',#37239,#37235,#33508,.T.);
#46729=EDGE_CURVE('',#37240,#37236,#33509,.T.);
#46730=EDGE_CURVE('',#37241,#37242,#4389,.T.);
#46731=EDGE_CURVE('',#37241,#37239,#33510,.T.);
#46732=EDGE_CURVE('',#37242,#37240,#33511,.T.);
#46733=EDGE_CURVE('',#37237,#37241,#33512,.T.);
#46734=EDGE_CURVE('',#37238,#37242,#33513,.T.);
#46735=EDGE_CURVE('',#37243,#37244,#4390,.T.);
#46736=EDGE_CURVE('',#37245,#37244,#4391,.T.);
#46737=EDGE_CURVE('',#37246,#37245,#4392,.T.);
#46738=EDGE_CURVE('',#37246,#37243,#4393,.T.);
#46739=EDGE_CURVE('',#37247,#37248,#4394,.T.);
#46740=EDGE_CURVE('',#37244,#37248,#4395,.T.);
#46741=EDGE_CURVE('',#37243,#37247,#4396,.T.);
#46742=EDGE_CURVE('',#37249,#37250,#4397,.T.);
#46743=EDGE_CURVE('',#37248,#37250,#4398,.T.);
#46744=EDGE_CURVE('',#37247,#37249,#4399,.T.);
#46745=EDGE_CURVE('',#37250,#37245,#4400,.T.);
#46746=EDGE_CURVE('',#37249,#37246,#4401,.T.);
#46747=EDGE_CURVE('',#37251,#37252,#4402,.T.);
#46748=EDGE_CURVE('',#37253,#37252,#4403,.T.);
#46749=EDGE_CURVE('',#37254,#37253,#4404,.T.);
#46750=EDGE_CURVE('',#37254,#37251,#4405,.T.);
#46751=EDGE_CURVE('',#37255,#37256,#4406,.T.);
#46752=EDGE_CURVE('',#37252,#37256,#4407,.T.);
#46753=EDGE_CURVE('',#37251,#37255,#4408,.T.);
#46754=EDGE_CURVE('',#37257,#37258,#4409,.T.);
#46755=EDGE_CURVE('',#37256,#37258,#4410,.T.);
#46756=EDGE_CURVE('',#37255,#37257,#4411,.T.);
#46757=EDGE_CURVE('',#37258,#37253,#4412,.T.);
#46758=EDGE_CURVE('',#37257,#37254,#4413,.T.);
#46759=EDGE_CURVE('',#37259,#37260,#4414,.T.);
#46760=EDGE_CURVE('',#37261,#37260,#4415,.T.);
#46761=EDGE_CURVE('',#37262,#37261,#4416,.T.);
#46762=EDGE_CURVE('',#37262,#37259,#4417,.T.);
#46763=EDGE_CURVE('',#37263,#37264,#4418,.T.);
#46764=EDGE_CURVE('',#37260,#37264,#4419,.T.);
#46765=EDGE_CURVE('',#37259,#37263,#4420,.T.);
#46766=EDGE_CURVE('',#37265,#37266,#4421,.T.);
#46767=EDGE_CURVE('',#37264,#37266,#4422,.T.);
#46768=EDGE_CURVE('',#37263,#37265,#4423,.T.);
#46769=EDGE_CURVE('',#37266,#37261,#4424,.T.);
#46770=EDGE_CURVE('',#37265,#37262,#4425,.T.);
#46771=EDGE_CURVE('',#37267,#37268,#4426,.T.);
#46772=EDGE_CURVE('',#37269,#37268,#4427,.T.);
#46773=EDGE_CURVE('',#37270,#37269,#4428,.T.);
#46774=EDGE_CURVE('',#37270,#37267,#4429,.T.);
#46775=EDGE_CURVE('',#37271,#37272,#4430,.T.);
#46776=EDGE_CURVE('',#37268,#37272,#4431,.T.);
#46777=EDGE_CURVE('',#37267,#37271,#4432,.T.);
#46778=EDGE_CURVE('',#37273,#37274,#4433,.T.);
#46779=EDGE_CURVE('',#37272,#37274,#4434,.T.);
#46780=EDGE_CURVE('',#37271,#37273,#4435,.T.);
#46781=EDGE_CURVE('',#37274,#37269,#4436,.T.);
#46782=EDGE_CURVE('',#37273,#37270,#4437,.T.);
#46783=EDGE_CURVE('',#37275,#37276,#4438,.T.);
#46784=EDGE_CURVE('',#37277,#37276,#4439,.T.);
#46785=EDGE_CURVE('',#37278,#37277,#4440,.T.);
#46786=EDGE_CURVE('',#37278,#37275,#4441,.T.);
#46787=EDGE_CURVE('',#37279,#37280,#4442,.T.);
#46788=EDGE_CURVE('',#37276,#37280,#4443,.T.);
#46789=EDGE_CURVE('',#37275,#37279,#4444,.T.);
#46790=EDGE_CURVE('',#37281,#37282,#4445,.T.);
#46791=EDGE_CURVE('',#37280,#37282,#4446,.T.);
#46792=EDGE_CURVE('',#37279,#37281,#4447,.T.);
#46793=EDGE_CURVE('',#37282,#37277,#4448,.T.);
#46794=EDGE_CURVE('',#37281,#37278,#4449,.T.);
#46795=EDGE_CURVE('',#37283,#37284,#4450,.T.);
#46796=EDGE_CURVE('',#37285,#37284,#4451,.T.);
#46797=EDGE_CURVE('',#37286,#37285,#4452,.T.);
#46798=EDGE_CURVE('',#37286,#37283,#4453,.T.);
#46799=EDGE_CURVE('',#37287,#37288,#4454,.T.);
#46800=EDGE_CURVE('',#37284,#37288,#4455,.T.);
#46801=EDGE_CURVE('',#37283,#37287,#4456,.T.);
#46802=EDGE_CURVE('',#37289,#37290,#4457,.T.);
#46803=EDGE_CURVE('',#37288,#37290,#4458,.T.);
#46804=EDGE_CURVE('',#37287,#37289,#4459,.T.);
#46805=EDGE_CURVE('',#37290,#37285,#4460,.T.);
#46806=EDGE_CURVE('',#37289,#37286,#4461,.T.);
#46807=EDGE_CURVE('',#37291,#37292,#4462,.T.);
#46808=EDGE_CURVE('',#37293,#37292,#4463,.T.);
#46809=EDGE_CURVE('',#37294,#37293,#4464,.T.);
#46810=EDGE_CURVE('',#37294,#37291,#4465,.T.);
#46811=EDGE_CURVE('',#37295,#37296,#4466,.T.);
#46812=EDGE_CURVE('',#37292,#37296,#4467,.T.);
#46813=EDGE_CURVE('',#37291,#37295,#4468,.T.);
#46814=EDGE_CURVE('',#37297,#37298,#4469,.T.);
#46815=EDGE_CURVE('',#37296,#37298,#4470,.T.);
#46816=EDGE_CURVE('',#37295,#37297,#4471,.T.);
#46817=EDGE_CURVE('',#37298,#37293,#4472,.T.);
#46818=EDGE_CURVE('',#37297,#37294,#4473,.T.);
#46819=EDGE_CURVE('',#37299,#37300,#4474,.T.);
#46820=EDGE_CURVE('',#37301,#37300,#4475,.T.);
#46821=EDGE_CURVE('',#37302,#37301,#4476,.T.);
#46822=EDGE_CURVE('',#37302,#37299,#4477,.T.);
#46823=EDGE_CURVE('',#37303,#37304,#4478,.T.);
#46824=EDGE_CURVE('',#37300,#37304,#4479,.T.);
#46825=EDGE_CURVE('',#37299,#37303,#4480,.T.);
#46826=EDGE_CURVE('',#37305,#37306,#4481,.T.);
#46827=EDGE_CURVE('',#37304,#37306,#4482,.T.);
#46828=EDGE_CURVE('',#37303,#37305,#4483,.T.);
#46829=EDGE_CURVE('',#37306,#37301,#4484,.T.);
#46830=EDGE_CURVE('',#37305,#37302,#4485,.T.);
#46831=EDGE_CURVE('',#37307,#37308,#4486,.T.);
#46832=EDGE_CURVE('',#37309,#37308,#4487,.T.);
#46833=EDGE_CURVE('',#37310,#37309,#4488,.T.);
#46834=EDGE_CURVE('',#37310,#37307,#4489,.T.);
#46835=EDGE_CURVE('',#37311,#37312,#4490,.T.);
#46836=EDGE_CURVE('',#37308,#37312,#4491,.T.);
#46837=EDGE_CURVE('',#37307,#37311,#4492,.T.);
#46838=EDGE_CURVE('',#37313,#37314,#4493,.T.);
#46839=EDGE_CURVE('',#37312,#37314,#4494,.T.);
#46840=EDGE_CURVE('',#37311,#37313,#4495,.T.);
#46841=EDGE_CURVE('',#37314,#37309,#4496,.T.);
#46842=EDGE_CURVE('',#37313,#37310,#4497,.T.);
#46843=EDGE_CURVE('',#37315,#37316,#4498,.T.);
#46844=EDGE_CURVE('',#37317,#37316,#4499,.T.);
#46845=EDGE_CURVE('',#37318,#37317,#4500,.T.);
#46846=EDGE_CURVE('',#37318,#37315,#4501,.T.);
#46847=EDGE_CURVE('',#37319,#37320,#4502,.T.);
#46848=EDGE_CURVE('',#37316,#37320,#4503,.T.);
#46849=EDGE_CURVE('',#37315,#37319,#4504,.T.);
#46850=EDGE_CURVE('',#37321,#37322,#4505,.T.);
#46851=EDGE_CURVE('',#37320,#37322,#4506,.T.);
#46852=EDGE_CURVE('',#37319,#37321,#4507,.T.);
#46853=EDGE_CURVE('',#37322,#37317,#4508,.T.);
#46854=EDGE_CURVE('',#37321,#37318,#4509,.T.);
#46855=EDGE_CURVE('',#37323,#37324,#4510,.T.);
#46856=EDGE_CURVE('',#37325,#37324,#4511,.T.);
#46857=EDGE_CURVE('',#37326,#37325,#4512,.T.);
#46858=EDGE_CURVE('',#37326,#37323,#4513,.T.);
#46859=EDGE_CURVE('',#37327,#37328,#4514,.T.);
#46860=EDGE_CURVE('',#37324,#37328,#4515,.T.);
#46861=EDGE_CURVE('',#37323,#37327,#4516,.T.);
#46862=EDGE_CURVE('',#37329,#37330,#4517,.T.);
#46863=EDGE_CURVE('',#37328,#37330,#4518,.T.);
#46864=EDGE_CURVE('',#37327,#37329,#4519,.T.);
#46865=EDGE_CURVE('',#37330,#37325,#4520,.T.);
#46866=EDGE_CURVE('',#37329,#37326,#4521,.T.);
#46867=EDGE_CURVE('',#37331,#37332,#4522,.T.);
#46868=EDGE_CURVE('',#37333,#37332,#4523,.T.);
#46869=EDGE_CURVE('',#37334,#37333,#4524,.T.);
#46870=EDGE_CURVE('',#37334,#37331,#4525,.T.);
#46871=EDGE_CURVE('',#37335,#37336,#4526,.T.);
#46872=EDGE_CURVE('',#37332,#37336,#4527,.T.);
#46873=EDGE_CURVE('',#37331,#37335,#4528,.T.);
#46874=EDGE_CURVE('',#37337,#37338,#4529,.T.);
#46875=EDGE_CURVE('',#37336,#37338,#4530,.T.);
#46876=EDGE_CURVE('',#37335,#37337,#4531,.T.);
#46877=EDGE_CURVE('',#37338,#37333,#4532,.T.);
#46878=EDGE_CURVE('',#37337,#37334,#4533,.T.);
#46879=EDGE_CURVE('',#37339,#37340,#4534,.T.);
#46880=EDGE_CURVE('',#37341,#37340,#4535,.T.);
#46881=EDGE_CURVE('',#37342,#37341,#4536,.T.);
#46882=EDGE_CURVE('',#37342,#37339,#4537,.T.);
#46883=EDGE_CURVE('',#37343,#37344,#4538,.T.);
#46884=EDGE_CURVE('',#37340,#37344,#4539,.T.);
#46885=EDGE_CURVE('',#37339,#37343,#4540,.T.);
#46886=EDGE_CURVE('',#37345,#37346,#4541,.T.);
#46887=EDGE_CURVE('',#37344,#37346,#4542,.T.);
#46888=EDGE_CURVE('',#37343,#37345,#4543,.T.);
#46889=EDGE_CURVE('',#37346,#37341,#4544,.T.);
#46890=EDGE_CURVE('',#37345,#37342,#4545,.T.);
#46891=EDGE_CURVE('',#37347,#37348,#4546,.T.);
#46892=EDGE_CURVE('',#37349,#37348,#4547,.T.);
#46893=EDGE_CURVE('',#37350,#37349,#4548,.T.);
#46894=EDGE_CURVE('',#37350,#37347,#4549,.T.);
#46895=EDGE_CURVE('',#37351,#37352,#4550,.T.);
#46896=EDGE_CURVE('',#37348,#37352,#4551,.T.);
#46897=EDGE_CURVE('',#37347,#37351,#4552,.T.);
#46898=EDGE_CURVE('',#37353,#37354,#4553,.T.);
#46899=EDGE_CURVE('',#37352,#37354,#4554,.T.);
#46900=EDGE_CURVE('',#37351,#37353,#4555,.T.);
#46901=EDGE_CURVE('',#37354,#37349,#4556,.T.);
#46902=EDGE_CURVE('',#37353,#37350,#4557,.T.);
#46903=EDGE_CURVE('',#37355,#37356,#4558,.T.);
#46904=EDGE_CURVE('',#37357,#37356,#4559,.T.);
#46905=EDGE_CURVE('',#37358,#37357,#4560,.T.);
#46906=EDGE_CURVE('',#37358,#37355,#4561,.T.);
#46907=EDGE_CURVE('',#37359,#37360,#4562,.T.);
#46908=EDGE_CURVE('',#37356,#37360,#4563,.T.);
#46909=EDGE_CURVE('',#37355,#37359,#4564,.T.);
#46910=EDGE_CURVE('',#37361,#37362,#4565,.T.);
#46911=EDGE_CURVE('',#37360,#37362,#4566,.T.);
#46912=EDGE_CURVE('',#37359,#37361,#4567,.T.);
#46913=EDGE_CURVE('',#37362,#37357,#4568,.T.);
#46914=EDGE_CURVE('',#37361,#37358,#4569,.T.);
#46915=EDGE_CURVE('',#37363,#37364,#4570,.T.);
#46916=EDGE_CURVE('',#37365,#37364,#4571,.T.);
#46917=EDGE_CURVE('',#37366,#37365,#4572,.T.);
#46918=EDGE_CURVE('',#37366,#37363,#4573,.T.);
#46919=EDGE_CURVE('',#37367,#37368,#4574,.T.);
#46920=EDGE_CURVE('',#37364,#37368,#4575,.T.);
#46921=EDGE_CURVE('',#37363,#37367,#4576,.T.);
#46922=EDGE_CURVE('',#37369,#37370,#4577,.T.);
#46923=EDGE_CURVE('',#37368,#37370,#4578,.T.);
#46924=EDGE_CURVE('',#37367,#37369,#4579,.T.);
#46925=EDGE_CURVE('',#37370,#37365,#4580,.T.);
#46926=EDGE_CURVE('',#37369,#37366,#4581,.T.);
#46927=EDGE_CURVE('',#37371,#37372,#4582,.T.);
#46928=EDGE_CURVE('',#37373,#37372,#4583,.T.);
#46929=EDGE_CURVE('',#37374,#37373,#4584,.T.);
#46930=EDGE_CURVE('',#37374,#37371,#4585,.T.);
#46931=EDGE_CURVE('',#37375,#37376,#4586,.T.);
#46932=EDGE_CURVE('',#37372,#37376,#4587,.T.);
#46933=EDGE_CURVE('',#37371,#37375,#4588,.T.);
#46934=EDGE_CURVE('',#37377,#37378,#4589,.T.);
#46935=EDGE_CURVE('',#37376,#37378,#4590,.T.);
#46936=EDGE_CURVE('',#37375,#37377,#4591,.T.);
#46937=EDGE_CURVE('',#37378,#37373,#4592,.T.);
#46938=EDGE_CURVE('',#37377,#37374,#4593,.T.);
#46939=EDGE_CURVE('',#37379,#37380,#4594,.T.);
#46940=EDGE_CURVE('',#37381,#37380,#4595,.T.);
#46941=EDGE_CURVE('',#37382,#37381,#4596,.T.);
#46942=EDGE_CURVE('',#37382,#37379,#4597,.T.);
#46943=EDGE_CURVE('',#37383,#37384,#4598,.T.);
#46944=EDGE_CURVE('',#37380,#37384,#4599,.T.);
#46945=EDGE_CURVE('',#37379,#37383,#4600,.T.);
#46946=EDGE_CURVE('',#37385,#37386,#4601,.T.);
#46947=EDGE_CURVE('',#37384,#37386,#4602,.T.);
#46948=EDGE_CURVE('',#37383,#37385,#4603,.T.);
#46949=EDGE_CURVE('',#37386,#37381,#4604,.T.);
#46950=EDGE_CURVE('',#37385,#37382,#4605,.T.);
#46951=EDGE_CURVE('',#37387,#37388,#4606,.T.);
#46952=EDGE_CURVE('',#37389,#37388,#4607,.T.);
#46953=EDGE_CURVE('',#37390,#37389,#4608,.T.);
#46954=EDGE_CURVE('',#37390,#37387,#4609,.T.);
#46955=EDGE_CURVE('',#37391,#37392,#4610,.T.);
#46956=EDGE_CURVE('',#37388,#37392,#4611,.T.);
#46957=EDGE_CURVE('',#37387,#37391,#4612,.T.);
#46958=EDGE_CURVE('',#37393,#37394,#4613,.T.);
#46959=EDGE_CURVE('',#37392,#37394,#4614,.T.);
#46960=EDGE_CURVE('',#37391,#37393,#4615,.T.);
#46961=EDGE_CURVE('',#37394,#37389,#4616,.T.);
#46962=EDGE_CURVE('',#37393,#37390,#4617,.T.);
#46963=EDGE_CURVE('',#37395,#37396,#4618,.T.);
#46964=EDGE_CURVE('',#37397,#37396,#4619,.T.);
#46965=EDGE_CURVE('',#37398,#37397,#4620,.T.);
#46966=EDGE_CURVE('',#37398,#37395,#4621,.T.);
#46967=EDGE_CURVE('',#37399,#37400,#4622,.T.);
#46968=EDGE_CURVE('',#37396,#37400,#4623,.T.);
#46969=EDGE_CURVE('',#37395,#37399,#4624,.T.);
#46970=EDGE_CURVE('',#37401,#37402,#4625,.T.);
#46971=EDGE_CURVE('',#37400,#37402,#4626,.T.);
#46972=EDGE_CURVE('',#37399,#37401,#4627,.T.);
#46973=EDGE_CURVE('',#37402,#37397,#4628,.T.);
#46974=EDGE_CURVE('',#37401,#37398,#4629,.T.);
#46975=EDGE_CURVE('',#37403,#37404,#4630,.T.);
#46976=EDGE_CURVE('',#37405,#37404,#4631,.T.);
#46977=EDGE_CURVE('',#37406,#37405,#4632,.T.);
#46978=EDGE_CURVE('',#37406,#37403,#4633,.T.);
#46979=EDGE_CURVE('',#37407,#37408,#4634,.T.);
#46980=EDGE_CURVE('',#37404,#37408,#4635,.T.);
#46981=EDGE_CURVE('',#37403,#37407,#4636,.T.);
#46982=EDGE_CURVE('',#37409,#37410,#4637,.T.);
#46983=EDGE_CURVE('',#37408,#37410,#4638,.T.);
#46984=EDGE_CURVE('',#37407,#37409,#4639,.T.);
#46985=EDGE_CURVE('',#37410,#37405,#4640,.T.);
#46986=EDGE_CURVE('',#37409,#37406,#4641,.T.);
#46987=EDGE_CURVE('',#37411,#37412,#4642,.T.);
#46988=EDGE_CURVE('',#37413,#37412,#4643,.T.);
#46989=EDGE_CURVE('',#37414,#37413,#4644,.T.);
#46990=EDGE_CURVE('',#37414,#37411,#4645,.T.);
#46991=EDGE_CURVE('',#37415,#37416,#4646,.T.);
#46992=EDGE_CURVE('',#37412,#37416,#4647,.T.);
#46993=EDGE_CURVE('',#37411,#37415,#4648,.T.);
#46994=EDGE_CURVE('',#37417,#37418,#4649,.T.);
#46995=EDGE_CURVE('',#37416,#37418,#4650,.T.);
#46996=EDGE_CURVE('',#37415,#37417,#4651,.T.);
#46997=EDGE_CURVE('',#37418,#37413,#4652,.T.);
#46998=EDGE_CURVE('',#37417,#37414,#4653,.T.);
#46999=EDGE_CURVE('',#37419,#37420,#4654,.T.);
#47000=EDGE_CURVE('',#37421,#37420,#4655,.T.);
#47001=EDGE_CURVE('',#37422,#37421,#4656,.T.);
#47002=EDGE_CURVE('',#37422,#37419,#4657,.T.);
#47003=EDGE_CURVE('',#37423,#37424,#4658,.T.);
#47004=EDGE_CURVE('',#37420,#37424,#4659,.T.);
#47005=EDGE_CURVE('',#37419,#37423,#4660,.T.);
#47006=EDGE_CURVE('',#37425,#37426,#4661,.T.);
#47007=EDGE_CURVE('',#37424,#37426,#4662,.T.);
#47008=EDGE_CURVE('',#37423,#37425,#4663,.T.);
#47009=EDGE_CURVE('',#37426,#37421,#4664,.T.);
#47010=EDGE_CURVE('',#37425,#37422,#4665,.T.);
#47011=EDGE_CURVE('',#37427,#37428,#4666,.T.);
#47012=EDGE_CURVE('',#37429,#37428,#4667,.T.);
#47013=EDGE_CURVE('',#37430,#37429,#4668,.T.);
#47014=EDGE_CURVE('',#37430,#37427,#4669,.T.);
#47015=EDGE_CURVE('',#37431,#37432,#4670,.T.);
#47016=EDGE_CURVE('',#37428,#37432,#4671,.T.);
#47017=EDGE_CURVE('',#37427,#37431,#4672,.T.);
#47018=EDGE_CURVE('',#37433,#37434,#4673,.T.);
#47019=EDGE_CURVE('',#37432,#37434,#4674,.T.);
#47020=EDGE_CURVE('',#37431,#37433,#4675,.T.);
#47021=EDGE_CURVE('',#37434,#37429,#4676,.T.);
#47022=EDGE_CURVE('',#37433,#37430,#4677,.T.);
#47023=EDGE_CURVE('',#37435,#37436,#4678,.T.);
#47024=EDGE_CURVE('',#37437,#37436,#4679,.T.);
#47025=EDGE_CURVE('',#37438,#37437,#4680,.T.);
#47026=EDGE_CURVE('',#37438,#37435,#4681,.T.);
#47027=EDGE_CURVE('',#37439,#37440,#4682,.T.);
#47028=EDGE_CURVE('',#37436,#37440,#4683,.T.);
#47029=EDGE_CURVE('',#37435,#37439,#4684,.T.);
#47030=EDGE_CURVE('',#37441,#37442,#4685,.T.);
#47031=EDGE_CURVE('',#37440,#37442,#4686,.T.);
#47032=EDGE_CURVE('',#37439,#37441,#4687,.T.);
#47033=EDGE_CURVE('',#37442,#37437,#4688,.T.);
#47034=EDGE_CURVE('',#37441,#37438,#4689,.T.);
#47035=EDGE_CURVE('',#37443,#37444,#4690,.T.);
#47036=EDGE_CURVE('',#37445,#37444,#4691,.T.);
#47037=EDGE_CURVE('',#37446,#37445,#4692,.T.);
#47038=EDGE_CURVE('',#37446,#37443,#4693,.T.);
#47039=EDGE_CURVE('',#37447,#37448,#4694,.T.);
#47040=EDGE_CURVE('',#37444,#37448,#4695,.T.);
#47041=EDGE_CURVE('',#37443,#37447,#4696,.T.);
#47042=EDGE_CURVE('',#37449,#37450,#4697,.T.);
#47043=EDGE_CURVE('',#37448,#37450,#4698,.T.);
#47044=EDGE_CURVE('',#37447,#37449,#4699,.T.);
#47045=EDGE_CURVE('',#37450,#37445,#4700,.T.);
#47046=EDGE_CURVE('',#37449,#37446,#4701,.T.);
#47047=EDGE_CURVE('',#37451,#37452,#4702,.T.);
#47048=EDGE_CURVE('',#37453,#37452,#4703,.T.);
#47049=EDGE_CURVE('',#37454,#37453,#4704,.T.);
#47050=EDGE_CURVE('',#37454,#37451,#4705,.T.);
#47051=EDGE_CURVE('',#37455,#37456,#4706,.T.);
#47052=EDGE_CURVE('',#37452,#37456,#4707,.T.);
#47053=EDGE_CURVE('',#37451,#37455,#4708,.T.);
#47054=EDGE_CURVE('',#37457,#37458,#4709,.T.);
#47055=EDGE_CURVE('',#37456,#37458,#4710,.T.);
#47056=EDGE_CURVE('',#37455,#37457,#4711,.T.);
#47057=EDGE_CURVE('',#37458,#37453,#4712,.T.);
#47058=EDGE_CURVE('',#37457,#37454,#4713,.T.);
#47059=EDGE_CURVE('',#37459,#37460,#4714,.T.);
#47060=EDGE_CURVE('',#37461,#37460,#4715,.T.);
#47061=EDGE_CURVE('',#37462,#37461,#4716,.T.);
#47062=EDGE_CURVE('',#37462,#37459,#4717,.T.);
#47063=EDGE_CURVE('',#37463,#37464,#4718,.T.);
#47064=EDGE_CURVE('',#37460,#37464,#4719,.T.);
#47065=EDGE_CURVE('',#37459,#37463,#4720,.T.);
#47066=EDGE_CURVE('',#37465,#37466,#4721,.T.);
#47067=EDGE_CURVE('',#37464,#37466,#4722,.T.);
#47068=EDGE_CURVE('',#37463,#37465,#4723,.T.);
#47069=EDGE_CURVE('',#37466,#37461,#4724,.T.);
#47070=EDGE_CURVE('',#37465,#37462,#4725,.T.);
#47071=EDGE_CURVE('',#37467,#37468,#4726,.T.);
#47072=EDGE_CURVE('',#37469,#37468,#4727,.T.);
#47073=EDGE_CURVE('',#37470,#37469,#4728,.T.);
#47074=EDGE_CURVE('',#37470,#37467,#4729,.T.);
#47075=EDGE_CURVE('',#37471,#37472,#4730,.T.);
#47076=EDGE_CURVE('',#37468,#37472,#4731,.T.);
#47077=EDGE_CURVE('',#37467,#37471,#4732,.T.);
#47078=EDGE_CURVE('',#37473,#37474,#4733,.T.);
#47079=EDGE_CURVE('',#37472,#37474,#4734,.T.);
#47080=EDGE_CURVE('',#37471,#37473,#4735,.T.);
#47081=EDGE_CURVE('',#37474,#37469,#4736,.T.);
#47082=EDGE_CURVE('',#37473,#37470,#4737,.T.);
#47083=EDGE_CURVE('',#37475,#37476,#4738,.T.);
#47084=EDGE_CURVE('',#37477,#37476,#4739,.T.);
#47085=EDGE_CURVE('',#37478,#37477,#4740,.T.);
#47086=EDGE_CURVE('',#37478,#37475,#4741,.T.);
#47087=EDGE_CURVE('',#37479,#37480,#4742,.T.);
#47088=EDGE_CURVE('',#37476,#37480,#4743,.T.);
#47089=EDGE_CURVE('',#37475,#37479,#4744,.T.);
#47090=EDGE_CURVE('',#37481,#37482,#4745,.T.);
#47091=EDGE_CURVE('',#37480,#37482,#4746,.T.);
#47092=EDGE_CURVE('',#37479,#37481,#4747,.T.);
#47093=EDGE_CURVE('',#37482,#37477,#4748,.T.);
#47094=EDGE_CURVE('',#37481,#37478,#4749,.T.);
#47095=EDGE_CURVE('',#37483,#37484,#4750,.T.);
#47096=EDGE_CURVE('',#37485,#37484,#4751,.T.);
#47097=EDGE_CURVE('',#37486,#37485,#4752,.T.);
#47098=EDGE_CURVE('',#37486,#37483,#4753,.T.);
#47099=EDGE_CURVE('',#37487,#37488,#4754,.T.);
#47100=EDGE_CURVE('',#37484,#37488,#4755,.T.);
#47101=EDGE_CURVE('',#37483,#37487,#4756,.T.);
#47102=EDGE_CURVE('',#37489,#37490,#4757,.T.);
#47103=EDGE_CURVE('',#37488,#37490,#4758,.T.);
#47104=EDGE_CURVE('',#37487,#37489,#4759,.T.);
#47105=EDGE_CURVE('',#37490,#37485,#4760,.T.);
#47106=EDGE_CURVE('',#37489,#37486,#4761,.T.);
#47107=EDGE_CURVE('',#37491,#37492,#4762,.T.);
#47108=EDGE_CURVE('',#37493,#37492,#4763,.T.);
#47109=EDGE_CURVE('',#37494,#37493,#4764,.T.);
#47110=EDGE_CURVE('',#37494,#37491,#4765,.T.);
#47111=EDGE_CURVE('',#37495,#37496,#4766,.T.);
#47112=EDGE_CURVE('',#37492,#37496,#4767,.T.);
#47113=EDGE_CURVE('',#37491,#37495,#4768,.T.);
#47114=EDGE_CURVE('',#37497,#37498,#4769,.T.);
#47115=EDGE_CURVE('',#37496,#37498,#4770,.T.);
#47116=EDGE_CURVE('',#37495,#37497,#4771,.T.);
#47117=EDGE_CURVE('',#37498,#37493,#4772,.T.);
#47118=EDGE_CURVE('',#37497,#37494,#4773,.T.);
#47119=EDGE_CURVE('',#37499,#37500,#4774,.T.);
#47120=EDGE_CURVE('',#37501,#37500,#4775,.T.);
#47121=EDGE_CURVE('',#37502,#37501,#4776,.T.);
#47122=EDGE_CURVE('',#37502,#37499,#4777,.T.);
#47123=EDGE_CURVE('',#37503,#37504,#4778,.T.);
#47124=EDGE_CURVE('',#37500,#37504,#4779,.T.);
#47125=EDGE_CURVE('',#37499,#37503,#4780,.T.);
#47126=EDGE_CURVE('',#37505,#37506,#4781,.T.);
#47127=EDGE_CURVE('',#37504,#37506,#4782,.T.);
#47128=EDGE_CURVE('',#37503,#37505,#4783,.T.);
#47129=EDGE_CURVE('',#37506,#37501,#4784,.T.);
#47130=EDGE_CURVE('',#37505,#37502,#4785,.T.);
#47131=EDGE_CURVE('',#37507,#37508,#4786,.T.);
#47132=EDGE_CURVE('',#37509,#37508,#4787,.T.);
#47133=EDGE_CURVE('',#37510,#37509,#4788,.T.);
#47134=EDGE_CURVE('',#37510,#37507,#4789,.T.);
#47135=EDGE_CURVE('',#37511,#37512,#4790,.T.);
#47136=EDGE_CURVE('',#37508,#37512,#4791,.T.);
#47137=EDGE_CURVE('',#37507,#37511,#4792,.T.);
#47138=EDGE_CURVE('',#37513,#37514,#4793,.T.);
#47139=EDGE_CURVE('',#37512,#37514,#4794,.T.);
#47140=EDGE_CURVE('',#37511,#37513,#4795,.T.);
#47141=EDGE_CURVE('',#37514,#37509,#4796,.T.);
#47142=EDGE_CURVE('',#37513,#37510,#4797,.T.);
#47143=EDGE_CURVE('',#37515,#37516,#4798,.T.);
#47144=EDGE_CURVE('',#37517,#37516,#4799,.T.);
#47145=EDGE_CURVE('',#37518,#37517,#4800,.T.);
#47146=EDGE_CURVE('',#37518,#37515,#4801,.T.);
#47147=EDGE_CURVE('',#37519,#37520,#4802,.T.);
#47148=EDGE_CURVE('',#37516,#37520,#4803,.T.);
#47149=EDGE_CURVE('',#37515,#37519,#4804,.T.);
#47150=EDGE_CURVE('',#37521,#37522,#4805,.T.);
#47151=EDGE_CURVE('',#37520,#37522,#4806,.T.);
#47152=EDGE_CURVE('',#37519,#37521,#4807,.T.);
#47153=EDGE_CURVE('',#37522,#37517,#4808,.T.);
#47154=EDGE_CURVE('',#37521,#37518,#4809,.T.);
#47155=EDGE_CURVE('',#37523,#37524,#4810,.T.);
#47156=EDGE_CURVE('',#37525,#37524,#4811,.T.);
#47157=EDGE_CURVE('',#37526,#37525,#4812,.T.);
#47158=EDGE_CURVE('',#37526,#37523,#4813,.T.);
#47159=EDGE_CURVE('',#37527,#37528,#4814,.T.);
#47160=EDGE_CURVE('',#37524,#37528,#4815,.T.);
#47161=EDGE_CURVE('',#37523,#37527,#4816,.T.);
#47162=EDGE_CURVE('',#37529,#37530,#4817,.T.);
#47163=EDGE_CURVE('',#37528,#37530,#4818,.T.);
#47164=EDGE_CURVE('',#37527,#37529,#4819,.T.);
#47165=EDGE_CURVE('',#37530,#37525,#4820,.T.);
#47166=EDGE_CURVE('',#37529,#37526,#4821,.T.);
#47167=EDGE_CURVE('',#37531,#37532,#4822,.T.);
#47168=EDGE_CURVE('',#37533,#37532,#4823,.T.);
#47169=EDGE_CURVE('',#37534,#37533,#4824,.T.);
#47170=EDGE_CURVE('',#37534,#37531,#4825,.T.);
#47171=EDGE_CURVE('',#37535,#37536,#4826,.T.);
#47172=EDGE_CURVE('',#37532,#37536,#4827,.T.);
#47173=EDGE_CURVE('',#37531,#37535,#4828,.T.);
#47174=EDGE_CURVE('',#37537,#37538,#4829,.T.);
#47175=EDGE_CURVE('',#37536,#37538,#4830,.T.);
#47176=EDGE_CURVE('',#37535,#37537,#4831,.T.);
#47177=EDGE_CURVE('',#37538,#37533,#4832,.T.);
#47178=EDGE_CURVE('',#37537,#37534,#4833,.T.);
#47179=EDGE_CURVE('',#37539,#37540,#4834,.T.);
#47180=EDGE_CURVE('',#37541,#37540,#4835,.T.);
#47181=EDGE_CURVE('',#37542,#37541,#4836,.T.);
#47182=EDGE_CURVE('',#37542,#37539,#4837,.T.);
#47183=EDGE_CURVE('',#37543,#37544,#4838,.T.);
#47184=EDGE_CURVE('',#37540,#37544,#4839,.T.);
#47185=EDGE_CURVE('',#37539,#37543,#4840,.T.);
#47186=EDGE_CURVE('',#37545,#37546,#4841,.T.);
#47187=EDGE_CURVE('',#37544,#37546,#4842,.T.);
#47188=EDGE_CURVE('',#37543,#37545,#4843,.T.);
#47189=EDGE_CURVE('',#37546,#37541,#4844,.T.);
#47190=EDGE_CURVE('',#37545,#37542,#4845,.T.);
#47191=EDGE_CURVE('',#37547,#37548,#4846,.T.);
#47192=EDGE_CURVE('',#37549,#37548,#4847,.T.);
#47193=EDGE_CURVE('',#37550,#37549,#4848,.T.);
#47194=EDGE_CURVE('',#37550,#37547,#4849,.T.);
#47195=EDGE_CURVE('',#37551,#37552,#4850,.T.);
#47196=EDGE_CURVE('',#37548,#37552,#4851,.T.);
#47197=EDGE_CURVE('',#37547,#37551,#4852,.T.);
#47198=EDGE_CURVE('',#37553,#37554,#4853,.T.);
#47199=EDGE_CURVE('',#37552,#37554,#4854,.T.);
#47200=EDGE_CURVE('',#37551,#37553,#4855,.T.);
#47201=EDGE_CURVE('',#37554,#37549,#4856,.T.);
#47202=EDGE_CURVE('',#37553,#37550,#4857,.T.);
#47203=EDGE_CURVE('',#37555,#37556,#4858,.T.);
#47204=EDGE_CURVE('',#37557,#37556,#4859,.T.);
#47205=EDGE_CURVE('',#37558,#37557,#4860,.T.);
#47206=EDGE_CURVE('',#37558,#37555,#4861,.T.);
#47207=EDGE_CURVE('',#37559,#37560,#4862,.T.);
#47208=EDGE_CURVE('',#37556,#37560,#4863,.T.);
#47209=EDGE_CURVE('',#37555,#37559,#4864,.T.);
#47210=EDGE_CURVE('',#37561,#37562,#4865,.T.);
#47211=EDGE_CURVE('',#37560,#37562,#4866,.T.);
#47212=EDGE_CURVE('',#37559,#37561,#4867,.T.);
#47213=EDGE_CURVE('',#37562,#37557,#4868,.T.);
#47214=EDGE_CURVE('',#37561,#37558,#4869,.T.);
#47215=EDGE_CURVE('',#37563,#37564,#4870,.T.);
#47216=EDGE_CURVE('',#37565,#37564,#4871,.T.);
#47217=EDGE_CURVE('',#37566,#37565,#4872,.T.);
#47218=EDGE_CURVE('',#37566,#37563,#4873,.T.);
#47219=EDGE_CURVE('',#37567,#37568,#4874,.T.);
#47220=EDGE_CURVE('',#37564,#37568,#4875,.T.);
#47221=EDGE_CURVE('',#37563,#37567,#4876,.T.);
#47222=EDGE_CURVE('',#37569,#37570,#4877,.T.);
#47223=EDGE_CURVE('',#37568,#37570,#4878,.T.);
#47224=EDGE_CURVE('',#37567,#37569,#4879,.T.);
#47225=EDGE_CURVE('',#37570,#37565,#4880,.T.);
#47226=EDGE_CURVE('',#37569,#37566,#4881,.T.);
#47227=EDGE_CURVE('',#37571,#37572,#4882,.T.);
#47228=EDGE_CURVE('',#37573,#37572,#4883,.T.);
#47229=EDGE_CURVE('',#37574,#37573,#4884,.T.);
#47230=EDGE_CURVE('',#37574,#37571,#4885,.T.);
#47231=EDGE_CURVE('',#37575,#37576,#4886,.T.);
#47232=EDGE_CURVE('',#37572,#37576,#4887,.T.);
#47233=EDGE_CURVE('',#37571,#37575,#4888,.T.);
#47234=EDGE_CURVE('',#37577,#37578,#4889,.T.);
#47235=EDGE_CURVE('',#37576,#37578,#4890,.T.);
#47236=EDGE_CURVE('',#37575,#37577,#4891,.T.);
#47237=EDGE_CURVE('',#37578,#37573,#4892,.T.);
#47238=EDGE_CURVE('',#37577,#37574,#4893,.T.);
#47239=EDGE_CURVE('',#37579,#37580,#4894,.T.);
#47240=EDGE_CURVE('',#37581,#37580,#4895,.T.);
#47241=EDGE_CURVE('',#37582,#37581,#4896,.T.);
#47242=EDGE_CURVE('',#37582,#37579,#4897,.T.);
#47243=EDGE_CURVE('',#37583,#37584,#4898,.T.);
#47244=EDGE_CURVE('',#37580,#37584,#4899,.T.);
#47245=EDGE_CURVE('',#37579,#37583,#4900,.T.);
#47246=EDGE_CURVE('',#37585,#37586,#4901,.T.);
#47247=EDGE_CURVE('',#37584,#37586,#4902,.T.);
#47248=EDGE_CURVE('',#37583,#37585,#4903,.T.);
#47249=EDGE_CURVE('',#37586,#37581,#4904,.T.);
#47250=EDGE_CURVE('',#37585,#37582,#4905,.T.);
#47251=EDGE_CURVE('',#37587,#37588,#4906,.T.);
#47252=EDGE_CURVE('',#37589,#37588,#4907,.T.);
#47253=EDGE_CURVE('',#37590,#37589,#4908,.T.);
#47254=EDGE_CURVE('',#37590,#37587,#4909,.T.);
#47255=EDGE_CURVE('',#37591,#37592,#4910,.T.);
#47256=EDGE_CURVE('',#37588,#37592,#4911,.T.);
#47257=EDGE_CURVE('',#37587,#37591,#4912,.T.);
#47258=EDGE_CURVE('',#37593,#37594,#4913,.T.);
#47259=EDGE_CURVE('',#37592,#37594,#4914,.T.);
#47260=EDGE_CURVE('',#37591,#37593,#4915,.T.);
#47261=EDGE_CURVE('',#37594,#37589,#4916,.T.);
#47262=EDGE_CURVE('',#37593,#37590,#4917,.T.);
#47263=EDGE_CURVE('',#37595,#37596,#4918,.T.);
#47264=EDGE_CURVE('',#37597,#37596,#4919,.T.);
#47265=EDGE_CURVE('',#37598,#37597,#4920,.T.);
#47266=EDGE_CURVE('',#37598,#37595,#4921,.T.);
#47267=EDGE_CURVE('',#37599,#37600,#4922,.T.);
#47268=EDGE_CURVE('',#37596,#37600,#4923,.T.);
#47269=EDGE_CURVE('',#37595,#37599,#4924,.T.);
#47270=EDGE_CURVE('',#37601,#37602,#4925,.T.);
#47271=EDGE_CURVE('',#37600,#37602,#4926,.T.);
#47272=EDGE_CURVE('',#37599,#37601,#4927,.T.);
#47273=EDGE_CURVE('',#37602,#37597,#4928,.T.);
#47274=EDGE_CURVE('',#37601,#37598,#4929,.T.);
#47275=EDGE_CURVE('',#37603,#37604,#4930,.T.);
#47276=EDGE_CURVE('',#37605,#37604,#4931,.T.);
#47277=EDGE_CURVE('',#37606,#37605,#4932,.T.);
#47278=EDGE_CURVE('',#37606,#37603,#4933,.T.);
#47279=EDGE_CURVE('',#37607,#37608,#4934,.T.);
#47280=EDGE_CURVE('',#37604,#37608,#4935,.T.);
#47281=EDGE_CURVE('',#37603,#37607,#4936,.T.);
#47282=EDGE_CURVE('',#37609,#37610,#4937,.T.);
#47283=EDGE_CURVE('',#37608,#37610,#4938,.T.);
#47284=EDGE_CURVE('',#37607,#37609,#4939,.T.);
#47285=EDGE_CURVE('',#37610,#37605,#4940,.T.);
#47286=EDGE_CURVE('',#37609,#37606,#4941,.T.);
#47287=EDGE_CURVE('',#37611,#37612,#4942,.T.);
#47288=EDGE_CURVE('',#37613,#37612,#4943,.T.);
#47289=EDGE_CURVE('',#37614,#37613,#4944,.T.);
#47290=EDGE_CURVE('',#37614,#37611,#4945,.T.);
#47291=EDGE_CURVE('',#37615,#37616,#4946,.T.);
#47292=EDGE_CURVE('',#37612,#37616,#4947,.T.);
#47293=EDGE_CURVE('',#37611,#37615,#4948,.T.);
#47294=EDGE_CURVE('',#37617,#37618,#4949,.T.);
#47295=EDGE_CURVE('',#37616,#37618,#4950,.T.);
#47296=EDGE_CURVE('',#37615,#37617,#4951,.T.);
#47297=EDGE_CURVE('',#37618,#37613,#4952,.T.);
#47298=EDGE_CURVE('',#37617,#37614,#4953,.T.);
#47299=EDGE_CURVE('',#37619,#37620,#4954,.T.);
#47300=EDGE_CURVE('',#37621,#37620,#4955,.T.);
#47301=EDGE_CURVE('',#37622,#37621,#4956,.T.);
#47302=EDGE_CURVE('',#37622,#37619,#4957,.T.);
#47303=EDGE_CURVE('',#37623,#37624,#4958,.T.);
#47304=EDGE_CURVE('',#37620,#37624,#4959,.T.);
#47305=EDGE_CURVE('',#37619,#37623,#4960,.T.);
#47306=EDGE_CURVE('',#37625,#37626,#4961,.T.);
#47307=EDGE_CURVE('',#37624,#37626,#4962,.T.);
#47308=EDGE_CURVE('',#37623,#37625,#4963,.T.);
#47309=EDGE_CURVE('',#37626,#37621,#4964,.T.);
#47310=EDGE_CURVE('',#37625,#37622,#4965,.T.);
#47311=EDGE_CURVE('',#37627,#37628,#4966,.T.);
#47312=EDGE_CURVE('',#37629,#37628,#4967,.T.);
#47313=EDGE_CURVE('',#37630,#37629,#4968,.T.);
#47314=EDGE_CURVE('',#37630,#37627,#4969,.T.);
#47315=EDGE_CURVE('',#37631,#37632,#4970,.T.);
#47316=EDGE_CURVE('',#37628,#37632,#4971,.T.);
#47317=EDGE_CURVE('',#37627,#37631,#4972,.T.);
#47318=EDGE_CURVE('',#37633,#37634,#4973,.T.);
#47319=EDGE_CURVE('',#37632,#37634,#4974,.T.);
#47320=EDGE_CURVE('',#37631,#37633,#4975,.T.);
#47321=EDGE_CURVE('',#37634,#37629,#4976,.T.);
#47322=EDGE_CURVE('',#37633,#37630,#4977,.T.);
#47323=EDGE_CURVE('',#37635,#37636,#4978,.T.);
#47324=EDGE_CURVE('',#37637,#37636,#4979,.T.);
#47325=EDGE_CURVE('',#37638,#37637,#4980,.T.);
#47326=EDGE_CURVE('',#37638,#37635,#4981,.T.);
#47327=EDGE_CURVE('',#37639,#37640,#4982,.T.);
#47328=EDGE_CURVE('',#37636,#37640,#4983,.T.);
#47329=EDGE_CURVE('',#37635,#37639,#4984,.T.);
#47330=EDGE_CURVE('',#37641,#37642,#4985,.T.);
#47331=EDGE_CURVE('',#37640,#37642,#4986,.T.);
#47332=EDGE_CURVE('',#37639,#37641,#4987,.T.);
#47333=EDGE_CURVE('',#37642,#37637,#4988,.T.);
#47334=EDGE_CURVE('',#37641,#37638,#4989,.T.);
#47335=EDGE_CURVE('',#37643,#37644,#4990,.T.);
#47336=EDGE_CURVE('',#37645,#37644,#4991,.T.);
#47337=EDGE_CURVE('',#37646,#37645,#4992,.T.);
#47338=EDGE_CURVE('',#37646,#37643,#4993,.T.);
#47339=EDGE_CURVE('',#37647,#37648,#4994,.T.);
#47340=EDGE_CURVE('',#37644,#37648,#4995,.T.);
#47341=EDGE_CURVE('',#37643,#37647,#4996,.T.);
#47342=EDGE_CURVE('',#37649,#37650,#4997,.T.);
#47343=EDGE_CURVE('',#37648,#37650,#4998,.T.);
#47344=EDGE_CURVE('',#37647,#37649,#4999,.T.);
#47345=EDGE_CURVE('',#37650,#37645,#5000,.T.);
#47346=EDGE_CURVE('',#37649,#37646,#5001,.T.);
#47347=EDGE_CURVE('',#37651,#37652,#5002,.T.);
#47348=EDGE_CURVE('',#37653,#37652,#5003,.T.);
#47349=EDGE_CURVE('',#37654,#37653,#5004,.T.);
#47350=EDGE_CURVE('',#37654,#37651,#5005,.T.);
#47351=EDGE_CURVE('',#37655,#37656,#5006,.T.);
#47352=EDGE_CURVE('',#37652,#37656,#5007,.T.);
#47353=EDGE_CURVE('',#37651,#37655,#5008,.T.);
#47354=EDGE_CURVE('',#37657,#37658,#5009,.T.);
#47355=EDGE_CURVE('',#37656,#37658,#5010,.T.);
#47356=EDGE_CURVE('',#37655,#37657,#5011,.T.);
#47357=EDGE_CURVE('',#37658,#37653,#5012,.T.);
#47358=EDGE_CURVE('',#37657,#37654,#5013,.T.);
#47359=EDGE_CURVE('',#37659,#37660,#5014,.T.);
#47360=EDGE_CURVE('',#37661,#37660,#5015,.T.);
#47361=EDGE_CURVE('',#37662,#37661,#5016,.T.);
#47362=EDGE_CURVE('',#37662,#37659,#5017,.T.);
#47363=EDGE_CURVE('',#37663,#37664,#5018,.T.);
#47364=EDGE_CURVE('',#37660,#37664,#5019,.T.);
#47365=EDGE_CURVE('',#37659,#37663,#5020,.T.);
#47366=EDGE_CURVE('',#37665,#37666,#5021,.T.);
#47367=EDGE_CURVE('',#37664,#37666,#5022,.T.);
#47368=EDGE_CURVE('',#37663,#37665,#5023,.T.);
#47369=EDGE_CURVE('',#37666,#37661,#5024,.T.);
#47370=EDGE_CURVE('',#37665,#37662,#5025,.T.);
#47371=EDGE_CURVE('',#37667,#37668,#5026,.T.);
#47372=EDGE_CURVE('',#37669,#37668,#5027,.T.);
#47373=EDGE_CURVE('',#37670,#37669,#5028,.T.);
#47374=EDGE_CURVE('',#37670,#37667,#5029,.T.);
#47375=EDGE_CURVE('',#37671,#37672,#5030,.T.);
#47376=EDGE_CURVE('',#37668,#37672,#5031,.T.);
#47377=EDGE_CURVE('',#37667,#37671,#5032,.T.);
#47378=EDGE_CURVE('',#37673,#37674,#5033,.T.);
#47379=EDGE_CURVE('',#37672,#37674,#5034,.T.);
#47380=EDGE_CURVE('',#37671,#37673,#5035,.T.);
#47381=EDGE_CURVE('',#37674,#37669,#5036,.T.);
#47382=EDGE_CURVE('',#37673,#37670,#5037,.T.);
#47383=EDGE_CURVE('',#37675,#37676,#5038,.T.);
#47384=EDGE_CURVE('',#37677,#37676,#5039,.T.);
#47385=EDGE_CURVE('',#37678,#37677,#5040,.T.);
#47386=EDGE_CURVE('',#37678,#37675,#5041,.T.);
#47387=EDGE_CURVE('',#37679,#37680,#5042,.T.);
#47388=EDGE_CURVE('',#37676,#37680,#5043,.T.);
#47389=EDGE_CURVE('',#37675,#37679,#5044,.T.);
#47390=EDGE_CURVE('',#37681,#37682,#5045,.T.);
#47391=EDGE_CURVE('',#37680,#37682,#5046,.T.);
#47392=EDGE_CURVE('',#37679,#37681,#5047,.T.);
#47393=EDGE_CURVE('',#37682,#37677,#5048,.T.);
#47394=EDGE_CURVE('',#37681,#37678,#5049,.T.);
#47395=EDGE_CURVE('',#37683,#37684,#5050,.T.);
#47396=EDGE_CURVE('',#37685,#37684,#5051,.T.);
#47397=EDGE_CURVE('',#37686,#37685,#5052,.T.);
#47398=EDGE_CURVE('',#37686,#37683,#5053,.T.);
#47399=EDGE_CURVE('',#37687,#37688,#5054,.T.);
#47400=EDGE_CURVE('',#37684,#37688,#5055,.T.);
#47401=EDGE_CURVE('',#37683,#37687,#5056,.T.);
#47402=EDGE_CURVE('',#37689,#37690,#5057,.T.);
#47403=EDGE_CURVE('',#37688,#37690,#5058,.T.);
#47404=EDGE_CURVE('',#37687,#37689,#5059,.T.);
#47405=EDGE_CURVE('',#37690,#37685,#5060,.T.);
#47406=EDGE_CURVE('',#37689,#37686,#5061,.T.);
#47407=EDGE_CURVE('',#37691,#37692,#5062,.T.);
#47408=EDGE_CURVE('',#37693,#37692,#5063,.T.);
#47409=EDGE_CURVE('',#37694,#37693,#5064,.T.);
#47410=EDGE_CURVE('',#37694,#37691,#5065,.T.);
#47411=EDGE_CURVE('',#37695,#37696,#5066,.T.);
#47412=EDGE_CURVE('',#37692,#37696,#5067,.T.);
#47413=EDGE_CURVE('',#37691,#37695,#5068,.T.);
#47414=EDGE_CURVE('',#37697,#37698,#5069,.T.);
#47415=EDGE_CURVE('',#37696,#37698,#5070,.T.);
#47416=EDGE_CURVE('',#37695,#37697,#5071,.T.);
#47417=EDGE_CURVE('',#37698,#37693,#5072,.T.);
#47418=EDGE_CURVE('',#37697,#37694,#5073,.T.);
#47419=EDGE_CURVE('',#37699,#37700,#5074,.T.);
#47420=EDGE_CURVE('',#37701,#37700,#5075,.T.);
#47421=EDGE_CURVE('',#37702,#37701,#5076,.T.);
#47422=EDGE_CURVE('',#37702,#37699,#5077,.T.);
#47423=EDGE_CURVE('',#37703,#37704,#5078,.T.);
#47424=EDGE_CURVE('',#37700,#37704,#5079,.T.);
#47425=EDGE_CURVE('',#37699,#37703,#5080,.T.);
#47426=EDGE_CURVE('',#37705,#37706,#5081,.T.);
#47427=EDGE_CURVE('',#37704,#37706,#5082,.T.);
#47428=EDGE_CURVE('',#37703,#37705,#5083,.T.);
#47429=EDGE_CURVE('',#37706,#37701,#5084,.T.);
#47430=EDGE_CURVE('',#37705,#37702,#5085,.T.);
#47431=EDGE_CURVE('',#37707,#37708,#5086,.T.);
#47432=EDGE_CURVE('',#37709,#37708,#5087,.T.);
#47433=EDGE_CURVE('',#37710,#37709,#5088,.T.);
#47434=EDGE_CURVE('',#37710,#37707,#5089,.T.);
#47435=EDGE_CURVE('',#37711,#37712,#5090,.T.);
#47436=EDGE_CURVE('',#37708,#37712,#5091,.T.);
#47437=EDGE_CURVE('',#37707,#37711,#5092,.T.);
#47438=EDGE_CURVE('',#37713,#37714,#5093,.T.);
#47439=EDGE_CURVE('',#37712,#37714,#5094,.T.);
#47440=EDGE_CURVE('',#37711,#37713,#5095,.T.);
#47441=EDGE_CURVE('',#37714,#37709,#5096,.T.);
#47442=EDGE_CURVE('',#37713,#37710,#5097,.T.);
#47443=EDGE_CURVE('',#37715,#37716,#5098,.T.);
#47444=EDGE_CURVE('',#37717,#37716,#5099,.T.);
#47445=EDGE_CURVE('',#37718,#37717,#5100,.T.);
#47446=EDGE_CURVE('',#37718,#37715,#5101,.T.);
#47447=EDGE_CURVE('',#37719,#37720,#5102,.T.);
#47448=EDGE_CURVE('',#37716,#37720,#5103,.T.);
#47449=EDGE_CURVE('',#37715,#37719,#5104,.T.);
#47450=EDGE_CURVE('',#37721,#37722,#5105,.T.);
#47451=EDGE_CURVE('',#37720,#37722,#5106,.T.);
#47452=EDGE_CURVE('',#37719,#37721,#5107,.T.);
#47453=EDGE_CURVE('',#37722,#37717,#5108,.T.);
#47454=EDGE_CURVE('',#37721,#37718,#5109,.T.);
#47455=EDGE_CURVE('',#37723,#37724,#5110,.T.);
#47456=EDGE_CURVE('',#37725,#37724,#5111,.T.);
#47457=EDGE_CURVE('',#37726,#37725,#5112,.T.);
#47458=EDGE_CURVE('',#37726,#37723,#5113,.T.);
#47459=EDGE_CURVE('',#37727,#37728,#5114,.T.);
#47460=EDGE_CURVE('',#37724,#37728,#5115,.T.);
#47461=EDGE_CURVE('',#37723,#37727,#5116,.T.);
#47462=EDGE_CURVE('',#37729,#37730,#5117,.T.);
#47463=EDGE_CURVE('',#37728,#37730,#5118,.T.);
#47464=EDGE_CURVE('',#37727,#37729,#5119,.T.);
#47465=EDGE_CURVE('',#37730,#37725,#5120,.T.);
#47466=EDGE_CURVE('',#37729,#37726,#5121,.T.);
#47467=EDGE_CURVE('',#37731,#37732,#5122,.T.);
#47468=EDGE_CURVE('',#37733,#37732,#5123,.T.);
#47469=EDGE_CURVE('',#37734,#37733,#5124,.T.);
#47470=EDGE_CURVE('',#37734,#37731,#5125,.T.);
#47471=EDGE_CURVE('',#37735,#37736,#5126,.T.);
#47472=EDGE_CURVE('',#37732,#37736,#5127,.T.);
#47473=EDGE_CURVE('',#37731,#37735,#5128,.T.);
#47474=EDGE_CURVE('',#37737,#37738,#5129,.T.);
#47475=EDGE_CURVE('',#37736,#37738,#5130,.T.);
#47476=EDGE_CURVE('',#37735,#37737,#5131,.T.);
#47477=EDGE_CURVE('',#37738,#37733,#5132,.T.);
#47478=EDGE_CURVE('',#37737,#37734,#5133,.T.);
#47479=EDGE_CURVE('',#37739,#37740,#5134,.T.);
#47480=EDGE_CURVE('',#37741,#37740,#5135,.T.);
#47481=EDGE_CURVE('',#37742,#37741,#5136,.T.);
#47482=EDGE_CURVE('',#37742,#37739,#5137,.T.);
#47483=EDGE_CURVE('',#37743,#37744,#5138,.T.);
#47484=EDGE_CURVE('',#37740,#37744,#5139,.T.);
#47485=EDGE_CURVE('',#37739,#37743,#5140,.T.);
#47486=EDGE_CURVE('',#37745,#37746,#5141,.T.);
#47487=EDGE_CURVE('',#37744,#37746,#5142,.T.);
#47488=EDGE_CURVE('',#37743,#37745,#5143,.T.);
#47489=EDGE_CURVE('',#37746,#37741,#5144,.T.);
#47490=EDGE_CURVE('',#37745,#37742,#5145,.T.);
#47491=EDGE_CURVE('',#37747,#37748,#5146,.T.);
#47492=EDGE_CURVE('',#37749,#37748,#5147,.T.);
#47493=EDGE_CURVE('',#37750,#37749,#5148,.T.);
#47494=EDGE_CURVE('',#37750,#37747,#5149,.T.);
#47495=EDGE_CURVE('',#37751,#37752,#5150,.T.);
#47496=EDGE_CURVE('',#37748,#37752,#5151,.T.);
#47497=EDGE_CURVE('',#37747,#37751,#5152,.T.);
#47498=EDGE_CURVE('',#37753,#37754,#5153,.T.);
#47499=EDGE_CURVE('',#37752,#37754,#5154,.T.);
#47500=EDGE_CURVE('',#37751,#37753,#5155,.T.);
#47501=EDGE_CURVE('',#37754,#37749,#5156,.T.);
#47502=EDGE_CURVE('',#37753,#37750,#5157,.T.);
#47503=EDGE_CURVE('',#37755,#37756,#5158,.T.);
#47504=EDGE_CURVE('',#37757,#37756,#5159,.T.);
#47505=EDGE_CURVE('',#37758,#37757,#5160,.T.);
#47506=EDGE_CURVE('',#37758,#37755,#5161,.T.);
#47507=EDGE_CURVE('',#37759,#37760,#5162,.T.);
#47508=EDGE_CURVE('',#37756,#37760,#5163,.T.);
#47509=EDGE_CURVE('',#37755,#37759,#5164,.T.);
#47510=EDGE_CURVE('',#37761,#37762,#5165,.T.);
#47511=EDGE_CURVE('',#37760,#37762,#5166,.T.);
#47512=EDGE_CURVE('',#37759,#37761,#5167,.T.);
#47513=EDGE_CURVE('',#37762,#37757,#5168,.T.);
#47514=EDGE_CURVE('',#37761,#37758,#5169,.T.);
#47515=EDGE_CURVE('',#37763,#37764,#5170,.T.);
#47516=EDGE_CURVE('',#37765,#37764,#5171,.T.);
#47517=EDGE_CURVE('',#37766,#37765,#5172,.T.);
#47518=EDGE_CURVE('',#37766,#37763,#5173,.T.);
#47519=EDGE_CURVE('',#37767,#37768,#5174,.T.);
#47520=EDGE_CURVE('',#37764,#37768,#5175,.T.);
#47521=EDGE_CURVE('',#37763,#37767,#5176,.T.);
#47522=EDGE_CURVE('',#37769,#37770,#5177,.T.);
#47523=EDGE_CURVE('',#37768,#37770,#5178,.T.);
#47524=EDGE_CURVE('',#37767,#37769,#5179,.T.);
#47525=EDGE_CURVE('',#37770,#37765,#5180,.T.);
#47526=EDGE_CURVE('',#37769,#37766,#5181,.T.);
#47527=EDGE_CURVE('',#37771,#37772,#5182,.T.);
#47528=EDGE_CURVE('',#37773,#37772,#5183,.T.);
#47529=EDGE_CURVE('',#37774,#37773,#5184,.T.);
#47530=EDGE_CURVE('',#37774,#37771,#5185,.T.);
#47531=EDGE_CURVE('',#37775,#37776,#5186,.T.);
#47532=EDGE_CURVE('',#37772,#37776,#5187,.T.);
#47533=EDGE_CURVE('',#37771,#37775,#5188,.T.);
#47534=EDGE_CURVE('',#37777,#37778,#5189,.T.);
#47535=EDGE_CURVE('',#37776,#37778,#5190,.T.);
#47536=EDGE_CURVE('',#37775,#37777,#5191,.T.);
#47537=EDGE_CURVE('',#37778,#37773,#5192,.T.);
#47538=EDGE_CURVE('',#37777,#37774,#5193,.T.);
#47539=EDGE_CURVE('',#37779,#37780,#5194,.T.);
#47540=EDGE_CURVE('',#37781,#37780,#5195,.T.);
#47541=EDGE_CURVE('',#37782,#37781,#5196,.T.);
#47542=EDGE_CURVE('',#37782,#37779,#5197,.T.);
#47543=EDGE_CURVE('',#37783,#37784,#5198,.T.);
#47544=EDGE_CURVE('',#37780,#37784,#5199,.T.);
#47545=EDGE_CURVE('',#37779,#37783,#5200,.T.);
#47546=EDGE_CURVE('',#37785,#37786,#5201,.T.);
#47547=EDGE_CURVE('',#37784,#37786,#5202,.T.);
#47548=EDGE_CURVE('',#37783,#37785,#5203,.T.);
#47549=EDGE_CURVE('',#37786,#37781,#5204,.T.);
#47550=EDGE_CURVE('',#37785,#37782,#5205,.T.);
#47551=EDGE_CURVE('',#37787,#37788,#5206,.T.);
#47552=EDGE_CURVE('',#37789,#37788,#5207,.T.);
#47553=EDGE_CURVE('',#37790,#37789,#5208,.T.);
#47554=EDGE_CURVE('',#37790,#37787,#5209,.T.);
#47555=EDGE_CURVE('',#37791,#37792,#5210,.T.);
#47556=EDGE_CURVE('',#37788,#37792,#5211,.T.);
#47557=EDGE_CURVE('',#37787,#37791,#5212,.T.);
#47558=EDGE_CURVE('',#37793,#37794,#5213,.T.);
#47559=EDGE_CURVE('',#37792,#37794,#5214,.T.);
#47560=EDGE_CURVE('',#37791,#37793,#5215,.T.);
#47561=EDGE_CURVE('',#37794,#37789,#5216,.T.);
#47562=EDGE_CURVE('',#37793,#37790,#5217,.T.);
#47563=EDGE_CURVE('',#37795,#37796,#5218,.T.);
#47564=EDGE_CURVE('',#37797,#37796,#5219,.T.);
#47565=EDGE_CURVE('',#37798,#37797,#5220,.T.);
#47566=EDGE_CURVE('',#37798,#37795,#5221,.T.);
#47567=EDGE_CURVE('',#37799,#37800,#5222,.T.);
#47568=EDGE_CURVE('',#37796,#37800,#5223,.T.);
#47569=EDGE_CURVE('',#37795,#37799,#5224,.T.);
#47570=EDGE_CURVE('',#37801,#37802,#5225,.T.);
#47571=EDGE_CURVE('',#37800,#37802,#5226,.T.);
#47572=EDGE_CURVE('',#37799,#37801,#5227,.T.);
#47573=EDGE_CURVE('',#37802,#37797,#5228,.T.);
#47574=EDGE_CURVE('',#37801,#37798,#5229,.T.);
#47575=EDGE_CURVE('',#37803,#37804,#5230,.T.);
#47576=EDGE_CURVE('',#37805,#37804,#5231,.T.);
#47577=EDGE_CURVE('',#37806,#37805,#5232,.T.);
#47578=EDGE_CURVE('',#37806,#37803,#5233,.T.);
#47579=EDGE_CURVE('',#37807,#37808,#5234,.T.);
#47580=EDGE_CURVE('',#37804,#37808,#5235,.T.);
#47581=EDGE_CURVE('',#37803,#37807,#5236,.T.);
#47582=EDGE_CURVE('',#37809,#37810,#5237,.T.);
#47583=EDGE_CURVE('',#37808,#37810,#5238,.T.);
#47584=EDGE_CURVE('',#37807,#37809,#5239,.T.);
#47585=EDGE_CURVE('',#37810,#37805,#5240,.T.);
#47586=EDGE_CURVE('',#37809,#37806,#5241,.T.);
#47587=EDGE_CURVE('',#37811,#37812,#5242,.T.);
#47588=EDGE_CURVE('',#37813,#37812,#5243,.T.);
#47589=EDGE_CURVE('',#37814,#37813,#5244,.T.);
#47590=EDGE_CURVE('',#37814,#37811,#5245,.T.);
#47591=EDGE_CURVE('',#37815,#37816,#5246,.T.);
#47592=EDGE_CURVE('',#37812,#37816,#5247,.T.);
#47593=EDGE_CURVE('',#37811,#37815,#5248,.T.);
#47594=EDGE_CURVE('',#37817,#37818,#5249,.T.);
#47595=EDGE_CURVE('',#37816,#37818,#5250,.T.);
#47596=EDGE_CURVE('',#37815,#37817,#5251,.T.);
#47597=EDGE_CURVE('',#37818,#37813,#5252,.T.);
#47598=EDGE_CURVE('',#37817,#37814,#5253,.T.);
#47599=EDGE_CURVE('',#37819,#37820,#5254,.T.);
#47600=EDGE_CURVE('',#37821,#37820,#5255,.T.);
#47601=EDGE_CURVE('',#37822,#37821,#5256,.T.);
#47602=EDGE_CURVE('',#37822,#37819,#5257,.T.);
#47603=EDGE_CURVE('',#37823,#37824,#5258,.T.);
#47604=EDGE_CURVE('',#37820,#37824,#5259,.T.);
#47605=EDGE_CURVE('',#37819,#37823,#5260,.T.);
#47606=EDGE_CURVE('',#37825,#37826,#5261,.T.);
#47607=EDGE_CURVE('',#37824,#37826,#5262,.T.);
#47608=EDGE_CURVE('',#37823,#37825,#5263,.T.);
#47609=EDGE_CURVE('',#37826,#37821,#5264,.T.);
#47610=EDGE_CURVE('',#37825,#37822,#5265,.T.);
#47611=EDGE_CURVE('',#37827,#37828,#5266,.T.);
#47612=EDGE_CURVE('',#37829,#37828,#5267,.T.);
#47613=EDGE_CURVE('',#37830,#37829,#5268,.T.);
#47614=EDGE_CURVE('',#37830,#37827,#5269,.T.);
#47615=EDGE_CURVE('',#37831,#37832,#5270,.T.);
#47616=EDGE_CURVE('',#37828,#37832,#5271,.T.);
#47617=EDGE_CURVE('',#37827,#37831,#5272,.T.);
#47618=EDGE_CURVE('',#37833,#37834,#5273,.T.);
#47619=EDGE_CURVE('',#37832,#37834,#5274,.T.);
#47620=EDGE_CURVE('',#37831,#37833,#5275,.T.);
#47621=EDGE_CURVE('',#37834,#37829,#5276,.T.);
#47622=EDGE_CURVE('',#37833,#37830,#5277,.T.);
#47623=EDGE_CURVE('',#37835,#37836,#5278,.T.);
#47624=EDGE_CURVE('',#37837,#37836,#5279,.T.);
#47625=EDGE_CURVE('',#37838,#37837,#5280,.T.);
#47626=EDGE_CURVE('',#37838,#37835,#5281,.T.);
#47627=EDGE_CURVE('',#37839,#37840,#5282,.T.);
#47628=EDGE_CURVE('',#37836,#37840,#5283,.T.);
#47629=EDGE_CURVE('',#37835,#37839,#5284,.T.);
#47630=EDGE_CURVE('',#37841,#37842,#5285,.T.);
#47631=EDGE_CURVE('',#37840,#37842,#5286,.T.);
#47632=EDGE_CURVE('',#37839,#37841,#5287,.T.);
#47633=EDGE_CURVE('',#37842,#37837,#5288,.T.);
#47634=EDGE_CURVE('',#37841,#37838,#5289,.T.);
#47635=EDGE_CURVE('',#37843,#37844,#5290,.T.);
#47636=EDGE_CURVE('',#37845,#37844,#5291,.T.);
#47637=EDGE_CURVE('',#37846,#37845,#5292,.T.);
#47638=EDGE_CURVE('',#37846,#37843,#5293,.T.);
#47639=EDGE_CURVE('',#37847,#37848,#5294,.T.);
#47640=EDGE_CURVE('',#37844,#37848,#5295,.T.);
#47641=EDGE_CURVE('',#37843,#37847,#5296,.T.);
#47642=EDGE_CURVE('',#37849,#37850,#5297,.T.);
#47643=EDGE_CURVE('',#37848,#37850,#5298,.T.);
#47644=EDGE_CURVE('',#37847,#37849,#5299,.T.);
#47645=EDGE_CURVE('',#37850,#37845,#5300,.T.);
#47646=EDGE_CURVE('',#37849,#37846,#5301,.T.);
#47647=EDGE_CURVE('',#37851,#37852,#5302,.T.);
#47648=EDGE_CURVE('',#37853,#37852,#5303,.T.);
#47649=EDGE_CURVE('',#37854,#37853,#5304,.T.);
#47650=EDGE_CURVE('',#37854,#37851,#5305,.T.);
#47651=EDGE_CURVE('',#37855,#37856,#5306,.T.);
#47652=EDGE_CURVE('',#37852,#37856,#5307,.T.);
#47653=EDGE_CURVE('',#37851,#37855,#5308,.T.);
#47654=EDGE_CURVE('',#37857,#37858,#5309,.T.);
#47655=EDGE_CURVE('',#37856,#37858,#5310,.T.);
#47656=EDGE_CURVE('',#37855,#37857,#5311,.T.);
#47657=EDGE_CURVE('',#37858,#37853,#5312,.T.);
#47658=EDGE_CURVE('',#37857,#37854,#5313,.T.);
#47659=EDGE_CURVE('',#37859,#37860,#5314,.T.);
#47660=EDGE_CURVE('',#37861,#37860,#5315,.T.);
#47661=EDGE_CURVE('',#37862,#37861,#5316,.T.);
#47662=EDGE_CURVE('',#37862,#37859,#5317,.T.);
#47663=EDGE_CURVE('',#37863,#37864,#5318,.T.);
#47664=EDGE_CURVE('',#37860,#37864,#5319,.T.);
#47665=EDGE_CURVE('',#37859,#37863,#5320,.T.);
#47666=EDGE_CURVE('',#37865,#37866,#5321,.T.);
#47667=EDGE_CURVE('',#37864,#37866,#5322,.T.);
#47668=EDGE_CURVE('',#37863,#37865,#5323,.T.);
#47669=EDGE_CURVE('',#37866,#37861,#5324,.T.);
#47670=EDGE_CURVE('',#37865,#37862,#5325,.T.);
#47671=EDGE_CURVE('',#37867,#37868,#5326,.T.);
#47672=EDGE_CURVE('',#37869,#37868,#5327,.T.);
#47673=EDGE_CURVE('',#37870,#37869,#5328,.T.);
#47674=EDGE_CURVE('',#37870,#37867,#5329,.T.);
#47675=EDGE_CURVE('',#37871,#37872,#5330,.T.);
#47676=EDGE_CURVE('',#37868,#37872,#5331,.T.);
#47677=EDGE_CURVE('',#37867,#37871,#5332,.T.);
#47678=EDGE_CURVE('',#37873,#37874,#5333,.T.);
#47679=EDGE_CURVE('',#37872,#37874,#5334,.T.);
#47680=EDGE_CURVE('',#37871,#37873,#5335,.T.);
#47681=EDGE_CURVE('',#37874,#37869,#5336,.T.);
#47682=EDGE_CURVE('',#37873,#37870,#5337,.T.);
#47683=EDGE_CURVE('',#37875,#37876,#5338,.T.);
#47684=EDGE_CURVE('',#37877,#37876,#5339,.T.);
#47685=EDGE_CURVE('',#37878,#37877,#5340,.T.);
#47686=EDGE_CURVE('',#37878,#37875,#5341,.T.);
#47687=EDGE_CURVE('',#37879,#37880,#5342,.T.);
#47688=EDGE_CURVE('',#37876,#37880,#5343,.T.);
#47689=EDGE_CURVE('',#37875,#37879,#5344,.T.);
#47690=EDGE_CURVE('',#37881,#37882,#5345,.T.);
#47691=EDGE_CURVE('',#37880,#37882,#5346,.T.);
#47692=EDGE_CURVE('',#37879,#37881,#5347,.T.);
#47693=EDGE_CURVE('',#37882,#37877,#5348,.T.);
#47694=EDGE_CURVE('',#37881,#37878,#5349,.T.);
#47695=EDGE_CURVE('',#37883,#37884,#5350,.T.);
#47696=EDGE_CURVE('',#37885,#37884,#5351,.T.);
#47697=EDGE_CURVE('',#37886,#37885,#5352,.T.);
#47698=EDGE_CURVE('',#37886,#37883,#5353,.T.);
#47699=EDGE_CURVE('',#37887,#37888,#5354,.T.);
#47700=EDGE_CURVE('',#37884,#37888,#5355,.T.);
#47701=EDGE_CURVE('',#37883,#37887,#5356,.T.);
#47702=EDGE_CURVE('',#37889,#37890,#5357,.T.);
#47703=EDGE_CURVE('',#37888,#37890,#5358,.T.);
#47704=EDGE_CURVE('',#37887,#37889,#5359,.T.);
#47705=EDGE_CURVE('',#37890,#37885,#5360,.T.);
#47706=EDGE_CURVE('',#37889,#37886,#5361,.T.);
#47707=EDGE_CURVE('',#37891,#37892,#5362,.T.);
#47708=EDGE_CURVE('',#37893,#37892,#5363,.T.);
#47709=EDGE_CURVE('',#37894,#37893,#5364,.T.);
#47710=EDGE_CURVE('',#37894,#37891,#5365,.T.);
#47711=EDGE_CURVE('',#37895,#37896,#5366,.T.);
#47712=EDGE_CURVE('',#37892,#37896,#5367,.T.);
#47713=EDGE_CURVE('',#37891,#37895,#5368,.T.);
#47714=EDGE_CURVE('',#37897,#37898,#5369,.T.);
#47715=EDGE_CURVE('',#37896,#37898,#5370,.T.);
#47716=EDGE_CURVE('',#37895,#37897,#5371,.T.);
#47717=EDGE_CURVE('',#37898,#37893,#5372,.T.);
#47718=EDGE_CURVE('',#37897,#37894,#5373,.T.);
#47719=EDGE_CURVE('',#37899,#37900,#5374,.T.);
#47720=EDGE_CURVE('',#37901,#37900,#5375,.T.);
#47721=EDGE_CURVE('',#37902,#37901,#5376,.T.);
#47722=EDGE_CURVE('',#37902,#37899,#5377,.T.);
#47723=EDGE_CURVE('',#37903,#37904,#5378,.T.);
#47724=EDGE_CURVE('',#37900,#37904,#5379,.T.);
#47725=EDGE_CURVE('',#37899,#37903,#5380,.T.);
#47726=EDGE_CURVE('',#37905,#37906,#5381,.T.);
#47727=EDGE_CURVE('',#37904,#37906,#5382,.T.);
#47728=EDGE_CURVE('',#37903,#37905,#5383,.T.);
#47729=EDGE_CURVE('',#37906,#37901,#5384,.T.);
#47730=EDGE_CURVE('',#37905,#37902,#5385,.T.);
#47731=EDGE_CURVE('',#37907,#37908,#5386,.T.);
#47732=EDGE_CURVE('',#37909,#37908,#5387,.T.);
#47733=EDGE_CURVE('',#37910,#37909,#5388,.T.);
#47734=EDGE_CURVE('',#37910,#37907,#5389,.T.);
#47735=EDGE_CURVE('',#37911,#37912,#5390,.T.);
#47736=EDGE_CURVE('',#37908,#37912,#5391,.T.);
#47737=EDGE_CURVE('',#37907,#37911,#5392,.T.);
#47738=EDGE_CURVE('',#37913,#37914,#5393,.T.);
#47739=EDGE_CURVE('',#37912,#37914,#5394,.T.);
#47740=EDGE_CURVE('',#37911,#37913,#5395,.T.);
#47741=EDGE_CURVE('',#37914,#37909,#5396,.T.);
#47742=EDGE_CURVE('',#37913,#37910,#5397,.T.);
#47743=EDGE_CURVE('',#37915,#37916,#5398,.T.);
#47744=EDGE_CURVE('',#37917,#37916,#5399,.T.);
#47745=EDGE_CURVE('',#37918,#37917,#5400,.T.);
#47746=EDGE_CURVE('',#37918,#37915,#5401,.T.);
#47747=EDGE_CURVE('',#37919,#37920,#5402,.T.);
#47748=EDGE_CURVE('',#37916,#37920,#5403,.T.);
#47749=EDGE_CURVE('',#37915,#37919,#5404,.T.);
#47750=EDGE_CURVE('',#37921,#37922,#5405,.T.);
#47751=EDGE_CURVE('',#37920,#37922,#5406,.T.);
#47752=EDGE_CURVE('',#37919,#37921,#5407,.T.);
#47753=EDGE_CURVE('',#37922,#37917,#5408,.T.);
#47754=EDGE_CURVE('',#37921,#37918,#5409,.T.);
#47755=EDGE_CURVE('',#37923,#37924,#5410,.T.);
#47756=EDGE_CURVE('',#37925,#37924,#5411,.T.);
#47757=EDGE_CURVE('',#37926,#37925,#5412,.T.);
#47758=EDGE_CURVE('',#37926,#37923,#5413,.T.);
#47759=EDGE_CURVE('',#37927,#37928,#5414,.T.);
#47760=EDGE_CURVE('',#37924,#37928,#5415,.T.);
#47761=EDGE_CURVE('',#37923,#37927,#5416,.T.);
#47762=EDGE_CURVE('',#37929,#37930,#5417,.T.);
#47763=EDGE_CURVE('',#37928,#37930,#5418,.T.);
#47764=EDGE_CURVE('',#37927,#37929,#5419,.T.);
#47765=EDGE_CURVE('',#37930,#37925,#5420,.T.);
#47766=EDGE_CURVE('',#37929,#37926,#5421,.T.);
#47767=EDGE_CURVE('',#37931,#37932,#5422,.T.);
#47768=EDGE_CURVE('',#37933,#37932,#5423,.T.);
#47769=EDGE_CURVE('',#37934,#37933,#5424,.T.);
#47770=EDGE_CURVE('',#37934,#37931,#5425,.T.);
#47771=EDGE_CURVE('',#37935,#37936,#5426,.T.);
#47772=EDGE_CURVE('',#37932,#37936,#5427,.T.);
#47773=EDGE_CURVE('',#37931,#37935,#5428,.T.);
#47774=EDGE_CURVE('',#37937,#37938,#5429,.T.);
#47775=EDGE_CURVE('',#37936,#37938,#5430,.T.);
#47776=EDGE_CURVE('',#37935,#37937,#5431,.T.);
#47777=EDGE_CURVE('',#37938,#37933,#5432,.T.);
#47778=EDGE_CURVE('',#37937,#37934,#5433,.T.);
#47779=EDGE_CURVE('',#37939,#37940,#5434,.T.);
#47780=EDGE_CURVE('',#37941,#37940,#5435,.T.);
#47781=EDGE_CURVE('',#37942,#37941,#5436,.T.);
#47782=EDGE_CURVE('',#37942,#37939,#5437,.T.);
#47783=EDGE_CURVE('',#37943,#37944,#5438,.T.);
#47784=EDGE_CURVE('',#37940,#37944,#5439,.T.);
#47785=EDGE_CURVE('',#37939,#37943,#5440,.T.);
#47786=EDGE_CURVE('',#37945,#37946,#5441,.T.);
#47787=EDGE_CURVE('',#37944,#37946,#5442,.T.);
#47788=EDGE_CURVE('',#37943,#37945,#5443,.T.);
#47789=EDGE_CURVE('',#37946,#37941,#5444,.T.);
#47790=EDGE_CURVE('',#37945,#37942,#5445,.T.);
#47791=EDGE_CURVE('',#37947,#37948,#5446,.T.);
#47792=EDGE_CURVE('',#37949,#37948,#5447,.T.);
#47793=EDGE_CURVE('',#37950,#37949,#5448,.T.);
#47794=EDGE_CURVE('',#37950,#37947,#5449,.T.);
#47795=EDGE_CURVE('',#37951,#37952,#5450,.T.);
#47796=EDGE_CURVE('',#37948,#37952,#5451,.T.);
#47797=EDGE_CURVE('',#37947,#37951,#5452,.T.);
#47798=EDGE_CURVE('',#37953,#37954,#5453,.T.);
#47799=EDGE_CURVE('',#37952,#37954,#5454,.T.);
#47800=EDGE_CURVE('',#37951,#37953,#5455,.T.);
#47801=EDGE_CURVE('',#37954,#37949,#5456,.T.);
#47802=EDGE_CURVE('',#37953,#37950,#5457,.T.);
#47803=EDGE_CURVE('',#37955,#37956,#5458,.T.);
#47804=EDGE_CURVE('',#37957,#37956,#5459,.T.);
#47805=EDGE_CURVE('',#37958,#37957,#5460,.T.);
#47806=EDGE_CURVE('',#37958,#37955,#5461,.T.);
#47807=EDGE_CURVE('',#37959,#37960,#5462,.T.);
#47808=EDGE_CURVE('',#37956,#37960,#5463,.T.);
#47809=EDGE_CURVE('',#37955,#37959,#5464,.T.);
#47810=EDGE_CURVE('',#37961,#37962,#5465,.T.);
#47811=EDGE_CURVE('',#37960,#37962,#5466,.T.);
#47812=EDGE_CURVE('',#37959,#37961,#5467,.T.);
#47813=EDGE_CURVE('',#37962,#37957,#5468,.T.);
#47814=EDGE_CURVE('',#37961,#37958,#5469,.T.);
#47815=EDGE_CURVE('',#37963,#37964,#5470,.T.);
#47816=EDGE_CURVE('',#37965,#37964,#5471,.T.);
#47817=EDGE_CURVE('',#37966,#37965,#5472,.T.);
#47818=EDGE_CURVE('',#37966,#37963,#5473,.T.);
#47819=EDGE_CURVE('',#37967,#37968,#5474,.T.);
#47820=EDGE_CURVE('',#37964,#37968,#5475,.T.);
#47821=EDGE_CURVE('',#37963,#37967,#5476,.T.);
#47822=EDGE_CURVE('',#37969,#37970,#5477,.T.);
#47823=EDGE_CURVE('',#37968,#37970,#5478,.T.);
#47824=EDGE_CURVE('',#37967,#37969,#5479,.T.);
#47825=EDGE_CURVE('',#37970,#37965,#5480,.T.);
#47826=EDGE_CURVE('',#37969,#37966,#5481,.T.);
#47827=EDGE_CURVE('',#37971,#37972,#5482,.T.);
#47828=EDGE_CURVE('',#37973,#37972,#5483,.T.);
#47829=EDGE_CURVE('',#37974,#37973,#5484,.T.);
#47830=EDGE_CURVE('',#37974,#37971,#5485,.T.);
#47831=EDGE_CURVE('',#37975,#37976,#5486,.T.);
#47832=EDGE_CURVE('',#37972,#37976,#5487,.T.);
#47833=EDGE_CURVE('',#37971,#37975,#5488,.T.);
#47834=EDGE_CURVE('',#37977,#37978,#5489,.T.);
#47835=EDGE_CURVE('',#37976,#37978,#5490,.T.);
#47836=EDGE_CURVE('',#37975,#37977,#5491,.T.);
#47837=EDGE_CURVE('',#37978,#37973,#5492,.T.);
#47838=EDGE_CURVE('',#37977,#37974,#5493,.T.);
#47839=EDGE_CURVE('',#37979,#37980,#5494,.T.);
#47840=EDGE_CURVE('',#37981,#37980,#5495,.T.);
#47841=EDGE_CURVE('',#37982,#37981,#5496,.T.);
#47842=EDGE_CURVE('',#37982,#37979,#5497,.T.);
#47843=EDGE_CURVE('',#37983,#37984,#5498,.T.);
#47844=EDGE_CURVE('',#37980,#37984,#5499,.T.);
#47845=EDGE_CURVE('',#37979,#37983,#5500,.T.);
#47846=EDGE_CURVE('',#37985,#37986,#5501,.T.);
#47847=EDGE_CURVE('',#37984,#37986,#5502,.T.);
#47848=EDGE_CURVE('',#37983,#37985,#5503,.T.);
#47849=EDGE_CURVE('',#37986,#37981,#5504,.T.);
#47850=EDGE_CURVE('',#37985,#37982,#5505,.T.);
#47851=EDGE_CURVE('',#37987,#37988,#5506,.T.);
#47852=EDGE_CURVE('',#37989,#37988,#5507,.T.);
#47853=EDGE_CURVE('',#37990,#37989,#5508,.T.);
#47854=EDGE_CURVE('',#37990,#37987,#5509,.T.);
#47855=EDGE_CURVE('',#37991,#37992,#5510,.T.);
#47856=EDGE_CURVE('',#37988,#37992,#5511,.T.);
#47857=EDGE_CURVE('',#37987,#37991,#5512,.T.);
#47858=EDGE_CURVE('',#37993,#37994,#5513,.T.);
#47859=EDGE_CURVE('',#37992,#37994,#5514,.T.);
#47860=EDGE_CURVE('',#37991,#37993,#5515,.T.);
#47861=EDGE_CURVE('',#37994,#37989,#5516,.T.);
#47862=EDGE_CURVE('',#37993,#37990,#5517,.T.);
#47863=EDGE_CURVE('',#37995,#37996,#5518,.T.);
#47864=EDGE_CURVE('',#37997,#37996,#5519,.T.);
#47865=EDGE_CURVE('',#37998,#37997,#5520,.T.);
#47866=EDGE_CURVE('',#37998,#37995,#5521,.T.);
#47867=EDGE_CURVE('',#37999,#38000,#5522,.T.);
#47868=EDGE_CURVE('',#37996,#38000,#5523,.T.);
#47869=EDGE_CURVE('',#37995,#37999,#5524,.T.);
#47870=EDGE_CURVE('',#38001,#38002,#5525,.T.);
#47871=EDGE_CURVE('',#38000,#38002,#5526,.T.);
#47872=EDGE_CURVE('',#37999,#38001,#5527,.T.);
#47873=EDGE_CURVE('',#38002,#37997,#5528,.T.);
#47874=EDGE_CURVE('',#38001,#37998,#5529,.T.);
#47875=EDGE_CURVE('',#38003,#38004,#5530,.T.);
#47876=EDGE_CURVE('',#38005,#38004,#5531,.T.);
#47877=EDGE_CURVE('',#38006,#38005,#5532,.T.);
#47878=EDGE_CURVE('',#38006,#38003,#5533,.T.);
#47879=EDGE_CURVE('',#38007,#38008,#5534,.T.);
#47880=EDGE_CURVE('',#38004,#38008,#5535,.T.);
#47881=EDGE_CURVE('',#38003,#38007,#5536,.T.);
#47882=EDGE_CURVE('',#38009,#38010,#5537,.T.);
#47883=EDGE_CURVE('',#38008,#38010,#5538,.T.);
#47884=EDGE_CURVE('',#38007,#38009,#5539,.T.);
#47885=EDGE_CURVE('',#38010,#38005,#5540,.T.);
#47886=EDGE_CURVE('',#38009,#38006,#5541,.T.);
#47887=EDGE_CURVE('',#38011,#38012,#5542,.T.);
#47888=EDGE_CURVE('',#38013,#38012,#5543,.T.);
#47889=EDGE_CURVE('',#38014,#38013,#5544,.T.);
#47890=EDGE_CURVE('',#38014,#38011,#5545,.T.);
#47891=EDGE_CURVE('',#38015,#38016,#5546,.T.);
#47892=EDGE_CURVE('',#38012,#38016,#5547,.T.);
#47893=EDGE_CURVE('',#38011,#38015,#5548,.T.);
#47894=EDGE_CURVE('',#38017,#38018,#5549,.T.);
#47895=EDGE_CURVE('',#38016,#38018,#5550,.T.);
#47896=EDGE_CURVE('',#38015,#38017,#5551,.T.);
#47897=EDGE_CURVE('',#38018,#38013,#5552,.T.);
#47898=EDGE_CURVE('',#38017,#38014,#5553,.T.);
#47899=EDGE_CURVE('',#38019,#38020,#5554,.T.);
#47900=EDGE_CURVE('',#38021,#38020,#5555,.T.);
#47901=EDGE_CURVE('',#38022,#38021,#5556,.T.);
#47902=EDGE_CURVE('',#38022,#38019,#5557,.T.);
#47903=EDGE_CURVE('',#38023,#38024,#5558,.T.);
#47904=EDGE_CURVE('',#38020,#38024,#5559,.T.);
#47905=EDGE_CURVE('',#38019,#38023,#5560,.T.);
#47906=EDGE_CURVE('',#38025,#38026,#5561,.T.);
#47907=EDGE_CURVE('',#38024,#38026,#5562,.T.);
#47908=EDGE_CURVE('',#38023,#38025,#5563,.T.);
#47909=EDGE_CURVE('',#38026,#38021,#5564,.T.);
#47910=EDGE_CURVE('',#38025,#38022,#5565,.T.);
#47911=EDGE_CURVE('',#38027,#38028,#5566,.T.);
#47912=EDGE_CURVE('',#38029,#38028,#5567,.T.);
#47913=EDGE_CURVE('',#38030,#38029,#5568,.T.);
#47914=EDGE_CURVE('',#38030,#38027,#5569,.T.);
#47915=EDGE_CURVE('',#38031,#38032,#5570,.T.);
#47916=EDGE_CURVE('',#38028,#38032,#5571,.T.);
#47917=EDGE_CURVE('',#38027,#38031,#5572,.T.);
#47918=EDGE_CURVE('',#38033,#38034,#5573,.T.);
#47919=EDGE_CURVE('',#38032,#38034,#5574,.T.);
#47920=EDGE_CURVE('',#38031,#38033,#5575,.T.);
#47921=EDGE_CURVE('',#38034,#38029,#5576,.T.);
#47922=EDGE_CURVE('',#38033,#38030,#5577,.T.);
#47923=EDGE_CURVE('',#38035,#38036,#5578,.T.);
#47924=EDGE_CURVE('',#38037,#38036,#5579,.T.);
#47925=EDGE_CURVE('',#38038,#38037,#5580,.T.);
#47926=EDGE_CURVE('',#38038,#38035,#5581,.T.);
#47927=EDGE_CURVE('',#38039,#38040,#5582,.T.);
#47928=EDGE_CURVE('',#38036,#38040,#5583,.T.);
#47929=EDGE_CURVE('',#38035,#38039,#5584,.T.);
#47930=EDGE_CURVE('',#38041,#38042,#5585,.T.);
#47931=EDGE_CURVE('',#38040,#38042,#5586,.T.);
#47932=EDGE_CURVE('',#38039,#38041,#5587,.T.);
#47933=EDGE_CURVE('',#38042,#38037,#5588,.T.);
#47934=EDGE_CURVE('',#38041,#38038,#5589,.T.);
#47935=EDGE_CURVE('',#38043,#38044,#5590,.T.);
#47936=EDGE_CURVE('',#38045,#38044,#5591,.T.);
#47937=EDGE_CURVE('',#38046,#38045,#5592,.T.);
#47938=EDGE_CURVE('',#38046,#38043,#5593,.T.);
#47939=EDGE_CURVE('',#38047,#38048,#5594,.T.);
#47940=EDGE_CURVE('',#38044,#38048,#5595,.T.);
#47941=EDGE_CURVE('',#38043,#38047,#5596,.T.);
#47942=EDGE_CURVE('',#38049,#38050,#5597,.T.);
#47943=EDGE_CURVE('',#38048,#38050,#5598,.T.);
#47944=EDGE_CURVE('',#38047,#38049,#5599,.T.);
#47945=EDGE_CURVE('',#38050,#38045,#5600,.T.);
#47946=EDGE_CURVE('',#38049,#38046,#5601,.T.);
#47947=EDGE_CURVE('',#38051,#38052,#5602,.T.);
#47948=EDGE_CURVE('',#38053,#38052,#5603,.T.);
#47949=EDGE_CURVE('',#38054,#38053,#5604,.T.);
#47950=EDGE_CURVE('',#38054,#38051,#5605,.T.);
#47951=EDGE_CURVE('',#38055,#38056,#5606,.T.);
#47952=EDGE_CURVE('',#38052,#38056,#5607,.T.);
#47953=EDGE_CURVE('',#38051,#38055,#5608,.T.);
#47954=EDGE_CURVE('',#38057,#38058,#5609,.T.);
#47955=EDGE_CURVE('',#38056,#38058,#5610,.T.);
#47956=EDGE_CURVE('',#38055,#38057,#5611,.T.);
#47957=EDGE_CURVE('',#38058,#38053,#5612,.T.);
#47958=EDGE_CURVE('',#38057,#38054,#5613,.T.);
#47959=EDGE_CURVE('',#38059,#38060,#5614,.T.);
#47960=EDGE_CURVE('',#38061,#38060,#5615,.T.);
#47961=EDGE_CURVE('',#38062,#38061,#5616,.T.);
#47962=EDGE_CURVE('',#38062,#38059,#5617,.T.);
#47963=EDGE_CURVE('',#38063,#38064,#5618,.T.);
#47964=EDGE_CURVE('',#38060,#38064,#5619,.T.);
#47965=EDGE_CURVE('',#38059,#38063,#5620,.T.);
#47966=EDGE_CURVE('',#38065,#38066,#5621,.T.);
#47967=EDGE_CURVE('',#38064,#38066,#5622,.T.);
#47968=EDGE_CURVE('',#38063,#38065,#5623,.T.);
#47969=EDGE_CURVE('',#38066,#38061,#5624,.T.);
#47970=EDGE_CURVE('',#38065,#38062,#5625,.T.);
#47971=EDGE_CURVE('',#38067,#38068,#5626,.T.);
#47972=EDGE_CURVE('',#38069,#38068,#5627,.T.);
#47973=EDGE_CURVE('',#38070,#38069,#5628,.T.);
#47974=EDGE_CURVE('',#38070,#38067,#5629,.T.);
#47975=EDGE_CURVE('',#38071,#38072,#5630,.T.);
#47976=EDGE_CURVE('',#38068,#38072,#5631,.T.);
#47977=EDGE_CURVE('',#38067,#38071,#5632,.T.);
#47978=EDGE_CURVE('',#38073,#38074,#5633,.T.);
#47979=EDGE_CURVE('',#38072,#38074,#5634,.T.);
#47980=EDGE_CURVE('',#38071,#38073,#5635,.T.);
#47981=EDGE_CURVE('',#38074,#38069,#5636,.T.);
#47982=EDGE_CURVE('',#38073,#38070,#5637,.T.);
#47983=EDGE_CURVE('',#38075,#38076,#5638,.T.);
#47984=EDGE_CURVE('',#38077,#38076,#5639,.T.);
#47985=EDGE_CURVE('',#38078,#38077,#5640,.T.);
#47986=EDGE_CURVE('',#38078,#38075,#5641,.T.);
#47987=EDGE_CURVE('',#38079,#38080,#5642,.T.);
#47988=EDGE_CURVE('',#38076,#38080,#5643,.T.);
#47989=EDGE_CURVE('',#38075,#38079,#5644,.T.);
#47990=EDGE_CURVE('',#38081,#38082,#5645,.T.);
#47991=EDGE_CURVE('',#38080,#38082,#5646,.T.);
#47992=EDGE_CURVE('',#38079,#38081,#5647,.T.);
#47993=EDGE_CURVE('',#38082,#38077,#5648,.T.);
#47994=EDGE_CURVE('',#38081,#38078,#5649,.T.);
#47995=EDGE_CURVE('',#38083,#38084,#5650,.T.);
#47996=EDGE_CURVE('',#38085,#38084,#5651,.T.);
#47997=EDGE_CURVE('',#38086,#38085,#5652,.T.);
#47998=EDGE_CURVE('',#38086,#38083,#5653,.T.);
#47999=EDGE_CURVE('',#38087,#38088,#5654,.T.);
#48000=EDGE_CURVE('',#38084,#38088,#5655,.T.);
#48001=EDGE_CURVE('',#38083,#38087,#5656,.T.);
#48002=EDGE_CURVE('',#38089,#38090,#5657,.T.);
#48003=EDGE_CURVE('',#38088,#38090,#5658,.T.);
#48004=EDGE_CURVE('',#38087,#38089,#5659,.T.);
#48005=EDGE_CURVE('',#38090,#38085,#5660,.T.);
#48006=EDGE_CURVE('',#38089,#38086,#5661,.T.);
#48007=EDGE_CURVE('',#38091,#38092,#5662,.T.);
#48008=EDGE_CURVE('',#38093,#38092,#5663,.T.);
#48009=EDGE_CURVE('',#38094,#38093,#5664,.T.);
#48010=EDGE_CURVE('',#38094,#38091,#5665,.T.);
#48011=EDGE_CURVE('',#38095,#38096,#5666,.T.);
#48012=EDGE_CURVE('',#38092,#38096,#5667,.T.);
#48013=EDGE_CURVE('',#38091,#38095,#5668,.T.);
#48014=EDGE_CURVE('',#38097,#38098,#5669,.T.);
#48015=EDGE_CURVE('',#38096,#38098,#5670,.T.);
#48016=EDGE_CURVE('',#38095,#38097,#5671,.T.);
#48017=EDGE_CURVE('',#38098,#38093,#5672,.T.);
#48018=EDGE_CURVE('',#38097,#38094,#5673,.T.);
#48019=EDGE_CURVE('',#38099,#38100,#5674,.T.);
#48020=EDGE_CURVE('',#38101,#38100,#5675,.T.);
#48021=EDGE_CURVE('',#38102,#38101,#5676,.T.);
#48022=EDGE_CURVE('',#38102,#38099,#5677,.T.);
#48023=EDGE_CURVE('',#38103,#38104,#5678,.T.);
#48024=EDGE_CURVE('',#38100,#38104,#5679,.T.);
#48025=EDGE_CURVE('',#38099,#38103,#5680,.T.);
#48026=EDGE_CURVE('',#38105,#38106,#5681,.T.);
#48027=EDGE_CURVE('',#38104,#38106,#5682,.T.);
#48028=EDGE_CURVE('',#38103,#38105,#5683,.T.);
#48029=EDGE_CURVE('',#38106,#38101,#5684,.T.);
#48030=EDGE_CURVE('',#38105,#38102,#5685,.T.);
#48031=EDGE_CURVE('',#38107,#38108,#5686,.T.);
#48032=EDGE_CURVE('',#38109,#38108,#5687,.T.);
#48033=EDGE_CURVE('',#38110,#38109,#5688,.T.);
#48034=EDGE_CURVE('',#38110,#38107,#5689,.T.);
#48035=EDGE_CURVE('',#38111,#38112,#5690,.T.);
#48036=EDGE_CURVE('',#38108,#38112,#5691,.T.);
#48037=EDGE_CURVE('',#38107,#38111,#5692,.T.);
#48038=EDGE_CURVE('',#38113,#38114,#5693,.T.);
#48039=EDGE_CURVE('',#38112,#38114,#5694,.T.);
#48040=EDGE_CURVE('',#38111,#38113,#5695,.T.);
#48041=EDGE_CURVE('',#38114,#38109,#5696,.T.);
#48042=EDGE_CURVE('',#38113,#38110,#5697,.T.);
#48043=EDGE_CURVE('',#38115,#38116,#5698,.T.);
#48044=EDGE_CURVE('',#38117,#38116,#5699,.T.);
#48045=EDGE_CURVE('',#38118,#38117,#5700,.T.);
#48046=EDGE_CURVE('',#38118,#38115,#5701,.T.);
#48047=EDGE_CURVE('',#38119,#38120,#5702,.T.);
#48048=EDGE_CURVE('',#38116,#38120,#5703,.T.);
#48049=EDGE_CURVE('',#38115,#38119,#5704,.T.);
#48050=EDGE_CURVE('',#38121,#38122,#5705,.T.);
#48051=EDGE_CURVE('',#38120,#38122,#5706,.T.);
#48052=EDGE_CURVE('',#38119,#38121,#5707,.T.);
#48053=EDGE_CURVE('',#38122,#38117,#5708,.T.);
#48054=EDGE_CURVE('',#38121,#38118,#5709,.T.);
#48055=EDGE_CURVE('',#38123,#38124,#5710,.T.);
#48056=EDGE_CURVE('',#38125,#38124,#5711,.T.);
#48057=EDGE_CURVE('',#38126,#38125,#5712,.T.);
#48058=EDGE_CURVE('',#38126,#38123,#5713,.T.);
#48059=EDGE_CURVE('',#38127,#38128,#5714,.T.);
#48060=EDGE_CURVE('',#38124,#38128,#5715,.T.);
#48061=EDGE_CURVE('',#38123,#38127,#5716,.T.);
#48062=EDGE_CURVE('',#38129,#38130,#5717,.T.);
#48063=EDGE_CURVE('',#38128,#38130,#5718,.T.);
#48064=EDGE_CURVE('',#38127,#38129,#5719,.T.);
#48065=EDGE_CURVE('',#38130,#38125,#5720,.T.);
#48066=EDGE_CURVE('',#38129,#38126,#5721,.T.);
#48067=EDGE_CURVE('',#38131,#38132,#5722,.T.);
#48068=EDGE_CURVE('',#38133,#38132,#5723,.T.);
#48069=EDGE_CURVE('',#38134,#38133,#5724,.T.);
#48070=EDGE_CURVE('',#38134,#38131,#5725,.T.);
#48071=EDGE_CURVE('',#38135,#38136,#5726,.T.);
#48072=EDGE_CURVE('',#38132,#38136,#5727,.T.);
#48073=EDGE_CURVE('',#38131,#38135,#5728,.T.);
#48074=EDGE_CURVE('',#38137,#38138,#5729,.T.);
#48075=EDGE_CURVE('',#38136,#38138,#5730,.T.);
#48076=EDGE_CURVE('',#38135,#38137,#5731,.T.);
#48077=EDGE_CURVE('',#38138,#38133,#5732,.T.);
#48078=EDGE_CURVE('',#38137,#38134,#5733,.T.);
#48079=EDGE_CURVE('',#38139,#38140,#5734,.T.);
#48080=EDGE_CURVE('',#38141,#38140,#5735,.T.);
#48081=EDGE_CURVE('',#38142,#38141,#5736,.T.);
#48082=EDGE_CURVE('',#38142,#38139,#5737,.T.);
#48083=EDGE_CURVE('',#38143,#38144,#5738,.T.);
#48084=EDGE_CURVE('',#38140,#38144,#5739,.T.);
#48085=EDGE_CURVE('',#38139,#38143,#5740,.T.);
#48086=EDGE_CURVE('',#38145,#38146,#5741,.T.);
#48087=EDGE_CURVE('',#38144,#38146,#5742,.T.);
#48088=EDGE_CURVE('',#38143,#38145,#5743,.T.);
#48089=EDGE_CURVE('',#38146,#38141,#5744,.T.);
#48090=EDGE_CURVE('',#38145,#38142,#5745,.T.);
#48091=EDGE_CURVE('',#38147,#38148,#5746,.T.);
#48092=EDGE_CURVE('',#38149,#38148,#5747,.T.);
#48093=EDGE_CURVE('',#38150,#38149,#5748,.T.);
#48094=EDGE_CURVE('',#38150,#38147,#5749,.T.);
#48095=EDGE_CURVE('',#38151,#38152,#5750,.T.);
#48096=EDGE_CURVE('',#38148,#38152,#5751,.T.);
#48097=EDGE_CURVE('',#38147,#38151,#5752,.T.);
#48098=EDGE_CURVE('',#38153,#38154,#5753,.T.);
#48099=EDGE_CURVE('',#38152,#38154,#5754,.T.);
#48100=EDGE_CURVE('',#38151,#38153,#5755,.T.);
#48101=EDGE_CURVE('',#38154,#38149,#5756,.T.);
#48102=EDGE_CURVE('',#38153,#38150,#5757,.T.);
#48103=EDGE_CURVE('',#38155,#38156,#5758,.T.);
#48104=EDGE_CURVE('',#38157,#38156,#5759,.T.);
#48105=EDGE_CURVE('',#38158,#38157,#5760,.T.);
#48106=EDGE_CURVE('',#38158,#38155,#5761,.T.);
#48107=EDGE_CURVE('',#38159,#38160,#5762,.T.);
#48108=EDGE_CURVE('',#38156,#38160,#5763,.T.);
#48109=EDGE_CURVE('',#38155,#38159,#5764,.T.);
#48110=EDGE_CURVE('',#38161,#38162,#5765,.T.);
#48111=EDGE_CURVE('',#38160,#38162,#5766,.T.);
#48112=EDGE_CURVE('',#38159,#38161,#5767,.T.);
#48113=EDGE_CURVE('',#38162,#38157,#5768,.T.);
#48114=EDGE_CURVE('',#38161,#38158,#5769,.T.);
#48115=EDGE_CURVE('',#38163,#38164,#5770,.T.);
#48116=EDGE_CURVE('',#38165,#38164,#5771,.T.);
#48117=EDGE_CURVE('',#38166,#38165,#5772,.T.);
#48118=EDGE_CURVE('',#38166,#38163,#5773,.T.);
#48119=EDGE_CURVE('',#38167,#38168,#5774,.T.);
#48120=EDGE_CURVE('',#38164,#38168,#5775,.T.);
#48121=EDGE_CURVE('',#38163,#38167,#5776,.T.);
#48122=EDGE_CURVE('',#38169,#38170,#5777,.T.);
#48123=EDGE_CURVE('',#38168,#38170,#5778,.T.);
#48124=EDGE_CURVE('',#38167,#38169,#5779,.T.);
#48125=EDGE_CURVE('',#38170,#38165,#5780,.T.);
#48126=EDGE_CURVE('',#38169,#38166,#5781,.T.);
#48127=EDGE_CURVE('',#38171,#38172,#5782,.T.);
#48128=EDGE_CURVE('',#38173,#38172,#5783,.T.);
#48129=EDGE_CURVE('',#38174,#38173,#5784,.T.);
#48130=EDGE_CURVE('',#38174,#38171,#5785,.T.);
#48131=EDGE_CURVE('',#38175,#38176,#5786,.T.);
#48132=EDGE_CURVE('',#38172,#38176,#5787,.T.);
#48133=EDGE_CURVE('',#38171,#38175,#5788,.T.);
#48134=EDGE_CURVE('',#38177,#38178,#5789,.T.);
#48135=EDGE_CURVE('',#38176,#38178,#5790,.T.);
#48136=EDGE_CURVE('',#38175,#38177,#5791,.T.);
#48137=EDGE_CURVE('',#38178,#38173,#5792,.T.);
#48138=EDGE_CURVE('',#38177,#38174,#5793,.T.);
#48139=EDGE_CURVE('',#38179,#38180,#5794,.T.);
#48140=EDGE_CURVE('',#38181,#38180,#5795,.T.);
#48141=EDGE_CURVE('',#38182,#38181,#5796,.T.);
#48142=EDGE_CURVE('',#38182,#38179,#5797,.T.);
#48143=EDGE_CURVE('',#38183,#38184,#5798,.T.);
#48144=EDGE_CURVE('',#38180,#38184,#5799,.T.);
#48145=EDGE_CURVE('',#38179,#38183,#5800,.T.);
#48146=EDGE_CURVE('',#38185,#38186,#5801,.T.);
#48147=EDGE_CURVE('',#38184,#38186,#5802,.T.);
#48148=EDGE_CURVE('',#38183,#38185,#5803,.T.);
#48149=EDGE_CURVE('',#38186,#38181,#5804,.T.);
#48150=EDGE_CURVE('',#38185,#38182,#5805,.T.);
#48151=EDGE_CURVE('',#38187,#38188,#5806,.T.);
#48152=EDGE_CURVE('',#38189,#38188,#5807,.T.);
#48153=EDGE_CURVE('',#38190,#38189,#5808,.T.);
#48154=EDGE_CURVE('',#38190,#38187,#5809,.T.);
#48155=EDGE_CURVE('',#38191,#38192,#5810,.T.);
#48156=EDGE_CURVE('',#38188,#38192,#5811,.T.);
#48157=EDGE_CURVE('',#38187,#38191,#5812,.T.);
#48158=EDGE_CURVE('',#38193,#38194,#5813,.T.);
#48159=EDGE_CURVE('',#38192,#38194,#5814,.T.);
#48160=EDGE_CURVE('',#38191,#38193,#5815,.T.);
#48161=EDGE_CURVE('',#38194,#38189,#5816,.T.);
#48162=EDGE_CURVE('',#38193,#38190,#5817,.T.);
#48163=EDGE_CURVE('',#38195,#38196,#5818,.T.);
#48164=EDGE_CURVE('',#38197,#38196,#5819,.T.);
#48165=EDGE_CURVE('',#38198,#38197,#5820,.T.);
#48166=EDGE_CURVE('',#38198,#38195,#5821,.T.);
#48167=EDGE_CURVE('',#38199,#38200,#5822,.T.);
#48168=EDGE_CURVE('',#38196,#38200,#5823,.T.);
#48169=EDGE_CURVE('',#38195,#38199,#5824,.T.);
#48170=EDGE_CURVE('',#38201,#38202,#5825,.T.);
#48171=EDGE_CURVE('',#38200,#38202,#5826,.T.);
#48172=EDGE_CURVE('',#38199,#38201,#5827,.T.);
#48173=EDGE_CURVE('',#38202,#38197,#5828,.T.);
#48174=EDGE_CURVE('',#38201,#38198,#5829,.T.);
#48175=EDGE_CURVE('',#38203,#38204,#5830,.T.);
#48176=EDGE_CURVE('',#38205,#38204,#5831,.T.);
#48177=EDGE_CURVE('',#38206,#38205,#5832,.T.);
#48178=EDGE_CURVE('',#38206,#38203,#5833,.T.);
#48179=EDGE_CURVE('',#38207,#38208,#5834,.T.);
#48180=EDGE_CURVE('',#38204,#38208,#5835,.T.);
#48181=EDGE_CURVE('',#38203,#38207,#5836,.T.);
#48182=EDGE_CURVE('',#38209,#38210,#5837,.T.);
#48183=EDGE_CURVE('',#38208,#38210,#5838,.T.);
#48184=EDGE_CURVE('',#38207,#38209,#5839,.T.);
#48185=EDGE_CURVE('',#38210,#38205,#5840,.T.);
#48186=EDGE_CURVE('',#38209,#38206,#5841,.T.);
#48187=EDGE_CURVE('',#38211,#38212,#5842,.T.);
#48188=EDGE_CURVE('',#38213,#38212,#5843,.T.);
#48189=EDGE_CURVE('',#38214,#38213,#5844,.T.);
#48190=EDGE_CURVE('',#38214,#38211,#5845,.T.);
#48191=EDGE_CURVE('',#38215,#38216,#5846,.T.);
#48192=EDGE_CURVE('',#38212,#38216,#5847,.T.);
#48193=EDGE_CURVE('',#38211,#38215,#5848,.T.);
#48194=EDGE_CURVE('',#38217,#38218,#5849,.T.);
#48195=EDGE_CURVE('',#38216,#38218,#5850,.T.);
#48196=EDGE_CURVE('',#38215,#38217,#5851,.T.);
#48197=EDGE_CURVE('',#38218,#38213,#5852,.T.);
#48198=EDGE_CURVE('',#38217,#38214,#5853,.T.);
#48199=EDGE_CURVE('',#38219,#38220,#5854,.T.);
#48200=EDGE_CURVE('',#38221,#38220,#5855,.T.);
#48201=EDGE_CURVE('',#38222,#38221,#5856,.T.);
#48202=EDGE_CURVE('',#38222,#38219,#5857,.T.);
#48203=EDGE_CURVE('',#38223,#38224,#5858,.T.);
#48204=EDGE_CURVE('',#38220,#38224,#5859,.T.);
#48205=EDGE_CURVE('',#38219,#38223,#5860,.T.);
#48206=EDGE_CURVE('',#38225,#38226,#5861,.T.);
#48207=EDGE_CURVE('',#38224,#38226,#5862,.T.);
#48208=EDGE_CURVE('',#38223,#38225,#5863,.T.);
#48209=EDGE_CURVE('',#38226,#38221,#5864,.T.);
#48210=EDGE_CURVE('',#38225,#38222,#5865,.T.);
#48211=EDGE_CURVE('',#38227,#38228,#5866,.T.);
#48212=EDGE_CURVE('',#38229,#38228,#5867,.T.);
#48213=EDGE_CURVE('',#38230,#38229,#5868,.T.);
#48214=EDGE_CURVE('',#38230,#38227,#5869,.T.);
#48215=EDGE_CURVE('',#38231,#38232,#5870,.T.);
#48216=EDGE_CURVE('',#38228,#38232,#5871,.T.);
#48217=EDGE_CURVE('',#38227,#38231,#5872,.T.);
#48218=EDGE_CURVE('',#38233,#38234,#5873,.T.);
#48219=EDGE_CURVE('',#38232,#38234,#5874,.T.);
#48220=EDGE_CURVE('',#38231,#38233,#5875,.T.);
#48221=EDGE_CURVE('',#38234,#38229,#5876,.T.);
#48222=EDGE_CURVE('',#38233,#38230,#5877,.T.);
#48223=EDGE_CURVE('',#38235,#38236,#5878,.T.);
#48224=EDGE_CURVE('',#38237,#38236,#5879,.T.);
#48225=EDGE_CURVE('',#38238,#38237,#5880,.T.);
#48226=EDGE_CURVE('',#38238,#38235,#5881,.T.);
#48227=EDGE_CURVE('',#38239,#38240,#5882,.T.);
#48228=EDGE_CURVE('',#38236,#38240,#5883,.T.);
#48229=EDGE_CURVE('',#38235,#38239,#5884,.T.);
#48230=EDGE_CURVE('',#38241,#38242,#5885,.T.);
#48231=EDGE_CURVE('',#38240,#38242,#5886,.T.);
#48232=EDGE_CURVE('',#38239,#38241,#5887,.T.);
#48233=EDGE_CURVE('',#38242,#38237,#5888,.T.);
#48234=EDGE_CURVE('',#38241,#38238,#5889,.T.);
#48235=EDGE_CURVE('',#38243,#38244,#5890,.T.);
#48236=EDGE_CURVE('',#38245,#38244,#5891,.T.);
#48237=EDGE_CURVE('',#38246,#38245,#5892,.T.);
#48238=EDGE_CURVE('',#38246,#38243,#5893,.T.);
#48239=EDGE_CURVE('',#38247,#38248,#5894,.T.);
#48240=EDGE_CURVE('',#38244,#38248,#5895,.T.);
#48241=EDGE_CURVE('',#38243,#38247,#5896,.T.);
#48242=EDGE_CURVE('',#38249,#38250,#5897,.T.);
#48243=EDGE_CURVE('',#38248,#38250,#5898,.T.);
#48244=EDGE_CURVE('',#38247,#38249,#5899,.T.);
#48245=EDGE_CURVE('',#38250,#38245,#5900,.T.);
#48246=EDGE_CURVE('',#38249,#38246,#5901,.T.);
#48247=EDGE_CURVE('',#38251,#38252,#5902,.T.);
#48248=EDGE_CURVE('',#38253,#38252,#5903,.T.);
#48249=EDGE_CURVE('',#38254,#38253,#5904,.T.);
#48250=EDGE_CURVE('',#38254,#38251,#5905,.T.);
#48251=EDGE_CURVE('',#38255,#38256,#5906,.T.);
#48252=EDGE_CURVE('',#38252,#38256,#5907,.T.);
#48253=EDGE_CURVE('',#38251,#38255,#5908,.T.);
#48254=EDGE_CURVE('',#38257,#38258,#5909,.T.);
#48255=EDGE_CURVE('',#38256,#38258,#5910,.T.);
#48256=EDGE_CURVE('',#38255,#38257,#5911,.T.);
#48257=EDGE_CURVE('',#38258,#38253,#5912,.T.);
#48258=EDGE_CURVE('',#38257,#38254,#5913,.T.);
#48259=EDGE_CURVE('',#38259,#38260,#5914,.T.);
#48260=EDGE_CURVE('',#38261,#38260,#5915,.T.);
#48261=EDGE_CURVE('',#38262,#38261,#5916,.T.);
#48262=EDGE_CURVE('',#38262,#38259,#5917,.T.);
#48263=EDGE_CURVE('',#38263,#38264,#5918,.T.);
#48264=EDGE_CURVE('',#38260,#38264,#5919,.T.);
#48265=EDGE_CURVE('',#38259,#38263,#5920,.T.);
#48266=EDGE_CURVE('',#38265,#38266,#5921,.T.);
#48267=EDGE_CURVE('',#38264,#38266,#5922,.T.);
#48268=EDGE_CURVE('',#38263,#38265,#5923,.T.);
#48269=EDGE_CURVE('',#38266,#38261,#5924,.T.);
#48270=EDGE_CURVE('',#38265,#38262,#5925,.T.);
#48271=EDGE_CURVE('',#38267,#38268,#5926,.T.);
#48272=EDGE_CURVE('',#38269,#38268,#5927,.T.);
#48273=EDGE_CURVE('',#38270,#38269,#5928,.T.);
#48274=EDGE_CURVE('',#38270,#38267,#5929,.T.);
#48275=EDGE_CURVE('',#38271,#38272,#5930,.T.);
#48276=EDGE_CURVE('',#38268,#38272,#5931,.T.);
#48277=EDGE_CURVE('',#38267,#38271,#5932,.T.);
#48278=EDGE_CURVE('',#38273,#38274,#5933,.T.);
#48279=EDGE_CURVE('',#38272,#38274,#5934,.T.);
#48280=EDGE_CURVE('',#38271,#38273,#5935,.T.);
#48281=EDGE_CURVE('',#38274,#38269,#5936,.T.);
#48282=EDGE_CURVE('',#38273,#38270,#5937,.T.);
#48283=EDGE_CURVE('',#38275,#38276,#5938,.T.);
#48284=EDGE_CURVE('',#38277,#38276,#5939,.T.);
#48285=EDGE_CURVE('',#38278,#38277,#5940,.T.);
#48286=EDGE_CURVE('',#38278,#38275,#5941,.T.);
#48287=EDGE_CURVE('',#38279,#38280,#5942,.T.);
#48288=EDGE_CURVE('',#38276,#38280,#5943,.T.);
#48289=EDGE_CURVE('',#38275,#38279,#5944,.T.);
#48290=EDGE_CURVE('',#38281,#38282,#5945,.T.);
#48291=EDGE_CURVE('',#38280,#38282,#5946,.T.);
#48292=EDGE_CURVE('',#38279,#38281,#5947,.T.);
#48293=EDGE_CURVE('',#38282,#38277,#5948,.T.);
#48294=EDGE_CURVE('',#38281,#38278,#5949,.T.);
#48295=EDGE_CURVE('',#38283,#38284,#5950,.T.);
#48296=EDGE_CURVE('',#38285,#38284,#5951,.T.);
#48297=EDGE_CURVE('',#38286,#38285,#5952,.T.);
#48298=EDGE_CURVE('',#38286,#38283,#5953,.T.);
#48299=EDGE_CURVE('',#38287,#38288,#5954,.T.);
#48300=EDGE_CURVE('',#38284,#38288,#5955,.T.);
#48301=EDGE_CURVE('',#38283,#38287,#5956,.T.);
#48302=EDGE_CURVE('',#38289,#38290,#5957,.T.);
#48303=EDGE_CURVE('',#38288,#38290,#5958,.T.);
#48304=EDGE_CURVE('',#38287,#38289,#5959,.T.);
#48305=EDGE_CURVE('',#38290,#38285,#5960,.T.);
#48306=EDGE_CURVE('',#38289,#38286,#5961,.T.);
#48307=EDGE_CURVE('',#38291,#38292,#5962,.T.);
#48308=EDGE_CURVE('',#38293,#38292,#5963,.T.);
#48309=EDGE_CURVE('',#38294,#38293,#5964,.T.);
#48310=EDGE_CURVE('',#38294,#38291,#5965,.T.);
#48311=EDGE_CURVE('',#38295,#38296,#5966,.T.);
#48312=EDGE_CURVE('',#38292,#38296,#5967,.T.);
#48313=EDGE_CURVE('',#38291,#38295,#5968,.T.);
#48314=EDGE_CURVE('',#38297,#38298,#5969,.T.);
#48315=EDGE_CURVE('',#38296,#38298,#5970,.T.);
#48316=EDGE_CURVE('',#38295,#38297,#5971,.T.);
#48317=EDGE_CURVE('',#38298,#38293,#5972,.T.);
#48318=EDGE_CURVE('',#38297,#38294,#5973,.T.);
#48319=EDGE_CURVE('',#38299,#38300,#5974,.T.);
#48320=EDGE_CURVE('',#38301,#38300,#5975,.T.);
#48321=EDGE_CURVE('',#38302,#38301,#5976,.T.);
#48322=EDGE_CURVE('',#38302,#38299,#5977,.T.);
#48323=EDGE_CURVE('',#38303,#38304,#5978,.T.);
#48324=EDGE_CURVE('',#38300,#38304,#5979,.T.);
#48325=EDGE_CURVE('',#38299,#38303,#5980,.T.);
#48326=EDGE_CURVE('',#38305,#38306,#5981,.T.);
#48327=EDGE_CURVE('',#38304,#38306,#5982,.T.);
#48328=EDGE_CURVE('',#38303,#38305,#5983,.T.);
#48329=EDGE_CURVE('',#38306,#38301,#5984,.T.);
#48330=EDGE_CURVE('',#38305,#38302,#5985,.T.);
#48331=EDGE_CURVE('',#38307,#38308,#5986,.T.);
#48332=EDGE_CURVE('',#38309,#38308,#5987,.T.);
#48333=EDGE_CURVE('',#38310,#38309,#5988,.T.);
#48334=EDGE_CURVE('',#38310,#38307,#5989,.T.);
#48335=EDGE_CURVE('',#38311,#38312,#5990,.T.);
#48336=EDGE_CURVE('',#38308,#38312,#5991,.T.);
#48337=EDGE_CURVE('',#38307,#38311,#5992,.T.);
#48338=EDGE_CURVE('',#38313,#38314,#5993,.T.);
#48339=EDGE_CURVE('',#38312,#38314,#5994,.T.);
#48340=EDGE_CURVE('',#38311,#38313,#5995,.T.);
#48341=EDGE_CURVE('',#38314,#38309,#5996,.T.);
#48342=EDGE_CURVE('',#38313,#38310,#5997,.T.);
#48343=EDGE_CURVE('',#38315,#38316,#5998,.T.);
#48344=EDGE_CURVE('',#38317,#38316,#5999,.T.);
#48345=EDGE_CURVE('',#38318,#38317,#6000,.T.);
#48346=EDGE_CURVE('',#38318,#38315,#6001,.T.);
#48347=EDGE_CURVE('',#38319,#38320,#6002,.T.);
#48348=EDGE_CURVE('',#38316,#38320,#6003,.T.);
#48349=EDGE_CURVE('',#38315,#38319,#6004,.T.);
#48350=EDGE_CURVE('',#38321,#38322,#6005,.T.);
#48351=EDGE_CURVE('',#38320,#38322,#6006,.T.);
#48352=EDGE_CURVE('',#38319,#38321,#6007,.T.);
#48353=EDGE_CURVE('',#38322,#38317,#6008,.T.);
#48354=EDGE_CURVE('',#38321,#38318,#6009,.T.);
#48355=EDGE_CURVE('',#38323,#38324,#6010,.T.);
#48356=EDGE_CURVE('',#38325,#38324,#6011,.T.);
#48357=EDGE_CURVE('',#38326,#38325,#6012,.T.);
#48358=EDGE_CURVE('',#38326,#38323,#6013,.T.);
#48359=EDGE_CURVE('',#38327,#38328,#6014,.T.);
#48360=EDGE_CURVE('',#38324,#38328,#6015,.T.);
#48361=EDGE_CURVE('',#38323,#38327,#6016,.T.);
#48362=EDGE_CURVE('',#38329,#38330,#6017,.T.);
#48363=EDGE_CURVE('',#38328,#38330,#6018,.T.);
#48364=EDGE_CURVE('',#38327,#38329,#6019,.T.);
#48365=EDGE_CURVE('',#38330,#38325,#6020,.T.);
#48366=EDGE_CURVE('',#38329,#38326,#6021,.T.);
#48367=EDGE_CURVE('',#38331,#38332,#6022,.T.);
#48368=EDGE_CURVE('',#38333,#38332,#6023,.T.);
#48369=EDGE_CURVE('',#38334,#38333,#6024,.T.);
#48370=EDGE_CURVE('',#38334,#38331,#6025,.T.);
#48371=EDGE_CURVE('',#38335,#38336,#6026,.T.);
#48372=EDGE_CURVE('',#38332,#38336,#6027,.T.);
#48373=EDGE_CURVE('',#38331,#38335,#6028,.T.);
#48374=EDGE_CURVE('',#38337,#38338,#6029,.T.);
#48375=EDGE_CURVE('',#38336,#38338,#6030,.T.);
#48376=EDGE_CURVE('',#38335,#38337,#6031,.T.);
#48377=EDGE_CURVE('',#38338,#38333,#6032,.T.);
#48378=EDGE_CURVE('',#38337,#38334,#6033,.T.);
#48379=EDGE_CURVE('',#38339,#38340,#6034,.T.);
#48380=EDGE_CURVE('',#38341,#38340,#6035,.T.);
#48381=EDGE_CURVE('',#38342,#38341,#6036,.T.);
#48382=EDGE_CURVE('',#38342,#38339,#6037,.T.);
#48383=EDGE_CURVE('',#38343,#38344,#6038,.T.);
#48384=EDGE_CURVE('',#38340,#38344,#6039,.T.);
#48385=EDGE_CURVE('',#38339,#38343,#6040,.T.);
#48386=EDGE_CURVE('',#38345,#38346,#6041,.T.);
#48387=EDGE_CURVE('',#38344,#38346,#6042,.T.);
#48388=EDGE_CURVE('',#38343,#38345,#6043,.T.);
#48389=EDGE_CURVE('',#38346,#38341,#6044,.T.);
#48390=EDGE_CURVE('',#38345,#38342,#6045,.T.);
#48391=EDGE_CURVE('',#38347,#38348,#6046,.T.);
#48392=EDGE_CURVE('',#38349,#38348,#6047,.T.);
#48393=EDGE_CURVE('',#38350,#38349,#6048,.T.);
#48394=EDGE_CURVE('',#38350,#38347,#6049,.T.);
#48395=EDGE_CURVE('',#38351,#38352,#6050,.T.);
#48396=EDGE_CURVE('',#38348,#38352,#6051,.T.);
#48397=EDGE_CURVE('',#38347,#38351,#6052,.T.);
#48398=EDGE_CURVE('',#38353,#38354,#6053,.T.);
#48399=EDGE_CURVE('',#38352,#38354,#6054,.T.);
#48400=EDGE_CURVE('',#38351,#38353,#6055,.T.);
#48401=EDGE_CURVE('',#38354,#38349,#6056,.T.);
#48402=EDGE_CURVE('',#38353,#38350,#6057,.T.);
#48403=EDGE_CURVE('',#38355,#38356,#6058,.T.);
#48404=EDGE_CURVE('',#38357,#38356,#6059,.T.);
#48405=EDGE_CURVE('',#38358,#38357,#6060,.T.);
#48406=EDGE_CURVE('',#38358,#38355,#6061,.T.);
#48407=EDGE_CURVE('',#38359,#38360,#6062,.T.);
#48408=EDGE_CURVE('',#38356,#38360,#6063,.T.);
#48409=EDGE_CURVE('',#38355,#38359,#6064,.T.);
#48410=EDGE_CURVE('',#38361,#38362,#6065,.T.);
#48411=EDGE_CURVE('',#38360,#38362,#6066,.T.);
#48412=EDGE_CURVE('',#38359,#38361,#6067,.T.);
#48413=EDGE_CURVE('',#38362,#38357,#6068,.T.);
#48414=EDGE_CURVE('',#38361,#38358,#6069,.T.);
#48415=EDGE_CURVE('',#38363,#38364,#6070,.T.);
#48416=EDGE_CURVE('',#38365,#38364,#6071,.T.);
#48417=EDGE_CURVE('',#38366,#38365,#6072,.T.);
#48418=EDGE_CURVE('',#38366,#38363,#6073,.T.);
#48419=EDGE_CURVE('',#38367,#38368,#6074,.T.);
#48420=EDGE_CURVE('',#38364,#38368,#6075,.T.);
#48421=EDGE_CURVE('',#38363,#38367,#6076,.T.);
#48422=EDGE_CURVE('',#38369,#38370,#6077,.T.);
#48423=EDGE_CURVE('',#38368,#38370,#6078,.T.);
#48424=EDGE_CURVE('',#38367,#38369,#6079,.T.);
#48425=EDGE_CURVE('',#38370,#38365,#6080,.T.);
#48426=EDGE_CURVE('',#38369,#38366,#6081,.T.);
#48427=EDGE_CURVE('',#38371,#38372,#6082,.T.);
#48428=EDGE_CURVE('',#38373,#38372,#6083,.T.);
#48429=EDGE_CURVE('',#38374,#38373,#6084,.T.);
#48430=EDGE_CURVE('',#38374,#38371,#6085,.T.);
#48431=EDGE_CURVE('',#38375,#38376,#6086,.T.);
#48432=EDGE_CURVE('',#38372,#38376,#6087,.T.);
#48433=EDGE_CURVE('',#38371,#38375,#6088,.T.);
#48434=EDGE_CURVE('',#38377,#38378,#6089,.T.);
#48435=EDGE_CURVE('',#38376,#38378,#6090,.T.);
#48436=EDGE_CURVE('',#38375,#38377,#6091,.T.);
#48437=EDGE_CURVE('',#38378,#38373,#6092,.T.);
#48438=EDGE_CURVE('',#38377,#38374,#6093,.T.);
#48439=EDGE_CURVE('',#38379,#38380,#6094,.T.);
#48440=EDGE_CURVE('',#38381,#38380,#6095,.T.);
#48441=EDGE_CURVE('',#38382,#38381,#6096,.T.);
#48442=EDGE_CURVE('',#38382,#38379,#6097,.T.);
#48443=EDGE_CURVE('',#38383,#38384,#6098,.T.);
#48444=EDGE_CURVE('',#38380,#38384,#6099,.T.);
#48445=EDGE_CURVE('',#38379,#38383,#6100,.T.);
#48446=EDGE_CURVE('',#38385,#38386,#6101,.T.);
#48447=EDGE_CURVE('',#38384,#38386,#6102,.T.);
#48448=EDGE_CURVE('',#38383,#38385,#6103,.T.);
#48449=EDGE_CURVE('',#38386,#38381,#6104,.T.);
#48450=EDGE_CURVE('',#38385,#38382,#6105,.T.);
#48451=EDGE_CURVE('',#38387,#38388,#6106,.T.);
#48452=EDGE_CURVE('',#38389,#38388,#6107,.T.);
#48453=EDGE_CURVE('',#38390,#38389,#6108,.T.);
#48454=EDGE_CURVE('',#38390,#38387,#6109,.T.);
#48455=EDGE_CURVE('',#38391,#38392,#6110,.T.);
#48456=EDGE_CURVE('',#38388,#38392,#6111,.T.);
#48457=EDGE_CURVE('',#38387,#38391,#6112,.T.);
#48458=EDGE_CURVE('',#38393,#38394,#6113,.T.);
#48459=EDGE_CURVE('',#38392,#38394,#6114,.T.);
#48460=EDGE_CURVE('',#38391,#38393,#6115,.T.);
#48461=EDGE_CURVE('',#38394,#38389,#6116,.T.);
#48462=EDGE_CURVE('',#38393,#38390,#6117,.T.);
#48463=EDGE_CURVE('',#38395,#38396,#6118,.T.);
#48464=EDGE_CURVE('',#38397,#38396,#6119,.T.);
#48465=EDGE_CURVE('',#38398,#38397,#6120,.T.);
#48466=EDGE_CURVE('',#38398,#38395,#6121,.T.);
#48467=EDGE_CURVE('',#38399,#38400,#6122,.T.);
#48468=EDGE_CURVE('',#38396,#38400,#6123,.T.);
#48469=EDGE_CURVE('',#38395,#38399,#6124,.T.);
#48470=EDGE_CURVE('',#38401,#38402,#6125,.T.);
#48471=EDGE_CURVE('',#38400,#38402,#6126,.T.);
#48472=EDGE_CURVE('',#38399,#38401,#6127,.T.);
#48473=EDGE_CURVE('',#38402,#38397,#6128,.T.);
#48474=EDGE_CURVE('',#38401,#38398,#6129,.T.);
#48475=EDGE_CURVE('',#38403,#38404,#6130,.T.);
#48476=EDGE_CURVE('',#38405,#38404,#6131,.T.);
#48477=EDGE_CURVE('',#38406,#38405,#6132,.T.);
#48478=EDGE_CURVE('',#38406,#38403,#6133,.T.);
#48479=EDGE_CURVE('',#38407,#38408,#6134,.T.);
#48480=EDGE_CURVE('',#38404,#38408,#6135,.T.);
#48481=EDGE_CURVE('',#38403,#38407,#6136,.T.);
#48482=EDGE_CURVE('',#38409,#38410,#6137,.T.);
#48483=EDGE_CURVE('',#38408,#38410,#6138,.T.);
#48484=EDGE_CURVE('',#38407,#38409,#6139,.T.);
#48485=EDGE_CURVE('',#38410,#38405,#6140,.T.);
#48486=EDGE_CURVE('',#38409,#38406,#6141,.T.);
#48487=EDGE_CURVE('',#38411,#38412,#6142,.T.);
#48488=EDGE_CURVE('',#38413,#38412,#6143,.T.);
#48489=EDGE_CURVE('',#38414,#38413,#6144,.T.);
#48490=EDGE_CURVE('',#38414,#38411,#6145,.T.);
#48491=EDGE_CURVE('',#38415,#38416,#6146,.T.);
#48492=EDGE_CURVE('',#38412,#38416,#6147,.T.);
#48493=EDGE_CURVE('',#38411,#38415,#6148,.T.);
#48494=EDGE_CURVE('',#38417,#38418,#6149,.T.);
#48495=EDGE_CURVE('',#38416,#38418,#6150,.T.);
#48496=EDGE_CURVE('',#38415,#38417,#6151,.T.);
#48497=EDGE_CURVE('',#38418,#38413,#6152,.T.);
#48498=EDGE_CURVE('',#38417,#38414,#6153,.T.);
#48499=EDGE_CURVE('',#38419,#38420,#6154,.T.);
#48500=EDGE_CURVE('',#38421,#38420,#6155,.T.);
#48501=EDGE_CURVE('',#38422,#38421,#6156,.T.);
#48502=EDGE_CURVE('',#38422,#38419,#6157,.T.);
#48503=EDGE_CURVE('',#38423,#38424,#6158,.T.);
#48504=EDGE_CURVE('',#38420,#38424,#6159,.T.);
#48505=EDGE_CURVE('',#38419,#38423,#6160,.T.);
#48506=EDGE_CURVE('',#38425,#38426,#6161,.T.);
#48507=EDGE_CURVE('',#38424,#38426,#6162,.T.);
#48508=EDGE_CURVE('',#38423,#38425,#6163,.T.);
#48509=EDGE_CURVE('',#38426,#38421,#6164,.T.);
#48510=EDGE_CURVE('',#38425,#38422,#6165,.T.);
#48511=EDGE_CURVE('',#38427,#38428,#6166,.T.);
#48512=EDGE_CURVE('',#38429,#38428,#6167,.T.);
#48513=EDGE_CURVE('',#38430,#38429,#6168,.T.);
#48514=EDGE_CURVE('',#38430,#38427,#6169,.T.);
#48515=EDGE_CURVE('',#38431,#38432,#6170,.T.);
#48516=EDGE_CURVE('',#38428,#38432,#6171,.T.);
#48517=EDGE_CURVE('',#38427,#38431,#6172,.T.);
#48518=EDGE_CURVE('',#38433,#38434,#6173,.T.);
#48519=EDGE_CURVE('',#38432,#38434,#6174,.T.);
#48520=EDGE_CURVE('',#38431,#38433,#6175,.T.);
#48521=EDGE_CURVE('',#38434,#38429,#6176,.T.);
#48522=EDGE_CURVE('',#38433,#38430,#6177,.T.);
#48523=EDGE_CURVE('',#38435,#38436,#6178,.T.);
#48524=EDGE_CURVE('',#38437,#38436,#6179,.T.);
#48525=EDGE_CURVE('',#38438,#38437,#6180,.T.);
#48526=EDGE_CURVE('',#38438,#38435,#6181,.T.);
#48527=EDGE_CURVE('',#38439,#38440,#6182,.T.);
#48528=EDGE_CURVE('',#38436,#38440,#6183,.T.);
#48529=EDGE_CURVE('',#38435,#38439,#6184,.T.);
#48530=EDGE_CURVE('',#38441,#38442,#6185,.T.);
#48531=EDGE_CURVE('',#38440,#38442,#6186,.T.);
#48532=EDGE_CURVE('',#38439,#38441,#6187,.T.);
#48533=EDGE_CURVE('',#38442,#38437,#6188,.T.);
#48534=EDGE_CURVE('',#38441,#38438,#6189,.T.);
#48535=EDGE_CURVE('',#38443,#38444,#6190,.T.);
#48536=EDGE_CURVE('',#38445,#38444,#6191,.T.);
#48537=EDGE_CURVE('',#38446,#38445,#6192,.T.);
#48538=EDGE_CURVE('',#38446,#38443,#6193,.T.);
#48539=EDGE_CURVE('',#38447,#38448,#6194,.T.);
#48540=EDGE_CURVE('',#38444,#38448,#6195,.T.);
#48541=EDGE_CURVE('',#38443,#38447,#6196,.T.);
#48542=EDGE_CURVE('',#38449,#38450,#6197,.T.);
#48543=EDGE_CURVE('',#38448,#38450,#6198,.T.);
#48544=EDGE_CURVE('',#38447,#38449,#6199,.T.);
#48545=EDGE_CURVE('',#38450,#38445,#6200,.T.);
#48546=EDGE_CURVE('',#38449,#38446,#6201,.T.);
#48547=EDGE_CURVE('',#38451,#38452,#6202,.T.);
#48548=EDGE_CURVE('',#38453,#38452,#6203,.T.);
#48549=EDGE_CURVE('',#38454,#38453,#6204,.T.);
#48550=EDGE_CURVE('',#38454,#38451,#6205,.T.);
#48551=EDGE_CURVE('',#38455,#38456,#6206,.T.);
#48552=EDGE_CURVE('',#38452,#38456,#6207,.T.);
#48553=EDGE_CURVE('',#38451,#38455,#6208,.T.);
#48554=EDGE_CURVE('',#38457,#38458,#6209,.T.);
#48555=EDGE_CURVE('',#38456,#38458,#6210,.T.);
#48556=EDGE_CURVE('',#38455,#38457,#6211,.T.);
#48557=EDGE_CURVE('',#38458,#38453,#6212,.T.);
#48558=EDGE_CURVE('',#38457,#38454,#6213,.T.);
#48559=EDGE_CURVE('',#38459,#38460,#6214,.T.);
#48560=EDGE_CURVE('',#38461,#38460,#6215,.T.);
#48561=EDGE_CURVE('',#38462,#38461,#6216,.T.);
#48562=EDGE_CURVE('',#38462,#38459,#6217,.T.);
#48563=EDGE_CURVE('',#38463,#38464,#6218,.T.);
#48564=EDGE_CURVE('',#38460,#38464,#6219,.T.);
#48565=EDGE_CURVE('',#38459,#38463,#6220,.T.);
#48566=EDGE_CURVE('',#38465,#38466,#6221,.T.);
#48567=EDGE_CURVE('',#38464,#38466,#6222,.T.);
#48568=EDGE_CURVE('',#38463,#38465,#6223,.T.);
#48569=EDGE_CURVE('',#38466,#38461,#6224,.T.);
#48570=EDGE_CURVE('',#38465,#38462,#6225,.T.);
#48571=EDGE_CURVE('',#38467,#38468,#6226,.T.);
#48572=EDGE_CURVE('',#38469,#38468,#6227,.T.);
#48573=EDGE_CURVE('',#38470,#38469,#6228,.T.);
#48574=EDGE_CURVE('',#38470,#38467,#6229,.T.);
#48575=EDGE_CURVE('',#38471,#38472,#6230,.T.);
#48576=EDGE_CURVE('',#38468,#38472,#6231,.T.);
#48577=EDGE_CURVE('',#38467,#38471,#6232,.T.);
#48578=EDGE_CURVE('',#38473,#38474,#6233,.T.);
#48579=EDGE_CURVE('',#38472,#38474,#6234,.T.);
#48580=EDGE_CURVE('',#38471,#38473,#6235,.T.);
#48581=EDGE_CURVE('',#38474,#38469,#6236,.T.);
#48582=EDGE_CURVE('',#38473,#38470,#6237,.T.);
#48583=EDGE_CURVE('',#38475,#38476,#6238,.T.);
#48584=EDGE_CURVE('',#38477,#38476,#6239,.T.);
#48585=EDGE_CURVE('',#38478,#38477,#6240,.T.);
#48586=EDGE_CURVE('',#38478,#38475,#6241,.T.);
#48587=EDGE_CURVE('',#38479,#38480,#6242,.T.);
#48588=EDGE_CURVE('',#38476,#38480,#6243,.T.);
#48589=EDGE_CURVE('',#38475,#38479,#6244,.T.);
#48590=EDGE_CURVE('',#38481,#38482,#6245,.T.);
#48591=EDGE_CURVE('',#38480,#38482,#6246,.T.);
#48592=EDGE_CURVE('',#38479,#38481,#6247,.T.);
#48593=EDGE_CURVE('',#38482,#38477,#6248,.T.);
#48594=EDGE_CURVE('',#38481,#38478,#6249,.T.);
#48595=EDGE_CURVE('',#38483,#38484,#6250,.T.);
#48596=EDGE_CURVE('',#38485,#38484,#6251,.T.);
#48597=EDGE_CURVE('',#38486,#38485,#6252,.T.);
#48598=EDGE_CURVE('',#38486,#38483,#6253,.T.);
#48599=EDGE_CURVE('',#38487,#38488,#6254,.T.);
#48600=EDGE_CURVE('',#38484,#38488,#6255,.T.);
#48601=EDGE_CURVE('',#38483,#38487,#6256,.T.);
#48602=EDGE_CURVE('',#38489,#38490,#6257,.T.);
#48603=EDGE_CURVE('',#38488,#38490,#6258,.T.);
#48604=EDGE_CURVE('',#38487,#38489,#6259,.T.);
#48605=EDGE_CURVE('',#38490,#38485,#6260,.T.);
#48606=EDGE_CURVE('',#38489,#38486,#6261,.T.);
#48607=EDGE_CURVE('',#38491,#38492,#6262,.T.);
#48608=EDGE_CURVE('',#38493,#38492,#6263,.T.);
#48609=EDGE_CURVE('',#38494,#38493,#6264,.T.);
#48610=EDGE_CURVE('',#38494,#38491,#6265,.T.);
#48611=EDGE_CURVE('',#38495,#38496,#6266,.T.);
#48612=EDGE_CURVE('',#38492,#38496,#6267,.T.);
#48613=EDGE_CURVE('',#38491,#38495,#6268,.T.);
#48614=EDGE_CURVE('',#38497,#38498,#6269,.T.);
#48615=EDGE_CURVE('',#38496,#38498,#6270,.T.);
#48616=EDGE_CURVE('',#38495,#38497,#6271,.T.);
#48617=EDGE_CURVE('',#38498,#38493,#6272,.T.);
#48618=EDGE_CURVE('',#38497,#38494,#6273,.T.);
#48619=EDGE_CURVE('',#38499,#38500,#6274,.T.);
#48620=EDGE_CURVE('',#38501,#38500,#6275,.T.);
#48621=EDGE_CURVE('',#38502,#38501,#6276,.T.);
#48622=EDGE_CURVE('',#38502,#38499,#6277,.T.);
#48623=EDGE_CURVE('',#38503,#38504,#6278,.T.);
#48624=EDGE_CURVE('',#38500,#38504,#6279,.T.);
#48625=EDGE_CURVE('',#38499,#38503,#6280,.T.);
#48626=EDGE_CURVE('',#38505,#38506,#6281,.T.);
#48627=EDGE_CURVE('',#38504,#38506,#6282,.T.);
#48628=EDGE_CURVE('',#38503,#38505,#6283,.T.);
#48629=EDGE_CURVE('',#38506,#38501,#6284,.T.);
#48630=EDGE_CURVE('',#38505,#38502,#6285,.T.);
#48631=EDGE_CURVE('',#38507,#38508,#6286,.T.);
#48632=EDGE_CURVE('',#38509,#38508,#6287,.T.);
#48633=EDGE_CURVE('',#38510,#38509,#6288,.T.);
#48634=EDGE_CURVE('',#38510,#38507,#6289,.T.);
#48635=EDGE_CURVE('',#38511,#38512,#6290,.T.);
#48636=EDGE_CURVE('',#38508,#38512,#6291,.T.);
#48637=EDGE_CURVE('',#38507,#38511,#6292,.T.);
#48638=EDGE_CURVE('',#38513,#38514,#6293,.T.);
#48639=EDGE_CURVE('',#38512,#38514,#6294,.T.);
#48640=EDGE_CURVE('',#38511,#38513,#6295,.T.);
#48641=EDGE_CURVE('',#38514,#38509,#6296,.T.);
#48642=EDGE_CURVE('',#38513,#38510,#6297,.T.);
#48643=EDGE_CURVE('',#38515,#38516,#6298,.T.);
#48644=EDGE_CURVE('',#38517,#38516,#6299,.T.);
#48645=EDGE_CURVE('',#38518,#38517,#6300,.T.);
#48646=EDGE_CURVE('',#38518,#38515,#6301,.T.);
#48647=EDGE_CURVE('',#38519,#38520,#6302,.T.);
#48648=EDGE_CURVE('',#38516,#38520,#6303,.T.);
#48649=EDGE_CURVE('',#38515,#38519,#6304,.T.);
#48650=EDGE_CURVE('',#38521,#38522,#6305,.T.);
#48651=EDGE_CURVE('',#38520,#38522,#6306,.T.);
#48652=EDGE_CURVE('',#38519,#38521,#6307,.T.);
#48653=EDGE_CURVE('',#38522,#38517,#6308,.T.);
#48654=EDGE_CURVE('',#38521,#38518,#6309,.T.);
#48655=EDGE_CURVE('',#38523,#38524,#6310,.T.);
#48656=EDGE_CURVE('',#38525,#38524,#6311,.T.);
#48657=EDGE_CURVE('',#38526,#38525,#6312,.T.);
#48658=EDGE_CURVE('',#38526,#38523,#6313,.T.);
#48659=EDGE_CURVE('',#38527,#38528,#6314,.T.);
#48660=EDGE_CURVE('',#38524,#38528,#6315,.T.);
#48661=EDGE_CURVE('',#38523,#38527,#6316,.T.);
#48662=EDGE_CURVE('',#38529,#38530,#6317,.T.);
#48663=EDGE_CURVE('',#38528,#38530,#6318,.T.);
#48664=EDGE_CURVE('',#38527,#38529,#6319,.T.);
#48665=EDGE_CURVE('',#38530,#38525,#6320,.T.);
#48666=EDGE_CURVE('',#38529,#38526,#6321,.T.);
#48667=EDGE_CURVE('',#38531,#38532,#6322,.T.);
#48668=EDGE_CURVE('',#38533,#38532,#6323,.T.);
#48669=EDGE_CURVE('',#38534,#38533,#6324,.T.);
#48670=EDGE_CURVE('',#38534,#38531,#6325,.T.);
#48671=EDGE_CURVE('',#38535,#38536,#6326,.T.);
#48672=EDGE_CURVE('',#38532,#38536,#6327,.T.);
#48673=EDGE_CURVE('',#38531,#38535,#6328,.T.);
#48674=EDGE_CURVE('',#38537,#38538,#6329,.T.);
#48675=EDGE_CURVE('',#38536,#38538,#6330,.T.);
#48676=EDGE_CURVE('',#38535,#38537,#6331,.T.);
#48677=EDGE_CURVE('',#38538,#38533,#6332,.T.);
#48678=EDGE_CURVE('',#38537,#38534,#6333,.T.);
#48679=EDGE_CURVE('',#38539,#38540,#6334,.T.);
#48680=EDGE_CURVE('',#38541,#38540,#6335,.T.);
#48681=EDGE_CURVE('',#38542,#38541,#6336,.T.);
#48682=EDGE_CURVE('',#38542,#38539,#6337,.T.);
#48683=EDGE_CURVE('',#38543,#38544,#6338,.T.);
#48684=EDGE_CURVE('',#38540,#38544,#6339,.T.);
#48685=EDGE_CURVE('',#38539,#38543,#6340,.T.);
#48686=EDGE_CURVE('',#38545,#38546,#6341,.T.);
#48687=EDGE_CURVE('',#38544,#38546,#6342,.T.);
#48688=EDGE_CURVE('',#38543,#38545,#6343,.T.);
#48689=EDGE_CURVE('',#38546,#38541,#6344,.T.);
#48690=EDGE_CURVE('',#38545,#38542,#6345,.T.);
#48691=EDGE_CURVE('',#38547,#38548,#6346,.T.);
#48692=EDGE_CURVE('',#38549,#38548,#6347,.T.);
#48693=EDGE_CURVE('',#38550,#38549,#6348,.T.);
#48694=EDGE_CURVE('',#38550,#38547,#6349,.T.);
#48695=EDGE_CURVE('',#38551,#38552,#6350,.T.);
#48696=EDGE_CURVE('',#38548,#38552,#6351,.T.);
#48697=EDGE_CURVE('',#38547,#38551,#6352,.T.);
#48698=EDGE_CURVE('',#38553,#38554,#6353,.T.);
#48699=EDGE_CURVE('',#38552,#38554,#6354,.T.);
#48700=EDGE_CURVE('',#38551,#38553,#6355,.T.);
#48701=EDGE_CURVE('',#38554,#38549,#6356,.T.);
#48702=EDGE_CURVE('',#38553,#38550,#6357,.T.);
#48703=EDGE_CURVE('',#38555,#38556,#6358,.T.);
#48704=EDGE_CURVE('',#38557,#38556,#6359,.T.);
#48705=EDGE_CURVE('',#38558,#38557,#6360,.T.);
#48706=EDGE_CURVE('',#38558,#38555,#6361,.T.);
#48707=EDGE_CURVE('',#38559,#38560,#6362,.T.);
#48708=EDGE_CURVE('',#38556,#38560,#6363,.T.);
#48709=EDGE_CURVE('',#38555,#38559,#6364,.T.);
#48710=EDGE_CURVE('',#38561,#38562,#6365,.T.);
#48711=EDGE_CURVE('',#38560,#38562,#6366,.T.);
#48712=EDGE_CURVE('',#38559,#38561,#6367,.T.);
#48713=EDGE_CURVE('',#38562,#38557,#6368,.T.);
#48714=EDGE_CURVE('',#38561,#38558,#6369,.T.);
#48715=EDGE_CURVE('',#38563,#38564,#6370,.T.);
#48716=EDGE_CURVE('',#38565,#38564,#6371,.T.);
#48717=EDGE_CURVE('',#38566,#38565,#6372,.T.);
#48718=EDGE_CURVE('',#38566,#38563,#6373,.T.);
#48719=EDGE_CURVE('',#38567,#38568,#6374,.T.);
#48720=EDGE_CURVE('',#38564,#38568,#6375,.T.);
#48721=EDGE_CURVE('',#38563,#38567,#6376,.T.);
#48722=EDGE_CURVE('',#38569,#38570,#6377,.T.);
#48723=EDGE_CURVE('',#38568,#38570,#6378,.T.);
#48724=EDGE_CURVE('',#38567,#38569,#6379,.T.);
#48725=EDGE_CURVE('',#38570,#38565,#6380,.T.);
#48726=EDGE_CURVE('',#38569,#38566,#6381,.T.);
#48727=EDGE_CURVE('',#38571,#38572,#6382,.T.);
#48728=EDGE_CURVE('',#38573,#38572,#6383,.T.);
#48729=EDGE_CURVE('',#38574,#38573,#6384,.T.);
#48730=EDGE_CURVE('',#38574,#38571,#6385,.T.);
#48731=EDGE_CURVE('',#38575,#38576,#6386,.T.);
#48732=EDGE_CURVE('',#38572,#38576,#6387,.T.);
#48733=EDGE_CURVE('',#38571,#38575,#6388,.T.);
#48734=EDGE_CURVE('',#38577,#38578,#6389,.T.);
#48735=EDGE_CURVE('',#38576,#38578,#6390,.T.);
#48736=EDGE_CURVE('',#38575,#38577,#6391,.T.);
#48737=EDGE_CURVE('',#38578,#38573,#6392,.T.);
#48738=EDGE_CURVE('',#38577,#38574,#6393,.T.);
#48739=EDGE_CURVE('',#38579,#38580,#6394,.T.);
#48740=EDGE_CURVE('',#38581,#38580,#6395,.T.);
#48741=EDGE_CURVE('',#38582,#38581,#6396,.T.);
#48742=EDGE_CURVE('',#38582,#38579,#6397,.T.);
#48743=EDGE_CURVE('',#38583,#38584,#6398,.T.);
#48744=EDGE_CURVE('',#38580,#38584,#6399,.T.);
#48745=EDGE_CURVE('',#38579,#38583,#6400,.T.);
#48746=EDGE_CURVE('',#38585,#38586,#6401,.T.);
#48747=EDGE_CURVE('',#38584,#38586,#6402,.T.);
#48748=EDGE_CURVE('',#38583,#38585,#6403,.T.);
#48749=EDGE_CURVE('',#38586,#38581,#6404,.T.);
#48750=EDGE_CURVE('',#38585,#38582,#6405,.T.);
#48751=EDGE_CURVE('',#38587,#38588,#6406,.T.);
#48752=EDGE_CURVE('',#38589,#38588,#6407,.T.);
#48753=EDGE_CURVE('',#38590,#38589,#6408,.T.);
#48754=EDGE_CURVE('',#38590,#38587,#6409,.T.);
#48755=EDGE_CURVE('',#38591,#38592,#6410,.T.);
#48756=EDGE_CURVE('',#38588,#38592,#6411,.T.);
#48757=EDGE_CURVE('',#38587,#38591,#6412,.T.);
#48758=EDGE_CURVE('',#38593,#38594,#6413,.T.);
#48759=EDGE_CURVE('',#38592,#38594,#6414,.T.);
#48760=EDGE_CURVE('',#38591,#38593,#6415,.T.);
#48761=EDGE_CURVE('',#38594,#38589,#6416,.T.);
#48762=EDGE_CURVE('',#38593,#38590,#6417,.T.);
#48763=EDGE_CURVE('',#38595,#38596,#6418,.T.);
#48764=EDGE_CURVE('',#38597,#38596,#6419,.T.);
#48765=EDGE_CURVE('',#38598,#38597,#6420,.T.);
#48766=EDGE_CURVE('',#38598,#38595,#6421,.T.);
#48767=EDGE_CURVE('',#38599,#38600,#6422,.T.);
#48768=EDGE_CURVE('',#38596,#38600,#6423,.T.);
#48769=EDGE_CURVE('',#38595,#38599,#6424,.T.);
#48770=EDGE_CURVE('',#38601,#38602,#6425,.T.);
#48771=EDGE_CURVE('',#38600,#38602,#6426,.T.);
#48772=EDGE_CURVE('',#38599,#38601,#6427,.T.);
#48773=EDGE_CURVE('',#38602,#38597,#6428,.T.);
#48774=EDGE_CURVE('',#38601,#38598,#6429,.T.);
#48775=EDGE_CURVE('',#38603,#38604,#6430,.T.);
#48776=EDGE_CURVE('',#38605,#38604,#6431,.T.);
#48777=EDGE_CURVE('',#38606,#38605,#6432,.T.);
#48778=EDGE_CURVE('',#38606,#38603,#6433,.T.);
#48779=EDGE_CURVE('',#38607,#38608,#6434,.T.);
#48780=EDGE_CURVE('',#38604,#38608,#6435,.T.);
#48781=EDGE_CURVE('',#38603,#38607,#6436,.T.);
#48782=EDGE_CURVE('',#38609,#38610,#6437,.T.);
#48783=EDGE_CURVE('',#38608,#38610,#6438,.T.);
#48784=EDGE_CURVE('',#38607,#38609,#6439,.T.);
#48785=EDGE_CURVE('',#38610,#38605,#6440,.T.);
#48786=EDGE_CURVE('',#38609,#38606,#6441,.T.);
#48787=EDGE_CURVE('',#38611,#38612,#6442,.T.);
#48788=EDGE_CURVE('',#38613,#38612,#6443,.T.);
#48789=EDGE_CURVE('',#38614,#38613,#6444,.T.);
#48790=EDGE_CURVE('',#38614,#38611,#6445,.T.);
#48791=EDGE_CURVE('',#38615,#38616,#6446,.T.);
#48792=EDGE_CURVE('',#38612,#38616,#6447,.T.);
#48793=EDGE_CURVE('',#38611,#38615,#6448,.T.);
#48794=EDGE_CURVE('',#38617,#38618,#6449,.T.);
#48795=EDGE_CURVE('',#38616,#38618,#6450,.T.);
#48796=EDGE_CURVE('',#38615,#38617,#6451,.T.);
#48797=EDGE_CURVE('',#38618,#38613,#6452,.T.);
#48798=EDGE_CURVE('',#38617,#38614,#6453,.T.);
#48799=EDGE_CURVE('',#38619,#38620,#6454,.T.);
#48800=EDGE_CURVE('',#38621,#38620,#6455,.T.);
#48801=EDGE_CURVE('',#38622,#38621,#6456,.T.);
#48802=EDGE_CURVE('',#38622,#38619,#6457,.T.);
#48803=EDGE_CURVE('',#38623,#38624,#6458,.T.);
#48804=EDGE_CURVE('',#38620,#38624,#6459,.T.);
#48805=EDGE_CURVE('',#38619,#38623,#6460,.T.);
#48806=EDGE_CURVE('',#38625,#38626,#6461,.T.);
#48807=EDGE_CURVE('',#38624,#38626,#6462,.T.);
#48808=EDGE_CURVE('',#38623,#38625,#6463,.T.);
#48809=EDGE_CURVE('',#38626,#38621,#6464,.T.);
#48810=EDGE_CURVE('',#38625,#38622,#6465,.T.);
#48811=EDGE_CURVE('',#38627,#38628,#6466,.T.);
#48812=EDGE_CURVE('',#38629,#38628,#6467,.T.);
#48813=EDGE_CURVE('',#38630,#38629,#6468,.T.);
#48814=EDGE_CURVE('',#38630,#38627,#6469,.T.);
#48815=EDGE_CURVE('',#38631,#38632,#6470,.T.);
#48816=EDGE_CURVE('',#38628,#38632,#6471,.T.);
#48817=EDGE_CURVE('',#38627,#38631,#6472,.T.);
#48818=EDGE_CURVE('',#38633,#38634,#6473,.T.);
#48819=EDGE_CURVE('',#38632,#38634,#6474,.T.);
#48820=EDGE_CURVE('',#38631,#38633,#6475,.T.);
#48821=EDGE_CURVE('',#38634,#38629,#6476,.T.);
#48822=EDGE_CURVE('',#38633,#38630,#6477,.T.);
#48823=EDGE_CURVE('',#38635,#38636,#6478,.T.);
#48824=EDGE_CURVE('',#38637,#38636,#6479,.T.);
#48825=EDGE_CURVE('',#38638,#38637,#6480,.T.);
#48826=EDGE_CURVE('',#38638,#38635,#6481,.T.);
#48827=EDGE_CURVE('',#38639,#38640,#6482,.T.);
#48828=EDGE_CURVE('',#38636,#38640,#6483,.T.);
#48829=EDGE_CURVE('',#38635,#38639,#6484,.T.);
#48830=EDGE_CURVE('',#38641,#38642,#6485,.T.);
#48831=EDGE_CURVE('',#38640,#38642,#6486,.T.);
#48832=EDGE_CURVE('',#38639,#38641,#6487,.T.);
#48833=EDGE_CURVE('',#38642,#38637,#6488,.T.);
#48834=EDGE_CURVE('',#38641,#38638,#6489,.T.);
#48835=EDGE_CURVE('',#38643,#38644,#6490,.T.);
#48836=EDGE_CURVE('',#38645,#38644,#6491,.T.);
#48837=EDGE_CURVE('',#38646,#38645,#6492,.T.);
#48838=EDGE_CURVE('',#38646,#38643,#6493,.T.);
#48839=EDGE_CURVE('',#38647,#38648,#6494,.T.);
#48840=EDGE_CURVE('',#38644,#38648,#6495,.T.);
#48841=EDGE_CURVE('',#38643,#38647,#6496,.T.);
#48842=EDGE_CURVE('',#38649,#38650,#6497,.T.);
#48843=EDGE_CURVE('',#38648,#38650,#6498,.T.);
#48844=EDGE_CURVE('',#38647,#38649,#6499,.T.);
#48845=EDGE_CURVE('',#38650,#38645,#6500,.T.);
#48846=EDGE_CURVE('',#38649,#38646,#6501,.T.);
#48847=EDGE_CURVE('',#38651,#38652,#6502,.T.);
#48848=EDGE_CURVE('',#38653,#38652,#6503,.T.);
#48849=EDGE_CURVE('',#38654,#38653,#6504,.T.);
#48850=EDGE_CURVE('',#38654,#38651,#6505,.T.);
#48851=EDGE_CURVE('',#38655,#38656,#6506,.T.);
#48852=EDGE_CURVE('',#38652,#38656,#6507,.T.);
#48853=EDGE_CURVE('',#38651,#38655,#6508,.T.);
#48854=EDGE_CURVE('',#38657,#38658,#6509,.T.);
#48855=EDGE_CURVE('',#38656,#38658,#6510,.T.);
#48856=EDGE_CURVE('',#38655,#38657,#6511,.T.);
#48857=EDGE_CURVE('',#38658,#38653,#6512,.T.);
#48858=EDGE_CURVE('',#38657,#38654,#6513,.T.);
#48859=EDGE_CURVE('',#38659,#38660,#6514,.T.);
#48860=EDGE_CURVE('',#38661,#38660,#6515,.T.);
#48861=EDGE_CURVE('',#38662,#38661,#6516,.T.);
#48862=EDGE_CURVE('',#38662,#38659,#6517,.T.);
#48863=EDGE_CURVE('',#38663,#38664,#6518,.T.);
#48864=EDGE_CURVE('',#38660,#38664,#6519,.T.);
#48865=EDGE_CURVE('',#38659,#38663,#6520,.T.);
#48866=EDGE_CURVE('',#38665,#38666,#6521,.T.);
#48867=EDGE_CURVE('',#38664,#38666,#6522,.T.);
#48868=EDGE_CURVE('',#38663,#38665,#6523,.T.);
#48869=EDGE_CURVE('',#38666,#38661,#6524,.T.);
#48870=EDGE_CURVE('',#38665,#38662,#6525,.T.);
#48871=EDGE_CURVE('',#38667,#38668,#6526,.T.);
#48872=EDGE_CURVE('',#38669,#38668,#6527,.T.);
#48873=EDGE_CURVE('',#38670,#38669,#6528,.T.);
#48874=EDGE_CURVE('',#38670,#38667,#6529,.T.);
#48875=EDGE_CURVE('',#38671,#38672,#6530,.T.);
#48876=EDGE_CURVE('',#38668,#38672,#6531,.T.);
#48877=EDGE_CURVE('',#38667,#38671,#6532,.T.);
#48878=EDGE_CURVE('',#38673,#38674,#6533,.T.);
#48879=EDGE_CURVE('',#38672,#38674,#6534,.T.);
#48880=EDGE_CURVE('',#38671,#38673,#6535,.T.);
#48881=EDGE_CURVE('',#38674,#38669,#6536,.T.);
#48882=EDGE_CURVE('',#38673,#38670,#6537,.T.);
#48883=EDGE_CURVE('',#38675,#38676,#6538,.T.);
#48884=EDGE_CURVE('',#38677,#38676,#6539,.T.);
#48885=EDGE_CURVE('',#38678,#38677,#6540,.T.);
#48886=EDGE_CURVE('',#38678,#38675,#6541,.T.);
#48887=EDGE_CURVE('',#38679,#38680,#6542,.T.);
#48888=EDGE_CURVE('',#38676,#38680,#6543,.T.);
#48889=EDGE_CURVE('',#38675,#38679,#6544,.T.);
#48890=EDGE_CURVE('',#38681,#38682,#6545,.T.);
#48891=EDGE_CURVE('',#38680,#38682,#6546,.T.);
#48892=EDGE_CURVE('',#38679,#38681,#6547,.T.);
#48893=EDGE_CURVE('',#38682,#38677,#6548,.T.);
#48894=EDGE_CURVE('',#38681,#38678,#6549,.T.);
#48895=EDGE_CURVE('',#38683,#38684,#6550,.T.);
#48896=EDGE_CURVE('',#38685,#38684,#6551,.T.);
#48897=EDGE_CURVE('',#38686,#38685,#6552,.T.);
#48898=EDGE_CURVE('',#38686,#38683,#6553,.T.);
#48899=EDGE_CURVE('',#38687,#38688,#6554,.T.);
#48900=EDGE_CURVE('',#38684,#38688,#6555,.T.);
#48901=EDGE_CURVE('',#38683,#38687,#6556,.T.);
#48902=EDGE_CURVE('',#38689,#38690,#6557,.T.);
#48903=EDGE_CURVE('',#38688,#38690,#6558,.T.);
#48904=EDGE_CURVE('',#38687,#38689,#6559,.T.);
#48905=EDGE_CURVE('',#38690,#38685,#6560,.T.);
#48906=EDGE_CURVE('',#38689,#38686,#6561,.T.);
#48907=EDGE_CURVE('',#38691,#38692,#6562,.T.);
#48908=EDGE_CURVE('',#38693,#38692,#6563,.T.);
#48909=EDGE_CURVE('',#38694,#38693,#6564,.T.);
#48910=EDGE_CURVE('',#38694,#38691,#6565,.T.);
#48911=EDGE_CURVE('',#38695,#38696,#6566,.T.);
#48912=EDGE_CURVE('',#38692,#38696,#6567,.T.);
#48913=EDGE_CURVE('',#38691,#38695,#6568,.T.);
#48914=EDGE_CURVE('',#38697,#38698,#6569,.T.);
#48915=EDGE_CURVE('',#38696,#38698,#6570,.T.);
#48916=EDGE_CURVE('',#38695,#38697,#6571,.T.);
#48917=EDGE_CURVE('',#38698,#38693,#6572,.T.);
#48918=EDGE_CURVE('',#38697,#38694,#6573,.T.);
#48919=EDGE_CURVE('',#38699,#38700,#6574,.T.);
#48920=EDGE_CURVE('',#38701,#38700,#6575,.T.);
#48921=EDGE_CURVE('',#38702,#38701,#6576,.T.);
#48922=EDGE_CURVE('',#38702,#38699,#6577,.T.);
#48923=EDGE_CURVE('',#38703,#38704,#6578,.T.);
#48924=EDGE_CURVE('',#38700,#38704,#6579,.T.);
#48925=EDGE_CURVE('',#38699,#38703,#6580,.T.);
#48926=EDGE_CURVE('',#38705,#38706,#6581,.T.);
#48927=EDGE_CURVE('',#38704,#38706,#6582,.T.);
#48928=EDGE_CURVE('',#38703,#38705,#6583,.T.);
#48929=EDGE_CURVE('',#38706,#38701,#6584,.T.);
#48930=EDGE_CURVE('',#38705,#38702,#6585,.T.);
#48931=EDGE_CURVE('',#38707,#38708,#6586,.T.);
#48932=EDGE_CURVE('',#38709,#38708,#6587,.T.);
#48933=EDGE_CURVE('',#38710,#38709,#6588,.T.);
#48934=EDGE_CURVE('',#38710,#38707,#6589,.T.);
#48935=EDGE_CURVE('',#38711,#38712,#6590,.T.);
#48936=EDGE_CURVE('',#38708,#38712,#6591,.T.);
#48937=EDGE_CURVE('',#38707,#38711,#6592,.T.);
#48938=EDGE_CURVE('',#38713,#38714,#6593,.T.);
#48939=EDGE_CURVE('',#38712,#38714,#6594,.T.);
#48940=EDGE_CURVE('',#38711,#38713,#6595,.T.);
#48941=EDGE_CURVE('',#38714,#38709,#6596,.T.);
#48942=EDGE_CURVE('',#38713,#38710,#6597,.T.);
#48943=EDGE_CURVE('',#38715,#38716,#6598,.T.);
#48944=EDGE_CURVE('',#38717,#38716,#6599,.T.);
#48945=EDGE_CURVE('',#38718,#38717,#6600,.T.);
#48946=EDGE_CURVE('',#38718,#38715,#6601,.T.);
#48947=EDGE_CURVE('',#38719,#38720,#6602,.T.);
#48948=EDGE_CURVE('',#38716,#38720,#6603,.T.);
#48949=EDGE_CURVE('',#38715,#38719,#6604,.T.);
#48950=EDGE_CURVE('',#38721,#38722,#6605,.T.);
#48951=EDGE_CURVE('',#38720,#38722,#6606,.T.);
#48952=EDGE_CURVE('',#38719,#38721,#6607,.T.);
#48953=EDGE_CURVE('',#38722,#38717,#6608,.T.);
#48954=EDGE_CURVE('',#38721,#38718,#6609,.T.);
#48955=EDGE_CURVE('',#38723,#38724,#6610,.T.);
#48956=EDGE_CURVE('',#38725,#38724,#6611,.T.);
#48957=EDGE_CURVE('',#38726,#38725,#6612,.T.);
#48958=EDGE_CURVE('',#38726,#38723,#6613,.T.);
#48959=EDGE_CURVE('',#38727,#38728,#6614,.T.);
#48960=EDGE_CURVE('',#38724,#38728,#6615,.T.);
#48961=EDGE_CURVE('',#38723,#38727,#6616,.T.);
#48962=EDGE_CURVE('',#38729,#38730,#6617,.T.);
#48963=EDGE_CURVE('',#38728,#38730,#6618,.T.);
#48964=EDGE_CURVE('',#38727,#38729,#6619,.T.);
#48965=EDGE_CURVE('',#38730,#38725,#6620,.T.);
#48966=EDGE_CURVE('',#38729,#38726,#6621,.T.);
#48967=EDGE_CURVE('',#38731,#38732,#6622,.T.);
#48968=EDGE_CURVE('',#38733,#38732,#6623,.T.);
#48969=EDGE_CURVE('',#38734,#38733,#6624,.T.);
#48970=EDGE_CURVE('',#38734,#38731,#6625,.T.);
#48971=EDGE_CURVE('',#38735,#38736,#6626,.T.);
#48972=EDGE_CURVE('',#38732,#38736,#6627,.T.);
#48973=EDGE_CURVE('',#38731,#38735,#6628,.T.);
#48974=EDGE_CURVE('',#38737,#38738,#6629,.T.);
#48975=EDGE_CURVE('',#38736,#38738,#6630,.T.);
#48976=EDGE_CURVE('',#38735,#38737,#6631,.T.);
#48977=EDGE_CURVE('',#38738,#38733,#6632,.T.);
#48978=EDGE_CURVE('',#38737,#38734,#6633,.T.);
#48979=EDGE_CURVE('',#38739,#38740,#6634,.T.);
#48980=EDGE_CURVE('',#38741,#38740,#6635,.T.);
#48981=EDGE_CURVE('',#38742,#38741,#6636,.T.);
#48982=EDGE_CURVE('',#38742,#38739,#6637,.T.);
#48983=EDGE_CURVE('',#38743,#38744,#6638,.T.);
#48984=EDGE_CURVE('',#38740,#38744,#6639,.T.);
#48985=EDGE_CURVE('',#38739,#38743,#6640,.T.);
#48986=EDGE_CURVE('',#38745,#38746,#6641,.T.);
#48987=EDGE_CURVE('',#38744,#38746,#6642,.T.);
#48988=EDGE_CURVE('',#38743,#38745,#6643,.T.);
#48989=EDGE_CURVE('',#38746,#38741,#6644,.T.);
#48990=EDGE_CURVE('',#38745,#38742,#6645,.T.);
#48991=EDGE_CURVE('',#38747,#38748,#6646,.T.);
#48992=EDGE_CURVE('',#38749,#38748,#6647,.T.);
#48993=EDGE_CURVE('',#38750,#38749,#6648,.T.);
#48994=EDGE_CURVE('',#38750,#38747,#6649,.T.);
#48995=EDGE_CURVE('',#38751,#38752,#6650,.T.);
#48996=EDGE_CURVE('',#38748,#38752,#6651,.T.);
#48997=EDGE_CURVE('',#38747,#38751,#6652,.T.);
#48998=EDGE_CURVE('',#38753,#38754,#6653,.T.);
#48999=EDGE_CURVE('',#38752,#38754,#6654,.T.);
#49000=EDGE_CURVE('',#38751,#38753,#6655,.T.);
#49001=EDGE_CURVE('',#38754,#38749,#6656,.T.);
#49002=EDGE_CURVE('',#38753,#38750,#6657,.T.);
#49003=EDGE_CURVE('',#38755,#38756,#6658,.T.);
#49004=EDGE_CURVE('',#38757,#38756,#6659,.T.);
#49005=EDGE_CURVE('',#38758,#38757,#6660,.T.);
#49006=EDGE_CURVE('',#38758,#38755,#6661,.T.);
#49007=EDGE_CURVE('',#38759,#38760,#6662,.T.);
#49008=EDGE_CURVE('',#38756,#38760,#6663,.T.);
#49009=EDGE_CURVE('',#38755,#38759,#6664,.T.);
#49010=EDGE_CURVE('',#38761,#38762,#6665,.T.);
#49011=EDGE_CURVE('',#38760,#38762,#6666,.T.);
#49012=EDGE_CURVE('',#38759,#38761,#6667,.T.);
#49013=EDGE_CURVE('',#38762,#38757,#6668,.T.);
#49014=EDGE_CURVE('',#38761,#38758,#6669,.T.);
#49015=EDGE_CURVE('',#38763,#38764,#6670,.T.);
#49016=EDGE_CURVE('',#38765,#38764,#6671,.T.);
#49017=EDGE_CURVE('',#38766,#38765,#6672,.T.);
#49018=EDGE_CURVE('',#38766,#38763,#6673,.T.);
#49019=EDGE_CURVE('',#38767,#38768,#6674,.T.);
#49020=EDGE_CURVE('',#38764,#38768,#6675,.T.);
#49021=EDGE_CURVE('',#38763,#38767,#6676,.T.);
#49022=EDGE_CURVE('',#38769,#38770,#6677,.T.);
#49023=EDGE_CURVE('',#38768,#38770,#6678,.T.);
#49024=EDGE_CURVE('',#38767,#38769,#6679,.T.);
#49025=EDGE_CURVE('',#38770,#38765,#6680,.T.);
#49026=EDGE_CURVE('',#38769,#38766,#6681,.T.);
#49027=EDGE_CURVE('',#38771,#38772,#6682,.T.);
#49028=EDGE_CURVE('',#38773,#38772,#6683,.T.);
#49029=EDGE_CURVE('',#38774,#38773,#6684,.T.);
#49030=EDGE_CURVE('',#38774,#38771,#6685,.T.);
#49031=EDGE_CURVE('',#38775,#38776,#6686,.T.);
#49032=EDGE_CURVE('',#38772,#38776,#6687,.T.);
#49033=EDGE_CURVE('',#38771,#38775,#6688,.T.);
#49034=EDGE_CURVE('',#38777,#38778,#6689,.T.);
#49035=EDGE_CURVE('',#38776,#38778,#6690,.T.);
#49036=EDGE_CURVE('',#38775,#38777,#6691,.T.);
#49037=EDGE_CURVE('',#38778,#38773,#6692,.T.);
#49038=EDGE_CURVE('',#38777,#38774,#6693,.T.);
#49039=EDGE_CURVE('',#38779,#38780,#6694,.T.);
#49040=EDGE_CURVE('',#38781,#38780,#6695,.T.);
#49041=EDGE_CURVE('',#38782,#38781,#6696,.T.);
#49042=EDGE_CURVE('',#38782,#38779,#6697,.T.);
#49043=EDGE_CURVE('',#38783,#38784,#6698,.T.);
#49044=EDGE_CURVE('',#38780,#38784,#6699,.T.);
#49045=EDGE_CURVE('',#38779,#38783,#6700,.T.);
#49046=EDGE_CURVE('',#38785,#38786,#6701,.T.);
#49047=EDGE_CURVE('',#38784,#38786,#6702,.T.);
#49048=EDGE_CURVE('',#38783,#38785,#6703,.T.);
#49049=EDGE_CURVE('',#38786,#38781,#6704,.T.);
#49050=EDGE_CURVE('',#38785,#38782,#6705,.T.);
#49051=EDGE_CURVE('',#38787,#38788,#6706,.T.);
#49052=EDGE_CURVE('',#38789,#38788,#6707,.T.);
#49053=EDGE_CURVE('',#38790,#38789,#6708,.T.);
#49054=EDGE_CURVE('',#38790,#38787,#6709,.T.);
#49055=EDGE_CURVE('',#38791,#38792,#6710,.T.);
#49056=EDGE_CURVE('',#38788,#38792,#6711,.T.);
#49057=EDGE_CURVE('',#38787,#38791,#6712,.T.);
#49058=EDGE_CURVE('',#38793,#38794,#6713,.T.);
#49059=EDGE_CURVE('',#38792,#38794,#6714,.T.);
#49060=EDGE_CURVE('',#38791,#38793,#6715,.T.);
#49061=EDGE_CURVE('',#38794,#38789,#6716,.T.);
#49062=EDGE_CURVE('',#38793,#38790,#6717,.T.);
#49063=EDGE_CURVE('',#38795,#38796,#6718,.T.);
#49064=EDGE_CURVE('',#38797,#38796,#6719,.T.);
#49065=EDGE_CURVE('',#38798,#38797,#6720,.T.);
#49066=EDGE_CURVE('',#38798,#38795,#6721,.T.);
#49067=EDGE_CURVE('',#38799,#38800,#6722,.T.);
#49068=EDGE_CURVE('',#38796,#38800,#6723,.T.);
#49069=EDGE_CURVE('',#38795,#38799,#6724,.T.);
#49070=EDGE_CURVE('',#38801,#38802,#6725,.T.);
#49071=EDGE_CURVE('',#38800,#38802,#6726,.T.);
#49072=EDGE_CURVE('',#38799,#38801,#6727,.T.);
#49073=EDGE_CURVE('',#38802,#38797,#6728,.T.);
#49074=EDGE_CURVE('',#38801,#38798,#6729,.T.);
#49075=EDGE_CURVE('',#38803,#38804,#6730,.T.);
#49076=EDGE_CURVE('',#38805,#38804,#6731,.T.);
#49077=EDGE_CURVE('',#38806,#38805,#6732,.T.);
#49078=EDGE_CURVE('',#38806,#38803,#6733,.T.);
#49079=EDGE_CURVE('',#38807,#38808,#6734,.T.);
#49080=EDGE_CURVE('',#38804,#38808,#6735,.T.);
#49081=EDGE_CURVE('',#38803,#38807,#6736,.T.);
#49082=EDGE_CURVE('',#38809,#38810,#6737,.T.);
#49083=EDGE_CURVE('',#38808,#38810,#6738,.T.);
#49084=EDGE_CURVE('',#38807,#38809,#6739,.T.);
#49085=EDGE_CURVE('',#38810,#38805,#6740,.T.);
#49086=EDGE_CURVE('',#38809,#38806,#6741,.T.);
#49087=EDGE_CURVE('',#38811,#38812,#6742,.T.);
#49088=EDGE_CURVE('',#38813,#38812,#6743,.T.);
#49089=EDGE_CURVE('',#38814,#38813,#6744,.T.);
#49090=EDGE_CURVE('',#38814,#38811,#6745,.T.);
#49091=EDGE_CURVE('',#38815,#38816,#6746,.T.);
#49092=EDGE_CURVE('',#38812,#38816,#6747,.T.);
#49093=EDGE_CURVE('',#38811,#38815,#6748,.T.);
#49094=EDGE_CURVE('',#38817,#38818,#6749,.T.);
#49095=EDGE_CURVE('',#38816,#38818,#6750,.T.);
#49096=EDGE_CURVE('',#38815,#38817,#6751,.T.);
#49097=EDGE_CURVE('',#38818,#38813,#6752,.T.);
#49098=EDGE_CURVE('',#38817,#38814,#6753,.T.);
#49099=EDGE_CURVE('',#38819,#38820,#6754,.T.);
#49100=EDGE_CURVE('',#38821,#38820,#6755,.T.);
#49101=EDGE_CURVE('',#38822,#38821,#6756,.T.);
#49102=EDGE_CURVE('',#38822,#38819,#6757,.T.);
#49103=EDGE_CURVE('',#38823,#38824,#6758,.T.);
#49104=EDGE_CURVE('',#38820,#38824,#6759,.T.);
#49105=EDGE_CURVE('',#38819,#38823,#6760,.T.);
#49106=EDGE_CURVE('',#38825,#38826,#6761,.T.);
#49107=EDGE_CURVE('',#38824,#38826,#6762,.T.);
#49108=EDGE_CURVE('',#38823,#38825,#6763,.T.);
#49109=EDGE_CURVE('',#38826,#38821,#6764,.T.);
#49110=EDGE_CURVE('',#38825,#38822,#6765,.T.);
#49111=EDGE_CURVE('',#38827,#38828,#6766,.T.);
#49112=EDGE_CURVE('',#38829,#38828,#6767,.T.);
#49113=EDGE_CURVE('',#38830,#38829,#6768,.T.);
#49114=EDGE_CURVE('',#38830,#38827,#6769,.T.);
#49115=EDGE_CURVE('',#38831,#38832,#6770,.T.);
#49116=EDGE_CURVE('',#38828,#38832,#6771,.T.);
#49117=EDGE_CURVE('',#38827,#38831,#6772,.T.);
#49118=EDGE_CURVE('',#38833,#38834,#6773,.T.);
#49119=EDGE_CURVE('',#38832,#38834,#6774,.T.);
#49120=EDGE_CURVE('',#38831,#38833,#6775,.T.);
#49121=EDGE_CURVE('',#38834,#38829,#6776,.T.);
#49122=EDGE_CURVE('',#38833,#38830,#6777,.T.);
#49123=EDGE_CURVE('',#38835,#38836,#6778,.T.);
#49124=EDGE_CURVE('',#38837,#38836,#6779,.T.);
#49125=EDGE_CURVE('',#38838,#38837,#6780,.T.);
#49126=EDGE_CURVE('',#38838,#38835,#6781,.T.);
#49127=EDGE_CURVE('',#38839,#38840,#6782,.T.);
#49128=EDGE_CURVE('',#38836,#38840,#6783,.T.);
#49129=EDGE_CURVE('',#38835,#38839,#6784,.T.);
#49130=EDGE_CURVE('',#38841,#38842,#6785,.T.);
#49131=EDGE_CURVE('',#38840,#38842,#6786,.T.);
#49132=EDGE_CURVE('',#38839,#38841,#6787,.T.);
#49133=EDGE_CURVE('',#38842,#38837,#6788,.T.);
#49134=EDGE_CURVE('',#38841,#38838,#6789,.T.);
#49135=EDGE_CURVE('',#38843,#38844,#6790,.T.);
#49136=EDGE_CURVE('',#38845,#38844,#6791,.T.);
#49137=EDGE_CURVE('',#38846,#38845,#6792,.T.);
#49138=EDGE_CURVE('',#38846,#38843,#6793,.T.);
#49139=EDGE_CURVE('',#38847,#38848,#6794,.T.);
#49140=EDGE_CURVE('',#38844,#38848,#6795,.T.);
#49141=EDGE_CURVE('',#38843,#38847,#6796,.T.);
#49142=EDGE_CURVE('',#38849,#38850,#6797,.T.);
#49143=EDGE_CURVE('',#38848,#38850,#6798,.T.);
#49144=EDGE_CURVE('',#38847,#38849,#6799,.T.);
#49145=EDGE_CURVE('',#38850,#38845,#6800,.T.);
#49146=EDGE_CURVE('',#38849,#38846,#6801,.T.);
#49147=EDGE_CURVE('',#38851,#38852,#6802,.T.);
#49148=EDGE_CURVE('',#38853,#38852,#6803,.T.);
#49149=EDGE_CURVE('',#38854,#38853,#6804,.T.);
#49150=EDGE_CURVE('',#38854,#38851,#6805,.T.);
#49151=EDGE_CURVE('',#38855,#38856,#6806,.T.);
#49152=EDGE_CURVE('',#38852,#38856,#6807,.T.);
#49153=EDGE_CURVE('',#38851,#38855,#6808,.T.);
#49154=EDGE_CURVE('',#38857,#38858,#6809,.T.);
#49155=EDGE_CURVE('',#38856,#38858,#6810,.T.);
#49156=EDGE_CURVE('',#38855,#38857,#6811,.T.);
#49157=EDGE_CURVE('',#38858,#38853,#6812,.T.);
#49158=EDGE_CURVE('',#38857,#38854,#6813,.T.);
#49159=EDGE_CURVE('',#38859,#38860,#6814,.T.);
#49160=EDGE_CURVE('',#38861,#38860,#6815,.T.);
#49161=EDGE_CURVE('',#38862,#38861,#6816,.T.);
#49162=EDGE_CURVE('',#38862,#38859,#6817,.T.);
#49163=EDGE_CURVE('',#38863,#38864,#6818,.T.);
#49164=EDGE_CURVE('',#38860,#38864,#6819,.T.);
#49165=EDGE_CURVE('',#38859,#38863,#6820,.T.);
#49166=EDGE_CURVE('',#38865,#38866,#6821,.T.);
#49167=EDGE_CURVE('',#38864,#38866,#6822,.T.);
#49168=EDGE_CURVE('',#38863,#38865,#6823,.T.);
#49169=EDGE_CURVE('',#38866,#38861,#6824,.T.);
#49170=EDGE_CURVE('',#38865,#38862,#6825,.T.);
#49171=EDGE_CURVE('',#38867,#38868,#6826,.T.);
#49172=EDGE_CURVE('',#38869,#38868,#6827,.T.);
#49173=EDGE_CURVE('',#38870,#38869,#6828,.T.);
#49174=EDGE_CURVE('',#38870,#38867,#6829,.T.);
#49175=EDGE_CURVE('',#38871,#38872,#6830,.T.);
#49176=EDGE_CURVE('',#38868,#38872,#6831,.T.);
#49177=EDGE_CURVE('',#38867,#38871,#6832,.T.);
#49178=EDGE_CURVE('',#38873,#38874,#6833,.T.);
#49179=EDGE_CURVE('',#38872,#38874,#6834,.T.);
#49180=EDGE_CURVE('',#38871,#38873,#6835,.T.);
#49181=EDGE_CURVE('',#38874,#38869,#6836,.T.);
#49182=EDGE_CURVE('',#38873,#38870,#6837,.T.);
#49183=EDGE_CURVE('',#38875,#38876,#6838,.T.);
#49184=EDGE_CURVE('',#38877,#38876,#6839,.T.);
#49185=EDGE_CURVE('',#38878,#38877,#6840,.T.);
#49186=EDGE_CURVE('',#38878,#38875,#6841,.T.);
#49187=EDGE_CURVE('',#38879,#38880,#6842,.T.);
#49188=EDGE_CURVE('',#38876,#38880,#6843,.T.);
#49189=EDGE_CURVE('',#38875,#38879,#6844,.T.);
#49190=EDGE_CURVE('',#38881,#38882,#6845,.T.);
#49191=EDGE_CURVE('',#38880,#38882,#6846,.T.);
#49192=EDGE_CURVE('',#38879,#38881,#6847,.T.);
#49193=EDGE_CURVE('',#38882,#38877,#6848,.T.);
#49194=EDGE_CURVE('',#38881,#38878,#6849,.T.);
#49195=EDGE_CURVE('',#38883,#38884,#6850,.T.);
#49196=EDGE_CURVE('',#38885,#38884,#6851,.T.);
#49197=EDGE_CURVE('',#38886,#38885,#6852,.T.);
#49198=EDGE_CURVE('',#38886,#38883,#6853,.T.);
#49199=EDGE_CURVE('',#38887,#38888,#6854,.T.);
#49200=EDGE_CURVE('',#38884,#38888,#6855,.T.);
#49201=EDGE_CURVE('',#38883,#38887,#6856,.T.);
#49202=EDGE_CURVE('',#38889,#38890,#6857,.T.);
#49203=EDGE_CURVE('',#38888,#38890,#6858,.T.);
#49204=EDGE_CURVE('',#38887,#38889,#6859,.T.);
#49205=EDGE_CURVE('',#38890,#38885,#6860,.T.);
#49206=EDGE_CURVE('',#38889,#38886,#6861,.T.);
#49207=EDGE_CURVE('',#38891,#38892,#6862,.T.);
#49208=EDGE_CURVE('',#38893,#38892,#6863,.T.);
#49209=EDGE_CURVE('',#38894,#38893,#6864,.T.);
#49210=EDGE_CURVE('',#38894,#38891,#6865,.T.);
#49211=EDGE_CURVE('',#38895,#38896,#6866,.T.);
#49212=EDGE_CURVE('',#38892,#38896,#6867,.T.);
#49213=EDGE_CURVE('',#38891,#38895,#6868,.T.);
#49214=EDGE_CURVE('',#38897,#38898,#6869,.T.);
#49215=EDGE_CURVE('',#38896,#38898,#6870,.T.);
#49216=EDGE_CURVE('',#38895,#38897,#6871,.T.);
#49217=EDGE_CURVE('',#38898,#38893,#6872,.T.);
#49218=EDGE_CURVE('',#38897,#38894,#6873,.T.);
#49219=EDGE_CURVE('',#38899,#38900,#6874,.T.);
#49220=EDGE_CURVE('',#38901,#38900,#6875,.T.);
#49221=EDGE_CURVE('',#38902,#38901,#6876,.T.);
#49222=EDGE_CURVE('',#38902,#38899,#6877,.T.);
#49223=EDGE_CURVE('',#38903,#38904,#6878,.T.);
#49224=EDGE_CURVE('',#38900,#38904,#6879,.T.);
#49225=EDGE_CURVE('',#38899,#38903,#6880,.T.);
#49226=EDGE_CURVE('',#38905,#38906,#6881,.T.);
#49227=EDGE_CURVE('',#38904,#38906,#6882,.T.);
#49228=EDGE_CURVE('',#38903,#38905,#6883,.T.);
#49229=EDGE_CURVE('',#38906,#38901,#6884,.T.);
#49230=EDGE_CURVE('',#38905,#38902,#6885,.T.);
#49231=EDGE_CURVE('',#38907,#38908,#6886,.T.);
#49232=EDGE_CURVE('',#38909,#38908,#6887,.T.);
#49233=EDGE_CURVE('',#38910,#38909,#6888,.T.);
#49234=EDGE_CURVE('',#38910,#38907,#6889,.T.);
#49235=EDGE_CURVE('',#38911,#38912,#6890,.T.);
#49236=EDGE_CURVE('',#38908,#38912,#6891,.T.);
#49237=EDGE_CURVE('',#38907,#38911,#6892,.T.);
#49238=EDGE_CURVE('',#38913,#38914,#6893,.T.);
#49239=EDGE_CURVE('',#38912,#38914,#6894,.T.);
#49240=EDGE_CURVE('',#38911,#38913,#6895,.T.);
#49241=EDGE_CURVE('',#38914,#38909,#6896,.T.);
#49242=EDGE_CURVE('',#38913,#38910,#6897,.T.);
#49243=EDGE_CURVE('',#38915,#38916,#6898,.T.);
#49244=EDGE_CURVE('',#38917,#38916,#6899,.T.);
#49245=EDGE_CURVE('',#38918,#38917,#6900,.T.);
#49246=EDGE_CURVE('',#38918,#38915,#6901,.T.);
#49247=EDGE_CURVE('',#38919,#38920,#6902,.T.);
#49248=EDGE_CURVE('',#38916,#38920,#6903,.T.);
#49249=EDGE_CURVE('',#38915,#38919,#6904,.T.);
#49250=EDGE_CURVE('',#38921,#38922,#6905,.T.);
#49251=EDGE_CURVE('',#38920,#38922,#6906,.T.);
#49252=EDGE_CURVE('',#38919,#38921,#6907,.T.);
#49253=EDGE_CURVE('',#38922,#38917,#6908,.T.);
#49254=EDGE_CURVE('',#38921,#38918,#6909,.T.);
#49255=EDGE_CURVE('',#38923,#38924,#6910,.T.);
#49256=EDGE_CURVE('',#38925,#38924,#6911,.T.);
#49257=EDGE_CURVE('',#38926,#38925,#6912,.T.);
#49258=EDGE_CURVE('',#38926,#38923,#6913,.T.);
#49259=EDGE_CURVE('',#38927,#38928,#6914,.T.);
#49260=EDGE_CURVE('',#38924,#38928,#6915,.T.);
#49261=EDGE_CURVE('',#38923,#38927,#6916,.T.);
#49262=EDGE_CURVE('',#38929,#38930,#6917,.T.);
#49263=EDGE_CURVE('',#38928,#38930,#6918,.T.);
#49264=EDGE_CURVE('',#38927,#38929,#6919,.T.);
#49265=EDGE_CURVE('',#38930,#38925,#6920,.T.);
#49266=EDGE_CURVE('',#38929,#38926,#6921,.T.);
#49267=EDGE_CURVE('',#38931,#38932,#6922,.T.);
#49268=EDGE_CURVE('',#38933,#38932,#6923,.T.);
#49269=EDGE_CURVE('',#38934,#38933,#6924,.T.);
#49270=EDGE_CURVE('',#38934,#38931,#6925,.T.);
#49271=EDGE_CURVE('',#38935,#38936,#6926,.T.);
#49272=EDGE_CURVE('',#38932,#38936,#6927,.T.);
#49273=EDGE_CURVE('',#38931,#38935,#6928,.T.);
#49274=EDGE_CURVE('',#38937,#38938,#6929,.T.);
#49275=EDGE_CURVE('',#38936,#38938,#6930,.T.);
#49276=EDGE_CURVE('',#38935,#38937,#6931,.T.);
#49277=EDGE_CURVE('',#38938,#38933,#6932,.T.);
#49278=EDGE_CURVE('',#38937,#38934,#6933,.T.);
#49279=EDGE_CURVE('',#38939,#38940,#6934,.T.);
#49280=EDGE_CURVE('',#38941,#38940,#6935,.T.);
#49281=EDGE_CURVE('',#38942,#38941,#6936,.T.);
#49282=EDGE_CURVE('',#38942,#38939,#6937,.T.);
#49283=EDGE_CURVE('',#38943,#38944,#6938,.T.);
#49284=EDGE_CURVE('',#38940,#38944,#6939,.T.);
#49285=EDGE_CURVE('',#38939,#38943,#6940,.T.);
#49286=EDGE_CURVE('',#38945,#38946,#6941,.T.);
#49287=EDGE_CURVE('',#38944,#38946,#6942,.T.);
#49288=EDGE_CURVE('',#38943,#38945,#6943,.T.);
#49289=EDGE_CURVE('',#38946,#38941,#6944,.T.);
#49290=EDGE_CURVE('',#38945,#38942,#6945,.T.);
#49291=EDGE_CURVE('',#38947,#38948,#6946,.T.);
#49292=EDGE_CURVE('',#38949,#38948,#6947,.T.);
#49293=EDGE_CURVE('',#38950,#38949,#6948,.T.);
#49294=EDGE_CURVE('',#38950,#38947,#6949,.T.);
#49295=EDGE_CURVE('',#38951,#38952,#6950,.T.);
#49296=EDGE_CURVE('',#38948,#38952,#6951,.T.);
#49297=EDGE_CURVE('',#38947,#38951,#6952,.T.);
#49298=EDGE_CURVE('',#38953,#38954,#6953,.T.);
#49299=EDGE_CURVE('',#38952,#38954,#6954,.T.);
#49300=EDGE_CURVE('',#38951,#38953,#6955,.T.);
#49301=EDGE_CURVE('',#38954,#38949,#6956,.T.);
#49302=EDGE_CURVE('',#38953,#38950,#6957,.T.);
#49303=EDGE_CURVE('',#38955,#38956,#6958,.T.);
#49304=EDGE_CURVE('',#38957,#38956,#6959,.T.);
#49305=EDGE_CURVE('',#38958,#38957,#6960,.T.);
#49306=EDGE_CURVE('',#38958,#38955,#6961,.T.);
#49307=EDGE_CURVE('',#38959,#38960,#6962,.T.);
#49308=EDGE_CURVE('',#38956,#38960,#6963,.T.);
#49309=EDGE_CURVE('',#38955,#38959,#6964,.T.);
#49310=EDGE_CURVE('',#38961,#38962,#6965,.T.);
#49311=EDGE_CURVE('',#38960,#38962,#6966,.T.);
#49312=EDGE_CURVE('',#38959,#38961,#6967,.T.);
#49313=EDGE_CURVE('',#38962,#38957,#6968,.T.);
#49314=EDGE_CURVE('',#38961,#38958,#6969,.T.);
#49315=EDGE_CURVE('',#38963,#38964,#6970,.T.);
#49316=EDGE_CURVE('',#38965,#38964,#6971,.T.);
#49317=EDGE_CURVE('',#38966,#38965,#6972,.T.);
#49318=EDGE_CURVE('',#38966,#38963,#6973,.T.);
#49319=EDGE_CURVE('',#38967,#38968,#6974,.T.);
#49320=EDGE_CURVE('',#38964,#38968,#6975,.T.);
#49321=EDGE_CURVE('',#38963,#38967,#6976,.T.);
#49322=EDGE_CURVE('',#38969,#38970,#6977,.T.);
#49323=EDGE_CURVE('',#38968,#38970,#6978,.T.);
#49324=EDGE_CURVE('',#38967,#38969,#6979,.T.);
#49325=EDGE_CURVE('',#38970,#38965,#6980,.T.);
#49326=EDGE_CURVE('',#38969,#38966,#6981,.T.);
#49327=EDGE_CURVE('',#38971,#38972,#6982,.T.);
#49328=EDGE_CURVE('',#38973,#38972,#6983,.T.);
#49329=EDGE_CURVE('',#38974,#38973,#6984,.T.);
#49330=EDGE_CURVE('',#38974,#38971,#6985,.T.);
#49331=EDGE_CURVE('',#38975,#38976,#6986,.T.);
#49332=EDGE_CURVE('',#38972,#38976,#6987,.T.);
#49333=EDGE_CURVE('',#38971,#38975,#6988,.T.);
#49334=EDGE_CURVE('',#38977,#38978,#6989,.T.);
#49335=EDGE_CURVE('',#38976,#38978,#6990,.T.);
#49336=EDGE_CURVE('',#38975,#38977,#6991,.T.);
#49337=EDGE_CURVE('',#38978,#38973,#6992,.T.);
#49338=EDGE_CURVE('',#38977,#38974,#6993,.T.);
#49339=EDGE_CURVE('',#38979,#38980,#6994,.T.);
#49340=EDGE_CURVE('',#38981,#38980,#6995,.T.);
#49341=EDGE_CURVE('',#38982,#38981,#6996,.T.);
#49342=EDGE_CURVE('',#38982,#38979,#6997,.T.);
#49343=EDGE_CURVE('',#38983,#38984,#6998,.T.);
#49344=EDGE_CURVE('',#38980,#38984,#6999,.T.);
#49345=EDGE_CURVE('',#38979,#38983,#7000,.T.);
#49346=EDGE_CURVE('',#38985,#38986,#7001,.T.);
#49347=EDGE_CURVE('',#38984,#38986,#7002,.T.);
#49348=EDGE_CURVE('',#38983,#38985,#7003,.T.);
#49349=EDGE_CURVE('',#38986,#38981,#7004,.T.);
#49350=EDGE_CURVE('',#38985,#38982,#7005,.T.);
#49351=EDGE_CURVE('',#38987,#38988,#7006,.T.);
#49352=EDGE_CURVE('',#38989,#38988,#7007,.T.);
#49353=EDGE_CURVE('',#38990,#38989,#7008,.T.);
#49354=EDGE_CURVE('',#38990,#38987,#7009,.T.);
#49355=EDGE_CURVE('',#38991,#38992,#7010,.T.);
#49356=EDGE_CURVE('',#38988,#38992,#7011,.T.);
#49357=EDGE_CURVE('',#38987,#38991,#7012,.T.);
#49358=EDGE_CURVE('',#38993,#38994,#7013,.T.);
#49359=EDGE_CURVE('',#38992,#38994,#7014,.T.);
#49360=EDGE_CURVE('',#38991,#38993,#7015,.T.);
#49361=EDGE_CURVE('',#38994,#38989,#7016,.T.);
#49362=EDGE_CURVE('',#38993,#38990,#7017,.T.);
#49363=EDGE_CURVE('',#38995,#38996,#7018,.T.);
#49364=EDGE_CURVE('',#38997,#38996,#7019,.T.);
#49365=EDGE_CURVE('',#38998,#38997,#7020,.T.);
#49366=EDGE_CURVE('',#38998,#38995,#7021,.T.);
#49367=EDGE_CURVE('',#38999,#39000,#7022,.T.);
#49368=EDGE_CURVE('',#38996,#39000,#7023,.T.);
#49369=EDGE_CURVE('',#38995,#38999,#7024,.T.);
#49370=EDGE_CURVE('',#39001,#39002,#7025,.T.);
#49371=EDGE_CURVE('',#39000,#39002,#7026,.T.);
#49372=EDGE_CURVE('',#38999,#39001,#7027,.T.);
#49373=EDGE_CURVE('',#39002,#38997,#7028,.T.);
#49374=EDGE_CURVE('',#39001,#38998,#7029,.T.);
#49375=EDGE_CURVE('',#39003,#39004,#7030,.T.);
#49376=EDGE_CURVE('',#39005,#39004,#7031,.T.);
#49377=EDGE_CURVE('',#39006,#39005,#7032,.T.);
#49378=EDGE_CURVE('',#39006,#39003,#7033,.T.);
#49379=EDGE_CURVE('',#39007,#39008,#7034,.T.);
#49380=EDGE_CURVE('',#39004,#39008,#7035,.T.);
#49381=EDGE_CURVE('',#39003,#39007,#7036,.T.);
#49382=EDGE_CURVE('',#39009,#39010,#7037,.T.);
#49383=EDGE_CURVE('',#39008,#39010,#7038,.T.);
#49384=EDGE_CURVE('',#39007,#39009,#7039,.T.);
#49385=EDGE_CURVE('',#39010,#39005,#7040,.T.);
#49386=EDGE_CURVE('',#39009,#39006,#7041,.T.);
#49387=EDGE_CURVE('',#39011,#39012,#7042,.T.);
#49388=EDGE_CURVE('',#39013,#39012,#7043,.T.);
#49389=EDGE_CURVE('',#39014,#39013,#7044,.T.);
#49390=EDGE_CURVE('',#39014,#39011,#7045,.T.);
#49391=EDGE_CURVE('',#39015,#39016,#7046,.T.);
#49392=EDGE_CURVE('',#39012,#39016,#7047,.T.);
#49393=EDGE_CURVE('',#39011,#39015,#7048,.T.);
#49394=EDGE_CURVE('',#39017,#39018,#7049,.T.);
#49395=EDGE_CURVE('',#39016,#39018,#7050,.T.);
#49396=EDGE_CURVE('',#39015,#39017,#7051,.T.);
#49397=EDGE_CURVE('',#39018,#39013,#7052,.T.);
#49398=EDGE_CURVE('',#39017,#39014,#7053,.T.);
#49399=EDGE_CURVE('',#39019,#39020,#7054,.T.);
#49400=EDGE_CURVE('',#39021,#39020,#7055,.T.);
#49401=EDGE_CURVE('',#39022,#39021,#7056,.T.);
#49402=EDGE_CURVE('',#39022,#39019,#7057,.T.);
#49403=EDGE_CURVE('',#39023,#39024,#7058,.T.);
#49404=EDGE_CURVE('',#39020,#39024,#7059,.T.);
#49405=EDGE_CURVE('',#39019,#39023,#7060,.T.);
#49406=EDGE_CURVE('',#39025,#39026,#7061,.T.);
#49407=EDGE_CURVE('',#39024,#39026,#7062,.T.);
#49408=EDGE_CURVE('',#39023,#39025,#7063,.T.);
#49409=EDGE_CURVE('',#39026,#39021,#7064,.T.);
#49410=EDGE_CURVE('',#39025,#39022,#7065,.T.);
#49411=EDGE_CURVE('',#39027,#39028,#7066,.T.);
#49412=EDGE_CURVE('',#39029,#39028,#7067,.T.);
#49413=EDGE_CURVE('',#39030,#39029,#7068,.T.);
#49414=EDGE_CURVE('',#39030,#39027,#7069,.T.);
#49415=EDGE_CURVE('',#39031,#39032,#7070,.T.);
#49416=EDGE_CURVE('',#39028,#39032,#7071,.T.);
#49417=EDGE_CURVE('',#39027,#39031,#7072,.T.);
#49418=EDGE_CURVE('',#39033,#39034,#7073,.T.);
#49419=EDGE_CURVE('',#39032,#39034,#7074,.T.);
#49420=EDGE_CURVE('',#39031,#39033,#7075,.T.);
#49421=EDGE_CURVE('',#39034,#39029,#7076,.T.);
#49422=EDGE_CURVE('',#39033,#39030,#7077,.T.);
#49423=EDGE_CURVE('',#39035,#39036,#7078,.T.);
#49424=EDGE_CURVE('',#39037,#39036,#7079,.T.);
#49425=EDGE_CURVE('',#39038,#39037,#7080,.T.);
#49426=EDGE_CURVE('',#39038,#39035,#7081,.T.);
#49427=EDGE_CURVE('',#39039,#39040,#7082,.T.);
#49428=EDGE_CURVE('',#39036,#39040,#7083,.T.);
#49429=EDGE_CURVE('',#39035,#39039,#7084,.T.);
#49430=EDGE_CURVE('',#39041,#39042,#7085,.T.);
#49431=EDGE_CURVE('',#39040,#39042,#7086,.T.);
#49432=EDGE_CURVE('',#39039,#39041,#7087,.T.);
#49433=EDGE_CURVE('',#39042,#39037,#7088,.T.);
#49434=EDGE_CURVE('',#39041,#39038,#7089,.T.);
#49435=EDGE_CURVE('',#39043,#39044,#7090,.T.);
#49436=EDGE_CURVE('',#39045,#39044,#7091,.T.);
#49437=EDGE_CURVE('',#39046,#39045,#7092,.T.);
#49438=EDGE_CURVE('',#39046,#39043,#7093,.T.);
#49439=EDGE_CURVE('',#39047,#39048,#7094,.T.);
#49440=EDGE_CURVE('',#39044,#39048,#7095,.T.);
#49441=EDGE_CURVE('',#39043,#39047,#7096,.T.);
#49442=EDGE_CURVE('',#39049,#39050,#7097,.T.);
#49443=EDGE_CURVE('',#39048,#39050,#7098,.T.);
#49444=EDGE_CURVE('',#39047,#39049,#7099,.T.);
#49445=EDGE_CURVE('',#39050,#39045,#7100,.T.);
#49446=EDGE_CURVE('',#39049,#39046,#7101,.T.);
#49447=EDGE_CURVE('',#39051,#39052,#7102,.T.);
#49448=EDGE_CURVE('',#39053,#39052,#7103,.T.);
#49449=EDGE_CURVE('',#39054,#39053,#7104,.T.);
#49450=EDGE_CURVE('',#39054,#39051,#7105,.T.);
#49451=EDGE_CURVE('',#39055,#39056,#7106,.T.);
#49452=EDGE_CURVE('',#39052,#39056,#7107,.T.);
#49453=EDGE_CURVE('',#39051,#39055,#7108,.T.);
#49454=EDGE_CURVE('',#39057,#39058,#7109,.T.);
#49455=EDGE_CURVE('',#39056,#39058,#7110,.T.);
#49456=EDGE_CURVE('',#39055,#39057,#7111,.T.);
#49457=EDGE_CURVE('',#39058,#39053,#7112,.T.);
#49458=EDGE_CURVE('',#39057,#39054,#7113,.T.);
#49459=EDGE_CURVE('',#39059,#39060,#7114,.T.);
#49460=EDGE_CURVE('',#39061,#39060,#7115,.T.);
#49461=EDGE_CURVE('',#39062,#39061,#7116,.T.);
#49462=EDGE_CURVE('',#39062,#39059,#7117,.T.);
#49463=EDGE_CURVE('',#39063,#39064,#7118,.T.);
#49464=EDGE_CURVE('',#39060,#39064,#7119,.T.);
#49465=EDGE_CURVE('',#39059,#39063,#7120,.T.);
#49466=EDGE_CURVE('',#39065,#39066,#7121,.T.);
#49467=EDGE_CURVE('',#39064,#39066,#7122,.T.);
#49468=EDGE_CURVE('',#39063,#39065,#7123,.T.);
#49469=EDGE_CURVE('',#39066,#39061,#7124,.T.);
#49470=EDGE_CURVE('',#39065,#39062,#7125,.T.);
#49471=EDGE_CURVE('',#39067,#39068,#7126,.T.);
#49472=EDGE_CURVE('',#39069,#39068,#7127,.T.);
#49473=EDGE_CURVE('',#39070,#39069,#7128,.T.);
#49474=EDGE_CURVE('',#39070,#39067,#7129,.T.);
#49475=EDGE_CURVE('',#39071,#39072,#7130,.T.);
#49476=EDGE_CURVE('',#39068,#39072,#7131,.T.);
#49477=EDGE_CURVE('',#39067,#39071,#7132,.T.);
#49478=EDGE_CURVE('',#39073,#39074,#7133,.T.);
#49479=EDGE_CURVE('',#39072,#39074,#7134,.T.);
#49480=EDGE_CURVE('',#39071,#39073,#7135,.T.);
#49481=EDGE_CURVE('',#39074,#39069,#7136,.T.);
#49482=EDGE_CURVE('',#39073,#39070,#7137,.T.);
#49483=EDGE_CURVE('',#39075,#39076,#7138,.T.);
#49484=EDGE_CURVE('',#39077,#39076,#7139,.T.);
#49485=EDGE_CURVE('',#39078,#39077,#7140,.T.);
#49486=EDGE_CURVE('',#39078,#39075,#7141,.T.);
#49487=EDGE_CURVE('',#39079,#39080,#7142,.T.);
#49488=EDGE_CURVE('',#39076,#39080,#7143,.T.);
#49489=EDGE_CURVE('',#39075,#39079,#7144,.T.);
#49490=EDGE_CURVE('',#39081,#39082,#7145,.T.);
#49491=EDGE_CURVE('',#39080,#39082,#7146,.T.);
#49492=EDGE_CURVE('',#39079,#39081,#7147,.T.);
#49493=EDGE_CURVE('',#39082,#39077,#7148,.T.);
#49494=EDGE_CURVE('',#39081,#39078,#7149,.T.);
#49495=EDGE_CURVE('',#39083,#39084,#7150,.T.);
#49496=EDGE_CURVE('',#39085,#39084,#7151,.T.);
#49497=EDGE_CURVE('',#39086,#39085,#7152,.T.);
#49498=EDGE_CURVE('',#39086,#39083,#7153,.T.);
#49499=EDGE_CURVE('',#39087,#39088,#7154,.T.);
#49500=EDGE_CURVE('',#39084,#39088,#7155,.T.);
#49501=EDGE_CURVE('',#39083,#39087,#7156,.T.);
#49502=EDGE_CURVE('',#39089,#39090,#7157,.T.);
#49503=EDGE_CURVE('',#39088,#39090,#7158,.T.);
#49504=EDGE_CURVE('',#39087,#39089,#7159,.T.);
#49505=EDGE_CURVE('',#39090,#39085,#7160,.T.);
#49506=EDGE_CURVE('',#39089,#39086,#7161,.T.);
#49507=EDGE_CURVE('',#39091,#39092,#7162,.T.);
#49508=EDGE_CURVE('',#39093,#39092,#7163,.T.);
#49509=EDGE_CURVE('',#39094,#39093,#7164,.T.);
#49510=EDGE_CURVE('',#39094,#39091,#7165,.T.);
#49511=EDGE_CURVE('',#39095,#39096,#7166,.T.);
#49512=EDGE_CURVE('',#39092,#39096,#7167,.T.);
#49513=EDGE_CURVE('',#39091,#39095,#7168,.T.);
#49514=EDGE_CURVE('',#39097,#39098,#7169,.T.);
#49515=EDGE_CURVE('',#39096,#39098,#7170,.T.);
#49516=EDGE_CURVE('',#39095,#39097,#7171,.T.);
#49517=EDGE_CURVE('',#39098,#39093,#7172,.T.);
#49518=EDGE_CURVE('',#39097,#39094,#7173,.T.);
#49519=EDGE_CURVE('',#39099,#39100,#7174,.T.);
#49520=EDGE_CURVE('',#39101,#39100,#7175,.T.);
#49521=EDGE_CURVE('',#39102,#39101,#7176,.T.);
#49522=EDGE_CURVE('',#39102,#39099,#7177,.T.);
#49523=EDGE_CURVE('',#39103,#39104,#7178,.T.);
#49524=EDGE_CURVE('',#39100,#39104,#7179,.T.);
#49525=EDGE_CURVE('',#39099,#39103,#7180,.T.);
#49526=EDGE_CURVE('',#39105,#39106,#7181,.T.);
#49527=EDGE_CURVE('',#39104,#39106,#7182,.T.);
#49528=EDGE_CURVE('',#39103,#39105,#7183,.T.);
#49529=EDGE_CURVE('',#39106,#39101,#7184,.T.);
#49530=EDGE_CURVE('',#39105,#39102,#7185,.T.);
#49531=EDGE_CURVE('',#39107,#39108,#7186,.T.);
#49532=EDGE_CURVE('',#39109,#39108,#7187,.T.);
#49533=EDGE_CURVE('',#39110,#39109,#7188,.T.);
#49534=EDGE_CURVE('',#39110,#39107,#7189,.T.);
#49535=EDGE_CURVE('',#39111,#39112,#7190,.T.);
#49536=EDGE_CURVE('',#39108,#39112,#7191,.T.);
#49537=EDGE_CURVE('',#39107,#39111,#7192,.T.);
#49538=EDGE_CURVE('',#39113,#39114,#7193,.T.);
#49539=EDGE_CURVE('',#39112,#39114,#7194,.T.);
#49540=EDGE_CURVE('',#39111,#39113,#7195,.T.);
#49541=EDGE_CURVE('',#39114,#39109,#7196,.T.);
#49542=EDGE_CURVE('',#39113,#39110,#7197,.T.);
#49543=EDGE_CURVE('',#39115,#39116,#7198,.T.);
#49544=EDGE_CURVE('',#39117,#39116,#7199,.T.);
#49545=EDGE_CURVE('',#39118,#39117,#7200,.T.);
#49546=EDGE_CURVE('',#39118,#39115,#7201,.T.);
#49547=EDGE_CURVE('',#39119,#39120,#7202,.T.);
#49548=EDGE_CURVE('',#39116,#39120,#7203,.T.);
#49549=EDGE_CURVE('',#39115,#39119,#7204,.T.);
#49550=EDGE_CURVE('',#39121,#39122,#7205,.T.);
#49551=EDGE_CURVE('',#39120,#39122,#7206,.T.);
#49552=EDGE_CURVE('',#39119,#39121,#7207,.T.);
#49553=EDGE_CURVE('',#39122,#39117,#7208,.T.);
#49554=EDGE_CURVE('',#39121,#39118,#7209,.T.);
#49555=EDGE_CURVE('',#39123,#39124,#7210,.T.);
#49556=EDGE_CURVE('',#39125,#39124,#7211,.T.);
#49557=EDGE_CURVE('',#39126,#39125,#7212,.T.);
#49558=EDGE_CURVE('',#39126,#39123,#7213,.T.);
#49559=EDGE_CURVE('',#39127,#39128,#7214,.T.);
#49560=EDGE_CURVE('',#39124,#39128,#7215,.T.);
#49561=EDGE_CURVE('',#39123,#39127,#7216,.T.);
#49562=EDGE_CURVE('',#39129,#39130,#7217,.T.);
#49563=EDGE_CURVE('',#39128,#39130,#7218,.T.);
#49564=EDGE_CURVE('',#39127,#39129,#7219,.T.);
#49565=EDGE_CURVE('',#39130,#39125,#7220,.T.);
#49566=EDGE_CURVE('',#39129,#39126,#7221,.T.);
#49567=EDGE_CURVE('',#39131,#39132,#7222,.T.);
#49568=EDGE_CURVE('',#39133,#39132,#7223,.T.);
#49569=EDGE_CURVE('',#39134,#39133,#7224,.T.);
#49570=EDGE_CURVE('',#39134,#39131,#7225,.T.);
#49571=EDGE_CURVE('',#39135,#39136,#7226,.T.);
#49572=EDGE_CURVE('',#39132,#39136,#7227,.T.);
#49573=EDGE_CURVE('',#39131,#39135,#7228,.T.);
#49574=EDGE_CURVE('',#39137,#39138,#7229,.T.);
#49575=EDGE_CURVE('',#39136,#39138,#7230,.T.);
#49576=EDGE_CURVE('',#39135,#39137,#7231,.T.);
#49577=EDGE_CURVE('',#39138,#39133,#7232,.T.);
#49578=EDGE_CURVE('',#39137,#39134,#7233,.T.);
#49579=EDGE_CURVE('',#39139,#39140,#7234,.T.);
#49580=EDGE_CURVE('',#39141,#39140,#7235,.T.);
#49581=EDGE_CURVE('',#39142,#39141,#7236,.T.);
#49582=EDGE_CURVE('',#39142,#39139,#7237,.T.);
#49583=EDGE_CURVE('',#39143,#39144,#7238,.T.);
#49584=EDGE_CURVE('',#39140,#39144,#7239,.T.);
#49585=EDGE_CURVE('',#39139,#39143,#7240,.T.);
#49586=EDGE_CURVE('',#39145,#39146,#7241,.T.);
#49587=EDGE_CURVE('',#39144,#39146,#7242,.T.);
#49588=EDGE_CURVE('',#39143,#39145,#7243,.T.);
#49589=EDGE_CURVE('',#39146,#39141,#7244,.T.);
#49590=EDGE_CURVE('',#39145,#39142,#7245,.T.);
#49591=EDGE_CURVE('',#39147,#39148,#7246,.T.);
#49592=EDGE_CURVE('',#39149,#39148,#7247,.T.);
#49593=EDGE_CURVE('',#39150,#39149,#7248,.T.);
#49594=EDGE_CURVE('',#39150,#39147,#7249,.T.);
#49595=EDGE_CURVE('',#39151,#39152,#7250,.T.);
#49596=EDGE_CURVE('',#39148,#39152,#7251,.T.);
#49597=EDGE_CURVE('',#39147,#39151,#7252,.T.);
#49598=EDGE_CURVE('',#39153,#39154,#7253,.T.);
#49599=EDGE_CURVE('',#39152,#39154,#7254,.T.);
#49600=EDGE_CURVE('',#39151,#39153,#7255,.T.);
#49601=EDGE_CURVE('',#39154,#39149,#7256,.T.);
#49602=EDGE_CURVE('',#39153,#39150,#7257,.T.);
#49603=EDGE_CURVE('',#39155,#39156,#7258,.T.);
#49604=EDGE_CURVE('',#39157,#39156,#7259,.T.);
#49605=EDGE_CURVE('',#39158,#39157,#7260,.T.);
#49606=EDGE_CURVE('',#39158,#39155,#7261,.T.);
#49607=EDGE_CURVE('',#39159,#39160,#7262,.T.);
#49608=EDGE_CURVE('',#39156,#39160,#7263,.T.);
#49609=EDGE_CURVE('',#39155,#39159,#7264,.T.);
#49610=EDGE_CURVE('',#39161,#39162,#7265,.T.);
#49611=EDGE_CURVE('',#39160,#39162,#7266,.T.);
#49612=EDGE_CURVE('',#39159,#39161,#7267,.T.);
#49613=EDGE_CURVE('',#39162,#39157,#7268,.T.);
#49614=EDGE_CURVE('',#39161,#39158,#7269,.T.);
#49615=EDGE_CURVE('',#39163,#39164,#7270,.T.);
#49616=EDGE_CURVE('',#39165,#39164,#7271,.T.);
#49617=EDGE_CURVE('',#39166,#39165,#7272,.T.);
#49618=EDGE_CURVE('',#39166,#39163,#7273,.T.);
#49619=EDGE_CURVE('',#39167,#39168,#7274,.T.);
#49620=EDGE_CURVE('',#39164,#39168,#7275,.T.);
#49621=EDGE_CURVE('',#39163,#39167,#7276,.T.);
#49622=EDGE_CURVE('',#39169,#39170,#7277,.T.);
#49623=EDGE_CURVE('',#39168,#39170,#7278,.T.);
#49624=EDGE_CURVE('',#39167,#39169,#7279,.T.);
#49625=EDGE_CURVE('',#39170,#39165,#7280,.T.);
#49626=EDGE_CURVE('',#39169,#39166,#7281,.T.);
#49627=EDGE_CURVE('',#39171,#39172,#7282,.T.);
#49628=EDGE_CURVE('',#39173,#39172,#7283,.T.);
#49629=EDGE_CURVE('',#39174,#39173,#7284,.T.);
#49630=EDGE_CURVE('',#39174,#39171,#7285,.T.);
#49631=EDGE_CURVE('',#39175,#39176,#7286,.T.);
#49632=EDGE_CURVE('',#39172,#39176,#7287,.T.);
#49633=EDGE_CURVE('',#39171,#39175,#7288,.T.);
#49634=EDGE_CURVE('',#39177,#39178,#7289,.T.);
#49635=EDGE_CURVE('',#39176,#39178,#7290,.T.);
#49636=EDGE_CURVE('',#39175,#39177,#7291,.T.);
#49637=EDGE_CURVE('',#39178,#39173,#7292,.T.);
#49638=EDGE_CURVE('',#39177,#39174,#7293,.T.);
#49639=EDGE_CURVE('',#39179,#39180,#7294,.T.);
#49640=EDGE_CURVE('',#39181,#39180,#7295,.T.);
#49641=EDGE_CURVE('',#39182,#39181,#7296,.T.);
#49642=EDGE_CURVE('',#39182,#39179,#7297,.T.);
#49643=EDGE_CURVE('',#39183,#39184,#7298,.T.);
#49644=EDGE_CURVE('',#39180,#39184,#7299,.T.);
#49645=EDGE_CURVE('',#39179,#39183,#7300,.T.);
#49646=EDGE_CURVE('',#39185,#39186,#7301,.T.);
#49647=EDGE_CURVE('',#39184,#39186,#7302,.T.);
#49648=EDGE_CURVE('',#39183,#39185,#7303,.T.);
#49649=EDGE_CURVE('',#39186,#39181,#7304,.T.);
#49650=EDGE_CURVE('',#39185,#39182,#7305,.T.);
#49651=EDGE_CURVE('',#39187,#39188,#7306,.T.);
#49652=EDGE_CURVE('',#39189,#39188,#7307,.T.);
#49653=EDGE_CURVE('',#39190,#39189,#7308,.T.);
#49654=EDGE_CURVE('',#39190,#39187,#7309,.T.);
#49655=EDGE_CURVE('',#39191,#39192,#7310,.T.);
#49656=EDGE_CURVE('',#39188,#39192,#7311,.T.);
#49657=EDGE_CURVE('',#39187,#39191,#7312,.T.);
#49658=EDGE_CURVE('',#39193,#39194,#7313,.T.);
#49659=EDGE_CURVE('',#39192,#39194,#7314,.T.);
#49660=EDGE_CURVE('',#39191,#39193,#7315,.T.);
#49661=EDGE_CURVE('',#39194,#39189,#7316,.T.);
#49662=EDGE_CURVE('',#39193,#39190,#7317,.T.);
#49663=EDGE_CURVE('',#39195,#39196,#7318,.T.);
#49664=EDGE_CURVE('',#39197,#39196,#7319,.T.);
#49665=EDGE_CURVE('',#39198,#39197,#7320,.T.);
#49666=EDGE_CURVE('',#39198,#39195,#7321,.T.);
#49667=EDGE_CURVE('',#39199,#39200,#7322,.T.);
#49668=EDGE_CURVE('',#39196,#39200,#7323,.T.);
#49669=EDGE_CURVE('',#39195,#39199,#7324,.T.);
#49670=EDGE_CURVE('',#39201,#39202,#7325,.T.);
#49671=EDGE_CURVE('',#39200,#39202,#7326,.T.);
#49672=EDGE_CURVE('',#39199,#39201,#7327,.T.);
#49673=EDGE_CURVE('',#39202,#39197,#7328,.T.);
#49674=EDGE_CURVE('',#39201,#39198,#7329,.T.);
#49675=EDGE_CURVE('',#39203,#39204,#7330,.T.);
#49676=EDGE_CURVE('',#39205,#39204,#7331,.T.);
#49677=EDGE_CURVE('',#39206,#39205,#7332,.T.);
#49678=EDGE_CURVE('',#39206,#39203,#7333,.T.);
#49679=EDGE_CURVE('',#39207,#39208,#7334,.T.);
#49680=EDGE_CURVE('',#39204,#39208,#7335,.T.);
#49681=EDGE_CURVE('',#39203,#39207,#7336,.T.);
#49682=EDGE_CURVE('',#39209,#39210,#7337,.T.);
#49683=EDGE_CURVE('',#39208,#39210,#7338,.T.);
#49684=EDGE_CURVE('',#39207,#39209,#7339,.T.);
#49685=EDGE_CURVE('',#39210,#39205,#7340,.T.);
#49686=EDGE_CURVE('',#39209,#39206,#7341,.T.);
#49687=EDGE_CURVE('',#39211,#39212,#7342,.T.);
#49688=EDGE_CURVE('',#39213,#39212,#7343,.T.);
#49689=EDGE_CURVE('',#39214,#39213,#7344,.T.);
#49690=EDGE_CURVE('',#39214,#39211,#7345,.T.);
#49691=EDGE_CURVE('',#39215,#39216,#7346,.T.);
#49692=EDGE_CURVE('',#39212,#39216,#7347,.T.);
#49693=EDGE_CURVE('',#39211,#39215,#7348,.T.);
#49694=EDGE_CURVE('',#39217,#39218,#7349,.T.);
#49695=EDGE_CURVE('',#39216,#39218,#7350,.T.);
#49696=EDGE_CURVE('',#39215,#39217,#7351,.T.);
#49697=EDGE_CURVE('',#39218,#39213,#7352,.T.);
#49698=EDGE_CURVE('',#39217,#39214,#7353,.T.);
#49699=EDGE_CURVE('',#39219,#39220,#7354,.T.);
#49700=EDGE_CURVE('',#39221,#39220,#7355,.T.);
#49701=EDGE_CURVE('',#39222,#39221,#7356,.T.);
#49702=EDGE_CURVE('',#39222,#39219,#7357,.T.);
#49703=EDGE_CURVE('',#39223,#39224,#7358,.T.);
#49704=EDGE_CURVE('',#39220,#39224,#7359,.T.);
#49705=EDGE_CURVE('',#39219,#39223,#7360,.T.);
#49706=EDGE_CURVE('',#39225,#39226,#7361,.T.);
#49707=EDGE_CURVE('',#39224,#39226,#7362,.T.);
#49708=EDGE_CURVE('',#39223,#39225,#7363,.T.);
#49709=EDGE_CURVE('',#39226,#39221,#7364,.T.);
#49710=EDGE_CURVE('',#39225,#39222,#7365,.T.);
#49711=EDGE_CURVE('',#39227,#39228,#7366,.T.);
#49712=EDGE_CURVE('',#39229,#39228,#7367,.T.);
#49713=EDGE_CURVE('',#39230,#39229,#7368,.T.);
#49714=EDGE_CURVE('',#39230,#39227,#7369,.T.);
#49715=EDGE_CURVE('',#39231,#39232,#7370,.T.);
#49716=EDGE_CURVE('',#39228,#39232,#7371,.T.);
#49717=EDGE_CURVE('',#39227,#39231,#7372,.T.);
#49718=EDGE_CURVE('',#39233,#39234,#7373,.T.);
#49719=EDGE_CURVE('',#39232,#39234,#7374,.T.);
#49720=EDGE_CURVE('',#39231,#39233,#7375,.T.);
#49721=EDGE_CURVE('',#39234,#39229,#7376,.T.);
#49722=EDGE_CURVE('',#39233,#39230,#7377,.T.);
#49723=EDGE_CURVE('',#39235,#39236,#7378,.T.);
#49724=EDGE_CURVE('',#39237,#39236,#7379,.T.);
#49725=EDGE_CURVE('',#39238,#39237,#7380,.T.);
#49726=EDGE_CURVE('',#39238,#39235,#7381,.T.);
#49727=EDGE_CURVE('',#39239,#39240,#7382,.T.);
#49728=EDGE_CURVE('',#39236,#39240,#7383,.T.);
#49729=EDGE_CURVE('',#39235,#39239,#7384,.T.);
#49730=EDGE_CURVE('',#39241,#39242,#7385,.T.);
#49731=EDGE_CURVE('',#39240,#39242,#7386,.T.);
#49732=EDGE_CURVE('',#39239,#39241,#7387,.T.);
#49733=EDGE_CURVE('',#39242,#39237,#7388,.T.);
#49734=EDGE_CURVE('',#39241,#39238,#7389,.T.);
#49735=EDGE_CURVE('',#39243,#39244,#7390,.T.);
#49736=EDGE_CURVE('',#39245,#39244,#7391,.T.);
#49737=EDGE_CURVE('',#39246,#39245,#7392,.T.);
#49738=EDGE_CURVE('',#39246,#39243,#7393,.T.);
#49739=EDGE_CURVE('',#39247,#39248,#7394,.T.);
#49740=EDGE_CURVE('',#39244,#39248,#7395,.T.);
#49741=EDGE_CURVE('',#39243,#39247,#7396,.T.);
#49742=EDGE_CURVE('',#39249,#39250,#7397,.T.);
#49743=EDGE_CURVE('',#39248,#39250,#7398,.T.);
#49744=EDGE_CURVE('',#39247,#39249,#7399,.T.);
#49745=EDGE_CURVE('',#39250,#39245,#7400,.T.);
#49746=EDGE_CURVE('',#39249,#39246,#7401,.T.);
#49747=EDGE_CURVE('',#39251,#39252,#7402,.T.);
#49748=EDGE_CURVE('',#39253,#39252,#7403,.T.);
#49749=EDGE_CURVE('',#39254,#39253,#7404,.T.);
#49750=EDGE_CURVE('',#39254,#39251,#7405,.T.);
#49751=EDGE_CURVE('',#39255,#39256,#7406,.T.);
#49752=EDGE_CURVE('',#39252,#39256,#7407,.T.);
#49753=EDGE_CURVE('',#39251,#39255,#7408,.T.);
#49754=EDGE_CURVE('',#39257,#39258,#7409,.T.);
#49755=EDGE_CURVE('',#39256,#39258,#7410,.T.);
#49756=EDGE_CURVE('',#39255,#39257,#7411,.T.);
#49757=EDGE_CURVE('',#39258,#39253,#7412,.T.);
#49758=EDGE_CURVE('',#39257,#39254,#7413,.T.);
#49759=EDGE_CURVE('',#39259,#39260,#7414,.T.);
#49760=EDGE_CURVE('',#39261,#39260,#7415,.T.);
#49761=EDGE_CURVE('',#39262,#39261,#7416,.T.);
#49762=EDGE_CURVE('',#39262,#39259,#7417,.T.);
#49763=EDGE_CURVE('',#39263,#39264,#7418,.T.);
#49764=EDGE_CURVE('',#39260,#39264,#7419,.T.);
#49765=EDGE_CURVE('',#39259,#39263,#7420,.T.);
#49766=EDGE_CURVE('',#39265,#39266,#7421,.T.);
#49767=EDGE_CURVE('',#39264,#39266,#7422,.T.);
#49768=EDGE_CURVE('',#39263,#39265,#7423,.T.);
#49769=EDGE_CURVE('',#39266,#39261,#7424,.T.);
#49770=EDGE_CURVE('',#39265,#39262,#7425,.T.);
#49771=EDGE_CURVE('',#39267,#39268,#7426,.T.);
#49772=EDGE_CURVE('',#39269,#39268,#7427,.T.);
#49773=EDGE_CURVE('',#39270,#39269,#7428,.T.);
#49774=EDGE_CURVE('',#39270,#39267,#7429,.T.);
#49775=EDGE_CURVE('',#39271,#39272,#7430,.T.);
#49776=EDGE_CURVE('',#39268,#39272,#7431,.T.);
#49777=EDGE_CURVE('',#39267,#39271,#7432,.T.);
#49778=EDGE_CURVE('',#39273,#39274,#7433,.T.);
#49779=EDGE_CURVE('',#39272,#39274,#7434,.T.);
#49780=EDGE_CURVE('',#39271,#39273,#7435,.T.);
#49781=EDGE_CURVE('',#39274,#39269,#7436,.T.);
#49782=EDGE_CURVE('',#39273,#39270,#7437,.T.);
#49783=EDGE_CURVE('',#39275,#39276,#7438,.T.);
#49784=EDGE_CURVE('',#39277,#39276,#7439,.T.);
#49785=EDGE_CURVE('',#39278,#39277,#7440,.T.);
#49786=EDGE_CURVE('',#39278,#39275,#7441,.T.);
#49787=EDGE_CURVE('',#39279,#39280,#7442,.T.);
#49788=EDGE_CURVE('',#39276,#39280,#7443,.T.);
#49789=EDGE_CURVE('',#39275,#39279,#7444,.T.);
#49790=EDGE_CURVE('',#39281,#39282,#7445,.T.);
#49791=EDGE_CURVE('',#39280,#39282,#7446,.T.);
#49792=EDGE_CURVE('',#39279,#39281,#7447,.T.);
#49793=EDGE_CURVE('',#39282,#39277,#7448,.T.);
#49794=EDGE_CURVE('',#39281,#39278,#7449,.T.);
#49795=EDGE_CURVE('',#39283,#39284,#7450,.T.);
#49796=EDGE_CURVE('',#39285,#39284,#7451,.T.);
#49797=EDGE_CURVE('',#39286,#39285,#7452,.T.);
#49798=EDGE_CURVE('',#39286,#39283,#7453,.T.);
#49799=EDGE_CURVE('',#39287,#39288,#7454,.T.);
#49800=EDGE_CURVE('',#39284,#39288,#7455,.T.);
#49801=EDGE_CURVE('',#39283,#39287,#7456,.T.);
#49802=EDGE_CURVE('',#39289,#39290,#7457,.T.);
#49803=EDGE_CURVE('',#39288,#39290,#7458,.T.);
#49804=EDGE_CURVE('',#39287,#39289,#7459,.T.);
#49805=EDGE_CURVE('',#39290,#39285,#7460,.T.);
#49806=EDGE_CURVE('',#39289,#39286,#7461,.T.);
#49807=EDGE_CURVE('',#39291,#39292,#7462,.T.);
#49808=EDGE_CURVE('',#39293,#39292,#7463,.T.);
#49809=EDGE_CURVE('',#39294,#39293,#7464,.T.);
#49810=EDGE_CURVE('',#39294,#39291,#7465,.T.);
#49811=EDGE_CURVE('',#39295,#39296,#7466,.T.);
#49812=EDGE_CURVE('',#39292,#39296,#7467,.T.);
#49813=EDGE_CURVE('',#39291,#39295,#7468,.T.);
#49814=EDGE_CURVE('',#39297,#39298,#7469,.T.);
#49815=EDGE_CURVE('',#39296,#39298,#7470,.T.);
#49816=EDGE_CURVE('',#39295,#39297,#7471,.T.);
#49817=EDGE_CURVE('',#39298,#39293,#7472,.T.);
#49818=EDGE_CURVE('',#39297,#39294,#7473,.T.);
#49819=EDGE_CURVE('',#39299,#39300,#7474,.T.);
#49820=EDGE_CURVE('',#39301,#39300,#7475,.T.);
#49821=EDGE_CURVE('',#39302,#39301,#7476,.T.);
#49822=EDGE_CURVE('',#39302,#39299,#7477,.T.);
#49823=EDGE_CURVE('',#39303,#39304,#7478,.T.);
#49824=EDGE_CURVE('',#39300,#39304,#7479,.T.);
#49825=EDGE_CURVE('',#39299,#39303,#7480,.T.);
#49826=EDGE_CURVE('',#39305,#39306,#7481,.T.);
#49827=EDGE_CURVE('',#39304,#39306,#7482,.T.);
#49828=EDGE_CURVE('',#39303,#39305,#7483,.T.);
#49829=EDGE_CURVE('',#39306,#39301,#7484,.T.);
#49830=EDGE_CURVE('',#39305,#39302,#7485,.T.);
#49831=EDGE_CURVE('',#39307,#39308,#7486,.T.);
#49832=EDGE_CURVE('',#39309,#39308,#7487,.T.);
#49833=EDGE_CURVE('',#39310,#39309,#7488,.T.);
#49834=EDGE_CURVE('',#39310,#39307,#7489,.T.);
#49835=EDGE_CURVE('',#39311,#39312,#7490,.T.);
#49836=EDGE_CURVE('',#39308,#39312,#7491,.T.);
#49837=EDGE_CURVE('',#39307,#39311,#7492,.T.);
#49838=EDGE_CURVE('',#39313,#39314,#7493,.T.);
#49839=EDGE_CURVE('',#39312,#39314,#7494,.T.);
#49840=EDGE_CURVE('',#39311,#39313,#7495,.T.);
#49841=EDGE_CURVE('',#39314,#39309,#7496,.T.);
#49842=EDGE_CURVE('',#39313,#39310,#7497,.T.);
#49843=EDGE_CURVE('',#39315,#39316,#7498,.T.);
#49844=EDGE_CURVE('',#39317,#39316,#7499,.T.);
#49845=EDGE_CURVE('',#39318,#39317,#7500,.T.);
#49846=EDGE_CURVE('',#39318,#39315,#7501,.T.);
#49847=EDGE_CURVE('',#39319,#39320,#7502,.T.);
#49848=EDGE_CURVE('',#39316,#39320,#7503,.T.);
#49849=EDGE_CURVE('',#39315,#39319,#7504,.T.);
#49850=EDGE_CURVE('',#39321,#39322,#7505,.T.);
#49851=EDGE_CURVE('',#39320,#39322,#7506,.T.);
#49852=EDGE_CURVE('',#39319,#39321,#7507,.T.);
#49853=EDGE_CURVE('',#39322,#39317,#7508,.T.);
#49854=EDGE_CURVE('',#39321,#39318,#7509,.T.);
#49855=EDGE_CURVE('',#39323,#39324,#7510,.T.);
#49856=EDGE_CURVE('',#39325,#39324,#7511,.T.);
#49857=EDGE_CURVE('',#39326,#39325,#7512,.T.);
#49858=EDGE_CURVE('',#39326,#39323,#7513,.T.);
#49859=EDGE_CURVE('',#39327,#39328,#7514,.T.);
#49860=EDGE_CURVE('',#39324,#39328,#7515,.T.);
#49861=EDGE_CURVE('',#39323,#39327,#7516,.T.);
#49862=EDGE_CURVE('',#39329,#39330,#7517,.T.);
#49863=EDGE_CURVE('',#39328,#39330,#7518,.T.);
#49864=EDGE_CURVE('',#39327,#39329,#7519,.T.);
#49865=EDGE_CURVE('',#39330,#39325,#7520,.T.);
#49866=EDGE_CURVE('',#39329,#39326,#7521,.T.);
#49867=EDGE_CURVE('',#39331,#39332,#7522,.T.);
#49868=EDGE_CURVE('',#39333,#39332,#7523,.T.);
#49869=EDGE_CURVE('',#39334,#39333,#7524,.T.);
#49870=EDGE_CURVE('',#39334,#39331,#7525,.T.);
#49871=EDGE_CURVE('',#39335,#39336,#7526,.T.);
#49872=EDGE_CURVE('',#39332,#39336,#7527,.T.);
#49873=EDGE_CURVE('',#39331,#39335,#7528,.T.);
#49874=EDGE_CURVE('',#39337,#39338,#7529,.T.);
#49875=EDGE_CURVE('',#39336,#39338,#7530,.T.);
#49876=EDGE_CURVE('',#39335,#39337,#7531,.T.);
#49877=EDGE_CURVE('',#39338,#39333,#7532,.T.);
#49878=EDGE_CURVE('',#39337,#39334,#7533,.T.);
#49879=EDGE_CURVE('',#39339,#39340,#7534,.T.);
#49880=EDGE_CURVE('',#39341,#39340,#7535,.T.);
#49881=EDGE_CURVE('',#39342,#39341,#7536,.T.);
#49882=EDGE_CURVE('',#39342,#39339,#7537,.T.);
#49883=EDGE_CURVE('',#39343,#39344,#7538,.T.);
#49884=EDGE_CURVE('',#39340,#39344,#7539,.T.);
#49885=EDGE_CURVE('',#39339,#39343,#7540,.T.);
#49886=EDGE_CURVE('',#39345,#39346,#7541,.T.);
#49887=EDGE_CURVE('',#39344,#39346,#7542,.T.);
#49888=EDGE_CURVE('',#39343,#39345,#7543,.T.);
#49889=EDGE_CURVE('',#39346,#39341,#7544,.T.);
#49890=EDGE_CURVE('',#39345,#39342,#7545,.T.);
#49891=EDGE_CURVE('',#39347,#39348,#7546,.T.);
#49892=EDGE_CURVE('',#39349,#39348,#7547,.T.);
#49893=EDGE_CURVE('',#39350,#39349,#7548,.T.);
#49894=EDGE_CURVE('',#39350,#39347,#7549,.T.);
#49895=EDGE_CURVE('',#39351,#39352,#7550,.T.);
#49896=EDGE_CURVE('',#39348,#39352,#7551,.T.);
#49897=EDGE_CURVE('',#39347,#39351,#7552,.T.);
#49898=EDGE_CURVE('',#39353,#39354,#7553,.T.);
#49899=EDGE_CURVE('',#39352,#39354,#7554,.T.);
#49900=EDGE_CURVE('',#39351,#39353,#7555,.T.);
#49901=EDGE_CURVE('',#39354,#39349,#7556,.T.);
#49902=EDGE_CURVE('',#39353,#39350,#7557,.T.);
#49903=EDGE_CURVE('',#39355,#39356,#7558,.T.);
#49904=EDGE_CURVE('',#39357,#39356,#7559,.T.);
#49905=EDGE_CURVE('',#39358,#39357,#7560,.T.);
#49906=EDGE_CURVE('',#39358,#39355,#7561,.T.);
#49907=EDGE_CURVE('',#39359,#39360,#7562,.T.);
#49908=EDGE_CURVE('',#39356,#39360,#7563,.T.);
#49909=EDGE_CURVE('',#39355,#39359,#7564,.T.);
#49910=EDGE_CURVE('',#39361,#39362,#7565,.T.);
#49911=EDGE_CURVE('',#39360,#39362,#7566,.T.);
#49912=EDGE_CURVE('',#39359,#39361,#7567,.T.);
#49913=EDGE_CURVE('',#39362,#39357,#7568,.T.);
#49914=EDGE_CURVE('',#39361,#39358,#7569,.T.);
#49915=EDGE_CURVE('',#39363,#39364,#7570,.T.);
#49916=EDGE_CURVE('',#39365,#39364,#7571,.T.);
#49917=EDGE_CURVE('',#39366,#39365,#7572,.T.);
#49918=EDGE_CURVE('',#39366,#39363,#7573,.T.);
#49919=EDGE_CURVE('',#39367,#39368,#7574,.T.);
#49920=EDGE_CURVE('',#39364,#39368,#7575,.T.);
#49921=EDGE_CURVE('',#39363,#39367,#7576,.T.);
#49922=EDGE_CURVE('',#39369,#39370,#7577,.T.);
#49923=EDGE_CURVE('',#39368,#39370,#7578,.T.);
#49924=EDGE_CURVE('',#39367,#39369,#7579,.T.);
#49925=EDGE_CURVE('',#39370,#39365,#7580,.T.);
#49926=EDGE_CURVE('',#39369,#39366,#7581,.T.);
#49927=EDGE_CURVE('',#39371,#39372,#7582,.T.);
#49928=EDGE_CURVE('',#39373,#39372,#7583,.T.);
#49929=EDGE_CURVE('',#39374,#39373,#7584,.T.);
#49930=EDGE_CURVE('',#39374,#39371,#7585,.T.);
#49931=EDGE_CURVE('',#39375,#39376,#7586,.T.);
#49932=EDGE_CURVE('',#39372,#39376,#7587,.T.);
#49933=EDGE_CURVE('',#39371,#39375,#7588,.T.);
#49934=EDGE_CURVE('',#39377,#39378,#7589,.T.);
#49935=EDGE_CURVE('',#39376,#39378,#7590,.T.);
#49936=EDGE_CURVE('',#39375,#39377,#7591,.T.);
#49937=EDGE_CURVE('',#39378,#39373,#7592,.T.);
#49938=EDGE_CURVE('',#39377,#39374,#7593,.T.);
#49939=EDGE_CURVE('',#39379,#39380,#7594,.T.);
#49940=EDGE_CURVE('',#39381,#39380,#7595,.T.);
#49941=EDGE_CURVE('',#39382,#39381,#7596,.T.);
#49942=EDGE_CURVE('',#39382,#39379,#7597,.T.);
#49943=EDGE_CURVE('',#39383,#39384,#7598,.T.);
#49944=EDGE_CURVE('',#39380,#39384,#7599,.T.);
#49945=EDGE_CURVE('',#39379,#39383,#7600,.T.);
#49946=EDGE_CURVE('',#39385,#39386,#7601,.T.);
#49947=EDGE_CURVE('',#39384,#39386,#7602,.T.);
#49948=EDGE_CURVE('',#39383,#39385,#7603,.T.);
#49949=EDGE_CURVE('',#39386,#39381,#7604,.T.);
#49950=EDGE_CURVE('',#39385,#39382,#7605,.T.);
#49951=EDGE_CURVE('',#39387,#39388,#7606,.T.);
#49952=EDGE_CURVE('',#39389,#39388,#7607,.T.);
#49953=EDGE_CURVE('',#39390,#39389,#7608,.T.);
#49954=EDGE_CURVE('',#39390,#39387,#7609,.T.);
#49955=EDGE_CURVE('',#39391,#39392,#7610,.T.);
#49956=EDGE_CURVE('',#39388,#39392,#7611,.T.);
#49957=EDGE_CURVE('',#39387,#39391,#7612,.T.);
#49958=EDGE_CURVE('',#39393,#39394,#7613,.T.);
#49959=EDGE_CURVE('',#39392,#39394,#7614,.T.);
#49960=EDGE_CURVE('',#39391,#39393,#7615,.T.);
#49961=EDGE_CURVE('',#39394,#39389,#7616,.T.);
#49962=EDGE_CURVE('',#39393,#39390,#7617,.T.);
#49963=EDGE_CURVE('',#39395,#39396,#7618,.T.);
#49964=EDGE_CURVE('',#39397,#39396,#7619,.T.);
#49965=EDGE_CURVE('',#39398,#39397,#7620,.T.);
#49966=EDGE_CURVE('',#39398,#39395,#7621,.T.);
#49967=EDGE_CURVE('',#39399,#39400,#7622,.T.);
#49968=EDGE_CURVE('',#39396,#39400,#7623,.T.);
#49969=EDGE_CURVE('',#39395,#39399,#7624,.T.);
#49970=EDGE_CURVE('',#39401,#39402,#7625,.T.);
#49971=EDGE_CURVE('',#39400,#39402,#7626,.T.);
#49972=EDGE_CURVE('',#39399,#39401,#7627,.T.);
#49973=EDGE_CURVE('',#39402,#39397,#7628,.T.);
#49974=EDGE_CURVE('',#39401,#39398,#7629,.T.);
#49975=EDGE_CURVE('',#39403,#39404,#7630,.T.);
#49976=EDGE_CURVE('',#39405,#39404,#7631,.T.);
#49977=EDGE_CURVE('',#39406,#39405,#7632,.T.);
#49978=EDGE_CURVE('',#39406,#39403,#7633,.T.);
#49979=EDGE_CURVE('',#39407,#39408,#7634,.T.);
#49980=EDGE_CURVE('',#39404,#39408,#7635,.T.);
#49981=EDGE_CURVE('',#39403,#39407,#7636,.T.);
#49982=EDGE_CURVE('',#39409,#39410,#7637,.T.);
#49983=EDGE_CURVE('',#39408,#39410,#7638,.T.);
#49984=EDGE_CURVE('',#39407,#39409,#7639,.T.);
#49985=EDGE_CURVE('',#39410,#39405,#7640,.T.);
#49986=EDGE_CURVE('',#39409,#39406,#7641,.T.);
#49987=EDGE_CURVE('',#39411,#39412,#7642,.T.);
#49988=EDGE_CURVE('',#39413,#39412,#7643,.T.);
#49989=EDGE_CURVE('',#39414,#39413,#7644,.T.);
#49990=EDGE_CURVE('',#39414,#39411,#7645,.T.);
#49991=EDGE_CURVE('',#39415,#39416,#7646,.T.);
#49992=EDGE_CURVE('',#39412,#39416,#7647,.T.);
#49993=EDGE_CURVE('',#39411,#39415,#7648,.T.);
#49994=EDGE_CURVE('',#39417,#39418,#7649,.T.);
#49995=EDGE_CURVE('',#39416,#39418,#7650,.T.);
#49996=EDGE_CURVE('',#39415,#39417,#7651,.T.);
#49997=EDGE_CURVE('',#39418,#39413,#7652,.T.);
#49998=EDGE_CURVE('',#39417,#39414,#7653,.T.);
#49999=EDGE_CURVE('',#39419,#39420,#7654,.T.);
#50000=EDGE_CURVE('',#39421,#39420,#7655,.T.);
#50001=EDGE_CURVE('',#39422,#39421,#7656,.T.);
#50002=EDGE_CURVE('',#39422,#39419,#7657,.T.);
#50003=EDGE_CURVE('',#39423,#39424,#7658,.T.);
#50004=EDGE_CURVE('',#39420,#39424,#7659,.T.);
#50005=EDGE_CURVE('',#39419,#39423,#7660,.T.);
#50006=EDGE_CURVE('',#39425,#39426,#7661,.T.);
#50007=EDGE_CURVE('',#39424,#39426,#7662,.T.);
#50008=EDGE_CURVE('',#39423,#39425,#7663,.T.);
#50009=EDGE_CURVE('',#39426,#39421,#7664,.T.);
#50010=EDGE_CURVE('',#39425,#39422,#7665,.T.);
#50011=EDGE_CURVE('',#39427,#39428,#7666,.T.);
#50012=EDGE_CURVE('',#39429,#39428,#7667,.T.);
#50013=EDGE_CURVE('',#39430,#39429,#7668,.T.);
#50014=EDGE_CURVE('',#39430,#39427,#7669,.T.);
#50015=EDGE_CURVE('',#39431,#39432,#7670,.T.);
#50016=EDGE_CURVE('',#39428,#39432,#7671,.T.);
#50017=EDGE_CURVE('',#39427,#39431,#7672,.T.);
#50018=EDGE_CURVE('',#39433,#39434,#7673,.T.);
#50019=EDGE_CURVE('',#39432,#39434,#7674,.T.);
#50020=EDGE_CURVE('',#39431,#39433,#7675,.T.);
#50021=EDGE_CURVE('',#39434,#39429,#7676,.T.);
#50022=EDGE_CURVE('',#39433,#39430,#7677,.T.);
#50023=EDGE_CURVE('',#39435,#39436,#7678,.T.);
#50024=EDGE_CURVE('',#39437,#39436,#7679,.T.);
#50025=EDGE_CURVE('',#39438,#39437,#7680,.T.);
#50026=EDGE_CURVE('',#39438,#39435,#7681,.T.);
#50027=EDGE_CURVE('',#39439,#39440,#7682,.T.);
#50028=EDGE_CURVE('',#39436,#39440,#7683,.T.);
#50029=EDGE_CURVE('',#39435,#39439,#7684,.T.);
#50030=EDGE_CURVE('',#39441,#39442,#7685,.T.);
#50031=EDGE_CURVE('',#39440,#39442,#7686,.T.);
#50032=EDGE_CURVE('',#39439,#39441,#7687,.T.);
#50033=EDGE_CURVE('',#39442,#39437,#7688,.T.);
#50034=EDGE_CURVE('',#39441,#39438,#7689,.T.);
#50035=EDGE_CURVE('',#39443,#39444,#7690,.T.);
#50036=EDGE_CURVE('',#39445,#39444,#7691,.T.);
#50037=EDGE_CURVE('',#39446,#39445,#7692,.T.);
#50038=EDGE_CURVE('',#39446,#39443,#7693,.T.);
#50039=EDGE_CURVE('',#39447,#39448,#7694,.T.);
#50040=EDGE_CURVE('',#39444,#39448,#7695,.T.);
#50041=EDGE_CURVE('',#39443,#39447,#7696,.T.);
#50042=EDGE_CURVE('',#39449,#39450,#7697,.T.);
#50043=EDGE_CURVE('',#39448,#39450,#7698,.T.);
#50044=EDGE_CURVE('',#39447,#39449,#7699,.T.);
#50045=EDGE_CURVE('',#39450,#39445,#7700,.T.);
#50046=EDGE_CURVE('',#39449,#39446,#7701,.T.);
#50047=EDGE_CURVE('',#39451,#39452,#7702,.T.);
#50048=EDGE_CURVE('',#39453,#39452,#7703,.T.);
#50049=EDGE_CURVE('',#39454,#39453,#7704,.T.);
#50050=EDGE_CURVE('',#39454,#39451,#7705,.T.);
#50051=EDGE_CURVE('',#39455,#39456,#7706,.T.);
#50052=EDGE_CURVE('',#39452,#39456,#7707,.T.);
#50053=EDGE_CURVE('',#39451,#39455,#7708,.T.);
#50054=EDGE_CURVE('',#39457,#39458,#7709,.T.);
#50055=EDGE_CURVE('',#39456,#39458,#7710,.T.);
#50056=EDGE_CURVE('',#39455,#39457,#7711,.T.);
#50057=EDGE_CURVE('',#39458,#39453,#7712,.T.);
#50058=EDGE_CURVE('',#39457,#39454,#7713,.T.);
#50059=EDGE_CURVE('',#39459,#39460,#7714,.T.);
#50060=EDGE_CURVE('',#39461,#39460,#7715,.T.);
#50061=EDGE_CURVE('',#39462,#39461,#7716,.T.);
#50062=EDGE_CURVE('',#39462,#39459,#7717,.T.);
#50063=EDGE_CURVE('',#39463,#39464,#7718,.T.);
#50064=EDGE_CURVE('',#39460,#39464,#7719,.T.);
#50065=EDGE_CURVE('',#39459,#39463,#7720,.T.);
#50066=EDGE_CURVE('',#39465,#39466,#7721,.T.);
#50067=EDGE_CURVE('',#39464,#39466,#7722,.T.);
#50068=EDGE_CURVE('',#39463,#39465,#7723,.T.);
#50069=EDGE_CURVE('',#39466,#39461,#7724,.T.);
#50070=EDGE_CURVE('',#39465,#39462,#7725,.T.);
#50071=EDGE_CURVE('',#39467,#39468,#7726,.T.);
#50072=EDGE_CURVE('',#39469,#39468,#7727,.T.);
#50073=EDGE_CURVE('',#39470,#39469,#7728,.T.);
#50074=EDGE_CURVE('',#39470,#39467,#7729,.T.);
#50075=EDGE_CURVE('',#39471,#39472,#7730,.T.);
#50076=EDGE_CURVE('',#39468,#39472,#7731,.T.);
#50077=EDGE_CURVE('',#39467,#39471,#7732,.T.);
#50078=EDGE_CURVE('',#39473,#39474,#7733,.T.);
#50079=EDGE_CURVE('',#39472,#39474,#7734,.T.);
#50080=EDGE_CURVE('',#39471,#39473,#7735,.T.);
#50081=EDGE_CURVE('',#39474,#39469,#7736,.T.);
#50082=EDGE_CURVE('',#39473,#39470,#7737,.T.);
#50083=EDGE_CURVE('',#39475,#39476,#7738,.T.);
#50084=EDGE_CURVE('',#39477,#39476,#7739,.T.);
#50085=EDGE_CURVE('',#39478,#39477,#7740,.T.);
#50086=EDGE_CURVE('',#39478,#39475,#7741,.T.);
#50087=EDGE_CURVE('',#39479,#39480,#7742,.T.);
#50088=EDGE_CURVE('',#39476,#39480,#7743,.T.);
#50089=EDGE_CURVE('',#39475,#39479,#7744,.T.);
#50090=EDGE_CURVE('',#39481,#39482,#7745,.T.);
#50091=EDGE_CURVE('',#39480,#39482,#7746,.T.);
#50092=EDGE_CURVE('',#39479,#39481,#7747,.T.);
#50093=EDGE_CURVE('',#39482,#39477,#7748,.T.);
#50094=EDGE_CURVE('',#39481,#39478,#7749,.T.);
#50095=EDGE_CURVE('',#39483,#39484,#7750,.T.);
#50096=EDGE_CURVE('',#39485,#39484,#7751,.T.);
#50097=EDGE_CURVE('',#39486,#39485,#7752,.T.);
#50098=EDGE_CURVE('',#39486,#39483,#7753,.T.);
#50099=EDGE_CURVE('',#39487,#39488,#7754,.T.);
#50100=EDGE_CURVE('',#39484,#39488,#7755,.T.);
#50101=EDGE_CURVE('',#39483,#39487,#7756,.T.);
#50102=EDGE_CURVE('',#39489,#39490,#7757,.T.);
#50103=EDGE_CURVE('',#39488,#39490,#7758,.T.);
#50104=EDGE_CURVE('',#39487,#39489,#7759,.T.);
#50105=EDGE_CURVE('',#39490,#39485,#7760,.T.);
#50106=EDGE_CURVE('',#39489,#39486,#7761,.T.);
#50107=EDGE_CURVE('',#39491,#39492,#7762,.T.);
#50108=EDGE_CURVE('',#39493,#39492,#7763,.T.);
#50109=EDGE_CURVE('',#39494,#39493,#7764,.T.);
#50110=EDGE_CURVE('',#39494,#39491,#7765,.T.);
#50111=EDGE_CURVE('',#39495,#39496,#7766,.T.);
#50112=EDGE_CURVE('',#39492,#39496,#7767,.T.);
#50113=EDGE_CURVE('',#39491,#39495,#7768,.T.);
#50114=EDGE_CURVE('',#39497,#39498,#7769,.T.);
#50115=EDGE_CURVE('',#39496,#39498,#7770,.T.);
#50116=EDGE_CURVE('',#39495,#39497,#7771,.T.);
#50117=EDGE_CURVE('',#39498,#39493,#7772,.T.);
#50118=EDGE_CURVE('',#39497,#39494,#7773,.T.);
#50119=EDGE_CURVE('',#39499,#39500,#7774,.T.);
#50120=EDGE_CURVE('',#39501,#39500,#7775,.T.);
#50121=EDGE_CURVE('',#39502,#39501,#7776,.T.);
#50122=EDGE_CURVE('',#39502,#39499,#7777,.T.);
#50123=EDGE_CURVE('',#39503,#39504,#7778,.T.);
#50124=EDGE_CURVE('',#39500,#39504,#7779,.T.);
#50125=EDGE_CURVE('',#39499,#39503,#7780,.T.);
#50126=EDGE_CURVE('',#39505,#39506,#7781,.T.);
#50127=EDGE_CURVE('',#39504,#39506,#7782,.T.);
#50128=EDGE_CURVE('',#39503,#39505,#7783,.T.);
#50129=EDGE_CURVE('',#39506,#39501,#7784,.T.);
#50130=EDGE_CURVE('',#39505,#39502,#7785,.T.);
#50131=EDGE_CURVE('',#39507,#39508,#7786,.T.);
#50132=EDGE_CURVE('',#39509,#39508,#7787,.T.);
#50133=EDGE_CURVE('',#39510,#39509,#7788,.T.);
#50134=EDGE_CURVE('',#39510,#39507,#7789,.T.);
#50135=EDGE_CURVE('',#39511,#39512,#7790,.T.);
#50136=EDGE_CURVE('',#39508,#39512,#7791,.T.);
#50137=EDGE_CURVE('',#39507,#39511,#7792,.T.);
#50138=EDGE_CURVE('',#39513,#39514,#7793,.T.);
#50139=EDGE_CURVE('',#39512,#39514,#7794,.T.);
#50140=EDGE_CURVE('',#39511,#39513,#7795,.T.);
#50141=EDGE_CURVE('',#39514,#39509,#7796,.T.);
#50142=EDGE_CURVE('',#39513,#39510,#7797,.T.);
#50143=EDGE_CURVE('',#39515,#39516,#7798,.T.);
#50144=EDGE_CURVE('',#39517,#39516,#7799,.T.);
#50145=EDGE_CURVE('',#39518,#39517,#7800,.T.);
#50146=EDGE_CURVE('',#39518,#39515,#7801,.T.);
#50147=EDGE_CURVE('',#39519,#39520,#7802,.T.);
#50148=EDGE_CURVE('',#39516,#39520,#7803,.T.);
#50149=EDGE_CURVE('',#39515,#39519,#7804,.T.);
#50150=EDGE_CURVE('',#39521,#39522,#7805,.T.);
#50151=EDGE_CURVE('',#39520,#39522,#7806,.T.);
#50152=EDGE_CURVE('',#39519,#39521,#7807,.T.);
#50153=EDGE_CURVE('',#39522,#39517,#7808,.T.);
#50154=EDGE_CURVE('',#39521,#39518,#7809,.T.);
#50155=EDGE_CURVE('',#39523,#39524,#7810,.T.);
#50156=EDGE_CURVE('',#39525,#39524,#7811,.T.);
#50157=EDGE_CURVE('',#39526,#39525,#7812,.T.);
#50158=EDGE_CURVE('',#39526,#39523,#7813,.T.);
#50159=EDGE_CURVE('',#39527,#39528,#7814,.T.);
#50160=EDGE_CURVE('',#39524,#39528,#7815,.T.);
#50161=EDGE_CURVE('',#39523,#39527,#7816,.T.);
#50162=EDGE_CURVE('',#39529,#39530,#7817,.T.);
#50163=EDGE_CURVE('',#39528,#39530,#7818,.T.);
#50164=EDGE_CURVE('',#39527,#39529,#7819,.T.);
#50165=EDGE_CURVE('',#39530,#39525,#7820,.T.);
#50166=EDGE_CURVE('',#39529,#39526,#7821,.T.);
#50167=EDGE_CURVE('',#39531,#39532,#7822,.T.);
#50168=EDGE_CURVE('',#39533,#39532,#7823,.T.);
#50169=EDGE_CURVE('',#39534,#39533,#7824,.T.);
#50170=EDGE_CURVE('',#39534,#39531,#7825,.T.);
#50171=EDGE_CURVE('',#39535,#39536,#7826,.T.);
#50172=EDGE_CURVE('',#39532,#39536,#7827,.T.);
#50173=EDGE_CURVE('',#39531,#39535,#7828,.T.);
#50174=EDGE_CURVE('',#39537,#39538,#7829,.T.);
#50175=EDGE_CURVE('',#39536,#39538,#7830,.T.);
#50176=EDGE_CURVE('',#39535,#39537,#7831,.T.);
#50177=EDGE_CURVE('',#39538,#39533,#7832,.T.);
#50178=EDGE_CURVE('',#39537,#39534,#7833,.T.);
#50179=EDGE_CURVE('',#39539,#39540,#7834,.T.);
#50180=EDGE_CURVE('',#39541,#39540,#7835,.T.);
#50181=EDGE_CURVE('',#39542,#39541,#7836,.T.);
#50182=EDGE_CURVE('',#39542,#39539,#7837,.T.);
#50183=EDGE_CURVE('',#39543,#39544,#7838,.T.);
#50184=EDGE_CURVE('',#39540,#39544,#7839,.T.);
#50185=EDGE_CURVE('',#39539,#39543,#7840,.T.);
#50186=EDGE_CURVE('',#39545,#39546,#7841,.T.);
#50187=EDGE_CURVE('',#39544,#39546,#7842,.T.);
#50188=EDGE_CURVE('',#39543,#39545,#7843,.T.);
#50189=EDGE_CURVE('',#39546,#39541,#7844,.T.);
#50190=EDGE_CURVE('',#39545,#39542,#7845,.T.);
#50191=EDGE_CURVE('',#39547,#39548,#7846,.T.);
#50192=EDGE_CURVE('',#39549,#39548,#7847,.T.);
#50193=EDGE_CURVE('',#39550,#39549,#7848,.T.);
#50194=EDGE_CURVE('',#39550,#39547,#7849,.T.);
#50195=EDGE_CURVE('',#39551,#39552,#7850,.T.);
#50196=EDGE_CURVE('',#39548,#39552,#7851,.T.);
#50197=EDGE_CURVE('',#39547,#39551,#7852,.T.);
#50198=EDGE_CURVE('',#39553,#39554,#7853,.T.);
#50199=EDGE_CURVE('',#39552,#39554,#7854,.T.);
#50200=EDGE_CURVE('',#39551,#39553,#7855,.T.);
#50201=EDGE_CURVE('',#39554,#39549,#7856,.T.);
#50202=EDGE_CURVE('',#39553,#39550,#7857,.T.);
#50203=EDGE_CURVE('',#39555,#39556,#7858,.T.);
#50204=EDGE_CURVE('',#39557,#39556,#7859,.T.);
#50205=EDGE_CURVE('',#39558,#39557,#7860,.T.);
#50206=EDGE_CURVE('',#39558,#39555,#7861,.T.);
#50207=EDGE_CURVE('',#39559,#39560,#7862,.T.);
#50208=EDGE_CURVE('',#39556,#39560,#7863,.T.);
#50209=EDGE_CURVE('',#39555,#39559,#7864,.T.);
#50210=EDGE_CURVE('',#39561,#39562,#7865,.T.);
#50211=EDGE_CURVE('',#39560,#39562,#7866,.T.);
#50212=EDGE_CURVE('',#39559,#39561,#7867,.T.);
#50213=EDGE_CURVE('',#39562,#39557,#7868,.T.);
#50214=EDGE_CURVE('',#39561,#39558,#7869,.T.);
#50215=EDGE_CURVE('',#39563,#39564,#7870,.T.);
#50216=EDGE_CURVE('',#39565,#39564,#7871,.T.);
#50217=EDGE_CURVE('',#39566,#39565,#7872,.T.);
#50218=EDGE_CURVE('',#39566,#39563,#7873,.T.);
#50219=EDGE_CURVE('',#39567,#39568,#7874,.T.);
#50220=EDGE_CURVE('',#39564,#39568,#7875,.T.);
#50221=EDGE_CURVE('',#39563,#39567,#7876,.T.);
#50222=EDGE_CURVE('',#39569,#39570,#7877,.T.);
#50223=EDGE_CURVE('',#39568,#39570,#7878,.T.);
#50224=EDGE_CURVE('',#39567,#39569,#7879,.T.);
#50225=EDGE_CURVE('',#39570,#39565,#7880,.T.);
#50226=EDGE_CURVE('',#39569,#39566,#7881,.T.);
#50227=EDGE_CURVE('',#39571,#39572,#7882,.T.);
#50228=EDGE_CURVE('',#39573,#39572,#7883,.T.);
#50229=EDGE_CURVE('',#39574,#39573,#7884,.T.);
#50230=EDGE_CURVE('',#39574,#39571,#7885,.T.);
#50231=EDGE_CURVE('',#39575,#39576,#7886,.T.);
#50232=EDGE_CURVE('',#39572,#39576,#7887,.T.);
#50233=EDGE_CURVE('',#39571,#39575,#7888,.T.);
#50234=EDGE_CURVE('',#39577,#39578,#7889,.T.);
#50235=EDGE_CURVE('',#39576,#39578,#7890,.T.);
#50236=EDGE_CURVE('',#39575,#39577,#7891,.T.);
#50237=EDGE_CURVE('',#39578,#39573,#7892,.T.);
#50238=EDGE_CURVE('',#39577,#39574,#7893,.T.);
#50239=EDGE_CURVE('',#39579,#39580,#7894,.T.);
#50240=EDGE_CURVE('',#39581,#39580,#7895,.T.);
#50241=EDGE_CURVE('',#39582,#39581,#7896,.T.);
#50242=EDGE_CURVE('',#39582,#39579,#7897,.T.);
#50243=EDGE_CURVE('',#39583,#39584,#7898,.T.);
#50244=EDGE_CURVE('',#39580,#39584,#7899,.T.);
#50245=EDGE_CURVE('',#39579,#39583,#7900,.T.);
#50246=EDGE_CURVE('',#39585,#39586,#7901,.T.);
#50247=EDGE_CURVE('',#39584,#39586,#7902,.T.);
#50248=EDGE_CURVE('',#39583,#39585,#7903,.T.);
#50249=EDGE_CURVE('',#39586,#39581,#7904,.T.);
#50250=EDGE_CURVE('',#39585,#39582,#7905,.T.);
#50251=EDGE_CURVE('',#39587,#39588,#7906,.T.);
#50252=EDGE_CURVE('',#39589,#39588,#7907,.T.);
#50253=EDGE_CURVE('',#39590,#39589,#7908,.T.);
#50254=EDGE_CURVE('',#39590,#39587,#7909,.T.);
#50255=EDGE_CURVE('',#39591,#39592,#7910,.T.);
#50256=EDGE_CURVE('',#39588,#39592,#7911,.T.);
#50257=EDGE_CURVE('',#39587,#39591,#7912,.T.);
#50258=EDGE_CURVE('',#39593,#39594,#7913,.T.);
#50259=EDGE_CURVE('',#39592,#39594,#7914,.T.);
#50260=EDGE_CURVE('',#39591,#39593,#7915,.T.);
#50261=EDGE_CURVE('',#39594,#39589,#7916,.T.);
#50262=EDGE_CURVE('',#39593,#39590,#7917,.T.);
#50263=EDGE_CURVE('',#39595,#39596,#7918,.T.);
#50264=EDGE_CURVE('',#39597,#39596,#7919,.T.);
#50265=EDGE_CURVE('',#39598,#39597,#7920,.T.);
#50266=EDGE_CURVE('',#39598,#39595,#7921,.T.);
#50267=EDGE_CURVE('',#39599,#39600,#7922,.T.);
#50268=EDGE_CURVE('',#39596,#39600,#7923,.T.);
#50269=EDGE_CURVE('',#39595,#39599,#7924,.T.);
#50270=EDGE_CURVE('',#39601,#39602,#7925,.T.);
#50271=EDGE_CURVE('',#39600,#39602,#7926,.T.);
#50272=EDGE_CURVE('',#39599,#39601,#7927,.T.);
#50273=EDGE_CURVE('',#39602,#39597,#7928,.T.);
#50274=EDGE_CURVE('',#39601,#39598,#7929,.T.);
#50275=EDGE_CURVE('',#39603,#39604,#7930,.T.);
#50276=EDGE_CURVE('',#39605,#39604,#7931,.T.);
#50277=EDGE_CURVE('',#39606,#39605,#7932,.T.);
#50278=EDGE_CURVE('',#39606,#39603,#7933,.T.);
#50279=EDGE_CURVE('',#39607,#39608,#7934,.T.);
#50280=EDGE_CURVE('',#39604,#39608,#7935,.T.);
#50281=EDGE_CURVE('',#39603,#39607,#7936,.T.);
#50282=EDGE_CURVE('',#39609,#39610,#7937,.T.);
#50283=EDGE_CURVE('',#39608,#39610,#7938,.T.);
#50284=EDGE_CURVE('',#39607,#39609,#7939,.T.);
#50285=EDGE_CURVE('',#39610,#39605,#7940,.T.);
#50286=EDGE_CURVE('',#39609,#39606,#7941,.T.);
#50287=EDGE_CURVE('',#39611,#39612,#7942,.T.);
#50288=EDGE_CURVE('',#39613,#39612,#7943,.T.);
#50289=EDGE_CURVE('',#39614,#39613,#7944,.T.);
#50290=EDGE_CURVE('',#39614,#39611,#7945,.T.);
#50291=EDGE_CURVE('',#39615,#39616,#7946,.T.);
#50292=EDGE_CURVE('',#39612,#39616,#7947,.T.);
#50293=EDGE_CURVE('',#39611,#39615,#7948,.T.);
#50294=EDGE_CURVE('',#39617,#39618,#7949,.T.);
#50295=EDGE_CURVE('',#39616,#39618,#7950,.T.);
#50296=EDGE_CURVE('',#39615,#39617,#7951,.T.);
#50297=EDGE_CURVE('',#39618,#39613,#7952,.T.);
#50298=EDGE_CURVE('',#39617,#39614,#7953,.T.);
#50299=EDGE_CURVE('',#39619,#39620,#7954,.T.);
#50300=EDGE_CURVE('',#39621,#39620,#7955,.T.);
#50301=EDGE_CURVE('',#39622,#39621,#7956,.T.);
#50302=EDGE_CURVE('',#39622,#39619,#7957,.T.);
#50303=EDGE_CURVE('',#39623,#39624,#7958,.T.);
#50304=EDGE_CURVE('',#39620,#39624,#7959,.T.);
#50305=EDGE_CURVE('',#39619,#39623,#7960,.T.);
#50306=EDGE_CURVE('',#39625,#39626,#7961,.T.);
#50307=EDGE_CURVE('',#39624,#39626,#7962,.T.);
#50308=EDGE_CURVE('',#39623,#39625,#7963,.T.);
#50309=EDGE_CURVE('',#39626,#39621,#7964,.T.);
#50310=EDGE_CURVE('',#39625,#39622,#7965,.T.);
#50311=EDGE_CURVE('',#39627,#39628,#7966,.T.);
#50312=EDGE_CURVE('',#39629,#39628,#7967,.T.);
#50313=EDGE_CURVE('',#39630,#39629,#7968,.T.);
#50314=EDGE_CURVE('',#39630,#39627,#7969,.T.);
#50315=EDGE_CURVE('',#39631,#39632,#7970,.T.);
#50316=EDGE_CURVE('',#39628,#39632,#7971,.T.);
#50317=EDGE_CURVE('',#39627,#39631,#7972,.T.);
#50318=EDGE_CURVE('',#39633,#39634,#7973,.T.);
#50319=EDGE_CURVE('',#39632,#39634,#7974,.T.);
#50320=EDGE_CURVE('',#39631,#39633,#7975,.T.);
#50321=EDGE_CURVE('',#39634,#39629,#7976,.T.);
#50322=EDGE_CURVE('',#39633,#39630,#7977,.T.);
#50323=EDGE_CURVE('',#39635,#39636,#7978,.T.);
#50324=EDGE_CURVE('',#39637,#39636,#7979,.T.);
#50325=EDGE_CURVE('',#39638,#39637,#7980,.T.);
#50326=EDGE_CURVE('',#39638,#39635,#7981,.T.);
#50327=EDGE_CURVE('',#39639,#39640,#7982,.T.);
#50328=EDGE_CURVE('',#39636,#39640,#7983,.T.);
#50329=EDGE_CURVE('',#39635,#39639,#7984,.T.);
#50330=EDGE_CURVE('',#39641,#39642,#7985,.T.);
#50331=EDGE_CURVE('',#39640,#39642,#7986,.T.);
#50332=EDGE_CURVE('',#39639,#39641,#7987,.T.);
#50333=EDGE_CURVE('',#39642,#39637,#7988,.T.);
#50334=EDGE_CURVE('',#39641,#39638,#7989,.T.);
#50335=EDGE_CURVE('',#39643,#39644,#7990,.T.);
#50336=EDGE_CURVE('',#39645,#39644,#7991,.T.);
#50337=EDGE_CURVE('',#39646,#39645,#7992,.T.);
#50338=EDGE_CURVE('',#39646,#39643,#7993,.T.);
#50339=EDGE_CURVE('',#39647,#39648,#7994,.T.);
#50340=EDGE_CURVE('',#39644,#39648,#7995,.T.);
#50341=EDGE_CURVE('',#39643,#39647,#7996,.T.);
#50342=EDGE_CURVE('',#39649,#39650,#7997,.T.);
#50343=EDGE_CURVE('',#39648,#39650,#7998,.T.);
#50344=EDGE_CURVE('',#39647,#39649,#7999,.T.);
#50345=EDGE_CURVE('',#39650,#39645,#8000,.T.);
#50346=EDGE_CURVE('',#39649,#39646,#8001,.T.);
#50347=EDGE_CURVE('',#39651,#39652,#8002,.T.);
#50348=EDGE_CURVE('',#39653,#39652,#8003,.T.);
#50349=EDGE_CURVE('',#39654,#39653,#8004,.T.);
#50350=EDGE_CURVE('',#39654,#39651,#8005,.T.);
#50351=EDGE_CURVE('',#39655,#39656,#8006,.T.);
#50352=EDGE_CURVE('',#39652,#39656,#8007,.T.);
#50353=EDGE_CURVE('',#39651,#39655,#8008,.T.);
#50354=EDGE_CURVE('',#39657,#39658,#8009,.T.);
#50355=EDGE_CURVE('',#39656,#39658,#8010,.T.);
#50356=EDGE_CURVE('',#39655,#39657,#8011,.T.);
#50357=EDGE_CURVE('',#39658,#39653,#8012,.T.);
#50358=EDGE_CURVE('',#39657,#39654,#8013,.T.);
#50359=EDGE_CURVE('',#39659,#39660,#8014,.T.);
#50360=EDGE_CURVE('',#39661,#39660,#8015,.T.);
#50361=EDGE_CURVE('',#39662,#39661,#8016,.T.);
#50362=EDGE_CURVE('',#39662,#39659,#8017,.T.);
#50363=EDGE_CURVE('',#39663,#39664,#8018,.T.);
#50364=EDGE_CURVE('',#39660,#39664,#8019,.T.);
#50365=EDGE_CURVE('',#39659,#39663,#8020,.T.);
#50366=EDGE_CURVE('',#39665,#39666,#8021,.T.);
#50367=EDGE_CURVE('',#39664,#39666,#8022,.T.);
#50368=EDGE_CURVE('',#39663,#39665,#8023,.T.);
#50369=EDGE_CURVE('',#39666,#39661,#8024,.T.);
#50370=EDGE_CURVE('',#39665,#39662,#8025,.T.);
#50371=EDGE_CURVE('',#39667,#39668,#8026,.T.);
#50372=EDGE_CURVE('',#39669,#39668,#8027,.T.);
#50373=EDGE_CURVE('',#39670,#39669,#8028,.T.);
#50374=EDGE_CURVE('',#39670,#39667,#8029,.T.);
#50375=EDGE_CURVE('',#39671,#39672,#8030,.T.);
#50376=EDGE_CURVE('',#39668,#39672,#8031,.T.);
#50377=EDGE_CURVE('',#39667,#39671,#8032,.T.);
#50378=EDGE_CURVE('',#39673,#39674,#8033,.T.);
#50379=EDGE_CURVE('',#39672,#39674,#8034,.T.);
#50380=EDGE_CURVE('',#39671,#39673,#8035,.T.);
#50381=EDGE_CURVE('',#39674,#39669,#8036,.T.);
#50382=EDGE_CURVE('',#39673,#39670,#8037,.T.);
#50383=EDGE_CURVE('',#39675,#39676,#8038,.T.);
#50384=EDGE_CURVE('',#39677,#39676,#8039,.T.);
#50385=EDGE_CURVE('',#39678,#39677,#8040,.T.);
#50386=EDGE_CURVE('',#39678,#39675,#8041,.T.);
#50387=EDGE_CURVE('',#39679,#39680,#8042,.T.);
#50388=EDGE_CURVE('',#39676,#39680,#8043,.T.);
#50389=EDGE_CURVE('',#39675,#39679,#8044,.T.);
#50390=EDGE_CURVE('',#39681,#39682,#8045,.T.);
#50391=EDGE_CURVE('',#39680,#39682,#8046,.T.);
#50392=EDGE_CURVE('',#39679,#39681,#8047,.T.);
#50393=EDGE_CURVE('',#39682,#39677,#8048,.T.);
#50394=EDGE_CURVE('',#39681,#39678,#8049,.T.);
#50395=EDGE_CURVE('',#39683,#39684,#8050,.T.);
#50396=EDGE_CURVE('',#39685,#39684,#8051,.T.);
#50397=EDGE_CURVE('',#39686,#39685,#8052,.T.);
#50398=EDGE_CURVE('',#39686,#39683,#8053,.T.);
#50399=EDGE_CURVE('',#39687,#39688,#8054,.T.);
#50400=EDGE_CURVE('',#39684,#39688,#8055,.T.);
#50401=EDGE_CURVE('',#39683,#39687,#8056,.T.);
#50402=EDGE_CURVE('',#39689,#39690,#8057,.T.);
#50403=EDGE_CURVE('',#39688,#39690,#8058,.T.);
#50404=EDGE_CURVE('',#39687,#39689,#8059,.T.);
#50405=EDGE_CURVE('',#39690,#39685,#8060,.T.);
#50406=EDGE_CURVE('',#39689,#39686,#8061,.T.);
#50407=EDGE_CURVE('',#39691,#39692,#8062,.T.);
#50408=EDGE_CURVE('',#39693,#39692,#8063,.T.);
#50409=EDGE_CURVE('',#39694,#39693,#8064,.T.);
#50410=EDGE_CURVE('',#39694,#39691,#8065,.T.);
#50411=EDGE_CURVE('',#39695,#39696,#8066,.T.);
#50412=EDGE_CURVE('',#39692,#39696,#8067,.T.);
#50413=EDGE_CURVE('',#39691,#39695,#8068,.T.);
#50414=EDGE_CURVE('',#39697,#39698,#8069,.T.);
#50415=EDGE_CURVE('',#39696,#39698,#8070,.T.);
#50416=EDGE_CURVE('',#39695,#39697,#8071,.T.);
#50417=EDGE_CURVE('',#39698,#39693,#8072,.T.);
#50418=EDGE_CURVE('',#39697,#39694,#8073,.T.);
#50419=EDGE_CURVE('',#39699,#39700,#8074,.T.);
#50420=EDGE_CURVE('',#39701,#39700,#8075,.T.);
#50421=EDGE_CURVE('',#39702,#39701,#8076,.T.);
#50422=EDGE_CURVE('',#39702,#39699,#8077,.T.);
#50423=EDGE_CURVE('',#39703,#39704,#8078,.T.);
#50424=EDGE_CURVE('',#39700,#39704,#8079,.T.);
#50425=EDGE_CURVE('',#39699,#39703,#8080,.T.);
#50426=EDGE_CURVE('',#39705,#39706,#8081,.T.);
#50427=EDGE_CURVE('',#39704,#39706,#8082,.T.);
#50428=EDGE_CURVE('',#39703,#39705,#8083,.T.);
#50429=EDGE_CURVE('',#39706,#39701,#8084,.T.);
#50430=EDGE_CURVE('',#39705,#39702,#8085,.T.);
#50431=EDGE_CURVE('',#39707,#39708,#8086,.T.);
#50432=EDGE_CURVE('',#39709,#39708,#8087,.T.);
#50433=EDGE_CURVE('',#39710,#39709,#8088,.T.);
#50434=EDGE_CURVE('',#39710,#39707,#8089,.T.);
#50435=EDGE_CURVE('',#39711,#39712,#8090,.T.);
#50436=EDGE_CURVE('',#39708,#39712,#8091,.T.);
#50437=EDGE_CURVE('',#39707,#39711,#8092,.T.);
#50438=EDGE_CURVE('',#39713,#39714,#8093,.T.);
#50439=EDGE_CURVE('',#39712,#39714,#8094,.T.);
#50440=EDGE_CURVE('',#39711,#39713,#8095,.T.);
#50441=EDGE_CURVE('',#39714,#39709,#8096,.T.);
#50442=EDGE_CURVE('',#39713,#39710,#8097,.T.);
#50443=EDGE_CURVE('',#39715,#39716,#8098,.T.);
#50444=EDGE_CURVE('',#39717,#39716,#8099,.T.);
#50445=EDGE_CURVE('',#39718,#39717,#8100,.T.);
#50446=EDGE_CURVE('',#39718,#39715,#8101,.T.);
#50447=EDGE_CURVE('',#39719,#39720,#8102,.T.);
#50448=EDGE_CURVE('',#39716,#39720,#8103,.T.);
#50449=EDGE_CURVE('',#39715,#39719,#8104,.T.);
#50450=EDGE_CURVE('',#39721,#39722,#8105,.T.);
#50451=EDGE_CURVE('',#39720,#39722,#8106,.T.);
#50452=EDGE_CURVE('',#39719,#39721,#8107,.T.);
#50453=EDGE_CURVE('',#39722,#39717,#8108,.T.);
#50454=EDGE_CURVE('',#39721,#39718,#8109,.T.);
#50455=EDGE_CURVE('',#39723,#39724,#8110,.T.);
#50456=EDGE_CURVE('',#39725,#39724,#8111,.T.);
#50457=EDGE_CURVE('',#39726,#39725,#8112,.T.);
#50458=EDGE_CURVE('',#39726,#39723,#8113,.T.);
#50459=EDGE_CURVE('',#39727,#39728,#8114,.T.);
#50460=EDGE_CURVE('',#39724,#39728,#8115,.T.);
#50461=EDGE_CURVE('',#39723,#39727,#8116,.T.);
#50462=EDGE_CURVE('',#39729,#39730,#8117,.T.);
#50463=EDGE_CURVE('',#39728,#39730,#8118,.T.);
#50464=EDGE_CURVE('',#39727,#39729,#8119,.T.);
#50465=EDGE_CURVE('',#39730,#39725,#8120,.T.);
#50466=EDGE_CURVE('',#39729,#39726,#8121,.T.);
#50467=EDGE_CURVE('',#39731,#39732,#8122,.T.);
#50468=EDGE_CURVE('',#39733,#39732,#8123,.T.);
#50469=EDGE_CURVE('',#39734,#39733,#8124,.T.);
#50470=EDGE_CURVE('',#39734,#39731,#8125,.T.);
#50471=EDGE_CURVE('',#39735,#39736,#8126,.T.);
#50472=EDGE_CURVE('',#39732,#39736,#8127,.T.);
#50473=EDGE_CURVE('',#39731,#39735,#8128,.T.);
#50474=EDGE_CURVE('',#39737,#39738,#8129,.T.);
#50475=EDGE_CURVE('',#39736,#39738,#8130,.T.);
#50476=EDGE_CURVE('',#39735,#39737,#8131,.T.);
#50477=EDGE_CURVE('',#39738,#39733,#8132,.T.);
#50478=EDGE_CURVE('',#39737,#39734,#8133,.T.);
#50479=EDGE_CURVE('',#39739,#39740,#8134,.T.);
#50480=EDGE_CURVE('',#39741,#39740,#8135,.T.);
#50481=EDGE_CURVE('',#39742,#39741,#8136,.T.);
#50482=EDGE_CURVE('',#39742,#39739,#8137,.T.);
#50483=EDGE_CURVE('',#39743,#39744,#8138,.T.);
#50484=EDGE_CURVE('',#39740,#39744,#8139,.T.);
#50485=EDGE_CURVE('',#39739,#39743,#8140,.T.);
#50486=EDGE_CURVE('',#39745,#39746,#8141,.T.);
#50487=EDGE_CURVE('',#39744,#39746,#8142,.T.);
#50488=EDGE_CURVE('',#39743,#39745,#8143,.T.);
#50489=EDGE_CURVE('',#39746,#39741,#8144,.T.);
#50490=EDGE_CURVE('',#39745,#39742,#8145,.T.);
#50491=EDGE_CURVE('',#39747,#39748,#8146,.T.);
#50492=EDGE_CURVE('',#39749,#39748,#8147,.T.);
#50493=EDGE_CURVE('',#39750,#39749,#8148,.T.);
#50494=EDGE_CURVE('',#39750,#39747,#8149,.T.);
#50495=EDGE_CURVE('',#39751,#39752,#8150,.T.);
#50496=EDGE_CURVE('',#39748,#39752,#8151,.T.);
#50497=EDGE_CURVE('',#39747,#39751,#8152,.T.);
#50498=EDGE_CURVE('',#39753,#39754,#8153,.T.);
#50499=EDGE_CURVE('',#39752,#39754,#8154,.T.);
#50500=EDGE_CURVE('',#39751,#39753,#8155,.T.);
#50501=EDGE_CURVE('',#39754,#39749,#8156,.T.);
#50502=EDGE_CURVE('',#39753,#39750,#8157,.T.);
#50503=EDGE_CURVE('',#39755,#39756,#8158,.T.);
#50504=EDGE_CURVE('',#39757,#39756,#8159,.T.);
#50505=EDGE_CURVE('',#39758,#39757,#8160,.T.);
#50506=EDGE_CURVE('',#39758,#39755,#8161,.T.);
#50507=EDGE_CURVE('',#39759,#39760,#8162,.T.);
#50508=EDGE_CURVE('',#39756,#39760,#8163,.T.);
#50509=EDGE_CURVE('',#39755,#39759,#8164,.T.);
#50510=EDGE_CURVE('',#39761,#39762,#8165,.T.);
#50511=EDGE_CURVE('',#39760,#39762,#8166,.T.);
#50512=EDGE_CURVE('',#39759,#39761,#8167,.T.);
#50513=EDGE_CURVE('',#39762,#39757,#8168,.T.);
#50514=EDGE_CURVE('',#39761,#39758,#8169,.T.);
#50515=EDGE_CURVE('',#39763,#39764,#8170,.T.);
#50516=EDGE_CURVE('',#39765,#39764,#8171,.T.);
#50517=EDGE_CURVE('',#39766,#39765,#8172,.T.);
#50518=EDGE_CURVE('',#39766,#39763,#8173,.T.);
#50519=EDGE_CURVE('',#39767,#39768,#8174,.T.);
#50520=EDGE_CURVE('',#39764,#39768,#8175,.T.);
#50521=EDGE_CURVE('',#39763,#39767,#8176,.T.);
#50522=EDGE_CURVE('',#39769,#39770,#8177,.T.);
#50523=EDGE_CURVE('',#39768,#39770,#8178,.T.);
#50524=EDGE_CURVE('',#39767,#39769,#8179,.T.);
#50525=EDGE_CURVE('',#39770,#39765,#8180,.T.);
#50526=EDGE_CURVE('',#39769,#39766,#8181,.T.);
#50527=EDGE_CURVE('',#39771,#39772,#8182,.T.);
#50528=EDGE_CURVE('',#39773,#39772,#8183,.T.);
#50529=EDGE_CURVE('',#39774,#39773,#8184,.T.);
#50530=EDGE_CURVE('',#39774,#39771,#8185,.T.);
#50531=EDGE_CURVE('',#39775,#39776,#8186,.T.);
#50532=EDGE_CURVE('',#39772,#39776,#8187,.T.);
#50533=EDGE_CURVE('',#39771,#39775,#8188,.T.);
#50534=EDGE_CURVE('',#39777,#39778,#8189,.T.);
#50535=EDGE_CURVE('',#39776,#39778,#8190,.T.);
#50536=EDGE_CURVE('',#39775,#39777,#8191,.T.);
#50537=EDGE_CURVE('',#39778,#39773,#8192,.T.);
#50538=EDGE_CURVE('',#39777,#39774,#8193,.T.);
#50539=EDGE_CURVE('',#39779,#39780,#8194,.T.);
#50540=EDGE_CURVE('',#39781,#39780,#8195,.T.);
#50541=EDGE_CURVE('',#39782,#39781,#8196,.T.);
#50542=EDGE_CURVE('',#39782,#39779,#8197,.T.);
#50543=EDGE_CURVE('',#39783,#39784,#8198,.T.);
#50544=EDGE_CURVE('',#39780,#39784,#8199,.T.);
#50545=EDGE_CURVE('',#39779,#39783,#8200,.T.);
#50546=EDGE_CURVE('',#39785,#39786,#8201,.T.);
#50547=EDGE_CURVE('',#39784,#39786,#8202,.T.);
#50548=EDGE_CURVE('',#39783,#39785,#8203,.T.);
#50549=EDGE_CURVE('',#39786,#39781,#8204,.T.);
#50550=EDGE_CURVE('',#39785,#39782,#8205,.T.);
#50551=EDGE_CURVE('',#39787,#39788,#8206,.T.);
#50552=EDGE_CURVE('',#39789,#39788,#8207,.T.);
#50553=EDGE_CURVE('',#39790,#39789,#8208,.T.);
#50554=EDGE_CURVE('',#39790,#39787,#8209,.T.);
#50555=EDGE_CURVE('',#39791,#39792,#8210,.T.);
#50556=EDGE_CURVE('',#39788,#39792,#8211,.T.);
#50557=EDGE_CURVE('',#39787,#39791,#8212,.T.);
#50558=EDGE_CURVE('',#39793,#39794,#8213,.T.);
#50559=EDGE_CURVE('',#39792,#39794,#8214,.T.);
#50560=EDGE_CURVE('',#39791,#39793,#8215,.T.);
#50561=EDGE_CURVE('',#39794,#39789,#8216,.T.);
#50562=EDGE_CURVE('',#39793,#39790,#8217,.T.);
#50563=EDGE_CURVE('',#39795,#39796,#8218,.T.);
#50564=EDGE_CURVE('',#39797,#39796,#8219,.T.);
#50565=EDGE_CURVE('',#39798,#39797,#8220,.T.);
#50566=EDGE_CURVE('',#39798,#39795,#8221,.T.);
#50567=EDGE_CURVE('',#39799,#39800,#8222,.T.);
#50568=EDGE_CURVE('',#39796,#39800,#8223,.T.);
#50569=EDGE_CURVE('',#39795,#39799,#8224,.T.);
#50570=EDGE_CURVE('',#39801,#39802,#8225,.T.);
#50571=EDGE_CURVE('',#39800,#39802,#8226,.T.);
#50572=EDGE_CURVE('',#39799,#39801,#8227,.T.);
#50573=EDGE_CURVE('',#39802,#39797,#8228,.T.);
#50574=EDGE_CURVE('',#39801,#39798,#8229,.T.);
#50575=EDGE_CURVE('',#39803,#39804,#8230,.T.);
#50576=EDGE_CURVE('',#39805,#39804,#8231,.T.);
#50577=EDGE_CURVE('',#39806,#39805,#8232,.T.);
#50578=EDGE_CURVE('',#39806,#39803,#8233,.T.);
#50579=EDGE_CURVE('',#39807,#39808,#8234,.T.);
#50580=EDGE_CURVE('',#39804,#39808,#8235,.T.);
#50581=EDGE_CURVE('',#39803,#39807,#8236,.T.);
#50582=EDGE_CURVE('',#39809,#39810,#8237,.T.);
#50583=EDGE_CURVE('',#39808,#39810,#8238,.T.);
#50584=EDGE_CURVE('',#39807,#39809,#8239,.T.);
#50585=EDGE_CURVE('',#39810,#39805,#8240,.T.);
#50586=EDGE_CURVE('',#39809,#39806,#8241,.T.);
#50587=EDGE_CURVE('',#39811,#39812,#8242,.T.);
#50588=EDGE_CURVE('',#39813,#39812,#8243,.T.);
#50589=EDGE_CURVE('',#39814,#39813,#8244,.T.);
#50590=EDGE_CURVE('',#39814,#39811,#8245,.T.);
#50591=EDGE_CURVE('',#39815,#39816,#8246,.T.);
#50592=EDGE_CURVE('',#39812,#39816,#8247,.T.);
#50593=EDGE_CURVE('',#39811,#39815,#8248,.T.);
#50594=EDGE_CURVE('',#39817,#39818,#8249,.T.);
#50595=EDGE_CURVE('',#39816,#39818,#8250,.T.);
#50596=EDGE_CURVE('',#39815,#39817,#8251,.T.);
#50597=EDGE_CURVE('',#39818,#39813,#8252,.T.);
#50598=EDGE_CURVE('',#39817,#39814,#8253,.T.);
#50599=EDGE_CURVE('',#39819,#39820,#8254,.T.);
#50600=EDGE_CURVE('',#39821,#39820,#8255,.T.);
#50601=EDGE_CURVE('',#39822,#39821,#8256,.T.);
#50602=EDGE_CURVE('',#39822,#39819,#8257,.T.);
#50603=EDGE_CURVE('',#39823,#39824,#8258,.T.);
#50604=EDGE_CURVE('',#39820,#39824,#8259,.T.);
#50605=EDGE_CURVE('',#39819,#39823,#8260,.T.);
#50606=EDGE_CURVE('',#39825,#39826,#8261,.T.);
#50607=EDGE_CURVE('',#39824,#39826,#8262,.T.);
#50608=EDGE_CURVE('',#39823,#39825,#8263,.T.);
#50609=EDGE_CURVE('',#39826,#39821,#8264,.T.);
#50610=EDGE_CURVE('',#39825,#39822,#8265,.T.);
#50611=EDGE_CURVE('',#39827,#39828,#8266,.T.);
#50612=EDGE_CURVE('',#39829,#39828,#8267,.T.);
#50613=EDGE_CURVE('',#39830,#39829,#8268,.T.);
#50614=EDGE_CURVE('',#39830,#39827,#8269,.T.);
#50615=EDGE_CURVE('',#39831,#39832,#8270,.T.);
#50616=EDGE_CURVE('',#39828,#39832,#8271,.T.);
#50617=EDGE_CURVE('',#39827,#39831,#8272,.T.);
#50618=EDGE_CURVE('',#39833,#39834,#8273,.T.);
#50619=EDGE_CURVE('',#39832,#39834,#8274,.T.);
#50620=EDGE_CURVE('',#39831,#39833,#8275,.T.);
#50621=EDGE_CURVE('',#39834,#39829,#8276,.T.);
#50622=EDGE_CURVE('',#39833,#39830,#8277,.T.);
#50623=EDGE_CURVE('',#39835,#39836,#8278,.T.);
#50624=EDGE_CURVE('',#39837,#39836,#8279,.T.);
#50625=EDGE_CURVE('',#39838,#39837,#8280,.T.);
#50626=EDGE_CURVE('',#39838,#39835,#8281,.T.);
#50627=EDGE_CURVE('',#39839,#39840,#8282,.T.);
#50628=EDGE_CURVE('',#39836,#39840,#8283,.T.);
#50629=EDGE_CURVE('',#39835,#39839,#8284,.T.);
#50630=EDGE_CURVE('',#39841,#39842,#8285,.T.);
#50631=EDGE_CURVE('',#39840,#39842,#8286,.T.);
#50632=EDGE_CURVE('',#39839,#39841,#8287,.T.);
#50633=EDGE_CURVE('',#39842,#39837,#8288,.T.);
#50634=EDGE_CURVE('',#39841,#39838,#8289,.T.);
#50635=EDGE_CURVE('',#39843,#39844,#8290,.T.);
#50636=EDGE_CURVE('',#39845,#39844,#8291,.T.);
#50637=EDGE_CURVE('',#39846,#39845,#8292,.T.);
#50638=EDGE_CURVE('',#39846,#39843,#8293,.T.);
#50639=EDGE_CURVE('',#39847,#39848,#8294,.T.);
#50640=EDGE_CURVE('',#39844,#39848,#8295,.T.);
#50641=EDGE_CURVE('',#39843,#39847,#8296,.T.);
#50642=EDGE_CURVE('',#39849,#39850,#8297,.T.);
#50643=EDGE_CURVE('',#39848,#39850,#8298,.T.);
#50644=EDGE_CURVE('',#39847,#39849,#8299,.T.);
#50645=EDGE_CURVE('',#39850,#39845,#8300,.T.);
#50646=EDGE_CURVE('',#39849,#39846,#8301,.T.);
#50647=EDGE_CURVE('',#39851,#39852,#8302,.T.);
#50648=EDGE_CURVE('',#39853,#39852,#8303,.T.);
#50649=EDGE_CURVE('',#39854,#39853,#8304,.T.);
#50650=EDGE_CURVE('',#39854,#39851,#8305,.T.);
#50651=EDGE_CURVE('',#39855,#39856,#8306,.T.);
#50652=EDGE_CURVE('',#39852,#39856,#8307,.T.);
#50653=EDGE_CURVE('',#39851,#39855,#8308,.T.);
#50654=EDGE_CURVE('',#39857,#39858,#8309,.T.);
#50655=EDGE_CURVE('',#39856,#39858,#8310,.T.);
#50656=EDGE_CURVE('',#39855,#39857,#8311,.T.);
#50657=EDGE_CURVE('',#39858,#39853,#8312,.T.);
#50658=EDGE_CURVE('',#39857,#39854,#8313,.T.);
#50659=EDGE_CURVE('',#39859,#39860,#8314,.T.);
#50660=EDGE_CURVE('',#39861,#39860,#8315,.T.);
#50661=EDGE_CURVE('',#39862,#39861,#8316,.T.);
#50662=EDGE_CURVE('',#39862,#39859,#8317,.T.);
#50663=EDGE_CURVE('',#39863,#39864,#8318,.T.);
#50664=EDGE_CURVE('',#39860,#39864,#8319,.T.);
#50665=EDGE_CURVE('',#39859,#39863,#8320,.T.);
#50666=EDGE_CURVE('',#39865,#39866,#8321,.T.);
#50667=EDGE_CURVE('',#39864,#39866,#8322,.T.);
#50668=EDGE_CURVE('',#39863,#39865,#8323,.T.);
#50669=EDGE_CURVE('',#39866,#39861,#8324,.T.);
#50670=EDGE_CURVE('',#39865,#39862,#8325,.T.);
#50671=EDGE_CURVE('',#39867,#39868,#8326,.T.);
#50672=EDGE_CURVE('',#39869,#39868,#8327,.T.);
#50673=EDGE_CURVE('',#39870,#39869,#8328,.T.);
#50674=EDGE_CURVE('',#39870,#39867,#8329,.T.);
#50675=EDGE_CURVE('',#39871,#39872,#8330,.T.);
#50676=EDGE_CURVE('',#39868,#39872,#8331,.T.);
#50677=EDGE_CURVE('',#39867,#39871,#8332,.T.);
#50678=EDGE_CURVE('',#39873,#39874,#8333,.T.);
#50679=EDGE_CURVE('',#39872,#39874,#8334,.T.);
#50680=EDGE_CURVE('',#39871,#39873,#8335,.T.);
#50681=EDGE_CURVE('',#39874,#39869,#8336,.T.);
#50682=EDGE_CURVE('',#39873,#39870,#8337,.T.);
#50683=EDGE_CURVE('',#39875,#39876,#8338,.T.);
#50684=EDGE_CURVE('',#39877,#39876,#8339,.T.);
#50685=EDGE_CURVE('',#39878,#39877,#8340,.T.);
#50686=EDGE_CURVE('',#39878,#39875,#8341,.T.);
#50687=EDGE_CURVE('',#39879,#39880,#8342,.T.);
#50688=EDGE_CURVE('',#39876,#39880,#8343,.T.);
#50689=EDGE_CURVE('',#39875,#39879,#8344,.T.);
#50690=EDGE_CURVE('',#39881,#39882,#8345,.T.);
#50691=EDGE_CURVE('',#39880,#39882,#8346,.T.);
#50692=EDGE_CURVE('',#39879,#39881,#8347,.T.);
#50693=EDGE_CURVE('',#39882,#39877,#8348,.T.);
#50694=EDGE_CURVE('',#39881,#39878,#8349,.T.);
#50695=EDGE_CURVE('',#39883,#39884,#8350,.T.);
#50696=EDGE_CURVE('',#39885,#39884,#8351,.T.);
#50697=EDGE_CURVE('',#39886,#39885,#8352,.T.);
#50698=EDGE_CURVE('',#39886,#39883,#8353,.T.);
#50699=EDGE_CURVE('',#39887,#39888,#8354,.T.);
#50700=EDGE_CURVE('',#39884,#39888,#8355,.T.);
#50701=EDGE_CURVE('',#39883,#39887,#8356,.T.);
#50702=EDGE_CURVE('',#39889,#39890,#8357,.T.);
#50703=EDGE_CURVE('',#39888,#39890,#8358,.T.);
#50704=EDGE_CURVE('',#39887,#39889,#8359,.T.);
#50705=EDGE_CURVE('',#39890,#39885,#8360,.T.);
#50706=EDGE_CURVE('',#39889,#39886,#8361,.T.);
#50707=EDGE_CURVE('',#39891,#39892,#8362,.T.);
#50708=EDGE_CURVE('',#39893,#39892,#8363,.T.);
#50709=EDGE_CURVE('',#39894,#39893,#8364,.T.);
#50710=EDGE_CURVE('',#39894,#39891,#8365,.T.);
#50711=EDGE_CURVE('',#39895,#39896,#8366,.T.);
#50712=EDGE_CURVE('',#39892,#39896,#8367,.T.);
#50713=EDGE_CURVE('',#39891,#39895,#8368,.T.);
#50714=EDGE_CURVE('',#39897,#39898,#8369,.T.);
#50715=EDGE_CURVE('',#39896,#39898,#8370,.T.);
#50716=EDGE_CURVE('',#39895,#39897,#8371,.T.);
#50717=EDGE_CURVE('',#39898,#39893,#8372,.T.);
#50718=EDGE_CURVE('',#39897,#39894,#8373,.T.);
#50719=EDGE_CURVE('',#39899,#39900,#8374,.T.);
#50720=EDGE_CURVE('',#39901,#39900,#8375,.T.);
#50721=EDGE_CURVE('',#39902,#39901,#8376,.T.);
#50722=EDGE_CURVE('',#39902,#39899,#8377,.T.);
#50723=EDGE_CURVE('',#39903,#39904,#8378,.T.);
#50724=EDGE_CURVE('',#39900,#39904,#8379,.T.);
#50725=EDGE_CURVE('',#39899,#39903,#8380,.T.);
#50726=EDGE_CURVE('',#39905,#39906,#8381,.T.);
#50727=EDGE_CURVE('',#39904,#39906,#8382,.T.);
#50728=EDGE_CURVE('',#39903,#39905,#8383,.T.);
#50729=EDGE_CURVE('',#39906,#39901,#8384,.T.);
#50730=EDGE_CURVE('',#39905,#39902,#8385,.T.);
#50731=EDGE_CURVE('',#39907,#39908,#8386,.T.);
#50732=EDGE_CURVE('',#39909,#39908,#8387,.T.);
#50733=EDGE_CURVE('',#39910,#39909,#8388,.T.);
#50734=EDGE_CURVE('',#39910,#39907,#8389,.T.);
#50735=EDGE_CURVE('',#39911,#39912,#8390,.T.);
#50736=EDGE_CURVE('',#39908,#39912,#8391,.T.);
#50737=EDGE_CURVE('',#39907,#39911,#8392,.T.);
#50738=EDGE_CURVE('',#39913,#39914,#8393,.T.);
#50739=EDGE_CURVE('',#39912,#39914,#8394,.T.);
#50740=EDGE_CURVE('',#39911,#39913,#8395,.T.);
#50741=EDGE_CURVE('',#39914,#39909,#8396,.T.);
#50742=EDGE_CURVE('',#39913,#39910,#8397,.T.);
#50743=EDGE_CURVE('',#39915,#39916,#8398,.T.);
#50744=EDGE_CURVE('',#39917,#39916,#8399,.T.);
#50745=EDGE_CURVE('',#39918,#39917,#8400,.T.);
#50746=EDGE_CURVE('',#39918,#39915,#8401,.T.);
#50747=EDGE_CURVE('',#39919,#39920,#8402,.T.);
#50748=EDGE_CURVE('',#39916,#39920,#8403,.T.);
#50749=EDGE_CURVE('',#39915,#39919,#8404,.T.);
#50750=EDGE_CURVE('',#39921,#39922,#8405,.T.);
#50751=EDGE_CURVE('',#39920,#39922,#8406,.T.);
#50752=EDGE_CURVE('',#39919,#39921,#8407,.T.);
#50753=EDGE_CURVE('',#39922,#39917,#8408,.T.);
#50754=EDGE_CURVE('',#39921,#39918,#8409,.T.);
#50755=EDGE_CURVE('',#39923,#39924,#8410,.T.);
#50756=EDGE_CURVE('',#39925,#39924,#8411,.T.);
#50757=EDGE_CURVE('',#39926,#39925,#8412,.T.);
#50758=EDGE_CURVE('',#39926,#39923,#8413,.T.);
#50759=EDGE_CURVE('',#39927,#39928,#8414,.T.);
#50760=EDGE_CURVE('',#39924,#39928,#8415,.T.);
#50761=EDGE_CURVE('',#39923,#39927,#8416,.T.);
#50762=EDGE_CURVE('',#39929,#39930,#8417,.T.);
#50763=EDGE_CURVE('',#39928,#39930,#8418,.T.);
#50764=EDGE_CURVE('',#39927,#39929,#8419,.T.);
#50765=EDGE_CURVE('',#39930,#39925,#8420,.T.);
#50766=EDGE_CURVE('',#39929,#39926,#8421,.T.);
#50767=EDGE_CURVE('',#39931,#39932,#8422,.T.);
#50768=EDGE_CURVE('',#39933,#39932,#8423,.T.);
#50769=EDGE_CURVE('',#39934,#39933,#8424,.T.);
#50770=EDGE_CURVE('',#39934,#39931,#8425,.T.);
#50771=EDGE_CURVE('',#39935,#39936,#8426,.T.);
#50772=EDGE_CURVE('',#39932,#39936,#8427,.T.);
#50773=EDGE_CURVE('',#39931,#39935,#8428,.T.);
#50774=EDGE_CURVE('',#39937,#39938,#8429,.T.);
#50775=EDGE_CURVE('',#39936,#39938,#8430,.T.);
#50776=EDGE_CURVE('',#39935,#39937,#8431,.T.);
#50777=EDGE_CURVE('',#39938,#39933,#8432,.T.);
#50778=EDGE_CURVE('',#39937,#39934,#8433,.T.);
#50779=EDGE_CURVE('',#39939,#39940,#8434,.T.);
#50780=EDGE_CURVE('',#39941,#39940,#8435,.T.);
#50781=EDGE_CURVE('',#39942,#39941,#8436,.T.);
#50782=EDGE_CURVE('',#39942,#39939,#8437,.T.);
#50783=EDGE_CURVE('',#39943,#39944,#8438,.T.);
#50784=EDGE_CURVE('',#39940,#39944,#8439,.T.);
#50785=EDGE_CURVE('',#39939,#39943,#8440,.T.);
#50786=EDGE_CURVE('',#39945,#39946,#8441,.T.);
#50787=EDGE_CURVE('',#39944,#39946,#8442,.T.);
#50788=EDGE_CURVE('',#39943,#39945,#8443,.T.);
#50789=EDGE_CURVE('',#39946,#39941,#8444,.T.);
#50790=EDGE_CURVE('',#39945,#39942,#8445,.T.);
#50791=EDGE_CURVE('',#39947,#39948,#8446,.T.);
#50792=EDGE_CURVE('',#39949,#39948,#8447,.T.);
#50793=EDGE_CURVE('',#39950,#39949,#8448,.T.);
#50794=EDGE_CURVE('',#39950,#39947,#8449,.T.);
#50795=EDGE_CURVE('',#39951,#39952,#8450,.T.);
#50796=EDGE_CURVE('',#39948,#39952,#8451,.T.);
#50797=EDGE_CURVE('',#39947,#39951,#8452,.T.);
#50798=EDGE_CURVE('',#39953,#39954,#8453,.T.);
#50799=EDGE_CURVE('',#39952,#39954,#8454,.T.);
#50800=EDGE_CURVE('',#39951,#39953,#8455,.T.);
#50801=EDGE_CURVE('',#39954,#39949,#8456,.T.);
#50802=EDGE_CURVE('',#39953,#39950,#8457,.T.);
#50803=EDGE_CURVE('',#39955,#39956,#8458,.T.);
#50804=EDGE_CURVE('',#39957,#39956,#8459,.T.);
#50805=EDGE_CURVE('',#39958,#39957,#8460,.T.);
#50806=EDGE_CURVE('',#39958,#39955,#8461,.T.);
#50807=EDGE_CURVE('',#39959,#39960,#8462,.T.);
#50808=EDGE_CURVE('',#39956,#39960,#8463,.T.);
#50809=EDGE_CURVE('',#39955,#39959,#8464,.T.);
#50810=EDGE_CURVE('',#39961,#39962,#8465,.T.);
#50811=EDGE_CURVE('',#39960,#39962,#8466,.T.);
#50812=EDGE_CURVE('',#39959,#39961,#8467,.T.);
#50813=EDGE_CURVE('',#39962,#39957,#8468,.T.);
#50814=EDGE_CURVE('',#39961,#39958,#8469,.T.);
#50815=EDGE_CURVE('',#39963,#39964,#8470,.T.);
#50816=EDGE_CURVE('',#39965,#39964,#8471,.T.);
#50817=EDGE_CURVE('',#39966,#39965,#8472,.T.);
#50818=EDGE_CURVE('',#39966,#39963,#8473,.T.);
#50819=EDGE_CURVE('',#39967,#39968,#8474,.T.);
#50820=EDGE_CURVE('',#39964,#39968,#8475,.T.);
#50821=EDGE_CURVE('',#39963,#39967,#8476,.T.);
#50822=EDGE_CURVE('',#39969,#39970,#8477,.T.);
#50823=EDGE_CURVE('',#39968,#39970,#8478,.T.);
#50824=EDGE_CURVE('',#39967,#39969,#8479,.T.);
#50825=EDGE_CURVE('',#39970,#39965,#8480,.T.);
#50826=EDGE_CURVE('',#39969,#39966,#8481,.T.);
#50827=EDGE_CURVE('',#39971,#39972,#8482,.T.);
#50828=EDGE_CURVE('',#39973,#39972,#8483,.T.);
#50829=EDGE_CURVE('',#39974,#39973,#8484,.T.);
#50830=EDGE_CURVE('',#39974,#39971,#8485,.T.);
#50831=EDGE_CURVE('',#39975,#39976,#8486,.T.);
#50832=EDGE_CURVE('',#39972,#39976,#8487,.T.);
#50833=EDGE_CURVE('',#39971,#39975,#8488,.T.);
#50834=EDGE_CURVE('',#39977,#39978,#8489,.T.);
#50835=EDGE_CURVE('',#39976,#39978,#8490,.T.);
#50836=EDGE_CURVE('',#39975,#39977,#8491,.T.);
#50837=EDGE_CURVE('',#39978,#39973,#8492,.T.);
#50838=EDGE_CURVE('',#39977,#39974,#8493,.T.);
#50839=EDGE_CURVE('',#39979,#39980,#8494,.T.);
#50840=EDGE_CURVE('',#39981,#39980,#8495,.T.);
#50841=EDGE_CURVE('',#39982,#39981,#8496,.T.);
#50842=EDGE_CURVE('',#39982,#39979,#8497,.T.);
#50843=EDGE_CURVE('',#39983,#39984,#8498,.T.);
#50844=EDGE_CURVE('',#39980,#39984,#8499,.T.);
#50845=EDGE_CURVE('',#39979,#39983,#8500,.T.);
#50846=EDGE_CURVE('',#39985,#39986,#8501,.T.);
#50847=EDGE_CURVE('',#39984,#39986,#8502,.T.);
#50848=EDGE_CURVE('',#39983,#39985,#8503,.T.);
#50849=EDGE_CURVE('',#39986,#39981,#8504,.T.);
#50850=EDGE_CURVE('',#39985,#39982,#8505,.T.);
#50851=EDGE_CURVE('',#39987,#39988,#8506,.T.);
#50852=EDGE_CURVE('',#39989,#39988,#8507,.T.);
#50853=EDGE_CURVE('',#39990,#39989,#8508,.T.);
#50854=EDGE_CURVE('',#39990,#39987,#8509,.T.);
#50855=EDGE_CURVE('',#39991,#39992,#8510,.T.);
#50856=EDGE_CURVE('',#39988,#39992,#8511,.T.);
#50857=EDGE_CURVE('',#39987,#39991,#8512,.T.);
#50858=EDGE_CURVE('',#39993,#39994,#8513,.T.);
#50859=EDGE_CURVE('',#39992,#39994,#8514,.T.);
#50860=EDGE_CURVE('',#39991,#39993,#8515,.T.);
#50861=EDGE_CURVE('',#39994,#39989,#8516,.T.);
#50862=EDGE_CURVE('',#39993,#39990,#8517,.T.);
#50863=EDGE_CURVE('',#39995,#39996,#8518,.T.);
#50864=EDGE_CURVE('',#39997,#39996,#8519,.T.);
#50865=EDGE_CURVE('',#39998,#39997,#8520,.T.);
#50866=EDGE_CURVE('',#39998,#39995,#8521,.T.);
#50867=EDGE_CURVE('',#39999,#40000,#8522,.T.);
#50868=EDGE_CURVE('',#39996,#40000,#8523,.T.);
#50869=EDGE_CURVE('',#39995,#39999,#8524,.T.);
#50870=EDGE_CURVE('',#40001,#40002,#8525,.T.);
#50871=EDGE_CURVE('',#40000,#40002,#8526,.T.);
#50872=EDGE_CURVE('',#39999,#40001,#8527,.T.);
#50873=EDGE_CURVE('',#40002,#39997,#8528,.T.);
#50874=EDGE_CURVE('',#40001,#39998,#8529,.T.);
#50875=EDGE_CURVE('',#40003,#40004,#8530,.T.);
#50876=EDGE_CURVE('',#40005,#40004,#8531,.T.);
#50877=EDGE_CURVE('',#40006,#40005,#8532,.T.);
#50878=EDGE_CURVE('',#40006,#40003,#8533,.T.);
#50879=EDGE_CURVE('',#40007,#40008,#8534,.T.);
#50880=EDGE_CURVE('',#40004,#40008,#8535,.T.);
#50881=EDGE_CURVE('',#40003,#40007,#8536,.T.);
#50882=EDGE_CURVE('',#40009,#40010,#8537,.T.);
#50883=EDGE_CURVE('',#40008,#40010,#8538,.T.);
#50884=EDGE_CURVE('',#40007,#40009,#8539,.T.);
#50885=EDGE_CURVE('',#40010,#40005,#8540,.T.);
#50886=EDGE_CURVE('',#40009,#40006,#8541,.T.);
#50887=EDGE_CURVE('',#40011,#40012,#8542,.T.);
#50888=EDGE_CURVE('',#40013,#40012,#8543,.T.);
#50889=EDGE_CURVE('',#40014,#40013,#8544,.T.);
#50890=EDGE_CURVE('',#40014,#40011,#8545,.T.);
#50891=EDGE_CURVE('',#40015,#40016,#8546,.T.);
#50892=EDGE_CURVE('',#40012,#40016,#8547,.T.);
#50893=EDGE_CURVE('',#40011,#40015,#8548,.T.);
#50894=EDGE_CURVE('',#40017,#40018,#8549,.T.);
#50895=EDGE_CURVE('',#40016,#40018,#8550,.T.);
#50896=EDGE_CURVE('',#40015,#40017,#8551,.T.);
#50897=EDGE_CURVE('',#40018,#40013,#8552,.T.);
#50898=EDGE_CURVE('',#40017,#40014,#8553,.T.);
#50899=EDGE_CURVE('',#40019,#40020,#8554,.T.);
#50900=EDGE_CURVE('',#40021,#40020,#8555,.T.);
#50901=EDGE_CURVE('',#40022,#40021,#8556,.T.);
#50902=EDGE_CURVE('',#40022,#40019,#8557,.T.);
#50903=EDGE_CURVE('',#40023,#40024,#8558,.T.);
#50904=EDGE_CURVE('',#40020,#40024,#8559,.T.);
#50905=EDGE_CURVE('',#40019,#40023,#8560,.T.);
#50906=EDGE_CURVE('',#40025,#40026,#8561,.T.);
#50907=EDGE_CURVE('',#40024,#40026,#8562,.T.);
#50908=EDGE_CURVE('',#40023,#40025,#8563,.T.);
#50909=EDGE_CURVE('',#40026,#40021,#8564,.T.);
#50910=EDGE_CURVE('',#40025,#40022,#8565,.T.);
#50911=EDGE_CURVE('',#40027,#40028,#8566,.T.);
#50912=EDGE_CURVE('',#40029,#40028,#8567,.T.);
#50913=EDGE_CURVE('',#40030,#40029,#8568,.T.);
#50914=EDGE_CURVE('',#40030,#40027,#8569,.T.);
#50915=EDGE_CURVE('',#40031,#40032,#8570,.T.);
#50916=EDGE_CURVE('',#40028,#40032,#8571,.T.);
#50917=EDGE_CURVE('',#40027,#40031,#8572,.T.);
#50918=EDGE_CURVE('',#40033,#40034,#8573,.T.);
#50919=EDGE_CURVE('',#40032,#40034,#8574,.T.);
#50920=EDGE_CURVE('',#40031,#40033,#8575,.T.);
#50921=EDGE_CURVE('',#40034,#40029,#8576,.T.);
#50922=EDGE_CURVE('',#40033,#40030,#8577,.T.);
#50923=EDGE_CURVE('',#40035,#40036,#8578,.T.);
#50924=EDGE_CURVE('',#40037,#40036,#8579,.T.);
#50925=EDGE_CURVE('',#40038,#40037,#8580,.T.);
#50926=EDGE_CURVE('',#40038,#40035,#8581,.T.);
#50927=EDGE_CURVE('',#40039,#40040,#8582,.T.);
#50928=EDGE_CURVE('',#40036,#40040,#8583,.T.);
#50929=EDGE_CURVE('',#40035,#40039,#8584,.T.);
#50930=EDGE_CURVE('',#40041,#40042,#8585,.T.);
#50931=EDGE_CURVE('',#40040,#40042,#8586,.T.);
#50932=EDGE_CURVE('',#40039,#40041,#8587,.T.);
#50933=EDGE_CURVE('',#40042,#40037,#8588,.T.);
#50934=EDGE_CURVE('',#40041,#40038,#8589,.T.);
#50935=EDGE_CURVE('',#40043,#40044,#8590,.T.);
#50936=EDGE_CURVE('',#40045,#40044,#8591,.T.);
#50937=EDGE_CURVE('',#40046,#40045,#8592,.T.);
#50938=EDGE_CURVE('',#40046,#40043,#8593,.T.);
#50939=EDGE_CURVE('',#40047,#40048,#8594,.T.);
#50940=EDGE_CURVE('',#40044,#40048,#8595,.T.);
#50941=EDGE_CURVE('',#40043,#40047,#8596,.T.);
#50942=EDGE_CURVE('',#40049,#40050,#8597,.T.);
#50943=EDGE_CURVE('',#40048,#40050,#8598,.T.);
#50944=EDGE_CURVE('',#40047,#40049,#8599,.T.);
#50945=EDGE_CURVE('',#40050,#40045,#8600,.T.);
#50946=EDGE_CURVE('',#40049,#40046,#8601,.T.);
#50947=EDGE_CURVE('',#40051,#40052,#8602,.T.);
#50948=EDGE_CURVE('',#40053,#40052,#8603,.T.);
#50949=EDGE_CURVE('',#40054,#40053,#8604,.T.);
#50950=EDGE_CURVE('',#40054,#40051,#8605,.T.);
#50951=EDGE_CURVE('',#40055,#40056,#8606,.T.);
#50952=EDGE_CURVE('',#40052,#40056,#8607,.T.);
#50953=EDGE_CURVE('',#40051,#40055,#8608,.T.);
#50954=EDGE_CURVE('',#40057,#40058,#8609,.T.);
#50955=EDGE_CURVE('',#40056,#40058,#8610,.T.);
#50956=EDGE_CURVE('',#40055,#40057,#8611,.T.);
#50957=EDGE_CURVE('',#40058,#40053,#8612,.T.);
#50958=EDGE_CURVE('',#40057,#40054,#8613,.T.);
#50959=EDGE_CURVE('',#40059,#40060,#8614,.T.);
#50960=EDGE_CURVE('',#40061,#40060,#8615,.T.);
#50961=EDGE_CURVE('',#40062,#40061,#8616,.T.);
#50962=EDGE_CURVE('',#40062,#40059,#8617,.T.);
#50963=EDGE_CURVE('',#40063,#40064,#8618,.T.);
#50964=EDGE_CURVE('',#40060,#40064,#8619,.T.);
#50965=EDGE_CURVE('',#40059,#40063,#8620,.T.);
#50966=EDGE_CURVE('',#40065,#40066,#8621,.T.);
#50967=EDGE_CURVE('',#40064,#40066,#8622,.T.);
#50968=EDGE_CURVE('',#40063,#40065,#8623,.T.);
#50969=EDGE_CURVE('',#40066,#40061,#8624,.T.);
#50970=EDGE_CURVE('',#40065,#40062,#8625,.T.);
#50971=EDGE_CURVE('',#40067,#40068,#8626,.T.);
#50972=EDGE_CURVE('',#40069,#40068,#8627,.T.);
#50973=EDGE_CURVE('',#40070,#40069,#8628,.T.);
#50974=EDGE_CURVE('',#40070,#40067,#8629,.T.);
#50975=EDGE_CURVE('',#40071,#40072,#8630,.T.);
#50976=EDGE_CURVE('',#40068,#40072,#8631,.T.);
#50977=EDGE_CURVE('',#40067,#40071,#8632,.T.);
#50978=EDGE_CURVE('',#40073,#40074,#8633,.T.);
#50979=EDGE_CURVE('',#40072,#40074,#8634,.T.);
#50980=EDGE_CURVE('',#40071,#40073,#8635,.T.);
#50981=EDGE_CURVE('',#40074,#40069,#8636,.T.);
#50982=EDGE_CURVE('',#40073,#40070,#8637,.T.);
#50983=EDGE_CURVE('',#40075,#40076,#8638,.T.);
#50984=EDGE_CURVE('',#40077,#40076,#8639,.T.);
#50985=EDGE_CURVE('',#40078,#40077,#8640,.T.);
#50986=EDGE_CURVE('',#40078,#40075,#8641,.T.);
#50987=EDGE_CURVE('',#40079,#40080,#8642,.T.);
#50988=EDGE_CURVE('',#40076,#40080,#8643,.T.);
#50989=EDGE_CURVE('',#40075,#40079,#8644,.T.);
#50990=EDGE_CURVE('',#40081,#40082,#8645,.T.);
#50991=EDGE_CURVE('',#40080,#40082,#8646,.T.);
#50992=EDGE_CURVE('',#40079,#40081,#8647,.T.);
#50993=EDGE_CURVE('',#40082,#40077,#8648,.T.);
#50994=EDGE_CURVE('',#40081,#40078,#8649,.T.);
#50995=EDGE_CURVE('',#40083,#40084,#8650,.T.);
#50996=EDGE_CURVE('',#40085,#40084,#8651,.T.);
#50997=EDGE_CURVE('',#40086,#40085,#8652,.T.);
#50998=EDGE_CURVE('',#40086,#40083,#8653,.T.);
#50999=EDGE_CURVE('',#40087,#40088,#8654,.T.);
#51000=EDGE_CURVE('',#40084,#40088,#8655,.T.);
#51001=EDGE_CURVE('',#40083,#40087,#8656,.T.);
#51002=EDGE_CURVE('',#40089,#40090,#8657,.T.);
#51003=EDGE_CURVE('',#40088,#40090,#8658,.T.);
#51004=EDGE_CURVE('',#40087,#40089,#8659,.T.);
#51005=EDGE_CURVE('',#40090,#40085,#8660,.T.);
#51006=EDGE_CURVE('',#40089,#40086,#8661,.T.);
#51007=EDGE_CURVE('',#40091,#40092,#8662,.T.);
#51008=EDGE_CURVE('',#40093,#40092,#8663,.T.);
#51009=EDGE_CURVE('',#40094,#40093,#8664,.T.);
#51010=EDGE_CURVE('',#40094,#40091,#8665,.T.);
#51011=EDGE_CURVE('',#40095,#40096,#8666,.T.);
#51012=EDGE_CURVE('',#40092,#40096,#8667,.T.);
#51013=EDGE_CURVE('',#40091,#40095,#8668,.T.);
#51014=EDGE_CURVE('',#40097,#40098,#8669,.T.);
#51015=EDGE_CURVE('',#40096,#40098,#8670,.T.);
#51016=EDGE_CURVE('',#40095,#40097,#8671,.T.);
#51017=EDGE_CURVE('',#40098,#40093,#8672,.T.);
#51018=EDGE_CURVE('',#40097,#40094,#8673,.T.);
#51019=EDGE_CURVE('',#40099,#40100,#8674,.T.);
#51020=EDGE_CURVE('',#40101,#40100,#8675,.T.);
#51021=EDGE_CURVE('',#40102,#40101,#8676,.T.);
#51022=EDGE_CURVE('',#40102,#40099,#8677,.T.);
#51023=EDGE_CURVE('',#40103,#40104,#8678,.T.);
#51024=EDGE_CURVE('',#40100,#40104,#8679,.T.);
#51025=EDGE_CURVE('',#40099,#40103,#8680,.T.);
#51026=EDGE_CURVE('',#40105,#40106,#8681,.T.);
#51027=EDGE_CURVE('',#40104,#40106,#8682,.T.);
#51028=EDGE_CURVE('',#40103,#40105,#8683,.T.);
#51029=EDGE_CURVE('',#40106,#40101,#8684,.T.);
#51030=EDGE_CURVE('',#40105,#40102,#8685,.T.);
#51031=EDGE_CURVE('',#40107,#40108,#8686,.T.);
#51032=EDGE_CURVE('',#40109,#40108,#8687,.T.);
#51033=EDGE_CURVE('',#40110,#40109,#8688,.T.);
#51034=EDGE_CURVE('',#40110,#40107,#8689,.T.);
#51035=EDGE_CURVE('',#40111,#40112,#8690,.T.);
#51036=EDGE_CURVE('',#40108,#40112,#8691,.T.);
#51037=EDGE_CURVE('',#40107,#40111,#8692,.T.);
#51038=EDGE_CURVE('',#40113,#40114,#8693,.T.);
#51039=EDGE_CURVE('',#40112,#40114,#8694,.T.);
#51040=EDGE_CURVE('',#40111,#40113,#8695,.T.);
#51041=EDGE_CURVE('',#40114,#40109,#8696,.T.);
#51042=EDGE_CURVE('',#40113,#40110,#8697,.T.);
#51043=EDGE_CURVE('',#40115,#40116,#8698,.T.);
#51044=EDGE_CURVE('',#40117,#40116,#8699,.T.);
#51045=EDGE_CURVE('',#40118,#40117,#8700,.T.);
#51046=EDGE_CURVE('',#40118,#40115,#8701,.T.);
#51047=EDGE_CURVE('',#40119,#40120,#8702,.T.);
#51048=EDGE_CURVE('',#40116,#40120,#8703,.T.);
#51049=EDGE_CURVE('',#40115,#40119,#8704,.T.);
#51050=EDGE_CURVE('',#40121,#40122,#8705,.T.);
#51051=EDGE_CURVE('',#40120,#40122,#8706,.T.);
#51052=EDGE_CURVE('',#40119,#40121,#8707,.T.);
#51053=EDGE_CURVE('',#40122,#40117,#8708,.T.);
#51054=EDGE_CURVE('',#40121,#40118,#8709,.T.);
#51055=EDGE_CURVE('',#40123,#40124,#8710,.T.);
#51056=EDGE_CURVE('',#40125,#40124,#8711,.T.);
#51057=EDGE_CURVE('',#40126,#40125,#8712,.T.);
#51058=EDGE_CURVE('',#40126,#40123,#8713,.T.);
#51059=EDGE_CURVE('',#40127,#40128,#8714,.T.);
#51060=EDGE_CURVE('',#40124,#40128,#8715,.T.);
#51061=EDGE_CURVE('',#40123,#40127,#8716,.T.);
#51062=EDGE_CURVE('',#40129,#40130,#8717,.T.);
#51063=EDGE_CURVE('',#40128,#40130,#8718,.T.);
#51064=EDGE_CURVE('',#40127,#40129,#8719,.T.);
#51065=EDGE_CURVE('',#40130,#40125,#8720,.T.);
#51066=EDGE_CURVE('',#40129,#40126,#8721,.T.);
#51067=EDGE_CURVE('',#40131,#40132,#8722,.T.);
#51068=EDGE_CURVE('',#40133,#40132,#8723,.T.);
#51069=EDGE_CURVE('',#40134,#40133,#8724,.T.);
#51070=EDGE_CURVE('',#40134,#40131,#8725,.T.);
#51071=EDGE_CURVE('',#40135,#40136,#8726,.T.);
#51072=EDGE_CURVE('',#40132,#40136,#8727,.T.);
#51073=EDGE_CURVE('',#40131,#40135,#8728,.T.);
#51074=EDGE_CURVE('',#40137,#40138,#8729,.T.);
#51075=EDGE_CURVE('',#40136,#40138,#8730,.T.);
#51076=EDGE_CURVE('',#40135,#40137,#8731,.T.);
#51077=EDGE_CURVE('',#40138,#40133,#8732,.T.);
#51078=EDGE_CURVE('',#40137,#40134,#8733,.T.);
#51079=EDGE_CURVE('',#40139,#40140,#8734,.T.);
#51080=EDGE_CURVE('',#40141,#40140,#8735,.T.);
#51081=EDGE_CURVE('',#40142,#40141,#8736,.T.);
#51082=EDGE_CURVE('',#40142,#40139,#8737,.T.);
#51083=EDGE_CURVE('',#40143,#40144,#8738,.T.);
#51084=EDGE_CURVE('',#40140,#40144,#8739,.T.);
#51085=EDGE_CURVE('',#40139,#40143,#8740,.T.);
#51086=EDGE_CURVE('',#40145,#40146,#8741,.T.);
#51087=EDGE_CURVE('',#40144,#40146,#8742,.T.);
#51088=EDGE_CURVE('',#40143,#40145,#8743,.T.);
#51089=EDGE_CURVE('',#40146,#40141,#8744,.T.);
#51090=EDGE_CURVE('',#40145,#40142,#8745,.T.);
#51091=EDGE_CURVE('',#40147,#40148,#8746,.T.);
#51092=EDGE_CURVE('',#40149,#40148,#8747,.T.);
#51093=EDGE_CURVE('',#40150,#40149,#8748,.T.);
#51094=EDGE_CURVE('',#40150,#40147,#8749,.T.);
#51095=EDGE_CURVE('',#40151,#40152,#8750,.T.);
#51096=EDGE_CURVE('',#40148,#40152,#8751,.T.);
#51097=EDGE_CURVE('',#40147,#40151,#8752,.T.);
#51098=EDGE_CURVE('',#40153,#40154,#8753,.T.);
#51099=EDGE_CURVE('',#40152,#40154,#8754,.T.);
#51100=EDGE_CURVE('',#40151,#40153,#8755,.T.);
#51101=EDGE_CURVE('',#40154,#40149,#8756,.T.);
#51102=EDGE_CURVE('',#40153,#40150,#8757,.T.);
#51103=EDGE_CURVE('',#40155,#40156,#8758,.T.);
#51104=EDGE_CURVE('',#40157,#40156,#8759,.T.);
#51105=EDGE_CURVE('',#40158,#40157,#8760,.T.);
#51106=EDGE_CURVE('',#40158,#40155,#8761,.T.);
#51107=EDGE_CURVE('',#40159,#40160,#8762,.T.);
#51108=EDGE_CURVE('',#40156,#40160,#8763,.T.);
#51109=EDGE_CURVE('',#40155,#40159,#8764,.T.);
#51110=EDGE_CURVE('',#40161,#40162,#8765,.T.);
#51111=EDGE_CURVE('',#40160,#40162,#8766,.T.);
#51112=EDGE_CURVE('',#40159,#40161,#8767,.T.);
#51113=EDGE_CURVE('',#40162,#40157,#8768,.T.);
#51114=EDGE_CURVE('',#40161,#40158,#8769,.T.);
#51115=EDGE_CURVE('',#40163,#40164,#8770,.T.);
#51116=EDGE_CURVE('',#40165,#40164,#8771,.T.);
#51117=EDGE_CURVE('',#40166,#40165,#8772,.T.);
#51118=EDGE_CURVE('',#40166,#40163,#8773,.T.);
#51119=EDGE_CURVE('',#40167,#40168,#8774,.T.);
#51120=EDGE_CURVE('',#40164,#40168,#8775,.T.);
#51121=EDGE_CURVE('',#40163,#40167,#8776,.T.);
#51122=EDGE_CURVE('',#40169,#40170,#8777,.T.);
#51123=EDGE_CURVE('',#40168,#40170,#8778,.T.);
#51124=EDGE_CURVE('',#40167,#40169,#8779,.T.);
#51125=EDGE_CURVE('',#40170,#40165,#8780,.T.);
#51126=EDGE_CURVE('',#40169,#40166,#8781,.T.);
#51127=EDGE_CURVE('',#40171,#40172,#8782,.T.);
#51128=EDGE_CURVE('',#40173,#40172,#8783,.T.);
#51129=EDGE_CURVE('',#40174,#40173,#8784,.T.);
#51130=EDGE_CURVE('',#40174,#40171,#8785,.T.);
#51131=EDGE_CURVE('',#40175,#40176,#8786,.T.);
#51132=EDGE_CURVE('',#40172,#40176,#8787,.T.);
#51133=EDGE_CURVE('',#40171,#40175,#8788,.T.);
#51134=EDGE_CURVE('',#40177,#40178,#8789,.T.);
#51135=EDGE_CURVE('',#40176,#40178,#8790,.T.);
#51136=EDGE_CURVE('',#40175,#40177,#8791,.T.);
#51137=EDGE_CURVE('',#40178,#40173,#8792,.T.);
#51138=EDGE_CURVE('',#40177,#40174,#8793,.T.);
#51139=EDGE_CURVE('',#40179,#40180,#8794,.T.);
#51140=EDGE_CURVE('',#40181,#40180,#8795,.T.);
#51141=EDGE_CURVE('',#40182,#40181,#8796,.T.);
#51142=EDGE_CURVE('',#40182,#40179,#8797,.T.);
#51143=EDGE_CURVE('',#40183,#40184,#8798,.T.);
#51144=EDGE_CURVE('',#40180,#40184,#8799,.T.);
#51145=EDGE_CURVE('',#40179,#40183,#8800,.T.);
#51146=EDGE_CURVE('',#40185,#40186,#8801,.T.);
#51147=EDGE_CURVE('',#40184,#40186,#8802,.T.);
#51148=EDGE_CURVE('',#40183,#40185,#8803,.T.);
#51149=EDGE_CURVE('',#40186,#40181,#8804,.T.);
#51150=EDGE_CURVE('',#40185,#40182,#8805,.T.);
#51151=EDGE_CURVE('',#40187,#40188,#8806,.T.);
#51152=EDGE_CURVE('',#40189,#40188,#8807,.T.);
#51153=EDGE_CURVE('',#40190,#40189,#8808,.T.);
#51154=EDGE_CURVE('',#40190,#40187,#8809,.T.);
#51155=EDGE_CURVE('',#40191,#40192,#8810,.T.);
#51156=EDGE_CURVE('',#40188,#40192,#8811,.T.);
#51157=EDGE_CURVE('',#40187,#40191,#8812,.T.);
#51158=EDGE_CURVE('',#40193,#40194,#8813,.T.);
#51159=EDGE_CURVE('',#40192,#40194,#8814,.T.);
#51160=EDGE_CURVE('',#40191,#40193,#8815,.T.);
#51161=EDGE_CURVE('',#40194,#40189,#8816,.T.);
#51162=EDGE_CURVE('',#40193,#40190,#8817,.T.);
#51163=EDGE_CURVE('',#40195,#40196,#8818,.T.);
#51164=EDGE_CURVE('',#40197,#40196,#8819,.T.);
#51165=EDGE_CURVE('',#40198,#40197,#8820,.T.);
#51166=EDGE_CURVE('',#40198,#40195,#8821,.T.);
#51167=EDGE_CURVE('',#40199,#40200,#8822,.T.);
#51168=EDGE_CURVE('',#40196,#40200,#8823,.T.);
#51169=EDGE_CURVE('',#40195,#40199,#8824,.T.);
#51170=EDGE_CURVE('',#40201,#40202,#8825,.T.);
#51171=EDGE_CURVE('',#40200,#40202,#8826,.T.);
#51172=EDGE_CURVE('',#40199,#40201,#8827,.T.);
#51173=EDGE_CURVE('',#40202,#40197,#8828,.T.);
#51174=EDGE_CURVE('',#40201,#40198,#8829,.T.);
#51175=EDGE_CURVE('',#40203,#40204,#8830,.T.);
#51176=EDGE_CURVE('',#40205,#40204,#8831,.T.);
#51177=EDGE_CURVE('',#40206,#40205,#8832,.T.);
#51178=EDGE_CURVE('',#40206,#40203,#8833,.T.);
#51179=EDGE_CURVE('',#40207,#40208,#8834,.T.);
#51180=EDGE_CURVE('',#40204,#40208,#8835,.T.);
#51181=EDGE_CURVE('',#40203,#40207,#8836,.T.);
#51182=EDGE_CURVE('',#40209,#40210,#8837,.T.);
#51183=EDGE_CURVE('',#40208,#40210,#8838,.T.);
#51184=EDGE_CURVE('',#40207,#40209,#8839,.T.);
#51185=EDGE_CURVE('',#40210,#40205,#8840,.T.);
#51186=EDGE_CURVE('',#40209,#40206,#8841,.T.);
#51187=EDGE_CURVE('',#40211,#40212,#8842,.T.);
#51188=EDGE_CURVE('',#40213,#40212,#8843,.T.);
#51189=EDGE_CURVE('',#40214,#40213,#8844,.T.);
#51190=EDGE_CURVE('',#40214,#40211,#8845,.T.);
#51191=EDGE_CURVE('',#40215,#40216,#8846,.T.);
#51192=EDGE_CURVE('',#40212,#40216,#8847,.T.);
#51193=EDGE_CURVE('',#40211,#40215,#8848,.T.);
#51194=EDGE_CURVE('',#40217,#40218,#8849,.T.);
#51195=EDGE_CURVE('',#40216,#40218,#8850,.T.);
#51196=EDGE_CURVE('',#40215,#40217,#8851,.T.);
#51197=EDGE_CURVE('',#40218,#40213,#8852,.T.);
#51198=EDGE_CURVE('',#40217,#40214,#8853,.T.);
#51199=EDGE_CURVE('',#40219,#40220,#8854,.T.);
#51200=EDGE_CURVE('',#40221,#40220,#8855,.T.);
#51201=EDGE_CURVE('',#40222,#40221,#8856,.T.);
#51202=EDGE_CURVE('',#40222,#40219,#8857,.T.);
#51203=EDGE_CURVE('',#40223,#40224,#8858,.T.);
#51204=EDGE_CURVE('',#40220,#40224,#8859,.T.);
#51205=EDGE_CURVE('',#40219,#40223,#8860,.T.);
#51206=EDGE_CURVE('',#40225,#40226,#8861,.T.);
#51207=EDGE_CURVE('',#40224,#40226,#8862,.T.);
#51208=EDGE_CURVE('',#40223,#40225,#8863,.T.);
#51209=EDGE_CURVE('',#40226,#40221,#8864,.T.);
#51210=EDGE_CURVE('',#40225,#40222,#8865,.T.);
#51211=EDGE_CURVE('',#40227,#40228,#8866,.T.);
#51212=EDGE_CURVE('',#40229,#40228,#8867,.T.);
#51213=EDGE_CURVE('',#40230,#40229,#8868,.T.);
#51214=EDGE_CURVE('',#40230,#40227,#8869,.T.);
#51215=EDGE_CURVE('',#40231,#40232,#8870,.T.);
#51216=EDGE_CURVE('',#40228,#40232,#8871,.T.);
#51217=EDGE_CURVE('',#40227,#40231,#8872,.T.);
#51218=EDGE_CURVE('',#40233,#40234,#8873,.T.);
#51219=EDGE_CURVE('',#40232,#40234,#8874,.T.);
#51220=EDGE_CURVE('',#40231,#40233,#8875,.T.);
#51221=EDGE_CURVE('',#40234,#40229,#8876,.T.);
#51222=EDGE_CURVE('',#40233,#40230,#8877,.T.);
#51223=EDGE_CURVE('',#40235,#40236,#8878,.T.);
#51224=EDGE_CURVE('',#40237,#40236,#8879,.T.);
#51225=EDGE_CURVE('',#40238,#40237,#8880,.T.);
#51226=EDGE_CURVE('',#40238,#40235,#8881,.T.);
#51227=EDGE_CURVE('',#40239,#40240,#8882,.T.);
#51228=EDGE_CURVE('',#40236,#40240,#8883,.T.);
#51229=EDGE_CURVE('',#40235,#40239,#8884,.T.);
#51230=EDGE_CURVE('',#40241,#40242,#8885,.T.);
#51231=EDGE_CURVE('',#40240,#40242,#8886,.T.);
#51232=EDGE_CURVE('',#40239,#40241,#8887,.T.);
#51233=EDGE_CURVE('',#40242,#40237,#8888,.T.);
#51234=EDGE_CURVE('',#40241,#40238,#8889,.T.);
#51235=EDGE_CURVE('',#40243,#40244,#8890,.T.);
#51236=EDGE_CURVE('',#40245,#40244,#8891,.T.);
#51237=EDGE_CURVE('',#40246,#40245,#8892,.T.);
#51238=EDGE_CURVE('',#40246,#40243,#8893,.T.);
#51239=EDGE_CURVE('',#40247,#40248,#8894,.T.);
#51240=EDGE_CURVE('',#40244,#40248,#8895,.T.);
#51241=EDGE_CURVE('',#40243,#40247,#8896,.T.);
#51242=EDGE_CURVE('',#40249,#40250,#8897,.T.);
#51243=EDGE_CURVE('',#40248,#40250,#8898,.T.);
#51244=EDGE_CURVE('',#40247,#40249,#8899,.T.);
#51245=EDGE_CURVE('',#40250,#40245,#8900,.T.);
#51246=EDGE_CURVE('',#40249,#40246,#8901,.T.);
#51247=EDGE_CURVE('',#40251,#40252,#8902,.T.);
#51248=EDGE_CURVE('',#40253,#40252,#8903,.T.);
#51249=EDGE_CURVE('',#40254,#40253,#8904,.T.);
#51250=EDGE_CURVE('',#40254,#40251,#8905,.T.);
#51251=EDGE_CURVE('',#40255,#40256,#8906,.T.);
#51252=EDGE_CURVE('',#40252,#40256,#8907,.T.);
#51253=EDGE_CURVE('',#40251,#40255,#8908,.T.);
#51254=EDGE_CURVE('',#40257,#40258,#8909,.T.);
#51255=EDGE_CURVE('',#40256,#40258,#8910,.T.);
#51256=EDGE_CURVE('',#40255,#40257,#8911,.T.);
#51257=EDGE_CURVE('',#40258,#40253,#8912,.T.);
#51258=EDGE_CURVE('',#40257,#40254,#8913,.T.);
#51259=EDGE_CURVE('',#40259,#40260,#8914,.T.);
#51260=EDGE_CURVE('',#40261,#40260,#8915,.T.);
#51261=EDGE_CURVE('',#40262,#40261,#8916,.T.);
#51262=EDGE_CURVE('',#40262,#40259,#8917,.T.);
#51263=EDGE_CURVE('',#40263,#40264,#8918,.T.);
#51264=EDGE_CURVE('',#40260,#40264,#8919,.T.);
#51265=EDGE_CURVE('',#40259,#40263,#8920,.T.);
#51266=EDGE_CURVE('',#40265,#40266,#8921,.T.);
#51267=EDGE_CURVE('',#40264,#40266,#8922,.T.);
#51268=EDGE_CURVE('',#40263,#40265,#8923,.T.);
#51269=EDGE_CURVE('',#40266,#40261,#8924,.T.);
#51270=EDGE_CURVE('',#40265,#40262,#8925,.T.);
#51271=EDGE_CURVE('',#40267,#40268,#8926,.T.);
#51272=EDGE_CURVE('',#40269,#40268,#8927,.T.);
#51273=EDGE_CURVE('',#40270,#40269,#8928,.T.);
#51274=EDGE_CURVE('',#40270,#40267,#8929,.T.);
#51275=EDGE_CURVE('',#40271,#40272,#8930,.T.);
#51276=EDGE_CURVE('',#40268,#40272,#8931,.T.);
#51277=EDGE_CURVE('',#40267,#40271,#8932,.T.);
#51278=EDGE_CURVE('',#40273,#40274,#8933,.T.);
#51279=EDGE_CURVE('',#40272,#40274,#8934,.T.);
#51280=EDGE_CURVE('',#40271,#40273,#8935,.T.);
#51281=EDGE_CURVE('',#40274,#40269,#8936,.T.);
#51282=EDGE_CURVE('',#40273,#40270,#8937,.T.);
#51283=EDGE_CURVE('',#40275,#40276,#8938,.T.);
#51284=EDGE_CURVE('',#40277,#40276,#8939,.T.);
#51285=EDGE_CURVE('',#40278,#40277,#8940,.T.);
#51286=EDGE_CURVE('',#40278,#40275,#8941,.T.);
#51287=EDGE_CURVE('',#40279,#40280,#8942,.T.);
#51288=EDGE_CURVE('',#40276,#40280,#8943,.T.);
#51289=EDGE_CURVE('',#40275,#40279,#8944,.T.);
#51290=EDGE_CURVE('',#40281,#40282,#8945,.T.);
#51291=EDGE_CURVE('',#40280,#40282,#8946,.T.);
#51292=EDGE_CURVE('',#40279,#40281,#8947,.T.);
#51293=EDGE_CURVE('',#40282,#40277,#8948,.T.);
#51294=EDGE_CURVE('',#40281,#40278,#8949,.T.);
#51295=EDGE_CURVE('',#40283,#40284,#8950,.T.);
#51296=EDGE_CURVE('',#40285,#40284,#8951,.T.);
#51297=EDGE_CURVE('',#40286,#40285,#8952,.T.);
#51298=EDGE_CURVE('',#40286,#40283,#8953,.T.);
#51299=EDGE_CURVE('',#40287,#40288,#8954,.T.);
#51300=EDGE_CURVE('',#40284,#40288,#8955,.T.);
#51301=EDGE_CURVE('',#40283,#40287,#8956,.T.);
#51302=EDGE_CURVE('',#40289,#40290,#8957,.T.);
#51303=EDGE_CURVE('',#40288,#40290,#8958,.T.);
#51304=EDGE_CURVE('',#40287,#40289,#8959,.T.);
#51305=EDGE_CURVE('',#40290,#40285,#8960,.T.);
#51306=EDGE_CURVE('',#40289,#40286,#8961,.T.);
#51307=EDGE_CURVE('',#40291,#40292,#8962,.T.);
#51308=EDGE_CURVE('',#40293,#40292,#8963,.T.);
#51309=EDGE_CURVE('',#40294,#40293,#8964,.T.);
#51310=EDGE_CURVE('',#40294,#40291,#8965,.T.);
#51311=EDGE_CURVE('',#40295,#40296,#8966,.T.);
#51312=EDGE_CURVE('',#40292,#40296,#8967,.T.);
#51313=EDGE_CURVE('',#40291,#40295,#8968,.T.);
#51314=EDGE_CURVE('',#40297,#40298,#8969,.T.);
#51315=EDGE_CURVE('',#40296,#40298,#8970,.T.);
#51316=EDGE_CURVE('',#40295,#40297,#8971,.T.);
#51317=EDGE_CURVE('',#40298,#40293,#8972,.T.);
#51318=EDGE_CURVE('',#40297,#40294,#8973,.T.);
#51319=EDGE_CURVE('',#40299,#40300,#8974,.T.);
#51320=EDGE_CURVE('',#40301,#40300,#8975,.T.);
#51321=EDGE_CURVE('',#40302,#40301,#8976,.T.);
#51322=EDGE_CURVE('',#40302,#40299,#8977,.T.);
#51323=EDGE_CURVE('',#40303,#40304,#8978,.T.);
#51324=EDGE_CURVE('',#40300,#40304,#8979,.T.);
#51325=EDGE_CURVE('',#40299,#40303,#8980,.T.);
#51326=EDGE_CURVE('',#40305,#40306,#8981,.T.);
#51327=EDGE_CURVE('',#40304,#40306,#8982,.T.);
#51328=EDGE_CURVE('',#40303,#40305,#8983,.T.);
#51329=EDGE_CURVE('',#40306,#40301,#8984,.T.);
#51330=EDGE_CURVE('',#40305,#40302,#8985,.T.);
#51331=EDGE_CURVE('',#40307,#40308,#8986,.T.);
#51332=EDGE_CURVE('',#40309,#40308,#8987,.T.);
#51333=EDGE_CURVE('',#40310,#40309,#8988,.T.);
#51334=EDGE_CURVE('',#40310,#40307,#8989,.T.);
#51335=EDGE_CURVE('',#40311,#40312,#8990,.T.);
#51336=EDGE_CURVE('',#40308,#40312,#8991,.T.);
#51337=EDGE_CURVE('',#40307,#40311,#8992,.T.);
#51338=EDGE_CURVE('',#40313,#40314,#8993,.T.);
#51339=EDGE_CURVE('',#40312,#40314,#8994,.T.);
#51340=EDGE_CURVE('',#40311,#40313,#8995,.T.);
#51341=EDGE_CURVE('',#40314,#40309,#8996,.T.);
#51342=EDGE_CURVE('',#40313,#40310,#8997,.T.);
#51343=EDGE_CURVE('',#40315,#40316,#8998,.T.);
#51344=EDGE_CURVE('',#40317,#40316,#8999,.T.);
#51345=EDGE_CURVE('',#40318,#40317,#9000,.T.);
#51346=EDGE_CURVE('',#40318,#40315,#9001,.T.);
#51347=EDGE_CURVE('',#40319,#40320,#9002,.T.);
#51348=EDGE_CURVE('',#40316,#40320,#9003,.T.);
#51349=EDGE_CURVE('',#40315,#40319,#9004,.T.);
#51350=EDGE_CURVE('',#40321,#40322,#9005,.T.);
#51351=EDGE_CURVE('',#40320,#40322,#9006,.T.);
#51352=EDGE_CURVE('',#40319,#40321,#9007,.T.);
#51353=EDGE_CURVE('',#40322,#40317,#9008,.T.);
#51354=EDGE_CURVE('',#40321,#40318,#9009,.T.);
#51355=EDGE_CURVE('',#40323,#40324,#9010,.T.);
#51356=EDGE_CURVE('',#40325,#40324,#9011,.T.);
#51357=EDGE_CURVE('',#40326,#40325,#9012,.T.);
#51358=EDGE_CURVE('',#40326,#40323,#9013,.T.);
#51359=EDGE_CURVE('',#40327,#40328,#9014,.T.);
#51360=EDGE_CURVE('',#40324,#40328,#9015,.T.);
#51361=EDGE_CURVE('',#40323,#40327,#9016,.T.);
#51362=EDGE_CURVE('',#40329,#40330,#9017,.T.);
#51363=EDGE_CURVE('',#40328,#40330,#9018,.T.);
#51364=EDGE_CURVE('',#40327,#40329,#9019,.T.);
#51365=EDGE_CURVE('',#40330,#40325,#9020,.T.);
#51366=EDGE_CURVE('',#40329,#40326,#9021,.T.);
#51367=EDGE_CURVE('',#40331,#40332,#9022,.T.);
#51368=EDGE_CURVE('',#40333,#40332,#9023,.T.);
#51369=EDGE_CURVE('',#40334,#40333,#9024,.T.);
#51370=EDGE_CURVE('',#40334,#40331,#9025,.T.);
#51371=EDGE_CURVE('',#40335,#40336,#9026,.T.);
#51372=EDGE_CURVE('',#40332,#40336,#9027,.T.);
#51373=EDGE_CURVE('',#40331,#40335,#9028,.T.);
#51374=EDGE_CURVE('',#40337,#40338,#9029,.T.);
#51375=EDGE_CURVE('',#40336,#40338,#9030,.T.);
#51376=EDGE_CURVE('',#40335,#40337,#9031,.T.);
#51377=EDGE_CURVE('',#40338,#40333,#9032,.T.);
#51378=EDGE_CURVE('',#40337,#40334,#9033,.T.);
#51379=EDGE_CURVE('',#40339,#40340,#9034,.T.);
#51380=EDGE_CURVE('',#40341,#40340,#9035,.T.);
#51381=EDGE_CURVE('',#40342,#40341,#9036,.T.);
#51382=EDGE_CURVE('',#40342,#40339,#9037,.T.);
#51383=EDGE_CURVE('',#40343,#40344,#9038,.T.);
#51384=EDGE_CURVE('',#40340,#40344,#9039,.T.);
#51385=EDGE_CURVE('',#40339,#40343,#9040,.T.);
#51386=EDGE_CURVE('',#40345,#40346,#9041,.T.);
#51387=EDGE_CURVE('',#40344,#40346,#9042,.T.);
#51388=EDGE_CURVE('',#40343,#40345,#9043,.T.);
#51389=EDGE_CURVE('',#40346,#40341,#9044,.T.);
#51390=EDGE_CURVE('',#40345,#40342,#9045,.T.);
#51391=EDGE_CURVE('',#40347,#40348,#9046,.T.);
#51392=EDGE_CURVE('',#40349,#40348,#9047,.T.);
#51393=EDGE_CURVE('',#40350,#40349,#9048,.T.);
#51394=EDGE_CURVE('',#40350,#40347,#9049,.T.);
#51395=EDGE_CURVE('',#40351,#40352,#9050,.T.);
#51396=EDGE_CURVE('',#40348,#40352,#9051,.T.);
#51397=EDGE_CURVE('',#40347,#40351,#9052,.T.);
#51398=EDGE_CURVE('',#40353,#40354,#9053,.T.);
#51399=EDGE_CURVE('',#40352,#40354,#9054,.T.);
#51400=EDGE_CURVE('',#40351,#40353,#9055,.T.);
#51401=EDGE_CURVE('',#40354,#40349,#9056,.T.);
#51402=EDGE_CURVE('',#40353,#40350,#9057,.T.);
#51403=EDGE_CURVE('',#40355,#40356,#9058,.T.);
#51404=EDGE_CURVE('',#40357,#40356,#9059,.T.);
#51405=EDGE_CURVE('',#40358,#40357,#9060,.T.);
#51406=EDGE_CURVE('',#40358,#40355,#9061,.T.);
#51407=EDGE_CURVE('',#40359,#40360,#9062,.T.);
#51408=EDGE_CURVE('',#40356,#40360,#9063,.T.);
#51409=EDGE_CURVE('',#40355,#40359,#9064,.T.);
#51410=EDGE_CURVE('',#40361,#40362,#9065,.T.);
#51411=EDGE_CURVE('',#40360,#40362,#9066,.T.);
#51412=EDGE_CURVE('',#40359,#40361,#9067,.T.);
#51413=EDGE_CURVE('',#40362,#40357,#9068,.T.);
#51414=EDGE_CURVE('',#40361,#40358,#9069,.T.);
#51415=EDGE_CURVE('',#40363,#40364,#9070,.T.);
#51416=EDGE_CURVE('',#40365,#40364,#9071,.T.);
#51417=EDGE_CURVE('',#40366,#40365,#9072,.T.);
#51418=EDGE_CURVE('',#40366,#40363,#9073,.T.);
#51419=EDGE_CURVE('',#40367,#40368,#9074,.T.);
#51420=EDGE_CURVE('',#40364,#40368,#9075,.T.);
#51421=EDGE_CURVE('',#40363,#40367,#9076,.T.);
#51422=EDGE_CURVE('',#40369,#40370,#9077,.T.);
#51423=EDGE_CURVE('',#40368,#40370,#9078,.T.);
#51424=EDGE_CURVE('',#40367,#40369,#9079,.T.);
#51425=EDGE_CURVE('',#40370,#40365,#9080,.T.);
#51426=EDGE_CURVE('',#40369,#40366,#9081,.T.);
#51427=EDGE_CURVE('',#40371,#40372,#9082,.T.);
#51428=EDGE_CURVE('',#40373,#40372,#9083,.T.);
#51429=EDGE_CURVE('',#40374,#40373,#9084,.T.);
#51430=EDGE_CURVE('',#40374,#40371,#9085,.T.);
#51431=EDGE_CURVE('',#40375,#40376,#9086,.T.);
#51432=EDGE_CURVE('',#40372,#40376,#9087,.T.);
#51433=EDGE_CURVE('',#40371,#40375,#9088,.T.);
#51434=EDGE_CURVE('',#40377,#40378,#9089,.T.);
#51435=EDGE_CURVE('',#40376,#40378,#9090,.T.);
#51436=EDGE_CURVE('',#40375,#40377,#9091,.T.);
#51437=EDGE_CURVE('',#40378,#40373,#9092,.T.);
#51438=EDGE_CURVE('',#40377,#40374,#9093,.T.);
#51439=EDGE_CURVE('',#40379,#40380,#9094,.T.);
#51440=EDGE_CURVE('',#40381,#40380,#9095,.T.);
#51441=EDGE_CURVE('',#40382,#40381,#9096,.T.);
#51442=EDGE_CURVE('',#40382,#40379,#9097,.T.);
#51443=EDGE_CURVE('',#40383,#40384,#9098,.T.);
#51444=EDGE_CURVE('',#40380,#40384,#9099,.T.);
#51445=EDGE_CURVE('',#40379,#40383,#9100,.T.);
#51446=EDGE_CURVE('',#40385,#40386,#9101,.T.);
#51447=EDGE_CURVE('',#40384,#40386,#9102,.T.);
#51448=EDGE_CURVE('',#40383,#40385,#9103,.T.);
#51449=EDGE_CURVE('',#40386,#40381,#9104,.T.);
#51450=EDGE_CURVE('',#40385,#40382,#9105,.T.);
#51451=EDGE_CURVE('',#40387,#40388,#9106,.T.);
#51452=EDGE_CURVE('',#40389,#40388,#9107,.T.);
#51453=EDGE_CURVE('',#40390,#40389,#9108,.T.);
#51454=EDGE_CURVE('',#40390,#40387,#9109,.T.);
#51455=EDGE_CURVE('',#40391,#40392,#9110,.T.);
#51456=EDGE_CURVE('',#40388,#40392,#9111,.T.);
#51457=EDGE_CURVE('',#40387,#40391,#9112,.T.);
#51458=EDGE_CURVE('',#40393,#40394,#9113,.T.);
#51459=EDGE_CURVE('',#40392,#40394,#9114,.T.);
#51460=EDGE_CURVE('',#40391,#40393,#9115,.T.);
#51461=EDGE_CURVE('',#40394,#40389,#9116,.T.);
#51462=EDGE_CURVE('',#40393,#40390,#9117,.T.);
#51463=EDGE_CURVE('',#40395,#40396,#9118,.T.);
#51464=EDGE_CURVE('',#40397,#40396,#9119,.T.);
#51465=EDGE_CURVE('',#40398,#40397,#9120,.T.);
#51466=EDGE_CURVE('',#40398,#40395,#9121,.T.);
#51467=EDGE_CURVE('',#40399,#40400,#9122,.T.);
#51468=EDGE_CURVE('',#40396,#40400,#9123,.T.);
#51469=EDGE_CURVE('',#40395,#40399,#9124,.T.);
#51470=EDGE_CURVE('',#40401,#40402,#9125,.T.);
#51471=EDGE_CURVE('',#40400,#40402,#9126,.T.);
#51472=EDGE_CURVE('',#40399,#40401,#9127,.T.);
#51473=EDGE_CURVE('',#40402,#40397,#9128,.T.);
#51474=EDGE_CURVE('',#40401,#40398,#9129,.T.);
#51475=EDGE_CURVE('',#40403,#40404,#9130,.T.);
#51476=EDGE_CURVE('',#40405,#40404,#9131,.T.);
#51477=EDGE_CURVE('',#40406,#40405,#9132,.T.);
#51478=EDGE_CURVE('',#40406,#40403,#9133,.T.);
#51479=EDGE_CURVE('',#40407,#40408,#9134,.T.);
#51480=EDGE_CURVE('',#40404,#40408,#9135,.T.);
#51481=EDGE_CURVE('',#40403,#40407,#9136,.T.);
#51482=EDGE_CURVE('',#40409,#40410,#9137,.T.);
#51483=EDGE_CURVE('',#40408,#40410,#9138,.T.);
#51484=EDGE_CURVE('',#40407,#40409,#9139,.T.);
#51485=EDGE_CURVE('',#40410,#40405,#9140,.T.);
#51486=EDGE_CURVE('',#40409,#40406,#9141,.T.);
#51487=EDGE_CURVE('',#40411,#40412,#9142,.T.);
#51488=EDGE_CURVE('',#40413,#40412,#9143,.T.);
#51489=EDGE_CURVE('',#40414,#40413,#9144,.T.);
#51490=EDGE_CURVE('',#40414,#40411,#9145,.T.);
#51491=EDGE_CURVE('',#40415,#40416,#9146,.T.);
#51492=EDGE_CURVE('',#40412,#40416,#9147,.T.);
#51493=EDGE_CURVE('',#40411,#40415,#9148,.T.);
#51494=EDGE_CURVE('',#40417,#40418,#9149,.T.);
#51495=EDGE_CURVE('',#40416,#40418,#9150,.T.);
#51496=EDGE_CURVE('',#40415,#40417,#9151,.T.);
#51497=EDGE_CURVE('',#40418,#40413,#9152,.T.);
#51498=EDGE_CURVE('',#40417,#40414,#9153,.T.);
#51499=EDGE_CURVE('',#40419,#40420,#9154,.T.);
#51500=EDGE_CURVE('',#40421,#40420,#9155,.T.);
#51501=EDGE_CURVE('',#40422,#40421,#9156,.T.);
#51502=EDGE_CURVE('',#40422,#40419,#9157,.T.);
#51503=EDGE_CURVE('',#40423,#40424,#9158,.T.);
#51504=EDGE_CURVE('',#40420,#40424,#9159,.T.);
#51505=EDGE_CURVE('',#40419,#40423,#9160,.T.);
#51506=EDGE_CURVE('',#40425,#40426,#9161,.T.);
#51507=EDGE_CURVE('',#40424,#40426,#9162,.T.);
#51508=EDGE_CURVE('',#40423,#40425,#9163,.T.);
#51509=EDGE_CURVE('',#40426,#40421,#9164,.T.);
#51510=EDGE_CURVE('',#40425,#40422,#9165,.T.);
#51511=EDGE_CURVE('',#40427,#40428,#9166,.T.);
#51512=EDGE_CURVE('',#40429,#40428,#9167,.T.);
#51513=EDGE_CURVE('',#40430,#40429,#9168,.T.);
#51514=EDGE_CURVE('',#40430,#40427,#9169,.T.);
#51515=EDGE_CURVE('',#40431,#40432,#9170,.T.);
#51516=EDGE_CURVE('',#40428,#40432,#9171,.T.);
#51517=EDGE_CURVE('',#40427,#40431,#9172,.T.);
#51518=EDGE_CURVE('',#40433,#40434,#9173,.T.);
#51519=EDGE_CURVE('',#40432,#40434,#9174,.T.);
#51520=EDGE_CURVE('',#40431,#40433,#9175,.T.);
#51521=EDGE_CURVE('',#40434,#40429,#9176,.T.);
#51522=EDGE_CURVE('',#40433,#40430,#9177,.T.);
#51523=EDGE_CURVE('',#40435,#40436,#9178,.T.);
#51524=EDGE_CURVE('',#40437,#40436,#9179,.T.);
#51525=EDGE_CURVE('',#40438,#40437,#9180,.T.);
#51526=EDGE_CURVE('',#40438,#40435,#9181,.T.);
#51527=EDGE_CURVE('',#40439,#40440,#9182,.T.);
#51528=EDGE_CURVE('',#40436,#40440,#9183,.T.);
#51529=EDGE_CURVE('',#40435,#40439,#9184,.T.);
#51530=EDGE_CURVE('',#40441,#40442,#9185,.T.);
#51531=EDGE_CURVE('',#40440,#40442,#9186,.T.);
#51532=EDGE_CURVE('',#40439,#40441,#9187,.T.);
#51533=EDGE_CURVE('',#40442,#40437,#9188,.T.);
#51534=EDGE_CURVE('',#40441,#40438,#9189,.T.);
#51535=EDGE_CURVE('',#40443,#40444,#9190,.T.);
#51536=EDGE_CURVE('',#40445,#40444,#9191,.T.);
#51537=EDGE_CURVE('',#40446,#40445,#9192,.T.);
#51538=EDGE_CURVE('',#40446,#40443,#9193,.T.);
#51539=EDGE_CURVE('',#40447,#40448,#9194,.T.);
#51540=EDGE_CURVE('',#40444,#40448,#9195,.T.);
#51541=EDGE_CURVE('',#40443,#40447,#9196,.T.);
#51542=EDGE_CURVE('',#40449,#40450,#9197,.T.);
#51543=EDGE_CURVE('',#40448,#40450,#9198,.T.);
#51544=EDGE_CURVE('',#40447,#40449,#9199,.T.);
#51545=EDGE_CURVE('',#40450,#40445,#9200,.T.);
#51546=EDGE_CURVE('',#40449,#40446,#9201,.T.);
#51547=EDGE_CURVE('',#40451,#40452,#9202,.T.);
#51548=EDGE_CURVE('',#40453,#40452,#9203,.T.);
#51549=EDGE_CURVE('',#40454,#40453,#9204,.T.);
#51550=EDGE_CURVE('',#40454,#40451,#9205,.T.);
#51551=EDGE_CURVE('',#40455,#40456,#9206,.T.);
#51552=EDGE_CURVE('',#40452,#40456,#9207,.T.);
#51553=EDGE_CURVE('',#40451,#40455,#9208,.T.);
#51554=EDGE_CURVE('',#40457,#40458,#9209,.T.);
#51555=EDGE_CURVE('',#40456,#40458,#9210,.T.);
#51556=EDGE_CURVE('',#40455,#40457,#9211,.T.);
#51557=EDGE_CURVE('',#40458,#40453,#9212,.T.);
#51558=EDGE_CURVE('',#40457,#40454,#9213,.T.);
#51559=EDGE_CURVE('',#40459,#40460,#9214,.T.);
#51560=EDGE_CURVE('',#40461,#40460,#9215,.T.);
#51561=EDGE_CURVE('',#40462,#40461,#9216,.T.);
#51562=EDGE_CURVE('',#40462,#40459,#9217,.T.);
#51563=EDGE_CURVE('',#40463,#40464,#9218,.T.);
#51564=EDGE_CURVE('',#40460,#40464,#9219,.T.);
#51565=EDGE_CURVE('',#40459,#40463,#9220,.T.);
#51566=EDGE_CURVE('',#40465,#40466,#9221,.T.);
#51567=EDGE_CURVE('',#40464,#40466,#9222,.T.);
#51568=EDGE_CURVE('',#40463,#40465,#9223,.T.);
#51569=EDGE_CURVE('',#40466,#40461,#9224,.T.);
#51570=EDGE_CURVE('',#40465,#40462,#9225,.T.);
#51571=EDGE_CURVE('',#40467,#40468,#9226,.T.);
#51572=EDGE_CURVE('',#40469,#40468,#9227,.T.);
#51573=EDGE_CURVE('',#40470,#40469,#9228,.T.);
#51574=EDGE_CURVE('',#40470,#40467,#9229,.T.);
#51575=EDGE_CURVE('',#40471,#40472,#9230,.T.);
#51576=EDGE_CURVE('',#40468,#40472,#9231,.T.);
#51577=EDGE_CURVE('',#40467,#40471,#9232,.T.);
#51578=EDGE_CURVE('',#40473,#40474,#9233,.T.);
#51579=EDGE_CURVE('',#40472,#40474,#9234,.T.);
#51580=EDGE_CURVE('',#40471,#40473,#9235,.T.);
#51581=EDGE_CURVE('',#40474,#40469,#9236,.T.);
#51582=EDGE_CURVE('',#40473,#40470,#9237,.T.);
#51583=EDGE_CURVE('',#40475,#40476,#9238,.T.);
#51584=EDGE_CURVE('',#40477,#40476,#9239,.T.);
#51585=EDGE_CURVE('',#40478,#40477,#9240,.T.);
#51586=EDGE_CURVE('',#40478,#40475,#9241,.T.);
#51587=EDGE_CURVE('',#40479,#40480,#9242,.T.);
#51588=EDGE_CURVE('',#40476,#40480,#9243,.T.);
#51589=EDGE_CURVE('',#40475,#40479,#9244,.T.);
#51590=EDGE_CURVE('',#40481,#40482,#9245,.T.);
#51591=EDGE_CURVE('',#40480,#40482,#9246,.T.);
#51592=EDGE_CURVE('',#40479,#40481,#9247,.T.);
#51593=EDGE_CURVE('',#40482,#40477,#9248,.T.);
#51594=EDGE_CURVE('',#40481,#40478,#9249,.T.);
#51595=EDGE_CURVE('',#40483,#40484,#9250,.T.);
#51596=EDGE_CURVE('',#40485,#40484,#9251,.T.);
#51597=EDGE_CURVE('',#40486,#40485,#9252,.T.);
#51598=EDGE_CURVE('',#40486,#40483,#9253,.T.);
#51599=EDGE_CURVE('',#40487,#40488,#9254,.T.);
#51600=EDGE_CURVE('',#40484,#40488,#9255,.T.);
#51601=EDGE_CURVE('',#40483,#40487,#9256,.T.);
#51602=EDGE_CURVE('',#40489,#40490,#9257,.T.);
#51603=EDGE_CURVE('',#40488,#40490,#9258,.T.);
#51604=EDGE_CURVE('',#40487,#40489,#9259,.T.);
#51605=EDGE_CURVE('',#40490,#40485,#9260,.T.);
#51606=EDGE_CURVE('',#40489,#40486,#9261,.T.);
#51607=EDGE_CURVE('',#40491,#40492,#9262,.T.);
#51608=EDGE_CURVE('',#40493,#40492,#9263,.T.);
#51609=EDGE_CURVE('',#40494,#40493,#9264,.T.);
#51610=EDGE_CURVE('',#40494,#40491,#9265,.T.);
#51611=EDGE_CURVE('',#40495,#40496,#9266,.T.);
#51612=EDGE_CURVE('',#40492,#40496,#9267,.T.);
#51613=EDGE_CURVE('',#40491,#40495,#9268,.T.);
#51614=EDGE_CURVE('',#40497,#40498,#9269,.T.);
#51615=EDGE_CURVE('',#40496,#40498,#9270,.T.);
#51616=EDGE_CURVE('',#40495,#40497,#9271,.T.);
#51617=EDGE_CURVE('',#40498,#40493,#9272,.T.);
#51618=EDGE_CURVE('',#40497,#40494,#9273,.T.);
#51619=EDGE_CURVE('',#40499,#40500,#9274,.T.);
#51620=EDGE_CURVE('',#40501,#40500,#9275,.T.);
#51621=EDGE_CURVE('',#40502,#40501,#9276,.T.);
#51622=EDGE_CURVE('',#40502,#40499,#9277,.T.);
#51623=EDGE_CURVE('',#40503,#40504,#9278,.T.);
#51624=EDGE_CURVE('',#40500,#40504,#9279,.T.);
#51625=EDGE_CURVE('',#40499,#40503,#9280,.T.);
#51626=EDGE_CURVE('',#40505,#40506,#9281,.T.);
#51627=EDGE_CURVE('',#40504,#40506,#9282,.T.);
#51628=EDGE_CURVE('',#40503,#40505,#9283,.T.);
#51629=EDGE_CURVE('',#40506,#40501,#9284,.T.);
#51630=EDGE_CURVE('',#40505,#40502,#9285,.T.);
#51631=EDGE_CURVE('',#40507,#40508,#9286,.T.);
#51632=EDGE_CURVE('',#40509,#40508,#9287,.T.);
#51633=EDGE_CURVE('',#40510,#40509,#9288,.T.);
#51634=EDGE_CURVE('',#40510,#40507,#9289,.T.);
#51635=EDGE_CURVE('',#40511,#40512,#9290,.T.);
#51636=EDGE_CURVE('',#40508,#40512,#9291,.T.);
#51637=EDGE_CURVE('',#40507,#40511,#9292,.T.);
#51638=EDGE_CURVE('',#40513,#40514,#9293,.T.);
#51639=EDGE_CURVE('',#40512,#40514,#9294,.T.);
#51640=EDGE_CURVE('',#40511,#40513,#9295,.T.);
#51641=EDGE_CURVE('',#40514,#40509,#9296,.T.);
#51642=EDGE_CURVE('',#40513,#40510,#9297,.T.);
#51643=EDGE_CURVE('',#40515,#40516,#9298,.T.);
#51644=EDGE_CURVE('',#40517,#40516,#9299,.T.);
#51645=EDGE_CURVE('',#40518,#40517,#9300,.T.);
#51646=EDGE_CURVE('',#40518,#40515,#9301,.T.);
#51647=EDGE_CURVE('',#40519,#40520,#9302,.T.);
#51648=EDGE_CURVE('',#40516,#40520,#9303,.T.);
#51649=EDGE_CURVE('',#40515,#40519,#9304,.T.);
#51650=EDGE_CURVE('',#40521,#40522,#9305,.T.);
#51651=EDGE_CURVE('',#40520,#40522,#9306,.T.);
#51652=EDGE_CURVE('',#40519,#40521,#9307,.T.);
#51653=EDGE_CURVE('',#40522,#40517,#9308,.T.);
#51654=EDGE_CURVE('',#40521,#40518,#9309,.T.);
#51655=EDGE_CURVE('',#40523,#40524,#9310,.T.);
#51656=EDGE_CURVE('',#40525,#40524,#9311,.T.);
#51657=EDGE_CURVE('',#40526,#40525,#9312,.T.);
#51658=EDGE_CURVE('',#40526,#40523,#9313,.T.);
#51659=EDGE_CURVE('',#40527,#40528,#9314,.T.);
#51660=EDGE_CURVE('',#40524,#40528,#9315,.T.);
#51661=EDGE_CURVE('',#40523,#40527,#9316,.T.);
#51662=EDGE_CURVE('',#40529,#40530,#9317,.T.);
#51663=EDGE_CURVE('',#40528,#40530,#9318,.T.);
#51664=EDGE_CURVE('',#40527,#40529,#9319,.T.);
#51665=EDGE_CURVE('',#40530,#40525,#9320,.T.);
#51666=EDGE_CURVE('',#40529,#40526,#9321,.T.);
#51667=EDGE_CURVE('',#40531,#40532,#9322,.T.);
#51668=EDGE_CURVE('',#40533,#40532,#9323,.T.);
#51669=EDGE_CURVE('',#40534,#40533,#9324,.T.);
#51670=EDGE_CURVE('',#40534,#40531,#9325,.T.);
#51671=EDGE_CURVE('',#40535,#40536,#9326,.T.);
#51672=EDGE_CURVE('',#40532,#40536,#9327,.T.);
#51673=EDGE_CURVE('',#40531,#40535,#9328,.T.);
#51674=EDGE_CURVE('',#40537,#40538,#9329,.T.);
#51675=EDGE_CURVE('',#40536,#40538,#9330,.T.);
#51676=EDGE_CURVE('',#40535,#40537,#9331,.T.);
#51677=EDGE_CURVE('',#40538,#40533,#9332,.T.);
#51678=EDGE_CURVE('',#40537,#40534,#9333,.T.);
#51679=EDGE_CURVE('',#40539,#40540,#9334,.T.);
#51680=EDGE_CURVE('',#40541,#40540,#9335,.T.);
#51681=EDGE_CURVE('',#40542,#40541,#9336,.T.);
#51682=EDGE_CURVE('',#40542,#40539,#9337,.T.);
#51683=EDGE_CURVE('',#40543,#40544,#9338,.T.);
#51684=EDGE_CURVE('',#40540,#40544,#9339,.T.);
#51685=EDGE_CURVE('',#40539,#40543,#9340,.T.);
#51686=EDGE_CURVE('',#40545,#40546,#9341,.T.);
#51687=EDGE_CURVE('',#40544,#40546,#9342,.T.);
#51688=EDGE_CURVE('',#40543,#40545,#9343,.T.);
#51689=EDGE_CURVE('',#40546,#40541,#9344,.T.);
#51690=EDGE_CURVE('',#40545,#40542,#9345,.T.);
#51691=EDGE_CURVE('',#40547,#40548,#9346,.T.);
#51692=EDGE_CURVE('',#40549,#40548,#9347,.T.);
#51693=EDGE_CURVE('',#40550,#40549,#9348,.T.);
#51694=EDGE_CURVE('',#40550,#40547,#9349,.T.);
#51695=EDGE_CURVE('',#40551,#40552,#9350,.T.);
#51696=EDGE_CURVE('',#40548,#40552,#9351,.T.);
#51697=EDGE_CURVE('',#40547,#40551,#9352,.T.);
#51698=EDGE_CURVE('',#40553,#40554,#9353,.T.);
#51699=EDGE_CURVE('',#40552,#40554,#9354,.T.);
#51700=EDGE_CURVE('',#40551,#40553,#9355,.T.);
#51701=EDGE_CURVE('',#40554,#40549,#9356,.T.);
#51702=EDGE_CURVE('',#40553,#40550,#9357,.T.);
#51703=EDGE_CURVE('',#40555,#40556,#9358,.T.);
#51704=EDGE_CURVE('',#40557,#40556,#9359,.T.);
#51705=EDGE_CURVE('',#40558,#40557,#9360,.T.);
#51706=EDGE_CURVE('',#40558,#40555,#9361,.T.);
#51707=EDGE_CURVE('',#40559,#40560,#9362,.T.);
#51708=EDGE_CURVE('',#40556,#40560,#9363,.T.);
#51709=EDGE_CURVE('',#40555,#40559,#9364,.T.);
#51710=EDGE_CURVE('',#40561,#40562,#9365,.T.);
#51711=EDGE_CURVE('',#40560,#40562,#9366,.T.);
#51712=EDGE_CURVE('',#40559,#40561,#9367,.T.);
#51713=EDGE_CURVE('',#40562,#40557,#9368,.T.);
#51714=EDGE_CURVE('',#40561,#40558,#9369,.T.);
#51715=EDGE_CURVE('',#40563,#40564,#9370,.T.);
#51716=EDGE_CURVE('',#40565,#40564,#9371,.T.);
#51717=EDGE_CURVE('',#40566,#40565,#9372,.T.);
#51718=EDGE_CURVE('',#40566,#40563,#9373,.T.);
#51719=EDGE_CURVE('',#40567,#40568,#9374,.T.);
#51720=EDGE_CURVE('',#40564,#40568,#9375,.T.);
#51721=EDGE_CURVE('',#40563,#40567,#9376,.T.);
#51722=EDGE_CURVE('',#40569,#40570,#9377,.T.);
#51723=EDGE_CURVE('',#40568,#40570,#9378,.T.);
#51724=EDGE_CURVE('',#40567,#40569,#9379,.T.);
#51725=EDGE_CURVE('',#40570,#40565,#9380,.T.);
#51726=EDGE_CURVE('',#40569,#40566,#9381,.T.);
#51727=EDGE_CURVE('',#40571,#40572,#9382,.T.);
#51728=EDGE_CURVE('',#40573,#40572,#9383,.T.);
#51729=EDGE_CURVE('',#40574,#40573,#9384,.T.);
#51730=EDGE_CURVE('',#40574,#40571,#9385,.T.);
#51731=EDGE_CURVE('',#40575,#40576,#9386,.T.);
#51732=EDGE_CURVE('',#40572,#40576,#9387,.T.);
#51733=EDGE_CURVE('',#40571,#40575,#9388,.T.);
#51734=EDGE_CURVE('',#40577,#40578,#9389,.T.);
#51735=EDGE_CURVE('',#40576,#40578,#9390,.T.);
#51736=EDGE_CURVE('',#40575,#40577,#9391,.T.);
#51737=EDGE_CURVE('',#40578,#40573,#9392,.T.);
#51738=EDGE_CURVE('',#40577,#40574,#9393,.T.);
#51739=EDGE_CURVE('',#40579,#40580,#9394,.T.);
#51740=EDGE_CURVE('',#40581,#40580,#9395,.T.);
#51741=EDGE_CURVE('',#40582,#40581,#9396,.T.);
#51742=EDGE_CURVE('',#40582,#40579,#9397,.T.);
#51743=EDGE_CURVE('',#40583,#40584,#9398,.T.);
#51744=EDGE_CURVE('',#40580,#40584,#9399,.T.);
#51745=EDGE_CURVE('',#40579,#40583,#9400,.T.);
#51746=EDGE_CURVE('',#40585,#40586,#9401,.T.);
#51747=EDGE_CURVE('',#40584,#40586,#9402,.T.);
#51748=EDGE_CURVE('',#40583,#40585,#9403,.T.);
#51749=EDGE_CURVE('',#40586,#40581,#9404,.T.);
#51750=EDGE_CURVE('',#40585,#40582,#9405,.T.);
#51751=EDGE_CURVE('',#40587,#40588,#9406,.T.);
#51752=EDGE_CURVE('',#40589,#40588,#9407,.T.);
#51753=EDGE_CURVE('',#40590,#40589,#9408,.T.);
#51754=EDGE_CURVE('',#40590,#40587,#9409,.T.);
#51755=EDGE_CURVE('',#40591,#40592,#9410,.T.);
#51756=EDGE_CURVE('',#40588,#40592,#9411,.T.);
#51757=EDGE_CURVE('',#40587,#40591,#9412,.T.);
#51758=EDGE_CURVE('',#40593,#40594,#9413,.T.);
#51759=EDGE_CURVE('',#40592,#40594,#9414,.T.);
#51760=EDGE_CURVE('',#40591,#40593,#9415,.T.);
#51761=EDGE_CURVE('',#40594,#40589,#9416,.T.);
#51762=EDGE_CURVE('',#40593,#40590,#9417,.T.);
#51763=EDGE_CURVE('',#40595,#40596,#9418,.T.);
#51764=EDGE_CURVE('',#40597,#40596,#9419,.T.);
#51765=EDGE_CURVE('',#40598,#40597,#9420,.T.);
#51766=EDGE_CURVE('',#40598,#40595,#9421,.T.);
#51767=EDGE_CURVE('',#40599,#40600,#9422,.T.);
#51768=EDGE_CURVE('',#40596,#40600,#9423,.T.);
#51769=EDGE_CURVE('',#40595,#40599,#9424,.T.);
#51770=EDGE_CURVE('',#40601,#40602,#9425,.T.);
#51771=EDGE_CURVE('',#40600,#40602,#9426,.T.);
#51772=EDGE_CURVE('',#40599,#40601,#9427,.T.);
#51773=EDGE_CURVE('',#40602,#40597,#9428,.T.);
#51774=EDGE_CURVE('',#40601,#40598,#9429,.T.);
#51775=EDGE_CURVE('',#40603,#40604,#9430,.T.);
#51776=EDGE_CURVE('',#40605,#40604,#9431,.T.);
#51777=EDGE_CURVE('',#40606,#40605,#9432,.T.);
#51778=EDGE_CURVE('',#40606,#40603,#9433,.T.);
#51779=EDGE_CURVE('',#40607,#40608,#9434,.T.);
#51780=EDGE_CURVE('',#40604,#40608,#9435,.T.);
#51781=EDGE_CURVE('',#40603,#40607,#9436,.T.);
#51782=EDGE_CURVE('',#40609,#40610,#9437,.T.);
#51783=EDGE_CURVE('',#40608,#40610,#9438,.T.);
#51784=EDGE_CURVE('',#40607,#40609,#9439,.T.);
#51785=EDGE_CURVE('',#40610,#40605,#9440,.T.);
#51786=EDGE_CURVE('',#40609,#40606,#9441,.T.);
#51787=EDGE_CURVE('',#40611,#40612,#9442,.T.);
#51788=EDGE_CURVE('',#40613,#40612,#9443,.T.);
#51789=EDGE_CURVE('',#40614,#40613,#9444,.T.);
#51790=EDGE_CURVE('',#40614,#40611,#9445,.T.);
#51791=EDGE_CURVE('',#40615,#40616,#9446,.T.);
#51792=EDGE_CURVE('',#40612,#40616,#9447,.T.);
#51793=EDGE_CURVE('',#40611,#40615,#9448,.T.);
#51794=EDGE_CURVE('',#40617,#40618,#9449,.T.);
#51795=EDGE_CURVE('',#40616,#40618,#9450,.T.);
#51796=EDGE_CURVE('',#40615,#40617,#9451,.T.);
#51797=EDGE_CURVE('',#40618,#40613,#9452,.T.);
#51798=EDGE_CURVE('',#40617,#40614,#9453,.T.);
#51799=EDGE_CURVE('',#40619,#40620,#9454,.T.);
#51800=EDGE_CURVE('',#40621,#40620,#9455,.T.);
#51801=EDGE_CURVE('',#40622,#40621,#9456,.T.);
#51802=EDGE_CURVE('',#40622,#40619,#9457,.T.);
#51803=EDGE_CURVE('',#40623,#40624,#9458,.T.);
#51804=EDGE_CURVE('',#40620,#40624,#9459,.T.);
#51805=EDGE_CURVE('',#40619,#40623,#9460,.T.);
#51806=EDGE_CURVE('',#40625,#40626,#9461,.T.);
#51807=EDGE_CURVE('',#40624,#40626,#9462,.T.);
#51808=EDGE_CURVE('',#40623,#40625,#9463,.T.);
#51809=EDGE_CURVE('',#40626,#40621,#9464,.T.);
#51810=EDGE_CURVE('',#40625,#40622,#9465,.T.);
#51811=EDGE_CURVE('',#40627,#40628,#9466,.T.);
#51812=EDGE_CURVE('',#40629,#40628,#9467,.T.);
#51813=EDGE_CURVE('',#40630,#40629,#9468,.T.);
#51814=EDGE_CURVE('',#40630,#40627,#9469,.T.);
#51815=EDGE_CURVE('',#40631,#40632,#9470,.T.);
#51816=EDGE_CURVE('',#40628,#40632,#9471,.T.);
#51817=EDGE_CURVE('',#40627,#40631,#9472,.T.);
#51818=EDGE_CURVE('',#40633,#40634,#9473,.T.);
#51819=EDGE_CURVE('',#40632,#40634,#9474,.T.);
#51820=EDGE_CURVE('',#40631,#40633,#9475,.T.);
#51821=EDGE_CURVE('',#40634,#40629,#9476,.T.);
#51822=EDGE_CURVE('',#40633,#40630,#9477,.T.);
#51823=EDGE_CURVE('',#40635,#40636,#9478,.T.);
#51824=EDGE_CURVE('',#40637,#40636,#9479,.T.);
#51825=EDGE_CURVE('',#40638,#40637,#9480,.T.);
#51826=EDGE_CURVE('',#40638,#40635,#9481,.T.);
#51827=EDGE_CURVE('',#40639,#40640,#9482,.T.);
#51828=EDGE_CURVE('',#40636,#40640,#9483,.T.);
#51829=EDGE_CURVE('',#40635,#40639,#9484,.T.);
#51830=EDGE_CURVE('',#40641,#40642,#9485,.T.);
#51831=EDGE_CURVE('',#40640,#40642,#9486,.T.);
#51832=EDGE_CURVE('',#40639,#40641,#9487,.T.);
#51833=EDGE_CURVE('',#40642,#40637,#9488,.T.);
#51834=EDGE_CURVE('',#40641,#40638,#9489,.T.);
#51835=EDGE_CURVE('',#40643,#40644,#9490,.T.);
#51836=EDGE_CURVE('',#40645,#40644,#9491,.T.);
#51837=EDGE_CURVE('',#40646,#40645,#9492,.T.);
#51838=EDGE_CURVE('',#40646,#40643,#9493,.T.);
#51839=EDGE_CURVE('',#40647,#40648,#9494,.T.);
#51840=EDGE_CURVE('',#40644,#40648,#9495,.T.);
#51841=EDGE_CURVE('',#40643,#40647,#9496,.T.);
#51842=EDGE_CURVE('',#40649,#40650,#9497,.T.);
#51843=EDGE_CURVE('',#40648,#40650,#9498,.T.);
#51844=EDGE_CURVE('',#40647,#40649,#9499,.T.);
#51845=EDGE_CURVE('',#40650,#40645,#9500,.T.);
#51846=EDGE_CURVE('',#40649,#40646,#9501,.T.);
#51847=EDGE_CURVE('',#40651,#40652,#9502,.T.);
#51848=EDGE_CURVE('',#40653,#40652,#9503,.T.);
#51849=EDGE_CURVE('',#40654,#40653,#9504,.T.);
#51850=EDGE_CURVE('',#40654,#40651,#9505,.T.);
#51851=EDGE_CURVE('',#40655,#40656,#9506,.T.);
#51852=EDGE_CURVE('',#40652,#40656,#9507,.T.);
#51853=EDGE_CURVE('',#40651,#40655,#9508,.T.);
#51854=EDGE_CURVE('',#40657,#40658,#9509,.T.);
#51855=EDGE_CURVE('',#40656,#40658,#9510,.T.);
#51856=EDGE_CURVE('',#40655,#40657,#9511,.T.);
#51857=EDGE_CURVE('',#40658,#40653,#9512,.T.);
#51858=EDGE_CURVE('',#40657,#40654,#9513,.T.);
#51859=EDGE_CURVE('',#40659,#40660,#9514,.T.);
#51860=EDGE_CURVE('',#40661,#40660,#9515,.T.);
#51861=EDGE_CURVE('',#40662,#40661,#9516,.T.);
#51862=EDGE_CURVE('',#40662,#40659,#9517,.T.);
#51863=EDGE_CURVE('',#40663,#40664,#9518,.T.);
#51864=EDGE_CURVE('',#40660,#40664,#9519,.T.);
#51865=EDGE_CURVE('',#40659,#40663,#9520,.T.);
#51866=EDGE_CURVE('',#40665,#40666,#9521,.T.);
#51867=EDGE_CURVE('',#40664,#40666,#9522,.T.);
#51868=EDGE_CURVE('',#40663,#40665,#9523,.T.);
#51869=EDGE_CURVE('',#40666,#40661,#9524,.T.);
#51870=EDGE_CURVE('',#40665,#40662,#9525,.T.);
#51871=EDGE_CURVE('',#40667,#40668,#9526,.T.);
#51872=EDGE_CURVE('',#40669,#40668,#9527,.T.);
#51873=EDGE_CURVE('',#40670,#40669,#9528,.T.);
#51874=EDGE_CURVE('',#40670,#40667,#9529,.T.);
#51875=EDGE_CURVE('',#40671,#40672,#9530,.T.);
#51876=EDGE_CURVE('',#40668,#40672,#9531,.T.);
#51877=EDGE_CURVE('',#40667,#40671,#9532,.T.);
#51878=EDGE_CURVE('',#40673,#40674,#9533,.T.);
#51879=EDGE_CURVE('',#40672,#40674,#9534,.T.);
#51880=EDGE_CURVE('',#40671,#40673,#9535,.T.);
#51881=EDGE_CURVE('',#40674,#40669,#9536,.T.);
#51882=EDGE_CURVE('',#40673,#40670,#9537,.T.);
#51883=EDGE_CURVE('',#40675,#40676,#9538,.T.);
#51884=EDGE_CURVE('',#40677,#40676,#9539,.T.);
#51885=EDGE_CURVE('',#40678,#40677,#9540,.T.);
#51886=EDGE_CURVE('',#40678,#40675,#9541,.T.);
#51887=EDGE_CURVE('',#40679,#40680,#9542,.T.);
#51888=EDGE_CURVE('',#40676,#40680,#9543,.T.);
#51889=EDGE_CURVE('',#40675,#40679,#9544,.T.);
#51890=EDGE_CURVE('',#40681,#40682,#9545,.T.);
#51891=EDGE_CURVE('',#40680,#40682,#9546,.T.);
#51892=EDGE_CURVE('',#40679,#40681,#9547,.T.);
#51893=EDGE_CURVE('',#40682,#40677,#9548,.T.);
#51894=EDGE_CURVE('',#40681,#40678,#9549,.T.);
#51895=EDGE_CURVE('',#40683,#40684,#9550,.T.);
#51896=EDGE_CURVE('',#40685,#40684,#9551,.T.);
#51897=EDGE_CURVE('',#40686,#40685,#9552,.T.);
#51898=EDGE_CURVE('',#40686,#40683,#9553,.T.);
#51899=EDGE_CURVE('',#40687,#40688,#9554,.T.);
#51900=EDGE_CURVE('',#40684,#40688,#9555,.T.);
#51901=EDGE_CURVE('',#40683,#40687,#9556,.T.);
#51902=EDGE_CURVE('',#40689,#40690,#9557,.T.);
#51903=EDGE_CURVE('',#40688,#40690,#9558,.T.);
#51904=EDGE_CURVE('',#40687,#40689,#9559,.T.);
#51905=EDGE_CURVE('',#40690,#40685,#9560,.T.);
#51906=EDGE_CURVE('',#40689,#40686,#9561,.T.);
#51907=EDGE_CURVE('',#40691,#40692,#9562,.T.);
#51908=EDGE_CURVE('',#40693,#40692,#9563,.T.);
#51909=EDGE_CURVE('',#40694,#40693,#9564,.T.);
#51910=EDGE_CURVE('',#40694,#40691,#9565,.T.);
#51911=EDGE_CURVE('',#40695,#40696,#9566,.T.);
#51912=EDGE_CURVE('',#40692,#40696,#9567,.T.);
#51913=EDGE_CURVE('',#40691,#40695,#9568,.T.);
#51914=EDGE_CURVE('',#40697,#40698,#9569,.T.);
#51915=EDGE_CURVE('',#40696,#40698,#9570,.T.);
#51916=EDGE_CURVE('',#40695,#40697,#9571,.T.);
#51917=EDGE_CURVE('',#40698,#40693,#9572,.T.);
#51918=EDGE_CURVE('',#40697,#40694,#9573,.T.);
#51919=EDGE_CURVE('',#40699,#40700,#9574,.T.);
#51920=EDGE_CURVE('',#40701,#40700,#9575,.T.);
#51921=EDGE_CURVE('',#40702,#40701,#9576,.T.);
#51922=EDGE_CURVE('',#40702,#40699,#9577,.T.);
#51923=EDGE_CURVE('',#40703,#40704,#9578,.T.);
#51924=EDGE_CURVE('',#40700,#40704,#9579,.T.);
#51925=EDGE_CURVE('',#40699,#40703,#9580,.T.);
#51926=EDGE_CURVE('',#40705,#40706,#9581,.T.);
#51927=EDGE_CURVE('',#40704,#40706,#9582,.T.);
#51928=EDGE_CURVE('',#40703,#40705,#9583,.T.);
#51929=EDGE_CURVE('',#40706,#40701,#9584,.T.);
#51930=EDGE_CURVE('',#40705,#40702,#9585,.T.);
#51931=EDGE_CURVE('',#40707,#40708,#9586,.T.);
#51932=EDGE_CURVE('',#40709,#40708,#9587,.T.);
#51933=EDGE_CURVE('',#40710,#40709,#9588,.T.);
#51934=EDGE_CURVE('',#40710,#40707,#9589,.T.);
#51935=EDGE_CURVE('',#40711,#40712,#9590,.T.);
#51936=EDGE_CURVE('',#40708,#40712,#9591,.T.);
#51937=EDGE_CURVE('',#40707,#40711,#9592,.T.);
#51938=EDGE_CURVE('',#40713,#40714,#9593,.T.);
#51939=EDGE_CURVE('',#40712,#40714,#9594,.T.);
#51940=EDGE_CURVE('',#40711,#40713,#9595,.T.);
#51941=EDGE_CURVE('',#40714,#40709,#9596,.T.);
#51942=EDGE_CURVE('',#40713,#40710,#9597,.T.);
#51943=EDGE_CURVE('',#40715,#40716,#9598,.T.);
#51944=EDGE_CURVE('',#40717,#40716,#9599,.T.);
#51945=EDGE_CURVE('',#40718,#40717,#9600,.T.);
#51946=EDGE_CURVE('',#40718,#40715,#9601,.T.);
#51947=EDGE_CURVE('',#40719,#40720,#9602,.T.);
#51948=EDGE_CURVE('',#40716,#40720,#9603,.T.);
#51949=EDGE_CURVE('',#40715,#40719,#9604,.T.);
#51950=EDGE_CURVE('',#40721,#40722,#9605,.T.);
#51951=EDGE_CURVE('',#40720,#40722,#9606,.T.);
#51952=EDGE_CURVE('',#40719,#40721,#9607,.T.);
#51953=EDGE_CURVE('',#40722,#40717,#9608,.T.);
#51954=EDGE_CURVE('',#40721,#40718,#9609,.T.);
#51955=EDGE_CURVE('',#40723,#40724,#9610,.T.);
#51956=EDGE_CURVE('',#40725,#40724,#9611,.T.);
#51957=EDGE_CURVE('',#40726,#40725,#9612,.T.);
#51958=EDGE_CURVE('',#40726,#40723,#9613,.T.);
#51959=EDGE_CURVE('',#40727,#40728,#9614,.T.);
#51960=EDGE_CURVE('',#40724,#40728,#9615,.T.);
#51961=EDGE_CURVE('',#40723,#40727,#9616,.T.);
#51962=EDGE_CURVE('',#40729,#40730,#9617,.T.);
#51963=EDGE_CURVE('',#40728,#40730,#9618,.T.);
#51964=EDGE_CURVE('',#40727,#40729,#9619,.T.);
#51965=EDGE_CURVE('',#40730,#40725,#9620,.T.);
#51966=EDGE_CURVE('',#40729,#40726,#9621,.T.);
#51967=EDGE_CURVE('',#40731,#40732,#9622,.T.);
#51968=EDGE_CURVE('',#40732,#40733,#9623,.T.);
#51969=EDGE_CURVE('',#40733,#40734,#9624,.T.);
#51970=EDGE_CURVE('',#40734,#40731,#9625,.T.);
#51971=EDGE_CURVE('',#40735,#40732,#9626,.T.);
#51972=EDGE_CURVE('',#40736,#40731,#9627,.T.);
#51973=EDGE_CURVE('',#40736,#40735,#9628,.T.);
#51974=EDGE_CURVE('',#40737,#40733,#9629,.T.);
#51975=EDGE_CURVE('',#40735,#40737,#9630,.T.);
#51976=EDGE_CURVE('',#40738,#40734,#9631,.T.);
#51977=EDGE_CURVE('',#40737,#40738,#9632,.T.);
#51978=EDGE_CURVE('',#40738,#40736,#9633,.T.);
#51979=EDGE_CURVE('',#35058,#35080,#9634,.T.);
#51980=EDGE_CURVE('',#35077,#35064,#9635,.T.);
#51981=EDGE_CURVE('',#35060,#35079,#9636,.T.);
#51982=EDGE_CURVE('',#35078,#35061,#9637,.T.);
#51983=EDGE_CURVE('',#35082,#35066,#9638,.T.);
#51984=EDGE_CURVE('',#35053,#35074,#9639,.T.);
#51985=EDGE_CURVE('',#35081,#35065,#9640,.T.);
#51986=EDGE_CURVE('',#35054,#35073,#9641,.T.);
#51987=EDGE_CURVE('',#40739,#40739,#33514,.T.);
#51988=EDGE_CURVE('',#40740,#40741,#33515,.T.);
#51989=EDGE_CURVE('',#40742,#40740,#33516,.T.);
#51990=EDGE_CURVE('',#40743,#40742,#33517,.T.);
#51991=EDGE_CURVE('',#40741,#40743,#33518,.T.);
#51992=EDGE_CURVE('',#40740,#40744,#9642,.T.);
#51993=EDGE_CURVE('',#40741,#40745,#9643,.T.);
#51994=EDGE_CURVE('',#40744,#40745,#33519,.T.);
#51995=EDGE_CURVE('',#40742,#40746,#9644,.T.);
#51996=EDGE_CURVE('',#40746,#40744,#33520,.T.);
#51997=EDGE_CURVE('',#40743,#40747,#9645,.T.);
#51998=EDGE_CURVE('',#40747,#40746,#33521,.T.);
#51999=EDGE_CURVE('',#40745,#40747,#33522,.T.);
#52000=EDGE_CURVE('',#40748,#40748,#33523,.T.);
#57171=ORIENTED_EDGE('',*,*,#43418,.F.);
#57172=ORIENTED_EDGE('',*,*,#43419,.T.);
#57173=ORIENTED_EDGE('',*,*,#43420,.T.);
#57174=ORIENTED_EDGE('',*,*,#43421,.F.);
#57175=ORIENTED_EDGE('',*,*,#43422,.F.);
#57176=ORIENTED_EDGE('',*,*,#43418,.T.);
#57177=ORIENTED_EDGE('',*,*,#43423,.T.);
#57178=ORIENTED_EDGE('',*,*,#43424,.F.);
#57179=ORIENTED_EDGE('',*,*,#43425,.F.);
#57180=ORIENTED_EDGE('',*,*,#43426,.F.);
#57181=ORIENTED_EDGE('',*,*,#43421,.T.);
#57182=ORIENTED_EDGE('',*,*,#43427,.T.);
#57183=ORIENTED_EDGE('',*,*,#43428,.F.);
#57184=ORIENTED_EDGE('',*,*,#43429,.F.);
#57185=ORIENTED_EDGE('',*,*,#43430,.F.);
#57186=ORIENTED_EDGE('',*,*,#43425,.T.);
#57187=ORIENTED_EDGE('',*,*,#43431,.T.);
#57188=ORIENTED_EDGE('',*,*,#43432,.T.);
#57189=ORIENTED_EDGE('',*,*,#43433,.T.);
#57190=ORIENTED_EDGE('',*,*,#43434,.T.);
#57191=ORIENTED_EDGE('',*,*,#43433,.F.);
#57192=ORIENTED_EDGE('',*,*,#43435,.T.);
#57193=ORIENTED_EDGE('',*,*,#43432,.F.);
#57194=ORIENTED_EDGE('',*,*,#43436,.T.);
#57195=ORIENTED_EDGE('',*,*,#43437,.F.);
#57196=ORIENTED_EDGE('',*,*,#43436,.F.);
#57197=ORIENTED_EDGE('',*,*,#43435,.F.);
#57198=ORIENTED_EDGE('',*,*,#43437,.T.);
#57199=ORIENTED_EDGE('',*,*,#43438,.T.);
#57200=ORIENTED_EDGE('',*,*,#43439,.F.);
#57201=ORIENTED_EDGE('',*,*,#43438,.F.);
#57202=ORIENTED_EDGE('',*,*,#43440,.F.);
#57203=ORIENTED_EDGE('',*,*,#43441,.T.);
#57204=ORIENTED_EDGE('',*,*,#43442,.F.);
#57205=ORIENTED_EDGE('',*,*,#43443,.F.);
#57206=ORIENTED_EDGE('',*,*,#43444,.F.);
#57207=ORIENTED_EDGE('',*,*,#43445,.T.);
#57208=ORIENTED_EDGE('',*,*,#43446,.F.);
#57209=ORIENTED_EDGE('',*,*,#43447,.F.);
#57210=ORIENTED_EDGE('',*,*,#43439,.T.);
#57211=ORIENTED_EDGE('',*,*,#43448,.T.);
#57212=ORIENTED_EDGE('',*,*,#43449,.T.);
#57213=ORIENTED_EDGE('',*,*,#43450,.T.);
#57214=ORIENTED_EDGE('',*,*,#43451,.F.);
#57215=ORIENTED_EDGE('',*,*,#43452,.T.);
#57216=ORIENTED_EDGE('',*,*,#43453,.F.);
#57217=ORIENTED_EDGE('',*,*,#43452,.F.);
#57218=ORIENTED_EDGE('',*,*,#43454,.F.);
#57219=ORIENTED_EDGE('',*,*,#43440,.T.);
#57220=ORIENTED_EDGE('',*,*,#43455,.T.);
#57221=ORIENTED_EDGE('',*,*,#43448,.F.);
#57222=ORIENTED_EDGE('',*,*,#43456,.F.);
#57223=ORIENTED_EDGE('',*,*,#43457,.T.);
#57224=ORIENTED_EDGE('',*,*,#43458,.T.);
#57225=ORIENTED_EDGE('',*,*,#43459,.T.);
#57226=ORIENTED_EDGE('',*,*,#43460,.T.);
#57227=ORIENTED_EDGE('',*,*,#43461,.T.);
#57228=ORIENTED_EDGE('',*,*,#43462,.F.);
#57229=ORIENTED_EDGE('',*,*,#43463,.T.);
#57230=ORIENTED_EDGE('',*,*,#43464,.F.);
#57231=ORIENTED_EDGE('',*,*,#43465,.T.);
#57232=ORIENTED_EDGE('',*,*,#43466,.T.);
#57233=ORIENTED_EDGE('',*,*,#43446,.T.);
#57234=ORIENTED_EDGE('',*,*,#43467,.F.);
#57235=ORIENTED_EDGE('',*,*,#43468,.T.);
#57236=ORIENTED_EDGE('',*,*,#43461,.F.);
#57237=ORIENTED_EDGE('',*,*,#43469,.F.);
#57238=ORIENTED_EDGE('',*,*,#43457,.F.);
#57239=ORIENTED_EDGE('',*,*,#43470,.T.);
#57240=ORIENTED_EDGE('',*,*,#43471,.F.);
#57241=ORIENTED_EDGE('',*,*,#43472,.F.);
#57242=ORIENTED_EDGE('',*,*,#43473,.T.);
#57243=ORIENTED_EDGE('',*,*,#43474,.T.);
#57244=ORIENTED_EDGE('',*,*,#43475,.T.);
#57245=ORIENTED_EDGE('',*,*,#43476,.T.);
#57246=ORIENTED_EDGE('',*,*,#43477,.F.);
#57247=ORIENTED_EDGE('',*,*,#43478,.T.);
#57248=ORIENTED_EDGE('',*,*,#43479,.F.);
#57249=ORIENTED_EDGE('',*,*,#43478,.F.);
#57250=ORIENTED_EDGE('',*,*,#43480,.F.);
#57251=ORIENTED_EDGE('',*,*,#43442,.T.);
#57252=ORIENTED_EDGE('',*,*,#43481,.T.);
#57253=ORIENTED_EDGE('',*,*,#43474,.F.);
#57254=ORIENTED_EDGE('',*,*,#43482,.T.);
#57255=ORIENTED_EDGE('',*,*,#43467,.T.);
#57256=ORIENTED_EDGE('',*,*,#43483,.F.);
#57257=ORIENTED_EDGE('',*,*,#43484,.T.);
#57258=ORIENTED_EDGE('',*,*,#43485,.F.);
#57259=ORIENTED_EDGE('',*,*,#43471,.T.);
#57260=ORIENTED_EDGE('',*,*,#43486,.T.);
#57261=ORIENTED_EDGE('',*,*,#43487,.T.);
#57262=ORIENTED_EDGE('',*,*,#43488,.T.);
#57263=ORIENTED_EDGE('',*,*,#43444,.T.);
#57264=ORIENTED_EDGE('',*,*,#43489,.F.);
#57265=ORIENTED_EDGE('',*,*,#43490,.T.);
#57266=ORIENTED_EDGE('',*,*,#43491,.T.);
#57267=ORIENTED_EDGE('',*,*,#43492,.T.);
#57268=ORIENTED_EDGE('',*,*,#43473,.F.);
#57269=ORIENTED_EDGE('',*,*,#43492,.F.);
#57270=ORIENTED_EDGE('',*,*,#43493,.T.);
#57271=ORIENTED_EDGE('',*,*,#43494,.T.);
#57272=ORIENTED_EDGE('',*,*,#43495,.F.);
#57273=ORIENTED_EDGE('',*,*,#43494,.F.);
#57274=ORIENTED_EDGE('',*,*,#43496,.T.);
#57275=ORIENTED_EDGE('',*,*,#43497,.T.);
#57276=ORIENTED_EDGE('',*,*,#43498,.F.);
#57277=ORIENTED_EDGE('',*,*,#43497,.F.);
#57278=ORIENTED_EDGE('',*,*,#43479,.T.);
#57279=ORIENTED_EDGE('',*,*,#43499,.T.);
#57280=ORIENTED_EDGE('',*,*,#43500,.F.);
#57281=ORIENTED_EDGE('',*,*,#43499,.F.);
#57282=ORIENTED_EDGE('',*,*,#43500,.T.);
#57283=ORIENTED_EDGE('',*,*,#43501,.T.);
#57284=ORIENTED_EDGE('',*,*,#43502,.F.);
#57285=ORIENTED_EDGE('',*,*,#43503,.F.);
#57286=ORIENTED_EDGE('',*,*,#43501,.F.);
#57287=ORIENTED_EDGE('',*,*,#43504,.T.);
#57288=ORIENTED_EDGE('',*,*,#43505,.T.);
#57289=ORIENTED_EDGE('',*,*,#43502,.T.);
#57290=ORIENTED_EDGE('',*,*,#43503,.T.);
#57291=ORIENTED_EDGE('',*,*,#43505,.F.);
#57292=ORIENTED_EDGE('',*,*,#43506,.T.);
#57293=ORIENTED_EDGE('',*,*,#43507,.T.);
#57294=ORIENTED_EDGE('',*,*,#43508,.F.);
#57295=ORIENTED_EDGE('',*,*,#43507,.F.);
#57296=ORIENTED_EDGE('',*,*,#43509,.T.);
#57297=ORIENTED_EDGE('',*,*,#43510,.T.);
#57298=ORIENTED_EDGE('',*,*,#43511,.F.);
#57299=ORIENTED_EDGE('',*,*,#43510,.F.);
#57300=ORIENTED_EDGE('',*,*,#43512,.T.);
#57301=ORIENTED_EDGE('',*,*,#43513,.T.);
#57302=ORIENTED_EDGE('',*,*,#43514,.F.);
#57303=ORIENTED_EDGE('',*,*,#43513,.F.);
#57304=ORIENTED_EDGE('',*,*,#43515,.T.);
#57305=ORIENTED_EDGE('',*,*,#43516,.F.);
#57306=ORIENTED_EDGE('',*,*,#43517,.F.);
#57307=ORIENTED_EDGE('',*,*,#43518,.T.);
#57308=ORIENTED_EDGE('',*,*,#43519,.T.);
#57309=ORIENTED_EDGE('',*,*,#43520,.T.);
#57310=ORIENTED_EDGE('',*,*,#43521,.F.);
#57311=ORIENTED_EDGE('',*,*,#43522,.T.);
#57312=ORIENTED_EDGE('',*,*,#43523,.F.);
#57313=ORIENTED_EDGE('',*,*,#43522,.F.);
#57314=ORIENTED_EDGE('',*,*,#43524,.F.);
#57315=ORIENTED_EDGE('',*,*,#43525,.F.);
#57316=ORIENTED_EDGE('',*,*,#43526,.F.);
#57317=ORIENTED_EDGE('',*,*,#43527,.F.);
#57318=ORIENTED_EDGE('',*,*,#43528,.T.);
#57319=ORIENTED_EDGE('',*,*,#43529,.T.);
#57320=ORIENTED_EDGE('',*,*,#43423,.F.);
#57321=ORIENTED_EDGE('',*,*,#43420,.F.);
#57322=ORIENTED_EDGE('',*,*,#43530,.T.);
#57323=ORIENTED_EDGE('',*,*,#43531,.T.);
#57324=ORIENTED_EDGE('',*,*,#43532,.F.);
#57325=ORIENTED_EDGE('',*,*,#43531,.F.);
#57326=ORIENTED_EDGE('',*,*,#43533,.T.);
#57327=ORIENTED_EDGE('',*,*,#43534,.F.);
#57328=ORIENTED_EDGE('',*,*,#43535,.F.);
#57329=ORIENTED_EDGE('',*,*,#43536,.F.);
#57330=ORIENTED_EDGE('',*,*,#43431,.F.);
#57331=ORIENTED_EDGE('',*,*,#43427,.F.);
#57332=ORIENTED_EDGE('',*,*,#43537,.F.);
#57333=ORIENTED_EDGE('',*,*,#43538,.T.);
#57334=ORIENTED_EDGE('',*,*,#43539,.F.);
#57335=ORIENTED_EDGE('',*,*,#43540,.F.);
#57336=ORIENTED_EDGE('',*,*,#43541,.T.);
#57337=ORIENTED_EDGE('',*,*,#43542,.T.);
#57338=ORIENTED_EDGE('',*,*,#43543,.T.);
#57339=ORIENTED_EDGE('',*,*,#43544,.F.);
#57340=ORIENTED_EDGE('',*,*,#43545,.F.);
#57341=ORIENTED_EDGE('',*,*,#43533,.F.);
#57342=ORIENTED_EDGE('',*,*,#43538,.F.);
#57343=ORIENTED_EDGE('',*,*,#43546,.F.);
#57344=ORIENTED_EDGE('',*,*,#43518,.F.);
#57345=ORIENTED_EDGE('',*,*,#43547,.F.);
#57346=ORIENTED_EDGE('',*,*,#43516,.T.);
#57347=ORIENTED_EDGE('',*,*,#43548,.F.);
#57348=ORIENTED_EDGE('',*,*,#43549,.T.);
#57349=ORIENTED_EDGE('',*,*,#43550,.T.);
#57350=ORIENTED_EDGE('',*,*,#43519,.F.);
#57351=ORIENTED_EDGE('',*,*,#43546,.T.);
#57352=ORIENTED_EDGE('',*,*,#43551,.F.);
#57353=ORIENTED_EDGE('',*,*,#43552,.T.);
#57354=ORIENTED_EDGE('',*,*,#43553,.F.);
#57355=ORIENTED_EDGE('',*,*,#43548,.T.);
#57356=ORIENTED_EDGE('',*,*,#43515,.F.);
#57357=ORIENTED_EDGE('',*,*,#43552,.F.);
#57358=ORIENTED_EDGE('',*,*,#43525,.T.);
#57359=ORIENTED_EDGE('',*,*,#43554,.F.);
#57360=ORIENTED_EDGE('',*,*,#43520,.F.);
#57361=ORIENTED_EDGE('',*,*,#43550,.F.);
#57362=ORIENTED_EDGE('',*,*,#43555,.T.);
#57363=ORIENTED_EDGE('',*,*,#43547,.T.);
#57364=ORIENTED_EDGE('',*,*,#43517,.T.);
#57365=ORIENTED_EDGE('',*,*,#43554,.T.);
#57366=ORIENTED_EDGE('',*,*,#43524,.T.);
#57367=ORIENTED_EDGE('',*,*,#43521,.T.);
#57368=ORIENTED_EDGE('',*,*,#43523,.T.);
#57369=ORIENTED_EDGE('',*,*,#43512,.F.);
#57370=ORIENTED_EDGE('',*,*,#43535,.T.);
#57371=ORIENTED_EDGE('',*,*,#43534,.T.);
#57372=ORIENTED_EDGE('',*,*,#43545,.T.);
#57373=ORIENTED_EDGE('',*,*,#43544,.T.);
#57374=ORIENTED_EDGE('',*,*,#43556,.T.);
#57375=ORIENTED_EDGE('',*,*,#43557,.T.);
#57376=ORIENTED_EDGE('',*,*,#43429,.T.);
#57377=ORIENTED_EDGE('',*,*,#43558,.T.);
#57378=ORIENTED_EDGE('',*,*,#43514,.T.);
#57379=ORIENTED_EDGE('',*,*,#43556,.F.);
#57380=ORIENTED_EDGE('',*,*,#43543,.F.);
#57381=ORIENTED_EDGE('',*,*,#43559,.F.);
#57382=ORIENTED_EDGE('',*,*,#43422,.T.);
#57383=ORIENTED_EDGE('',*,*,#43426,.T.);
#57384=ORIENTED_EDGE('',*,*,#43430,.T.);
#57385=ORIENTED_EDGE('',*,*,#43557,.F.);
#57386=ORIENTED_EDGE('',*,*,#43428,.T.);
#57387=ORIENTED_EDGE('',*,*,#43536,.T.);
#57388=ORIENTED_EDGE('',*,*,#43558,.F.);
#57389=ORIENTED_EDGE('',*,*,#43424,.T.);
#57390=ORIENTED_EDGE('',*,*,#43529,.F.);
#57391=ORIENTED_EDGE('',*,*,#43528,.F.);
#57392=ORIENTED_EDGE('',*,*,#43560,.F.);
#57393=ORIENTED_EDGE('',*,*,#43539,.T.);
#57394=ORIENTED_EDGE('',*,*,#43537,.T.);
#57395=ORIENTED_EDGE('',*,*,#43542,.F.);
#57396=ORIENTED_EDGE('',*,*,#43561,.F.);
#57397=ORIENTED_EDGE('',*,*,#43562,.T.);
#57398=ORIENTED_EDGE('',*,*,#43526,.T.);
#57399=ORIENTED_EDGE('',*,*,#43419,.F.);
#57400=ORIENTED_EDGE('',*,*,#43559,.T.);
#57401=ORIENTED_EDGE('',*,*,#43540,.T.);
#57402=ORIENTED_EDGE('',*,*,#43560,.T.);
#57403=ORIENTED_EDGE('',*,*,#43527,.T.);
#57404=ORIENTED_EDGE('',*,*,#43562,.F.);
#57405=ORIENTED_EDGE('',*,*,#43561,.T.);
#57406=ORIENTED_EDGE('',*,*,#43541,.F.);
#57407=ORIENTED_EDGE('',*,*,#43530,.F.);
#57408=ORIENTED_EDGE('',*,*,#43511,.T.);
#57409=ORIENTED_EDGE('',*,*,#43506,.F.);
#57410=ORIENTED_EDGE('',*,*,#43551,.T.);
#57411=ORIENTED_EDGE('',*,*,#43549,.F.);
#57412=ORIENTED_EDGE('',*,*,#43553,.T.);
#57413=ORIENTED_EDGE('',*,*,#43555,.F.);
#57414=ORIENTED_EDGE('',*,*,#43508,.T.);
#57415=ORIENTED_EDGE('',*,*,#43563,.F.);
#57416=ORIENTED_EDGE('',*,*,#43564,.F.);
#57417=ORIENTED_EDGE('',*,*,#43565,.F.);
#57418=ORIENTED_EDGE('',*,*,#43566,.T.);
#57419=ORIENTED_EDGE('',*,*,#43567,.F.);
#57420=ORIENTED_EDGE('',*,*,#43568,.T.);
#57421=ORIENTED_EDGE('',*,*,#43569,.T.);
#57422=ORIENTED_EDGE('',*,*,#43570,.F.);
#57423=ORIENTED_EDGE('',*,*,#43566,.F.);
#57424=ORIENTED_EDGE('',*,*,#43571,.F.);
#57425=ORIENTED_EDGE('',*,*,#43569,.F.);
#57426=ORIENTED_EDGE('',*,*,#43572,.T.);
#57427=ORIENTED_EDGE('',*,*,#43573,.T.);
#57428=ORIENTED_EDGE('',*,*,#43564,.T.);
#57429=ORIENTED_EDGE('',*,*,#43574,.F.);
#57430=ORIENTED_EDGE('',*,*,#43573,.F.);
#57431=ORIENTED_EDGE('',*,*,#43575,.T.);
#57432=ORIENTED_EDGE('',*,*,#43576,.F.);
#57433=ORIENTED_EDGE('',*,*,#43577,.T.);
#57434=ORIENTED_EDGE('',*,*,#43567,.T.);
#57435=ORIENTED_EDGE('',*,*,#43565,.T.);
#57436=ORIENTED_EDGE('',*,*,#43576,.T.);
#57437=ORIENTED_EDGE('',*,*,#43578,.F.);
#57438=ORIENTED_EDGE('',*,*,#43579,.F.);
#57439=ORIENTED_EDGE('',*,*,#43580,.F.);
#57440=ORIENTED_EDGE('',*,*,#43581,.T.);
#57441=ORIENTED_EDGE('',*,*,#43582,.T.);
#57442=ORIENTED_EDGE('',*,*,#43583,.T.);
#57443=ORIENTED_EDGE('',*,*,#43584,.F.);
#57444=ORIENTED_EDGE('',*,*,#43581,.F.);
#57445=ORIENTED_EDGE('',*,*,#43585,.F.);
#57446=ORIENTED_EDGE('',*,*,#43586,.F.);
#57447=ORIENTED_EDGE('',*,*,#43583,.F.);
#57448=ORIENTED_EDGE('',*,*,#43587,.T.);
#57449=ORIENTED_EDGE('',*,*,#43588,.T.);
#57450=ORIENTED_EDGE('',*,*,#43579,.T.);
#57451=ORIENTED_EDGE('',*,*,#43589,.F.);
#57452=ORIENTED_EDGE('',*,*,#43588,.F.);
#57453=ORIENTED_EDGE('',*,*,#43590,.T.);
#57454=ORIENTED_EDGE('',*,*,#43591,.F.);
#57455=ORIENTED_EDGE('',*,*,#43592,.T.);
#57456=ORIENTED_EDGE('',*,*,#43585,.T.);
#57457=ORIENTED_EDGE('',*,*,#43580,.T.);
#57458=ORIENTED_EDGE('',*,*,#43591,.T.);
#57459=ORIENTED_EDGE('',*,*,#43593,.F.);
#57460=ORIENTED_EDGE('',*,*,#43594,.T.);
#57461=ORIENTED_EDGE('',*,*,#43595,.T.);
#57462=ORIENTED_EDGE('',*,*,#43596,.F.);
#57463=ORIENTED_EDGE('',*,*,#43597,.F.);
#57464=ORIENTED_EDGE('',*,*,#43598,.F.);
#57465=ORIENTED_EDGE('',*,*,#43593,.T.);
#57466=ORIENTED_EDGE('',*,*,#43599,.F.);
#57467=ORIENTED_EDGE('',*,*,#43600,.F.);
#57468=ORIENTED_EDGE('',*,*,#43601,.F.);
#57469=ORIENTED_EDGE('',*,*,#43597,.T.);
#57470=ORIENTED_EDGE('',*,*,#43602,.F.);
#57471=ORIENTED_EDGE('',*,*,#43595,.F.);
#57472=ORIENTED_EDGE('',*,*,#43603,.T.);
#57473=ORIENTED_EDGE('',*,*,#43604,.F.);
#57474=ORIENTED_EDGE('',*,*,#43600,.T.);
#57475=ORIENTED_EDGE('',*,*,#43605,.F.);
#57476=ORIENTED_EDGE('',*,*,#43598,.T.);
#57477=ORIENTED_EDGE('',*,*,#43601,.T.);
#57478=ORIENTED_EDGE('',*,*,#43604,.T.);
#57479=ORIENTED_EDGE('',*,*,#43606,.T.);
#57480=ORIENTED_EDGE('',*,*,#43607,.F.);
#57481=ORIENTED_EDGE('',*,*,#43608,.T.);
#57482=ORIENTED_EDGE('',*,*,#43609,.T.);
#57483=ORIENTED_EDGE('',*,*,#43610,.F.);
#57484=ORIENTED_EDGE('',*,*,#43611,.F.);
#57485=ORIENTED_EDGE('',*,*,#43612,.T.);
#57486=ORIENTED_EDGE('',*,*,#43607,.T.);
#57487=ORIENTED_EDGE('',*,*,#43613,.F.);
#57488=ORIENTED_EDGE('',*,*,#43614,.F.);
#57489=ORIENTED_EDGE('',*,*,#43615,.T.);
#57490=ORIENTED_EDGE('',*,*,#43611,.T.);
#57491=ORIENTED_EDGE('',*,*,#43616,.F.);
#57492=ORIENTED_EDGE('',*,*,#43609,.F.);
#57493=ORIENTED_EDGE('',*,*,#43617,.T.);
#57494=ORIENTED_EDGE('',*,*,#43614,.T.);
#57495=ORIENTED_EDGE('',*,*,#43618,.F.);
#57496=ORIENTED_EDGE('',*,*,#43619,.F.);
#57497=ORIENTED_EDGE('',*,*,#43620,.T.);
#57498=ORIENTED_EDGE('',*,*,#43621,.T.);
#57499=ORIENTED_EDGE('',*,*,#43622,.F.);
#57500=ORIENTED_EDGE('',*,*,#43623,.F.);
#57501=ORIENTED_EDGE('',*,*,#43624,.T.);
#57502=ORIENTED_EDGE('',*,*,#43619,.T.);
#57503=ORIENTED_EDGE('',*,*,#43625,.F.);
#57504=ORIENTED_EDGE('',*,*,#43626,.F.);
#57505=ORIENTED_EDGE('',*,*,#43627,.T.);
#57506=ORIENTED_EDGE('',*,*,#43623,.T.);
#57507=ORIENTED_EDGE('',*,*,#43628,.F.);
#57508=ORIENTED_EDGE('',*,*,#43621,.F.);
#57509=ORIENTED_EDGE('',*,*,#43629,.T.);
#57510=ORIENTED_EDGE('',*,*,#43626,.T.);
#57511=ORIENTED_EDGE('',*,*,#43630,.F.);
#57512=ORIENTED_EDGE('',*,*,#43631,.F.);
#57513=ORIENTED_EDGE('',*,*,#43632,.T.);
#57514=ORIENTED_EDGE('',*,*,#43633,.T.);
#57515=ORIENTED_EDGE('',*,*,#43634,.F.);
#57516=ORIENTED_EDGE('',*,*,#43635,.F.);
#57517=ORIENTED_EDGE('',*,*,#43636,.T.);
#57518=ORIENTED_EDGE('',*,*,#43631,.T.);
#57519=ORIENTED_EDGE('',*,*,#43637,.F.);
#57520=ORIENTED_EDGE('',*,*,#43638,.F.);
#57521=ORIENTED_EDGE('',*,*,#43639,.T.);
#57522=ORIENTED_EDGE('',*,*,#43635,.T.);
#57523=ORIENTED_EDGE('',*,*,#43640,.F.);
#57524=ORIENTED_EDGE('',*,*,#43633,.F.);
#57525=ORIENTED_EDGE('',*,*,#43641,.T.);
#57526=ORIENTED_EDGE('',*,*,#43638,.T.);
#57527=ORIENTED_EDGE('',*,*,#43642,.F.);
#57528=ORIENTED_EDGE('',*,*,#43643,.F.);
#57529=ORIENTED_EDGE('',*,*,#43644,.T.);
#57530=ORIENTED_EDGE('',*,*,#43645,.T.);
#57531=ORIENTED_EDGE('',*,*,#43646,.F.);
#57532=ORIENTED_EDGE('',*,*,#43647,.F.);
#57533=ORIENTED_EDGE('',*,*,#43648,.T.);
#57534=ORIENTED_EDGE('',*,*,#43643,.T.);
#57535=ORIENTED_EDGE('',*,*,#43649,.F.);
#57536=ORIENTED_EDGE('',*,*,#43650,.F.);
#57537=ORIENTED_EDGE('',*,*,#43651,.T.);
#57538=ORIENTED_EDGE('',*,*,#43647,.T.);
#57539=ORIENTED_EDGE('',*,*,#43652,.F.);
#57540=ORIENTED_EDGE('',*,*,#43645,.F.);
#57541=ORIENTED_EDGE('',*,*,#43653,.T.);
#57542=ORIENTED_EDGE('',*,*,#43650,.T.);
#57543=ORIENTED_EDGE('',*,*,#43654,.F.);
#57544=ORIENTED_EDGE('',*,*,#43655,.F.);
#57545=ORIENTED_EDGE('',*,*,#43656,.F.);
#57546=ORIENTED_EDGE('',*,*,#43657,.F.);
#57547=ORIENTED_EDGE('',*,*,#43658,.T.);
#57548=ORIENTED_EDGE('',*,*,#43659,.T.);
#57549=ORIENTED_EDGE('',*,*,#43660,.T.);
#57550=ORIENTED_EDGE('',*,*,#43661,.F.);
#57551=ORIENTED_EDGE('',*,*,#43658,.F.);
#57552=ORIENTED_EDGE('',*,*,#43662,.F.);
#57553=ORIENTED_EDGE('',*,*,#43663,.F.);
#57554=ORIENTED_EDGE('',*,*,#43660,.F.);
#57555=ORIENTED_EDGE('',*,*,#43664,.T.);
#57556=ORIENTED_EDGE('',*,*,#43665,.T.);
#57557=ORIENTED_EDGE('',*,*,#43656,.T.);
#57558=ORIENTED_EDGE('',*,*,#43666,.F.);
#57559=ORIENTED_EDGE('',*,*,#43665,.F.);
#57560=ORIENTED_EDGE('',*,*,#43667,.T.);
#57561=ORIENTED_EDGE('',*,*,#43668,.F.);
#57562=ORIENTED_EDGE('',*,*,#43669,.T.);
#57563=ORIENTED_EDGE('',*,*,#43662,.T.);
#57564=ORIENTED_EDGE('',*,*,#43657,.T.);
#57565=ORIENTED_EDGE('',*,*,#43668,.T.);
#57566=ORIENTED_EDGE('',*,*,#43670,.F.);
#57567=ORIENTED_EDGE('',*,*,#43671,.T.);
#57568=ORIENTED_EDGE('',*,*,#43672,.T.);
#57569=ORIENTED_EDGE('',*,*,#43673,.F.);
#57570=ORIENTED_EDGE('',*,*,#43674,.F.);
#57571=ORIENTED_EDGE('',*,*,#43675,.F.);
#57572=ORIENTED_EDGE('',*,*,#43676,.T.);
#57573=ORIENTED_EDGE('',*,*,#43670,.T.);
#57574=ORIENTED_EDGE('',*,*,#43677,.F.);
#57575=ORIENTED_EDGE('',*,*,#43678,.F.);
#57576=ORIENTED_EDGE('',*,*,#43679,.F.);
#57577=ORIENTED_EDGE('',*,*,#43674,.T.);
#57578=ORIENTED_EDGE('',*,*,#43680,.F.);
#57579=ORIENTED_EDGE('',*,*,#43672,.F.);
#57580=ORIENTED_EDGE('',*,*,#43681,.T.);
#57581=ORIENTED_EDGE('',*,*,#43682,.F.);
#57582=ORIENTED_EDGE('',*,*,#43678,.T.);
#57583=ORIENTED_EDGE('',*,*,#43683,.F.);
#57584=ORIENTED_EDGE('',*,*,#43675,.T.);
#57585=ORIENTED_EDGE('',*,*,#43679,.T.);
#57586=ORIENTED_EDGE('',*,*,#43682,.T.);
#57587=ORIENTED_EDGE('',*,*,#43684,.T.);
#57588=ORIENTED_EDGE('',*,*,#43685,.F.);
#57589=ORIENTED_EDGE('',*,*,#43686,.T.);
#57590=ORIENTED_EDGE('',*,*,#43687,.T.);
#57591=ORIENTED_EDGE('',*,*,#43688,.F.);
#57592=ORIENTED_EDGE('',*,*,#43689,.F.);
#57593=ORIENTED_EDGE('',*,*,#43690,.F.);
#57594=ORIENTED_EDGE('',*,*,#43691,.T.);
#57595=ORIENTED_EDGE('',*,*,#43685,.T.);
#57596=ORIENTED_EDGE('',*,*,#43692,.F.);
#57597=ORIENTED_EDGE('',*,*,#43693,.F.);
#57598=ORIENTED_EDGE('',*,*,#43694,.F.);
#57599=ORIENTED_EDGE('',*,*,#43689,.T.);
#57600=ORIENTED_EDGE('',*,*,#43695,.F.);
#57601=ORIENTED_EDGE('',*,*,#43687,.F.);
#57602=ORIENTED_EDGE('',*,*,#43696,.T.);
#57603=ORIENTED_EDGE('',*,*,#43697,.F.);
#57604=ORIENTED_EDGE('',*,*,#43693,.T.);
#57605=ORIENTED_EDGE('',*,*,#43698,.F.);
#57606=ORIENTED_EDGE('',*,*,#43690,.T.);
#57607=ORIENTED_EDGE('',*,*,#43694,.T.);
#57608=ORIENTED_EDGE('',*,*,#43697,.T.);
#57609=ORIENTED_EDGE('',*,*,#43699,.T.);
#57610=ORIENTED_EDGE('',*,*,#43700,.F.);
#57611=ORIENTED_EDGE('',*,*,#43701,.T.);
#57612=ORIENTED_EDGE('',*,*,#43702,.T.);
#57613=ORIENTED_EDGE('',*,*,#43703,.F.);
#57614=ORIENTED_EDGE('',*,*,#43704,.F.);
#57615=ORIENTED_EDGE('',*,*,#43705,.T.);
#57616=ORIENTED_EDGE('',*,*,#43700,.T.);
#57617=ORIENTED_EDGE('',*,*,#43706,.F.);
#57618=ORIENTED_EDGE('',*,*,#43707,.F.);
#57619=ORIENTED_EDGE('',*,*,#43708,.F.);
#57620=ORIENTED_EDGE('',*,*,#43709,.T.);
#57621=ORIENTED_EDGE('',*,*,#43704,.T.);
#57622=ORIENTED_EDGE('',*,*,#43710,.F.);
#57623=ORIENTED_EDGE('',*,*,#43702,.F.);
#57624=ORIENTED_EDGE('',*,*,#43711,.T.);
#57625=ORIENTED_EDGE('',*,*,#43712,.F.);
#57626=ORIENTED_EDGE('',*,*,#43707,.T.);
#57627=ORIENTED_EDGE('',*,*,#43713,.F.);
#57628=ORIENTED_EDGE('',*,*,#43708,.T.);
#57629=ORIENTED_EDGE('',*,*,#43712,.T.);
#57630=ORIENTED_EDGE('',*,*,#43714,.T.);
#57631=ORIENTED_EDGE('',*,*,#43715,.F.);
#57632=ORIENTED_EDGE('',*,*,#43716,.T.);
#57633=ORIENTED_EDGE('',*,*,#43717,.T.);
#57634=ORIENTED_EDGE('',*,*,#43718,.F.);
#57635=ORIENTED_EDGE('',*,*,#43719,.F.);
#57636=ORIENTED_EDGE('',*,*,#43720,.T.);
#57637=ORIENTED_EDGE('',*,*,#43715,.T.);
#57638=ORIENTED_EDGE('',*,*,#43721,.F.);
#57639=ORIENTED_EDGE('',*,*,#43722,.F.);
#57640=ORIENTED_EDGE('',*,*,#43723,.T.);
#57641=ORIENTED_EDGE('',*,*,#43719,.T.);
#57642=ORIENTED_EDGE('',*,*,#43724,.F.);
#57643=ORIENTED_EDGE('',*,*,#43717,.F.);
#57644=ORIENTED_EDGE('',*,*,#43725,.T.);
#57645=ORIENTED_EDGE('',*,*,#43722,.T.);
#57646=ORIENTED_EDGE('',*,*,#43726,.F.);
#57647=ORIENTED_EDGE('',*,*,#43727,.F.);
#57648=ORIENTED_EDGE('',*,*,#43728,.T.);
#57649=ORIENTED_EDGE('',*,*,#43729,.T.);
#57650=ORIENTED_EDGE('',*,*,#43730,.F.);
#57651=ORIENTED_EDGE('',*,*,#43731,.F.);
#57652=ORIENTED_EDGE('',*,*,#43732,.F.);
#57653=ORIENTED_EDGE('',*,*,#43733,.T.);
#57654=ORIENTED_EDGE('',*,*,#43727,.T.);
#57655=ORIENTED_EDGE('',*,*,#43734,.F.);
#57656=ORIENTED_EDGE('',*,*,#43735,.F.);
#57657=ORIENTED_EDGE('',*,*,#43736,.F.);
#57658=ORIENTED_EDGE('',*,*,#43731,.T.);
#57659=ORIENTED_EDGE('',*,*,#43737,.F.);
#57660=ORIENTED_EDGE('',*,*,#43729,.F.);
#57661=ORIENTED_EDGE('',*,*,#43738,.T.);
#57662=ORIENTED_EDGE('',*,*,#43739,.F.);
#57663=ORIENTED_EDGE('',*,*,#43735,.T.);
#57664=ORIENTED_EDGE('',*,*,#43740,.F.);
#57665=ORIENTED_EDGE('',*,*,#43732,.T.);
#57666=ORIENTED_EDGE('',*,*,#43736,.T.);
#57667=ORIENTED_EDGE('',*,*,#43739,.T.);
#57668=ORIENTED_EDGE('',*,*,#43741,.T.);
#57669=ORIENTED_EDGE('',*,*,#43742,.F.);
#57670=ORIENTED_EDGE('',*,*,#43743,.T.);
#57671=ORIENTED_EDGE('',*,*,#43744,.T.);
#57672=ORIENTED_EDGE('',*,*,#43745,.F.);
#57673=ORIENTED_EDGE('',*,*,#43746,.F.);
#57674=ORIENTED_EDGE('',*,*,#43747,.F.);
#57675=ORIENTED_EDGE('',*,*,#43748,.T.);
#57676=ORIENTED_EDGE('',*,*,#43742,.T.);
#57677=ORIENTED_EDGE('',*,*,#43749,.F.);
#57678=ORIENTED_EDGE('',*,*,#43750,.F.);
#57679=ORIENTED_EDGE('',*,*,#43751,.F.);
#57680=ORIENTED_EDGE('',*,*,#43746,.T.);
#57681=ORIENTED_EDGE('',*,*,#43752,.F.);
#57682=ORIENTED_EDGE('',*,*,#43744,.F.);
#57683=ORIENTED_EDGE('',*,*,#43753,.T.);
#57684=ORIENTED_EDGE('',*,*,#43754,.F.);
#57685=ORIENTED_EDGE('',*,*,#43750,.T.);
#57686=ORIENTED_EDGE('',*,*,#43755,.F.);
#57687=ORIENTED_EDGE('',*,*,#43747,.T.);
#57688=ORIENTED_EDGE('',*,*,#43751,.T.);
#57689=ORIENTED_EDGE('',*,*,#43754,.T.);
#57690=ORIENTED_EDGE('',*,*,#43756,.T.);
#57691=ORIENTED_EDGE('',*,*,#43757,.F.);
#57692=ORIENTED_EDGE('',*,*,#43758,.T.);
#57693=ORIENTED_EDGE('',*,*,#43759,.T.);
#57694=ORIENTED_EDGE('',*,*,#43760,.F.);
#57695=ORIENTED_EDGE('',*,*,#43761,.F.);
#57696=ORIENTED_EDGE('',*,*,#43762,.F.);
#57697=ORIENTED_EDGE('',*,*,#43763,.T.);
#57698=ORIENTED_EDGE('',*,*,#43757,.T.);
#57699=ORIENTED_EDGE('',*,*,#43764,.F.);
#57700=ORIENTED_EDGE('',*,*,#43765,.F.);
#57701=ORIENTED_EDGE('',*,*,#43766,.F.);
#57702=ORIENTED_EDGE('',*,*,#43761,.T.);
#57703=ORIENTED_EDGE('',*,*,#43767,.F.);
#57704=ORIENTED_EDGE('',*,*,#43759,.F.);
#57705=ORIENTED_EDGE('',*,*,#43768,.T.);
#57706=ORIENTED_EDGE('',*,*,#43769,.F.);
#57707=ORIENTED_EDGE('',*,*,#43765,.T.);
#57708=ORIENTED_EDGE('',*,*,#43770,.F.);
#57709=ORIENTED_EDGE('',*,*,#43762,.T.);
#57710=ORIENTED_EDGE('',*,*,#43766,.T.);
#57711=ORIENTED_EDGE('',*,*,#43769,.T.);
#57712=ORIENTED_EDGE('',*,*,#43771,.T.);
#57713=ORIENTED_EDGE('',*,*,#43772,.F.);
#57714=ORIENTED_EDGE('',*,*,#43773,.T.);
#57715=ORIENTED_EDGE('',*,*,#43774,.T.);
#57716=ORIENTED_EDGE('',*,*,#43775,.F.);
#57717=ORIENTED_EDGE('',*,*,#43776,.F.);
#57718=ORIENTED_EDGE('',*,*,#43777,.F.);
#57719=ORIENTED_EDGE('',*,*,#43778,.T.);
#57720=ORIENTED_EDGE('',*,*,#43772,.T.);
#57721=ORIENTED_EDGE('',*,*,#43779,.F.);
#57722=ORIENTED_EDGE('',*,*,#43780,.F.);
#57723=ORIENTED_EDGE('',*,*,#43781,.F.);
#57724=ORIENTED_EDGE('',*,*,#43776,.T.);
#57725=ORIENTED_EDGE('',*,*,#43782,.F.);
#57726=ORIENTED_EDGE('',*,*,#43774,.F.);
#57727=ORIENTED_EDGE('',*,*,#43783,.T.);
#57728=ORIENTED_EDGE('',*,*,#43784,.F.);
#57729=ORIENTED_EDGE('',*,*,#43780,.T.);
#57730=ORIENTED_EDGE('',*,*,#43785,.F.);
#57731=ORIENTED_EDGE('',*,*,#43777,.T.);
#57732=ORIENTED_EDGE('',*,*,#43781,.T.);
#57733=ORIENTED_EDGE('',*,*,#43784,.T.);
#57734=ORIENTED_EDGE('',*,*,#43786,.T.);
#57735=ORIENTED_EDGE('',*,*,#43787,.F.);
#57736=ORIENTED_EDGE('',*,*,#43788,.T.);
#57737=ORIENTED_EDGE('',*,*,#43789,.T.);
#57738=ORIENTED_EDGE('',*,*,#43790,.F.);
#57739=ORIENTED_EDGE('',*,*,#43791,.F.);
#57740=ORIENTED_EDGE('',*,*,#43792,.T.);
#57741=ORIENTED_EDGE('',*,*,#43787,.T.);
#57742=ORIENTED_EDGE('',*,*,#43793,.F.);
#57743=ORIENTED_EDGE('',*,*,#43794,.F.);
#57744=ORIENTED_EDGE('',*,*,#43795,.T.);
#57745=ORIENTED_EDGE('',*,*,#43791,.T.);
#57746=ORIENTED_EDGE('',*,*,#43796,.F.);
#57747=ORIENTED_EDGE('',*,*,#43789,.F.);
#57748=ORIENTED_EDGE('',*,*,#43797,.T.);
#57749=ORIENTED_EDGE('',*,*,#43794,.T.);
#57750=ORIENTED_EDGE('',*,*,#43798,.F.);
#57751=ORIENTED_EDGE('',*,*,#43799,.F.);
#57752=ORIENTED_EDGE('',*,*,#43800,.T.);
#57753=ORIENTED_EDGE('',*,*,#43801,.T.);
#57754=ORIENTED_EDGE('',*,*,#43802,.F.);
#57755=ORIENTED_EDGE('',*,*,#43803,.F.);
#57756=ORIENTED_EDGE('',*,*,#43804,.T.);
#57757=ORIENTED_EDGE('',*,*,#43799,.T.);
#57758=ORIENTED_EDGE('',*,*,#43805,.F.);
#57759=ORIENTED_EDGE('',*,*,#43806,.F.);
#57760=ORIENTED_EDGE('',*,*,#43807,.T.);
#57761=ORIENTED_EDGE('',*,*,#43803,.T.);
#57762=ORIENTED_EDGE('',*,*,#43808,.F.);
#57763=ORIENTED_EDGE('',*,*,#43801,.F.);
#57764=ORIENTED_EDGE('',*,*,#43809,.T.);
#57765=ORIENTED_EDGE('',*,*,#43806,.T.);
#57766=ORIENTED_EDGE('',*,*,#43810,.F.);
#57767=ORIENTED_EDGE('',*,*,#43811,.F.);
#57768=ORIENTED_EDGE('',*,*,#43812,.T.);
#57769=ORIENTED_EDGE('',*,*,#43813,.T.);
#57770=ORIENTED_EDGE('',*,*,#43814,.F.);
#57771=ORIENTED_EDGE('',*,*,#43815,.F.);
#57772=ORIENTED_EDGE('',*,*,#43816,.T.);
#57773=ORIENTED_EDGE('',*,*,#43811,.T.);
#57774=ORIENTED_EDGE('',*,*,#43817,.F.);
#57775=ORIENTED_EDGE('',*,*,#43818,.F.);
#57776=ORIENTED_EDGE('',*,*,#43819,.T.);
#57777=ORIENTED_EDGE('',*,*,#43815,.T.);
#57778=ORIENTED_EDGE('',*,*,#43820,.F.);
#57779=ORIENTED_EDGE('',*,*,#43813,.F.);
#57780=ORIENTED_EDGE('',*,*,#43821,.T.);
#57781=ORIENTED_EDGE('',*,*,#43818,.T.);
#57782=ORIENTED_EDGE('',*,*,#43822,.F.);
#57783=ORIENTED_EDGE('',*,*,#43823,.F.);
#57784=ORIENTED_EDGE('',*,*,#43824,.T.);
#57785=ORIENTED_EDGE('',*,*,#43825,.T.);
#57786=ORIENTED_EDGE('',*,*,#43826,.F.);
#57787=ORIENTED_EDGE('',*,*,#43827,.F.);
#57788=ORIENTED_EDGE('',*,*,#43828,.T.);
#57789=ORIENTED_EDGE('',*,*,#43823,.T.);
#57790=ORIENTED_EDGE('',*,*,#43829,.F.);
#57791=ORIENTED_EDGE('',*,*,#43830,.F.);
#57792=ORIENTED_EDGE('',*,*,#43831,.T.);
#57793=ORIENTED_EDGE('',*,*,#43827,.T.);
#57794=ORIENTED_EDGE('',*,*,#43832,.F.);
#57795=ORIENTED_EDGE('',*,*,#43825,.F.);
#57796=ORIENTED_EDGE('',*,*,#43833,.T.);
#57797=ORIENTED_EDGE('',*,*,#43830,.T.);
#57798=ORIENTED_EDGE('',*,*,#43834,.F.);
#57799=ORIENTED_EDGE('',*,*,#43835,.F.);
#57800=ORIENTED_EDGE('',*,*,#43836,.T.);
#57801=ORIENTED_EDGE('',*,*,#43837,.T.);
#57802=ORIENTED_EDGE('',*,*,#43838,.F.);
#57803=ORIENTED_EDGE('',*,*,#43839,.F.);
#57804=ORIENTED_EDGE('',*,*,#43840,.T.);
#57805=ORIENTED_EDGE('',*,*,#43835,.T.);
#57806=ORIENTED_EDGE('',*,*,#43841,.F.);
#57807=ORIENTED_EDGE('',*,*,#43842,.F.);
#57808=ORIENTED_EDGE('',*,*,#43843,.T.);
#57809=ORIENTED_EDGE('',*,*,#43839,.T.);
#57810=ORIENTED_EDGE('',*,*,#43844,.F.);
#57811=ORIENTED_EDGE('',*,*,#43837,.F.);
#57812=ORIENTED_EDGE('',*,*,#43845,.T.);
#57813=ORIENTED_EDGE('',*,*,#43842,.T.);
#57814=ORIENTED_EDGE('',*,*,#43846,.F.);
#57815=ORIENTED_EDGE('',*,*,#43847,.F.);
#57816=ORIENTED_EDGE('',*,*,#43848,.T.);
#57817=ORIENTED_EDGE('',*,*,#43849,.T.);
#57818=ORIENTED_EDGE('',*,*,#43850,.F.);
#57819=ORIENTED_EDGE('',*,*,#43851,.F.);
#57820=ORIENTED_EDGE('',*,*,#43852,.T.);
#57821=ORIENTED_EDGE('',*,*,#43847,.T.);
#57822=ORIENTED_EDGE('',*,*,#43853,.F.);
#57823=ORIENTED_EDGE('',*,*,#43854,.F.);
#57824=ORIENTED_EDGE('',*,*,#43855,.T.);
#57825=ORIENTED_EDGE('',*,*,#43851,.T.);
#57826=ORIENTED_EDGE('',*,*,#43856,.F.);
#57827=ORIENTED_EDGE('',*,*,#43849,.F.);
#57828=ORIENTED_EDGE('',*,*,#43857,.T.);
#57829=ORIENTED_EDGE('',*,*,#43854,.T.);
#57830=ORIENTED_EDGE('',*,*,#43858,.F.);
#57831=ORIENTED_EDGE('',*,*,#43859,.F.);
#57832=ORIENTED_EDGE('',*,*,#43860,.F.);
#57833=ORIENTED_EDGE('',*,*,#43861,.T.);
#57834=ORIENTED_EDGE('',*,*,#43862,.T.);
#57835=ORIENTED_EDGE('',*,*,#43863,.F.);
#57836=ORIENTED_EDGE('',*,*,#43864,.F.);
#57837=ORIENTED_EDGE('',*,*,#43865,.T.);
#57838=ORIENTED_EDGE('',*,*,#43860,.T.);
#57839=ORIENTED_EDGE('',*,*,#43866,.F.);
#57840=ORIENTED_EDGE('',*,*,#43867,.T.);
#57841=ORIENTED_EDGE('',*,*,#43864,.T.);
#57842=ORIENTED_EDGE('',*,*,#43868,.F.);
#57843=ORIENTED_EDGE('',*,*,#43869,.F.);
#57844=ORIENTED_EDGE('',*,*,#43870,.F.);
#57845=ORIENTED_EDGE('',*,*,#43862,.F.);
#57846=ORIENTED_EDGE('',*,*,#43871,.T.);
#57847=ORIENTED_EDGE('',*,*,#43872,.F.);
#57848=ORIENTED_EDGE('',*,*,#43869,.T.);
#57849=ORIENTED_EDGE('',*,*,#43866,.T.);
#57850=ORIENTED_EDGE('',*,*,#43872,.T.);
#57851=ORIENTED_EDGE('',*,*,#43873,.T.);
#57852=ORIENTED_EDGE('',*,*,#43874,.F.);
#57853=ORIENTED_EDGE('',*,*,#43875,.T.);
#57854=ORIENTED_EDGE('',*,*,#43876,.T.);
#57855=ORIENTED_EDGE('',*,*,#43877,.F.);
#57856=ORIENTED_EDGE('',*,*,#43878,.F.);
#57857=ORIENTED_EDGE('',*,*,#43879,.F.);
#57858=ORIENTED_EDGE('',*,*,#43880,.T.);
#57859=ORIENTED_EDGE('',*,*,#43874,.T.);
#57860=ORIENTED_EDGE('',*,*,#43881,.F.);
#57861=ORIENTED_EDGE('',*,*,#43882,.F.);
#57862=ORIENTED_EDGE('',*,*,#43883,.F.);
#57863=ORIENTED_EDGE('',*,*,#43878,.T.);
#57864=ORIENTED_EDGE('',*,*,#43884,.F.);
#57865=ORIENTED_EDGE('',*,*,#43876,.F.);
#57866=ORIENTED_EDGE('',*,*,#43885,.T.);
#57867=ORIENTED_EDGE('',*,*,#43886,.F.);
#57868=ORIENTED_EDGE('',*,*,#43882,.T.);
#57869=ORIENTED_EDGE('',*,*,#43887,.F.);
#57870=ORIENTED_EDGE('',*,*,#43879,.T.);
#57871=ORIENTED_EDGE('',*,*,#43883,.T.);
#57872=ORIENTED_EDGE('',*,*,#43886,.T.);
#57873=ORIENTED_EDGE('',*,*,#43888,.T.);
#57874=ORIENTED_EDGE('',*,*,#43889,.F.);
#57875=ORIENTED_EDGE('',*,*,#43890,.T.);
#57876=ORIENTED_EDGE('',*,*,#43891,.T.);
#57877=ORIENTED_EDGE('',*,*,#43892,.F.);
#57878=ORIENTED_EDGE('',*,*,#43893,.F.);
#57879=ORIENTED_EDGE('',*,*,#43894,.T.);
#57880=ORIENTED_EDGE('',*,*,#43889,.T.);
#57881=ORIENTED_EDGE('',*,*,#43895,.F.);
#57882=ORIENTED_EDGE('',*,*,#43896,.F.);
#57883=ORIENTED_EDGE('',*,*,#43897,.T.);
#57884=ORIENTED_EDGE('',*,*,#43893,.T.);
#57885=ORIENTED_EDGE('',*,*,#43898,.F.);
#57886=ORIENTED_EDGE('',*,*,#43891,.F.);
#57887=ORIENTED_EDGE('',*,*,#43899,.T.);
#57888=ORIENTED_EDGE('',*,*,#43896,.T.);
#57889=ORIENTED_EDGE('',*,*,#43900,.F.);
#57890=ORIENTED_EDGE('',*,*,#43901,.F.);
#57891=ORIENTED_EDGE('',*,*,#43902,.T.);
#57892=ORIENTED_EDGE('',*,*,#43903,.T.);
#57893=ORIENTED_EDGE('',*,*,#43904,.F.);
#57894=ORIENTED_EDGE('',*,*,#43905,.F.);
#57895=ORIENTED_EDGE('',*,*,#43906,.T.);
#57896=ORIENTED_EDGE('',*,*,#43901,.T.);
#57897=ORIENTED_EDGE('',*,*,#43907,.F.);
#57898=ORIENTED_EDGE('',*,*,#43908,.F.);
#57899=ORIENTED_EDGE('',*,*,#43909,.T.);
#57900=ORIENTED_EDGE('',*,*,#43905,.T.);
#57901=ORIENTED_EDGE('',*,*,#43910,.F.);
#57902=ORIENTED_EDGE('',*,*,#43903,.F.);
#57903=ORIENTED_EDGE('',*,*,#43911,.T.);
#57904=ORIENTED_EDGE('',*,*,#43908,.T.);
#57905=ORIENTED_EDGE('',*,*,#43912,.F.);
#57906=ORIENTED_EDGE('',*,*,#43913,.F.);
#57907=ORIENTED_EDGE('',*,*,#43914,.T.);
#57908=ORIENTED_EDGE('',*,*,#43915,.T.);
#57909=ORIENTED_EDGE('',*,*,#43916,.F.);
#57910=ORIENTED_EDGE('',*,*,#43917,.F.);
#57911=ORIENTED_EDGE('',*,*,#43918,.T.);
#57912=ORIENTED_EDGE('',*,*,#43913,.T.);
#57913=ORIENTED_EDGE('',*,*,#43919,.F.);
#57914=ORIENTED_EDGE('',*,*,#43920,.F.);
#57915=ORIENTED_EDGE('',*,*,#43921,.T.);
#57916=ORIENTED_EDGE('',*,*,#43917,.T.);
#57917=ORIENTED_EDGE('',*,*,#43922,.F.);
#57918=ORIENTED_EDGE('',*,*,#43915,.F.);
#57919=ORIENTED_EDGE('',*,*,#43923,.T.);
#57920=ORIENTED_EDGE('',*,*,#43920,.T.);
#57921=ORIENTED_EDGE('',*,*,#43924,.F.);
#57922=ORIENTED_EDGE('',*,*,#43925,.F.);
#57923=ORIENTED_EDGE('',*,*,#43926,.T.);
#57924=ORIENTED_EDGE('',*,*,#43927,.T.);
#57925=ORIENTED_EDGE('',*,*,#43928,.F.);
#57926=ORIENTED_EDGE('',*,*,#43929,.F.);
#57927=ORIENTED_EDGE('',*,*,#43930,.T.);
#57928=ORIENTED_EDGE('',*,*,#43925,.T.);
#57929=ORIENTED_EDGE('',*,*,#43931,.F.);
#57930=ORIENTED_EDGE('',*,*,#43932,.F.);
#57931=ORIENTED_EDGE('',*,*,#43933,.T.);
#57932=ORIENTED_EDGE('',*,*,#43929,.T.);
#57933=ORIENTED_EDGE('',*,*,#43934,.F.);
#57934=ORIENTED_EDGE('',*,*,#43927,.F.);
#57935=ORIENTED_EDGE('',*,*,#43935,.T.);
#57936=ORIENTED_EDGE('',*,*,#43932,.T.);
#57937=ORIENTED_EDGE('',*,*,#43936,.F.);
#57938=ORIENTED_EDGE('',*,*,#43937,.F.);
#57939=ORIENTED_EDGE('',*,*,#43938,.T.);
#57940=ORIENTED_EDGE('',*,*,#43939,.T.);
#57941=ORIENTED_EDGE('',*,*,#43940,.F.);
#57942=ORIENTED_EDGE('',*,*,#43941,.F.);
#57943=ORIENTED_EDGE('',*,*,#43942,.T.);
#57944=ORIENTED_EDGE('',*,*,#43937,.T.);
#57945=ORIENTED_EDGE('',*,*,#43943,.F.);
#57946=ORIENTED_EDGE('',*,*,#43944,.F.);
#57947=ORIENTED_EDGE('',*,*,#43945,.T.);
#57948=ORIENTED_EDGE('',*,*,#43941,.T.);
#57949=ORIENTED_EDGE('',*,*,#43946,.F.);
#57950=ORIENTED_EDGE('',*,*,#43939,.F.);
#57951=ORIENTED_EDGE('',*,*,#43947,.T.);
#57952=ORIENTED_EDGE('',*,*,#43944,.T.);
#57953=ORIENTED_EDGE('',*,*,#43948,.F.);
#57954=ORIENTED_EDGE('',*,*,#43949,.F.);
#57955=ORIENTED_EDGE('',*,*,#43950,.T.);
#57956=ORIENTED_EDGE('',*,*,#43951,.T.);
#57957=ORIENTED_EDGE('',*,*,#43952,.F.);
#57958=ORIENTED_EDGE('',*,*,#43953,.F.);
#57959=ORIENTED_EDGE('',*,*,#43954,.T.);
#57960=ORIENTED_EDGE('',*,*,#43949,.T.);
#57961=ORIENTED_EDGE('',*,*,#43955,.F.);
#57962=ORIENTED_EDGE('',*,*,#43956,.F.);
#57963=ORIENTED_EDGE('',*,*,#43957,.T.);
#57964=ORIENTED_EDGE('',*,*,#43953,.T.);
#57965=ORIENTED_EDGE('',*,*,#43958,.F.);
#57966=ORIENTED_EDGE('',*,*,#43951,.F.);
#57967=ORIENTED_EDGE('',*,*,#43959,.T.);
#57968=ORIENTED_EDGE('',*,*,#43956,.T.);
#57969=ORIENTED_EDGE('',*,*,#43960,.F.);
#57970=ORIENTED_EDGE('',*,*,#43961,.F.);
#57971=ORIENTED_EDGE('',*,*,#43962,.T.);
#57972=ORIENTED_EDGE('',*,*,#43963,.T.);
#57973=ORIENTED_EDGE('',*,*,#43964,.F.);
#57974=ORIENTED_EDGE('',*,*,#43965,.F.);
#57975=ORIENTED_EDGE('',*,*,#43966,.T.);
#57976=ORIENTED_EDGE('',*,*,#43961,.T.);
#57977=ORIENTED_EDGE('',*,*,#43967,.F.);
#57978=ORIENTED_EDGE('',*,*,#43968,.F.);
#57979=ORIENTED_EDGE('',*,*,#43969,.T.);
#57980=ORIENTED_EDGE('',*,*,#43965,.T.);
#57981=ORIENTED_EDGE('',*,*,#43970,.F.);
#57982=ORIENTED_EDGE('',*,*,#43963,.F.);
#57983=ORIENTED_EDGE('',*,*,#43971,.T.);
#57984=ORIENTED_EDGE('',*,*,#43968,.T.);
#57985=ORIENTED_EDGE('',*,*,#43972,.F.);
#57986=ORIENTED_EDGE('',*,*,#43973,.F.);
#57987=ORIENTED_EDGE('',*,*,#43974,.T.);
#57988=ORIENTED_EDGE('',*,*,#43975,.T.);
#57989=ORIENTED_EDGE('',*,*,#43976,.F.);
#57990=ORIENTED_EDGE('',*,*,#43977,.F.);
#57991=ORIENTED_EDGE('',*,*,#43978,.T.);
#57992=ORIENTED_EDGE('',*,*,#43973,.T.);
#57993=ORIENTED_EDGE('',*,*,#43979,.F.);
#57994=ORIENTED_EDGE('',*,*,#43980,.F.);
#57995=ORIENTED_EDGE('',*,*,#43981,.T.);
#57996=ORIENTED_EDGE('',*,*,#43977,.T.);
#57997=ORIENTED_EDGE('',*,*,#43982,.F.);
#57998=ORIENTED_EDGE('',*,*,#43975,.F.);
#57999=ORIENTED_EDGE('',*,*,#43983,.T.);
#58000=ORIENTED_EDGE('',*,*,#43980,.T.);
#58001=ORIENTED_EDGE('',*,*,#43984,.F.);
#58002=ORIENTED_EDGE('',*,*,#43985,.F.);
#58003=ORIENTED_EDGE('',*,*,#43986,.T.);
#58004=ORIENTED_EDGE('',*,*,#43987,.T.);
#58005=ORIENTED_EDGE('',*,*,#43988,.F.);
#58006=ORIENTED_EDGE('',*,*,#43989,.F.);
#58007=ORIENTED_EDGE('',*,*,#43990,.F.);
#58008=ORIENTED_EDGE('',*,*,#43991,.T.);
#58009=ORIENTED_EDGE('',*,*,#43985,.T.);
#58010=ORIENTED_EDGE('',*,*,#43992,.F.);
#58011=ORIENTED_EDGE('',*,*,#43993,.F.);
#58012=ORIENTED_EDGE('',*,*,#43994,.F.);
#58013=ORIENTED_EDGE('',*,*,#43989,.T.);
#58014=ORIENTED_EDGE('',*,*,#43995,.F.);
#58015=ORIENTED_EDGE('',*,*,#43987,.F.);
#58016=ORIENTED_EDGE('',*,*,#43996,.T.);
#58017=ORIENTED_EDGE('',*,*,#43997,.F.);
#58018=ORIENTED_EDGE('',*,*,#43993,.T.);
#58019=ORIENTED_EDGE('',*,*,#43998,.F.);
#58020=ORIENTED_EDGE('',*,*,#43990,.T.);
#58021=ORIENTED_EDGE('',*,*,#43994,.T.);
#58022=ORIENTED_EDGE('',*,*,#43997,.T.);
#58023=ORIENTED_EDGE('',*,*,#43999,.T.);
#58024=ORIENTED_EDGE('',*,*,#44000,.F.);
#58025=ORIENTED_EDGE('',*,*,#44001,.T.);
#58026=ORIENTED_EDGE('',*,*,#44002,.T.);
#58027=ORIENTED_EDGE('',*,*,#44003,.F.);
#58028=ORIENTED_EDGE('',*,*,#44004,.F.);
#58029=ORIENTED_EDGE('',*,*,#44005,.F.);
#58030=ORIENTED_EDGE('',*,*,#44006,.T.);
#58031=ORIENTED_EDGE('',*,*,#44000,.T.);
#58032=ORIENTED_EDGE('',*,*,#44007,.F.);
#58033=ORIENTED_EDGE('',*,*,#44008,.F.);
#58034=ORIENTED_EDGE('',*,*,#44009,.F.);
#58035=ORIENTED_EDGE('',*,*,#44004,.T.);
#58036=ORIENTED_EDGE('',*,*,#44010,.F.);
#58037=ORIENTED_EDGE('',*,*,#44002,.F.);
#58038=ORIENTED_EDGE('',*,*,#44011,.T.);
#58039=ORIENTED_EDGE('',*,*,#44012,.F.);
#58040=ORIENTED_EDGE('',*,*,#44008,.T.);
#58041=ORIENTED_EDGE('',*,*,#44013,.F.);
#58042=ORIENTED_EDGE('',*,*,#44005,.T.);
#58043=ORIENTED_EDGE('',*,*,#44009,.T.);
#58044=ORIENTED_EDGE('',*,*,#44012,.T.);
#58045=ORIENTED_EDGE('',*,*,#44014,.T.);
#58046=ORIENTED_EDGE('',*,*,#44015,.F.);
#58047=ORIENTED_EDGE('',*,*,#44016,.T.);
#58048=ORIENTED_EDGE('',*,*,#44017,.T.);
#58049=ORIENTED_EDGE('',*,*,#44018,.F.);
#58050=ORIENTED_EDGE('',*,*,#44019,.F.);
#58051=ORIENTED_EDGE('',*,*,#44020,.T.);
#58052=ORIENTED_EDGE('',*,*,#44015,.T.);
#58053=ORIENTED_EDGE('',*,*,#44021,.F.);
#58054=ORIENTED_EDGE('',*,*,#44022,.F.);
#58055=ORIENTED_EDGE('',*,*,#44023,.T.);
#58056=ORIENTED_EDGE('',*,*,#44019,.T.);
#58057=ORIENTED_EDGE('',*,*,#44024,.F.);
#58058=ORIENTED_EDGE('',*,*,#44017,.F.);
#58059=ORIENTED_EDGE('',*,*,#44025,.T.);
#58060=ORIENTED_EDGE('',*,*,#44022,.T.);
#58061=ORIENTED_EDGE('',*,*,#44026,.F.);
#58062=ORIENTED_EDGE('',*,*,#44027,.F.);
#58063=ORIENTED_EDGE('',*,*,#44028,.T.);
#58064=ORIENTED_EDGE('',*,*,#44029,.T.);
#58065=ORIENTED_EDGE('',*,*,#44030,.F.);
#58066=ORIENTED_EDGE('',*,*,#44031,.F.);
#58067=ORIENTED_EDGE('',*,*,#44032,.T.);
#58068=ORIENTED_EDGE('',*,*,#44027,.T.);
#58069=ORIENTED_EDGE('',*,*,#44033,.F.);
#58070=ORIENTED_EDGE('',*,*,#44034,.F.);
#58071=ORIENTED_EDGE('',*,*,#44035,.T.);
#58072=ORIENTED_EDGE('',*,*,#44031,.T.);
#58073=ORIENTED_EDGE('',*,*,#44036,.F.);
#58074=ORIENTED_EDGE('',*,*,#44029,.F.);
#58075=ORIENTED_EDGE('',*,*,#44037,.T.);
#58076=ORIENTED_EDGE('',*,*,#44034,.T.);
#58077=ORIENTED_EDGE('',*,*,#44038,.F.);
#58078=ORIENTED_EDGE('',*,*,#44039,.F.);
#58079=ORIENTED_EDGE('',*,*,#44040,.T.);
#58080=ORIENTED_EDGE('',*,*,#44041,.T.);
#58081=ORIENTED_EDGE('',*,*,#44042,.F.);
#58082=ORIENTED_EDGE('',*,*,#44043,.F.);
#58083=ORIENTED_EDGE('',*,*,#44044,.T.);
#58084=ORIENTED_EDGE('',*,*,#44039,.T.);
#58085=ORIENTED_EDGE('',*,*,#44045,.F.);
#58086=ORIENTED_EDGE('',*,*,#44046,.F.);
#58087=ORIENTED_EDGE('',*,*,#44047,.T.);
#58088=ORIENTED_EDGE('',*,*,#44043,.T.);
#58089=ORIENTED_EDGE('',*,*,#44048,.F.);
#58090=ORIENTED_EDGE('',*,*,#44041,.F.);
#58091=ORIENTED_EDGE('',*,*,#44049,.T.);
#58092=ORIENTED_EDGE('',*,*,#44046,.T.);
#58093=ORIENTED_EDGE('',*,*,#44050,.F.);
#58094=ORIENTED_EDGE('',*,*,#44051,.F.);
#58095=ORIENTED_EDGE('',*,*,#44052,.T.);
#58096=ORIENTED_EDGE('',*,*,#44053,.T.);
#58097=ORIENTED_EDGE('',*,*,#44054,.F.);
#58098=ORIENTED_EDGE('',*,*,#44055,.F.);
#58099=ORIENTED_EDGE('',*,*,#44056,.T.);
#58100=ORIENTED_EDGE('',*,*,#44051,.T.);
#58101=ORIENTED_EDGE('',*,*,#44057,.F.);
#58102=ORIENTED_EDGE('',*,*,#44058,.F.);
#58103=ORIENTED_EDGE('',*,*,#44059,.T.);
#58104=ORIENTED_EDGE('',*,*,#44055,.T.);
#58105=ORIENTED_EDGE('',*,*,#44060,.F.);
#58106=ORIENTED_EDGE('',*,*,#44053,.F.);
#58107=ORIENTED_EDGE('',*,*,#44061,.T.);
#58108=ORIENTED_EDGE('',*,*,#44058,.T.);
#58109=ORIENTED_EDGE('',*,*,#44062,.F.);
#58110=ORIENTED_EDGE('',*,*,#44063,.F.);
#58111=ORIENTED_EDGE('',*,*,#44064,.T.);
#58112=ORIENTED_EDGE('',*,*,#44065,.T.);
#58113=ORIENTED_EDGE('',*,*,#44066,.F.);
#58114=ORIENTED_EDGE('',*,*,#44067,.F.);
#58115=ORIENTED_EDGE('',*,*,#44068,.T.);
#58116=ORIENTED_EDGE('',*,*,#44063,.T.);
#58117=ORIENTED_EDGE('',*,*,#44069,.F.);
#58118=ORIENTED_EDGE('',*,*,#44070,.F.);
#58119=ORIENTED_EDGE('',*,*,#44071,.T.);
#58120=ORIENTED_EDGE('',*,*,#44067,.T.);
#58121=ORIENTED_EDGE('',*,*,#44072,.F.);
#58122=ORIENTED_EDGE('',*,*,#44065,.F.);
#58123=ORIENTED_EDGE('',*,*,#44073,.T.);
#58124=ORIENTED_EDGE('',*,*,#44070,.T.);
#58125=ORIENTED_EDGE('',*,*,#44074,.F.);
#58126=ORIENTED_EDGE('',*,*,#44075,.F.);
#58127=ORIENTED_EDGE('',*,*,#44076,.T.);
#58128=ORIENTED_EDGE('',*,*,#44077,.T.);
#58129=ORIENTED_EDGE('',*,*,#44078,.F.);
#58130=ORIENTED_EDGE('',*,*,#44079,.F.);
#58131=ORIENTED_EDGE('',*,*,#44080,.T.);
#58132=ORIENTED_EDGE('',*,*,#44075,.T.);
#58133=ORIENTED_EDGE('',*,*,#44081,.F.);
#58134=ORIENTED_EDGE('',*,*,#44082,.F.);
#58135=ORIENTED_EDGE('',*,*,#44083,.T.);
#58136=ORIENTED_EDGE('',*,*,#44079,.T.);
#58137=ORIENTED_EDGE('',*,*,#44084,.F.);
#58138=ORIENTED_EDGE('',*,*,#44077,.F.);
#58139=ORIENTED_EDGE('',*,*,#44085,.T.);
#58140=ORIENTED_EDGE('',*,*,#44082,.T.);
#58141=ORIENTED_EDGE('',*,*,#44086,.F.);
#58142=ORIENTED_EDGE('',*,*,#44087,.F.);
#58143=ORIENTED_EDGE('',*,*,#44088,.T.);
#58144=ORIENTED_EDGE('',*,*,#44089,.T.);
#58145=ORIENTED_EDGE('',*,*,#44090,.F.);
#58146=ORIENTED_EDGE('',*,*,#44091,.F.);
#58147=ORIENTED_EDGE('',*,*,#44092,.T.);
#58148=ORIENTED_EDGE('',*,*,#44087,.T.);
#58149=ORIENTED_EDGE('',*,*,#44093,.F.);
#58150=ORIENTED_EDGE('',*,*,#44094,.F.);
#58151=ORIENTED_EDGE('',*,*,#44095,.T.);
#58152=ORIENTED_EDGE('',*,*,#44091,.T.);
#58153=ORIENTED_EDGE('',*,*,#44096,.F.);
#58154=ORIENTED_EDGE('',*,*,#44089,.F.);
#58155=ORIENTED_EDGE('',*,*,#44097,.T.);
#58156=ORIENTED_EDGE('',*,*,#44094,.T.);
#58157=ORIENTED_EDGE('',*,*,#44098,.F.);
#58158=ORIENTED_EDGE('',*,*,#44099,.F.);
#58159=ORIENTED_EDGE('',*,*,#44100,.T.);
#58160=ORIENTED_EDGE('',*,*,#44101,.T.);
#58161=ORIENTED_EDGE('',*,*,#44102,.F.);
#58162=ORIENTED_EDGE('',*,*,#44103,.F.);
#58163=ORIENTED_EDGE('',*,*,#44104,.T.);
#58164=ORIENTED_EDGE('',*,*,#44099,.T.);
#58165=ORIENTED_EDGE('',*,*,#44105,.F.);
#58166=ORIENTED_EDGE('',*,*,#44106,.F.);
#58167=ORIENTED_EDGE('',*,*,#44107,.T.);
#58168=ORIENTED_EDGE('',*,*,#44103,.T.);
#58169=ORIENTED_EDGE('',*,*,#44108,.F.);
#58170=ORIENTED_EDGE('',*,*,#44101,.F.);
#58171=ORIENTED_EDGE('',*,*,#44109,.T.);
#58172=ORIENTED_EDGE('',*,*,#44106,.T.);
#58173=ORIENTED_EDGE('',*,*,#44110,.F.);
#58174=ORIENTED_EDGE('',*,*,#44111,.F.);
#58175=ORIENTED_EDGE('',*,*,#44112,.T.);
#58176=ORIENTED_EDGE('',*,*,#44113,.T.);
#58177=ORIENTED_EDGE('',*,*,#44114,.F.);
#58178=ORIENTED_EDGE('',*,*,#44115,.F.);
#58179=ORIENTED_EDGE('',*,*,#44116,.T.);
#58180=ORIENTED_EDGE('',*,*,#44111,.T.);
#58181=ORIENTED_EDGE('',*,*,#44117,.F.);
#58182=ORIENTED_EDGE('',*,*,#44118,.F.);
#58183=ORIENTED_EDGE('',*,*,#44119,.T.);
#58184=ORIENTED_EDGE('',*,*,#44115,.T.);
#58185=ORIENTED_EDGE('',*,*,#44120,.F.);
#58186=ORIENTED_EDGE('',*,*,#44113,.F.);
#58187=ORIENTED_EDGE('',*,*,#44121,.T.);
#58188=ORIENTED_EDGE('',*,*,#44118,.T.);
#58189=ORIENTED_EDGE('',*,*,#44122,.F.);
#58190=ORIENTED_EDGE('',*,*,#44123,.F.);
#58191=ORIENTED_EDGE('',*,*,#44124,.T.);
#58192=ORIENTED_EDGE('',*,*,#44125,.T.);
#58193=ORIENTED_EDGE('',*,*,#44126,.F.);
#58194=ORIENTED_EDGE('',*,*,#44127,.F.);
#58195=ORIENTED_EDGE('',*,*,#44128,.T.);
#58196=ORIENTED_EDGE('',*,*,#44123,.T.);
#58197=ORIENTED_EDGE('',*,*,#44129,.F.);
#58198=ORIENTED_EDGE('',*,*,#44130,.F.);
#58199=ORIENTED_EDGE('',*,*,#44131,.T.);
#58200=ORIENTED_EDGE('',*,*,#44127,.T.);
#58201=ORIENTED_EDGE('',*,*,#44132,.F.);
#58202=ORIENTED_EDGE('',*,*,#44125,.F.);
#58203=ORIENTED_EDGE('',*,*,#44133,.T.);
#58204=ORIENTED_EDGE('',*,*,#44130,.T.);
#58205=ORIENTED_EDGE('',*,*,#44134,.F.);
#58206=ORIENTED_EDGE('',*,*,#44135,.T.);
#58207=ORIENTED_EDGE('',*,*,#44136,.T.);
#58208=ORIENTED_EDGE('',*,*,#44137,.T.);
#58209=ORIENTED_EDGE('',*,*,#44138,.F.);
#58210=ORIENTED_EDGE('',*,*,#44139,.T.);
#58211=ORIENTED_EDGE('',*,*,#44140,.T.);
#58212=ORIENTED_EDGE('',*,*,#44141,.F.);
#58213=ORIENTED_EDGE('',*,*,#44142,.F.);
#58214=ORIENTED_EDGE('',*,*,#44143,.T.);
#58215=ORIENTED_EDGE('',*,*,#44138,.T.);
#58216=ORIENTED_EDGE('',*,*,#44144,.F.);
#58217=ORIENTED_EDGE('',*,*,#44145,.F.);
#58218=ORIENTED_EDGE('',*,*,#44135,.F.);
#58219=ORIENTED_EDGE('',*,*,#44146,.T.);
#58220=ORIENTED_EDGE('',*,*,#44142,.T.);
#58221=ORIENTED_EDGE('',*,*,#44147,.F.);
#58222=ORIENTED_EDGE('',*,*,#44140,.F.);
#58223=ORIENTED_EDGE('',*,*,#44148,.T.);
#58224=ORIENTED_EDGE('',*,*,#44136,.F.);
#58225=ORIENTED_EDGE('',*,*,#44145,.T.);
#58226=ORIENTED_EDGE('',*,*,#44149,.F.);
#58227=ORIENTED_EDGE('',*,*,#44150,.F.);
#58228=ORIENTED_EDGE('',*,*,#44151,.T.);
#58229=ORIENTED_EDGE('',*,*,#44152,.T.);
#58230=ORIENTED_EDGE('',*,*,#44153,.F.);
#58231=ORIENTED_EDGE('',*,*,#44154,.F.);
#58232=ORIENTED_EDGE('',*,*,#44155,.T.);
#58233=ORIENTED_EDGE('',*,*,#44150,.T.);
#58234=ORIENTED_EDGE('',*,*,#44156,.F.);
#58235=ORIENTED_EDGE('',*,*,#44157,.F.);
#58236=ORIENTED_EDGE('',*,*,#44158,.T.);
#58237=ORIENTED_EDGE('',*,*,#44154,.T.);
#58238=ORIENTED_EDGE('',*,*,#44159,.F.);
#58239=ORIENTED_EDGE('',*,*,#44152,.F.);
#58240=ORIENTED_EDGE('',*,*,#44160,.T.);
#58241=ORIENTED_EDGE('',*,*,#44157,.T.);
#58242=ORIENTED_EDGE('',*,*,#44161,.F.);
#58243=ORIENTED_EDGE('',*,*,#44162,.F.);
#58244=ORIENTED_EDGE('',*,*,#44163,.T.);
#58245=ORIENTED_EDGE('',*,*,#44164,.T.);
#58246=ORIENTED_EDGE('',*,*,#44165,.F.);
#58247=ORIENTED_EDGE('',*,*,#44166,.F.);
#58248=ORIENTED_EDGE('',*,*,#44167,.T.);
#58249=ORIENTED_EDGE('',*,*,#44162,.T.);
#58250=ORIENTED_EDGE('',*,*,#44168,.F.);
#58251=ORIENTED_EDGE('',*,*,#44169,.F.);
#58252=ORIENTED_EDGE('',*,*,#44170,.T.);
#58253=ORIENTED_EDGE('',*,*,#44166,.T.);
#58254=ORIENTED_EDGE('',*,*,#44171,.F.);
#58255=ORIENTED_EDGE('',*,*,#44164,.F.);
#58256=ORIENTED_EDGE('',*,*,#44172,.T.);
#58257=ORIENTED_EDGE('',*,*,#44169,.T.);
#58258=ORIENTED_EDGE('',*,*,#44173,.F.);
#58259=ORIENTED_EDGE('',*,*,#44174,.F.);
#58260=ORIENTED_EDGE('',*,*,#44175,.T.);
#58261=ORIENTED_EDGE('',*,*,#44176,.T.);
#58262=ORIENTED_EDGE('',*,*,#44177,.F.);
#58263=ORIENTED_EDGE('',*,*,#44178,.F.);
#58264=ORIENTED_EDGE('',*,*,#44179,.T.);
#58265=ORIENTED_EDGE('',*,*,#44174,.T.);
#58266=ORIENTED_EDGE('',*,*,#44180,.F.);
#58267=ORIENTED_EDGE('',*,*,#44181,.F.);
#58268=ORIENTED_EDGE('',*,*,#44182,.T.);
#58269=ORIENTED_EDGE('',*,*,#44178,.T.);
#58270=ORIENTED_EDGE('',*,*,#44183,.F.);
#58271=ORIENTED_EDGE('',*,*,#44176,.F.);
#58272=ORIENTED_EDGE('',*,*,#44184,.T.);
#58273=ORIENTED_EDGE('',*,*,#44181,.T.);
#58274=ORIENTED_EDGE('',*,*,#44185,.F.);
#58275=ORIENTED_EDGE('',*,*,#44186,.F.);
#58276=ORIENTED_EDGE('',*,*,#44187,.T.);
#58277=ORIENTED_EDGE('',*,*,#44188,.T.);
#58278=ORIENTED_EDGE('',*,*,#44189,.F.);
#58279=ORIENTED_EDGE('',*,*,#44190,.F.);
#58280=ORIENTED_EDGE('',*,*,#44191,.T.);
#58281=ORIENTED_EDGE('',*,*,#44186,.T.);
#58282=ORIENTED_EDGE('',*,*,#44192,.F.);
#58283=ORIENTED_EDGE('',*,*,#44193,.F.);
#58284=ORIENTED_EDGE('',*,*,#44194,.T.);
#58285=ORIENTED_EDGE('',*,*,#44190,.T.);
#58286=ORIENTED_EDGE('',*,*,#44195,.F.);
#58287=ORIENTED_EDGE('',*,*,#44188,.F.);
#58288=ORIENTED_EDGE('',*,*,#44196,.T.);
#58289=ORIENTED_EDGE('',*,*,#44193,.T.);
#58290=ORIENTED_EDGE('',*,*,#44197,.F.);
#58291=ORIENTED_EDGE('',*,*,#44198,.F.);
#58292=ORIENTED_EDGE('',*,*,#44199,.T.);
#58293=ORIENTED_EDGE('',*,*,#44200,.T.);
#58294=ORIENTED_EDGE('',*,*,#44201,.F.);
#58295=ORIENTED_EDGE('',*,*,#44202,.F.);
#58296=ORIENTED_EDGE('',*,*,#44203,.T.);
#58297=ORIENTED_EDGE('',*,*,#44198,.T.);
#58298=ORIENTED_EDGE('',*,*,#44204,.F.);
#58299=ORIENTED_EDGE('',*,*,#44205,.F.);
#58300=ORIENTED_EDGE('',*,*,#44206,.T.);
#58301=ORIENTED_EDGE('',*,*,#44202,.T.);
#58302=ORIENTED_EDGE('',*,*,#44207,.F.);
#58303=ORIENTED_EDGE('',*,*,#44200,.F.);
#58304=ORIENTED_EDGE('',*,*,#44208,.T.);
#58305=ORIENTED_EDGE('',*,*,#44205,.T.);
#58306=ORIENTED_EDGE('',*,*,#44209,.F.);
#58307=ORIENTED_EDGE('',*,*,#44210,.F.);
#58308=ORIENTED_EDGE('',*,*,#44211,.T.);
#58309=ORIENTED_EDGE('',*,*,#44212,.T.);
#58310=ORIENTED_EDGE('',*,*,#44213,.F.);
#58311=ORIENTED_EDGE('',*,*,#44214,.F.);
#58312=ORIENTED_EDGE('',*,*,#44215,.T.);
#58313=ORIENTED_EDGE('',*,*,#44210,.T.);
#58314=ORIENTED_EDGE('',*,*,#44216,.F.);
#58315=ORIENTED_EDGE('',*,*,#44217,.F.);
#58316=ORIENTED_EDGE('',*,*,#44218,.T.);
#58317=ORIENTED_EDGE('',*,*,#44214,.T.);
#58318=ORIENTED_EDGE('',*,*,#44219,.F.);
#58319=ORIENTED_EDGE('',*,*,#44212,.F.);
#58320=ORIENTED_EDGE('',*,*,#44220,.T.);
#58321=ORIENTED_EDGE('',*,*,#44217,.T.);
#58322=ORIENTED_EDGE('',*,*,#44221,.F.);
#58323=ORIENTED_EDGE('',*,*,#44222,.F.);
#58324=ORIENTED_EDGE('',*,*,#44223,.T.);
#58325=ORIENTED_EDGE('',*,*,#44224,.T.);
#58326=ORIENTED_EDGE('',*,*,#44225,.F.);
#58327=ORIENTED_EDGE('',*,*,#44226,.F.);
#58328=ORIENTED_EDGE('',*,*,#44227,.T.);
#58329=ORIENTED_EDGE('',*,*,#44222,.T.);
#58330=ORIENTED_EDGE('',*,*,#44228,.F.);
#58331=ORIENTED_EDGE('',*,*,#44229,.F.);
#58332=ORIENTED_EDGE('',*,*,#44230,.T.);
#58333=ORIENTED_EDGE('',*,*,#44226,.T.);
#58334=ORIENTED_EDGE('',*,*,#44231,.F.);
#58335=ORIENTED_EDGE('',*,*,#44224,.F.);
#58336=ORIENTED_EDGE('',*,*,#44232,.T.);
#58337=ORIENTED_EDGE('',*,*,#44229,.T.);
#58338=ORIENTED_EDGE('',*,*,#44233,.F.);
#58339=ORIENTED_EDGE('',*,*,#44234,.F.);
#58340=ORIENTED_EDGE('',*,*,#44235,.T.);
#58341=ORIENTED_EDGE('',*,*,#44236,.T.);
#58342=ORIENTED_EDGE('',*,*,#44237,.F.);
#58343=ORIENTED_EDGE('',*,*,#44238,.F.);
#58344=ORIENTED_EDGE('',*,*,#44239,.T.);
#58345=ORIENTED_EDGE('',*,*,#44234,.T.);
#58346=ORIENTED_EDGE('',*,*,#44240,.F.);
#58347=ORIENTED_EDGE('',*,*,#44241,.F.);
#58348=ORIENTED_EDGE('',*,*,#44242,.T.);
#58349=ORIENTED_EDGE('',*,*,#44238,.T.);
#58350=ORIENTED_EDGE('',*,*,#44243,.F.);
#58351=ORIENTED_EDGE('',*,*,#44236,.F.);
#58352=ORIENTED_EDGE('',*,*,#44244,.T.);
#58353=ORIENTED_EDGE('',*,*,#44241,.T.);
#58354=ORIENTED_EDGE('',*,*,#44245,.F.);
#58355=ORIENTED_EDGE('',*,*,#44246,.F.);
#58356=ORIENTED_EDGE('',*,*,#44247,.T.);
#58357=ORIENTED_EDGE('',*,*,#44248,.T.);
#58358=ORIENTED_EDGE('',*,*,#44249,.F.);
#58359=ORIENTED_EDGE('',*,*,#44250,.F.);
#58360=ORIENTED_EDGE('',*,*,#44251,.T.);
#58361=ORIENTED_EDGE('',*,*,#44246,.T.);
#58362=ORIENTED_EDGE('',*,*,#44252,.F.);
#58363=ORIENTED_EDGE('',*,*,#44253,.F.);
#58364=ORIENTED_EDGE('',*,*,#44254,.T.);
#58365=ORIENTED_EDGE('',*,*,#44250,.T.);
#58366=ORIENTED_EDGE('',*,*,#44255,.F.);
#58367=ORIENTED_EDGE('',*,*,#44248,.F.);
#58368=ORIENTED_EDGE('',*,*,#44256,.T.);
#58369=ORIENTED_EDGE('',*,*,#44253,.T.);
#58370=ORIENTED_EDGE('',*,*,#44257,.F.);
#58371=ORIENTED_EDGE('',*,*,#44258,.F.);
#58372=ORIENTED_EDGE('',*,*,#44259,.T.);
#58373=ORIENTED_EDGE('',*,*,#44260,.T.);
#58374=ORIENTED_EDGE('',*,*,#44261,.F.);
#58375=ORIENTED_EDGE('',*,*,#44262,.F.);
#58376=ORIENTED_EDGE('',*,*,#44263,.T.);
#58377=ORIENTED_EDGE('',*,*,#44258,.T.);
#58378=ORIENTED_EDGE('',*,*,#44264,.F.);
#58379=ORIENTED_EDGE('',*,*,#44265,.F.);
#58380=ORIENTED_EDGE('',*,*,#44266,.T.);
#58381=ORIENTED_EDGE('',*,*,#44262,.T.);
#58382=ORIENTED_EDGE('',*,*,#44267,.F.);
#58383=ORIENTED_EDGE('',*,*,#44260,.F.);
#58384=ORIENTED_EDGE('',*,*,#44268,.T.);
#58385=ORIENTED_EDGE('',*,*,#44265,.T.);
#58386=ORIENTED_EDGE('',*,*,#44269,.F.);
#58387=ORIENTED_EDGE('',*,*,#44270,.F.);
#58388=ORIENTED_EDGE('',*,*,#44271,.T.);
#58389=ORIENTED_EDGE('',*,*,#44272,.T.);
#58390=ORIENTED_EDGE('',*,*,#44273,.F.);
#58391=ORIENTED_EDGE('',*,*,#44274,.F.);
#58392=ORIENTED_EDGE('',*,*,#44275,.T.);
#58393=ORIENTED_EDGE('',*,*,#44270,.T.);
#58394=ORIENTED_EDGE('',*,*,#44276,.F.);
#58395=ORIENTED_EDGE('',*,*,#44277,.F.);
#58396=ORIENTED_EDGE('',*,*,#44278,.F.);
#58397=ORIENTED_EDGE('',*,*,#44279,.T.);
#58398=ORIENTED_EDGE('',*,*,#44274,.T.);
#58399=ORIENTED_EDGE('',*,*,#44280,.F.);
#58400=ORIENTED_EDGE('',*,*,#44272,.F.);
#58401=ORIENTED_EDGE('',*,*,#44281,.T.);
#58402=ORIENTED_EDGE('',*,*,#44282,.F.);
#58403=ORIENTED_EDGE('',*,*,#44277,.T.);
#58404=ORIENTED_EDGE('',*,*,#44283,.F.);
#58405=ORIENTED_EDGE('',*,*,#44278,.T.);
#58406=ORIENTED_EDGE('',*,*,#44282,.T.);
#58407=ORIENTED_EDGE('',*,*,#44284,.T.);
#58408=ORIENTED_EDGE('',*,*,#44285,.F.);
#58409=ORIENTED_EDGE('',*,*,#44286,.T.);
#58410=ORIENTED_EDGE('',*,*,#44287,.T.);
#58411=ORIENTED_EDGE('',*,*,#44288,.F.);
#58412=ORIENTED_EDGE('',*,*,#44289,.F.);
#58413=ORIENTED_EDGE('',*,*,#44290,.T.);
#58414=ORIENTED_EDGE('',*,*,#44285,.T.);
#58415=ORIENTED_EDGE('',*,*,#44291,.F.);
#58416=ORIENTED_EDGE('',*,*,#44292,.F.);
#58417=ORIENTED_EDGE('',*,*,#44293,.F.);
#58418=ORIENTED_EDGE('',*,*,#44294,.T.);
#58419=ORIENTED_EDGE('',*,*,#44289,.T.);
#58420=ORIENTED_EDGE('',*,*,#44295,.F.);
#58421=ORIENTED_EDGE('',*,*,#44287,.F.);
#58422=ORIENTED_EDGE('',*,*,#44296,.T.);
#58423=ORIENTED_EDGE('',*,*,#44297,.F.);
#58424=ORIENTED_EDGE('',*,*,#44292,.T.);
#58425=ORIENTED_EDGE('',*,*,#44298,.F.);
#58426=ORIENTED_EDGE('',*,*,#44293,.T.);
#58427=ORIENTED_EDGE('',*,*,#44297,.T.);
#58428=ORIENTED_EDGE('',*,*,#44299,.T.);
#58429=ORIENTED_EDGE('',*,*,#44300,.F.);
#58430=ORIENTED_EDGE('',*,*,#44301,.T.);
#58431=ORIENTED_EDGE('',*,*,#44302,.T.);
#58432=ORIENTED_EDGE('',*,*,#44303,.F.);
#58433=ORIENTED_EDGE('',*,*,#44304,.F.);
#58434=ORIENTED_EDGE('',*,*,#44305,.T.);
#58435=ORIENTED_EDGE('',*,*,#44300,.T.);
#58436=ORIENTED_EDGE('',*,*,#44306,.F.);
#58437=ORIENTED_EDGE('',*,*,#44307,.F.);
#58438=ORIENTED_EDGE('',*,*,#44308,.T.);
#58439=ORIENTED_EDGE('',*,*,#44304,.T.);
#58440=ORIENTED_EDGE('',*,*,#44309,.F.);
#58441=ORIENTED_EDGE('',*,*,#44302,.F.);
#58442=ORIENTED_EDGE('',*,*,#44310,.T.);
#58443=ORIENTED_EDGE('',*,*,#44307,.T.);
#58444=ORIENTED_EDGE('',*,*,#44311,.F.);
#58445=ORIENTED_EDGE('',*,*,#44312,.F.);
#58446=ORIENTED_EDGE('',*,*,#44313,.T.);
#58447=ORIENTED_EDGE('',*,*,#44314,.T.);
#58448=ORIENTED_EDGE('',*,*,#44315,.F.);
#58449=ORIENTED_EDGE('',*,*,#44316,.F.);
#58450=ORIENTED_EDGE('',*,*,#44317,.T.);
#58451=ORIENTED_EDGE('',*,*,#44312,.T.);
#58452=ORIENTED_EDGE('',*,*,#44318,.F.);
#58453=ORIENTED_EDGE('',*,*,#44319,.F.);
#58454=ORIENTED_EDGE('',*,*,#44320,.T.);
#58455=ORIENTED_EDGE('',*,*,#44316,.T.);
#58456=ORIENTED_EDGE('',*,*,#44321,.F.);
#58457=ORIENTED_EDGE('',*,*,#44314,.F.);
#58458=ORIENTED_EDGE('',*,*,#44322,.T.);
#58459=ORIENTED_EDGE('',*,*,#44319,.T.);
#58460=ORIENTED_EDGE('',*,*,#44323,.F.);
#58461=ORIENTED_EDGE('',*,*,#44324,.F.);
#58462=ORIENTED_EDGE('',*,*,#44325,.T.);
#58463=ORIENTED_EDGE('',*,*,#44326,.T.);
#58464=ORIENTED_EDGE('',*,*,#44327,.F.);
#58465=ORIENTED_EDGE('',*,*,#44328,.F.);
#58466=ORIENTED_EDGE('',*,*,#44329,.T.);
#58467=ORIENTED_EDGE('',*,*,#44324,.T.);
#58468=ORIENTED_EDGE('',*,*,#44330,.F.);
#58469=ORIENTED_EDGE('',*,*,#44331,.F.);
#58470=ORIENTED_EDGE('',*,*,#44332,.T.);
#58471=ORIENTED_EDGE('',*,*,#44328,.T.);
#58472=ORIENTED_EDGE('',*,*,#44333,.F.);
#58473=ORIENTED_EDGE('',*,*,#44326,.F.);
#58474=ORIENTED_EDGE('',*,*,#44334,.T.);
#58475=ORIENTED_EDGE('',*,*,#44331,.T.);
#58476=ORIENTED_EDGE('',*,*,#44335,.F.);
#58477=ORIENTED_EDGE('',*,*,#44336,.F.);
#58478=ORIENTED_EDGE('',*,*,#44337,.T.);
#58479=ORIENTED_EDGE('',*,*,#44338,.T.);
#58480=ORIENTED_EDGE('',*,*,#44339,.F.);
#58481=ORIENTED_EDGE('',*,*,#44340,.F.);
#58482=ORIENTED_EDGE('',*,*,#44341,.T.);
#58483=ORIENTED_EDGE('',*,*,#44336,.T.);
#58484=ORIENTED_EDGE('',*,*,#44342,.F.);
#58485=ORIENTED_EDGE('',*,*,#44343,.F.);
#58486=ORIENTED_EDGE('',*,*,#44344,.T.);
#58487=ORIENTED_EDGE('',*,*,#44340,.T.);
#58488=ORIENTED_EDGE('',*,*,#44345,.F.);
#58489=ORIENTED_EDGE('',*,*,#44338,.F.);
#58490=ORIENTED_EDGE('',*,*,#44346,.T.);
#58491=ORIENTED_EDGE('',*,*,#44343,.T.);
#58492=ORIENTED_EDGE('',*,*,#44347,.F.);
#58493=ORIENTED_EDGE('',*,*,#44348,.F.);
#58494=ORIENTED_EDGE('',*,*,#44349,.T.);
#58495=ORIENTED_EDGE('',*,*,#44350,.T.);
#58496=ORIENTED_EDGE('',*,*,#44351,.F.);
#58497=ORIENTED_EDGE('',*,*,#44352,.F.);
#58498=ORIENTED_EDGE('',*,*,#44353,.T.);
#58499=ORIENTED_EDGE('',*,*,#44348,.T.);
#58500=ORIENTED_EDGE('',*,*,#44354,.F.);
#58501=ORIENTED_EDGE('',*,*,#44355,.F.);
#58502=ORIENTED_EDGE('',*,*,#44356,.T.);
#58503=ORIENTED_EDGE('',*,*,#44352,.T.);
#58504=ORIENTED_EDGE('',*,*,#44357,.F.);
#58505=ORIENTED_EDGE('',*,*,#44350,.F.);
#58506=ORIENTED_EDGE('',*,*,#44358,.T.);
#58507=ORIENTED_EDGE('',*,*,#44355,.T.);
#58508=ORIENTED_EDGE('',*,*,#44359,.F.);
#58509=ORIENTED_EDGE('',*,*,#44360,.F.);
#58510=ORIENTED_EDGE('',*,*,#44361,.T.);
#58511=ORIENTED_EDGE('',*,*,#44362,.T.);
#58512=ORIENTED_EDGE('',*,*,#44363,.F.);
#58513=ORIENTED_EDGE('',*,*,#44364,.F.);
#58514=ORIENTED_EDGE('',*,*,#44365,.T.);
#58515=ORIENTED_EDGE('',*,*,#44360,.T.);
#58516=ORIENTED_EDGE('',*,*,#44366,.F.);
#58517=ORIENTED_EDGE('',*,*,#44367,.F.);
#58518=ORIENTED_EDGE('',*,*,#44368,.T.);
#58519=ORIENTED_EDGE('',*,*,#44364,.T.);
#58520=ORIENTED_EDGE('',*,*,#44369,.F.);
#58521=ORIENTED_EDGE('',*,*,#44362,.F.);
#58522=ORIENTED_EDGE('',*,*,#44370,.T.);
#58523=ORIENTED_EDGE('',*,*,#44367,.T.);
#58524=ORIENTED_EDGE('',*,*,#44371,.F.);
#58525=ORIENTED_EDGE('',*,*,#44372,.F.);
#58526=ORIENTED_EDGE('',*,*,#44373,.T.);
#58527=ORIENTED_EDGE('',*,*,#44374,.T.);
#58528=ORIENTED_EDGE('',*,*,#44375,.F.);
#58529=ORIENTED_EDGE('',*,*,#44376,.F.);
#58530=ORIENTED_EDGE('',*,*,#44377,.T.);
#58531=ORIENTED_EDGE('',*,*,#44372,.T.);
#58532=ORIENTED_EDGE('',*,*,#44378,.F.);
#58533=ORIENTED_EDGE('',*,*,#44379,.F.);
#58534=ORIENTED_EDGE('',*,*,#44380,.T.);
#58535=ORIENTED_EDGE('',*,*,#44376,.T.);
#58536=ORIENTED_EDGE('',*,*,#44381,.F.);
#58537=ORIENTED_EDGE('',*,*,#44374,.F.);
#58538=ORIENTED_EDGE('',*,*,#44382,.T.);
#58539=ORIENTED_EDGE('',*,*,#44379,.T.);
#58540=ORIENTED_EDGE('',*,*,#44383,.F.);
#58541=ORIENTED_EDGE('',*,*,#44384,.F.);
#58542=ORIENTED_EDGE('',*,*,#44385,.T.);
#58543=ORIENTED_EDGE('',*,*,#44386,.T.);
#58544=ORIENTED_EDGE('',*,*,#44387,.F.);
#58545=ORIENTED_EDGE('',*,*,#44388,.F.);
#58546=ORIENTED_EDGE('',*,*,#44389,.T.);
#58547=ORIENTED_EDGE('',*,*,#44384,.T.);
#58548=ORIENTED_EDGE('',*,*,#44390,.F.);
#58549=ORIENTED_EDGE('',*,*,#44391,.F.);
#58550=ORIENTED_EDGE('',*,*,#44392,.T.);
#58551=ORIENTED_EDGE('',*,*,#44388,.T.);
#58552=ORIENTED_EDGE('',*,*,#44393,.F.);
#58553=ORIENTED_EDGE('',*,*,#44386,.F.);
#58554=ORIENTED_EDGE('',*,*,#44394,.T.);
#58555=ORIENTED_EDGE('',*,*,#44391,.T.);
#58556=ORIENTED_EDGE('',*,*,#44395,.F.);
#58557=ORIENTED_EDGE('',*,*,#44396,.F.);
#58558=ORIENTED_EDGE('',*,*,#44397,.T.);
#58559=ORIENTED_EDGE('',*,*,#44398,.T.);
#58560=ORIENTED_EDGE('',*,*,#44399,.F.);
#58561=ORIENTED_EDGE('',*,*,#44400,.F.);
#58562=ORIENTED_EDGE('',*,*,#44401,.T.);
#58563=ORIENTED_EDGE('',*,*,#44396,.T.);
#58564=ORIENTED_EDGE('',*,*,#44402,.F.);
#58565=ORIENTED_EDGE('',*,*,#44403,.F.);
#58566=ORIENTED_EDGE('',*,*,#44404,.T.);
#58567=ORIENTED_EDGE('',*,*,#44400,.T.);
#58568=ORIENTED_EDGE('',*,*,#44405,.F.);
#58569=ORIENTED_EDGE('',*,*,#44398,.F.);
#58570=ORIENTED_EDGE('',*,*,#44406,.T.);
#58571=ORIENTED_EDGE('',*,*,#44403,.T.);
#58572=ORIENTED_EDGE('',*,*,#44407,.F.);
#58573=ORIENTED_EDGE('',*,*,#44408,.F.);
#58574=ORIENTED_EDGE('',*,*,#44409,.T.);
#58575=ORIENTED_EDGE('',*,*,#44410,.T.);
#58576=ORIENTED_EDGE('',*,*,#44411,.F.);
#58577=ORIENTED_EDGE('',*,*,#44412,.F.);
#58578=ORIENTED_EDGE('',*,*,#44413,.T.);
#58579=ORIENTED_EDGE('',*,*,#44408,.T.);
#58580=ORIENTED_EDGE('',*,*,#44414,.F.);
#58581=ORIENTED_EDGE('',*,*,#44415,.F.);
#58582=ORIENTED_EDGE('',*,*,#44416,.T.);
#58583=ORIENTED_EDGE('',*,*,#44412,.T.);
#58584=ORIENTED_EDGE('',*,*,#44417,.F.);
#58585=ORIENTED_EDGE('',*,*,#44410,.F.);
#58586=ORIENTED_EDGE('',*,*,#44418,.T.);
#58587=ORIENTED_EDGE('',*,*,#44415,.T.);
#58588=ORIENTED_EDGE('',*,*,#44419,.F.);
#58589=ORIENTED_EDGE('',*,*,#44420,.F.);
#58590=ORIENTED_EDGE('',*,*,#44421,.T.);
#58591=ORIENTED_EDGE('',*,*,#44422,.T.);
#58592=ORIENTED_EDGE('',*,*,#44423,.F.);
#58593=ORIENTED_EDGE('',*,*,#44424,.F.);
#58594=ORIENTED_EDGE('',*,*,#44425,.T.);
#58595=ORIENTED_EDGE('',*,*,#44420,.T.);
#58596=ORIENTED_EDGE('',*,*,#44426,.F.);
#58597=ORIENTED_EDGE('',*,*,#44427,.F.);
#58598=ORIENTED_EDGE('',*,*,#44428,.T.);
#58599=ORIENTED_EDGE('',*,*,#44424,.T.);
#58600=ORIENTED_EDGE('',*,*,#44429,.F.);
#58601=ORIENTED_EDGE('',*,*,#44422,.F.);
#58602=ORIENTED_EDGE('',*,*,#44430,.T.);
#58603=ORIENTED_EDGE('',*,*,#44427,.T.);
#58604=ORIENTED_EDGE('',*,*,#44431,.F.);
#58605=ORIENTED_EDGE('',*,*,#44432,.F.);
#58606=ORIENTED_EDGE('',*,*,#44433,.T.);
#58607=ORIENTED_EDGE('',*,*,#44434,.T.);
#58608=ORIENTED_EDGE('',*,*,#44435,.F.);
#58609=ORIENTED_EDGE('',*,*,#44436,.F.);
#58610=ORIENTED_EDGE('',*,*,#44437,.T.);
#58611=ORIENTED_EDGE('',*,*,#44432,.T.);
#58612=ORIENTED_EDGE('',*,*,#44438,.F.);
#58613=ORIENTED_EDGE('',*,*,#44439,.F.);
#58614=ORIENTED_EDGE('',*,*,#44440,.T.);
#58615=ORIENTED_EDGE('',*,*,#44436,.T.);
#58616=ORIENTED_EDGE('',*,*,#44441,.F.);
#58617=ORIENTED_EDGE('',*,*,#44434,.F.);
#58618=ORIENTED_EDGE('',*,*,#44442,.T.);
#58619=ORIENTED_EDGE('',*,*,#44439,.T.);
#58620=ORIENTED_EDGE('',*,*,#44443,.F.);
#58621=ORIENTED_EDGE('',*,*,#44444,.F.);
#58622=ORIENTED_EDGE('',*,*,#44445,.T.);
#58623=ORIENTED_EDGE('',*,*,#44446,.T.);
#58624=ORIENTED_EDGE('',*,*,#44447,.F.);
#58625=ORIENTED_EDGE('',*,*,#44448,.F.);
#58626=ORIENTED_EDGE('',*,*,#44449,.T.);
#58627=ORIENTED_EDGE('',*,*,#44444,.T.);
#58628=ORIENTED_EDGE('',*,*,#44450,.F.);
#58629=ORIENTED_EDGE('',*,*,#44451,.F.);
#58630=ORIENTED_EDGE('',*,*,#44452,.T.);
#58631=ORIENTED_EDGE('',*,*,#44448,.T.);
#58632=ORIENTED_EDGE('',*,*,#44453,.F.);
#58633=ORIENTED_EDGE('',*,*,#44446,.F.);
#58634=ORIENTED_EDGE('',*,*,#44454,.T.);
#58635=ORIENTED_EDGE('',*,*,#44451,.T.);
#58636=ORIENTED_EDGE('',*,*,#44455,.F.);
#58637=ORIENTED_EDGE('',*,*,#44456,.F.);
#58638=ORIENTED_EDGE('',*,*,#44457,.T.);
#58639=ORIENTED_EDGE('',*,*,#44458,.T.);
#58640=ORIENTED_EDGE('',*,*,#44459,.F.);
#58641=ORIENTED_EDGE('',*,*,#44460,.F.);
#58642=ORIENTED_EDGE('',*,*,#44461,.T.);
#58643=ORIENTED_EDGE('',*,*,#44456,.T.);
#58644=ORIENTED_EDGE('',*,*,#44462,.F.);
#58645=ORIENTED_EDGE('',*,*,#44463,.F.);
#58646=ORIENTED_EDGE('',*,*,#44464,.T.);
#58647=ORIENTED_EDGE('',*,*,#44460,.T.);
#58648=ORIENTED_EDGE('',*,*,#44465,.F.);
#58649=ORIENTED_EDGE('',*,*,#44458,.F.);
#58650=ORIENTED_EDGE('',*,*,#44466,.T.);
#58651=ORIENTED_EDGE('',*,*,#44463,.T.);
#58652=ORIENTED_EDGE('',*,*,#44467,.F.);
#58653=ORIENTED_EDGE('',*,*,#44468,.F.);
#58654=ORIENTED_EDGE('',*,*,#44469,.T.);
#58655=ORIENTED_EDGE('',*,*,#44470,.T.);
#58656=ORIENTED_EDGE('',*,*,#44471,.F.);
#58657=ORIENTED_EDGE('',*,*,#44472,.F.);
#58658=ORIENTED_EDGE('',*,*,#44473,.T.);
#58659=ORIENTED_EDGE('',*,*,#44468,.T.);
#58660=ORIENTED_EDGE('',*,*,#44474,.F.);
#58661=ORIENTED_EDGE('',*,*,#44475,.F.);
#58662=ORIENTED_EDGE('',*,*,#44476,.T.);
#58663=ORIENTED_EDGE('',*,*,#44472,.T.);
#58664=ORIENTED_EDGE('',*,*,#44477,.F.);
#58665=ORIENTED_EDGE('',*,*,#44470,.F.);
#58666=ORIENTED_EDGE('',*,*,#44478,.T.);
#58667=ORIENTED_EDGE('',*,*,#44475,.T.);
#58668=ORIENTED_EDGE('',*,*,#44479,.F.);
#58669=ORIENTED_EDGE('',*,*,#44480,.F.);
#58670=ORIENTED_EDGE('',*,*,#44481,.T.);
#58671=ORIENTED_EDGE('',*,*,#44482,.T.);
#58672=ORIENTED_EDGE('',*,*,#44483,.F.);
#58673=ORIENTED_EDGE('',*,*,#44484,.F.);
#58674=ORIENTED_EDGE('',*,*,#44485,.T.);
#58675=ORIENTED_EDGE('',*,*,#44480,.T.);
#58676=ORIENTED_EDGE('',*,*,#44486,.F.);
#58677=ORIENTED_EDGE('',*,*,#44487,.F.);
#58678=ORIENTED_EDGE('',*,*,#44488,.T.);
#58679=ORIENTED_EDGE('',*,*,#44484,.T.);
#58680=ORIENTED_EDGE('',*,*,#44489,.F.);
#58681=ORIENTED_EDGE('',*,*,#44482,.F.);
#58682=ORIENTED_EDGE('',*,*,#44490,.T.);
#58683=ORIENTED_EDGE('',*,*,#44487,.T.);
#58684=ORIENTED_EDGE('',*,*,#44491,.F.);
#58685=ORIENTED_EDGE('',*,*,#44492,.F.);
#58686=ORIENTED_EDGE('',*,*,#44493,.T.);
#58687=ORIENTED_EDGE('',*,*,#44494,.T.);
#58688=ORIENTED_EDGE('',*,*,#44495,.F.);
#58689=ORIENTED_EDGE('',*,*,#44496,.F.);
#58690=ORIENTED_EDGE('',*,*,#44497,.T.);
#58691=ORIENTED_EDGE('',*,*,#44492,.T.);
#58692=ORIENTED_EDGE('',*,*,#44498,.F.);
#58693=ORIENTED_EDGE('',*,*,#44499,.F.);
#58694=ORIENTED_EDGE('',*,*,#44500,.T.);
#58695=ORIENTED_EDGE('',*,*,#44496,.T.);
#58696=ORIENTED_EDGE('',*,*,#44501,.F.);
#58697=ORIENTED_EDGE('',*,*,#44494,.F.);
#58698=ORIENTED_EDGE('',*,*,#44502,.T.);
#58699=ORIENTED_EDGE('',*,*,#44499,.T.);
#58700=ORIENTED_EDGE('',*,*,#44503,.F.);
#58701=ORIENTED_EDGE('',*,*,#44504,.F.);
#58702=ORIENTED_EDGE('',*,*,#44505,.T.);
#58703=ORIENTED_EDGE('',*,*,#44506,.T.);
#58704=ORIENTED_EDGE('',*,*,#44507,.F.);
#58705=ORIENTED_EDGE('',*,*,#44508,.F.);
#58706=ORIENTED_EDGE('',*,*,#44509,.T.);
#58707=ORIENTED_EDGE('',*,*,#44504,.T.);
#58708=ORIENTED_EDGE('',*,*,#44510,.F.);
#58709=ORIENTED_EDGE('',*,*,#44511,.F.);
#58710=ORIENTED_EDGE('',*,*,#44512,.T.);
#58711=ORIENTED_EDGE('',*,*,#44508,.T.);
#58712=ORIENTED_EDGE('',*,*,#44513,.F.);
#58713=ORIENTED_EDGE('',*,*,#44506,.F.);
#58714=ORIENTED_EDGE('',*,*,#44514,.T.);
#58715=ORIENTED_EDGE('',*,*,#44511,.T.);
#58716=ORIENTED_EDGE('',*,*,#44515,.F.);
#58717=ORIENTED_EDGE('',*,*,#44516,.F.);
#58718=ORIENTED_EDGE('',*,*,#44517,.T.);
#58719=ORIENTED_EDGE('',*,*,#44518,.T.);
#58720=ORIENTED_EDGE('',*,*,#44519,.F.);
#58721=ORIENTED_EDGE('',*,*,#44520,.F.);
#58722=ORIENTED_EDGE('',*,*,#44521,.T.);
#58723=ORIENTED_EDGE('',*,*,#44516,.T.);
#58724=ORIENTED_EDGE('',*,*,#44522,.F.);
#58725=ORIENTED_EDGE('',*,*,#44523,.F.);
#58726=ORIENTED_EDGE('',*,*,#44524,.T.);
#58727=ORIENTED_EDGE('',*,*,#44520,.T.);
#58728=ORIENTED_EDGE('',*,*,#44525,.F.);
#58729=ORIENTED_EDGE('',*,*,#44518,.F.);
#58730=ORIENTED_EDGE('',*,*,#44526,.T.);
#58731=ORIENTED_EDGE('',*,*,#44523,.T.);
#58732=ORIENTED_EDGE('',*,*,#44527,.F.);
#58733=ORIENTED_EDGE('',*,*,#44528,.F.);
#58734=ORIENTED_EDGE('',*,*,#44529,.T.);
#58735=ORIENTED_EDGE('',*,*,#44530,.T.);
#58736=ORIENTED_EDGE('',*,*,#44531,.F.);
#58737=ORIENTED_EDGE('',*,*,#44532,.F.);
#58738=ORIENTED_EDGE('',*,*,#44533,.T.);
#58739=ORIENTED_EDGE('',*,*,#44528,.T.);
#58740=ORIENTED_EDGE('',*,*,#44534,.F.);
#58741=ORIENTED_EDGE('',*,*,#44535,.F.);
#58742=ORIENTED_EDGE('',*,*,#44536,.T.);
#58743=ORIENTED_EDGE('',*,*,#44532,.T.);
#58744=ORIENTED_EDGE('',*,*,#44537,.F.);
#58745=ORIENTED_EDGE('',*,*,#44530,.F.);
#58746=ORIENTED_EDGE('',*,*,#44538,.T.);
#58747=ORIENTED_EDGE('',*,*,#44535,.T.);
#58748=ORIENTED_EDGE('',*,*,#44539,.F.);
#58749=ORIENTED_EDGE('',*,*,#44540,.F.);
#58750=ORIENTED_EDGE('',*,*,#44541,.T.);
#58751=ORIENTED_EDGE('',*,*,#44542,.T.);
#58752=ORIENTED_EDGE('',*,*,#44543,.F.);
#58753=ORIENTED_EDGE('',*,*,#44544,.F.);
#58754=ORIENTED_EDGE('',*,*,#44545,.T.);
#58755=ORIENTED_EDGE('',*,*,#44540,.T.);
#58756=ORIENTED_EDGE('',*,*,#44546,.F.);
#58757=ORIENTED_EDGE('',*,*,#44547,.F.);
#58758=ORIENTED_EDGE('',*,*,#44548,.T.);
#58759=ORIENTED_EDGE('',*,*,#44544,.T.);
#58760=ORIENTED_EDGE('',*,*,#44549,.F.);
#58761=ORIENTED_EDGE('',*,*,#44542,.F.);
#58762=ORIENTED_EDGE('',*,*,#44550,.T.);
#58763=ORIENTED_EDGE('',*,*,#44547,.T.);
#58764=ORIENTED_EDGE('',*,*,#44551,.F.);
#58765=ORIENTED_EDGE('',*,*,#44552,.F.);
#58766=ORIENTED_EDGE('',*,*,#44553,.T.);
#58767=ORIENTED_EDGE('',*,*,#44554,.T.);
#58768=ORIENTED_EDGE('',*,*,#44555,.F.);
#58769=ORIENTED_EDGE('',*,*,#44556,.F.);
#58770=ORIENTED_EDGE('',*,*,#44557,.T.);
#58771=ORIENTED_EDGE('',*,*,#44552,.T.);
#58772=ORIENTED_EDGE('',*,*,#44558,.F.);
#58773=ORIENTED_EDGE('',*,*,#44559,.F.);
#58774=ORIENTED_EDGE('',*,*,#44560,.T.);
#58775=ORIENTED_EDGE('',*,*,#44556,.T.);
#58776=ORIENTED_EDGE('',*,*,#44561,.F.);
#58777=ORIENTED_EDGE('',*,*,#44554,.F.);
#58778=ORIENTED_EDGE('',*,*,#44562,.T.);
#58779=ORIENTED_EDGE('',*,*,#44559,.T.);
#58780=ORIENTED_EDGE('',*,*,#44563,.F.);
#58781=ORIENTED_EDGE('',*,*,#44564,.F.);
#58782=ORIENTED_EDGE('',*,*,#44565,.T.);
#58783=ORIENTED_EDGE('',*,*,#44566,.T.);
#58784=ORIENTED_EDGE('',*,*,#44567,.F.);
#58785=ORIENTED_EDGE('',*,*,#44568,.F.);
#58786=ORIENTED_EDGE('',*,*,#44569,.T.);
#58787=ORIENTED_EDGE('',*,*,#44564,.T.);
#58788=ORIENTED_EDGE('',*,*,#44570,.F.);
#58789=ORIENTED_EDGE('',*,*,#44571,.F.);
#58790=ORIENTED_EDGE('',*,*,#44572,.T.);
#58791=ORIENTED_EDGE('',*,*,#44568,.T.);
#58792=ORIENTED_EDGE('',*,*,#44573,.F.);
#58793=ORIENTED_EDGE('',*,*,#44566,.F.);
#58794=ORIENTED_EDGE('',*,*,#44574,.T.);
#58795=ORIENTED_EDGE('',*,*,#44571,.T.);
#58796=ORIENTED_EDGE('',*,*,#44575,.F.);
#58797=ORIENTED_EDGE('',*,*,#44576,.F.);
#58798=ORIENTED_EDGE('',*,*,#44577,.T.);
#58799=ORIENTED_EDGE('',*,*,#44578,.T.);
#58800=ORIENTED_EDGE('',*,*,#44579,.F.);
#58801=ORIENTED_EDGE('',*,*,#44580,.F.);
#58802=ORIENTED_EDGE('',*,*,#44581,.T.);
#58803=ORIENTED_EDGE('',*,*,#44576,.T.);
#58804=ORIENTED_EDGE('',*,*,#44582,.F.);
#58805=ORIENTED_EDGE('',*,*,#44583,.F.);
#58806=ORIENTED_EDGE('',*,*,#44584,.T.);
#58807=ORIENTED_EDGE('',*,*,#44580,.T.);
#58808=ORIENTED_EDGE('',*,*,#44585,.F.);
#58809=ORIENTED_EDGE('',*,*,#44578,.F.);
#58810=ORIENTED_EDGE('',*,*,#44586,.T.);
#58811=ORIENTED_EDGE('',*,*,#44583,.T.);
#58812=ORIENTED_EDGE('',*,*,#44587,.F.);
#58813=ORIENTED_EDGE('',*,*,#44588,.F.);
#58814=ORIENTED_EDGE('',*,*,#44589,.T.);
#58815=ORIENTED_EDGE('',*,*,#44590,.T.);
#58816=ORIENTED_EDGE('',*,*,#44591,.F.);
#58817=ORIENTED_EDGE('',*,*,#44592,.F.);
#58818=ORIENTED_EDGE('',*,*,#44593,.T.);
#58819=ORIENTED_EDGE('',*,*,#44588,.T.);
#58820=ORIENTED_EDGE('',*,*,#44594,.F.);
#58821=ORIENTED_EDGE('',*,*,#44595,.F.);
#58822=ORIENTED_EDGE('',*,*,#44596,.T.);
#58823=ORIENTED_EDGE('',*,*,#44592,.T.);
#58824=ORIENTED_EDGE('',*,*,#44597,.F.);
#58825=ORIENTED_EDGE('',*,*,#44590,.F.);
#58826=ORIENTED_EDGE('',*,*,#44598,.T.);
#58827=ORIENTED_EDGE('',*,*,#44595,.T.);
#58828=ORIENTED_EDGE('',*,*,#44599,.F.);
#58829=ORIENTED_EDGE('',*,*,#44600,.F.);
#58830=ORIENTED_EDGE('',*,*,#44601,.T.);
#58831=ORIENTED_EDGE('',*,*,#44602,.T.);
#58832=ORIENTED_EDGE('',*,*,#44603,.F.);
#58833=ORIENTED_EDGE('',*,*,#44604,.F.);
#58834=ORIENTED_EDGE('',*,*,#44605,.T.);
#58835=ORIENTED_EDGE('',*,*,#44600,.T.);
#58836=ORIENTED_EDGE('',*,*,#44606,.F.);
#58837=ORIENTED_EDGE('',*,*,#44607,.F.);
#58838=ORIENTED_EDGE('',*,*,#44608,.T.);
#58839=ORIENTED_EDGE('',*,*,#44604,.T.);
#58840=ORIENTED_EDGE('',*,*,#44609,.F.);
#58841=ORIENTED_EDGE('',*,*,#44602,.F.);
#58842=ORIENTED_EDGE('',*,*,#44610,.T.);
#58843=ORIENTED_EDGE('',*,*,#44607,.T.);
#58844=ORIENTED_EDGE('',*,*,#44611,.F.);
#58845=ORIENTED_EDGE('',*,*,#44612,.F.);
#58846=ORIENTED_EDGE('',*,*,#44613,.T.);
#58847=ORIENTED_EDGE('',*,*,#44614,.T.);
#58848=ORIENTED_EDGE('',*,*,#44615,.F.);
#58849=ORIENTED_EDGE('',*,*,#44616,.F.);
#58850=ORIENTED_EDGE('',*,*,#44617,.T.);
#58851=ORIENTED_EDGE('',*,*,#44612,.T.);
#58852=ORIENTED_EDGE('',*,*,#44618,.F.);
#58853=ORIENTED_EDGE('',*,*,#44619,.F.);
#58854=ORIENTED_EDGE('',*,*,#44620,.T.);
#58855=ORIENTED_EDGE('',*,*,#44616,.T.);
#58856=ORIENTED_EDGE('',*,*,#44621,.F.);
#58857=ORIENTED_EDGE('',*,*,#44614,.F.);
#58858=ORIENTED_EDGE('',*,*,#44622,.T.);
#58859=ORIENTED_EDGE('',*,*,#44619,.T.);
#58860=ORIENTED_EDGE('',*,*,#44623,.F.);
#58861=ORIENTED_EDGE('',*,*,#44624,.F.);
#58862=ORIENTED_EDGE('',*,*,#44625,.T.);
#58863=ORIENTED_EDGE('',*,*,#44626,.T.);
#58864=ORIENTED_EDGE('',*,*,#44627,.F.);
#58865=ORIENTED_EDGE('',*,*,#44628,.F.);
#58866=ORIENTED_EDGE('',*,*,#44629,.T.);
#58867=ORIENTED_EDGE('',*,*,#44624,.T.);
#58868=ORIENTED_EDGE('',*,*,#44630,.F.);
#58869=ORIENTED_EDGE('',*,*,#44631,.F.);
#58870=ORIENTED_EDGE('',*,*,#44632,.T.);
#58871=ORIENTED_EDGE('',*,*,#44628,.T.);
#58872=ORIENTED_EDGE('',*,*,#44633,.F.);
#58873=ORIENTED_EDGE('',*,*,#44626,.F.);
#58874=ORIENTED_EDGE('',*,*,#44634,.T.);
#58875=ORIENTED_EDGE('',*,*,#44631,.T.);
#58876=ORIENTED_EDGE('',*,*,#44635,.F.);
#58877=ORIENTED_EDGE('',*,*,#44636,.F.);
#58878=ORIENTED_EDGE('',*,*,#44637,.T.);
#58879=ORIENTED_EDGE('',*,*,#44638,.T.);
#58880=ORIENTED_EDGE('',*,*,#44639,.F.);
#58881=ORIENTED_EDGE('',*,*,#44640,.F.);
#58882=ORIENTED_EDGE('',*,*,#44641,.T.);
#58883=ORIENTED_EDGE('',*,*,#44636,.T.);
#58884=ORIENTED_EDGE('',*,*,#44642,.F.);
#58885=ORIENTED_EDGE('',*,*,#44643,.F.);
#58886=ORIENTED_EDGE('',*,*,#44644,.T.);
#58887=ORIENTED_EDGE('',*,*,#44640,.T.);
#58888=ORIENTED_EDGE('',*,*,#44645,.F.);
#58889=ORIENTED_EDGE('',*,*,#44638,.F.);
#58890=ORIENTED_EDGE('',*,*,#44646,.T.);
#58891=ORIENTED_EDGE('',*,*,#44643,.T.);
#58892=ORIENTED_EDGE('',*,*,#44647,.F.);
#58893=ORIENTED_EDGE('',*,*,#44648,.F.);
#58894=ORIENTED_EDGE('',*,*,#44649,.T.);
#58895=ORIENTED_EDGE('',*,*,#44650,.T.);
#58896=ORIENTED_EDGE('',*,*,#44651,.F.);
#58897=ORIENTED_EDGE('',*,*,#44652,.F.);
#58898=ORIENTED_EDGE('',*,*,#44653,.T.);
#58899=ORIENTED_EDGE('',*,*,#44648,.T.);
#58900=ORIENTED_EDGE('',*,*,#44654,.F.);
#58901=ORIENTED_EDGE('',*,*,#44655,.F.);
#58902=ORIENTED_EDGE('',*,*,#44656,.T.);
#58903=ORIENTED_EDGE('',*,*,#44652,.T.);
#58904=ORIENTED_EDGE('',*,*,#44657,.F.);
#58905=ORIENTED_EDGE('',*,*,#44650,.F.);
#58906=ORIENTED_EDGE('',*,*,#44658,.T.);
#58907=ORIENTED_EDGE('',*,*,#44655,.T.);
#58908=ORIENTED_EDGE('',*,*,#44659,.F.);
#58909=ORIENTED_EDGE('',*,*,#44660,.F.);
#58910=ORIENTED_EDGE('',*,*,#44661,.T.);
#58911=ORIENTED_EDGE('',*,*,#44662,.T.);
#58912=ORIENTED_EDGE('',*,*,#44663,.F.);
#58913=ORIENTED_EDGE('',*,*,#44664,.F.);
#58914=ORIENTED_EDGE('',*,*,#44665,.T.);
#58915=ORIENTED_EDGE('',*,*,#44660,.T.);
#58916=ORIENTED_EDGE('',*,*,#44666,.F.);
#58917=ORIENTED_EDGE('',*,*,#44667,.F.);
#58918=ORIENTED_EDGE('',*,*,#44668,.T.);
#58919=ORIENTED_EDGE('',*,*,#44664,.T.);
#58920=ORIENTED_EDGE('',*,*,#44669,.F.);
#58921=ORIENTED_EDGE('',*,*,#44662,.F.);
#58922=ORIENTED_EDGE('',*,*,#44670,.T.);
#58923=ORIENTED_EDGE('',*,*,#44667,.T.);
#58924=ORIENTED_EDGE('',*,*,#44671,.F.);
#58925=ORIENTED_EDGE('',*,*,#44672,.F.);
#58926=ORIENTED_EDGE('',*,*,#44673,.T.);
#58927=ORIENTED_EDGE('',*,*,#44674,.T.);
#58928=ORIENTED_EDGE('',*,*,#44675,.F.);
#58929=ORIENTED_EDGE('',*,*,#44676,.F.);
#58930=ORIENTED_EDGE('',*,*,#44677,.T.);
#58931=ORIENTED_EDGE('',*,*,#44672,.T.);
#58932=ORIENTED_EDGE('',*,*,#44678,.F.);
#58933=ORIENTED_EDGE('',*,*,#44679,.F.);
#58934=ORIENTED_EDGE('',*,*,#44680,.T.);
#58935=ORIENTED_EDGE('',*,*,#44676,.T.);
#58936=ORIENTED_EDGE('',*,*,#44681,.F.);
#58937=ORIENTED_EDGE('',*,*,#44674,.F.);
#58938=ORIENTED_EDGE('',*,*,#44682,.T.);
#58939=ORIENTED_EDGE('',*,*,#44679,.T.);
#58940=ORIENTED_EDGE('',*,*,#44683,.F.);
#58941=ORIENTED_EDGE('',*,*,#44684,.F.);
#58942=ORIENTED_EDGE('',*,*,#44685,.T.);
#58943=ORIENTED_EDGE('',*,*,#44686,.T.);
#58944=ORIENTED_EDGE('',*,*,#44687,.F.);
#58945=ORIENTED_EDGE('',*,*,#44688,.F.);
#58946=ORIENTED_EDGE('',*,*,#44689,.T.);
#58947=ORIENTED_EDGE('',*,*,#44684,.T.);
#58948=ORIENTED_EDGE('',*,*,#44690,.F.);
#58949=ORIENTED_EDGE('',*,*,#44691,.F.);
#58950=ORIENTED_EDGE('',*,*,#44692,.T.);
#58951=ORIENTED_EDGE('',*,*,#44688,.T.);
#58952=ORIENTED_EDGE('',*,*,#44693,.F.);
#58953=ORIENTED_EDGE('',*,*,#44686,.F.);
#58954=ORIENTED_EDGE('',*,*,#44694,.T.);
#58955=ORIENTED_EDGE('',*,*,#44691,.T.);
#58956=ORIENTED_EDGE('',*,*,#44695,.F.);
#58957=ORIENTED_EDGE('',*,*,#44696,.F.);
#58958=ORIENTED_EDGE('',*,*,#44697,.T.);
#58959=ORIENTED_EDGE('',*,*,#44698,.T.);
#58960=ORIENTED_EDGE('',*,*,#44699,.F.);
#58961=ORIENTED_EDGE('',*,*,#44700,.F.);
#58962=ORIENTED_EDGE('',*,*,#44701,.T.);
#58963=ORIENTED_EDGE('',*,*,#44696,.T.);
#58964=ORIENTED_EDGE('',*,*,#44702,.F.);
#58965=ORIENTED_EDGE('',*,*,#44703,.F.);
#58966=ORIENTED_EDGE('',*,*,#44704,.T.);
#58967=ORIENTED_EDGE('',*,*,#44700,.T.);
#58968=ORIENTED_EDGE('',*,*,#44705,.F.);
#58969=ORIENTED_EDGE('',*,*,#44698,.F.);
#58970=ORIENTED_EDGE('',*,*,#44706,.T.);
#58971=ORIENTED_EDGE('',*,*,#44703,.T.);
#58972=ORIENTED_EDGE('',*,*,#44707,.F.);
#58973=ORIENTED_EDGE('',*,*,#44708,.F.);
#58974=ORIENTED_EDGE('',*,*,#44709,.T.);
#58975=ORIENTED_EDGE('',*,*,#44710,.T.);
#58976=ORIENTED_EDGE('',*,*,#44711,.F.);
#58977=ORIENTED_EDGE('',*,*,#44712,.F.);
#58978=ORIENTED_EDGE('',*,*,#44713,.T.);
#58979=ORIENTED_EDGE('',*,*,#44708,.T.);
#58980=ORIENTED_EDGE('',*,*,#44714,.F.);
#58981=ORIENTED_EDGE('',*,*,#44715,.F.);
#58982=ORIENTED_EDGE('',*,*,#44716,.T.);
#58983=ORIENTED_EDGE('',*,*,#44712,.T.);
#58984=ORIENTED_EDGE('',*,*,#44717,.F.);
#58985=ORIENTED_EDGE('',*,*,#44710,.F.);
#58986=ORIENTED_EDGE('',*,*,#44718,.T.);
#58987=ORIENTED_EDGE('',*,*,#44715,.T.);
#58988=ORIENTED_EDGE('',*,*,#44719,.F.);
#58989=ORIENTED_EDGE('',*,*,#44720,.F.);
#58990=ORIENTED_EDGE('',*,*,#44721,.T.);
#58991=ORIENTED_EDGE('',*,*,#44722,.T.);
#58992=ORIENTED_EDGE('',*,*,#44723,.F.);
#58993=ORIENTED_EDGE('',*,*,#44724,.F.);
#58994=ORIENTED_EDGE('',*,*,#44725,.T.);
#58995=ORIENTED_EDGE('',*,*,#44720,.T.);
#58996=ORIENTED_EDGE('',*,*,#44726,.F.);
#58997=ORIENTED_EDGE('',*,*,#44727,.F.);
#58998=ORIENTED_EDGE('',*,*,#44728,.T.);
#58999=ORIENTED_EDGE('',*,*,#44724,.T.);
#59000=ORIENTED_EDGE('',*,*,#44729,.F.);
#59001=ORIENTED_EDGE('',*,*,#44722,.F.);
#59002=ORIENTED_EDGE('',*,*,#44730,.T.);
#59003=ORIENTED_EDGE('',*,*,#44727,.T.);
#59004=ORIENTED_EDGE('',*,*,#44731,.F.);
#59005=ORIENTED_EDGE('',*,*,#44732,.F.);
#59006=ORIENTED_EDGE('',*,*,#44733,.T.);
#59007=ORIENTED_EDGE('',*,*,#44734,.T.);
#59008=ORIENTED_EDGE('',*,*,#44735,.F.);
#59009=ORIENTED_EDGE('',*,*,#44736,.F.);
#59010=ORIENTED_EDGE('',*,*,#44737,.T.);
#59011=ORIENTED_EDGE('',*,*,#44732,.T.);
#59012=ORIENTED_EDGE('',*,*,#44738,.F.);
#59013=ORIENTED_EDGE('',*,*,#44739,.F.);
#59014=ORIENTED_EDGE('',*,*,#44740,.T.);
#59015=ORIENTED_EDGE('',*,*,#44736,.T.);
#59016=ORIENTED_EDGE('',*,*,#44741,.F.);
#59017=ORIENTED_EDGE('',*,*,#44734,.F.);
#59018=ORIENTED_EDGE('',*,*,#44742,.T.);
#59019=ORIENTED_EDGE('',*,*,#44739,.T.);
#59020=ORIENTED_EDGE('',*,*,#44743,.F.);
#59021=ORIENTED_EDGE('',*,*,#44744,.F.);
#59022=ORIENTED_EDGE('',*,*,#44745,.T.);
#59023=ORIENTED_EDGE('',*,*,#44746,.T.);
#59024=ORIENTED_EDGE('',*,*,#44747,.F.);
#59025=ORIENTED_EDGE('',*,*,#44748,.F.);
#59026=ORIENTED_EDGE('',*,*,#44749,.T.);
#59027=ORIENTED_EDGE('',*,*,#44744,.T.);
#59028=ORIENTED_EDGE('',*,*,#44750,.F.);
#59029=ORIENTED_EDGE('',*,*,#44751,.F.);
#59030=ORIENTED_EDGE('',*,*,#44752,.T.);
#59031=ORIENTED_EDGE('',*,*,#44748,.T.);
#59032=ORIENTED_EDGE('',*,*,#44753,.F.);
#59033=ORIENTED_EDGE('',*,*,#44746,.F.);
#59034=ORIENTED_EDGE('',*,*,#44754,.T.);
#59035=ORIENTED_EDGE('',*,*,#44751,.T.);
#59036=ORIENTED_EDGE('',*,*,#44755,.F.);
#59037=ORIENTED_EDGE('',*,*,#44756,.F.);
#59038=ORIENTED_EDGE('',*,*,#44757,.T.);
#59039=ORIENTED_EDGE('',*,*,#44758,.T.);
#59040=ORIENTED_EDGE('',*,*,#44759,.F.);
#59041=ORIENTED_EDGE('',*,*,#44760,.F.);
#59042=ORIENTED_EDGE('',*,*,#44761,.T.);
#59043=ORIENTED_EDGE('',*,*,#44756,.T.);
#59044=ORIENTED_EDGE('',*,*,#44762,.F.);
#59045=ORIENTED_EDGE('',*,*,#44763,.F.);
#59046=ORIENTED_EDGE('',*,*,#44764,.T.);
#59047=ORIENTED_EDGE('',*,*,#44760,.T.);
#59048=ORIENTED_EDGE('',*,*,#44765,.F.);
#59049=ORIENTED_EDGE('',*,*,#44758,.F.);
#59050=ORIENTED_EDGE('',*,*,#44766,.T.);
#59051=ORIENTED_EDGE('',*,*,#44763,.T.);
#59052=ORIENTED_EDGE('',*,*,#44767,.F.);
#59053=ORIENTED_EDGE('',*,*,#44768,.F.);
#59054=ORIENTED_EDGE('',*,*,#44769,.T.);
#59055=ORIENTED_EDGE('',*,*,#44770,.T.);
#59056=ORIENTED_EDGE('',*,*,#44771,.F.);
#59057=ORIENTED_EDGE('',*,*,#44772,.F.);
#59058=ORIENTED_EDGE('',*,*,#44773,.T.);
#59059=ORIENTED_EDGE('',*,*,#44768,.T.);
#59060=ORIENTED_EDGE('',*,*,#44774,.F.);
#59061=ORIENTED_EDGE('',*,*,#44775,.F.);
#59062=ORIENTED_EDGE('',*,*,#44776,.T.);
#59063=ORIENTED_EDGE('',*,*,#44772,.T.);
#59064=ORIENTED_EDGE('',*,*,#44777,.F.);
#59065=ORIENTED_EDGE('',*,*,#44770,.F.);
#59066=ORIENTED_EDGE('',*,*,#44778,.T.);
#59067=ORIENTED_EDGE('',*,*,#44775,.T.);
#59068=ORIENTED_EDGE('',*,*,#44779,.F.);
#59069=ORIENTED_EDGE('',*,*,#44780,.F.);
#59070=ORIENTED_EDGE('',*,*,#44781,.T.);
#59071=ORIENTED_EDGE('',*,*,#44782,.T.);
#59072=ORIENTED_EDGE('',*,*,#44783,.F.);
#59073=ORIENTED_EDGE('',*,*,#44784,.F.);
#59074=ORIENTED_EDGE('',*,*,#44785,.T.);
#59075=ORIENTED_EDGE('',*,*,#44780,.T.);
#59076=ORIENTED_EDGE('',*,*,#44786,.F.);
#59077=ORIENTED_EDGE('',*,*,#44787,.F.);
#59078=ORIENTED_EDGE('',*,*,#44788,.T.);
#59079=ORIENTED_EDGE('',*,*,#44784,.T.);
#59080=ORIENTED_EDGE('',*,*,#44789,.F.);
#59081=ORIENTED_EDGE('',*,*,#44782,.F.);
#59082=ORIENTED_EDGE('',*,*,#44790,.T.);
#59083=ORIENTED_EDGE('',*,*,#44787,.T.);
#59084=ORIENTED_EDGE('',*,*,#44791,.F.);
#59085=ORIENTED_EDGE('',*,*,#44792,.F.);
#59086=ORIENTED_EDGE('',*,*,#44793,.T.);
#59087=ORIENTED_EDGE('',*,*,#44794,.T.);
#59088=ORIENTED_EDGE('',*,*,#44795,.F.);
#59089=ORIENTED_EDGE('',*,*,#44796,.F.);
#59090=ORIENTED_EDGE('',*,*,#44797,.T.);
#59091=ORIENTED_EDGE('',*,*,#44792,.T.);
#59092=ORIENTED_EDGE('',*,*,#44798,.F.);
#59093=ORIENTED_EDGE('',*,*,#44799,.F.);
#59094=ORIENTED_EDGE('',*,*,#44800,.T.);
#59095=ORIENTED_EDGE('',*,*,#44796,.T.);
#59096=ORIENTED_EDGE('',*,*,#44801,.F.);
#59097=ORIENTED_EDGE('',*,*,#44794,.F.);
#59098=ORIENTED_EDGE('',*,*,#44802,.T.);
#59099=ORIENTED_EDGE('',*,*,#44799,.T.);
#59100=ORIENTED_EDGE('',*,*,#44803,.F.);
#59101=ORIENTED_EDGE('',*,*,#44804,.F.);
#59102=ORIENTED_EDGE('',*,*,#44805,.T.);
#59103=ORIENTED_EDGE('',*,*,#44806,.T.);
#59104=ORIENTED_EDGE('',*,*,#44807,.F.);
#59105=ORIENTED_EDGE('',*,*,#44808,.F.);
#59106=ORIENTED_EDGE('',*,*,#44809,.T.);
#59107=ORIENTED_EDGE('',*,*,#44804,.T.);
#59108=ORIENTED_EDGE('',*,*,#44810,.F.);
#59109=ORIENTED_EDGE('',*,*,#44811,.F.);
#59110=ORIENTED_EDGE('',*,*,#44812,.T.);
#59111=ORIENTED_EDGE('',*,*,#44808,.T.);
#59112=ORIENTED_EDGE('',*,*,#44813,.F.);
#59113=ORIENTED_EDGE('',*,*,#44806,.F.);
#59114=ORIENTED_EDGE('',*,*,#44814,.T.);
#59115=ORIENTED_EDGE('',*,*,#44811,.T.);
#59116=ORIENTED_EDGE('',*,*,#44815,.F.);
#59117=ORIENTED_EDGE('',*,*,#44816,.F.);
#59118=ORIENTED_EDGE('',*,*,#44817,.T.);
#59119=ORIENTED_EDGE('',*,*,#44818,.T.);
#59120=ORIENTED_EDGE('',*,*,#44819,.F.);
#59121=ORIENTED_EDGE('',*,*,#44820,.F.);
#59122=ORIENTED_EDGE('',*,*,#44821,.T.);
#59123=ORIENTED_EDGE('',*,*,#44816,.T.);
#59124=ORIENTED_EDGE('',*,*,#44822,.F.);
#59125=ORIENTED_EDGE('',*,*,#44823,.F.);
#59126=ORIENTED_EDGE('',*,*,#44824,.T.);
#59127=ORIENTED_EDGE('',*,*,#44820,.T.);
#59128=ORIENTED_EDGE('',*,*,#44825,.F.);
#59129=ORIENTED_EDGE('',*,*,#44818,.F.);
#59130=ORIENTED_EDGE('',*,*,#44826,.T.);
#59131=ORIENTED_EDGE('',*,*,#44823,.T.);
#59132=ORIENTED_EDGE('',*,*,#44827,.F.);
#59133=ORIENTED_EDGE('',*,*,#44828,.F.);
#59134=ORIENTED_EDGE('',*,*,#44829,.T.);
#59135=ORIENTED_EDGE('',*,*,#44830,.T.);
#59136=ORIENTED_EDGE('',*,*,#44831,.F.);
#59137=ORIENTED_EDGE('',*,*,#44832,.F.);
#59138=ORIENTED_EDGE('',*,*,#44833,.T.);
#59139=ORIENTED_EDGE('',*,*,#44828,.T.);
#59140=ORIENTED_EDGE('',*,*,#44834,.F.);
#59141=ORIENTED_EDGE('',*,*,#44835,.F.);
#59142=ORIENTED_EDGE('',*,*,#44836,.T.);
#59143=ORIENTED_EDGE('',*,*,#44832,.T.);
#59144=ORIENTED_EDGE('',*,*,#44837,.F.);
#59145=ORIENTED_EDGE('',*,*,#44830,.F.);
#59146=ORIENTED_EDGE('',*,*,#44838,.T.);
#59147=ORIENTED_EDGE('',*,*,#44835,.T.);
#59148=ORIENTED_EDGE('',*,*,#44839,.F.);
#59149=ORIENTED_EDGE('',*,*,#44840,.F.);
#59150=ORIENTED_EDGE('',*,*,#44841,.T.);
#59151=ORIENTED_EDGE('',*,*,#44842,.T.);
#59152=ORIENTED_EDGE('',*,*,#44843,.F.);
#59153=ORIENTED_EDGE('',*,*,#44844,.F.);
#59154=ORIENTED_EDGE('',*,*,#44845,.T.);
#59155=ORIENTED_EDGE('',*,*,#44840,.T.);
#59156=ORIENTED_EDGE('',*,*,#44846,.F.);
#59157=ORIENTED_EDGE('',*,*,#44847,.F.);
#59158=ORIENTED_EDGE('',*,*,#44848,.T.);
#59159=ORIENTED_EDGE('',*,*,#44844,.T.);
#59160=ORIENTED_EDGE('',*,*,#44849,.F.);
#59161=ORIENTED_EDGE('',*,*,#44842,.F.);
#59162=ORIENTED_EDGE('',*,*,#44850,.T.);
#59163=ORIENTED_EDGE('',*,*,#44847,.T.);
#59164=ORIENTED_EDGE('',*,*,#44851,.F.);
#59165=ORIENTED_EDGE('',*,*,#44852,.F.);
#59166=ORIENTED_EDGE('',*,*,#44853,.T.);
#59167=ORIENTED_EDGE('',*,*,#44854,.T.);
#59168=ORIENTED_EDGE('',*,*,#44855,.F.);
#59169=ORIENTED_EDGE('',*,*,#44856,.F.);
#59170=ORIENTED_EDGE('',*,*,#44857,.T.);
#59171=ORIENTED_EDGE('',*,*,#44852,.T.);
#59172=ORIENTED_EDGE('',*,*,#44858,.F.);
#59173=ORIENTED_EDGE('',*,*,#44859,.F.);
#59174=ORIENTED_EDGE('',*,*,#44860,.T.);
#59175=ORIENTED_EDGE('',*,*,#44856,.T.);
#59176=ORIENTED_EDGE('',*,*,#44861,.F.);
#59177=ORIENTED_EDGE('',*,*,#44854,.F.);
#59178=ORIENTED_EDGE('',*,*,#44862,.T.);
#59179=ORIENTED_EDGE('',*,*,#44859,.T.);
#59180=ORIENTED_EDGE('',*,*,#44863,.F.);
#59181=ORIENTED_EDGE('',*,*,#44864,.F.);
#59182=ORIENTED_EDGE('',*,*,#44865,.T.);
#59183=ORIENTED_EDGE('',*,*,#44866,.T.);
#59184=ORIENTED_EDGE('',*,*,#44867,.F.);
#59185=ORIENTED_EDGE('',*,*,#44868,.F.);
#59186=ORIENTED_EDGE('',*,*,#44869,.T.);
#59187=ORIENTED_EDGE('',*,*,#44864,.T.);
#59188=ORIENTED_EDGE('',*,*,#44870,.F.);
#59189=ORIENTED_EDGE('',*,*,#44871,.F.);
#59190=ORIENTED_EDGE('',*,*,#44872,.T.);
#59191=ORIENTED_EDGE('',*,*,#44868,.T.);
#59192=ORIENTED_EDGE('',*,*,#44873,.F.);
#59193=ORIENTED_EDGE('',*,*,#44866,.F.);
#59194=ORIENTED_EDGE('',*,*,#44874,.T.);
#59195=ORIENTED_EDGE('',*,*,#44871,.T.);
#59196=ORIENTED_EDGE('',*,*,#44875,.F.);
#59197=ORIENTED_EDGE('',*,*,#44876,.F.);
#59198=ORIENTED_EDGE('',*,*,#44877,.T.);
#59199=ORIENTED_EDGE('',*,*,#44878,.T.);
#59200=ORIENTED_EDGE('',*,*,#44879,.F.);
#59201=ORIENTED_EDGE('',*,*,#44880,.F.);
#59202=ORIENTED_EDGE('',*,*,#44881,.T.);
#59203=ORIENTED_EDGE('',*,*,#44876,.T.);
#59204=ORIENTED_EDGE('',*,*,#44882,.F.);
#59205=ORIENTED_EDGE('',*,*,#44883,.F.);
#59206=ORIENTED_EDGE('',*,*,#44884,.T.);
#59207=ORIENTED_EDGE('',*,*,#44880,.T.);
#59208=ORIENTED_EDGE('',*,*,#44885,.F.);
#59209=ORIENTED_EDGE('',*,*,#44878,.F.);
#59210=ORIENTED_EDGE('',*,*,#44886,.T.);
#59211=ORIENTED_EDGE('',*,*,#44883,.T.);
#59212=ORIENTED_EDGE('',*,*,#44887,.F.);
#59213=ORIENTED_EDGE('',*,*,#44888,.F.);
#59214=ORIENTED_EDGE('',*,*,#44889,.T.);
#59215=ORIENTED_EDGE('',*,*,#44890,.T.);
#59216=ORIENTED_EDGE('',*,*,#44891,.F.);
#59217=ORIENTED_EDGE('',*,*,#44892,.F.);
#59218=ORIENTED_EDGE('',*,*,#44893,.T.);
#59219=ORIENTED_EDGE('',*,*,#44888,.T.);
#59220=ORIENTED_EDGE('',*,*,#44894,.F.);
#59221=ORIENTED_EDGE('',*,*,#44895,.F.);
#59222=ORIENTED_EDGE('',*,*,#44896,.T.);
#59223=ORIENTED_EDGE('',*,*,#44892,.T.);
#59224=ORIENTED_EDGE('',*,*,#44897,.F.);
#59225=ORIENTED_EDGE('',*,*,#44890,.F.);
#59226=ORIENTED_EDGE('',*,*,#44898,.T.);
#59227=ORIENTED_EDGE('',*,*,#44895,.T.);
#59228=ORIENTED_EDGE('',*,*,#44899,.F.);
#59229=ORIENTED_EDGE('',*,*,#44900,.F.);
#59230=ORIENTED_EDGE('',*,*,#44901,.T.);
#59231=ORIENTED_EDGE('',*,*,#44902,.T.);
#59232=ORIENTED_EDGE('',*,*,#44903,.F.);
#59233=ORIENTED_EDGE('',*,*,#44904,.F.);
#59234=ORIENTED_EDGE('',*,*,#44905,.T.);
#59235=ORIENTED_EDGE('',*,*,#44900,.T.);
#59236=ORIENTED_EDGE('',*,*,#44906,.F.);
#59237=ORIENTED_EDGE('',*,*,#44907,.F.);
#59238=ORIENTED_EDGE('',*,*,#44908,.T.);
#59239=ORIENTED_EDGE('',*,*,#44904,.T.);
#59240=ORIENTED_EDGE('',*,*,#44909,.F.);
#59241=ORIENTED_EDGE('',*,*,#44902,.F.);
#59242=ORIENTED_EDGE('',*,*,#44910,.T.);
#59243=ORIENTED_EDGE('',*,*,#44907,.T.);
#59244=ORIENTED_EDGE('',*,*,#44911,.F.);
#59245=ORIENTED_EDGE('',*,*,#44912,.F.);
#59246=ORIENTED_EDGE('',*,*,#44913,.T.);
#59247=ORIENTED_EDGE('',*,*,#44914,.T.);
#59248=ORIENTED_EDGE('',*,*,#44915,.F.);
#59249=ORIENTED_EDGE('',*,*,#44916,.F.);
#59250=ORIENTED_EDGE('',*,*,#44917,.T.);
#59251=ORIENTED_EDGE('',*,*,#44912,.T.);
#59252=ORIENTED_EDGE('',*,*,#44918,.F.);
#59253=ORIENTED_EDGE('',*,*,#44919,.F.);
#59254=ORIENTED_EDGE('',*,*,#44920,.T.);
#59255=ORIENTED_EDGE('',*,*,#44916,.T.);
#59256=ORIENTED_EDGE('',*,*,#44921,.F.);
#59257=ORIENTED_EDGE('',*,*,#44914,.F.);
#59258=ORIENTED_EDGE('',*,*,#44922,.T.);
#59259=ORIENTED_EDGE('',*,*,#44919,.T.);
#59260=ORIENTED_EDGE('',*,*,#44923,.F.);
#59261=ORIENTED_EDGE('',*,*,#44924,.F.);
#59262=ORIENTED_EDGE('',*,*,#44925,.T.);
#59263=ORIENTED_EDGE('',*,*,#44926,.T.);
#59264=ORIENTED_EDGE('',*,*,#44927,.F.);
#59265=ORIENTED_EDGE('',*,*,#44928,.F.);
#59266=ORIENTED_EDGE('',*,*,#44929,.T.);
#59267=ORIENTED_EDGE('',*,*,#44924,.T.);
#59268=ORIENTED_EDGE('',*,*,#44930,.F.);
#59269=ORIENTED_EDGE('',*,*,#44931,.F.);
#59270=ORIENTED_EDGE('',*,*,#44932,.T.);
#59271=ORIENTED_EDGE('',*,*,#44928,.T.);
#59272=ORIENTED_EDGE('',*,*,#44933,.F.);
#59273=ORIENTED_EDGE('',*,*,#44926,.F.);
#59274=ORIENTED_EDGE('',*,*,#44934,.T.);
#59275=ORIENTED_EDGE('',*,*,#44931,.T.);
#59276=ORIENTED_EDGE('',*,*,#44935,.F.);
#59277=ORIENTED_EDGE('',*,*,#44936,.F.);
#59278=ORIENTED_EDGE('',*,*,#44937,.T.);
#59279=ORIENTED_EDGE('',*,*,#44938,.T.);
#59280=ORIENTED_EDGE('',*,*,#44939,.F.);
#59281=ORIENTED_EDGE('',*,*,#44940,.F.);
#59282=ORIENTED_EDGE('',*,*,#44941,.T.);
#59283=ORIENTED_EDGE('',*,*,#44936,.T.);
#59284=ORIENTED_EDGE('',*,*,#44942,.F.);
#59285=ORIENTED_EDGE('',*,*,#44943,.F.);
#59286=ORIENTED_EDGE('',*,*,#44944,.T.);
#59287=ORIENTED_EDGE('',*,*,#44940,.T.);
#59288=ORIENTED_EDGE('',*,*,#44945,.F.);
#59289=ORIENTED_EDGE('',*,*,#44938,.F.);
#59290=ORIENTED_EDGE('',*,*,#44946,.T.);
#59291=ORIENTED_EDGE('',*,*,#44943,.T.);
#59292=ORIENTED_EDGE('',*,*,#44947,.F.);
#59293=ORIENTED_EDGE('',*,*,#44948,.F.);
#59294=ORIENTED_EDGE('',*,*,#44949,.T.);
#59295=ORIENTED_EDGE('',*,*,#44950,.T.);
#59296=ORIENTED_EDGE('',*,*,#44951,.F.);
#59297=ORIENTED_EDGE('',*,*,#44952,.F.);
#59298=ORIENTED_EDGE('',*,*,#44953,.T.);
#59299=ORIENTED_EDGE('',*,*,#44948,.T.);
#59300=ORIENTED_EDGE('',*,*,#44954,.F.);
#59301=ORIENTED_EDGE('',*,*,#44955,.F.);
#59302=ORIENTED_EDGE('',*,*,#44956,.T.);
#59303=ORIENTED_EDGE('',*,*,#44952,.T.);
#59304=ORIENTED_EDGE('',*,*,#44957,.F.);
#59305=ORIENTED_EDGE('',*,*,#44950,.F.);
#59306=ORIENTED_EDGE('',*,*,#44958,.T.);
#59307=ORIENTED_EDGE('',*,*,#44955,.T.);
#59308=ORIENTED_EDGE('',*,*,#44959,.F.);
#59309=ORIENTED_EDGE('',*,*,#44960,.F.);
#59310=ORIENTED_EDGE('',*,*,#44961,.T.);
#59311=ORIENTED_EDGE('',*,*,#44962,.T.);
#59312=ORIENTED_EDGE('',*,*,#44963,.F.);
#59313=ORIENTED_EDGE('',*,*,#44964,.F.);
#59314=ORIENTED_EDGE('',*,*,#44965,.T.);
#59315=ORIENTED_EDGE('',*,*,#44960,.T.);
#59316=ORIENTED_EDGE('',*,*,#44966,.F.);
#59317=ORIENTED_EDGE('',*,*,#44967,.F.);
#59318=ORIENTED_EDGE('',*,*,#44968,.T.);
#59319=ORIENTED_EDGE('',*,*,#44964,.T.);
#59320=ORIENTED_EDGE('',*,*,#44969,.F.);
#59321=ORIENTED_EDGE('',*,*,#44962,.F.);
#59322=ORIENTED_EDGE('',*,*,#44970,.T.);
#59323=ORIENTED_EDGE('',*,*,#44967,.T.);
#59324=ORIENTED_EDGE('',*,*,#44971,.F.);
#59325=ORIENTED_EDGE('',*,*,#44972,.F.);
#59326=ORIENTED_EDGE('',*,*,#44973,.T.);
#59327=ORIENTED_EDGE('',*,*,#44974,.T.);
#59328=ORIENTED_EDGE('',*,*,#44975,.F.);
#59329=ORIENTED_EDGE('',*,*,#44976,.F.);
#59330=ORIENTED_EDGE('',*,*,#44977,.T.);
#59331=ORIENTED_EDGE('',*,*,#44972,.T.);
#59332=ORIENTED_EDGE('',*,*,#44978,.F.);
#59333=ORIENTED_EDGE('',*,*,#44979,.F.);
#59334=ORIENTED_EDGE('',*,*,#44980,.T.);
#59335=ORIENTED_EDGE('',*,*,#44976,.T.);
#59336=ORIENTED_EDGE('',*,*,#44981,.F.);
#59337=ORIENTED_EDGE('',*,*,#44974,.F.);
#59338=ORIENTED_EDGE('',*,*,#44982,.T.);
#59339=ORIENTED_EDGE('',*,*,#44979,.T.);
#59340=ORIENTED_EDGE('',*,*,#44983,.F.);
#59341=ORIENTED_EDGE('',*,*,#44984,.F.);
#59342=ORIENTED_EDGE('',*,*,#44985,.T.);
#59343=ORIENTED_EDGE('',*,*,#44986,.T.);
#59344=ORIENTED_EDGE('',*,*,#44987,.F.);
#59345=ORIENTED_EDGE('',*,*,#44988,.F.);
#59346=ORIENTED_EDGE('',*,*,#44989,.T.);
#59347=ORIENTED_EDGE('',*,*,#44984,.T.);
#59348=ORIENTED_EDGE('',*,*,#44990,.F.);
#59349=ORIENTED_EDGE('',*,*,#44991,.F.);
#59350=ORIENTED_EDGE('',*,*,#44992,.T.);
#59351=ORIENTED_EDGE('',*,*,#44988,.T.);
#59352=ORIENTED_EDGE('',*,*,#44993,.F.);
#59353=ORIENTED_EDGE('',*,*,#44986,.F.);
#59354=ORIENTED_EDGE('',*,*,#44994,.T.);
#59355=ORIENTED_EDGE('',*,*,#44991,.T.);
#59356=ORIENTED_EDGE('',*,*,#44995,.F.);
#59357=ORIENTED_EDGE('',*,*,#44996,.F.);
#59358=ORIENTED_EDGE('',*,*,#44997,.T.);
#59359=ORIENTED_EDGE('',*,*,#44998,.T.);
#59360=ORIENTED_EDGE('',*,*,#44999,.F.);
#59361=ORIENTED_EDGE('',*,*,#45000,.F.);
#59362=ORIENTED_EDGE('',*,*,#45001,.T.);
#59363=ORIENTED_EDGE('',*,*,#44996,.T.);
#59364=ORIENTED_EDGE('',*,*,#45002,.F.);
#59365=ORIENTED_EDGE('',*,*,#45003,.F.);
#59366=ORIENTED_EDGE('',*,*,#45004,.T.);
#59367=ORIENTED_EDGE('',*,*,#45000,.T.);
#59368=ORIENTED_EDGE('',*,*,#45005,.F.);
#59369=ORIENTED_EDGE('',*,*,#44998,.F.);
#59370=ORIENTED_EDGE('',*,*,#45006,.T.);
#59371=ORIENTED_EDGE('',*,*,#45003,.T.);
#59372=ORIENTED_EDGE('',*,*,#45007,.F.);
#59373=ORIENTED_EDGE('',*,*,#45008,.F.);
#59374=ORIENTED_EDGE('',*,*,#45009,.T.);
#59375=ORIENTED_EDGE('',*,*,#45010,.T.);
#59376=ORIENTED_EDGE('',*,*,#45011,.F.);
#59377=ORIENTED_EDGE('',*,*,#45012,.F.);
#59378=ORIENTED_EDGE('',*,*,#45013,.T.);
#59379=ORIENTED_EDGE('',*,*,#45008,.T.);
#59380=ORIENTED_EDGE('',*,*,#45014,.F.);
#59381=ORIENTED_EDGE('',*,*,#45015,.F.);
#59382=ORIENTED_EDGE('',*,*,#45016,.T.);
#59383=ORIENTED_EDGE('',*,*,#45012,.T.);
#59384=ORIENTED_EDGE('',*,*,#45017,.F.);
#59385=ORIENTED_EDGE('',*,*,#45010,.F.);
#59386=ORIENTED_EDGE('',*,*,#45018,.T.);
#59387=ORIENTED_EDGE('',*,*,#45015,.T.);
#59388=ORIENTED_EDGE('',*,*,#45019,.F.);
#59389=ORIENTED_EDGE('',*,*,#45020,.F.);
#59390=ORIENTED_EDGE('',*,*,#45021,.T.);
#59391=ORIENTED_EDGE('',*,*,#45022,.T.);
#59392=ORIENTED_EDGE('',*,*,#45023,.F.);
#59393=ORIENTED_EDGE('',*,*,#45024,.F.);
#59394=ORIENTED_EDGE('',*,*,#45025,.T.);
#59395=ORIENTED_EDGE('',*,*,#45020,.T.);
#59396=ORIENTED_EDGE('',*,*,#45026,.F.);
#59397=ORIENTED_EDGE('',*,*,#45027,.F.);
#59398=ORIENTED_EDGE('',*,*,#45028,.T.);
#59399=ORIENTED_EDGE('',*,*,#45024,.T.);
#59400=ORIENTED_EDGE('',*,*,#45029,.F.);
#59401=ORIENTED_EDGE('',*,*,#45022,.F.);
#59402=ORIENTED_EDGE('',*,*,#45030,.T.);
#59403=ORIENTED_EDGE('',*,*,#45027,.T.);
#59404=ORIENTED_EDGE('',*,*,#45031,.F.);
#59405=ORIENTED_EDGE('',*,*,#45032,.F.);
#59406=ORIENTED_EDGE('',*,*,#45033,.T.);
#59407=ORIENTED_EDGE('',*,*,#45034,.T.);
#59408=ORIENTED_EDGE('',*,*,#45035,.F.);
#59409=ORIENTED_EDGE('',*,*,#45036,.F.);
#59410=ORIENTED_EDGE('',*,*,#45037,.T.);
#59411=ORIENTED_EDGE('',*,*,#45032,.T.);
#59412=ORIENTED_EDGE('',*,*,#45038,.F.);
#59413=ORIENTED_EDGE('',*,*,#45039,.F.);
#59414=ORIENTED_EDGE('',*,*,#45040,.T.);
#59415=ORIENTED_EDGE('',*,*,#45036,.T.);
#59416=ORIENTED_EDGE('',*,*,#45041,.F.);
#59417=ORIENTED_EDGE('',*,*,#45034,.F.);
#59418=ORIENTED_EDGE('',*,*,#45042,.T.);
#59419=ORIENTED_EDGE('',*,*,#45039,.T.);
#59420=ORIENTED_EDGE('',*,*,#45043,.F.);
#59421=ORIENTED_EDGE('',*,*,#45044,.F.);
#59422=ORIENTED_EDGE('',*,*,#45045,.T.);
#59423=ORIENTED_EDGE('',*,*,#45046,.T.);
#59424=ORIENTED_EDGE('',*,*,#45047,.F.);
#59425=ORIENTED_EDGE('',*,*,#45048,.F.);
#59426=ORIENTED_EDGE('',*,*,#45049,.T.);
#59427=ORIENTED_EDGE('',*,*,#45044,.T.);
#59428=ORIENTED_EDGE('',*,*,#45050,.F.);
#59429=ORIENTED_EDGE('',*,*,#45051,.F.);
#59430=ORIENTED_EDGE('',*,*,#45052,.T.);
#59431=ORIENTED_EDGE('',*,*,#45048,.T.);
#59432=ORIENTED_EDGE('',*,*,#45053,.F.);
#59433=ORIENTED_EDGE('',*,*,#45046,.F.);
#59434=ORIENTED_EDGE('',*,*,#45054,.T.);
#59435=ORIENTED_EDGE('',*,*,#45051,.T.);
#59436=ORIENTED_EDGE('',*,*,#45055,.F.);
#59437=ORIENTED_EDGE('',*,*,#45056,.F.);
#59438=ORIENTED_EDGE('',*,*,#45057,.T.);
#59439=ORIENTED_EDGE('',*,*,#45058,.T.);
#59440=ORIENTED_EDGE('',*,*,#45059,.F.);
#59441=ORIENTED_EDGE('',*,*,#45060,.F.);
#59442=ORIENTED_EDGE('',*,*,#45061,.T.);
#59443=ORIENTED_EDGE('',*,*,#45056,.T.);
#59444=ORIENTED_EDGE('',*,*,#45062,.F.);
#59445=ORIENTED_EDGE('',*,*,#45063,.F.);
#59446=ORIENTED_EDGE('',*,*,#45064,.T.);
#59447=ORIENTED_EDGE('',*,*,#45060,.T.);
#59448=ORIENTED_EDGE('',*,*,#45065,.F.);
#59449=ORIENTED_EDGE('',*,*,#45058,.F.);
#59450=ORIENTED_EDGE('',*,*,#45066,.T.);
#59451=ORIENTED_EDGE('',*,*,#45063,.T.);
#59452=ORIENTED_EDGE('',*,*,#45067,.F.);
#59453=ORIENTED_EDGE('',*,*,#45068,.F.);
#59454=ORIENTED_EDGE('',*,*,#45069,.T.);
#59455=ORIENTED_EDGE('',*,*,#45070,.T.);
#59456=ORIENTED_EDGE('',*,*,#45071,.F.);
#59457=ORIENTED_EDGE('',*,*,#45072,.F.);
#59458=ORIENTED_EDGE('',*,*,#45073,.T.);
#59459=ORIENTED_EDGE('',*,*,#45068,.T.);
#59460=ORIENTED_EDGE('',*,*,#45074,.F.);
#59461=ORIENTED_EDGE('',*,*,#45075,.F.);
#59462=ORIENTED_EDGE('',*,*,#45076,.T.);
#59463=ORIENTED_EDGE('',*,*,#45072,.T.);
#59464=ORIENTED_EDGE('',*,*,#45077,.F.);
#59465=ORIENTED_EDGE('',*,*,#45070,.F.);
#59466=ORIENTED_EDGE('',*,*,#45078,.T.);
#59467=ORIENTED_EDGE('',*,*,#45075,.T.);
#59468=ORIENTED_EDGE('',*,*,#45079,.F.);
#59469=ORIENTED_EDGE('',*,*,#45080,.F.);
#59470=ORIENTED_EDGE('',*,*,#45081,.T.);
#59471=ORIENTED_EDGE('',*,*,#45082,.T.);
#59472=ORIENTED_EDGE('',*,*,#45083,.F.);
#59473=ORIENTED_EDGE('',*,*,#45084,.F.);
#59474=ORIENTED_EDGE('',*,*,#45085,.T.);
#59475=ORIENTED_EDGE('',*,*,#45080,.T.);
#59476=ORIENTED_EDGE('',*,*,#45086,.F.);
#59477=ORIENTED_EDGE('',*,*,#45087,.F.);
#59478=ORIENTED_EDGE('',*,*,#45088,.T.);
#59479=ORIENTED_EDGE('',*,*,#45084,.T.);
#59480=ORIENTED_EDGE('',*,*,#45089,.F.);
#59481=ORIENTED_EDGE('',*,*,#45082,.F.);
#59482=ORIENTED_EDGE('',*,*,#45090,.T.);
#59483=ORIENTED_EDGE('',*,*,#45087,.T.);
#59484=ORIENTED_EDGE('',*,*,#45091,.F.);
#59485=ORIENTED_EDGE('',*,*,#45092,.F.);
#59486=ORIENTED_EDGE('',*,*,#45093,.T.);
#59487=ORIENTED_EDGE('',*,*,#45094,.T.);
#59488=ORIENTED_EDGE('',*,*,#45095,.F.);
#59489=ORIENTED_EDGE('',*,*,#45096,.F.);
#59490=ORIENTED_EDGE('',*,*,#45097,.T.);
#59491=ORIENTED_EDGE('',*,*,#45092,.T.);
#59492=ORIENTED_EDGE('',*,*,#45098,.F.);
#59493=ORIENTED_EDGE('',*,*,#45099,.F.);
#59494=ORIENTED_EDGE('',*,*,#45100,.T.);
#59495=ORIENTED_EDGE('',*,*,#45096,.T.);
#59496=ORIENTED_EDGE('',*,*,#45101,.F.);
#59497=ORIENTED_EDGE('',*,*,#45094,.F.);
#59498=ORIENTED_EDGE('',*,*,#45102,.T.);
#59499=ORIENTED_EDGE('',*,*,#45099,.T.);
#59500=ORIENTED_EDGE('',*,*,#45103,.F.);
#59501=ORIENTED_EDGE('',*,*,#45104,.F.);
#59502=ORIENTED_EDGE('',*,*,#45105,.T.);
#59503=ORIENTED_EDGE('',*,*,#45106,.T.);
#59504=ORIENTED_EDGE('',*,*,#45107,.F.);
#59505=ORIENTED_EDGE('',*,*,#45108,.F.);
#59506=ORIENTED_EDGE('',*,*,#45109,.T.);
#59507=ORIENTED_EDGE('',*,*,#45104,.T.);
#59508=ORIENTED_EDGE('',*,*,#45110,.F.);
#59509=ORIENTED_EDGE('',*,*,#45111,.F.);
#59510=ORIENTED_EDGE('',*,*,#45112,.T.);
#59511=ORIENTED_EDGE('',*,*,#45108,.T.);
#59512=ORIENTED_EDGE('',*,*,#45113,.F.);
#59513=ORIENTED_EDGE('',*,*,#45106,.F.);
#59514=ORIENTED_EDGE('',*,*,#45114,.T.);
#59515=ORIENTED_EDGE('',*,*,#45111,.T.);
#59516=ORIENTED_EDGE('',*,*,#45115,.F.);
#59517=ORIENTED_EDGE('',*,*,#45116,.F.);
#59518=ORIENTED_EDGE('',*,*,#45117,.T.);
#59519=ORIENTED_EDGE('',*,*,#45118,.T.);
#59520=ORIENTED_EDGE('',*,*,#45119,.F.);
#59521=ORIENTED_EDGE('',*,*,#45120,.F.);
#59522=ORIENTED_EDGE('',*,*,#45121,.T.);
#59523=ORIENTED_EDGE('',*,*,#45116,.T.);
#59524=ORIENTED_EDGE('',*,*,#45122,.F.);
#59525=ORIENTED_EDGE('',*,*,#45123,.F.);
#59526=ORIENTED_EDGE('',*,*,#45124,.T.);
#59527=ORIENTED_EDGE('',*,*,#45120,.T.);
#59528=ORIENTED_EDGE('',*,*,#45125,.F.);
#59529=ORIENTED_EDGE('',*,*,#45118,.F.);
#59530=ORIENTED_EDGE('',*,*,#45126,.T.);
#59531=ORIENTED_EDGE('',*,*,#45123,.T.);
#59532=ORIENTED_EDGE('',*,*,#45127,.F.);
#59533=ORIENTED_EDGE('',*,*,#45128,.F.);
#59534=ORIENTED_EDGE('',*,*,#45129,.T.);
#59535=ORIENTED_EDGE('',*,*,#45130,.T.);
#59536=ORIENTED_EDGE('',*,*,#45131,.F.);
#59537=ORIENTED_EDGE('',*,*,#45132,.F.);
#59538=ORIENTED_EDGE('',*,*,#45133,.T.);
#59539=ORIENTED_EDGE('',*,*,#45128,.T.);
#59540=ORIENTED_EDGE('',*,*,#45134,.F.);
#59541=ORIENTED_EDGE('',*,*,#45135,.F.);
#59542=ORIENTED_EDGE('',*,*,#45136,.T.);
#59543=ORIENTED_EDGE('',*,*,#45132,.T.);
#59544=ORIENTED_EDGE('',*,*,#45137,.F.);
#59545=ORIENTED_EDGE('',*,*,#45130,.F.);
#59546=ORIENTED_EDGE('',*,*,#45138,.T.);
#59547=ORIENTED_EDGE('',*,*,#45135,.T.);
#59548=ORIENTED_EDGE('',*,*,#45139,.F.);
#59549=ORIENTED_EDGE('',*,*,#45140,.F.);
#59550=ORIENTED_EDGE('',*,*,#45141,.T.);
#59551=ORIENTED_EDGE('',*,*,#45142,.T.);
#59552=ORIENTED_EDGE('',*,*,#45143,.F.);
#59553=ORIENTED_EDGE('',*,*,#45144,.F.);
#59554=ORIENTED_EDGE('',*,*,#45145,.F.);
#59555=ORIENTED_EDGE('',*,*,#45146,.T.);
#59556=ORIENTED_EDGE('',*,*,#45140,.T.);
#59557=ORIENTED_EDGE('',*,*,#45147,.F.);
#59558=ORIENTED_EDGE('',*,*,#45148,.F.);
#59559=ORIENTED_EDGE('',*,*,#45149,.F.);
#59560=ORIENTED_EDGE('',*,*,#45144,.T.);
#59561=ORIENTED_EDGE('',*,*,#45150,.F.);
#59562=ORIENTED_EDGE('',*,*,#45142,.F.);
#59563=ORIENTED_EDGE('',*,*,#45151,.F.);
#59564=ORIENTED_EDGE('',*,*,#45148,.T.);
#59565=ORIENTED_EDGE('',*,*,#45152,.F.);
#59566=ORIENTED_EDGE('',*,*,#45145,.T.);
#59567=ORIENTED_EDGE('',*,*,#45149,.T.);
#59568=ORIENTED_EDGE('',*,*,#45151,.T.);
#59569=ORIENTED_EDGE('',*,*,#45153,.T.);
#59570=ORIENTED_EDGE('',*,*,#45154,.F.);
#59571=ORIENTED_EDGE('',*,*,#45155,.T.);
#59572=ORIENTED_EDGE('',*,*,#45156,.T.);
#59573=ORIENTED_EDGE('',*,*,#45157,.F.);
#59574=ORIENTED_EDGE('',*,*,#45158,.F.);
#59575=ORIENTED_EDGE('',*,*,#45159,.F.);
#59576=ORIENTED_EDGE('',*,*,#45160,.T.);
#59577=ORIENTED_EDGE('',*,*,#45154,.T.);
#59578=ORIENTED_EDGE('',*,*,#45161,.F.);
#59579=ORIENTED_EDGE('',*,*,#45162,.F.);
#59580=ORIENTED_EDGE('',*,*,#45163,.F.);
#59581=ORIENTED_EDGE('',*,*,#45158,.T.);
#59582=ORIENTED_EDGE('',*,*,#45164,.F.);
#59583=ORIENTED_EDGE('',*,*,#45156,.F.);
#59584=ORIENTED_EDGE('',*,*,#45165,.T.);
#59585=ORIENTED_EDGE('',*,*,#45166,.F.);
#59586=ORIENTED_EDGE('',*,*,#45162,.T.);
#59587=ORIENTED_EDGE('',*,*,#45167,.F.);
#59588=ORIENTED_EDGE('',*,*,#45159,.T.);
#59589=ORIENTED_EDGE('',*,*,#45163,.T.);
#59590=ORIENTED_EDGE('',*,*,#45166,.T.);
#59591=ORIENTED_EDGE('',*,*,#45168,.T.);
#59592=ORIENTED_EDGE('',*,*,#45169,.F.);
#59593=ORIENTED_EDGE('',*,*,#45170,.T.);
#59594=ORIENTED_EDGE('',*,*,#45171,.T.);
#59595=ORIENTED_EDGE('',*,*,#45172,.F.);
#59596=ORIENTED_EDGE('',*,*,#45173,.F.);
#59597=ORIENTED_EDGE('',*,*,#45174,.F.);
#59598=ORIENTED_EDGE('',*,*,#45175,.T.);
#59599=ORIENTED_EDGE('',*,*,#45169,.T.);
#59600=ORIENTED_EDGE('',*,*,#45176,.F.);
#59601=ORIENTED_EDGE('',*,*,#45177,.F.);
#59602=ORIENTED_EDGE('',*,*,#45178,.F.);
#59603=ORIENTED_EDGE('',*,*,#45173,.T.);
#59604=ORIENTED_EDGE('',*,*,#45179,.F.);
#59605=ORIENTED_EDGE('',*,*,#45171,.F.);
#59606=ORIENTED_EDGE('',*,*,#45180,.T.);
#59607=ORIENTED_EDGE('',*,*,#45181,.F.);
#59608=ORIENTED_EDGE('',*,*,#45177,.T.);
#59609=ORIENTED_EDGE('',*,*,#45182,.F.);
#59610=ORIENTED_EDGE('',*,*,#45174,.T.);
#59611=ORIENTED_EDGE('',*,*,#45178,.T.);
#59612=ORIENTED_EDGE('',*,*,#45181,.T.);
#59613=ORIENTED_EDGE('',*,*,#45183,.T.);
#59614=ORIENTED_EDGE('',*,*,#45184,.F.);
#59615=ORIENTED_EDGE('',*,*,#45185,.T.);
#59616=ORIENTED_EDGE('',*,*,#45186,.T.);
#59617=ORIENTED_EDGE('',*,*,#45187,.F.);
#59618=ORIENTED_EDGE('',*,*,#45188,.F.);
#59619=ORIENTED_EDGE('',*,*,#45189,.F.);
#59620=ORIENTED_EDGE('',*,*,#45190,.T.);
#59621=ORIENTED_EDGE('',*,*,#45184,.T.);
#59622=ORIENTED_EDGE('',*,*,#45191,.F.);
#59623=ORIENTED_EDGE('',*,*,#45192,.F.);
#59624=ORIENTED_EDGE('',*,*,#45193,.F.);
#59625=ORIENTED_EDGE('',*,*,#45188,.T.);
#59626=ORIENTED_EDGE('',*,*,#45194,.F.);
#59627=ORIENTED_EDGE('',*,*,#45186,.F.);
#59628=ORIENTED_EDGE('',*,*,#45195,.T.);
#59629=ORIENTED_EDGE('',*,*,#45196,.F.);
#59630=ORIENTED_EDGE('',*,*,#45192,.T.);
#59631=ORIENTED_EDGE('',*,*,#45197,.F.);
#59632=ORIENTED_EDGE('',*,*,#45189,.T.);
#59633=ORIENTED_EDGE('',*,*,#45193,.T.);
#59634=ORIENTED_EDGE('',*,*,#45196,.T.);
#59635=ORIENTED_EDGE('',*,*,#45198,.T.);
#59636=ORIENTED_EDGE('',*,*,#45199,.F.);
#59637=ORIENTED_EDGE('',*,*,#45200,.T.);
#59638=ORIENTED_EDGE('',*,*,#45201,.T.);
#59639=ORIENTED_EDGE('',*,*,#45202,.F.);
#59640=ORIENTED_EDGE('',*,*,#45203,.F.);
#59641=ORIENTED_EDGE('',*,*,#45204,.F.);
#59642=ORIENTED_EDGE('',*,*,#45205,.T.);
#59643=ORIENTED_EDGE('',*,*,#45199,.T.);
#59644=ORIENTED_EDGE('',*,*,#45206,.F.);
#59645=ORIENTED_EDGE('',*,*,#45207,.F.);
#59646=ORIENTED_EDGE('',*,*,#45208,.F.);
#59647=ORIENTED_EDGE('',*,*,#45203,.T.);
#59648=ORIENTED_EDGE('',*,*,#45209,.F.);
#59649=ORIENTED_EDGE('',*,*,#45201,.F.);
#59650=ORIENTED_EDGE('',*,*,#45210,.T.);
#59651=ORIENTED_EDGE('',*,*,#45211,.F.);
#59652=ORIENTED_EDGE('',*,*,#45207,.T.);
#59653=ORIENTED_EDGE('',*,*,#45212,.F.);
#59654=ORIENTED_EDGE('',*,*,#45204,.T.);
#59655=ORIENTED_EDGE('',*,*,#45208,.T.);
#59656=ORIENTED_EDGE('',*,*,#45211,.T.);
#59657=ORIENTED_EDGE('',*,*,#45213,.T.);
#59658=ORIENTED_EDGE('',*,*,#45214,.F.);
#59659=ORIENTED_EDGE('',*,*,#45215,.F.);
#59660=ORIENTED_EDGE('',*,*,#45216,.T.);
#59661=ORIENTED_EDGE('',*,*,#45217,.T.);
#59662=ORIENTED_EDGE('',*,*,#45218,.F.);
#59663=ORIENTED_EDGE('',*,*,#45219,.F.);
#59664=ORIENTED_EDGE('',*,*,#45220,.F.);
#59665=ORIENTED_EDGE('',*,*,#45214,.T.);
#59666=ORIENTED_EDGE('',*,*,#45221,.F.);
#59667=ORIENTED_EDGE('',*,*,#45222,.F.);
#59668=ORIENTED_EDGE('',*,*,#45223,.F.);
#59669=ORIENTED_EDGE('',*,*,#45219,.T.);
#59670=ORIENTED_EDGE('',*,*,#45224,.F.);
#59671=ORIENTED_EDGE('',*,*,#45217,.F.);
#59672=ORIENTED_EDGE('',*,*,#45225,.T.);
#59673=ORIENTED_EDGE('',*,*,#45226,.F.);
#59674=ORIENTED_EDGE('',*,*,#45222,.T.);
#59675=ORIENTED_EDGE('',*,*,#45227,.F.);
#59676=ORIENTED_EDGE('',*,*,#45215,.T.);
#59677=ORIENTED_EDGE('',*,*,#45220,.T.);
#59678=ORIENTED_EDGE('',*,*,#45223,.T.);
#59679=ORIENTED_EDGE('',*,*,#45226,.T.);
#59680=ORIENTED_EDGE('',*,*,#45228,.T.);
#59681=ORIENTED_EDGE('',*,*,#45229,.F.);
#59682=ORIENTED_EDGE('',*,*,#45230,.F.);
#59683=ORIENTED_EDGE('',*,*,#45231,.T.);
#59684=ORIENTED_EDGE('',*,*,#45232,.T.);
#59685=ORIENTED_EDGE('',*,*,#45233,.F.);
#59686=ORIENTED_EDGE('',*,*,#45234,.F.);
#59687=ORIENTED_EDGE('',*,*,#45235,.F.);
#59688=ORIENTED_EDGE('',*,*,#45229,.T.);
#59689=ORIENTED_EDGE('',*,*,#45236,.F.);
#59690=ORIENTED_EDGE('',*,*,#45237,.F.);
#59691=ORIENTED_EDGE('',*,*,#45238,.F.);
#59692=ORIENTED_EDGE('',*,*,#45234,.T.);
#59693=ORIENTED_EDGE('',*,*,#45239,.F.);
#59694=ORIENTED_EDGE('',*,*,#45232,.F.);
#59695=ORIENTED_EDGE('',*,*,#45240,.T.);
#59696=ORIENTED_EDGE('',*,*,#45241,.F.);
#59697=ORIENTED_EDGE('',*,*,#45237,.T.);
#59698=ORIENTED_EDGE('',*,*,#45242,.F.);
#59699=ORIENTED_EDGE('',*,*,#45230,.T.);
#59700=ORIENTED_EDGE('',*,*,#45235,.T.);
#59701=ORIENTED_EDGE('',*,*,#45238,.T.);
#59702=ORIENTED_EDGE('',*,*,#45241,.T.);
#59703=ORIENTED_EDGE('',*,*,#45243,.T.);
#59704=ORIENTED_EDGE('',*,*,#45244,.F.);
#59705=ORIENTED_EDGE('',*,*,#45245,.T.);
#59706=ORIENTED_EDGE('',*,*,#45246,.T.);
#59707=ORIENTED_EDGE('',*,*,#45247,.F.);
#59708=ORIENTED_EDGE('',*,*,#45248,.F.);
#59709=ORIENTED_EDGE('',*,*,#45249,.F.);
#59710=ORIENTED_EDGE('',*,*,#45250,.T.);
#59711=ORIENTED_EDGE('',*,*,#45244,.T.);
#59712=ORIENTED_EDGE('',*,*,#45251,.F.);
#59713=ORIENTED_EDGE('',*,*,#45252,.F.);
#59714=ORIENTED_EDGE('',*,*,#45253,.F.);
#59715=ORIENTED_EDGE('',*,*,#45248,.T.);
#59716=ORIENTED_EDGE('',*,*,#45254,.F.);
#59717=ORIENTED_EDGE('',*,*,#45246,.F.);
#59718=ORIENTED_EDGE('',*,*,#45255,.T.);
#59719=ORIENTED_EDGE('',*,*,#45256,.F.);
#59720=ORIENTED_EDGE('',*,*,#45252,.T.);
#59721=ORIENTED_EDGE('',*,*,#45257,.F.);
#59722=ORIENTED_EDGE('',*,*,#45249,.T.);
#59723=ORIENTED_EDGE('',*,*,#45253,.T.);
#59724=ORIENTED_EDGE('',*,*,#45256,.T.);
#59725=ORIENTED_EDGE('',*,*,#45258,.T.);
#59726=ORIENTED_EDGE('',*,*,#45259,.F.);
#59727=ORIENTED_EDGE('',*,*,#45260,.T.);
#59728=ORIENTED_EDGE('',*,*,#45261,.T.);
#59729=ORIENTED_EDGE('',*,*,#45262,.F.);
#59730=ORIENTED_EDGE('',*,*,#45263,.F.);
#59731=ORIENTED_EDGE('',*,*,#45264,.F.);
#59732=ORIENTED_EDGE('',*,*,#45265,.T.);
#59733=ORIENTED_EDGE('',*,*,#45259,.T.);
#59734=ORIENTED_EDGE('',*,*,#45266,.F.);
#59735=ORIENTED_EDGE('',*,*,#45267,.F.);
#59736=ORIENTED_EDGE('',*,*,#45268,.F.);
#59737=ORIENTED_EDGE('',*,*,#45263,.T.);
#59738=ORIENTED_EDGE('',*,*,#45269,.F.);
#59739=ORIENTED_EDGE('',*,*,#45261,.F.);
#59740=ORIENTED_EDGE('',*,*,#45270,.T.);
#59741=ORIENTED_EDGE('',*,*,#45271,.F.);
#59742=ORIENTED_EDGE('',*,*,#45267,.T.);
#59743=ORIENTED_EDGE('',*,*,#45272,.F.);
#59744=ORIENTED_EDGE('',*,*,#45264,.T.);
#59745=ORIENTED_EDGE('',*,*,#45268,.T.);
#59746=ORIENTED_EDGE('',*,*,#45271,.T.);
#59747=ORIENTED_EDGE('',*,*,#45273,.T.);
#59748=ORIENTED_EDGE('',*,*,#45274,.F.);
#59749=ORIENTED_EDGE('',*,*,#45275,.T.);
#59750=ORIENTED_EDGE('',*,*,#45276,.T.);
#59751=ORIENTED_EDGE('',*,*,#45277,.F.);
#59752=ORIENTED_EDGE('',*,*,#45278,.F.);
#59753=ORIENTED_EDGE('',*,*,#45279,.F.);
#59754=ORIENTED_EDGE('',*,*,#45280,.T.);
#59755=ORIENTED_EDGE('',*,*,#45274,.T.);
#59756=ORIENTED_EDGE('',*,*,#45281,.F.);
#59757=ORIENTED_EDGE('',*,*,#45282,.F.);
#59758=ORIENTED_EDGE('',*,*,#45283,.F.);
#59759=ORIENTED_EDGE('',*,*,#45278,.T.);
#59760=ORIENTED_EDGE('',*,*,#45284,.F.);
#59761=ORIENTED_EDGE('',*,*,#45276,.F.);
#59762=ORIENTED_EDGE('',*,*,#45285,.T.);
#59763=ORIENTED_EDGE('',*,*,#45286,.F.);
#59764=ORIENTED_EDGE('',*,*,#45282,.T.);
#59765=ORIENTED_EDGE('',*,*,#45287,.F.);
#59766=ORIENTED_EDGE('',*,*,#45279,.T.);
#59767=ORIENTED_EDGE('',*,*,#45283,.T.);
#59768=ORIENTED_EDGE('',*,*,#45286,.T.);
#59769=ORIENTED_EDGE('',*,*,#45288,.T.);
#59770=ORIENTED_EDGE('',*,*,#45289,.F.);
#59771=ORIENTED_EDGE('',*,*,#45290,.T.);
#59772=ORIENTED_EDGE('',*,*,#45291,.T.);
#59773=ORIENTED_EDGE('',*,*,#45292,.F.);
#59774=ORIENTED_EDGE('',*,*,#45293,.F.);
#59775=ORIENTED_EDGE('',*,*,#45294,.T.);
#59776=ORIENTED_EDGE('',*,*,#45289,.T.);
#59777=ORIENTED_EDGE('',*,*,#45295,.F.);
#59778=ORIENTED_EDGE('',*,*,#45296,.F.);
#59779=ORIENTED_EDGE('',*,*,#45297,.T.);
#59780=ORIENTED_EDGE('',*,*,#45293,.T.);
#59781=ORIENTED_EDGE('',*,*,#45298,.F.);
#59782=ORIENTED_EDGE('',*,*,#45291,.F.);
#59783=ORIENTED_EDGE('',*,*,#45299,.T.);
#59784=ORIENTED_EDGE('',*,*,#45296,.T.);
#59785=ORIENTED_EDGE('',*,*,#45300,.F.);
#59786=ORIENTED_EDGE('',*,*,#45301,.F.);
#59787=ORIENTED_EDGE('',*,*,#45302,.T.);
#59788=ORIENTED_EDGE('',*,*,#45303,.T.);
#59789=ORIENTED_EDGE('',*,*,#45304,.F.);
#59790=ORIENTED_EDGE('',*,*,#45305,.F.);
#59791=ORIENTED_EDGE('',*,*,#45306,.T.);
#59792=ORIENTED_EDGE('',*,*,#45301,.T.);
#59793=ORIENTED_EDGE('',*,*,#45307,.F.);
#59794=ORIENTED_EDGE('',*,*,#45308,.F.);
#59795=ORIENTED_EDGE('',*,*,#45309,.T.);
#59796=ORIENTED_EDGE('',*,*,#45305,.T.);
#59797=ORIENTED_EDGE('',*,*,#45310,.F.);
#59798=ORIENTED_EDGE('',*,*,#45303,.F.);
#59799=ORIENTED_EDGE('',*,*,#45311,.T.);
#59800=ORIENTED_EDGE('',*,*,#45308,.T.);
#59801=ORIENTED_EDGE('',*,*,#45312,.F.);
#59802=ORIENTED_EDGE('',*,*,#45313,.F.);
#59803=ORIENTED_EDGE('',*,*,#45314,.T.);
#59804=ORIENTED_EDGE('',*,*,#45315,.T.);
#59805=ORIENTED_EDGE('',*,*,#45316,.F.);
#59806=ORIENTED_EDGE('',*,*,#45317,.F.);
#59807=ORIENTED_EDGE('',*,*,#45318,.T.);
#59808=ORIENTED_EDGE('',*,*,#45313,.T.);
#59809=ORIENTED_EDGE('',*,*,#45319,.F.);
#59810=ORIENTED_EDGE('',*,*,#45320,.F.);
#59811=ORIENTED_EDGE('',*,*,#45321,.T.);
#59812=ORIENTED_EDGE('',*,*,#45317,.T.);
#59813=ORIENTED_EDGE('',*,*,#45322,.F.);
#59814=ORIENTED_EDGE('',*,*,#45315,.F.);
#59815=ORIENTED_EDGE('',*,*,#45323,.T.);
#59816=ORIENTED_EDGE('',*,*,#45320,.T.);
#59817=ORIENTED_EDGE('',*,*,#45324,.F.);
#59818=ORIENTED_EDGE('',*,*,#45325,.F.);
#59819=ORIENTED_EDGE('',*,*,#45326,.T.);
#59820=ORIENTED_EDGE('',*,*,#45327,.T.);
#59821=ORIENTED_EDGE('',*,*,#45328,.F.);
#59822=ORIENTED_EDGE('',*,*,#45329,.F.);
#59823=ORIENTED_EDGE('',*,*,#45330,.T.);
#59824=ORIENTED_EDGE('',*,*,#45325,.T.);
#59825=ORIENTED_EDGE('',*,*,#45331,.F.);
#59826=ORIENTED_EDGE('',*,*,#45332,.F.);
#59827=ORIENTED_EDGE('',*,*,#45333,.T.);
#59828=ORIENTED_EDGE('',*,*,#45329,.T.);
#59829=ORIENTED_EDGE('',*,*,#45334,.F.);
#59830=ORIENTED_EDGE('',*,*,#45327,.F.);
#59831=ORIENTED_EDGE('',*,*,#45335,.T.);
#59832=ORIENTED_EDGE('',*,*,#45332,.T.);
#59833=ORIENTED_EDGE('',*,*,#45336,.F.);
#59834=ORIENTED_EDGE('',*,*,#45337,.F.);
#59835=ORIENTED_EDGE('',*,*,#45338,.T.);
#59836=ORIENTED_EDGE('',*,*,#45339,.T.);
#59837=ORIENTED_EDGE('',*,*,#45340,.F.);
#59838=ORIENTED_EDGE('',*,*,#45341,.F.);
#59839=ORIENTED_EDGE('',*,*,#45342,.T.);
#59840=ORIENTED_EDGE('',*,*,#45337,.T.);
#59841=ORIENTED_EDGE('',*,*,#45343,.F.);
#59842=ORIENTED_EDGE('',*,*,#45344,.F.);
#59843=ORIENTED_EDGE('',*,*,#45345,.T.);
#59844=ORIENTED_EDGE('',*,*,#45341,.T.);
#59845=ORIENTED_EDGE('',*,*,#45346,.F.);
#59846=ORIENTED_EDGE('',*,*,#45339,.F.);
#59847=ORIENTED_EDGE('',*,*,#45347,.T.);
#59848=ORIENTED_EDGE('',*,*,#45344,.T.);
#59849=ORIENTED_EDGE('',*,*,#45348,.F.);
#59850=ORIENTED_EDGE('',*,*,#45349,.F.);
#59851=ORIENTED_EDGE('',*,*,#45350,.T.);
#59852=ORIENTED_EDGE('',*,*,#45351,.T.);
#59853=ORIENTED_EDGE('',*,*,#45352,.F.);
#59854=ORIENTED_EDGE('',*,*,#45353,.F.);
#59855=ORIENTED_EDGE('',*,*,#45354,.T.);
#59856=ORIENTED_EDGE('',*,*,#45349,.T.);
#59857=ORIENTED_EDGE('',*,*,#45355,.F.);
#59858=ORIENTED_EDGE('',*,*,#45356,.F.);
#59859=ORIENTED_EDGE('',*,*,#45357,.T.);
#59860=ORIENTED_EDGE('',*,*,#45353,.T.);
#59861=ORIENTED_EDGE('',*,*,#45358,.F.);
#59862=ORIENTED_EDGE('',*,*,#45351,.F.);
#59863=ORIENTED_EDGE('',*,*,#45359,.T.);
#59864=ORIENTED_EDGE('',*,*,#45356,.T.);
#59865=ORIENTED_EDGE('',*,*,#45360,.F.);
#59866=ORIENTED_EDGE('',*,*,#45361,.F.);
#59867=ORIENTED_EDGE('',*,*,#45362,.T.);
#59868=ORIENTED_EDGE('',*,*,#45363,.T.);
#59869=ORIENTED_EDGE('',*,*,#45364,.F.);
#59870=ORIENTED_EDGE('',*,*,#45365,.F.);
#59871=ORIENTED_EDGE('',*,*,#45366,.T.);
#59872=ORIENTED_EDGE('',*,*,#45361,.T.);
#59873=ORIENTED_EDGE('',*,*,#45367,.F.);
#59874=ORIENTED_EDGE('',*,*,#45368,.F.);
#59875=ORIENTED_EDGE('',*,*,#45369,.T.);
#59876=ORIENTED_EDGE('',*,*,#45365,.T.);
#59877=ORIENTED_EDGE('',*,*,#45370,.F.);
#59878=ORIENTED_EDGE('',*,*,#45363,.F.);
#59879=ORIENTED_EDGE('',*,*,#45371,.T.);
#59880=ORIENTED_EDGE('',*,*,#45368,.T.);
#59881=ORIENTED_EDGE('',*,*,#45372,.F.);
#59882=ORIENTED_EDGE('',*,*,#45373,.F.);
#59883=ORIENTED_EDGE('',*,*,#45374,.T.);
#59884=ORIENTED_EDGE('',*,*,#45375,.T.);
#59885=ORIENTED_EDGE('',*,*,#45376,.F.);
#59886=ORIENTED_EDGE('',*,*,#45377,.F.);
#59887=ORIENTED_EDGE('',*,*,#45378,.T.);
#59888=ORIENTED_EDGE('',*,*,#45373,.T.);
#59889=ORIENTED_EDGE('',*,*,#45379,.F.);
#59890=ORIENTED_EDGE('',*,*,#45380,.F.);
#59891=ORIENTED_EDGE('',*,*,#45381,.T.);
#59892=ORIENTED_EDGE('',*,*,#45377,.T.);
#59893=ORIENTED_EDGE('',*,*,#45382,.F.);
#59894=ORIENTED_EDGE('',*,*,#45375,.F.);
#59895=ORIENTED_EDGE('',*,*,#45383,.T.);
#59896=ORIENTED_EDGE('',*,*,#45380,.T.);
#59897=ORIENTED_EDGE('',*,*,#45384,.F.);
#59898=ORIENTED_EDGE('',*,*,#45385,.F.);
#59899=ORIENTED_EDGE('',*,*,#45386,.F.);
#59900=ORIENTED_EDGE('',*,*,#45387,.T.);
#59901=ORIENTED_EDGE('',*,*,#45388,.T.);
#59902=ORIENTED_EDGE('',*,*,#45389,.F.);
#59903=ORIENTED_EDGE('',*,*,#45390,.F.);
#59904=ORIENTED_EDGE('',*,*,#45391,.F.);
#59905=ORIENTED_EDGE('',*,*,#45385,.T.);
#59906=ORIENTED_EDGE('',*,*,#45392,.F.);
#59907=ORIENTED_EDGE('',*,*,#45393,.F.);
#59908=ORIENTED_EDGE('',*,*,#45394,.F.);
#59909=ORIENTED_EDGE('',*,*,#45390,.T.);
#59910=ORIENTED_EDGE('',*,*,#45395,.F.);
#59911=ORIENTED_EDGE('',*,*,#45388,.F.);
#59912=ORIENTED_EDGE('',*,*,#45396,.T.);
#59913=ORIENTED_EDGE('',*,*,#45397,.F.);
#59914=ORIENTED_EDGE('',*,*,#45393,.T.);
#59915=ORIENTED_EDGE('',*,*,#45398,.F.);
#59916=ORIENTED_EDGE('',*,*,#45386,.T.);
#59917=ORIENTED_EDGE('',*,*,#45391,.T.);
#59918=ORIENTED_EDGE('',*,*,#45394,.T.);
#59919=ORIENTED_EDGE('',*,*,#45397,.T.);
#59920=ORIENTED_EDGE('',*,*,#45399,.T.);
#59921=ORIENTED_EDGE('',*,*,#45400,.F.);
#59922=ORIENTED_EDGE('',*,*,#45401,.F.);
#59923=ORIENTED_EDGE('',*,*,#45402,.T.);
#59924=ORIENTED_EDGE('',*,*,#45403,.T.);
#59925=ORIENTED_EDGE('',*,*,#45404,.F.);
#59926=ORIENTED_EDGE('',*,*,#45405,.F.);
#59927=ORIENTED_EDGE('',*,*,#45406,.F.);
#59928=ORIENTED_EDGE('',*,*,#45400,.T.);
#59929=ORIENTED_EDGE('',*,*,#45407,.F.);
#59930=ORIENTED_EDGE('',*,*,#45408,.F.);
#59931=ORIENTED_EDGE('',*,*,#45409,.F.);
#59932=ORIENTED_EDGE('',*,*,#45405,.T.);
#59933=ORIENTED_EDGE('',*,*,#45410,.F.);
#59934=ORIENTED_EDGE('',*,*,#45403,.F.);
#59935=ORIENTED_EDGE('',*,*,#45411,.T.);
#59936=ORIENTED_EDGE('',*,*,#45412,.F.);
#59937=ORIENTED_EDGE('',*,*,#45408,.T.);
#59938=ORIENTED_EDGE('',*,*,#45413,.F.);
#59939=ORIENTED_EDGE('',*,*,#45401,.T.);
#59940=ORIENTED_EDGE('',*,*,#45406,.T.);
#59941=ORIENTED_EDGE('',*,*,#45409,.T.);
#59942=ORIENTED_EDGE('',*,*,#45412,.T.);
#59943=ORIENTED_EDGE('',*,*,#45414,.T.);
#59944=ORIENTED_EDGE('',*,*,#45415,.F.);
#59945=ORIENTED_EDGE('',*,*,#45416,.T.);
#59946=ORIENTED_EDGE('',*,*,#45417,.T.);
#59947=ORIENTED_EDGE('',*,*,#45418,.F.);
#59948=ORIENTED_EDGE('',*,*,#45419,.F.);
#59949=ORIENTED_EDGE('',*,*,#45420,.T.);
#59950=ORIENTED_EDGE('',*,*,#45415,.T.);
#59951=ORIENTED_EDGE('',*,*,#45421,.F.);
#59952=ORIENTED_EDGE('',*,*,#45422,.F.);
#59953=ORIENTED_EDGE('',*,*,#45423,.T.);
#59954=ORIENTED_EDGE('',*,*,#45419,.T.);
#59955=ORIENTED_EDGE('',*,*,#45424,.F.);
#59956=ORIENTED_EDGE('',*,*,#45417,.F.);
#59957=ORIENTED_EDGE('',*,*,#45425,.T.);
#59958=ORIENTED_EDGE('',*,*,#45422,.T.);
#59959=ORIENTED_EDGE('',*,*,#45426,.F.);
#59960=ORIENTED_EDGE('',*,*,#45427,.F.);
#59961=ORIENTED_EDGE('',*,*,#45428,.T.);
#59962=ORIENTED_EDGE('',*,*,#45429,.T.);
#59963=ORIENTED_EDGE('',*,*,#45430,.F.);
#59964=ORIENTED_EDGE('',*,*,#45431,.F.);
#59965=ORIENTED_EDGE('',*,*,#45432,.T.);
#59966=ORIENTED_EDGE('',*,*,#45427,.T.);
#59967=ORIENTED_EDGE('',*,*,#45433,.F.);
#59968=ORIENTED_EDGE('',*,*,#45434,.F.);
#59969=ORIENTED_EDGE('',*,*,#45435,.T.);
#59970=ORIENTED_EDGE('',*,*,#45431,.T.);
#59971=ORIENTED_EDGE('',*,*,#45436,.F.);
#59972=ORIENTED_EDGE('',*,*,#45429,.F.);
#59973=ORIENTED_EDGE('',*,*,#45437,.T.);
#59974=ORIENTED_EDGE('',*,*,#45434,.T.);
#59975=ORIENTED_EDGE('',*,*,#45438,.F.);
#59976=ORIENTED_EDGE('',*,*,#45439,.F.);
#59977=ORIENTED_EDGE('',*,*,#45440,.T.);
#59978=ORIENTED_EDGE('',*,*,#45441,.T.);
#59979=ORIENTED_EDGE('',*,*,#45442,.F.);
#59980=ORIENTED_EDGE('',*,*,#45443,.F.);
#59981=ORIENTED_EDGE('',*,*,#45444,.T.);
#59982=ORIENTED_EDGE('',*,*,#45439,.T.);
#59983=ORIENTED_EDGE('',*,*,#45445,.F.);
#59984=ORIENTED_EDGE('',*,*,#45446,.F.);
#59985=ORIENTED_EDGE('',*,*,#45447,.T.);
#59986=ORIENTED_EDGE('',*,*,#45443,.T.);
#59987=ORIENTED_EDGE('',*,*,#45448,.F.);
#59988=ORIENTED_EDGE('',*,*,#45441,.F.);
#59989=ORIENTED_EDGE('',*,*,#45449,.T.);
#59990=ORIENTED_EDGE('',*,*,#45446,.T.);
#59991=ORIENTED_EDGE('',*,*,#45450,.F.);
#59992=ORIENTED_EDGE('',*,*,#45451,.F.);
#59993=ORIENTED_EDGE('',*,*,#45452,.T.);
#59994=ORIENTED_EDGE('',*,*,#45453,.T.);
#59995=ORIENTED_EDGE('',*,*,#45454,.F.);
#59996=ORIENTED_EDGE('',*,*,#45455,.F.);
#59997=ORIENTED_EDGE('',*,*,#45456,.T.);
#59998=ORIENTED_EDGE('',*,*,#45451,.T.);
#59999=ORIENTED_EDGE('',*,*,#45457,.F.);
#60000=ORIENTED_EDGE('',*,*,#45458,.F.);
#60001=ORIENTED_EDGE('',*,*,#45459,.T.);
#60002=ORIENTED_EDGE('',*,*,#45455,.T.);
#60003=ORIENTED_EDGE('',*,*,#45460,.F.);
#60004=ORIENTED_EDGE('',*,*,#45453,.F.);
#60005=ORIENTED_EDGE('',*,*,#45461,.T.);
#60006=ORIENTED_EDGE('',*,*,#45458,.T.);
#60007=ORIENTED_EDGE('',*,*,#45462,.F.);
#60008=ORIENTED_EDGE('',*,*,#45463,.F.);
#60009=ORIENTED_EDGE('',*,*,#45464,.T.);
#60010=ORIENTED_EDGE('',*,*,#45465,.T.);
#60011=ORIENTED_EDGE('',*,*,#45466,.F.);
#60012=ORIENTED_EDGE('',*,*,#45467,.F.);
#60013=ORIENTED_EDGE('',*,*,#45468,.T.);
#60014=ORIENTED_EDGE('',*,*,#45463,.T.);
#60015=ORIENTED_EDGE('',*,*,#45469,.F.);
#60016=ORIENTED_EDGE('',*,*,#45470,.F.);
#60017=ORIENTED_EDGE('',*,*,#45471,.F.);
#60018=ORIENTED_EDGE('',*,*,#45472,.T.);
#60019=ORIENTED_EDGE('',*,*,#45467,.T.);
#60020=ORIENTED_EDGE('',*,*,#45473,.F.);
#60021=ORIENTED_EDGE('',*,*,#45465,.F.);
#60022=ORIENTED_EDGE('',*,*,#45474,.T.);
#60023=ORIENTED_EDGE('',*,*,#45475,.F.);
#60024=ORIENTED_EDGE('',*,*,#45470,.T.);
#60025=ORIENTED_EDGE('',*,*,#45476,.F.);
#60026=ORIENTED_EDGE('',*,*,#45471,.T.);
#60027=ORIENTED_EDGE('',*,*,#45475,.T.);
#60028=ORIENTED_EDGE('',*,*,#45477,.T.);
#60029=ORIENTED_EDGE('',*,*,#45478,.F.);
#60030=ORIENTED_EDGE('',*,*,#45479,.T.);
#60031=ORIENTED_EDGE('',*,*,#45480,.T.);
#60032=ORIENTED_EDGE('',*,*,#45481,.F.);
#60033=ORIENTED_EDGE('',*,*,#45482,.F.);
#60034=ORIENTED_EDGE('',*,*,#45483,.F.);
#60035=ORIENTED_EDGE('',*,*,#45484,.T.);
#60036=ORIENTED_EDGE('',*,*,#45478,.T.);
#60037=ORIENTED_EDGE('',*,*,#45485,.F.);
#60038=ORIENTED_EDGE('',*,*,#45486,.F.);
#60039=ORIENTED_EDGE('',*,*,#45487,.F.);
#60040=ORIENTED_EDGE('',*,*,#45482,.T.);
#60041=ORIENTED_EDGE('',*,*,#45488,.F.);
#60042=ORIENTED_EDGE('',*,*,#45480,.F.);
#60043=ORIENTED_EDGE('',*,*,#45489,.T.);
#60044=ORIENTED_EDGE('',*,*,#45490,.F.);
#60045=ORIENTED_EDGE('',*,*,#45486,.T.);
#60046=ORIENTED_EDGE('',*,*,#45491,.F.);
#60047=ORIENTED_EDGE('',*,*,#45483,.T.);
#60048=ORIENTED_EDGE('',*,*,#45487,.T.);
#60049=ORIENTED_EDGE('',*,*,#45490,.T.);
#60050=ORIENTED_EDGE('',*,*,#45492,.T.);
#60051=ORIENTED_EDGE('',*,*,#45493,.F.);
#60052=ORIENTED_EDGE('',*,*,#45494,.T.);
#60053=ORIENTED_EDGE('',*,*,#45495,.T.);
#60054=ORIENTED_EDGE('',*,*,#45496,.F.);
#60055=ORIENTED_EDGE('',*,*,#45497,.F.);
#60056=ORIENTED_EDGE('',*,*,#45498,.F.);
#60057=ORIENTED_EDGE('',*,*,#45499,.T.);
#60058=ORIENTED_EDGE('',*,*,#45493,.T.);
#60059=ORIENTED_EDGE('',*,*,#45500,.F.);
#60060=ORIENTED_EDGE('',*,*,#45501,.F.);
#60061=ORIENTED_EDGE('',*,*,#45502,.F.);
#60062=ORIENTED_EDGE('',*,*,#45497,.T.);
#60063=ORIENTED_EDGE('',*,*,#45503,.F.);
#60064=ORIENTED_EDGE('',*,*,#45495,.F.);
#60065=ORIENTED_EDGE('',*,*,#45504,.T.);
#60066=ORIENTED_EDGE('',*,*,#45505,.F.);
#60067=ORIENTED_EDGE('',*,*,#45501,.T.);
#60068=ORIENTED_EDGE('',*,*,#45506,.F.);
#60069=ORIENTED_EDGE('',*,*,#45498,.T.);
#60070=ORIENTED_EDGE('',*,*,#45502,.T.);
#60071=ORIENTED_EDGE('',*,*,#45505,.T.);
#60072=ORIENTED_EDGE('',*,*,#45507,.T.);
#60073=ORIENTED_EDGE('',*,*,#45508,.F.);
#60074=ORIENTED_EDGE('',*,*,#45509,.T.);
#60075=ORIENTED_EDGE('',*,*,#45510,.T.);
#60076=ORIENTED_EDGE('',*,*,#45511,.F.);
#60077=ORIENTED_EDGE('',*,*,#45512,.F.);
#60078=ORIENTED_EDGE('',*,*,#45513,.T.);
#60079=ORIENTED_EDGE('',*,*,#45508,.T.);
#60080=ORIENTED_EDGE('',*,*,#45514,.F.);
#60081=ORIENTED_EDGE('',*,*,#45515,.F.);
#60082=ORIENTED_EDGE('',*,*,#45516,.F.);
#60083=ORIENTED_EDGE('',*,*,#45517,.T.);
#60084=ORIENTED_EDGE('',*,*,#45512,.T.);
#60085=ORIENTED_EDGE('',*,*,#45518,.F.);
#60086=ORIENTED_EDGE('',*,*,#45510,.F.);
#60087=ORIENTED_EDGE('',*,*,#45519,.T.);
#60088=ORIENTED_EDGE('',*,*,#45520,.F.);
#60089=ORIENTED_EDGE('',*,*,#45515,.T.);
#60090=ORIENTED_EDGE('',*,*,#45521,.F.);
#60091=ORIENTED_EDGE('',*,*,#45516,.T.);
#60092=ORIENTED_EDGE('',*,*,#45520,.T.);
#60093=ORIENTED_EDGE('',*,*,#45522,.T.);
#60094=ORIENTED_EDGE('',*,*,#45523,.F.);
#60095=ORIENTED_EDGE('',*,*,#45524,.T.);
#60096=ORIENTED_EDGE('',*,*,#45525,.T.);
#60097=ORIENTED_EDGE('',*,*,#45526,.F.);
#60098=ORIENTED_EDGE('',*,*,#45527,.F.);
#60099=ORIENTED_EDGE('',*,*,#45528,.T.);
#60100=ORIENTED_EDGE('',*,*,#45523,.T.);
#60101=ORIENTED_EDGE('',*,*,#45529,.F.);
#60102=ORIENTED_EDGE('',*,*,#45530,.F.);
#60103=ORIENTED_EDGE('',*,*,#45531,.T.);
#60104=ORIENTED_EDGE('',*,*,#45527,.T.);
#60105=ORIENTED_EDGE('',*,*,#45532,.F.);
#60106=ORIENTED_EDGE('',*,*,#45525,.F.);
#60107=ORIENTED_EDGE('',*,*,#45533,.T.);
#60108=ORIENTED_EDGE('',*,*,#45530,.T.);
#60109=ORIENTED_EDGE('',*,*,#45534,.F.);
#60110=ORIENTED_EDGE('',*,*,#45535,.F.);
#60111=ORIENTED_EDGE('',*,*,#45536,.T.);
#60112=ORIENTED_EDGE('',*,*,#45537,.T.);
#60113=ORIENTED_EDGE('',*,*,#45538,.F.);
#60114=ORIENTED_EDGE('',*,*,#45539,.F.);
#60115=ORIENTED_EDGE('',*,*,#45540,.T.);
#60116=ORIENTED_EDGE('',*,*,#45535,.T.);
#60117=ORIENTED_EDGE('',*,*,#45541,.F.);
#60118=ORIENTED_EDGE('',*,*,#45542,.F.);
#60119=ORIENTED_EDGE('',*,*,#45543,.T.);
#60120=ORIENTED_EDGE('',*,*,#45539,.T.);
#60121=ORIENTED_EDGE('',*,*,#45544,.F.);
#60122=ORIENTED_EDGE('',*,*,#45537,.F.);
#60123=ORIENTED_EDGE('',*,*,#45545,.T.);
#60124=ORIENTED_EDGE('',*,*,#45542,.T.);
#60125=ORIENTED_EDGE('',*,*,#45546,.F.);
#60126=ORIENTED_EDGE('',*,*,#45547,.F.);
#60127=ORIENTED_EDGE('',*,*,#45548,.T.);
#60128=ORIENTED_EDGE('',*,*,#45549,.T.);
#60129=ORIENTED_EDGE('',*,*,#45550,.F.);
#60130=ORIENTED_EDGE('',*,*,#45551,.F.);
#60131=ORIENTED_EDGE('',*,*,#45552,.T.);
#60132=ORIENTED_EDGE('',*,*,#45547,.T.);
#60133=ORIENTED_EDGE('',*,*,#45553,.F.);
#60134=ORIENTED_EDGE('',*,*,#45554,.F.);
#60135=ORIENTED_EDGE('',*,*,#45555,.T.);
#60136=ORIENTED_EDGE('',*,*,#45551,.T.);
#60137=ORIENTED_EDGE('',*,*,#45556,.F.);
#60138=ORIENTED_EDGE('',*,*,#45549,.F.);
#60139=ORIENTED_EDGE('',*,*,#45557,.T.);
#60140=ORIENTED_EDGE('',*,*,#45554,.T.);
#60141=ORIENTED_EDGE('',*,*,#45558,.F.);
#60142=ORIENTED_EDGE('',*,*,#45559,.F.);
#60143=ORIENTED_EDGE('',*,*,#45560,.T.);
#60144=ORIENTED_EDGE('',*,*,#45561,.T.);
#60145=ORIENTED_EDGE('',*,*,#45562,.F.);
#60146=ORIENTED_EDGE('',*,*,#45563,.F.);
#60147=ORIENTED_EDGE('',*,*,#45564,.T.);
#60148=ORIENTED_EDGE('',*,*,#45559,.T.);
#60149=ORIENTED_EDGE('',*,*,#45565,.F.);
#60150=ORIENTED_EDGE('',*,*,#45566,.F.);
#60151=ORIENTED_EDGE('',*,*,#45567,.T.);
#60152=ORIENTED_EDGE('',*,*,#45563,.T.);
#60153=ORIENTED_EDGE('',*,*,#45568,.F.);
#60154=ORIENTED_EDGE('',*,*,#45561,.F.);
#60155=ORIENTED_EDGE('',*,*,#45569,.T.);
#60156=ORIENTED_EDGE('',*,*,#45566,.T.);
#60157=ORIENTED_EDGE('',*,*,#45570,.F.);
#60158=ORIENTED_EDGE('',*,*,#45571,.F.);
#60159=ORIENTED_EDGE('',*,*,#45572,.T.);
#60160=ORIENTED_EDGE('',*,*,#45573,.T.);
#60161=ORIENTED_EDGE('',*,*,#45574,.F.);
#60162=ORIENTED_EDGE('',*,*,#45575,.F.);
#60163=ORIENTED_EDGE('',*,*,#45576,.T.);
#60164=ORIENTED_EDGE('',*,*,#45571,.T.);
#60165=ORIENTED_EDGE('',*,*,#45577,.F.);
#60166=ORIENTED_EDGE('',*,*,#45578,.F.);
#60167=ORIENTED_EDGE('',*,*,#45579,.T.);
#60168=ORIENTED_EDGE('',*,*,#45575,.T.);
#60169=ORIENTED_EDGE('',*,*,#45580,.F.);
#60170=ORIENTED_EDGE('',*,*,#45573,.F.);
#60171=ORIENTED_EDGE('',*,*,#45581,.T.);
#60172=ORIENTED_EDGE('',*,*,#45578,.T.);
#60173=ORIENTED_EDGE('',*,*,#45582,.F.);
#60174=ORIENTED_EDGE('',*,*,#45583,.F.);
#60175=ORIENTED_EDGE('',*,*,#45584,.T.);
#60176=ORIENTED_EDGE('',*,*,#45585,.T.);
#60177=ORIENTED_EDGE('',*,*,#45586,.F.);
#60178=ORIENTED_EDGE('',*,*,#45587,.F.);
#60179=ORIENTED_EDGE('',*,*,#45588,.T.);
#60180=ORIENTED_EDGE('',*,*,#45583,.T.);
#60181=ORIENTED_EDGE('',*,*,#45589,.F.);
#60182=ORIENTED_EDGE('',*,*,#45590,.F.);
#60183=ORIENTED_EDGE('',*,*,#45591,.T.);
#60184=ORIENTED_EDGE('',*,*,#45587,.T.);
#60185=ORIENTED_EDGE('',*,*,#45592,.F.);
#60186=ORIENTED_EDGE('',*,*,#45585,.F.);
#60187=ORIENTED_EDGE('',*,*,#45593,.T.);
#60188=ORIENTED_EDGE('',*,*,#45590,.T.);
#60189=ORIENTED_EDGE('',*,*,#45594,.F.);
#60190=ORIENTED_EDGE('',*,*,#45595,.F.);
#60191=ORIENTED_EDGE('',*,*,#45596,.T.);
#60192=ORIENTED_EDGE('',*,*,#45597,.T.);
#60193=ORIENTED_EDGE('',*,*,#45598,.F.);
#60194=ORIENTED_EDGE('',*,*,#45599,.F.);
#60195=ORIENTED_EDGE('',*,*,#45600,.T.);
#60196=ORIENTED_EDGE('',*,*,#45595,.T.);
#60197=ORIENTED_EDGE('',*,*,#45601,.F.);
#60198=ORIENTED_EDGE('',*,*,#45602,.F.);
#60199=ORIENTED_EDGE('',*,*,#45603,.T.);
#60200=ORIENTED_EDGE('',*,*,#45599,.T.);
#60201=ORIENTED_EDGE('',*,*,#45604,.F.);
#60202=ORIENTED_EDGE('',*,*,#45597,.F.);
#60203=ORIENTED_EDGE('',*,*,#45605,.T.);
#60204=ORIENTED_EDGE('',*,*,#45602,.T.);
#60205=ORIENTED_EDGE('',*,*,#45606,.F.);
#60206=ORIENTED_EDGE('',*,*,#45607,.F.);
#60207=ORIENTED_EDGE('',*,*,#45608,.T.);
#60208=ORIENTED_EDGE('',*,*,#45609,.T.);
#60209=ORIENTED_EDGE('',*,*,#45610,.F.);
#60210=ORIENTED_EDGE('',*,*,#45611,.F.);
#60211=ORIENTED_EDGE('',*,*,#45612,.T.);
#60212=ORIENTED_EDGE('',*,*,#45607,.T.);
#60213=ORIENTED_EDGE('',*,*,#45613,.F.);
#60214=ORIENTED_EDGE('',*,*,#45614,.F.);
#60215=ORIENTED_EDGE('',*,*,#45615,.T.);
#60216=ORIENTED_EDGE('',*,*,#45611,.T.);
#60217=ORIENTED_EDGE('',*,*,#45616,.F.);
#60218=ORIENTED_EDGE('',*,*,#45609,.F.);
#60219=ORIENTED_EDGE('',*,*,#45617,.T.);
#60220=ORIENTED_EDGE('',*,*,#45614,.T.);
#60221=ORIENTED_EDGE('',*,*,#45618,.F.);
#60222=ORIENTED_EDGE('',*,*,#45619,.F.);
#60223=ORIENTED_EDGE('',*,*,#45620,.T.);
#60224=ORIENTED_EDGE('',*,*,#45621,.T.);
#60225=ORIENTED_EDGE('',*,*,#45622,.F.);
#60226=ORIENTED_EDGE('',*,*,#45623,.F.);
#60227=ORIENTED_EDGE('',*,*,#45624,.T.);
#60228=ORIENTED_EDGE('',*,*,#45619,.T.);
#60229=ORIENTED_EDGE('',*,*,#45625,.F.);
#60230=ORIENTED_EDGE('',*,*,#45626,.F.);
#60231=ORIENTED_EDGE('',*,*,#45627,.T.);
#60232=ORIENTED_EDGE('',*,*,#45623,.T.);
#60233=ORIENTED_EDGE('',*,*,#45628,.F.);
#60234=ORIENTED_EDGE('',*,*,#45621,.F.);
#60235=ORIENTED_EDGE('',*,*,#45629,.T.);
#60236=ORIENTED_EDGE('',*,*,#45626,.T.);
#60237=ORIENTED_EDGE('',*,*,#45630,.F.);
#60238=ORIENTED_EDGE('',*,*,#45631,.F.);
#60239=ORIENTED_EDGE('',*,*,#45632,.T.);
#60240=ORIENTED_EDGE('',*,*,#45633,.T.);
#60241=ORIENTED_EDGE('',*,*,#45634,.F.);
#60242=ORIENTED_EDGE('',*,*,#45635,.F.);
#60243=ORIENTED_EDGE('',*,*,#45636,.T.);
#60244=ORIENTED_EDGE('',*,*,#45631,.T.);
#60245=ORIENTED_EDGE('',*,*,#45637,.F.);
#60246=ORIENTED_EDGE('',*,*,#45638,.F.);
#60247=ORIENTED_EDGE('',*,*,#45639,.T.);
#60248=ORIENTED_EDGE('',*,*,#45635,.T.);
#60249=ORIENTED_EDGE('',*,*,#45640,.F.);
#60250=ORIENTED_EDGE('',*,*,#45633,.F.);
#60251=ORIENTED_EDGE('',*,*,#45641,.T.);
#60252=ORIENTED_EDGE('',*,*,#45638,.T.);
#60253=ORIENTED_EDGE('',*,*,#45642,.F.);
#60254=ORIENTED_EDGE('',*,*,#45643,.F.);
#60255=ORIENTED_EDGE('',*,*,#45644,.T.);
#60256=ORIENTED_EDGE('',*,*,#45645,.T.);
#60257=ORIENTED_EDGE('',*,*,#45646,.F.);
#60258=ORIENTED_EDGE('',*,*,#45647,.F.);
#60259=ORIENTED_EDGE('',*,*,#45648,.T.);
#60260=ORIENTED_EDGE('',*,*,#45643,.T.);
#60261=ORIENTED_EDGE('',*,*,#45649,.F.);
#60262=ORIENTED_EDGE('',*,*,#45650,.F.);
#60263=ORIENTED_EDGE('',*,*,#45651,.F.);
#60264=ORIENTED_EDGE('',*,*,#45652,.T.);
#60265=ORIENTED_EDGE('',*,*,#45647,.T.);
#60266=ORIENTED_EDGE('',*,*,#45653,.F.);
#60267=ORIENTED_EDGE('',*,*,#45645,.F.);
#60268=ORIENTED_EDGE('',*,*,#45654,.T.);
#60269=ORIENTED_EDGE('',*,*,#45655,.F.);
#60270=ORIENTED_EDGE('',*,*,#45650,.T.);
#60271=ORIENTED_EDGE('',*,*,#45656,.F.);
#60272=ORIENTED_EDGE('',*,*,#45651,.T.);
#60273=ORIENTED_EDGE('',*,*,#45655,.T.);
#60274=ORIENTED_EDGE('',*,*,#45657,.T.);
#60275=ORIENTED_EDGE('',*,*,#45658,.F.);
#60276=ORIENTED_EDGE('',*,*,#45659,.T.);
#60277=ORIENTED_EDGE('',*,*,#45660,.T.);
#60278=ORIENTED_EDGE('',*,*,#45661,.F.);
#60279=ORIENTED_EDGE('',*,*,#45662,.F.);
#60280=ORIENTED_EDGE('',*,*,#45663,.T.);
#60281=ORIENTED_EDGE('',*,*,#45658,.T.);
#60282=ORIENTED_EDGE('',*,*,#45664,.F.);
#60283=ORIENTED_EDGE('',*,*,#45665,.F.);
#60284=ORIENTED_EDGE('',*,*,#45666,.F.);
#60285=ORIENTED_EDGE('',*,*,#45667,.T.);
#60286=ORIENTED_EDGE('',*,*,#45662,.T.);
#60287=ORIENTED_EDGE('',*,*,#45668,.F.);
#60288=ORIENTED_EDGE('',*,*,#45660,.F.);
#60289=ORIENTED_EDGE('',*,*,#45669,.T.);
#60290=ORIENTED_EDGE('',*,*,#45670,.F.);
#60291=ORIENTED_EDGE('',*,*,#45665,.T.);
#60292=ORIENTED_EDGE('',*,*,#45671,.F.);
#60293=ORIENTED_EDGE('',*,*,#45666,.T.);
#60294=ORIENTED_EDGE('',*,*,#45670,.T.);
#60295=ORIENTED_EDGE('',*,*,#45672,.T.);
#60296=ORIENTED_EDGE('',*,*,#45673,.F.);
#60297=ORIENTED_EDGE('',*,*,#45674,.T.);
#60298=ORIENTED_EDGE('',*,*,#45675,.T.);
#60299=ORIENTED_EDGE('',*,*,#45676,.F.);
#60300=ORIENTED_EDGE('',*,*,#45677,.F.);
#60301=ORIENTED_EDGE('',*,*,#45678,.T.);
#60302=ORIENTED_EDGE('',*,*,#45673,.T.);
#60303=ORIENTED_EDGE('',*,*,#45679,.F.);
#60304=ORIENTED_EDGE('',*,*,#45680,.F.);
#60305=ORIENTED_EDGE('',*,*,#45681,.T.);
#60306=ORIENTED_EDGE('',*,*,#45677,.T.);
#60307=ORIENTED_EDGE('',*,*,#45682,.F.);
#60308=ORIENTED_EDGE('',*,*,#45675,.F.);
#60309=ORIENTED_EDGE('',*,*,#45683,.T.);
#60310=ORIENTED_EDGE('',*,*,#45680,.T.);
#60311=ORIENTED_EDGE('',*,*,#45684,.F.);
#60312=ORIENTED_EDGE('',*,*,#45685,.F.);
#60313=ORIENTED_EDGE('',*,*,#45686,.T.);
#60314=ORIENTED_EDGE('',*,*,#45687,.T.);
#60315=ORIENTED_EDGE('',*,*,#45688,.F.);
#60316=ORIENTED_EDGE('',*,*,#45689,.F.);
#60317=ORIENTED_EDGE('',*,*,#45690,.T.);
#60318=ORIENTED_EDGE('',*,*,#45685,.T.);
#60319=ORIENTED_EDGE('',*,*,#45691,.F.);
#60320=ORIENTED_EDGE('',*,*,#45692,.F.);
#60321=ORIENTED_EDGE('',*,*,#45693,.T.);
#60322=ORIENTED_EDGE('',*,*,#45689,.T.);
#60323=ORIENTED_EDGE('',*,*,#45694,.F.);
#60324=ORIENTED_EDGE('',*,*,#45687,.F.);
#60325=ORIENTED_EDGE('',*,*,#45695,.T.);
#60326=ORIENTED_EDGE('',*,*,#45692,.T.);
#60327=ORIENTED_EDGE('',*,*,#45696,.F.);
#60328=ORIENTED_EDGE('',*,*,#45697,.F.);
#60329=ORIENTED_EDGE('',*,*,#45698,.T.);
#60330=ORIENTED_EDGE('',*,*,#45699,.T.);
#60331=ORIENTED_EDGE('',*,*,#45700,.F.);
#60332=ORIENTED_EDGE('',*,*,#45701,.F.);
#60333=ORIENTED_EDGE('',*,*,#45702,.T.);
#60334=ORIENTED_EDGE('',*,*,#45697,.T.);
#60335=ORIENTED_EDGE('',*,*,#45703,.F.);
#60336=ORIENTED_EDGE('',*,*,#45704,.F.);
#60337=ORIENTED_EDGE('',*,*,#45705,.T.);
#60338=ORIENTED_EDGE('',*,*,#45701,.T.);
#60339=ORIENTED_EDGE('',*,*,#45706,.F.);
#60340=ORIENTED_EDGE('',*,*,#45699,.F.);
#60341=ORIENTED_EDGE('',*,*,#45707,.T.);
#60342=ORIENTED_EDGE('',*,*,#45704,.T.);
#60343=ORIENTED_EDGE('',*,*,#45708,.F.);
#60344=ORIENTED_EDGE('',*,*,#45709,.F.);
#60345=ORIENTED_EDGE('',*,*,#45710,.T.);
#60346=ORIENTED_EDGE('',*,*,#45711,.T.);
#60347=ORIENTED_EDGE('',*,*,#45712,.F.);
#60348=ORIENTED_EDGE('',*,*,#45713,.F.);
#60349=ORIENTED_EDGE('',*,*,#45714,.T.);
#60350=ORIENTED_EDGE('',*,*,#45709,.T.);
#60351=ORIENTED_EDGE('',*,*,#45715,.F.);
#60352=ORIENTED_EDGE('',*,*,#45716,.F.);
#60353=ORIENTED_EDGE('',*,*,#45717,.T.);
#60354=ORIENTED_EDGE('',*,*,#45713,.T.);
#60355=ORIENTED_EDGE('',*,*,#45718,.F.);
#60356=ORIENTED_EDGE('',*,*,#45711,.F.);
#60357=ORIENTED_EDGE('',*,*,#45719,.T.);
#60358=ORIENTED_EDGE('',*,*,#45716,.T.);
#60359=ORIENTED_EDGE('',*,*,#45720,.F.);
#60360=ORIENTED_EDGE('',*,*,#45721,.F.);
#60361=ORIENTED_EDGE('',*,*,#45722,.T.);
#60362=ORIENTED_EDGE('',*,*,#45723,.T.);
#60363=ORIENTED_EDGE('',*,*,#45724,.F.);
#60364=ORIENTED_EDGE('',*,*,#45725,.F.);
#60365=ORIENTED_EDGE('',*,*,#45726,.T.);
#60366=ORIENTED_EDGE('',*,*,#45721,.T.);
#60367=ORIENTED_EDGE('',*,*,#45727,.F.);
#60368=ORIENTED_EDGE('',*,*,#45728,.F.);
#60369=ORIENTED_EDGE('',*,*,#45729,.T.);
#60370=ORIENTED_EDGE('',*,*,#45725,.T.);
#60371=ORIENTED_EDGE('',*,*,#45730,.F.);
#60372=ORIENTED_EDGE('',*,*,#45723,.F.);
#60373=ORIENTED_EDGE('',*,*,#45731,.T.);
#60374=ORIENTED_EDGE('',*,*,#45728,.T.);
#60375=ORIENTED_EDGE('',*,*,#45732,.F.);
#60376=ORIENTED_EDGE('',*,*,#45733,.F.);
#60377=ORIENTED_EDGE('',*,*,#45734,.T.);
#60378=ORIENTED_EDGE('',*,*,#45735,.T.);
#60379=ORIENTED_EDGE('',*,*,#45736,.F.);
#60380=ORIENTED_EDGE('',*,*,#45737,.F.);
#60381=ORIENTED_EDGE('',*,*,#45738,.T.);
#60382=ORIENTED_EDGE('',*,*,#45733,.T.);
#60383=ORIENTED_EDGE('',*,*,#45739,.F.);
#60384=ORIENTED_EDGE('',*,*,#45740,.F.);
#60385=ORIENTED_EDGE('',*,*,#45741,.T.);
#60386=ORIENTED_EDGE('',*,*,#45737,.T.);
#60387=ORIENTED_EDGE('',*,*,#45742,.F.);
#60388=ORIENTED_EDGE('',*,*,#45735,.F.);
#60389=ORIENTED_EDGE('',*,*,#45743,.T.);
#60390=ORIENTED_EDGE('',*,*,#45740,.T.);
#60391=ORIENTED_EDGE('',*,*,#45744,.F.);
#60392=ORIENTED_EDGE('',*,*,#45745,.F.);
#60393=ORIENTED_EDGE('',*,*,#45746,.T.);
#60394=ORIENTED_EDGE('',*,*,#45747,.T.);
#60395=ORIENTED_EDGE('',*,*,#45748,.F.);
#60396=ORIENTED_EDGE('',*,*,#45749,.F.);
#60397=ORIENTED_EDGE('',*,*,#45750,.T.);
#60398=ORIENTED_EDGE('',*,*,#45745,.T.);
#60399=ORIENTED_EDGE('',*,*,#45751,.F.);
#60400=ORIENTED_EDGE('',*,*,#45752,.F.);
#60401=ORIENTED_EDGE('',*,*,#45753,.T.);
#60402=ORIENTED_EDGE('',*,*,#45749,.T.);
#60403=ORIENTED_EDGE('',*,*,#45754,.F.);
#60404=ORIENTED_EDGE('',*,*,#45747,.F.);
#60405=ORIENTED_EDGE('',*,*,#45755,.T.);
#60406=ORIENTED_EDGE('',*,*,#45752,.T.);
#60407=ORIENTED_EDGE('',*,*,#45756,.F.);
#60408=ORIENTED_EDGE('',*,*,#45757,.F.);
#60409=ORIENTED_EDGE('',*,*,#45758,.T.);
#60410=ORIENTED_EDGE('',*,*,#45759,.T.);
#60411=ORIENTED_EDGE('',*,*,#45760,.F.);
#60412=ORIENTED_EDGE('',*,*,#45761,.F.);
#60413=ORIENTED_EDGE('',*,*,#45762,.T.);
#60414=ORIENTED_EDGE('',*,*,#45757,.T.);
#60415=ORIENTED_EDGE('',*,*,#45763,.F.);
#60416=ORIENTED_EDGE('',*,*,#45764,.F.);
#60417=ORIENTED_EDGE('',*,*,#45765,.T.);
#60418=ORIENTED_EDGE('',*,*,#45761,.T.);
#60419=ORIENTED_EDGE('',*,*,#45766,.F.);
#60420=ORIENTED_EDGE('',*,*,#45759,.F.);
#60421=ORIENTED_EDGE('',*,*,#45767,.T.);
#60422=ORIENTED_EDGE('',*,*,#45764,.T.);
#60423=ORIENTED_EDGE('',*,*,#45768,.F.);
#60424=ORIENTED_EDGE('',*,*,#45769,.F.);
#60425=ORIENTED_EDGE('',*,*,#45770,.T.);
#60426=ORIENTED_EDGE('',*,*,#45771,.T.);
#60427=ORIENTED_EDGE('',*,*,#45772,.F.);
#60428=ORIENTED_EDGE('',*,*,#45773,.F.);
#60429=ORIENTED_EDGE('',*,*,#45774,.T.);
#60430=ORIENTED_EDGE('',*,*,#45769,.T.);
#60431=ORIENTED_EDGE('',*,*,#45775,.F.);
#60432=ORIENTED_EDGE('',*,*,#45776,.F.);
#60433=ORIENTED_EDGE('',*,*,#45777,.T.);
#60434=ORIENTED_EDGE('',*,*,#45773,.T.);
#60435=ORIENTED_EDGE('',*,*,#45778,.F.);
#60436=ORIENTED_EDGE('',*,*,#45771,.F.);
#60437=ORIENTED_EDGE('',*,*,#45779,.T.);
#60438=ORIENTED_EDGE('',*,*,#45776,.T.);
#60439=ORIENTED_EDGE('',*,*,#45780,.F.);
#60440=ORIENTED_EDGE('',*,*,#45781,.F.);
#60441=ORIENTED_EDGE('',*,*,#45782,.T.);
#60442=ORIENTED_EDGE('',*,*,#45783,.T.);
#60443=ORIENTED_EDGE('',*,*,#45784,.F.);
#60444=ORIENTED_EDGE('',*,*,#45785,.F.);
#60445=ORIENTED_EDGE('',*,*,#45786,.F.);
#60446=ORIENTED_EDGE('',*,*,#45787,.T.);
#60447=ORIENTED_EDGE('',*,*,#45781,.T.);
#60448=ORIENTED_EDGE('',*,*,#45788,.F.);
#60449=ORIENTED_EDGE('',*,*,#45789,.F.);
#60450=ORIENTED_EDGE('',*,*,#45790,.F.);
#60451=ORIENTED_EDGE('',*,*,#45785,.T.);
#60452=ORIENTED_EDGE('',*,*,#45791,.F.);
#60453=ORIENTED_EDGE('',*,*,#45783,.F.);
#60454=ORIENTED_EDGE('',*,*,#45792,.T.);
#60455=ORIENTED_EDGE('',*,*,#45793,.F.);
#60456=ORIENTED_EDGE('',*,*,#45789,.T.);
#60457=ORIENTED_EDGE('',*,*,#45794,.F.);
#60458=ORIENTED_EDGE('',*,*,#45786,.T.);
#60459=ORIENTED_EDGE('',*,*,#45790,.T.);
#60460=ORIENTED_EDGE('',*,*,#45793,.T.);
#60461=ORIENTED_EDGE('',*,*,#45795,.T.);
#60462=ORIENTED_EDGE('',*,*,#45796,.F.);
#60463=ORIENTED_EDGE('',*,*,#45797,.T.);
#60464=ORIENTED_EDGE('',*,*,#45798,.T.);
#60465=ORIENTED_EDGE('',*,*,#45799,.F.);
#60466=ORIENTED_EDGE('',*,*,#45800,.F.);
#60467=ORIENTED_EDGE('',*,*,#45801,.T.);
#60468=ORIENTED_EDGE('',*,*,#45796,.T.);
#60469=ORIENTED_EDGE('',*,*,#45802,.F.);
#60470=ORIENTED_EDGE('',*,*,#45803,.F.);
#60471=ORIENTED_EDGE('',*,*,#45804,.F.);
#60472=ORIENTED_EDGE('',*,*,#45805,.T.);
#60473=ORIENTED_EDGE('',*,*,#45800,.T.);
#60474=ORIENTED_EDGE('',*,*,#45806,.F.);
#60475=ORIENTED_EDGE('',*,*,#45798,.F.);
#60476=ORIENTED_EDGE('',*,*,#45807,.T.);
#60477=ORIENTED_EDGE('',*,*,#45808,.F.);
#60478=ORIENTED_EDGE('',*,*,#45803,.T.);
#60479=ORIENTED_EDGE('',*,*,#45809,.F.);
#60480=ORIENTED_EDGE('',*,*,#45804,.T.);
#60481=ORIENTED_EDGE('',*,*,#45808,.T.);
#60482=ORIENTED_EDGE('',*,*,#45810,.T.);
#60483=ORIENTED_EDGE('',*,*,#45811,.F.);
#60484=ORIENTED_EDGE('',*,*,#45812,.T.);
#60485=ORIENTED_EDGE('',*,*,#45813,.T.);
#60486=ORIENTED_EDGE('',*,*,#45814,.F.);
#60487=ORIENTED_EDGE('',*,*,#45815,.F.);
#60488=ORIENTED_EDGE('',*,*,#45816,.T.);
#60489=ORIENTED_EDGE('',*,*,#45811,.T.);
#60490=ORIENTED_EDGE('',*,*,#45817,.F.);
#60491=ORIENTED_EDGE('',*,*,#45818,.F.);
#60492=ORIENTED_EDGE('',*,*,#45819,.T.);
#60493=ORIENTED_EDGE('',*,*,#45815,.T.);
#60494=ORIENTED_EDGE('',*,*,#45820,.F.);
#60495=ORIENTED_EDGE('',*,*,#45813,.F.);
#60496=ORIENTED_EDGE('',*,*,#45821,.T.);
#60497=ORIENTED_EDGE('',*,*,#45818,.T.);
#60498=ORIENTED_EDGE('',*,*,#45822,.F.);
#60499=ORIENTED_EDGE('',*,*,#45823,.F.);
#60500=ORIENTED_EDGE('',*,*,#45824,.T.);
#60501=ORIENTED_EDGE('',*,*,#45825,.T.);
#60502=ORIENTED_EDGE('',*,*,#45826,.F.);
#60503=ORIENTED_EDGE('',*,*,#45827,.F.);
#60504=ORIENTED_EDGE('',*,*,#45828,.T.);
#60505=ORIENTED_EDGE('',*,*,#45823,.T.);
#60506=ORIENTED_EDGE('',*,*,#45829,.F.);
#60507=ORIENTED_EDGE('',*,*,#45830,.F.);
#60508=ORIENTED_EDGE('',*,*,#45831,.T.);
#60509=ORIENTED_EDGE('',*,*,#45827,.T.);
#60510=ORIENTED_EDGE('',*,*,#45832,.F.);
#60511=ORIENTED_EDGE('',*,*,#45825,.F.);
#60512=ORIENTED_EDGE('',*,*,#45833,.T.);
#60513=ORIENTED_EDGE('',*,*,#45830,.T.);
#60514=ORIENTED_EDGE('',*,*,#45834,.F.);
#60515=ORIENTED_EDGE('',*,*,#45835,.F.);
#60516=ORIENTED_EDGE('',*,*,#45836,.T.);
#60517=ORIENTED_EDGE('',*,*,#45837,.T.);
#60518=ORIENTED_EDGE('',*,*,#45838,.F.);
#60519=ORIENTED_EDGE('',*,*,#45839,.F.);
#60520=ORIENTED_EDGE('',*,*,#45840,.T.);
#60521=ORIENTED_EDGE('',*,*,#45835,.T.);
#60522=ORIENTED_EDGE('',*,*,#45841,.F.);
#60523=ORIENTED_EDGE('',*,*,#45842,.F.);
#60524=ORIENTED_EDGE('',*,*,#45843,.T.);
#60525=ORIENTED_EDGE('',*,*,#45839,.T.);
#60526=ORIENTED_EDGE('',*,*,#45844,.F.);
#60527=ORIENTED_EDGE('',*,*,#45837,.F.);
#60528=ORIENTED_EDGE('',*,*,#45845,.T.);
#60529=ORIENTED_EDGE('',*,*,#45842,.T.);
#60530=ORIENTED_EDGE('',*,*,#45846,.F.);
#60531=ORIENTED_EDGE('',*,*,#45847,.F.);
#60532=ORIENTED_EDGE('',*,*,#45848,.T.);
#60533=ORIENTED_EDGE('',*,*,#45849,.T.);
#60534=ORIENTED_EDGE('',*,*,#45850,.F.);
#60535=ORIENTED_EDGE('',*,*,#45851,.F.);
#60536=ORIENTED_EDGE('',*,*,#45852,.T.);
#60537=ORIENTED_EDGE('',*,*,#45847,.T.);
#60538=ORIENTED_EDGE('',*,*,#45853,.F.);
#60539=ORIENTED_EDGE('',*,*,#45854,.F.);
#60540=ORIENTED_EDGE('',*,*,#45855,.T.);
#60541=ORIENTED_EDGE('',*,*,#45851,.T.);
#60542=ORIENTED_EDGE('',*,*,#45856,.F.);
#60543=ORIENTED_EDGE('',*,*,#45849,.F.);
#60544=ORIENTED_EDGE('',*,*,#45857,.T.);
#60545=ORIENTED_EDGE('',*,*,#45854,.T.);
#60546=ORIENTED_EDGE('',*,*,#45858,.F.);
#60547=ORIENTED_EDGE('',*,*,#45859,.F.);
#60548=ORIENTED_EDGE('',*,*,#45860,.T.);
#60549=ORIENTED_EDGE('',*,*,#45861,.T.);
#60550=ORIENTED_EDGE('',*,*,#45862,.F.);
#60551=ORIENTED_EDGE('',*,*,#45863,.F.);
#60552=ORIENTED_EDGE('',*,*,#45864,.T.);
#60553=ORIENTED_EDGE('',*,*,#45859,.T.);
#60554=ORIENTED_EDGE('',*,*,#45865,.F.);
#60555=ORIENTED_EDGE('',*,*,#45866,.F.);
#60556=ORIENTED_EDGE('',*,*,#45867,.T.);
#60557=ORIENTED_EDGE('',*,*,#45863,.T.);
#60558=ORIENTED_EDGE('',*,*,#45868,.F.);
#60559=ORIENTED_EDGE('',*,*,#45861,.F.);
#60560=ORIENTED_EDGE('',*,*,#45869,.T.);
#60561=ORIENTED_EDGE('',*,*,#45866,.T.);
#60562=ORIENTED_EDGE('',*,*,#45870,.F.);
#60563=ORIENTED_EDGE('',*,*,#45871,.F.);
#60564=ORIENTED_EDGE('',*,*,#45872,.T.);
#60565=ORIENTED_EDGE('',*,*,#45873,.T.);
#60566=ORIENTED_EDGE('',*,*,#45874,.F.);
#60567=ORIENTED_EDGE('',*,*,#45875,.F.);
#60568=ORIENTED_EDGE('',*,*,#45876,.T.);
#60569=ORIENTED_EDGE('',*,*,#45871,.T.);
#60570=ORIENTED_EDGE('',*,*,#45877,.F.);
#60571=ORIENTED_EDGE('',*,*,#45878,.F.);
#60572=ORIENTED_EDGE('',*,*,#45879,.T.);
#60573=ORIENTED_EDGE('',*,*,#45875,.T.);
#60574=ORIENTED_EDGE('',*,*,#45880,.F.);
#60575=ORIENTED_EDGE('',*,*,#45873,.F.);
#60576=ORIENTED_EDGE('',*,*,#45881,.T.);
#60577=ORIENTED_EDGE('',*,*,#45878,.T.);
#60578=ORIENTED_EDGE('',*,*,#45882,.F.);
#60579=ORIENTED_EDGE('',*,*,#45883,.F.);
#60580=ORIENTED_EDGE('',*,*,#45884,.T.);
#60581=ORIENTED_EDGE('',*,*,#45885,.T.);
#60582=ORIENTED_EDGE('',*,*,#45886,.F.);
#60583=ORIENTED_EDGE('',*,*,#45887,.F.);
#60584=ORIENTED_EDGE('',*,*,#45888,.T.);
#60585=ORIENTED_EDGE('',*,*,#45883,.T.);
#60586=ORIENTED_EDGE('',*,*,#45889,.F.);
#60587=ORIENTED_EDGE('',*,*,#45890,.F.);
#60588=ORIENTED_EDGE('',*,*,#45891,.T.);
#60589=ORIENTED_EDGE('',*,*,#45887,.T.);
#60590=ORIENTED_EDGE('',*,*,#45892,.F.);
#60591=ORIENTED_EDGE('',*,*,#45885,.F.);
#60592=ORIENTED_EDGE('',*,*,#45893,.T.);
#60593=ORIENTED_EDGE('',*,*,#45890,.T.);
#60594=ORIENTED_EDGE('',*,*,#45894,.F.);
#60595=ORIENTED_EDGE('',*,*,#45895,.F.);
#60596=ORIENTED_EDGE('',*,*,#45896,.T.);
#60597=ORIENTED_EDGE('',*,*,#45897,.T.);
#60598=ORIENTED_EDGE('',*,*,#45898,.F.);
#60599=ORIENTED_EDGE('',*,*,#45899,.F.);
#60600=ORIENTED_EDGE('',*,*,#45900,.T.);
#60601=ORIENTED_EDGE('',*,*,#45895,.T.);
#60602=ORIENTED_EDGE('',*,*,#45901,.F.);
#60603=ORIENTED_EDGE('',*,*,#45902,.F.);
#60604=ORIENTED_EDGE('',*,*,#45903,.T.);
#60605=ORIENTED_EDGE('',*,*,#45899,.T.);
#60606=ORIENTED_EDGE('',*,*,#45904,.F.);
#60607=ORIENTED_EDGE('',*,*,#45897,.F.);
#60608=ORIENTED_EDGE('',*,*,#45905,.T.);
#60609=ORIENTED_EDGE('',*,*,#45902,.T.);
#60610=ORIENTED_EDGE('',*,*,#45906,.F.);
#60611=ORIENTED_EDGE('',*,*,#45907,.F.);
#60612=ORIENTED_EDGE('',*,*,#45908,.T.);
#60613=ORIENTED_EDGE('',*,*,#45909,.T.);
#60614=ORIENTED_EDGE('',*,*,#45910,.F.);
#60615=ORIENTED_EDGE('',*,*,#45911,.F.);
#60616=ORIENTED_EDGE('',*,*,#45912,.T.);
#60617=ORIENTED_EDGE('',*,*,#45907,.T.);
#60618=ORIENTED_EDGE('',*,*,#45913,.F.);
#60619=ORIENTED_EDGE('',*,*,#45914,.F.);
#60620=ORIENTED_EDGE('',*,*,#45915,.T.);
#60621=ORIENTED_EDGE('',*,*,#45911,.T.);
#60622=ORIENTED_EDGE('',*,*,#45916,.F.);
#60623=ORIENTED_EDGE('',*,*,#45909,.F.);
#60624=ORIENTED_EDGE('',*,*,#45917,.T.);
#60625=ORIENTED_EDGE('',*,*,#45914,.T.);
#60626=ORIENTED_EDGE('',*,*,#45918,.F.);
#60627=ORIENTED_EDGE('',*,*,#45919,.F.);
#60628=ORIENTED_EDGE('',*,*,#45920,.T.);
#60629=ORIENTED_EDGE('',*,*,#45921,.T.);
#60630=ORIENTED_EDGE('',*,*,#45922,.F.);
#60631=ORIENTED_EDGE('',*,*,#45923,.F.);
#60632=ORIENTED_EDGE('',*,*,#45924,.T.);
#60633=ORIENTED_EDGE('',*,*,#45919,.T.);
#60634=ORIENTED_EDGE('',*,*,#45925,.F.);
#60635=ORIENTED_EDGE('',*,*,#45926,.F.);
#60636=ORIENTED_EDGE('',*,*,#45927,.T.);
#60637=ORIENTED_EDGE('',*,*,#45923,.T.);
#60638=ORIENTED_EDGE('',*,*,#45928,.F.);
#60639=ORIENTED_EDGE('',*,*,#45921,.F.);
#60640=ORIENTED_EDGE('',*,*,#45929,.T.);
#60641=ORIENTED_EDGE('',*,*,#45926,.T.);
#60642=ORIENTED_EDGE('',*,*,#45930,.F.);
#60643=ORIENTED_EDGE('',*,*,#45931,.F.);
#60644=ORIENTED_EDGE('',*,*,#45932,.T.);
#60645=ORIENTED_EDGE('',*,*,#45933,.T.);
#60646=ORIENTED_EDGE('',*,*,#45934,.F.);
#60647=ORIENTED_EDGE('',*,*,#45935,.F.);
#60648=ORIENTED_EDGE('',*,*,#45936,.T.);
#60649=ORIENTED_EDGE('',*,*,#45931,.T.);
#60650=ORIENTED_EDGE('',*,*,#45937,.F.);
#60651=ORIENTED_EDGE('',*,*,#45938,.F.);
#60652=ORIENTED_EDGE('',*,*,#45939,.T.);
#60653=ORIENTED_EDGE('',*,*,#45935,.T.);
#60654=ORIENTED_EDGE('',*,*,#45940,.F.);
#60655=ORIENTED_EDGE('',*,*,#45933,.F.);
#60656=ORIENTED_EDGE('',*,*,#45941,.T.);
#60657=ORIENTED_EDGE('',*,*,#45938,.T.);
#60658=ORIENTED_EDGE('',*,*,#45942,.F.);
#60659=ORIENTED_EDGE('',*,*,#45943,.F.);
#60660=ORIENTED_EDGE('',*,*,#45944,.T.);
#60661=ORIENTED_EDGE('',*,*,#45945,.T.);
#60662=ORIENTED_EDGE('',*,*,#45946,.F.);
#60663=ORIENTED_EDGE('',*,*,#45947,.F.);
#60664=ORIENTED_EDGE('',*,*,#45948,.T.);
#60665=ORIENTED_EDGE('',*,*,#45943,.T.);
#60666=ORIENTED_EDGE('',*,*,#45949,.F.);
#60667=ORIENTED_EDGE('',*,*,#45950,.F.);
#60668=ORIENTED_EDGE('',*,*,#45951,.T.);
#60669=ORIENTED_EDGE('',*,*,#45947,.T.);
#60670=ORIENTED_EDGE('',*,*,#45952,.F.);
#60671=ORIENTED_EDGE('',*,*,#45945,.F.);
#60672=ORIENTED_EDGE('',*,*,#45953,.T.);
#60673=ORIENTED_EDGE('',*,*,#45950,.T.);
#60674=ORIENTED_EDGE('',*,*,#45954,.F.);
#60675=ORIENTED_EDGE('',*,*,#45955,.F.);
#60676=ORIENTED_EDGE('',*,*,#45956,.T.);
#60677=ORIENTED_EDGE('',*,*,#45957,.T.);
#60678=ORIENTED_EDGE('',*,*,#45958,.F.);
#60679=ORIENTED_EDGE('',*,*,#45959,.F.);
#60680=ORIENTED_EDGE('',*,*,#45960,.T.);
#60681=ORIENTED_EDGE('',*,*,#45955,.T.);
#60682=ORIENTED_EDGE('',*,*,#45961,.F.);
#60683=ORIENTED_EDGE('',*,*,#45962,.F.);
#60684=ORIENTED_EDGE('',*,*,#45963,.T.);
#60685=ORIENTED_EDGE('',*,*,#45959,.T.);
#60686=ORIENTED_EDGE('',*,*,#45964,.F.);
#60687=ORIENTED_EDGE('',*,*,#45957,.F.);
#60688=ORIENTED_EDGE('',*,*,#45965,.T.);
#60689=ORIENTED_EDGE('',*,*,#45962,.T.);
#60690=ORIENTED_EDGE('',*,*,#45966,.F.);
#60691=ORIENTED_EDGE('',*,*,#45967,.F.);
#60692=ORIENTED_EDGE('',*,*,#45968,.T.);
#60693=ORIENTED_EDGE('',*,*,#45969,.T.);
#60694=ORIENTED_EDGE('',*,*,#45970,.F.);
#60695=ORIENTED_EDGE('',*,*,#45971,.F.);
#60696=ORIENTED_EDGE('',*,*,#45972,.T.);
#60697=ORIENTED_EDGE('',*,*,#45967,.T.);
#60698=ORIENTED_EDGE('',*,*,#45973,.F.);
#60699=ORIENTED_EDGE('',*,*,#45974,.F.);
#60700=ORIENTED_EDGE('',*,*,#45975,.T.);
#60701=ORIENTED_EDGE('',*,*,#45971,.T.);
#60702=ORIENTED_EDGE('',*,*,#45976,.F.);
#60703=ORIENTED_EDGE('',*,*,#45969,.F.);
#60704=ORIENTED_EDGE('',*,*,#45977,.T.);
#60705=ORIENTED_EDGE('',*,*,#45974,.T.);
#60706=ORIENTED_EDGE('',*,*,#45978,.F.);
#60707=ORIENTED_EDGE('',*,*,#45979,.F.);
#60708=ORIENTED_EDGE('',*,*,#45980,.T.);
#60709=ORIENTED_EDGE('',*,*,#45981,.T.);
#60710=ORIENTED_EDGE('',*,*,#45982,.F.);
#60711=ORIENTED_EDGE('',*,*,#45983,.F.);
#60712=ORIENTED_EDGE('',*,*,#45984,.T.);
#60713=ORIENTED_EDGE('',*,*,#45979,.T.);
#60714=ORIENTED_EDGE('',*,*,#45985,.F.);
#60715=ORIENTED_EDGE('',*,*,#45986,.F.);
#60716=ORIENTED_EDGE('',*,*,#45987,.T.);
#60717=ORIENTED_EDGE('',*,*,#45983,.T.);
#60718=ORIENTED_EDGE('',*,*,#45988,.F.);
#60719=ORIENTED_EDGE('',*,*,#45981,.F.);
#60720=ORIENTED_EDGE('',*,*,#45989,.T.);
#60721=ORIENTED_EDGE('',*,*,#45986,.T.);
#60722=ORIENTED_EDGE('',*,*,#45990,.F.);
#60723=ORIENTED_EDGE('',*,*,#45991,.F.);
#60724=ORIENTED_EDGE('',*,*,#45992,.T.);
#60725=ORIENTED_EDGE('',*,*,#45993,.T.);
#60726=ORIENTED_EDGE('',*,*,#45994,.F.);
#60727=ORIENTED_EDGE('',*,*,#45995,.F.);
#60728=ORIENTED_EDGE('',*,*,#45996,.T.);
#60729=ORIENTED_EDGE('',*,*,#45991,.T.);
#60730=ORIENTED_EDGE('',*,*,#45997,.F.);
#60731=ORIENTED_EDGE('',*,*,#45998,.F.);
#60732=ORIENTED_EDGE('',*,*,#45999,.T.);
#60733=ORIENTED_EDGE('',*,*,#45995,.T.);
#60734=ORIENTED_EDGE('',*,*,#46000,.F.);
#60735=ORIENTED_EDGE('',*,*,#45993,.F.);
#60736=ORIENTED_EDGE('',*,*,#46001,.T.);
#60737=ORIENTED_EDGE('',*,*,#45998,.T.);
#60738=ORIENTED_EDGE('',*,*,#46002,.F.);
#60739=ORIENTED_EDGE('',*,*,#46003,.F.);
#60740=ORIENTED_EDGE('',*,*,#46004,.T.);
#60741=ORIENTED_EDGE('',*,*,#46005,.T.);
#60742=ORIENTED_EDGE('',*,*,#46006,.F.);
#60743=ORIENTED_EDGE('',*,*,#46007,.F.);
#60744=ORIENTED_EDGE('',*,*,#46008,.T.);
#60745=ORIENTED_EDGE('',*,*,#46003,.T.);
#60746=ORIENTED_EDGE('',*,*,#46009,.F.);
#60747=ORIENTED_EDGE('',*,*,#46010,.F.);
#60748=ORIENTED_EDGE('',*,*,#46011,.T.);
#60749=ORIENTED_EDGE('',*,*,#46007,.T.);
#60750=ORIENTED_EDGE('',*,*,#46012,.F.);
#60751=ORIENTED_EDGE('',*,*,#46005,.F.);
#60752=ORIENTED_EDGE('',*,*,#46013,.T.);
#60753=ORIENTED_EDGE('',*,*,#46010,.T.);
#60754=ORIENTED_EDGE('',*,*,#46014,.F.);
#60755=ORIENTED_EDGE('',*,*,#46015,.F.);
#60756=ORIENTED_EDGE('',*,*,#46016,.T.);
#60757=ORIENTED_EDGE('',*,*,#46017,.T.);
#60758=ORIENTED_EDGE('',*,*,#46018,.F.);
#60759=ORIENTED_EDGE('',*,*,#46019,.F.);
#60760=ORIENTED_EDGE('',*,*,#46020,.T.);
#60761=ORIENTED_EDGE('',*,*,#46015,.T.);
#60762=ORIENTED_EDGE('',*,*,#46021,.F.);
#60763=ORIENTED_EDGE('',*,*,#46022,.F.);
#60764=ORIENTED_EDGE('',*,*,#46023,.T.);
#60765=ORIENTED_EDGE('',*,*,#46019,.T.);
#60766=ORIENTED_EDGE('',*,*,#46024,.F.);
#60767=ORIENTED_EDGE('',*,*,#46017,.F.);
#60768=ORIENTED_EDGE('',*,*,#46025,.T.);
#60769=ORIENTED_EDGE('',*,*,#46022,.T.);
#60770=ORIENTED_EDGE('',*,*,#46026,.F.);
#60771=ORIENTED_EDGE('',*,*,#46027,.F.);
#60772=ORIENTED_EDGE('',*,*,#46028,.T.);
#60773=ORIENTED_EDGE('',*,*,#46029,.T.);
#60774=ORIENTED_EDGE('',*,*,#46030,.F.);
#60775=ORIENTED_EDGE('',*,*,#46031,.F.);
#60776=ORIENTED_EDGE('',*,*,#46032,.T.);
#60777=ORIENTED_EDGE('',*,*,#46027,.T.);
#60778=ORIENTED_EDGE('',*,*,#46033,.F.);
#60779=ORIENTED_EDGE('',*,*,#46034,.F.);
#60780=ORIENTED_EDGE('',*,*,#46035,.T.);
#60781=ORIENTED_EDGE('',*,*,#46031,.T.);
#60782=ORIENTED_EDGE('',*,*,#46036,.F.);
#60783=ORIENTED_EDGE('',*,*,#46029,.F.);
#60784=ORIENTED_EDGE('',*,*,#46037,.T.);
#60785=ORIENTED_EDGE('',*,*,#46034,.T.);
#60786=ORIENTED_EDGE('',*,*,#46038,.F.);
#60787=ORIENTED_EDGE('',*,*,#46039,.F.);
#60788=ORIENTED_EDGE('',*,*,#46040,.T.);
#60789=ORIENTED_EDGE('',*,*,#46041,.T.);
#60790=ORIENTED_EDGE('',*,*,#46042,.F.);
#60791=ORIENTED_EDGE('',*,*,#46043,.F.);
#60792=ORIENTED_EDGE('',*,*,#46044,.T.);
#60793=ORIENTED_EDGE('',*,*,#46039,.T.);
#60794=ORIENTED_EDGE('',*,*,#46045,.F.);
#60795=ORIENTED_EDGE('',*,*,#46046,.F.);
#60796=ORIENTED_EDGE('',*,*,#46047,.T.);
#60797=ORIENTED_EDGE('',*,*,#46043,.T.);
#60798=ORIENTED_EDGE('',*,*,#46048,.F.);
#60799=ORIENTED_EDGE('',*,*,#46041,.F.);
#60800=ORIENTED_EDGE('',*,*,#46049,.T.);
#60801=ORIENTED_EDGE('',*,*,#46046,.T.);
#60802=ORIENTED_EDGE('',*,*,#46050,.F.);
#60803=ORIENTED_EDGE('',*,*,#46051,.F.);
#60804=ORIENTED_EDGE('',*,*,#46052,.T.);
#60805=ORIENTED_EDGE('',*,*,#46053,.T.);
#60806=ORIENTED_EDGE('',*,*,#46054,.F.);
#60807=ORIENTED_EDGE('',*,*,#46055,.F.);
#60808=ORIENTED_EDGE('',*,*,#46056,.T.);
#60809=ORIENTED_EDGE('',*,*,#46051,.T.);
#60810=ORIENTED_EDGE('',*,*,#46057,.F.);
#60811=ORIENTED_EDGE('',*,*,#46058,.F.);
#60812=ORIENTED_EDGE('',*,*,#46059,.T.);
#60813=ORIENTED_EDGE('',*,*,#46055,.T.);
#60814=ORIENTED_EDGE('',*,*,#46060,.F.);
#60815=ORIENTED_EDGE('',*,*,#46053,.F.);
#60816=ORIENTED_EDGE('',*,*,#46061,.T.);
#60817=ORIENTED_EDGE('',*,*,#46058,.T.);
#60818=ORIENTED_EDGE('',*,*,#46062,.F.);
#60819=ORIENTED_EDGE('',*,*,#46063,.F.);
#60820=ORIENTED_EDGE('',*,*,#46064,.T.);
#60821=ORIENTED_EDGE('',*,*,#46065,.T.);
#60822=ORIENTED_EDGE('',*,*,#46066,.F.);
#60823=ORIENTED_EDGE('',*,*,#46067,.F.);
#60824=ORIENTED_EDGE('',*,*,#46068,.T.);
#60825=ORIENTED_EDGE('',*,*,#46063,.T.);
#60826=ORIENTED_EDGE('',*,*,#46069,.F.);
#60827=ORIENTED_EDGE('',*,*,#46070,.F.);
#60828=ORIENTED_EDGE('',*,*,#46071,.T.);
#60829=ORIENTED_EDGE('',*,*,#46067,.T.);
#60830=ORIENTED_EDGE('',*,*,#46072,.F.);
#60831=ORIENTED_EDGE('',*,*,#46065,.F.);
#60832=ORIENTED_EDGE('',*,*,#46073,.T.);
#60833=ORIENTED_EDGE('',*,*,#46070,.T.);
#60834=ORIENTED_EDGE('',*,*,#46074,.F.);
#60835=ORIENTED_EDGE('',*,*,#46075,.F.);
#60836=ORIENTED_EDGE('',*,*,#46076,.T.);
#60837=ORIENTED_EDGE('',*,*,#46077,.T.);
#60838=ORIENTED_EDGE('',*,*,#46078,.F.);
#60839=ORIENTED_EDGE('',*,*,#46079,.F.);
#60840=ORIENTED_EDGE('',*,*,#46080,.T.);
#60841=ORIENTED_EDGE('',*,*,#46075,.T.);
#60842=ORIENTED_EDGE('',*,*,#46081,.F.);
#60843=ORIENTED_EDGE('',*,*,#46082,.F.);
#60844=ORIENTED_EDGE('',*,*,#46083,.T.);
#60845=ORIENTED_EDGE('',*,*,#46079,.T.);
#60846=ORIENTED_EDGE('',*,*,#46084,.F.);
#60847=ORIENTED_EDGE('',*,*,#46077,.F.);
#60848=ORIENTED_EDGE('',*,*,#46085,.T.);
#60849=ORIENTED_EDGE('',*,*,#46082,.T.);
#60850=ORIENTED_EDGE('',*,*,#46086,.F.);
#60851=ORIENTED_EDGE('',*,*,#46087,.F.);
#60852=ORIENTED_EDGE('',*,*,#46088,.T.);
#60853=ORIENTED_EDGE('',*,*,#46089,.T.);
#60854=ORIENTED_EDGE('',*,*,#46090,.F.);
#60855=ORIENTED_EDGE('',*,*,#46091,.F.);
#60856=ORIENTED_EDGE('',*,*,#46092,.T.);
#60857=ORIENTED_EDGE('',*,*,#46087,.T.);
#60858=ORIENTED_EDGE('',*,*,#46093,.F.);
#60859=ORIENTED_EDGE('',*,*,#46094,.F.);
#60860=ORIENTED_EDGE('',*,*,#46095,.T.);
#60861=ORIENTED_EDGE('',*,*,#46091,.T.);
#60862=ORIENTED_EDGE('',*,*,#46096,.F.);
#60863=ORIENTED_EDGE('',*,*,#46089,.F.);
#60864=ORIENTED_EDGE('',*,*,#46097,.T.);
#60865=ORIENTED_EDGE('',*,*,#46094,.T.);
#60866=ORIENTED_EDGE('',*,*,#46098,.F.);
#60867=ORIENTED_EDGE('',*,*,#46099,.F.);
#60868=ORIENTED_EDGE('',*,*,#46100,.T.);
#60869=ORIENTED_EDGE('',*,*,#46101,.T.);
#60870=ORIENTED_EDGE('',*,*,#46102,.F.);
#60871=ORIENTED_EDGE('',*,*,#46103,.F.);
#60872=ORIENTED_EDGE('',*,*,#46104,.T.);
#60873=ORIENTED_EDGE('',*,*,#46099,.T.);
#60874=ORIENTED_EDGE('',*,*,#46105,.F.);
#60875=ORIENTED_EDGE('',*,*,#46106,.F.);
#60876=ORIENTED_EDGE('',*,*,#46107,.T.);
#60877=ORIENTED_EDGE('',*,*,#46103,.T.);
#60878=ORIENTED_EDGE('',*,*,#46108,.F.);
#60879=ORIENTED_EDGE('',*,*,#46101,.F.);
#60880=ORIENTED_EDGE('',*,*,#46109,.T.);
#60881=ORIENTED_EDGE('',*,*,#46106,.T.);
#60882=ORIENTED_EDGE('',*,*,#46110,.F.);
#60883=ORIENTED_EDGE('',*,*,#46111,.F.);
#60884=ORIENTED_EDGE('',*,*,#46112,.T.);
#60885=ORIENTED_EDGE('',*,*,#46113,.T.);
#60886=ORIENTED_EDGE('',*,*,#46114,.F.);
#60887=ORIENTED_EDGE('',*,*,#46115,.F.);
#60888=ORIENTED_EDGE('',*,*,#46116,.T.);
#60889=ORIENTED_EDGE('',*,*,#46111,.T.);
#60890=ORIENTED_EDGE('',*,*,#46117,.F.);
#60891=ORIENTED_EDGE('',*,*,#46118,.F.);
#60892=ORIENTED_EDGE('',*,*,#46119,.T.);
#60893=ORIENTED_EDGE('',*,*,#46115,.T.);
#60894=ORIENTED_EDGE('',*,*,#46120,.F.);
#60895=ORIENTED_EDGE('',*,*,#46113,.F.);
#60896=ORIENTED_EDGE('',*,*,#46121,.T.);
#60897=ORIENTED_EDGE('',*,*,#46118,.T.);
#60898=ORIENTED_EDGE('',*,*,#46122,.F.);
#60899=ORIENTED_EDGE('',*,*,#46123,.F.);
#60900=ORIENTED_EDGE('',*,*,#46124,.T.);
#60901=ORIENTED_EDGE('',*,*,#46125,.T.);
#60902=ORIENTED_EDGE('',*,*,#46126,.F.);
#60903=ORIENTED_EDGE('',*,*,#46127,.F.);
#60904=ORIENTED_EDGE('',*,*,#46128,.T.);
#60905=ORIENTED_EDGE('',*,*,#46123,.T.);
#60906=ORIENTED_EDGE('',*,*,#46129,.F.);
#60907=ORIENTED_EDGE('',*,*,#46130,.F.);
#60908=ORIENTED_EDGE('',*,*,#46131,.T.);
#60909=ORIENTED_EDGE('',*,*,#46127,.T.);
#60910=ORIENTED_EDGE('',*,*,#46132,.F.);
#60911=ORIENTED_EDGE('',*,*,#46125,.F.);
#60912=ORIENTED_EDGE('',*,*,#46133,.T.);
#60913=ORIENTED_EDGE('',*,*,#46130,.T.);
#60914=ORIENTED_EDGE('',*,*,#46134,.F.);
#60915=ORIENTED_EDGE('',*,*,#46135,.F.);
#60916=ORIENTED_EDGE('',*,*,#46136,.T.);
#60917=ORIENTED_EDGE('',*,*,#46137,.T.);
#60918=ORIENTED_EDGE('',*,*,#46138,.F.);
#60919=ORIENTED_EDGE('',*,*,#46139,.F.);
#60920=ORIENTED_EDGE('',*,*,#46140,.T.);
#60921=ORIENTED_EDGE('',*,*,#46135,.T.);
#60922=ORIENTED_EDGE('',*,*,#46141,.F.);
#60923=ORIENTED_EDGE('',*,*,#46142,.F.);
#60924=ORIENTED_EDGE('',*,*,#46143,.T.);
#60925=ORIENTED_EDGE('',*,*,#46139,.T.);
#60926=ORIENTED_EDGE('',*,*,#46144,.F.);
#60927=ORIENTED_EDGE('',*,*,#46137,.F.);
#60928=ORIENTED_EDGE('',*,*,#46145,.T.);
#60929=ORIENTED_EDGE('',*,*,#46142,.T.);
#60930=ORIENTED_EDGE('',*,*,#46146,.F.);
#60931=ORIENTED_EDGE('',*,*,#46147,.F.);
#60932=ORIENTED_EDGE('',*,*,#46148,.T.);
#60933=ORIENTED_EDGE('',*,*,#46149,.T.);
#60934=ORIENTED_EDGE('',*,*,#46150,.F.);
#60935=ORIENTED_EDGE('',*,*,#46151,.F.);
#60936=ORIENTED_EDGE('',*,*,#46152,.T.);
#60937=ORIENTED_EDGE('',*,*,#46147,.T.);
#60938=ORIENTED_EDGE('',*,*,#46153,.F.);
#60939=ORIENTED_EDGE('',*,*,#46154,.F.);
#60940=ORIENTED_EDGE('',*,*,#46155,.T.);
#60941=ORIENTED_EDGE('',*,*,#46151,.T.);
#60942=ORIENTED_EDGE('',*,*,#46156,.F.);
#60943=ORIENTED_EDGE('',*,*,#46149,.F.);
#60944=ORIENTED_EDGE('',*,*,#46157,.T.);
#60945=ORIENTED_EDGE('',*,*,#46154,.T.);
#60946=ORIENTED_EDGE('',*,*,#46158,.F.);
#60947=ORIENTED_EDGE('',*,*,#46159,.F.);
#60948=ORIENTED_EDGE('',*,*,#46160,.T.);
#60949=ORIENTED_EDGE('',*,*,#46161,.T.);
#60950=ORIENTED_EDGE('',*,*,#46162,.F.);
#60951=ORIENTED_EDGE('',*,*,#46163,.F.);
#60952=ORIENTED_EDGE('',*,*,#46164,.T.);
#60953=ORIENTED_EDGE('',*,*,#46159,.T.);
#60954=ORIENTED_EDGE('',*,*,#46165,.F.);
#60955=ORIENTED_EDGE('',*,*,#46166,.F.);
#60956=ORIENTED_EDGE('',*,*,#46167,.T.);
#60957=ORIENTED_EDGE('',*,*,#46163,.T.);
#60958=ORIENTED_EDGE('',*,*,#46168,.F.);
#60959=ORIENTED_EDGE('',*,*,#46161,.F.);
#60960=ORIENTED_EDGE('',*,*,#46169,.T.);
#60961=ORIENTED_EDGE('',*,*,#46166,.T.);
#60962=ORIENTED_EDGE('',*,*,#46170,.F.);
#60963=ORIENTED_EDGE('',*,*,#46171,.F.);
#60964=ORIENTED_EDGE('',*,*,#46172,.T.);
#60965=ORIENTED_EDGE('',*,*,#46173,.T.);
#60966=ORIENTED_EDGE('',*,*,#46174,.F.);
#60967=ORIENTED_EDGE('',*,*,#46175,.F.);
#60968=ORIENTED_EDGE('',*,*,#46176,.T.);
#60969=ORIENTED_EDGE('',*,*,#46171,.T.);
#60970=ORIENTED_EDGE('',*,*,#46177,.F.);
#60971=ORIENTED_EDGE('',*,*,#46178,.F.);
#60972=ORIENTED_EDGE('',*,*,#46179,.T.);
#60973=ORIENTED_EDGE('',*,*,#46175,.T.);
#60974=ORIENTED_EDGE('',*,*,#46180,.F.);
#60975=ORIENTED_EDGE('',*,*,#46173,.F.);
#60976=ORIENTED_EDGE('',*,*,#46181,.T.);
#60977=ORIENTED_EDGE('',*,*,#46178,.T.);
#60978=ORIENTED_EDGE('',*,*,#46182,.F.);
#60979=ORIENTED_EDGE('',*,*,#46183,.F.);
#60980=ORIENTED_EDGE('',*,*,#46184,.T.);
#60981=ORIENTED_EDGE('',*,*,#46185,.T.);
#60982=ORIENTED_EDGE('',*,*,#46186,.F.);
#60983=ORIENTED_EDGE('',*,*,#46187,.F.);
#60984=ORIENTED_EDGE('',*,*,#46188,.T.);
#60985=ORIENTED_EDGE('',*,*,#46183,.T.);
#60986=ORIENTED_EDGE('',*,*,#46189,.F.);
#60987=ORIENTED_EDGE('',*,*,#46190,.F.);
#60988=ORIENTED_EDGE('',*,*,#46191,.T.);
#60989=ORIENTED_EDGE('',*,*,#46187,.T.);
#60990=ORIENTED_EDGE('',*,*,#46192,.F.);
#60991=ORIENTED_EDGE('',*,*,#46185,.F.);
#60992=ORIENTED_EDGE('',*,*,#46193,.T.);
#60993=ORIENTED_EDGE('',*,*,#46190,.T.);
#60994=ORIENTED_EDGE('',*,*,#46194,.F.);
#60995=ORIENTED_EDGE('',*,*,#46195,.F.);
#60996=ORIENTED_EDGE('',*,*,#46196,.T.);
#60997=ORIENTED_EDGE('',*,*,#46197,.T.);
#60998=ORIENTED_EDGE('',*,*,#46198,.F.);
#60999=ORIENTED_EDGE('',*,*,#46199,.F.);
#61000=ORIENTED_EDGE('',*,*,#46200,.T.);
#61001=ORIENTED_EDGE('',*,*,#46195,.T.);
#61002=ORIENTED_EDGE('',*,*,#46201,.F.);
#61003=ORIENTED_EDGE('',*,*,#46202,.F.);
#61004=ORIENTED_EDGE('',*,*,#46203,.T.);
#61005=ORIENTED_EDGE('',*,*,#46199,.T.);
#61006=ORIENTED_EDGE('',*,*,#46204,.F.);
#61007=ORIENTED_EDGE('',*,*,#46197,.F.);
#61008=ORIENTED_EDGE('',*,*,#46205,.T.);
#61009=ORIENTED_EDGE('',*,*,#46202,.T.);
#61010=ORIENTED_EDGE('',*,*,#46206,.F.);
#61011=ORIENTED_EDGE('',*,*,#46207,.F.);
#61012=ORIENTED_EDGE('',*,*,#46208,.T.);
#61013=ORIENTED_EDGE('',*,*,#46209,.T.);
#61014=ORIENTED_EDGE('',*,*,#46210,.F.);
#61015=ORIENTED_EDGE('',*,*,#46211,.F.);
#61016=ORIENTED_EDGE('',*,*,#46212,.T.);
#61017=ORIENTED_EDGE('',*,*,#46207,.T.);
#61018=ORIENTED_EDGE('',*,*,#46213,.F.);
#61019=ORIENTED_EDGE('',*,*,#46214,.F.);
#61020=ORIENTED_EDGE('',*,*,#46215,.T.);
#61021=ORIENTED_EDGE('',*,*,#46211,.T.);
#61022=ORIENTED_EDGE('',*,*,#46216,.F.);
#61023=ORIENTED_EDGE('',*,*,#46209,.F.);
#61024=ORIENTED_EDGE('',*,*,#46217,.T.);
#61025=ORIENTED_EDGE('',*,*,#46214,.T.);
#61026=ORIENTED_EDGE('',*,*,#46218,.F.);
#61027=ORIENTED_EDGE('',*,*,#46219,.F.);
#61028=ORIENTED_EDGE('',*,*,#46220,.T.);
#61029=ORIENTED_EDGE('',*,*,#46221,.T.);
#61030=ORIENTED_EDGE('',*,*,#46222,.F.);
#61031=ORIENTED_EDGE('',*,*,#46223,.F.);
#61032=ORIENTED_EDGE('',*,*,#46224,.T.);
#61033=ORIENTED_EDGE('',*,*,#46219,.T.);
#61034=ORIENTED_EDGE('',*,*,#46225,.F.);
#61035=ORIENTED_EDGE('',*,*,#46226,.F.);
#61036=ORIENTED_EDGE('',*,*,#46227,.T.);
#61037=ORIENTED_EDGE('',*,*,#46223,.T.);
#61038=ORIENTED_EDGE('',*,*,#46228,.F.);
#61039=ORIENTED_EDGE('',*,*,#46221,.F.);
#61040=ORIENTED_EDGE('',*,*,#46229,.T.);
#61041=ORIENTED_EDGE('',*,*,#46226,.T.);
#61042=ORIENTED_EDGE('',*,*,#46230,.F.);
#61043=ORIENTED_EDGE('',*,*,#46231,.F.);
#61044=ORIENTED_EDGE('',*,*,#46232,.T.);
#61045=ORIENTED_EDGE('',*,*,#46233,.T.);
#61046=ORIENTED_EDGE('',*,*,#46234,.F.);
#61047=ORIENTED_EDGE('',*,*,#46235,.F.);
#61048=ORIENTED_EDGE('',*,*,#46236,.T.);
#61049=ORIENTED_EDGE('',*,*,#46231,.T.);
#61050=ORIENTED_EDGE('',*,*,#46237,.F.);
#61051=ORIENTED_EDGE('',*,*,#46238,.F.);
#61052=ORIENTED_EDGE('',*,*,#46239,.T.);
#61053=ORIENTED_EDGE('',*,*,#46235,.T.);
#61054=ORIENTED_EDGE('',*,*,#46240,.F.);
#61055=ORIENTED_EDGE('',*,*,#46233,.F.);
#61056=ORIENTED_EDGE('',*,*,#46241,.T.);
#61057=ORIENTED_EDGE('',*,*,#46238,.T.);
#61058=ORIENTED_EDGE('',*,*,#46242,.F.);
#61059=ORIENTED_EDGE('',*,*,#46243,.F.);
#61060=ORIENTED_EDGE('',*,*,#46244,.T.);
#61061=ORIENTED_EDGE('',*,*,#46245,.T.);
#61062=ORIENTED_EDGE('',*,*,#46246,.F.);
#61063=ORIENTED_EDGE('',*,*,#46247,.F.);
#61064=ORIENTED_EDGE('',*,*,#46248,.T.);
#61065=ORIENTED_EDGE('',*,*,#46243,.T.);
#61066=ORIENTED_EDGE('',*,*,#46249,.F.);
#61067=ORIENTED_EDGE('',*,*,#46250,.F.);
#61068=ORIENTED_EDGE('',*,*,#46251,.T.);
#61069=ORIENTED_EDGE('',*,*,#46247,.T.);
#61070=ORIENTED_EDGE('',*,*,#46252,.F.);
#61071=ORIENTED_EDGE('',*,*,#46245,.F.);
#61072=ORIENTED_EDGE('',*,*,#46253,.T.);
#61073=ORIENTED_EDGE('',*,*,#46250,.T.);
#61074=ORIENTED_EDGE('',*,*,#46254,.F.);
#61075=ORIENTED_EDGE('',*,*,#46255,.F.);
#61076=ORIENTED_EDGE('',*,*,#46256,.T.);
#61077=ORIENTED_EDGE('',*,*,#46257,.T.);
#61078=ORIENTED_EDGE('',*,*,#46258,.F.);
#61079=ORIENTED_EDGE('',*,*,#46259,.F.);
#61080=ORIENTED_EDGE('',*,*,#46260,.T.);
#61081=ORIENTED_EDGE('',*,*,#46255,.T.);
#61082=ORIENTED_EDGE('',*,*,#46261,.F.);
#61083=ORIENTED_EDGE('',*,*,#46262,.F.);
#61084=ORIENTED_EDGE('',*,*,#46263,.T.);
#61085=ORIENTED_EDGE('',*,*,#46259,.T.);
#61086=ORIENTED_EDGE('',*,*,#46264,.F.);
#61087=ORIENTED_EDGE('',*,*,#46257,.F.);
#61088=ORIENTED_EDGE('',*,*,#46265,.T.);
#61089=ORIENTED_EDGE('',*,*,#46262,.T.);
#61090=ORIENTED_EDGE('',*,*,#46266,.F.);
#61091=ORIENTED_EDGE('',*,*,#46267,.F.);
#61092=ORIENTED_EDGE('',*,*,#46268,.T.);
#61093=ORIENTED_EDGE('',*,*,#46269,.T.);
#61094=ORIENTED_EDGE('',*,*,#46270,.F.);
#61095=ORIENTED_EDGE('',*,*,#46271,.F.);
#61096=ORIENTED_EDGE('',*,*,#46272,.T.);
#61097=ORIENTED_EDGE('',*,*,#46267,.T.);
#61098=ORIENTED_EDGE('',*,*,#46273,.F.);
#61099=ORIENTED_EDGE('',*,*,#46274,.F.);
#61100=ORIENTED_EDGE('',*,*,#46275,.T.);
#61101=ORIENTED_EDGE('',*,*,#46271,.T.);
#61102=ORIENTED_EDGE('',*,*,#46276,.F.);
#61103=ORIENTED_EDGE('',*,*,#46269,.F.);
#61104=ORIENTED_EDGE('',*,*,#46277,.T.);
#61105=ORIENTED_EDGE('',*,*,#46274,.T.);
#61106=ORIENTED_EDGE('',*,*,#46278,.F.);
#61107=ORIENTED_EDGE('',*,*,#46279,.F.);
#61108=ORIENTED_EDGE('',*,*,#46280,.T.);
#61109=ORIENTED_EDGE('',*,*,#46281,.T.);
#61110=ORIENTED_EDGE('',*,*,#46282,.F.);
#61111=ORIENTED_EDGE('',*,*,#46283,.F.);
#61112=ORIENTED_EDGE('',*,*,#46284,.T.);
#61113=ORIENTED_EDGE('',*,*,#46279,.T.);
#61114=ORIENTED_EDGE('',*,*,#46285,.F.);
#61115=ORIENTED_EDGE('',*,*,#46286,.F.);
#61116=ORIENTED_EDGE('',*,*,#46287,.T.);
#61117=ORIENTED_EDGE('',*,*,#46283,.T.);
#61118=ORIENTED_EDGE('',*,*,#46288,.F.);
#61119=ORIENTED_EDGE('',*,*,#46281,.F.);
#61120=ORIENTED_EDGE('',*,*,#46289,.T.);
#61121=ORIENTED_EDGE('',*,*,#46286,.T.);
#61122=ORIENTED_EDGE('',*,*,#46290,.F.);
#61123=ORIENTED_EDGE('',*,*,#46291,.F.);
#61124=ORIENTED_EDGE('',*,*,#46292,.T.);
#61125=ORIENTED_EDGE('',*,*,#46293,.T.);
#61126=ORIENTED_EDGE('',*,*,#46294,.F.);
#61127=ORIENTED_EDGE('',*,*,#46295,.F.);
#61128=ORIENTED_EDGE('',*,*,#46296,.T.);
#61129=ORIENTED_EDGE('',*,*,#46291,.T.);
#61130=ORIENTED_EDGE('',*,*,#46297,.F.);
#61131=ORIENTED_EDGE('',*,*,#46298,.F.);
#61132=ORIENTED_EDGE('',*,*,#46299,.T.);
#61133=ORIENTED_EDGE('',*,*,#46295,.T.);
#61134=ORIENTED_EDGE('',*,*,#46300,.F.);
#61135=ORIENTED_EDGE('',*,*,#46293,.F.);
#61136=ORIENTED_EDGE('',*,*,#46301,.T.);
#61137=ORIENTED_EDGE('',*,*,#46298,.T.);
#61138=ORIENTED_EDGE('',*,*,#46302,.F.);
#61139=ORIENTED_EDGE('',*,*,#46303,.F.);
#61140=ORIENTED_EDGE('',*,*,#46304,.T.);
#61141=ORIENTED_EDGE('',*,*,#46305,.T.);
#61142=ORIENTED_EDGE('',*,*,#46306,.F.);
#61143=ORIENTED_EDGE('',*,*,#46307,.F.);
#61144=ORIENTED_EDGE('',*,*,#46308,.T.);
#61145=ORIENTED_EDGE('',*,*,#46303,.T.);
#61146=ORIENTED_EDGE('',*,*,#46309,.F.);
#61147=ORIENTED_EDGE('',*,*,#46310,.F.);
#61148=ORIENTED_EDGE('',*,*,#46311,.T.);
#61149=ORIENTED_EDGE('',*,*,#46307,.T.);
#61150=ORIENTED_EDGE('',*,*,#46312,.F.);
#61151=ORIENTED_EDGE('',*,*,#46305,.F.);
#61152=ORIENTED_EDGE('',*,*,#46313,.T.);
#61153=ORIENTED_EDGE('',*,*,#46310,.T.);
#61154=ORIENTED_EDGE('',*,*,#46314,.F.);
#61155=ORIENTED_EDGE('',*,*,#46315,.F.);
#61156=ORIENTED_EDGE('',*,*,#46316,.T.);
#61157=ORIENTED_EDGE('',*,*,#46317,.T.);
#61158=ORIENTED_EDGE('',*,*,#46318,.F.);
#61159=ORIENTED_EDGE('',*,*,#46319,.F.);
#61160=ORIENTED_EDGE('',*,*,#46320,.T.);
#61161=ORIENTED_EDGE('',*,*,#46315,.T.);
#61162=ORIENTED_EDGE('',*,*,#46321,.F.);
#61163=ORIENTED_EDGE('',*,*,#46322,.F.);
#61164=ORIENTED_EDGE('',*,*,#46323,.T.);
#61165=ORIENTED_EDGE('',*,*,#46319,.T.);
#61166=ORIENTED_EDGE('',*,*,#46324,.F.);
#61167=ORIENTED_EDGE('',*,*,#46317,.F.);
#61168=ORIENTED_EDGE('',*,*,#46325,.T.);
#61169=ORIENTED_EDGE('',*,*,#46322,.T.);
#61170=ORIENTED_EDGE('',*,*,#46326,.F.);
#61171=ORIENTED_EDGE('',*,*,#46327,.F.);
#61172=ORIENTED_EDGE('',*,*,#46328,.T.);
#61173=ORIENTED_EDGE('',*,*,#46329,.T.);
#61174=ORIENTED_EDGE('',*,*,#46330,.F.);
#61175=ORIENTED_EDGE('',*,*,#46331,.F.);
#61176=ORIENTED_EDGE('',*,*,#46332,.T.);
#61177=ORIENTED_EDGE('',*,*,#46327,.T.);
#61178=ORIENTED_EDGE('',*,*,#46333,.F.);
#61179=ORIENTED_EDGE('',*,*,#46334,.F.);
#61180=ORIENTED_EDGE('',*,*,#46335,.T.);
#61181=ORIENTED_EDGE('',*,*,#46331,.T.);
#61182=ORIENTED_EDGE('',*,*,#46336,.F.);
#61183=ORIENTED_EDGE('',*,*,#46329,.F.);
#61184=ORIENTED_EDGE('',*,*,#46337,.T.);
#61185=ORIENTED_EDGE('',*,*,#46334,.T.);
#61186=ORIENTED_EDGE('',*,*,#46338,.F.);
#61187=ORIENTED_EDGE('',*,*,#46339,.F.);
#61188=ORIENTED_EDGE('',*,*,#46340,.T.);
#61189=ORIENTED_EDGE('',*,*,#46341,.T.);
#61190=ORIENTED_EDGE('',*,*,#46342,.F.);
#61191=ORIENTED_EDGE('',*,*,#46343,.F.);
#61192=ORIENTED_EDGE('',*,*,#46344,.T.);
#61193=ORIENTED_EDGE('',*,*,#46339,.T.);
#61194=ORIENTED_EDGE('',*,*,#46345,.F.);
#61195=ORIENTED_EDGE('',*,*,#46346,.F.);
#61196=ORIENTED_EDGE('',*,*,#46347,.T.);
#61197=ORIENTED_EDGE('',*,*,#46343,.T.);
#61198=ORIENTED_EDGE('',*,*,#46348,.F.);
#61199=ORIENTED_EDGE('',*,*,#46341,.F.);
#61200=ORIENTED_EDGE('',*,*,#46349,.T.);
#61201=ORIENTED_EDGE('',*,*,#46346,.T.);
#61202=ORIENTED_EDGE('',*,*,#46350,.F.);
#61203=ORIENTED_EDGE('',*,*,#46351,.F.);
#61204=ORIENTED_EDGE('',*,*,#46352,.T.);
#61205=ORIENTED_EDGE('',*,*,#46353,.T.);
#61206=ORIENTED_EDGE('',*,*,#46354,.F.);
#61207=ORIENTED_EDGE('',*,*,#46355,.F.);
#61208=ORIENTED_EDGE('',*,*,#46356,.T.);
#61209=ORIENTED_EDGE('',*,*,#46351,.T.);
#61210=ORIENTED_EDGE('',*,*,#46357,.F.);
#61211=ORIENTED_EDGE('',*,*,#46358,.F.);
#61212=ORIENTED_EDGE('',*,*,#46359,.T.);
#61213=ORIENTED_EDGE('',*,*,#46355,.T.);
#61214=ORIENTED_EDGE('',*,*,#46360,.F.);
#61215=ORIENTED_EDGE('',*,*,#46353,.F.);
#61216=ORIENTED_EDGE('',*,*,#46361,.T.);
#61217=ORIENTED_EDGE('',*,*,#46358,.T.);
#61218=ORIENTED_EDGE('',*,*,#46362,.F.);
#61219=ORIENTED_EDGE('',*,*,#46363,.F.);
#61220=ORIENTED_EDGE('',*,*,#46364,.T.);
#61221=ORIENTED_EDGE('',*,*,#46365,.T.);
#61222=ORIENTED_EDGE('',*,*,#46366,.F.);
#61223=ORIENTED_EDGE('',*,*,#46367,.F.);
#61224=ORIENTED_EDGE('',*,*,#46368,.T.);
#61225=ORIENTED_EDGE('',*,*,#46363,.T.);
#61226=ORIENTED_EDGE('',*,*,#46369,.F.);
#61227=ORIENTED_EDGE('',*,*,#46370,.F.);
#61228=ORIENTED_EDGE('',*,*,#46371,.T.);
#61229=ORIENTED_EDGE('',*,*,#46367,.T.);
#61230=ORIENTED_EDGE('',*,*,#46372,.F.);
#61231=ORIENTED_EDGE('',*,*,#46365,.F.);
#61232=ORIENTED_EDGE('',*,*,#46373,.T.);
#61233=ORIENTED_EDGE('',*,*,#46370,.T.);
#61234=ORIENTED_EDGE('',*,*,#46374,.F.);
#61235=ORIENTED_EDGE('',*,*,#46375,.F.);
#61236=ORIENTED_EDGE('',*,*,#46376,.T.);
#61237=ORIENTED_EDGE('',*,*,#46377,.T.);
#61238=ORIENTED_EDGE('',*,*,#46378,.F.);
#61239=ORIENTED_EDGE('',*,*,#46379,.F.);
#61240=ORIENTED_EDGE('',*,*,#46380,.T.);
#61241=ORIENTED_EDGE('',*,*,#46375,.T.);
#61242=ORIENTED_EDGE('',*,*,#46381,.F.);
#61243=ORIENTED_EDGE('',*,*,#46382,.F.);
#61244=ORIENTED_EDGE('',*,*,#46383,.T.);
#61245=ORIENTED_EDGE('',*,*,#46379,.T.);
#61246=ORIENTED_EDGE('',*,*,#46384,.F.);
#61247=ORIENTED_EDGE('',*,*,#46377,.F.);
#61248=ORIENTED_EDGE('',*,*,#46385,.T.);
#61249=ORIENTED_EDGE('',*,*,#46382,.T.);
#61250=ORIENTED_EDGE('',*,*,#46386,.F.);
#61251=ORIENTED_EDGE('',*,*,#46387,.F.);
#61252=ORIENTED_EDGE('',*,*,#46388,.T.);
#61253=ORIENTED_EDGE('',*,*,#46389,.T.);
#61254=ORIENTED_EDGE('',*,*,#46390,.F.);
#61255=ORIENTED_EDGE('',*,*,#46391,.F.);
#61256=ORIENTED_EDGE('',*,*,#46392,.T.);
#61257=ORIENTED_EDGE('',*,*,#46387,.T.);
#61258=ORIENTED_EDGE('',*,*,#46393,.F.);
#61259=ORIENTED_EDGE('',*,*,#46394,.F.);
#61260=ORIENTED_EDGE('',*,*,#46395,.T.);
#61261=ORIENTED_EDGE('',*,*,#46391,.T.);
#61262=ORIENTED_EDGE('',*,*,#46396,.F.);
#61263=ORIENTED_EDGE('',*,*,#46389,.F.);
#61264=ORIENTED_EDGE('',*,*,#46397,.T.);
#61265=ORIENTED_EDGE('',*,*,#46394,.T.);
#61266=ORIENTED_EDGE('',*,*,#46398,.F.);
#61267=ORIENTED_EDGE('',*,*,#46399,.F.);
#61268=ORIENTED_EDGE('',*,*,#46400,.T.);
#61269=ORIENTED_EDGE('',*,*,#46401,.T.);
#61270=ORIENTED_EDGE('',*,*,#46402,.F.);
#61271=ORIENTED_EDGE('',*,*,#46403,.F.);
#61272=ORIENTED_EDGE('',*,*,#46404,.T.);
#61273=ORIENTED_EDGE('',*,*,#46399,.T.);
#61274=ORIENTED_EDGE('',*,*,#46405,.F.);
#61275=ORIENTED_EDGE('',*,*,#46406,.F.);
#61276=ORIENTED_EDGE('',*,*,#46407,.T.);
#61277=ORIENTED_EDGE('',*,*,#46403,.T.);
#61278=ORIENTED_EDGE('',*,*,#46408,.F.);
#61279=ORIENTED_EDGE('',*,*,#46401,.F.);
#61280=ORIENTED_EDGE('',*,*,#46409,.T.);
#61281=ORIENTED_EDGE('',*,*,#46406,.T.);
#61282=ORIENTED_EDGE('',*,*,#46410,.F.);
#61283=ORIENTED_EDGE('',*,*,#46411,.F.);
#61284=ORIENTED_EDGE('',*,*,#46412,.T.);
#61285=ORIENTED_EDGE('',*,*,#46413,.T.);
#61286=ORIENTED_EDGE('',*,*,#46414,.F.);
#61287=ORIENTED_EDGE('',*,*,#46415,.F.);
#61288=ORIENTED_EDGE('',*,*,#46416,.T.);
#61289=ORIENTED_EDGE('',*,*,#46411,.T.);
#61290=ORIENTED_EDGE('',*,*,#46417,.F.);
#61291=ORIENTED_EDGE('',*,*,#46418,.F.);
#61292=ORIENTED_EDGE('',*,*,#46419,.T.);
#61293=ORIENTED_EDGE('',*,*,#46415,.T.);
#61294=ORIENTED_EDGE('',*,*,#46420,.F.);
#61295=ORIENTED_EDGE('',*,*,#46413,.F.);
#61296=ORIENTED_EDGE('',*,*,#46421,.T.);
#61297=ORIENTED_EDGE('',*,*,#46418,.T.);
#61298=ORIENTED_EDGE('',*,*,#46422,.F.);
#61299=ORIENTED_EDGE('',*,*,#46423,.F.);
#61300=ORIENTED_EDGE('',*,*,#46424,.T.);
#61301=ORIENTED_EDGE('',*,*,#46425,.T.);
#61302=ORIENTED_EDGE('',*,*,#46426,.F.);
#61303=ORIENTED_EDGE('',*,*,#46427,.F.);
#61304=ORIENTED_EDGE('',*,*,#46428,.T.);
#61305=ORIENTED_EDGE('',*,*,#46423,.T.);
#61306=ORIENTED_EDGE('',*,*,#46429,.F.);
#61307=ORIENTED_EDGE('',*,*,#46430,.F.);
#61308=ORIENTED_EDGE('',*,*,#46431,.T.);
#61309=ORIENTED_EDGE('',*,*,#46427,.T.);
#61310=ORIENTED_EDGE('',*,*,#46432,.F.);
#61311=ORIENTED_EDGE('',*,*,#46425,.F.);
#61312=ORIENTED_EDGE('',*,*,#46433,.T.);
#61313=ORIENTED_EDGE('',*,*,#46430,.T.);
#61314=ORIENTED_EDGE('',*,*,#46434,.F.);
#61315=ORIENTED_EDGE('',*,*,#46435,.F.);
#61316=ORIENTED_EDGE('',*,*,#46436,.T.);
#61317=ORIENTED_EDGE('',*,*,#46437,.T.);
#61318=ORIENTED_EDGE('',*,*,#46438,.F.);
#61319=ORIENTED_EDGE('',*,*,#46439,.F.);
#61320=ORIENTED_EDGE('',*,*,#46440,.T.);
#61321=ORIENTED_EDGE('',*,*,#46435,.T.);
#61322=ORIENTED_EDGE('',*,*,#46441,.F.);
#61323=ORIENTED_EDGE('',*,*,#46442,.F.);
#61324=ORIENTED_EDGE('',*,*,#46443,.T.);
#61325=ORIENTED_EDGE('',*,*,#46439,.T.);
#61326=ORIENTED_EDGE('',*,*,#46444,.F.);
#61327=ORIENTED_EDGE('',*,*,#46437,.F.);
#61328=ORIENTED_EDGE('',*,*,#46445,.T.);
#61329=ORIENTED_EDGE('',*,*,#46442,.T.);
#61330=ORIENTED_EDGE('',*,*,#46446,.F.);
#61331=ORIENTED_EDGE('',*,*,#46447,.F.);
#61332=ORIENTED_EDGE('',*,*,#46448,.T.);
#61333=ORIENTED_EDGE('',*,*,#46449,.T.);
#61334=ORIENTED_EDGE('',*,*,#46450,.F.);
#61335=ORIENTED_EDGE('',*,*,#46451,.F.);
#61336=ORIENTED_EDGE('',*,*,#46452,.T.);
#61337=ORIENTED_EDGE('',*,*,#46447,.T.);
#61338=ORIENTED_EDGE('',*,*,#46453,.F.);
#61339=ORIENTED_EDGE('',*,*,#46454,.F.);
#61340=ORIENTED_EDGE('',*,*,#46455,.T.);
#61341=ORIENTED_EDGE('',*,*,#46451,.T.);
#61342=ORIENTED_EDGE('',*,*,#46456,.F.);
#61343=ORIENTED_EDGE('',*,*,#46449,.F.);
#61344=ORIENTED_EDGE('',*,*,#46457,.T.);
#61345=ORIENTED_EDGE('',*,*,#46454,.T.);
#61346=ORIENTED_EDGE('',*,*,#46458,.F.);
#61347=ORIENTED_EDGE('',*,*,#46459,.F.);
#61348=ORIENTED_EDGE('',*,*,#46460,.T.);
#61349=ORIENTED_EDGE('',*,*,#46461,.T.);
#61350=ORIENTED_EDGE('',*,*,#46462,.F.);
#61351=ORIENTED_EDGE('',*,*,#46463,.F.);
#61352=ORIENTED_EDGE('',*,*,#46464,.T.);
#61353=ORIENTED_EDGE('',*,*,#46459,.T.);
#61354=ORIENTED_EDGE('',*,*,#46465,.F.);
#61355=ORIENTED_EDGE('',*,*,#46466,.F.);
#61356=ORIENTED_EDGE('',*,*,#46467,.T.);
#61357=ORIENTED_EDGE('',*,*,#46463,.T.);
#61358=ORIENTED_EDGE('',*,*,#46468,.F.);
#61359=ORIENTED_EDGE('',*,*,#46461,.F.);
#61360=ORIENTED_EDGE('',*,*,#46469,.T.);
#61361=ORIENTED_EDGE('',*,*,#46466,.T.);
#61362=ORIENTED_EDGE('',*,*,#46470,.F.);
#61363=ORIENTED_EDGE('',*,*,#46471,.F.);
#61364=ORIENTED_EDGE('',*,*,#46472,.T.);
#61365=ORIENTED_EDGE('',*,*,#46473,.T.);
#61366=ORIENTED_EDGE('',*,*,#46474,.F.);
#61367=ORIENTED_EDGE('',*,*,#46475,.F.);
#61368=ORIENTED_EDGE('',*,*,#46476,.T.);
#61369=ORIENTED_EDGE('',*,*,#46471,.T.);
#61370=ORIENTED_EDGE('',*,*,#46477,.F.);
#61371=ORIENTED_EDGE('',*,*,#46478,.F.);
#61372=ORIENTED_EDGE('',*,*,#46479,.T.);
#61373=ORIENTED_EDGE('',*,*,#46475,.T.);
#61374=ORIENTED_EDGE('',*,*,#46480,.F.);
#61375=ORIENTED_EDGE('',*,*,#46473,.F.);
#61376=ORIENTED_EDGE('',*,*,#46481,.T.);
#61377=ORIENTED_EDGE('',*,*,#46478,.T.);
#61378=ORIENTED_EDGE('',*,*,#46482,.F.);
#61379=ORIENTED_EDGE('',*,*,#46483,.F.);
#61380=ORIENTED_EDGE('',*,*,#46484,.T.);
#61381=ORIENTED_EDGE('',*,*,#46485,.T.);
#61382=ORIENTED_EDGE('',*,*,#46486,.F.);
#61383=ORIENTED_EDGE('',*,*,#46487,.F.);
#61384=ORIENTED_EDGE('',*,*,#46488,.T.);
#61385=ORIENTED_EDGE('',*,*,#46483,.T.);
#61386=ORIENTED_EDGE('',*,*,#46489,.F.);
#61387=ORIENTED_EDGE('',*,*,#46490,.F.);
#61388=ORIENTED_EDGE('',*,*,#46491,.T.);
#61389=ORIENTED_EDGE('',*,*,#46487,.T.);
#61390=ORIENTED_EDGE('',*,*,#46492,.F.);
#61391=ORIENTED_EDGE('',*,*,#46485,.F.);
#61392=ORIENTED_EDGE('',*,*,#46493,.T.);
#61393=ORIENTED_EDGE('',*,*,#46490,.T.);
#61394=ORIENTED_EDGE('',*,*,#46494,.F.);
#61395=ORIENTED_EDGE('',*,*,#46495,.F.);
#61396=ORIENTED_EDGE('',*,*,#46496,.T.);
#61397=ORIENTED_EDGE('',*,*,#46497,.T.);
#61398=ORIENTED_EDGE('',*,*,#46498,.F.);
#61399=ORIENTED_EDGE('',*,*,#46499,.F.);
#61400=ORIENTED_EDGE('',*,*,#46500,.T.);
#61401=ORIENTED_EDGE('',*,*,#46495,.T.);
#61402=ORIENTED_EDGE('',*,*,#46501,.F.);
#61403=ORIENTED_EDGE('',*,*,#46502,.F.);
#61404=ORIENTED_EDGE('',*,*,#46503,.T.);
#61405=ORIENTED_EDGE('',*,*,#46499,.T.);
#61406=ORIENTED_EDGE('',*,*,#46504,.F.);
#61407=ORIENTED_EDGE('',*,*,#46497,.F.);
#61408=ORIENTED_EDGE('',*,*,#46505,.T.);
#61409=ORIENTED_EDGE('',*,*,#46502,.T.);
#61410=ORIENTED_EDGE('',*,*,#46506,.F.);
#61411=ORIENTED_EDGE('',*,*,#46507,.F.);
#61412=ORIENTED_EDGE('',*,*,#46508,.T.);
#61413=ORIENTED_EDGE('',*,*,#46509,.T.);
#61414=ORIENTED_EDGE('',*,*,#46510,.F.);
#61415=ORIENTED_EDGE('',*,*,#46511,.F.);
#61416=ORIENTED_EDGE('',*,*,#46512,.T.);
#61417=ORIENTED_EDGE('',*,*,#46507,.T.);
#61418=ORIENTED_EDGE('',*,*,#46513,.F.);
#61419=ORIENTED_EDGE('',*,*,#46514,.F.);
#61420=ORIENTED_EDGE('',*,*,#46515,.T.);
#61421=ORIENTED_EDGE('',*,*,#46511,.T.);
#61422=ORIENTED_EDGE('',*,*,#46516,.F.);
#61423=ORIENTED_EDGE('',*,*,#46509,.F.);
#61424=ORIENTED_EDGE('',*,*,#46517,.T.);
#61425=ORIENTED_EDGE('',*,*,#46514,.T.);
#61426=ORIENTED_EDGE('',*,*,#46518,.F.);
#61427=ORIENTED_EDGE('',*,*,#46519,.F.);
#61428=ORIENTED_EDGE('',*,*,#46520,.T.);
#61429=ORIENTED_EDGE('',*,*,#46521,.T.);
#61430=ORIENTED_EDGE('',*,*,#46522,.F.);
#61431=ORIENTED_EDGE('',*,*,#46523,.F.);
#61432=ORIENTED_EDGE('',*,*,#46524,.T.);
#61433=ORIENTED_EDGE('',*,*,#46519,.T.);
#61434=ORIENTED_EDGE('',*,*,#46525,.F.);
#61435=ORIENTED_EDGE('',*,*,#46526,.F.);
#61436=ORIENTED_EDGE('',*,*,#46527,.T.);
#61437=ORIENTED_EDGE('',*,*,#46523,.T.);
#61438=ORIENTED_EDGE('',*,*,#46528,.F.);
#61439=ORIENTED_EDGE('',*,*,#46521,.F.);
#61440=ORIENTED_EDGE('',*,*,#46529,.T.);
#61441=ORIENTED_EDGE('',*,*,#46526,.T.);
#61442=ORIENTED_EDGE('',*,*,#46530,.F.);
#61443=ORIENTED_EDGE('',*,*,#46531,.F.);
#61444=ORIENTED_EDGE('',*,*,#46532,.T.);
#61445=ORIENTED_EDGE('',*,*,#46533,.T.);
#61446=ORIENTED_EDGE('',*,*,#46534,.F.);
#61447=ORIENTED_EDGE('',*,*,#46535,.F.);
#61448=ORIENTED_EDGE('',*,*,#46536,.T.);
#61449=ORIENTED_EDGE('',*,*,#46531,.T.);
#61450=ORIENTED_EDGE('',*,*,#46537,.F.);
#61451=ORIENTED_EDGE('',*,*,#46538,.F.);
#61452=ORIENTED_EDGE('',*,*,#46539,.T.);
#61453=ORIENTED_EDGE('',*,*,#46535,.T.);
#61454=ORIENTED_EDGE('',*,*,#46540,.F.);
#61455=ORIENTED_EDGE('',*,*,#46533,.F.);
#61456=ORIENTED_EDGE('',*,*,#46541,.T.);
#61457=ORIENTED_EDGE('',*,*,#46538,.T.);
#61458=ORIENTED_EDGE('',*,*,#46542,.F.);
#61459=ORIENTED_EDGE('',*,*,#46543,.F.);
#61460=ORIENTED_EDGE('',*,*,#46544,.T.);
#61461=ORIENTED_EDGE('',*,*,#46545,.T.);
#61462=ORIENTED_EDGE('',*,*,#46546,.F.);
#61463=ORIENTED_EDGE('',*,*,#46547,.F.);
#61464=ORIENTED_EDGE('',*,*,#46548,.T.);
#61465=ORIENTED_EDGE('',*,*,#46543,.T.);
#61466=ORIENTED_EDGE('',*,*,#46549,.F.);
#61467=ORIENTED_EDGE('',*,*,#46550,.F.);
#61468=ORIENTED_EDGE('',*,*,#46551,.T.);
#61469=ORIENTED_EDGE('',*,*,#46547,.T.);
#61470=ORIENTED_EDGE('',*,*,#46552,.F.);
#61471=ORIENTED_EDGE('',*,*,#46545,.F.);
#61472=ORIENTED_EDGE('',*,*,#46553,.T.);
#61473=ORIENTED_EDGE('',*,*,#46550,.T.);
#61474=ORIENTED_EDGE('',*,*,#46554,.F.);
#61475=ORIENTED_EDGE('',*,*,#46555,.F.);
#61476=ORIENTED_EDGE('',*,*,#46556,.T.);
#61477=ORIENTED_EDGE('',*,*,#46557,.T.);
#61478=ORIENTED_EDGE('',*,*,#46558,.F.);
#61479=ORIENTED_EDGE('',*,*,#46559,.F.);
#61480=ORIENTED_EDGE('',*,*,#46560,.T.);
#61481=ORIENTED_EDGE('',*,*,#46555,.T.);
#61482=ORIENTED_EDGE('',*,*,#46561,.F.);
#61483=ORIENTED_EDGE('',*,*,#46562,.F.);
#61484=ORIENTED_EDGE('',*,*,#46563,.T.);
#61485=ORIENTED_EDGE('',*,*,#46559,.T.);
#61486=ORIENTED_EDGE('',*,*,#46564,.F.);
#61487=ORIENTED_EDGE('',*,*,#46557,.F.);
#61488=ORIENTED_EDGE('',*,*,#46565,.T.);
#61489=ORIENTED_EDGE('',*,*,#46562,.T.);
#61490=ORIENTED_EDGE('',*,*,#46566,.F.);
#61491=ORIENTED_EDGE('',*,*,#46567,.F.);
#61492=ORIENTED_EDGE('',*,*,#46568,.T.);
#61493=ORIENTED_EDGE('',*,*,#46569,.T.);
#61494=ORIENTED_EDGE('',*,*,#46570,.F.);
#61495=ORIENTED_EDGE('',*,*,#46571,.F.);
#61496=ORIENTED_EDGE('',*,*,#46572,.T.);
#61497=ORIENTED_EDGE('',*,*,#46567,.T.);
#61498=ORIENTED_EDGE('',*,*,#46573,.F.);
#61499=ORIENTED_EDGE('',*,*,#46574,.F.);
#61500=ORIENTED_EDGE('',*,*,#46575,.T.);
#61501=ORIENTED_EDGE('',*,*,#46571,.T.);
#61502=ORIENTED_EDGE('',*,*,#46576,.F.);
#61503=ORIENTED_EDGE('',*,*,#46569,.F.);
#61504=ORIENTED_EDGE('',*,*,#46577,.T.);
#61505=ORIENTED_EDGE('',*,*,#46574,.T.);
#61506=ORIENTED_EDGE('',*,*,#46578,.F.);
#61507=ORIENTED_EDGE('',*,*,#46579,.F.);
#61508=ORIENTED_EDGE('',*,*,#46580,.T.);
#61509=ORIENTED_EDGE('',*,*,#46581,.T.);
#61510=ORIENTED_EDGE('',*,*,#46582,.F.);
#61511=ORIENTED_EDGE('',*,*,#46583,.F.);
#61512=ORIENTED_EDGE('',*,*,#46584,.T.);
#61513=ORIENTED_EDGE('',*,*,#46579,.T.);
#61514=ORIENTED_EDGE('',*,*,#46585,.F.);
#61515=ORIENTED_EDGE('',*,*,#46586,.F.);
#61516=ORIENTED_EDGE('',*,*,#46587,.T.);
#61517=ORIENTED_EDGE('',*,*,#46583,.T.);
#61518=ORIENTED_EDGE('',*,*,#46588,.F.);
#61519=ORIENTED_EDGE('',*,*,#46581,.F.);
#61520=ORIENTED_EDGE('',*,*,#46589,.T.);
#61521=ORIENTED_EDGE('',*,*,#46586,.T.);
#61522=ORIENTED_EDGE('',*,*,#46590,.F.);
#61523=ORIENTED_EDGE('',*,*,#46591,.F.);
#61524=ORIENTED_EDGE('',*,*,#46592,.T.);
#61525=ORIENTED_EDGE('',*,*,#46593,.T.);
#61526=ORIENTED_EDGE('',*,*,#46594,.F.);
#61527=ORIENTED_EDGE('',*,*,#46595,.F.);
#61528=ORIENTED_EDGE('',*,*,#46596,.T.);
#61529=ORIENTED_EDGE('',*,*,#46591,.T.);
#61530=ORIENTED_EDGE('',*,*,#46597,.F.);
#61531=ORIENTED_EDGE('',*,*,#46598,.F.);
#61532=ORIENTED_EDGE('',*,*,#46599,.T.);
#61533=ORIENTED_EDGE('',*,*,#46595,.T.);
#61534=ORIENTED_EDGE('',*,*,#46600,.F.);
#61535=ORIENTED_EDGE('',*,*,#46593,.F.);
#61536=ORIENTED_EDGE('',*,*,#46601,.T.);
#61537=ORIENTED_EDGE('',*,*,#46598,.T.);
#61538=ORIENTED_EDGE('',*,*,#46602,.F.);
#61539=ORIENTED_EDGE('',*,*,#46603,.F.);
#61540=ORIENTED_EDGE('',*,*,#46604,.T.);
#61541=ORIENTED_EDGE('',*,*,#46605,.T.);
#61542=ORIENTED_EDGE('',*,*,#46606,.F.);
#61543=ORIENTED_EDGE('',*,*,#46607,.F.);
#61544=ORIENTED_EDGE('',*,*,#46608,.T.);
#61545=ORIENTED_EDGE('',*,*,#46603,.T.);
#61546=ORIENTED_EDGE('',*,*,#46609,.F.);
#61547=ORIENTED_EDGE('',*,*,#46610,.F.);
#61548=ORIENTED_EDGE('',*,*,#46611,.T.);
#61549=ORIENTED_EDGE('',*,*,#46607,.T.);
#61550=ORIENTED_EDGE('',*,*,#46612,.F.);
#61551=ORIENTED_EDGE('',*,*,#46605,.F.);
#61552=ORIENTED_EDGE('',*,*,#46613,.T.);
#61553=ORIENTED_EDGE('',*,*,#46610,.T.);
#61554=ORIENTED_EDGE('',*,*,#46614,.F.);
#61555=ORIENTED_EDGE('',*,*,#46615,.F.);
#61556=ORIENTED_EDGE('',*,*,#46616,.T.);
#61557=ORIENTED_EDGE('',*,*,#46617,.T.);
#61558=ORIENTED_EDGE('',*,*,#46618,.F.);
#61559=ORIENTED_EDGE('',*,*,#46619,.F.);
#61560=ORIENTED_EDGE('',*,*,#46620,.T.);
#61561=ORIENTED_EDGE('',*,*,#46615,.T.);
#61562=ORIENTED_EDGE('',*,*,#46621,.F.);
#61563=ORIENTED_EDGE('',*,*,#46622,.F.);
#61564=ORIENTED_EDGE('',*,*,#46623,.T.);
#61565=ORIENTED_EDGE('',*,*,#46619,.T.);
#61566=ORIENTED_EDGE('',*,*,#46624,.F.);
#61567=ORIENTED_EDGE('',*,*,#46617,.F.);
#61568=ORIENTED_EDGE('',*,*,#46625,.T.);
#61569=ORIENTED_EDGE('',*,*,#46622,.T.);
#61570=ORIENTED_EDGE('',*,*,#46626,.F.);
#61571=ORIENTED_EDGE('',*,*,#46627,.F.);
#61572=ORIENTED_EDGE('',*,*,#46628,.T.);
#61573=ORIENTED_EDGE('',*,*,#46629,.T.);
#61574=ORIENTED_EDGE('',*,*,#46630,.F.);
#61575=ORIENTED_EDGE('',*,*,#46631,.F.);
#61576=ORIENTED_EDGE('',*,*,#46632,.T.);
#61577=ORIENTED_EDGE('',*,*,#46627,.T.);
#61578=ORIENTED_EDGE('',*,*,#46633,.F.);
#61579=ORIENTED_EDGE('',*,*,#46634,.F.);
#61580=ORIENTED_EDGE('',*,*,#46635,.T.);
#61581=ORIENTED_EDGE('',*,*,#46631,.T.);
#61582=ORIENTED_EDGE('',*,*,#46636,.F.);
#61583=ORIENTED_EDGE('',*,*,#46629,.F.);
#61584=ORIENTED_EDGE('',*,*,#46637,.T.);
#61585=ORIENTED_EDGE('',*,*,#46634,.T.);
#61586=ORIENTED_EDGE('',*,*,#46638,.F.);
#61587=ORIENTED_EDGE('',*,*,#46639,.F.);
#61588=ORIENTED_EDGE('',*,*,#46640,.T.);
#61589=ORIENTED_EDGE('',*,*,#46641,.T.);
#61590=ORIENTED_EDGE('',*,*,#46642,.F.);
#61591=ORIENTED_EDGE('',*,*,#46643,.F.);
#61592=ORIENTED_EDGE('',*,*,#46644,.T.);
#61593=ORIENTED_EDGE('',*,*,#46639,.T.);
#61594=ORIENTED_EDGE('',*,*,#46645,.F.);
#61595=ORIENTED_EDGE('',*,*,#46646,.F.);
#61596=ORIENTED_EDGE('',*,*,#46647,.T.);
#61597=ORIENTED_EDGE('',*,*,#46643,.T.);
#61598=ORIENTED_EDGE('',*,*,#46648,.F.);
#61599=ORIENTED_EDGE('',*,*,#46641,.F.);
#61600=ORIENTED_EDGE('',*,*,#46649,.T.);
#61601=ORIENTED_EDGE('',*,*,#46646,.T.);
#61602=ORIENTED_EDGE('',*,*,#46650,.F.);
#61603=ORIENTED_EDGE('',*,*,#46651,.F.);
#61604=ORIENTED_EDGE('',*,*,#46652,.T.);
#61605=ORIENTED_EDGE('',*,*,#46653,.T.);
#61606=ORIENTED_EDGE('',*,*,#46654,.F.);
#61607=ORIENTED_EDGE('',*,*,#46655,.F.);
#61608=ORIENTED_EDGE('',*,*,#46656,.T.);
#61609=ORIENTED_EDGE('',*,*,#46651,.T.);
#61610=ORIENTED_EDGE('',*,*,#46657,.F.);
#61611=ORIENTED_EDGE('',*,*,#46658,.F.);
#61612=ORIENTED_EDGE('',*,*,#46659,.T.);
#61613=ORIENTED_EDGE('',*,*,#46655,.T.);
#61614=ORIENTED_EDGE('',*,*,#46660,.F.);
#61615=ORIENTED_EDGE('',*,*,#46653,.F.);
#61616=ORIENTED_EDGE('',*,*,#46661,.T.);
#61617=ORIENTED_EDGE('',*,*,#46658,.T.);
#61618=ORIENTED_EDGE('',*,*,#46662,.F.);
#61619=ORIENTED_EDGE('',*,*,#46663,.F.);
#61620=ORIENTED_EDGE('',*,*,#46664,.T.);
#61621=ORIENTED_EDGE('',*,*,#46665,.T.);
#61622=ORIENTED_EDGE('',*,*,#46666,.F.);
#61623=ORIENTED_EDGE('',*,*,#46667,.F.);
#61624=ORIENTED_EDGE('',*,*,#46668,.T.);
#61625=ORIENTED_EDGE('',*,*,#46663,.T.);
#61626=ORIENTED_EDGE('',*,*,#46669,.F.);
#61627=ORIENTED_EDGE('',*,*,#46670,.F.);
#61628=ORIENTED_EDGE('',*,*,#46671,.T.);
#61629=ORIENTED_EDGE('',*,*,#46667,.T.);
#61630=ORIENTED_EDGE('',*,*,#46672,.F.);
#61631=ORIENTED_EDGE('',*,*,#46665,.F.);
#61632=ORIENTED_EDGE('',*,*,#46673,.T.);
#61633=ORIENTED_EDGE('',*,*,#46670,.T.);
#61634=ORIENTED_EDGE('',*,*,#46674,.F.);
#61635=ORIENTED_EDGE('',*,*,#46675,.F.);
#61636=ORIENTED_EDGE('',*,*,#46676,.T.);
#61637=ORIENTED_EDGE('',*,*,#46677,.T.);
#61638=ORIENTED_EDGE('',*,*,#46678,.F.);
#61639=ORIENTED_EDGE('',*,*,#46679,.F.);
#61640=ORIENTED_EDGE('',*,*,#46680,.T.);
#61641=ORIENTED_EDGE('',*,*,#46675,.T.);
#61642=ORIENTED_EDGE('',*,*,#46681,.F.);
#61643=ORIENTED_EDGE('',*,*,#46682,.F.);
#61644=ORIENTED_EDGE('',*,*,#46683,.T.);
#61645=ORIENTED_EDGE('',*,*,#46679,.T.);
#61646=ORIENTED_EDGE('',*,*,#46684,.F.);
#61647=ORIENTED_EDGE('',*,*,#46677,.F.);
#61648=ORIENTED_EDGE('',*,*,#46685,.T.);
#61649=ORIENTED_EDGE('',*,*,#46682,.T.);
#61650=ORIENTED_EDGE('',*,*,#46686,.F.);
#61651=ORIENTED_EDGE('',*,*,#46687,.F.);
#61652=ORIENTED_EDGE('',*,*,#46688,.T.);
#61653=ORIENTED_EDGE('',*,*,#46689,.T.);
#61654=ORIENTED_EDGE('',*,*,#46690,.F.);
#61655=ORIENTED_EDGE('',*,*,#46691,.F.);
#61656=ORIENTED_EDGE('',*,*,#46692,.T.);
#61657=ORIENTED_EDGE('',*,*,#46687,.T.);
#61658=ORIENTED_EDGE('',*,*,#46693,.F.);
#61659=ORIENTED_EDGE('',*,*,#46694,.F.);
#61660=ORIENTED_EDGE('',*,*,#46695,.T.);
#61661=ORIENTED_EDGE('',*,*,#46691,.T.);
#61662=ORIENTED_EDGE('',*,*,#46696,.F.);
#61663=ORIENTED_EDGE('',*,*,#46689,.F.);
#61664=ORIENTED_EDGE('',*,*,#46697,.T.);
#61665=ORIENTED_EDGE('',*,*,#46694,.T.);
#61666=ORIENTED_EDGE('',*,*,#46698,.F.);
#61667=ORIENTED_EDGE('',*,*,#46699,.F.);
#61668=ORIENTED_EDGE('',*,*,#46700,.T.);
#61669=ORIENTED_EDGE('',*,*,#46701,.T.);
#61670=ORIENTED_EDGE('',*,*,#46702,.F.);
#61671=ORIENTED_EDGE('',*,*,#46703,.F.);
#61672=ORIENTED_EDGE('',*,*,#46704,.T.);
#61673=ORIENTED_EDGE('',*,*,#46699,.T.);
#61674=ORIENTED_EDGE('',*,*,#46705,.F.);
#61675=ORIENTED_EDGE('',*,*,#46706,.F.);
#61676=ORIENTED_EDGE('',*,*,#46707,.T.);
#61677=ORIENTED_EDGE('',*,*,#46703,.T.);
#61678=ORIENTED_EDGE('',*,*,#46708,.F.);
#61679=ORIENTED_EDGE('',*,*,#46701,.F.);
#61680=ORIENTED_EDGE('',*,*,#46709,.T.);
#61681=ORIENTED_EDGE('',*,*,#46706,.T.);
#61682=ORIENTED_EDGE('',*,*,#46710,.F.);
#61683=ORIENTED_EDGE('',*,*,#46711,.F.);
#61684=ORIENTED_EDGE('',*,*,#46712,.T.);
#61685=ORIENTED_EDGE('',*,*,#46713,.T.);
#61686=ORIENTED_EDGE('',*,*,#46714,.F.);
#61687=ORIENTED_EDGE('',*,*,#46715,.F.);
#61688=ORIENTED_EDGE('',*,*,#46716,.T.);
#61689=ORIENTED_EDGE('',*,*,#46711,.T.);
#61690=ORIENTED_EDGE('',*,*,#46717,.F.);
#61691=ORIENTED_EDGE('',*,*,#46718,.F.);
#61692=ORIENTED_EDGE('',*,*,#46719,.T.);
#61693=ORIENTED_EDGE('',*,*,#46715,.T.);
#61694=ORIENTED_EDGE('',*,*,#46720,.F.);
#61695=ORIENTED_EDGE('',*,*,#46713,.F.);
#61696=ORIENTED_EDGE('',*,*,#46721,.T.);
#61697=ORIENTED_EDGE('',*,*,#46718,.T.);
#61698=ORIENTED_EDGE('',*,*,#46722,.F.);
#61699=ORIENTED_EDGE('',*,*,#46723,.F.);
#61700=ORIENTED_EDGE('',*,*,#46724,.T.);
#61701=ORIENTED_EDGE('',*,*,#46725,.T.);
#61702=ORIENTED_EDGE('',*,*,#46726,.F.);
#61703=ORIENTED_EDGE('',*,*,#46727,.F.);
#61704=ORIENTED_EDGE('',*,*,#46728,.T.);
#61705=ORIENTED_EDGE('',*,*,#46723,.T.);
#61706=ORIENTED_EDGE('',*,*,#46729,.F.);
#61707=ORIENTED_EDGE('',*,*,#46730,.F.);
#61708=ORIENTED_EDGE('',*,*,#46731,.T.);
#61709=ORIENTED_EDGE('',*,*,#46727,.T.);
#61710=ORIENTED_EDGE('',*,*,#46732,.F.);
#61711=ORIENTED_EDGE('',*,*,#46725,.F.);
#61712=ORIENTED_EDGE('',*,*,#46733,.T.);
#61713=ORIENTED_EDGE('',*,*,#46730,.T.);
#61714=ORIENTED_EDGE('',*,*,#46734,.F.);
#61715=ORIENTED_EDGE('',*,*,#43509,.F.);
#61716=ORIENTED_EDGE('',*,*,#43504,.F.);
#61717=ORIENTED_EDGE('',*,*,#46735,.T.);
#61718=ORIENTED_EDGE('',*,*,#46736,.F.);
#61719=ORIENTED_EDGE('',*,*,#46737,.F.);
#61720=ORIENTED_EDGE('',*,*,#46738,.T.);
#61721=ORIENTED_EDGE('',*,*,#46739,.T.);
#61722=ORIENTED_EDGE('',*,*,#46740,.F.);
#61723=ORIENTED_EDGE('',*,*,#46735,.F.);
#61724=ORIENTED_EDGE('',*,*,#46741,.T.);
#61725=ORIENTED_EDGE('',*,*,#46742,.T.);
#61726=ORIENTED_EDGE('',*,*,#46743,.F.);
#61727=ORIENTED_EDGE('',*,*,#46739,.F.);
#61728=ORIENTED_EDGE('',*,*,#46744,.T.);
#61729=ORIENTED_EDGE('',*,*,#46737,.T.);
#61730=ORIENTED_EDGE('',*,*,#46745,.F.);
#61731=ORIENTED_EDGE('',*,*,#46742,.F.);
#61732=ORIENTED_EDGE('',*,*,#46746,.T.);
#61733=ORIENTED_EDGE('',*,*,#46747,.T.);
#61734=ORIENTED_EDGE('',*,*,#46748,.F.);
#61735=ORIENTED_EDGE('',*,*,#46749,.F.);
#61736=ORIENTED_EDGE('',*,*,#46750,.T.);
#61737=ORIENTED_EDGE('',*,*,#46751,.T.);
#61738=ORIENTED_EDGE('',*,*,#46752,.F.);
#61739=ORIENTED_EDGE('',*,*,#46747,.F.);
#61740=ORIENTED_EDGE('',*,*,#46753,.T.);
#61741=ORIENTED_EDGE('',*,*,#46754,.T.);
#61742=ORIENTED_EDGE('',*,*,#46755,.F.);
#61743=ORIENTED_EDGE('',*,*,#46751,.F.);
#61744=ORIENTED_EDGE('',*,*,#46756,.T.);
#61745=ORIENTED_EDGE('',*,*,#46749,.T.);
#61746=ORIENTED_EDGE('',*,*,#46757,.F.);
#61747=ORIENTED_EDGE('',*,*,#46754,.F.);
#61748=ORIENTED_EDGE('',*,*,#46758,.T.);
#61749=ORIENTED_EDGE('',*,*,#46759,.T.);
#61750=ORIENTED_EDGE('',*,*,#46760,.F.);
#61751=ORIENTED_EDGE('',*,*,#46761,.F.);
#61752=ORIENTED_EDGE('',*,*,#46762,.T.);
#61753=ORIENTED_EDGE('',*,*,#46763,.T.);
#61754=ORIENTED_EDGE('',*,*,#46764,.F.);
#61755=ORIENTED_EDGE('',*,*,#46759,.F.);
#61756=ORIENTED_EDGE('',*,*,#46765,.T.);
#61757=ORIENTED_EDGE('',*,*,#46766,.T.);
#61758=ORIENTED_EDGE('',*,*,#46767,.F.);
#61759=ORIENTED_EDGE('',*,*,#46763,.F.);
#61760=ORIENTED_EDGE('',*,*,#46768,.T.);
#61761=ORIENTED_EDGE('',*,*,#46761,.T.);
#61762=ORIENTED_EDGE('',*,*,#46769,.F.);
#61763=ORIENTED_EDGE('',*,*,#46766,.F.);
#61764=ORIENTED_EDGE('',*,*,#46770,.T.);
#61765=ORIENTED_EDGE('',*,*,#46771,.T.);
#61766=ORIENTED_EDGE('',*,*,#46772,.F.);
#61767=ORIENTED_EDGE('',*,*,#46773,.F.);
#61768=ORIENTED_EDGE('',*,*,#46774,.T.);
#61769=ORIENTED_EDGE('',*,*,#46775,.T.);
#61770=ORIENTED_EDGE('',*,*,#46776,.F.);
#61771=ORIENTED_EDGE('',*,*,#46771,.F.);
#61772=ORIENTED_EDGE('',*,*,#46777,.T.);
#61773=ORIENTED_EDGE('',*,*,#46778,.T.);
#61774=ORIENTED_EDGE('',*,*,#46779,.F.);
#61775=ORIENTED_EDGE('',*,*,#46775,.F.);
#61776=ORIENTED_EDGE('',*,*,#46780,.T.);
#61777=ORIENTED_EDGE('',*,*,#46773,.T.);
#61778=ORIENTED_EDGE('',*,*,#46781,.F.);
#61779=ORIENTED_EDGE('',*,*,#46778,.F.);
#61780=ORIENTED_EDGE('',*,*,#46782,.T.);
#61781=ORIENTED_EDGE('',*,*,#46783,.T.);
#61782=ORIENTED_EDGE('',*,*,#46784,.F.);
#61783=ORIENTED_EDGE('',*,*,#46785,.F.);
#61784=ORIENTED_EDGE('',*,*,#46786,.T.);
#61785=ORIENTED_EDGE('',*,*,#46787,.T.);
#61786=ORIENTED_EDGE('',*,*,#46788,.F.);
#61787=ORIENTED_EDGE('',*,*,#46783,.F.);
#61788=ORIENTED_EDGE('',*,*,#46789,.T.);
#61789=ORIENTED_EDGE('',*,*,#46790,.T.);
#61790=ORIENTED_EDGE('',*,*,#46791,.F.);
#61791=ORIENTED_EDGE('',*,*,#46787,.F.);
#61792=ORIENTED_EDGE('',*,*,#46792,.T.);
#61793=ORIENTED_EDGE('',*,*,#46785,.T.);
#61794=ORIENTED_EDGE('',*,*,#46793,.F.);
#61795=ORIENTED_EDGE('',*,*,#46790,.F.);
#61796=ORIENTED_EDGE('',*,*,#46794,.T.);
#61797=ORIENTED_EDGE('',*,*,#46795,.T.);
#61798=ORIENTED_EDGE('',*,*,#46796,.F.);
#61799=ORIENTED_EDGE('',*,*,#46797,.F.);
#61800=ORIENTED_EDGE('',*,*,#46798,.T.);
#61801=ORIENTED_EDGE('',*,*,#46799,.T.);
#61802=ORIENTED_EDGE('',*,*,#46800,.F.);
#61803=ORIENTED_EDGE('',*,*,#46795,.F.);
#61804=ORIENTED_EDGE('',*,*,#46801,.T.);
#61805=ORIENTED_EDGE('',*,*,#46802,.T.);
#61806=ORIENTED_EDGE('',*,*,#46803,.F.);
#61807=ORIENTED_EDGE('',*,*,#46799,.F.);
#61808=ORIENTED_EDGE('',*,*,#46804,.T.);
#61809=ORIENTED_EDGE('',*,*,#46797,.T.);
#61810=ORIENTED_EDGE('',*,*,#46805,.F.);
#61811=ORIENTED_EDGE('',*,*,#46802,.F.);
#61812=ORIENTED_EDGE('',*,*,#46806,.T.);
#61813=ORIENTED_EDGE('',*,*,#46807,.T.);
#61814=ORIENTED_EDGE('',*,*,#46808,.F.);
#61815=ORIENTED_EDGE('',*,*,#46809,.F.);
#61816=ORIENTED_EDGE('',*,*,#46810,.T.);
#61817=ORIENTED_EDGE('',*,*,#46811,.T.);
#61818=ORIENTED_EDGE('',*,*,#46812,.F.);
#61819=ORIENTED_EDGE('',*,*,#46807,.F.);
#61820=ORIENTED_EDGE('',*,*,#46813,.T.);
#61821=ORIENTED_EDGE('',*,*,#46814,.T.);
#61822=ORIENTED_EDGE('',*,*,#46815,.F.);
#61823=ORIENTED_EDGE('',*,*,#46811,.F.);
#61824=ORIENTED_EDGE('',*,*,#46816,.T.);
#61825=ORIENTED_EDGE('',*,*,#46809,.T.);
#61826=ORIENTED_EDGE('',*,*,#46817,.F.);
#61827=ORIENTED_EDGE('',*,*,#46814,.F.);
#61828=ORIENTED_EDGE('',*,*,#46818,.T.);
#61829=ORIENTED_EDGE('',*,*,#46819,.T.);
#61830=ORIENTED_EDGE('',*,*,#46820,.F.);
#61831=ORIENTED_EDGE('',*,*,#46821,.F.);
#61832=ORIENTED_EDGE('',*,*,#46822,.T.);
#61833=ORIENTED_EDGE('',*,*,#46823,.T.);
#61834=ORIENTED_EDGE('',*,*,#46824,.F.);
#61835=ORIENTED_EDGE('',*,*,#46819,.F.);
#61836=ORIENTED_EDGE('',*,*,#46825,.T.);
#61837=ORIENTED_EDGE('',*,*,#46826,.T.);
#61838=ORIENTED_EDGE('',*,*,#46827,.F.);
#61839=ORIENTED_EDGE('',*,*,#46823,.F.);
#61840=ORIENTED_EDGE('',*,*,#46828,.T.);
#61841=ORIENTED_EDGE('',*,*,#46821,.T.);
#61842=ORIENTED_EDGE('',*,*,#46829,.F.);
#61843=ORIENTED_EDGE('',*,*,#46826,.F.);
#61844=ORIENTED_EDGE('',*,*,#46830,.T.);
#61845=ORIENTED_EDGE('',*,*,#46831,.T.);
#61846=ORIENTED_EDGE('',*,*,#46832,.F.);
#61847=ORIENTED_EDGE('',*,*,#46833,.F.);
#61848=ORIENTED_EDGE('',*,*,#46834,.T.);
#61849=ORIENTED_EDGE('',*,*,#46835,.T.);
#61850=ORIENTED_EDGE('',*,*,#46836,.F.);
#61851=ORIENTED_EDGE('',*,*,#46831,.F.);
#61852=ORIENTED_EDGE('',*,*,#46837,.T.);
#61853=ORIENTED_EDGE('',*,*,#46838,.T.);
#61854=ORIENTED_EDGE('',*,*,#46839,.F.);
#61855=ORIENTED_EDGE('',*,*,#46835,.F.);
#61856=ORIENTED_EDGE('',*,*,#46840,.T.);
#61857=ORIENTED_EDGE('',*,*,#46833,.T.);
#61858=ORIENTED_EDGE('',*,*,#46841,.F.);
#61859=ORIENTED_EDGE('',*,*,#46838,.F.);
#61860=ORIENTED_EDGE('',*,*,#46842,.T.);
#61861=ORIENTED_EDGE('',*,*,#46843,.T.);
#61862=ORIENTED_EDGE('',*,*,#46844,.F.);
#61863=ORIENTED_EDGE('',*,*,#46845,.F.);
#61864=ORIENTED_EDGE('',*,*,#46846,.T.);
#61865=ORIENTED_EDGE('',*,*,#46847,.T.);
#61866=ORIENTED_EDGE('',*,*,#46848,.F.);
#61867=ORIENTED_EDGE('',*,*,#46843,.F.);
#61868=ORIENTED_EDGE('',*,*,#46849,.T.);
#61869=ORIENTED_EDGE('',*,*,#46850,.T.);
#61870=ORIENTED_EDGE('',*,*,#46851,.F.);
#61871=ORIENTED_EDGE('',*,*,#46847,.F.);
#61872=ORIENTED_EDGE('',*,*,#46852,.T.);
#61873=ORIENTED_EDGE('',*,*,#46845,.T.);
#61874=ORIENTED_EDGE('',*,*,#46853,.F.);
#61875=ORIENTED_EDGE('',*,*,#46850,.F.);
#61876=ORIENTED_EDGE('',*,*,#46854,.T.);
#61877=ORIENTED_EDGE('',*,*,#46855,.T.);
#61878=ORIENTED_EDGE('',*,*,#46856,.F.);
#61879=ORIENTED_EDGE('',*,*,#46857,.F.);
#61880=ORIENTED_EDGE('',*,*,#46858,.T.);
#61881=ORIENTED_EDGE('',*,*,#46859,.T.);
#61882=ORIENTED_EDGE('',*,*,#46860,.F.);
#61883=ORIENTED_EDGE('',*,*,#46855,.F.);
#61884=ORIENTED_EDGE('',*,*,#46861,.T.);
#61885=ORIENTED_EDGE('',*,*,#46862,.T.);
#61886=ORIENTED_EDGE('',*,*,#46863,.F.);
#61887=ORIENTED_EDGE('',*,*,#46859,.F.);
#61888=ORIENTED_EDGE('',*,*,#46864,.T.);
#61889=ORIENTED_EDGE('',*,*,#46857,.T.);
#61890=ORIENTED_EDGE('',*,*,#46865,.F.);
#61891=ORIENTED_EDGE('',*,*,#46862,.F.);
#61892=ORIENTED_EDGE('',*,*,#46866,.T.);
#61893=ORIENTED_EDGE('',*,*,#46867,.T.);
#61894=ORIENTED_EDGE('',*,*,#46868,.F.);
#61895=ORIENTED_EDGE('',*,*,#46869,.F.);
#61896=ORIENTED_EDGE('',*,*,#46870,.T.);
#61897=ORIENTED_EDGE('',*,*,#46871,.T.);
#61898=ORIENTED_EDGE('',*,*,#46872,.F.);
#61899=ORIENTED_EDGE('',*,*,#46867,.F.);
#61900=ORIENTED_EDGE('',*,*,#46873,.T.);
#61901=ORIENTED_EDGE('',*,*,#46874,.T.);
#61902=ORIENTED_EDGE('',*,*,#46875,.F.);
#61903=ORIENTED_EDGE('',*,*,#46871,.F.);
#61904=ORIENTED_EDGE('',*,*,#46876,.T.);
#61905=ORIENTED_EDGE('',*,*,#46869,.T.);
#61906=ORIENTED_EDGE('',*,*,#46877,.F.);
#61907=ORIENTED_EDGE('',*,*,#46874,.F.);
#61908=ORIENTED_EDGE('',*,*,#46878,.T.);
#61909=ORIENTED_EDGE('',*,*,#46879,.T.);
#61910=ORIENTED_EDGE('',*,*,#46880,.F.);
#61911=ORIENTED_EDGE('',*,*,#46881,.F.);
#61912=ORIENTED_EDGE('',*,*,#46882,.T.);
#61913=ORIENTED_EDGE('',*,*,#46883,.T.);
#61914=ORIENTED_EDGE('',*,*,#46884,.F.);
#61915=ORIENTED_EDGE('',*,*,#46879,.F.);
#61916=ORIENTED_EDGE('',*,*,#46885,.T.);
#61917=ORIENTED_EDGE('',*,*,#46886,.T.);
#61918=ORIENTED_EDGE('',*,*,#46887,.F.);
#61919=ORIENTED_EDGE('',*,*,#46883,.F.);
#61920=ORIENTED_EDGE('',*,*,#46888,.T.);
#61921=ORIENTED_EDGE('',*,*,#46881,.T.);
#61922=ORIENTED_EDGE('',*,*,#46889,.F.);
#61923=ORIENTED_EDGE('',*,*,#46886,.F.);
#61924=ORIENTED_EDGE('',*,*,#46890,.T.);
#61925=ORIENTED_EDGE('',*,*,#46891,.T.);
#61926=ORIENTED_EDGE('',*,*,#46892,.F.);
#61927=ORIENTED_EDGE('',*,*,#46893,.F.);
#61928=ORIENTED_EDGE('',*,*,#46894,.T.);
#61929=ORIENTED_EDGE('',*,*,#46895,.T.);
#61930=ORIENTED_EDGE('',*,*,#46896,.F.);
#61931=ORIENTED_EDGE('',*,*,#46891,.F.);
#61932=ORIENTED_EDGE('',*,*,#46897,.T.);
#61933=ORIENTED_EDGE('',*,*,#46898,.T.);
#61934=ORIENTED_EDGE('',*,*,#46899,.F.);
#61935=ORIENTED_EDGE('',*,*,#46895,.F.);
#61936=ORIENTED_EDGE('',*,*,#46900,.T.);
#61937=ORIENTED_EDGE('',*,*,#46893,.T.);
#61938=ORIENTED_EDGE('',*,*,#46901,.F.);
#61939=ORIENTED_EDGE('',*,*,#46898,.F.);
#61940=ORIENTED_EDGE('',*,*,#46902,.T.);
#61941=ORIENTED_EDGE('',*,*,#46903,.T.);
#61942=ORIENTED_EDGE('',*,*,#46904,.F.);
#61943=ORIENTED_EDGE('',*,*,#46905,.F.);
#61944=ORIENTED_EDGE('',*,*,#46906,.T.);
#61945=ORIENTED_EDGE('',*,*,#46907,.T.);
#61946=ORIENTED_EDGE('',*,*,#46908,.F.);
#61947=ORIENTED_EDGE('',*,*,#46903,.F.);
#61948=ORIENTED_EDGE('',*,*,#46909,.T.);
#61949=ORIENTED_EDGE('',*,*,#46910,.T.);
#61950=ORIENTED_EDGE('',*,*,#46911,.F.);
#61951=ORIENTED_EDGE('',*,*,#46907,.F.);
#61952=ORIENTED_EDGE('',*,*,#46912,.T.);
#61953=ORIENTED_EDGE('',*,*,#46905,.T.);
#61954=ORIENTED_EDGE('',*,*,#46913,.F.);
#61955=ORIENTED_EDGE('',*,*,#46910,.F.);
#61956=ORIENTED_EDGE('',*,*,#46914,.T.);
#61957=ORIENTED_EDGE('',*,*,#46915,.T.);
#61958=ORIENTED_EDGE('',*,*,#46916,.F.);
#61959=ORIENTED_EDGE('',*,*,#46917,.F.);
#61960=ORIENTED_EDGE('',*,*,#46918,.T.);
#61961=ORIENTED_EDGE('',*,*,#46919,.T.);
#61962=ORIENTED_EDGE('',*,*,#46920,.F.);
#61963=ORIENTED_EDGE('',*,*,#46915,.F.);
#61964=ORIENTED_EDGE('',*,*,#46921,.T.);
#61965=ORIENTED_EDGE('',*,*,#46922,.T.);
#61966=ORIENTED_EDGE('',*,*,#46923,.F.);
#61967=ORIENTED_EDGE('',*,*,#46919,.F.);
#61968=ORIENTED_EDGE('',*,*,#46924,.T.);
#61969=ORIENTED_EDGE('',*,*,#46917,.T.);
#61970=ORIENTED_EDGE('',*,*,#46925,.F.);
#61971=ORIENTED_EDGE('',*,*,#46922,.F.);
#61972=ORIENTED_EDGE('',*,*,#46926,.T.);
#61973=ORIENTED_EDGE('',*,*,#46927,.T.);
#61974=ORIENTED_EDGE('',*,*,#46928,.F.);
#61975=ORIENTED_EDGE('',*,*,#46929,.F.);
#61976=ORIENTED_EDGE('',*,*,#46930,.T.);
#61977=ORIENTED_EDGE('',*,*,#46931,.T.);
#61978=ORIENTED_EDGE('',*,*,#46932,.F.);
#61979=ORIENTED_EDGE('',*,*,#46927,.F.);
#61980=ORIENTED_EDGE('',*,*,#46933,.T.);
#61981=ORIENTED_EDGE('',*,*,#46934,.T.);
#61982=ORIENTED_EDGE('',*,*,#46935,.F.);
#61983=ORIENTED_EDGE('',*,*,#46931,.F.);
#61984=ORIENTED_EDGE('',*,*,#46936,.T.);
#61985=ORIENTED_EDGE('',*,*,#46929,.T.);
#61986=ORIENTED_EDGE('',*,*,#46937,.F.);
#61987=ORIENTED_EDGE('',*,*,#46934,.F.);
#61988=ORIENTED_EDGE('',*,*,#46938,.T.);
#61989=ORIENTED_EDGE('',*,*,#46939,.T.);
#61990=ORIENTED_EDGE('',*,*,#46940,.F.);
#61991=ORIENTED_EDGE('',*,*,#46941,.F.);
#61992=ORIENTED_EDGE('',*,*,#46942,.T.);
#61993=ORIENTED_EDGE('',*,*,#46943,.T.);
#61994=ORIENTED_EDGE('',*,*,#46944,.F.);
#61995=ORIENTED_EDGE('',*,*,#46939,.F.);
#61996=ORIENTED_EDGE('',*,*,#46945,.T.);
#61997=ORIENTED_EDGE('',*,*,#46946,.T.);
#61998=ORIENTED_EDGE('',*,*,#46947,.F.);
#61999=ORIENTED_EDGE('',*,*,#46943,.F.);
#62000=ORIENTED_EDGE('',*,*,#46948,.T.);
#62001=ORIENTED_EDGE('',*,*,#46941,.T.);
#62002=ORIENTED_EDGE('',*,*,#46949,.F.);
#62003=ORIENTED_EDGE('',*,*,#46946,.F.);
#62004=ORIENTED_EDGE('',*,*,#46950,.T.);
#62005=ORIENTED_EDGE('',*,*,#46951,.T.);
#62006=ORIENTED_EDGE('',*,*,#46952,.F.);
#62007=ORIENTED_EDGE('',*,*,#46953,.F.);
#62008=ORIENTED_EDGE('',*,*,#46954,.T.);
#62009=ORIENTED_EDGE('',*,*,#46955,.T.);
#62010=ORIENTED_EDGE('',*,*,#46956,.F.);
#62011=ORIENTED_EDGE('',*,*,#46951,.F.);
#62012=ORIENTED_EDGE('',*,*,#46957,.T.);
#62013=ORIENTED_EDGE('',*,*,#46958,.T.);
#62014=ORIENTED_EDGE('',*,*,#46959,.F.);
#62015=ORIENTED_EDGE('',*,*,#46955,.F.);
#62016=ORIENTED_EDGE('',*,*,#46960,.T.);
#62017=ORIENTED_EDGE('',*,*,#46953,.T.);
#62018=ORIENTED_EDGE('',*,*,#46961,.F.);
#62019=ORIENTED_EDGE('',*,*,#46958,.F.);
#62020=ORIENTED_EDGE('',*,*,#46962,.T.);
#62021=ORIENTED_EDGE('',*,*,#46963,.T.);
#62022=ORIENTED_EDGE('',*,*,#46964,.F.);
#62023=ORIENTED_EDGE('',*,*,#46965,.F.);
#62024=ORIENTED_EDGE('',*,*,#46966,.T.);
#62025=ORIENTED_EDGE('',*,*,#46967,.T.);
#62026=ORIENTED_EDGE('',*,*,#46968,.F.);
#62027=ORIENTED_EDGE('',*,*,#46963,.F.);
#62028=ORIENTED_EDGE('',*,*,#46969,.T.);
#62029=ORIENTED_EDGE('',*,*,#46970,.T.);
#62030=ORIENTED_EDGE('',*,*,#46971,.F.);
#62031=ORIENTED_EDGE('',*,*,#46967,.F.);
#62032=ORIENTED_EDGE('',*,*,#46972,.T.);
#62033=ORIENTED_EDGE('',*,*,#46965,.T.);
#62034=ORIENTED_EDGE('',*,*,#46973,.F.);
#62035=ORIENTED_EDGE('',*,*,#46970,.F.);
#62036=ORIENTED_EDGE('',*,*,#46974,.T.);
#62037=ORIENTED_EDGE('',*,*,#46975,.T.);
#62038=ORIENTED_EDGE('',*,*,#46976,.F.);
#62039=ORIENTED_EDGE('',*,*,#46977,.F.);
#62040=ORIENTED_EDGE('',*,*,#46978,.T.);
#62041=ORIENTED_EDGE('',*,*,#46979,.T.);
#62042=ORIENTED_EDGE('',*,*,#46980,.F.);
#62043=ORIENTED_EDGE('',*,*,#46975,.F.);
#62044=ORIENTED_EDGE('',*,*,#46981,.T.);
#62045=ORIENTED_EDGE('',*,*,#46982,.T.);
#62046=ORIENTED_EDGE('',*,*,#46983,.F.);
#62047=ORIENTED_EDGE('',*,*,#46979,.F.);
#62048=ORIENTED_EDGE('',*,*,#46984,.T.);
#62049=ORIENTED_EDGE('',*,*,#46977,.T.);
#62050=ORIENTED_EDGE('',*,*,#46985,.F.);
#62051=ORIENTED_EDGE('',*,*,#46982,.F.);
#62052=ORIENTED_EDGE('',*,*,#46986,.T.);
#62053=ORIENTED_EDGE('',*,*,#46987,.T.);
#62054=ORIENTED_EDGE('',*,*,#46988,.F.);
#62055=ORIENTED_EDGE('',*,*,#46989,.F.);
#62056=ORIENTED_EDGE('',*,*,#46990,.T.);
#62057=ORIENTED_EDGE('',*,*,#46991,.T.);
#62058=ORIENTED_EDGE('',*,*,#46992,.F.);
#62059=ORIENTED_EDGE('',*,*,#46987,.F.);
#62060=ORIENTED_EDGE('',*,*,#46993,.T.);
#62061=ORIENTED_EDGE('',*,*,#46994,.T.);
#62062=ORIENTED_EDGE('',*,*,#46995,.F.);
#62063=ORIENTED_EDGE('',*,*,#46991,.F.);
#62064=ORIENTED_EDGE('',*,*,#46996,.T.);
#62065=ORIENTED_EDGE('',*,*,#46989,.T.);
#62066=ORIENTED_EDGE('',*,*,#46997,.F.);
#62067=ORIENTED_EDGE('',*,*,#46994,.F.);
#62068=ORIENTED_EDGE('',*,*,#46998,.T.);
#62069=ORIENTED_EDGE('',*,*,#46999,.T.);
#62070=ORIENTED_EDGE('',*,*,#47000,.F.);
#62071=ORIENTED_EDGE('',*,*,#47001,.F.);
#62072=ORIENTED_EDGE('',*,*,#47002,.T.);
#62073=ORIENTED_EDGE('',*,*,#47003,.T.);
#62074=ORIENTED_EDGE('',*,*,#47004,.F.);
#62075=ORIENTED_EDGE('',*,*,#46999,.F.);
#62076=ORIENTED_EDGE('',*,*,#47005,.T.);
#62077=ORIENTED_EDGE('',*,*,#47006,.T.);
#62078=ORIENTED_EDGE('',*,*,#47007,.F.);
#62079=ORIENTED_EDGE('',*,*,#47003,.F.);
#62080=ORIENTED_EDGE('',*,*,#47008,.T.);
#62081=ORIENTED_EDGE('',*,*,#47001,.T.);
#62082=ORIENTED_EDGE('',*,*,#47009,.F.);
#62083=ORIENTED_EDGE('',*,*,#47006,.F.);
#62084=ORIENTED_EDGE('',*,*,#47010,.T.);
#62085=ORIENTED_EDGE('',*,*,#47011,.T.);
#62086=ORIENTED_EDGE('',*,*,#47012,.F.);
#62087=ORIENTED_EDGE('',*,*,#47013,.F.);
#62088=ORIENTED_EDGE('',*,*,#47014,.T.);
#62089=ORIENTED_EDGE('',*,*,#47015,.T.);
#62090=ORIENTED_EDGE('',*,*,#47016,.F.);
#62091=ORIENTED_EDGE('',*,*,#47011,.F.);
#62092=ORIENTED_EDGE('',*,*,#47017,.T.);
#62093=ORIENTED_EDGE('',*,*,#47018,.T.);
#62094=ORIENTED_EDGE('',*,*,#47019,.F.);
#62095=ORIENTED_EDGE('',*,*,#47015,.F.);
#62096=ORIENTED_EDGE('',*,*,#47020,.T.);
#62097=ORIENTED_EDGE('',*,*,#47013,.T.);
#62098=ORIENTED_EDGE('',*,*,#47021,.F.);
#62099=ORIENTED_EDGE('',*,*,#47018,.F.);
#62100=ORIENTED_EDGE('',*,*,#47022,.T.);
#62101=ORIENTED_EDGE('',*,*,#47023,.T.);
#62102=ORIENTED_EDGE('',*,*,#47024,.F.);
#62103=ORIENTED_EDGE('',*,*,#47025,.F.);
#62104=ORIENTED_EDGE('',*,*,#47026,.T.);
#62105=ORIENTED_EDGE('',*,*,#47027,.T.);
#62106=ORIENTED_EDGE('',*,*,#47028,.F.);
#62107=ORIENTED_EDGE('',*,*,#47023,.F.);
#62108=ORIENTED_EDGE('',*,*,#47029,.T.);
#62109=ORIENTED_EDGE('',*,*,#47030,.T.);
#62110=ORIENTED_EDGE('',*,*,#47031,.F.);
#62111=ORIENTED_EDGE('',*,*,#47027,.F.);
#62112=ORIENTED_EDGE('',*,*,#47032,.T.);
#62113=ORIENTED_EDGE('',*,*,#47025,.T.);
#62114=ORIENTED_EDGE('',*,*,#47033,.F.);
#62115=ORIENTED_EDGE('',*,*,#47030,.F.);
#62116=ORIENTED_EDGE('',*,*,#47034,.T.);
#62117=ORIENTED_EDGE('',*,*,#47035,.T.);
#62118=ORIENTED_EDGE('',*,*,#47036,.F.);
#62119=ORIENTED_EDGE('',*,*,#47037,.F.);
#62120=ORIENTED_EDGE('',*,*,#47038,.T.);
#62121=ORIENTED_EDGE('',*,*,#47039,.T.);
#62122=ORIENTED_EDGE('',*,*,#47040,.F.);
#62123=ORIENTED_EDGE('',*,*,#47035,.F.);
#62124=ORIENTED_EDGE('',*,*,#47041,.T.);
#62125=ORIENTED_EDGE('',*,*,#47042,.T.);
#62126=ORIENTED_EDGE('',*,*,#47043,.F.);
#62127=ORIENTED_EDGE('',*,*,#47039,.F.);
#62128=ORIENTED_EDGE('',*,*,#47044,.T.);
#62129=ORIENTED_EDGE('',*,*,#47037,.T.);
#62130=ORIENTED_EDGE('',*,*,#47045,.F.);
#62131=ORIENTED_EDGE('',*,*,#47042,.F.);
#62132=ORIENTED_EDGE('',*,*,#47046,.T.);
#62133=ORIENTED_EDGE('',*,*,#47047,.T.);
#62134=ORIENTED_EDGE('',*,*,#47048,.F.);
#62135=ORIENTED_EDGE('',*,*,#47049,.F.);
#62136=ORIENTED_EDGE('',*,*,#47050,.T.);
#62137=ORIENTED_EDGE('',*,*,#47051,.T.);
#62138=ORIENTED_EDGE('',*,*,#47052,.F.);
#62139=ORIENTED_EDGE('',*,*,#47047,.F.);
#62140=ORIENTED_EDGE('',*,*,#47053,.T.);
#62141=ORIENTED_EDGE('',*,*,#47054,.T.);
#62142=ORIENTED_EDGE('',*,*,#47055,.F.);
#62143=ORIENTED_EDGE('',*,*,#47051,.F.);
#62144=ORIENTED_EDGE('',*,*,#47056,.T.);
#62145=ORIENTED_EDGE('',*,*,#47049,.T.);
#62146=ORIENTED_EDGE('',*,*,#47057,.F.);
#62147=ORIENTED_EDGE('',*,*,#47054,.F.);
#62148=ORIENTED_EDGE('',*,*,#47058,.T.);
#62149=ORIENTED_EDGE('',*,*,#47059,.T.);
#62150=ORIENTED_EDGE('',*,*,#47060,.F.);
#62151=ORIENTED_EDGE('',*,*,#47061,.F.);
#62152=ORIENTED_EDGE('',*,*,#47062,.T.);
#62153=ORIENTED_EDGE('',*,*,#47063,.T.);
#62154=ORIENTED_EDGE('',*,*,#47064,.F.);
#62155=ORIENTED_EDGE('',*,*,#47059,.F.);
#62156=ORIENTED_EDGE('',*,*,#47065,.T.);
#62157=ORIENTED_EDGE('',*,*,#47066,.T.);
#62158=ORIENTED_EDGE('',*,*,#47067,.F.);
#62159=ORIENTED_EDGE('',*,*,#47063,.F.);
#62160=ORIENTED_EDGE('',*,*,#47068,.T.);
#62161=ORIENTED_EDGE('',*,*,#47061,.T.);
#62162=ORIENTED_EDGE('',*,*,#47069,.F.);
#62163=ORIENTED_EDGE('',*,*,#47066,.F.);
#62164=ORIENTED_EDGE('',*,*,#47070,.T.);
#62165=ORIENTED_EDGE('',*,*,#47071,.T.);
#62166=ORIENTED_EDGE('',*,*,#47072,.F.);
#62167=ORIENTED_EDGE('',*,*,#47073,.F.);
#62168=ORIENTED_EDGE('',*,*,#47074,.T.);
#62169=ORIENTED_EDGE('',*,*,#47075,.T.);
#62170=ORIENTED_EDGE('',*,*,#47076,.F.);
#62171=ORIENTED_EDGE('',*,*,#47071,.F.);
#62172=ORIENTED_EDGE('',*,*,#47077,.T.);
#62173=ORIENTED_EDGE('',*,*,#47078,.T.);
#62174=ORIENTED_EDGE('',*,*,#47079,.F.);
#62175=ORIENTED_EDGE('',*,*,#47075,.F.);
#62176=ORIENTED_EDGE('',*,*,#47080,.T.);
#62177=ORIENTED_EDGE('',*,*,#47073,.T.);
#62178=ORIENTED_EDGE('',*,*,#47081,.F.);
#62179=ORIENTED_EDGE('',*,*,#47078,.F.);
#62180=ORIENTED_EDGE('',*,*,#47082,.T.);
#62181=ORIENTED_EDGE('',*,*,#47083,.T.);
#62182=ORIENTED_EDGE('',*,*,#47084,.F.);
#62183=ORIENTED_EDGE('',*,*,#47085,.F.);
#62184=ORIENTED_EDGE('',*,*,#47086,.T.);
#62185=ORIENTED_EDGE('',*,*,#47087,.T.);
#62186=ORIENTED_EDGE('',*,*,#47088,.F.);
#62187=ORIENTED_EDGE('',*,*,#47083,.F.);
#62188=ORIENTED_EDGE('',*,*,#47089,.T.);
#62189=ORIENTED_EDGE('',*,*,#47090,.T.);
#62190=ORIENTED_EDGE('',*,*,#47091,.F.);
#62191=ORIENTED_EDGE('',*,*,#47087,.F.);
#62192=ORIENTED_EDGE('',*,*,#47092,.T.);
#62193=ORIENTED_EDGE('',*,*,#47085,.T.);
#62194=ORIENTED_EDGE('',*,*,#47093,.F.);
#62195=ORIENTED_EDGE('',*,*,#47090,.F.);
#62196=ORIENTED_EDGE('',*,*,#47094,.T.);
#62197=ORIENTED_EDGE('',*,*,#47095,.T.);
#62198=ORIENTED_EDGE('',*,*,#47096,.F.);
#62199=ORIENTED_EDGE('',*,*,#47097,.F.);
#62200=ORIENTED_EDGE('',*,*,#47098,.T.);
#62201=ORIENTED_EDGE('',*,*,#47099,.T.);
#62202=ORIENTED_EDGE('',*,*,#47100,.F.);
#62203=ORIENTED_EDGE('',*,*,#47095,.F.);
#62204=ORIENTED_EDGE('',*,*,#47101,.T.);
#62205=ORIENTED_EDGE('',*,*,#47102,.T.);
#62206=ORIENTED_EDGE('',*,*,#47103,.F.);
#62207=ORIENTED_EDGE('',*,*,#47099,.F.);
#62208=ORIENTED_EDGE('',*,*,#47104,.T.);
#62209=ORIENTED_EDGE('',*,*,#47097,.T.);
#62210=ORIENTED_EDGE('',*,*,#47105,.F.);
#62211=ORIENTED_EDGE('',*,*,#47102,.F.);
#62212=ORIENTED_EDGE('',*,*,#47106,.T.);
#62213=ORIENTED_EDGE('',*,*,#47107,.T.);
#62214=ORIENTED_EDGE('',*,*,#47108,.F.);
#62215=ORIENTED_EDGE('',*,*,#47109,.F.);
#62216=ORIENTED_EDGE('',*,*,#47110,.T.);
#62217=ORIENTED_EDGE('',*,*,#47111,.T.);
#62218=ORIENTED_EDGE('',*,*,#47112,.F.);
#62219=ORIENTED_EDGE('',*,*,#47107,.F.);
#62220=ORIENTED_EDGE('',*,*,#47113,.T.);
#62221=ORIENTED_EDGE('',*,*,#47114,.T.);
#62222=ORIENTED_EDGE('',*,*,#47115,.F.);
#62223=ORIENTED_EDGE('',*,*,#47111,.F.);
#62224=ORIENTED_EDGE('',*,*,#47116,.T.);
#62225=ORIENTED_EDGE('',*,*,#47109,.T.);
#62226=ORIENTED_EDGE('',*,*,#47117,.F.);
#62227=ORIENTED_EDGE('',*,*,#47114,.F.);
#62228=ORIENTED_EDGE('',*,*,#47118,.T.);
#62229=ORIENTED_EDGE('',*,*,#47119,.T.);
#62230=ORIENTED_EDGE('',*,*,#47120,.F.);
#62231=ORIENTED_EDGE('',*,*,#47121,.F.);
#62232=ORIENTED_EDGE('',*,*,#47122,.T.);
#62233=ORIENTED_EDGE('',*,*,#47123,.T.);
#62234=ORIENTED_EDGE('',*,*,#47124,.F.);
#62235=ORIENTED_EDGE('',*,*,#47119,.F.);
#62236=ORIENTED_EDGE('',*,*,#47125,.T.);
#62237=ORIENTED_EDGE('',*,*,#47126,.T.);
#62238=ORIENTED_EDGE('',*,*,#47127,.F.);
#62239=ORIENTED_EDGE('',*,*,#47123,.F.);
#62240=ORIENTED_EDGE('',*,*,#47128,.T.);
#62241=ORIENTED_EDGE('',*,*,#47121,.T.);
#62242=ORIENTED_EDGE('',*,*,#47129,.F.);
#62243=ORIENTED_EDGE('',*,*,#47126,.F.);
#62244=ORIENTED_EDGE('',*,*,#47130,.T.);
#62245=ORIENTED_EDGE('',*,*,#47131,.T.);
#62246=ORIENTED_EDGE('',*,*,#47132,.F.);
#62247=ORIENTED_EDGE('',*,*,#47133,.F.);
#62248=ORIENTED_EDGE('',*,*,#47134,.T.);
#62249=ORIENTED_EDGE('',*,*,#47135,.T.);
#62250=ORIENTED_EDGE('',*,*,#47136,.F.);
#62251=ORIENTED_EDGE('',*,*,#47131,.F.);
#62252=ORIENTED_EDGE('',*,*,#47137,.T.);
#62253=ORIENTED_EDGE('',*,*,#47138,.T.);
#62254=ORIENTED_EDGE('',*,*,#47139,.F.);
#62255=ORIENTED_EDGE('',*,*,#47135,.F.);
#62256=ORIENTED_EDGE('',*,*,#47140,.T.);
#62257=ORIENTED_EDGE('',*,*,#47133,.T.);
#62258=ORIENTED_EDGE('',*,*,#47141,.F.);
#62259=ORIENTED_EDGE('',*,*,#47138,.F.);
#62260=ORIENTED_EDGE('',*,*,#47142,.T.);
#62261=ORIENTED_EDGE('',*,*,#47143,.T.);
#62262=ORIENTED_EDGE('',*,*,#47144,.F.);
#62263=ORIENTED_EDGE('',*,*,#47145,.F.);
#62264=ORIENTED_EDGE('',*,*,#47146,.T.);
#62265=ORIENTED_EDGE('',*,*,#47147,.T.);
#62266=ORIENTED_EDGE('',*,*,#47148,.F.);
#62267=ORIENTED_EDGE('',*,*,#47143,.F.);
#62268=ORIENTED_EDGE('',*,*,#47149,.T.);
#62269=ORIENTED_EDGE('',*,*,#47150,.T.);
#62270=ORIENTED_EDGE('',*,*,#47151,.F.);
#62271=ORIENTED_EDGE('',*,*,#47147,.F.);
#62272=ORIENTED_EDGE('',*,*,#47152,.T.);
#62273=ORIENTED_EDGE('',*,*,#47145,.T.);
#62274=ORIENTED_EDGE('',*,*,#47153,.F.);
#62275=ORIENTED_EDGE('',*,*,#47150,.F.);
#62276=ORIENTED_EDGE('',*,*,#47154,.T.);
#62277=ORIENTED_EDGE('',*,*,#47155,.T.);
#62278=ORIENTED_EDGE('',*,*,#47156,.F.);
#62279=ORIENTED_EDGE('',*,*,#47157,.F.);
#62280=ORIENTED_EDGE('',*,*,#47158,.T.);
#62281=ORIENTED_EDGE('',*,*,#47159,.T.);
#62282=ORIENTED_EDGE('',*,*,#47160,.F.);
#62283=ORIENTED_EDGE('',*,*,#47155,.F.);
#62284=ORIENTED_EDGE('',*,*,#47161,.T.);
#62285=ORIENTED_EDGE('',*,*,#47162,.T.);
#62286=ORIENTED_EDGE('',*,*,#47163,.F.);
#62287=ORIENTED_EDGE('',*,*,#47159,.F.);
#62288=ORIENTED_EDGE('',*,*,#47164,.T.);
#62289=ORIENTED_EDGE('',*,*,#47157,.T.);
#62290=ORIENTED_EDGE('',*,*,#47165,.F.);
#62291=ORIENTED_EDGE('',*,*,#47162,.F.);
#62292=ORIENTED_EDGE('',*,*,#47166,.T.);
#62293=ORIENTED_EDGE('',*,*,#47167,.T.);
#62294=ORIENTED_EDGE('',*,*,#47168,.F.);
#62295=ORIENTED_EDGE('',*,*,#47169,.F.);
#62296=ORIENTED_EDGE('',*,*,#47170,.T.);
#62297=ORIENTED_EDGE('',*,*,#47171,.T.);
#62298=ORIENTED_EDGE('',*,*,#47172,.F.);
#62299=ORIENTED_EDGE('',*,*,#47167,.F.);
#62300=ORIENTED_EDGE('',*,*,#47173,.T.);
#62301=ORIENTED_EDGE('',*,*,#47174,.T.);
#62302=ORIENTED_EDGE('',*,*,#47175,.F.);
#62303=ORIENTED_EDGE('',*,*,#47171,.F.);
#62304=ORIENTED_EDGE('',*,*,#47176,.T.);
#62305=ORIENTED_EDGE('',*,*,#47169,.T.);
#62306=ORIENTED_EDGE('',*,*,#47177,.F.);
#62307=ORIENTED_EDGE('',*,*,#47174,.F.);
#62308=ORIENTED_EDGE('',*,*,#47178,.T.);
#62309=ORIENTED_EDGE('',*,*,#47179,.T.);
#62310=ORIENTED_EDGE('',*,*,#47180,.F.);
#62311=ORIENTED_EDGE('',*,*,#47181,.F.);
#62312=ORIENTED_EDGE('',*,*,#47182,.T.);
#62313=ORIENTED_EDGE('',*,*,#47183,.T.);
#62314=ORIENTED_EDGE('',*,*,#47184,.F.);
#62315=ORIENTED_EDGE('',*,*,#47179,.F.);
#62316=ORIENTED_EDGE('',*,*,#47185,.T.);
#62317=ORIENTED_EDGE('',*,*,#47186,.T.);
#62318=ORIENTED_EDGE('',*,*,#47187,.F.);
#62319=ORIENTED_EDGE('',*,*,#47183,.F.);
#62320=ORIENTED_EDGE('',*,*,#47188,.T.);
#62321=ORIENTED_EDGE('',*,*,#47181,.T.);
#62322=ORIENTED_EDGE('',*,*,#47189,.F.);
#62323=ORIENTED_EDGE('',*,*,#47186,.F.);
#62324=ORIENTED_EDGE('',*,*,#47190,.T.);
#62325=ORIENTED_EDGE('',*,*,#47191,.T.);
#62326=ORIENTED_EDGE('',*,*,#47192,.F.);
#62327=ORIENTED_EDGE('',*,*,#47193,.F.);
#62328=ORIENTED_EDGE('',*,*,#47194,.T.);
#62329=ORIENTED_EDGE('',*,*,#47195,.T.);
#62330=ORIENTED_EDGE('',*,*,#47196,.F.);
#62331=ORIENTED_EDGE('',*,*,#47191,.F.);
#62332=ORIENTED_EDGE('',*,*,#47197,.T.);
#62333=ORIENTED_EDGE('',*,*,#47198,.T.);
#62334=ORIENTED_EDGE('',*,*,#47199,.F.);
#62335=ORIENTED_EDGE('',*,*,#47195,.F.);
#62336=ORIENTED_EDGE('',*,*,#47200,.T.);
#62337=ORIENTED_EDGE('',*,*,#47193,.T.);
#62338=ORIENTED_EDGE('',*,*,#47201,.F.);
#62339=ORIENTED_EDGE('',*,*,#47198,.F.);
#62340=ORIENTED_EDGE('',*,*,#47202,.T.);
#62341=ORIENTED_EDGE('',*,*,#47203,.T.);
#62342=ORIENTED_EDGE('',*,*,#47204,.F.);
#62343=ORIENTED_EDGE('',*,*,#47205,.F.);
#62344=ORIENTED_EDGE('',*,*,#47206,.T.);
#62345=ORIENTED_EDGE('',*,*,#47207,.T.);
#62346=ORIENTED_EDGE('',*,*,#47208,.F.);
#62347=ORIENTED_EDGE('',*,*,#47203,.F.);
#62348=ORIENTED_EDGE('',*,*,#47209,.T.);
#62349=ORIENTED_EDGE('',*,*,#47210,.T.);
#62350=ORIENTED_EDGE('',*,*,#47211,.F.);
#62351=ORIENTED_EDGE('',*,*,#47207,.F.);
#62352=ORIENTED_EDGE('',*,*,#47212,.T.);
#62353=ORIENTED_EDGE('',*,*,#47205,.T.);
#62354=ORIENTED_EDGE('',*,*,#47213,.F.);
#62355=ORIENTED_EDGE('',*,*,#47210,.F.);
#62356=ORIENTED_EDGE('',*,*,#47214,.T.);
#62357=ORIENTED_EDGE('',*,*,#47215,.T.);
#62358=ORIENTED_EDGE('',*,*,#47216,.F.);
#62359=ORIENTED_EDGE('',*,*,#47217,.F.);
#62360=ORIENTED_EDGE('',*,*,#47218,.T.);
#62361=ORIENTED_EDGE('',*,*,#47219,.T.);
#62362=ORIENTED_EDGE('',*,*,#47220,.F.);
#62363=ORIENTED_EDGE('',*,*,#47215,.F.);
#62364=ORIENTED_EDGE('',*,*,#47221,.T.);
#62365=ORIENTED_EDGE('',*,*,#47222,.T.);
#62366=ORIENTED_EDGE('',*,*,#47223,.F.);
#62367=ORIENTED_EDGE('',*,*,#47219,.F.);
#62368=ORIENTED_EDGE('',*,*,#47224,.T.);
#62369=ORIENTED_EDGE('',*,*,#47217,.T.);
#62370=ORIENTED_EDGE('',*,*,#47225,.F.);
#62371=ORIENTED_EDGE('',*,*,#47222,.F.);
#62372=ORIENTED_EDGE('',*,*,#47226,.T.);
#62373=ORIENTED_EDGE('',*,*,#47227,.T.);
#62374=ORIENTED_EDGE('',*,*,#47228,.F.);
#62375=ORIENTED_EDGE('',*,*,#47229,.F.);
#62376=ORIENTED_EDGE('',*,*,#47230,.T.);
#62377=ORIENTED_EDGE('',*,*,#47231,.T.);
#62378=ORIENTED_EDGE('',*,*,#47232,.F.);
#62379=ORIENTED_EDGE('',*,*,#47227,.F.);
#62380=ORIENTED_EDGE('',*,*,#47233,.T.);
#62381=ORIENTED_EDGE('',*,*,#47234,.T.);
#62382=ORIENTED_EDGE('',*,*,#47235,.F.);
#62383=ORIENTED_EDGE('',*,*,#47231,.F.);
#62384=ORIENTED_EDGE('',*,*,#47236,.T.);
#62385=ORIENTED_EDGE('',*,*,#47229,.T.);
#62386=ORIENTED_EDGE('',*,*,#47237,.F.);
#62387=ORIENTED_EDGE('',*,*,#47234,.F.);
#62388=ORIENTED_EDGE('',*,*,#47238,.T.);
#62389=ORIENTED_EDGE('',*,*,#47239,.T.);
#62390=ORIENTED_EDGE('',*,*,#47240,.F.);
#62391=ORIENTED_EDGE('',*,*,#47241,.F.);
#62392=ORIENTED_EDGE('',*,*,#47242,.T.);
#62393=ORIENTED_EDGE('',*,*,#47243,.T.);
#62394=ORIENTED_EDGE('',*,*,#47244,.F.);
#62395=ORIENTED_EDGE('',*,*,#47239,.F.);
#62396=ORIENTED_EDGE('',*,*,#47245,.T.);
#62397=ORIENTED_EDGE('',*,*,#47246,.T.);
#62398=ORIENTED_EDGE('',*,*,#47247,.F.);
#62399=ORIENTED_EDGE('',*,*,#47243,.F.);
#62400=ORIENTED_EDGE('',*,*,#47248,.T.);
#62401=ORIENTED_EDGE('',*,*,#47241,.T.);
#62402=ORIENTED_EDGE('',*,*,#47249,.F.);
#62403=ORIENTED_EDGE('',*,*,#47246,.F.);
#62404=ORIENTED_EDGE('',*,*,#47250,.T.);
#62405=ORIENTED_EDGE('',*,*,#47251,.T.);
#62406=ORIENTED_EDGE('',*,*,#47252,.F.);
#62407=ORIENTED_EDGE('',*,*,#47253,.F.);
#62408=ORIENTED_EDGE('',*,*,#47254,.T.);
#62409=ORIENTED_EDGE('',*,*,#47255,.T.);
#62410=ORIENTED_EDGE('',*,*,#47256,.F.);
#62411=ORIENTED_EDGE('',*,*,#47251,.F.);
#62412=ORIENTED_EDGE('',*,*,#47257,.T.);
#62413=ORIENTED_EDGE('',*,*,#47258,.T.);
#62414=ORIENTED_EDGE('',*,*,#47259,.F.);
#62415=ORIENTED_EDGE('',*,*,#47255,.F.);
#62416=ORIENTED_EDGE('',*,*,#47260,.T.);
#62417=ORIENTED_EDGE('',*,*,#47253,.T.);
#62418=ORIENTED_EDGE('',*,*,#47261,.F.);
#62419=ORIENTED_EDGE('',*,*,#47258,.F.);
#62420=ORIENTED_EDGE('',*,*,#47262,.T.);
#62421=ORIENTED_EDGE('',*,*,#47263,.T.);
#62422=ORIENTED_EDGE('',*,*,#47264,.F.);
#62423=ORIENTED_EDGE('',*,*,#47265,.F.);
#62424=ORIENTED_EDGE('',*,*,#47266,.T.);
#62425=ORIENTED_EDGE('',*,*,#47267,.T.);
#62426=ORIENTED_EDGE('',*,*,#47268,.F.);
#62427=ORIENTED_EDGE('',*,*,#47263,.F.);
#62428=ORIENTED_EDGE('',*,*,#47269,.T.);
#62429=ORIENTED_EDGE('',*,*,#47270,.T.);
#62430=ORIENTED_EDGE('',*,*,#47271,.F.);
#62431=ORIENTED_EDGE('',*,*,#47267,.F.);
#62432=ORIENTED_EDGE('',*,*,#47272,.T.);
#62433=ORIENTED_EDGE('',*,*,#47265,.T.);
#62434=ORIENTED_EDGE('',*,*,#47273,.F.);
#62435=ORIENTED_EDGE('',*,*,#47270,.F.);
#62436=ORIENTED_EDGE('',*,*,#47274,.T.);
#62437=ORIENTED_EDGE('',*,*,#47275,.T.);
#62438=ORIENTED_EDGE('',*,*,#47276,.F.);
#62439=ORIENTED_EDGE('',*,*,#47277,.F.);
#62440=ORIENTED_EDGE('',*,*,#47278,.T.);
#62441=ORIENTED_EDGE('',*,*,#47279,.T.);
#62442=ORIENTED_EDGE('',*,*,#47280,.F.);
#62443=ORIENTED_EDGE('',*,*,#47275,.F.);
#62444=ORIENTED_EDGE('',*,*,#47281,.T.);
#62445=ORIENTED_EDGE('',*,*,#47282,.T.);
#62446=ORIENTED_EDGE('',*,*,#47283,.F.);
#62447=ORIENTED_EDGE('',*,*,#47279,.F.);
#62448=ORIENTED_EDGE('',*,*,#47284,.T.);
#62449=ORIENTED_EDGE('',*,*,#47277,.T.);
#62450=ORIENTED_EDGE('',*,*,#47285,.F.);
#62451=ORIENTED_EDGE('',*,*,#47282,.F.);
#62452=ORIENTED_EDGE('',*,*,#47286,.T.);
#62453=ORIENTED_EDGE('',*,*,#47287,.T.);
#62454=ORIENTED_EDGE('',*,*,#47288,.F.);
#62455=ORIENTED_EDGE('',*,*,#47289,.F.);
#62456=ORIENTED_EDGE('',*,*,#47290,.T.);
#62457=ORIENTED_EDGE('',*,*,#47291,.T.);
#62458=ORIENTED_EDGE('',*,*,#47292,.F.);
#62459=ORIENTED_EDGE('',*,*,#47287,.F.);
#62460=ORIENTED_EDGE('',*,*,#47293,.T.);
#62461=ORIENTED_EDGE('',*,*,#47294,.T.);
#62462=ORIENTED_EDGE('',*,*,#47295,.F.);
#62463=ORIENTED_EDGE('',*,*,#47291,.F.);
#62464=ORIENTED_EDGE('',*,*,#47296,.T.);
#62465=ORIENTED_EDGE('',*,*,#47289,.T.);
#62466=ORIENTED_EDGE('',*,*,#47297,.F.);
#62467=ORIENTED_EDGE('',*,*,#47294,.F.);
#62468=ORIENTED_EDGE('',*,*,#47298,.T.);
#62469=ORIENTED_EDGE('',*,*,#47299,.T.);
#62470=ORIENTED_EDGE('',*,*,#47300,.F.);
#62471=ORIENTED_EDGE('',*,*,#47301,.F.);
#62472=ORIENTED_EDGE('',*,*,#47302,.T.);
#62473=ORIENTED_EDGE('',*,*,#47303,.T.);
#62474=ORIENTED_EDGE('',*,*,#47304,.F.);
#62475=ORIENTED_EDGE('',*,*,#47299,.F.);
#62476=ORIENTED_EDGE('',*,*,#47305,.T.);
#62477=ORIENTED_EDGE('',*,*,#47306,.T.);
#62478=ORIENTED_EDGE('',*,*,#47307,.F.);
#62479=ORIENTED_EDGE('',*,*,#47303,.F.);
#62480=ORIENTED_EDGE('',*,*,#47308,.T.);
#62481=ORIENTED_EDGE('',*,*,#47301,.T.);
#62482=ORIENTED_EDGE('',*,*,#47309,.F.);
#62483=ORIENTED_EDGE('',*,*,#47306,.F.);
#62484=ORIENTED_EDGE('',*,*,#47310,.T.);
#62485=ORIENTED_EDGE('',*,*,#47311,.T.);
#62486=ORIENTED_EDGE('',*,*,#47312,.F.);
#62487=ORIENTED_EDGE('',*,*,#47313,.F.);
#62488=ORIENTED_EDGE('',*,*,#47314,.T.);
#62489=ORIENTED_EDGE('',*,*,#47315,.T.);
#62490=ORIENTED_EDGE('',*,*,#47316,.F.);
#62491=ORIENTED_EDGE('',*,*,#47311,.F.);
#62492=ORIENTED_EDGE('',*,*,#47317,.T.);
#62493=ORIENTED_EDGE('',*,*,#47318,.T.);
#62494=ORIENTED_EDGE('',*,*,#47319,.F.);
#62495=ORIENTED_EDGE('',*,*,#47315,.F.);
#62496=ORIENTED_EDGE('',*,*,#47320,.T.);
#62497=ORIENTED_EDGE('',*,*,#47313,.T.);
#62498=ORIENTED_EDGE('',*,*,#47321,.F.);
#62499=ORIENTED_EDGE('',*,*,#47318,.F.);
#62500=ORIENTED_EDGE('',*,*,#47322,.T.);
#62501=ORIENTED_EDGE('',*,*,#47323,.T.);
#62502=ORIENTED_EDGE('',*,*,#47324,.F.);
#62503=ORIENTED_EDGE('',*,*,#47325,.F.);
#62504=ORIENTED_EDGE('',*,*,#47326,.T.);
#62505=ORIENTED_EDGE('',*,*,#47327,.T.);
#62506=ORIENTED_EDGE('',*,*,#47328,.F.);
#62507=ORIENTED_EDGE('',*,*,#47323,.F.);
#62508=ORIENTED_EDGE('',*,*,#47329,.T.);
#62509=ORIENTED_EDGE('',*,*,#47330,.T.);
#62510=ORIENTED_EDGE('',*,*,#47331,.F.);
#62511=ORIENTED_EDGE('',*,*,#47327,.F.);
#62512=ORIENTED_EDGE('',*,*,#47332,.T.);
#62513=ORIENTED_EDGE('',*,*,#47325,.T.);
#62514=ORIENTED_EDGE('',*,*,#47333,.F.);
#62515=ORIENTED_EDGE('',*,*,#47330,.F.);
#62516=ORIENTED_EDGE('',*,*,#47334,.T.);
#62517=ORIENTED_EDGE('',*,*,#47335,.T.);
#62518=ORIENTED_EDGE('',*,*,#47336,.F.);
#62519=ORIENTED_EDGE('',*,*,#47337,.F.);
#62520=ORIENTED_EDGE('',*,*,#47338,.T.);
#62521=ORIENTED_EDGE('',*,*,#47339,.T.);
#62522=ORIENTED_EDGE('',*,*,#47340,.F.);
#62523=ORIENTED_EDGE('',*,*,#47335,.F.);
#62524=ORIENTED_EDGE('',*,*,#47341,.T.);
#62525=ORIENTED_EDGE('',*,*,#47342,.T.);
#62526=ORIENTED_EDGE('',*,*,#47343,.F.);
#62527=ORIENTED_EDGE('',*,*,#47339,.F.);
#62528=ORIENTED_EDGE('',*,*,#47344,.T.);
#62529=ORIENTED_EDGE('',*,*,#47337,.T.);
#62530=ORIENTED_EDGE('',*,*,#47345,.F.);
#62531=ORIENTED_EDGE('',*,*,#47342,.F.);
#62532=ORIENTED_EDGE('',*,*,#47346,.T.);
#62533=ORIENTED_EDGE('',*,*,#47347,.T.);
#62534=ORIENTED_EDGE('',*,*,#47348,.F.);
#62535=ORIENTED_EDGE('',*,*,#47349,.F.);
#62536=ORIENTED_EDGE('',*,*,#47350,.T.);
#62537=ORIENTED_EDGE('',*,*,#47351,.T.);
#62538=ORIENTED_EDGE('',*,*,#47352,.F.);
#62539=ORIENTED_EDGE('',*,*,#47347,.F.);
#62540=ORIENTED_EDGE('',*,*,#47353,.T.);
#62541=ORIENTED_EDGE('',*,*,#47354,.T.);
#62542=ORIENTED_EDGE('',*,*,#47355,.F.);
#62543=ORIENTED_EDGE('',*,*,#47351,.F.);
#62544=ORIENTED_EDGE('',*,*,#47356,.T.);
#62545=ORIENTED_EDGE('',*,*,#47349,.T.);
#62546=ORIENTED_EDGE('',*,*,#47357,.F.);
#62547=ORIENTED_EDGE('',*,*,#47354,.F.);
#62548=ORIENTED_EDGE('',*,*,#47358,.T.);
#62549=ORIENTED_EDGE('',*,*,#47359,.T.);
#62550=ORIENTED_EDGE('',*,*,#47360,.F.);
#62551=ORIENTED_EDGE('',*,*,#47361,.F.);
#62552=ORIENTED_EDGE('',*,*,#47362,.T.);
#62553=ORIENTED_EDGE('',*,*,#47363,.T.);
#62554=ORIENTED_EDGE('',*,*,#47364,.F.);
#62555=ORIENTED_EDGE('',*,*,#47359,.F.);
#62556=ORIENTED_EDGE('',*,*,#47365,.T.);
#62557=ORIENTED_EDGE('',*,*,#47366,.T.);
#62558=ORIENTED_EDGE('',*,*,#47367,.F.);
#62559=ORIENTED_EDGE('',*,*,#47363,.F.);
#62560=ORIENTED_EDGE('',*,*,#47368,.T.);
#62561=ORIENTED_EDGE('',*,*,#47361,.T.);
#62562=ORIENTED_EDGE('',*,*,#47369,.F.);
#62563=ORIENTED_EDGE('',*,*,#47366,.F.);
#62564=ORIENTED_EDGE('',*,*,#47370,.T.);
#62565=ORIENTED_EDGE('',*,*,#47371,.T.);
#62566=ORIENTED_EDGE('',*,*,#47372,.F.);
#62567=ORIENTED_EDGE('',*,*,#47373,.F.);
#62568=ORIENTED_EDGE('',*,*,#47374,.T.);
#62569=ORIENTED_EDGE('',*,*,#47375,.T.);
#62570=ORIENTED_EDGE('',*,*,#47376,.F.);
#62571=ORIENTED_EDGE('',*,*,#47371,.F.);
#62572=ORIENTED_EDGE('',*,*,#47377,.T.);
#62573=ORIENTED_EDGE('',*,*,#47378,.T.);
#62574=ORIENTED_EDGE('',*,*,#47379,.F.);
#62575=ORIENTED_EDGE('',*,*,#47375,.F.);
#62576=ORIENTED_EDGE('',*,*,#47380,.T.);
#62577=ORIENTED_EDGE('',*,*,#47373,.T.);
#62578=ORIENTED_EDGE('',*,*,#47381,.F.);
#62579=ORIENTED_EDGE('',*,*,#47378,.F.);
#62580=ORIENTED_EDGE('',*,*,#47382,.T.);
#62581=ORIENTED_EDGE('',*,*,#47383,.T.);
#62582=ORIENTED_EDGE('',*,*,#47384,.F.);
#62583=ORIENTED_EDGE('',*,*,#47385,.F.);
#62584=ORIENTED_EDGE('',*,*,#47386,.T.);
#62585=ORIENTED_EDGE('',*,*,#47387,.T.);
#62586=ORIENTED_EDGE('',*,*,#47388,.F.);
#62587=ORIENTED_EDGE('',*,*,#47383,.F.);
#62588=ORIENTED_EDGE('',*,*,#47389,.T.);
#62589=ORIENTED_EDGE('',*,*,#47390,.T.);
#62590=ORIENTED_EDGE('',*,*,#47391,.F.);
#62591=ORIENTED_EDGE('',*,*,#47387,.F.);
#62592=ORIENTED_EDGE('',*,*,#47392,.T.);
#62593=ORIENTED_EDGE('',*,*,#47385,.T.);
#62594=ORIENTED_EDGE('',*,*,#47393,.F.);
#62595=ORIENTED_EDGE('',*,*,#47390,.F.);
#62596=ORIENTED_EDGE('',*,*,#47394,.T.);
#62597=ORIENTED_EDGE('',*,*,#47395,.T.);
#62598=ORIENTED_EDGE('',*,*,#47396,.F.);
#62599=ORIENTED_EDGE('',*,*,#47397,.F.);
#62600=ORIENTED_EDGE('',*,*,#47398,.T.);
#62601=ORIENTED_EDGE('',*,*,#47399,.T.);
#62602=ORIENTED_EDGE('',*,*,#47400,.F.);
#62603=ORIENTED_EDGE('',*,*,#47395,.F.);
#62604=ORIENTED_EDGE('',*,*,#47401,.T.);
#62605=ORIENTED_EDGE('',*,*,#47402,.T.);
#62606=ORIENTED_EDGE('',*,*,#47403,.F.);
#62607=ORIENTED_EDGE('',*,*,#47399,.F.);
#62608=ORIENTED_EDGE('',*,*,#47404,.T.);
#62609=ORIENTED_EDGE('',*,*,#47397,.T.);
#62610=ORIENTED_EDGE('',*,*,#47405,.F.);
#62611=ORIENTED_EDGE('',*,*,#47402,.F.);
#62612=ORIENTED_EDGE('',*,*,#47406,.T.);
#62613=ORIENTED_EDGE('',*,*,#47407,.T.);
#62614=ORIENTED_EDGE('',*,*,#47408,.F.);
#62615=ORIENTED_EDGE('',*,*,#47409,.F.);
#62616=ORIENTED_EDGE('',*,*,#47410,.T.);
#62617=ORIENTED_EDGE('',*,*,#47411,.T.);
#62618=ORIENTED_EDGE('',*,*,#47412,.F.);
#62619=ORIENTED_EDGE('',*,*,#47407,.F.);
#62620=ORIENTED_EDGE('',*,*,#47413,.T.);
#62621=ORIENTED_EDGE('',*,*,#47414,.T.);
#62622=ORIENTED_EDGE('',*,*,#47415,.F.);
#62623=ORIENTED_EDGE('',*,*,#47411,.F.);
#62624=ORIENTED_EDGE('',*,*,#47416,.T.);
#62625=ORIENTED_EDGE('',*,*,#47409,.T.);
#62626=ORIENTED_EDGE('',*,*,#47417,.F.);
#62627=ORIENTED_EDGE('',*,*,#47414,.F.);
#62628=ORIENTED_EDGE('',*,*,#47418,.T.);
#62629=ORIENTED_EDGE('',*,*,#47419,.T.);
#62630=ORIENTED_EDGE('',*,*,#47420,.F.);
#62631=ORIENTED_EDGE('',*,*,#47421,.F.);
#62632=ORIENTED_EDGE('',*,*,#47422,.T.);
#62633=ORIENTED_EDGE('',*,*,#47423,.T.);
#62634=ORIENTED_EDGE('',*,*,#47424,.F.);
#62635=ORIENTED_EDGE('',*,*,#47419,.F.);
#62636=ORIENTED_EDGE('',*,*,#47425,.T.);
#62637=ORIENTED_EDGE('',*,*,#47426,.T.);
#62638=ORIENTED_EDGE('',*,*,#47427,.F.);
#62639=ORIENTED_EDGE('',*,*,#47423,.F.);
#62640=ORIENTED_EDGE('',*,*,#47428,.T.);
#62641=ORIENTED_EDGE('',*,*,#47421,.T.);
#62642=ORIENTED_EDGE('',*,*,#47429,.F.);
#62643=ORIENTED_EDGE('',*,*,#47426,.F.);
#62644=ORIENTED_EDGE('',*,*,#47430,.T.);
#62645=ORIENTED_EDGE('',*,*,#47431,.T.);
#62646=ORIENTED_EDGE('',*,*,#47432,.F.);
#62647=ORIENTED_EDGE('',*,*,#47433,.F.);
#62648=ORIENTED_EDGE('',*,*,#47434,.T.);
#62649=ORIENTED_EDGE('',*,*,#47435,.T.);
#62650=ORIENTED_EDGE('',*,*,#47436,.F.);
#62651=ORIENTED_EDGE('',*,*,#47431,.F.);
#62652=ORIENTED_EDGE('',*,*,#47437,.T.);
#62653=ORIENTED_EDGE('',*,*,#47438,.T.);
#62654=ORIENTED_EDGE('',*,*,#47439,.F.);
#62655=ORIENTED_EDGE('',*,*,#47435,.F.);
#62656=ORIENTED_EDGE('',*,*,#47440,.T.);
#62657=ORIENTED_EDGE('',*,*,#47433,.T.);
#62658=ORIENTED_EDGE('',*,*,#47441,.F.);
#62659=ORIENTED_EDGE('',*,*,#47438,.F.);
#62660=ORIENTED_EDGE('',*,*,#47442,.T.);
#62661=ORIENTED_EDGE('',*,*,#47443,.T.);
#62662=ORIENTED_EDGE('',*,*,#47444,.F.);
#62663=ORIENTED_EDGE('',*,*,#47445,.F.);
#62664=ORIENTED_EDGE('',*,*,#47446,.T.);
#62665=ORIENTED_EDGE('',*,*,#47447,.T.);
#62666=ORIENTED_EDGE('',*,*,#47448,.F.);
#62667=ORIENTED_EDGE('',*,*,#47443,.F.);
#62668=ORIENTED_EDGE('',*,*,#47449,.T.);
#62669=ORIENTED_EDGE('',*,*,#47450,.T.);
#62670=ORIENTED_EDGE('',*,*,#47451,.F.);
#62671=ORIENTED_EDGE('',*,*,#47447,.F.);
#62672=ORIENTED_EDGE('',*,*,#47452,.T.);
#62673=ORIENTED_EDGE('',*,*,#47445,.T.);
#62674=ORIENTED_EDGE('',*,*,#47453,.F.);
#62675=ORIENTED_EDGE('',*,*,#47450,.F.);
#62676=ORIENTED_EDGE('',*,*,#47454,.T.);
#62677=ORIENTED_EDGE('',*,*,#47455,.T.);
#62678=ORIENTED_EDGE('',*,*,#47456,.F.);
#62679=ORIENTED_EDGE('',*,*,#47457,.F.);
#62680=ORIENTED_EDGE('',*,*,#47458,.T.);
#62681=ORIENTED_EDGE('',*,*,#47459,.T.);
#62682=ORIENTED_EDGE('',*,*,#47460,.F.);
#62683=ORIENTED_EDGE('',*,*,#47455,.F.);
#62684=ORIENTED_EDGE('',*,*,#47461,.T.);
#62685=ORIENTED_EDGE('',*,*,#47462,.T.);
#62686=ORIENTED_EDGE('',*,*,#47463,.F.);
#62687=ORIENTED_EDGE('',*,*,#47459,.F.);
#62688=ORIENTED_EDGE('',*,*,#47464,.T.);
#62689=ORIENTED_EDGE('',*,*,#47457,.T.);
#62690=ORIENTED_EDGE('',*,*,#47465,.F.);
#62691=ORIENTED_EDGE('',*,*,#47462,.F.);
#62692=ORIENTED_EDGE('',*,*,#47466,.T.);
#62693=ORIENTED_EDGE('',*,*,#47467,.T.);
#62694=ORIENTED_EDGE('',*,*,#47468,.F.);
#62695=ORIENTED_EDGE('',*,*,#47469,.F.);
#62696=ORIENTED_EDGE('',*,*,#47470,.T.);
#62697=ORIENTED_EDGE('',*,*,#47471,.T.);
#62698=ORIENTED_EDGE('',*,*,#47472,.F.);
#62699=ORIENTED_EDGE('',*,*,#47467,.F.);
#62700=ORIENTED_EDGE('',*,*,#47473,.T.);
#62701=ORIENTED_EDGE('',*,*,#47474,.T.);
#62702=ORIENTED_EDGE('',*,*,#47475,.F.);
#62703=ORIENTED_EDGE('',*,*,#47471,.F.);
#62704=ORIENTED_EDGE('',*,*,#47476,.T.);
#62705=ORIENTED_EDGE('',*,*,#47469,.T.);
#62706=ORIENTED_EDGE('',*,*,#47477,.F.);
#62707=ORIENTED_EDGE('',*,*,#47474,.F.);
#62708=ORIENTED_EDGE('',*,*,#47478,.T.);
#62709=ORIENTED_EDGE('',*,*,#47479,.T.);
#62710=ORIENTED_EDGE('',*,*,#47480,.F.);
#62711=ORIENTED_EDGE('',*,*,#47481,.F.);
#62712=ORIENTED_EDGE('',*,*,#47482,.T.);
#62713=ORIENTED_EDGE('',*,*,#47483,.T.);
#62714=ORIENTED_EDGE('',*,*,#47484,.F.);
#62715=ORIENTED_EDGE('',*,*,#47479,.F.);
#62716=ORIENTED_EDGE('',*,*,#47485,.T.);
#62717=ORIENTED_EDGE('',*,*,#47486,.T.);
#62718=ORIENTED_EDGE('',*,*,#47487,.F.);
#62719=ORIENTED_EDGE('',*,*,#47483,.F.);
#62720=ORIENTED_EDGE('',*,*,#47488,.T.);
#62721=ORIENTED_EDGE('',*,*,#47481,.T.);
#62722=ORIENTED_EDGE('',*,*,#47489,.F.);
#62723=ORIENTED_EDGE('',*,*,#47486,.F.);
#62724=ORIENTED_EDGE('',*,*,#47490,.T.);
#62725=ORIENTED_EDGE('',*,*,#47491,.T.);
#62726=ORIENTED_EDGE('',*,*,#47492,.F.);
#62727=ORIENTED_EDGE('',*,*,#47493,.F.);
#62728=ORIENTED_EDGE('',*,*,#47494,.T.);
#62729=ORIENTED_EDGE('',*,*,#47495,.T.);
#62730=ORIENTED_EDGE('',*,*,#47496,.F.);
#62731=ORIENTED_EDGE('',*,*,#47491,.F.);
#62732=ORIENTED_EDGE('',*,*,#47497,.T.);
#62733=ORIENTED_EDGE('',*,*,#47498,.T.);
#62734=ORIENTED_EDGE('',*,*,#47499,.F.);
#62735=ORIENTED_EDGE('',*,*,#47495,.F.);
#62736=ORIENTED_EDGE('',*,*,#47500,.T.);
#62737=ORIENTED_EDGE('',*,*,#47493,.T.);
#62738=ORIENTED_EDGE('',*,*,#47501,.F.);
#62739=ORIENTED_EDGE('',*,*,#47498,.F.);
#62740=ORIENTED_EDGE('',*,*,#47502,.T.);
#62741=ORIENTED_EDGE('',*,*,#47503,.T.);
#62742=ORIENTED_EDGE('',*,*,#47504,.F.);
#62743=ORIENTED_EDGE('',*,*,#47505,.F.);
#62744=ORIENTED_EDGE('',*,*,#47506,.T.);
#62745=ORIENTED_EDGE('',*,*,#47507,.T.);
#62746=ORIENTED_EDGE('',*,*,#47508,.F.);
#62747=ORIENTED_EDGE('',*,*,#47503,.F.);
#62748=ORIENTED_EDGE('',*,*,#47509,.T.);
#62749=ORIENTED_EDGE('',*,*,#47510,.T.);
#62750=ORIENTED_EDGE('',*,*,#47511,.F.);
#62751=ORIENTED_EDGE('',*,*,#47507,.F.);
#62752=ORIENTED_EDGE('',*,*,#47512,.T.);
#62753=ORIENTED_EDGE('',*,*,#47505,.T.);
#62754=ORIENTED_EDGE('',*,*,#47513,.F.);
#62755=ORIENTED_EDGE('',*,*,#47510,.F.);
#62756=ORIENTED_EDGE('',*,*,#47514,.T.);
#62757=ORIENTED_EDGE('',*,*,#47515,.T.);
#62758=ORIENTED_EDGE('',*,*,#47516,.F.);
#62759=ORIENTED_EDGE('',*,*,#47517,.F.);
#62760=ORIENTED_EDGE('',*,*,#47518,.T.);
#62761=ORIENTED_EDGE('',*,*,#47519,.T.);
#62762=ORIENTED_EDGE('',*,*,#47520,.F.);
#62763=ORIENTED_EDGE('',*,*,#47515,.F.);
#62764=ORIENTED_EDGE('',*,*,#47521,.T.);
#62765=ORIENTED_EDGE('',*,*,#47522,.T.);
#62766=ORIENTED_EDGE('',*,*,#47523,.F.);
#62767=ORIENTED_EDGE('',*,*,#47519,.F.);
#62768=ORIENTED_EDGE('',*,*,#47524,.T.);
#62769=ORIENTED_EDGE('',*,*,#47517,.T.);
#62770=ORIENTED_EDGE('',*,*,#47525,.F.);
#62771=ORIENTED_EDGE('',*,*,#47522,.F.);
#62772=ORIENTED_EDGE('',*,*,#47526,.T.);
#62773=ORIENTED_EDGE('',*,*,#47527,.T.);
#62774=ORIENTED_EDGE('',*,*,#47528,.F.);
#62775=ORIENTED_EDGE('',*,*,#47529,.F.);
#62776=ORIENTED_EDGE('',*,*,#47530,.T.);
#62777=ORIENTED_EDGE('',*,*,#47531,.T.);
#62778=ORIENTED_EDGE('',*,*,#47532,.F.);
#62779=ORIENTED_EDGE('',*,*,#47527,.F.);
#62780=ORIENTED_EDGE('',*,*,#47533,.T.);
#62781=ORIENTED_EDGE('',*,*,#47534,.T.);
#62782=ORIENTED_EDGE('',*,*,#47535,.F.);
#62783=ORIENTED_EDGE('',*,*,#47531,.F.);
#62784=ORIENTED_EDGE('',*,*,#47536,.T.);
#62785=ORIENTED_EDGE('',*,*,#47529,.T.);
#62786=ORIENTED_EDGE('',*,*,#47537,.F.);
#62787=ORIENTED_EDGE('',*,*,#47534,.F.);
#62788=ORIENTED_EDGE('',*,*,#47538,.T.);
#62789=ORIENTED_EDGE('',*,*,#47539,.T.);
#62790=ORIENTED_EDGE('',*,*,#47540,.F.);
#62791=ORIENTED_EDGE('',*,*,#47541,.F.);
#62792=ORIENTED_EDGE('',*,*,#47542,.T.);
#62793=ORIENTED_EDGE('',*,*,#47543,.T.);
#62794=ORIENTED_EDGE('',*,*,#47544,.F.);
#62795=ORIENTED_EDGE('',*,*,#47539,.F.);
#62796=ORIENTED_EDGE('',*,*,#47545,.T.);
#62797=ORIENTED_EDGE('',*,*,#47546,.T.);
#62798=ORIENTED_EDGE('',*,*,#47547,.F.);
#62799=ORIENTED_EDGE('',*,*,#47543,.F.);
#62800=ORIENTED_EDGE('',*,*,#47548,.T.);
#62801=ORIENTED_EDGE('',*,*,#47541,.T.);
#62802=ORIENTED_EDGE('',*,*,#47549,.F.);
#62803=ORIENTED_EDGE('',*,*,#47546,.F.);
#62804=ORIENTED_EDGE('',*,*,#47550,.T.);
#62805=ORIENTED_EDGE('',*,*,#47551,.T.);
#62806=ORIENTED_EDGE('',*,*,#47552,.F.);
#62807=ORIENTED_EDGE('',*,*,#47553,.F.);
#62808=ORIENTED_EDGE('',*,*,#47554,.T.);
#62809=ORIENTED_EDGE('',*,*,#47555,.T.);
#62810=ORIENTED_EDGE('',*,*,#47556,.F.);
#62811=ORIENTED_EDGE('',*,*,#47551,.F.);
#62812=ORIENTED_EDGE('',*,*,#47557,.T.);
#62813=ORIENTED_EDGE('',*,*,#47558,.T.);
#62814=ORIENTED_EDGE('',*,*,#47559,.F.);
#62815=ORIENTED_EDGE('',*,*,#47555,.F.);
#62816=ORIENTED_EDGE('',*,*,#47560,.T.);
#62817=ORIENTED_EDGE('',*,*,#47553,.T.);
#62818=ORIENTED_EDGE('',*,*,#47561,.F.);
#62819=ORIENTED_EDGE('',*,*,#47558,.F.);
#62820=ORIENTED_EDGE('',*,*,#47562,.T.);
#62821=ORIENTED_EDGE('',*,*,#47563,.T.);
#62822=ORIENTED_EDGE('',*,*,#47564,.F.);
#62823=ORIENTED_EDGE('',*,*,#47565,.F.);
#62824=ORIENTED_EDGE('',*,*,#47566,.T.);
#62825=ORIENTED_EDGE('',*,*,#47567,.T.);
#62826=ORIENTED_EDGE('',*,*,#47568,.F.);
#62827=ORIENTED_EDGE('',*,*,#47563,.F.);
#62828=ORIENTED_EDGE('',*,*,#47569,.T.);
#62829=ORIENTED_EDGE('',*,*,#47570,.T.);
#62830=ORIENTED_EDGE('',*,*,#47571,.F.);
#62831=ORIENTED_EDGE('',*,*,#47567,.F.);
#62832=ORIENTED_EDGE('',*,*,#47572,.T.);
#62833=ORIENTED_EDGE('',*,*,#47565,.T.);
#62834=ORIENTED_EDGE('',*,*,#47573,.F.);
#62835=ORIENTED_EDGE('',*,*,#47570,.F.);
#62836=ORIENTED_EDGE('',*,*,#47574,.T.);
#62837=ORIENTED_EDGE('',*,*,#47575,.T.);
#62838=ORIENTED_EDGE('',*,*,#47576,.F.);
#62839=ORIENTED_EDGE('',*,*,#47577,.F.);
#62840=ORIENTED_EDGE('',*,*,#47578,.T.);
#62841=ORIENTED_EDGE('',*,*,#47579,.T.);
#62842=ORIENTED_EDGE('',*,*,#47580,.F.);
#62843=ORIENTED_EDGE('',*,*,#47575,.F.);
#62844=ORIENTED_EDGE('',*,*,#47581,.T.);
#62845=ORIENTED_EDGE('',*,*,#47582,.T.);
#62846=ORIENTED_EDGE('',*,*,#47583,.F.);
#62847=ORIENTED_EDGE('',*,*,#47579,.F.);
#62848=ORIENTED_EDGE('',*,*,#47584,.T.);
#62849=ORIENTED_EDGE('',*,*,#47577,.T.);
#62850=ORIENTED_EDGE('',*,*,#47585,.F.);
#62851=ORIENTED_EDGE('',*,*,#47582,.F.);
#62852=ORIENTED_EDGE('',*,*,#47586,.T.);
#62853=ORIENTED_EDGE('',*,*,#47587,.T.);
#62854=ORIENTED_EDGE('',*,*,#47588,.F.);
#62855=ORIENTED_EDGE('',*,*,#47589,.F.);
#62856=ORIENTED_EDGE('',*,*,#47590,.T.);
#62857=ORIENTED_EDGE('',*,*,#47591,.T.);
#62858=ORIENTED_EDGE('',*,*,#47592,.F.);
#62859=ORIENTED_EDGE('',*,*,#47587,.F.);
#62860=ORIENTED_EDGE('',*,*,#47593,.T.);
#62861=ORIENTED_EDGE('',*,*,#47594,.T.);
#62862=ORIENTED_EDGE('',*,*,#47595,.F.);
#62863=ORIENTED_EDGE('',*,*,#47591,.F.);
#62864=ORIENTED_EDGE('',*,*,#47596,.T.);
#62865=ORIENTED_EDGE('',*,*,#47589,.T.);
#62866=ORIENTED_EDGE('',*,*,#47597,.F.);
#62867=ORIENTED_EDGE('',*,*,#47594,.F.);
#62868=ORIENTED_EDGE('',*,*,#47598,.T.);
#62869=ORIENTED_EDGE('',*,*,#47599,.T.);
#62870=ORIENTED_EDGE('',*,*,#47600,.F.);
#62871=ORIENTED_EDGE('',*,*,#47601,.F.);
#62872=ORIENTED_EDGE('',*,*,#47602,.T.);
#62873=ORIENTED_EDGE('',*,*,#47603,.T.);
#62874=ORIENTED_EDGE('',*,*,#47604,.F.);
#62875=ORIENTED_EDGE('',*,*,#47599,.F.);
#62876=ORIENTED_EDGE('',*,*,#47605,.T.);
#62877=ORIENTED_EDGE('',*,*,#47606,.T.);
#62878=ORIENTED_EDGE('',*,*,#47607,.F.);
#62879=ORIENTED_EDGE('',*,*,#47603,.F.);
#62880=ORIENTED_EDGE('',*,*,#47608,.T.);
#62881=ORIENTED_EDGE('',*,*,#47601,.T.);
#62882=ORIENTED_EDGE('',*,*,#47609,.F.);
#62883=ORIENTED_EDGE('',*,*,#47606,.F.);
#62884=ORIENTED_EDGE('',*,*,#47610,.T.);
#62885=ORIENTED_EDGE('',*,*,#47611,.T.);
#62886=ORIENTED_EDGE('',*,*,#47612,.F.);
#62887=ORIENTED_EDGE('',*,*,#47613,.F.);
#62888=ORIENTED_EDGE('',*,*,#47614,.T.);
#62889=ORIENTED_EDGE('',*,*,#47615,.T.);
#62890=ORIENTED_EDGE('',*,*,#47616,.F.);
#62891=ORIENTED_EDGE('',*,*,#47611,.F.);
#62892=ORIENTED_EDGE('',*,*,#47617,.T.);
#62893=ORIENTED_EDGE('',*,*,#47618,.T.);
#62894=ORIENTED_EDGE('',*,*,#47619,.F.);
#62895=ORIENTED_EDGE('',*,*,#47615,.F.);
#62896=ORIENTED_EDGE('',*,*,#47620,.T.);
#62897=ORIENTED_EDGE('',*,*,#47613,.T.);
#62898=ORIENTED_EDGE('',*,*,#47621,.F.);
#62899=ORIENTED_EDGE('',*,*,#47618,.F.);
#62900=ORIENTED_EDGE('',*,*,#47622,.T.);
#62901=ORIENTED_EDGE('',*,*,#47623,.T.);
#62902=ORIENTED_EDGE('',*,*,#47624,.F.);
#62903=ORIENTED_EDGE('',*,*,#47625,.F.);
#62904=ORIENTED_EDGE('',*,*,#47626,.T.);
#62905=ORIENTED_EDGE('',*,*,#47627,.T.);
#62906=ORIENTED_EDGE('',*,*,#47628,.F.);
#62907=ORIENTED_EDGE('',*,*,#47623,.F.);
#62908=ORIENTED_EDGE('',*,*,#47629,.T.);
#62909=ORIENTED_EDGE('',*,*,#47630,.T.);
#62910=ORIENTED_EDGE('',*,*,#47631,.F.);
#62911=ORIENTED_EDGE('',*,*,#47627,.F.);
#62912=ORIENTED_EDGE('',*,*,#47632,.T.);
#62913=ORIENTED_EDGE('',*,*,#47625,.T.);
#62914=ORIENTED_EDGE('',*,*,#47633,.F.);
#62915=ORIENTED_EDGE('',*,*,#47630,.F.);
#62916=ORIENTED_EDGE('',*,*,#47634,.T.);
#62917=ORIENTED_EDGE('',*,*,#47635,.T.);
#62918=ORIENTED_EDGE('',*,*,#47636,.F.);
#62919=ORIENTED_EDGE('',*,*,#47637,.F.);
#62920=ORIENTED_EDGE('',*,*,#47638,.T.);
#62921=ORIENTED_EDGE('',*,*,#47639,.T.);
#62922=ORIENTED_EDGE('',*,*,#47640,.F.);
#62923=ORIENTED_EDGE('',*,*,#47635,.F.);
#62924=ORIENTED_EDGE('',*,*,#47641,.T.);
#62925=ORIENTED_EDGE('',*,*,#47642,.T.);
#62926=ORIENTED_EDGE('',*,*,#47643,.F.);
#62927=ORIENTED_EDGE('',*,*,#47639,.F.);
#62928=ORIENTED_EDGE('',*,*,#47644,.T.);
#62929=ORIENTED_EDGE('',*,*,#47637,.T.);
#62930=ORIENTED_EDGE('',*,*,#47645,.F.);
#62931=ORIENTED_EDGE('',*,*,#47642,.F.);
#62932=ORIENTED_EDGE('',*,*,#47646,.T.);
#62933=ORIENTED_EDGE('',*,*,#47647,.T.);
#62934=ORIENTED_EDGE('',*,*,#47648,.F.);
#62935=ORIENTED_EDGE('',*,*,#47649,.F.);
#62936=ORIENTED_EDGE('',*,*,#47650,.T.);
#62937=ORIENTED_EDGE('',*,*,#47651,.T.);
#62938=ORIENTED_EDGE('',*,*,#47652,.F.);
#62939=ORIENTED_EDGE('',*,*,#47647,.F.);
#62940=ORIENTED_EDGE('',*,*,#47653,.T.);
#62941=ORIENTED_EDGE('',*,*,#47654,.T.);
#62942=ORIENTED_EDGE('',*,*,#47655,.F.);
#62943=ORIENTED_EDGE('',*,*,#47651,.F.);
#62944=ORIENTED_EDGE('',*,*,#47656,.T.);
#62945=ORIENTED_EDGE('',*,*,#47649,.T.);
#62946=ORIENTED_EDGE('',*,*,#47657,.F.);
#62947=ORIENTED_EDGE('',*,*,#47654,.F.);
#62948=ORIENTED_EDGE('',*,*,#47658,.T.);
#62949=ORIENTED_EDGE('',*,*,#47659,.T.);
#62950=ORIENTED_EDGE('',*,*,#47660,.F.);
#62951=ORIENTED_EDGE('',*,*,#47661,.F.);
#62952=ORIENTED_EDGE('',*,*,#47662,.T.);
#62953=ORIENTED_EDGE('',*,*,#47663,.T.);
#62954=ORIENTED_EDGE('',*,*,#47664,.F.);
#62955=ORIENTED_EDGE('',*,*,#47659,.F.);
#62956=ORIENTED_EDGE('',*,*,#47665,.T.);
#62957=ORIENTED_EDGE('',*,*,#47666,.T.);
#62958=ORIENTED_EDGE('',*,*,#47667,.F.);
#62959=ORIENTED_EDGE('',*,*,#47663,.F.);
#62960=ORIENTED_EDGE('',*,*,#47668,.T.);
#62961=ORIENTED_EDGE('',*,*,#47661,.T.);
#62962=ORIENTED_EDGE('',*,*,#47669,.F.);
#62963=ORIENTED_EDGE('',*,*,#47666,.F.);
#62964=ORIENTED_EDGE('',*,*,#47670,.T.);
#62965=ORIENTED_EDGE('',*,*,#47671,.T.);
#62966=ORIENTED_EDGE('',*,*,#47672,.F.);
#62967=ORIENTED_EDGE('',*,*,#47673,.F.);
#62968=ORIENTED_EDGE('',*,*,#47674,.T.);
#62969=ORIENTED_EDGE('',*,*,#47675,.T.);
#62970=ORIENTED_EDGE('',*,*,#47676,.F.);
#62971=ORIENTED_EDGE('',*,*,#47671,.F.);
#62972=ORIENTED_EDGE('',*,*,#47677,.T.);
#62973=ORIENTED_EDGE('',*,*,#47678,.T.);
#62974=ORIENTED_EDGE('',*,*,#47679,.F.);
#62975=ORIENTED_EDGE('',*,*,#47675,.F.);
#62976=ORIENTED_EDGE('',*,*,#47680,.T.);
#62977=ORIENTED_EDGE('',*,*,#47673,.T.);
#62978=ORIENTED_EDGE('',*,*,#47681,.F.);
#62979=ORIENTED_EDGE('',*,*,#47678,.F.);
#62980=ORIENTED_EDGE('',*,*,#47682,.T.);
#62981=ORIENTED_EDGE('',*,*,#47683,.T.);
#62982=ORIENTED_EDGE('',*,*,#47684,.F.);
#62983=ORIENTED_EDGE('',*,*,#47685,.F.);
#62984=ORIENTED_EDGE('',*,*,#47686,.T.);
#62985=ORIENTED_EDGE('',*,*,#47687,.T.);
#62986=ORIENTED_EDGE('',*,*,#47688,.F.);
#62987=ORIENTED_EDGE('',*,*,#47683,.F.);
#62988=ORIENTED_EDGE('',*,*,#47689,.T.);
#62989=ORIENTED_EDGE('',*,*,#47690,.T.);
#62990=ORIENTED_EDGE('',*,*,#47691,.F.);
#62991=ORIENTED_EDGE('',*,*,#47687,.F.);
#62992=ORIENTED_EDGE('',*,*,#47692,.T.);
#62993=ORIENTED_EDGE('',*,*,#47685,.T.);
#62994=ORIENTED_EDGE('',*,*,#47693,.F.);
#62995=ORIENTED_EDGE('',*,*,#47690,.F.);
#62996=ORIENTED_EDGE('',*,*,#47694,.T.);
#62997=ORIENTED_EDGE('',*,*,#47695,.T.);
#62998=ORIENTED_EDGE('',*,*,#47696,.F.);
#62999=ORIENTED_EDGE('',*,*,#47697,.F.);
#63000=ORIENTED_EDGE('',*,*,#47698,.T.);
#63001=ORIENTED_EDGE('',*,*,#47699,.T.);
#63002=ORIENTED_EDGE('',*,*,#47700,.F.);
#63003=ORIENTED_EDGE('',*,*,#47695,.F.);
#63004=ORIENTED_EDGE('',*,*,#47701,.T.);
#63005=ORIENTED_EDGE('',*,*,#47702,.T.);
#63006=ORIENTED_EDGE('',*,*,#47703,.F.);
#63007=ORIENTED_EDGE('',*,*,#47699,.F.);
#63008=ORIENTED_EDGE('',*,*,#47704,.T.);
#63009=ORIENTED_EDGE('',*,*,#47697,.T.);
#63010=ORIENTED_EDGE('',*,*,#47705,.F.);
#63011=ORIENTED_EDGE('',*,*,#47702,.F.);
#63012=ORIENTED_EDGE('',*,*,#47706,.T.);
#63013=ORIENTED_EDGE('',*,*,#47707,.T.);
#63014=ORIENTED_EDGE('',*,*,#47708,.F.);
#63015=ORIENTED_EDGE('',*,*,#47709,.F.);
#63016=ORIENTED_EDGE('',*,*,#47710,.T.);
#63017=ORIENTED_EDGE('',*,*,#47711,.T.);
#63018=ORIENTED_EDGE('',*,*,#47712,.F.);
#63019=ORIENTED_EDGE('',*,*,#47707,.F.);
#63020=ORIENTED_EDGE('',*,*,#47713,.T.);
#63021=ORIENTED_EDGE('',*,*,#47714,.T.);
#63022=ORIENTED_EDGE('',*,*,#47715,.F.);
#63023=ORIENTED_EDGE('',*,*,#47711,.F.);
#63024=ORIENTED_EDGE('',*,*,#47716,.T.);
#63025=ORIENTED_EDGE('',*,*,#47709,.T.);
#63026=ORIENTED_EDGE('',*,*,#47717,.F.);
#63027=ORIENTED_EDGE('',*,*,#47714,.F.);
#63028=ORIENTED_EDGE('',*,*,#47718,.T.);
#63029=ORIENTED_EDGE('',*,*,#47719,.T.);
#63030=ORIENTED_EDGE('',*,*,#47720,.F.);
#63031=ORIENTED_EDGE('',*,*,#47721,.F.);
#63032=ORIENTED_EDGE('',*,*,#47722,.T.);
#63033=ORIENTED_EDGE('',*,*,#47723,.T.);
#63034=ORIENTED_EDGE('',*,*,#47724,.F.);
#63035=ORIENTED_EDGE('',*,*,#47719,.F.);
#63036=ORIENTED_EDGE('',*,*,#47725,.T.);
#63037=ORIENTED_EDGE('',*,*,#47726,.T.);
#63038=ORIENTED_EDGE('',*,*,#47727,.F.);
#63039=ORIENTED_EDGE('',*,*,#47723,.F.);
#63040=ORIENTED_EDGE('',*,*,#47728,.T.);
#63041=ORIENTED_EDGE('',*,*,#47721,.T.);
#63042=ORIENTED_EDGE('',*,*,#47729,.F.);
#63043=ORIENTED_EDGE('',*,*,#47726,.F.);
#63044=ORIENTED_EDGE('',*,*,#47730,.T.);
#63045=ORIENTED_EDGE('',*,*,#47731,.T.);
#63046=ORIENTED_EDGE('',*,*,#47732,.F.);
#63047=ORIENTED_EDGE('',*,*,#47733,.F.);
#63048=ORIENTED_EDGE('',*,*,#47734,.T.);
#63049=ORIENTED_EDGE('',*,*,#47735,.T.);
#63050=ORIENTED_EDGE('',*,*,#47736,.F.);
#63051=ORIENTED_EDGE('',*,*,#47731,.F.);
#63052=ORIENTED_EDGE('',*,*,#47737,.T.);
#63053=ORIENTED_EDGE('',*,*,#47738,.T.);
#63054=ORIENTED_EDGE('',*,*,#47739,.F.);
#63055=ORIENTED_EDGE('',*,*,#47735,.F.);
#63056=ORIENTED_EDGE('',*,*,#47740,.T.);
#63057=ORIENTED_EDGE('',*,*,#47733,.T.);
#63058=ORIENTED_EDGE('',*,*,#47741,.F.);
#63059=ORIENTED_EDGE('',*,*,#47738,.F.);
#63060=ORIENTED_EDGE('',*,*,#47742,.T.);
#63061=ORIENTED_EDGE('',*,*,#47743,.T.);
#63062=ORIENTED_EDGE('',*,*,#47744,.F.);
#63063=ORIENTED_EDGE('',*,*,#47745,.F.);
#63064=ORIENTED_EDGE('',*,*,#47746,.T.);
#63065=ORIENTED_EDGE('',*,*,#47747,.T.);
#63066=ORIENTED_EDGE('',*,*,#47748,.F.);
#63067=ORIENTED_EDGE('',*,*,#47743,.F.);
#63068=ORIENTED_EDGE('',*,*,#47749,.T.);
#63069=ORIENTED_EDGE('',*,*,#47750,.T.);
#63070=ORIENTED_EDGE('',*,*,#47751,.F.);
#63071=ORIENTED_EDGE('',*,*,#47747,.F.);
#63072=ORIENTED_EDGE('',*,*,#47752,.T.);
#63073=ORIENTED_EDGE('',*,*,#47745,.T.);
#63074=ORIENTED_EDGE('',*,*,#47753,.F.);
#63075=ORIENTED_EDGE('',*,*,#47750,.F.);
#63076=ORIENTED_EDGE('',*,*,#47754,.T.);
#63077=ORIENTED_EDGE('',*,*,#47755,.T.);
#63078=ORIENTED_EDGE('',*,*,#47756,.F.);
#63079=ORIENTED_EDGE('',*,*,#47757,.F.);
#63080=ORIENTED_EDGE('',*,*,#47758,.T.);
#63081=ORIENTED_EDGE('',*,*,#47759,.T.);
#63082=ORIENTED_EDGE('',*,*,#47760,.F.);
#63083=ORIENTED_EDGE('',*,*,#47755,.F.);
#63084=ORIENTED_EDGE('',*,*,#47761,.T.);
#63085=ORIENTED_EDGE('',*,*,#47762,.T.);
#63086=ORIENTED_EDGE('',*,*,#47763,.F.);
#63087=ORIENTED_EDGE('',*,*,#47759,.F.);
#63088=ORIENTED_EDGE('',*,*,#47764,.T.);
#63089=ORIENTED_EDGE('',*,*,#47757,.T.);
#63090=ORIENTED_EDGE('',*,*,#47765,.F.);
#63091=ORIENTED_EDGE('',*,*,#47762,.F.);
#63092=ORIENTED_EDGE('',*,*,#47766,.T.);
#63093=ORIENTED_EDGE('',*,*,#47767,.T.);
#63094=ORIENTED_EDGE('',*,*,#47768,.F.);
#63095=ORIENTED_EDGE('',*,*,#47769,.F.);
#63096=ORIENTED_EDGE('',*,*,#47770,.T.);
#63097=ORIENTED_EDGE('',*,*,#47771,.T.);
#63098=ORIENTED_EDGE('',*,*,#47772,.F.);
#63099=ORIENTED_EDGE('',*,*,#47767,.F.);
#63100=ORIENTED_EDGE('',*,*,#47773,.T.);
#63101=ORIENTED_EDGE('',*,*,#47774,.T.);
#63102=ORIENTED_EDGE('',*,*,#47775,.F.);
#63103=ORIENTED_EDGE('',*,*,#47771,.F.);
#63104=ORIENTED_EDGE('',*,*,#47776,.T.);
#63105=ORIENTED_EDGE('',*,*,#47769,.T.);
#63106=ORIENTED_EDGE('',*,*,#47777,.F.);
#63107=ORIENTED_EDGE('',*,*,#47774,.F.);
#63108=ORIENTED_EDGE('',*,*,#47778,.T.);
#63109=ORIENTED_EDGE('',*,*,#47779,.T.);
#63110=ORIENTED_EDGE('',*,*,#47780,.F.);
#63111=ORIENTED_EDGE('',*,*,#47781,.F.);
#63112=ORIENTED_EDGE('',*,*,#47782,.T.);
#63113=ORIENTED_EDGE('',*,*,#47783,.T.);
#63114=ORIENTED_EDGE('',*,*,#47784,.F.);
#63115=ORIENTED_EDGE('',*,*,#47779,.F.);
#63116=ORIENTED_EDGE('',*,*,#47785,.T.);
#63117=ORIENTED_EDGE('',*,*,#47786,.T.);
#63118=ORIENTED_EDGE('',*,*,#47787,.F.);
#63119=ORIENTED_EDGE('',*,*,#47783,.F.);
#63120=ORIENTED_EDGE('',*,*,#47788,.T.);
#63121=ORIENTED_EDGE('',*,*,#47781,.T.);
#63122=ORIENTED_EDGE('',*,*,#47789,.F.);
#63123=ORIENTED_EDGE('',*,*,#47786,.F.);
#63124=ORIENTED_EDGE('',*,*,#47790,.T.);
#63125=ORIENTED_EDGE('',*,*,#47791,.T.);
#63126=ORIENTED_EDGE('',*,*,#47792,.F.);
#63127=ORIENTED_EDGE('',*,*,#47793,.F.);
#63128=ORIENTED_EDGE('',*,*,#47794,.T.);
#63129=ORIENTED_EDGE('',*,*,#47795,.T.);
#63130=ORIENTED_EDGE('',*,*,#47796,.F.);
#63131=ORIENTED_EDGE('',*,*,#47791,.F.);
#63132=ORIENTED_EDGE('',*,*,#47797,.T.);
#63133=ORIENTED_EDGE('',*,*,#47798,.T.);
#63134=ORIENTED_EDGE('',*,*,#47799,.F.);
#63135=ORIENTED_EDGE('',*,*,#47795,.F.);
#63136=ORIENTED_EDGE('',*,*,#47800,.T.);
#63137=ORIENTED_EDGE('',*,*,#47793,.T.);
#63138=ORIENTED_EDGE('',*,*,#47801,.F.);
#63139=ORIENTED_EDGE('',*,*,#47798,.F.);
#63140=ORIENTED_EDGE('',*,*,#47802,.T.);
#63141=ORIENTED_EDGE('',*,*,#47803,.T.);
#63142=ORIENTED_EDGE('',*,*,#47804,.F.);
#63143=ORIENTED_EDGE('',*,*,#47805,.F.);
#63144=ORIENTED_EDGE('',*,*,#47806,.T.);
#63145=ORIENTED_EDGE('',*,*,#47807,.T.);
#63146=ORIENTED_EDGE('',*,*,#47808,.F.);
#63147=ORIENTED_EDGE('',*,*,#47803,.F.);
#63148=ORIENTED_EDGE('',*,*,#47809,.T.);
#63149=ORIENTED_EDGE('',*,*,#47810,.T.);
#63150=ORIENTED_EDGE('',*,*,#47811,.F.);
#63151=ORIENTED_EDGE('',*,*,#47807,.F.);
#63152=ORIENTED_EDGE('',*,*,#47812,.T.);
#63153=ORIENTED_EDGE('',*,*,#47805,.T.);
#63154=ORIENTED_EDGE('',*,*,#47813,.F.);
#63155=ORIENTED_EDGE('',*,*,#47810,.F.);
#63156=ORIENTED_EDGE('',*,*,#47814,.T.);
#63157=ORIENTED_EDGE('',*,*,#47815,.T.);
#63158=ORIENTED_EDGE('',*,*,#47816,.F.);
#63159=ORIENTED_EDGE('',*,*,#47817,.F.);
#63160=ORIENTED_EDGE('',*,*,#47818,.T.);
#63161=ORIENTED_EDGE('',*,*,#47819,.T.);
#63162=ORIENTED_EDGE('',*,*,#47820,.F.);
#63163=ORIENTED_EDGE('',*,*,#47815,.F.);
#63164=ORIENTED_EDGE('',*,*,#47821,.T.);
#63165=ORIENTED_EDGE('',*,*,#47822,.T.);
#63166=ORIENTED_EDGE('',*,*,#47823,.F.);
#63167=ORIENTED_EDGE('',*,*,#47819,.F.);
#63168=ORIENTED_EDGE('',*,*,#47824,.T.);
#63169=ORIENTED_EDGE('',*,*,#47817,.T.);
#63170=ORIENTED_EDGE('',*,*,#47825,.F.);
#63171=ORIENTED_EDGE('',*,*,#47822,.F.);
#63172=ORIENTED_EDGE('',*,*,#47826,.T.);
#63173=ORIENTED_EDGE('',*,*,#47827,.T.);
#63174=ORIENTED_EDGE('',*,*,#47828,.F.);
#63175=ORIENTED_EDGE('',*,*,#47829,.F.);
#63176=ORIENTED_EDGE('',*,*,#47830,.T.);
#63177=ORIENTED_EDGE('',*,*,#47831,.T.);
#63178=ORIENTED_EDGE('',*,*,#47832,.F.);
#63179=ORIENTED_EDGE('',*,*,#47827,.F.);
#63180=ORIENTED_EDGE('',*,*,#47833,.T.);
#63181=ORIENTED_EDGE('',*,*,#47834,.T.);
#63182=ORIENTED_EDGE('',*,*,#47835,.F.);
#63183=ORIENTED_EDGE('',*,*,#47831,.F.);
#63184=ORIENTED_EDGE('',*,*,#47836,.T.);
#63185=ORIENTED_EDGE('',*,*,#47829,.T.);
#63186=ORIENTED_EDGE('',*,*,#47837,.F.);
#63187=ORIENTED_EDGE('',*,*,#47834,.F.);
#63188=ORIENTED_EDGE('',*,*,#47838,.T.);
#63189=ORIENTED_EDGE('',*,*,#47839,.T.);
#63190=ORIENTED_EDGE('',*,*,#47840,.F.);
#63191=ORIENTED_EDGE('',*,*,#47841,.F.);
#63192=ORIENTED_EDGE('',*,*,#47842,.T.);
#63193=ORIENTED_EDGE('',*,*,#47843,.T.);
#63194=ORIENTED_EDGE('',*,*,#47844,.F.);
#63195=ORIENTED_EDGE('',*,*,#47839,.F.);
#63196=ORIENTED_EDGE('',*,*,#47845,.T.);
#63197=ORIENTED_EDGE('',*,*,#47846,.T.);
#63198=ORIENTED_EDGE('',*,*,#47847,.F.);
#63199=ORIENTED_EDGE('',*,*,#47843,.F.);
#63200=ORIENTED_EDGE('',*,*,#47848,.T.);
#63201=ORIENTED_EDGE('',*,*,#47841,.T.);
#63202=ORIENTED_EDGE('',*,*,#47849,.F.);
#63203=ORIENTED_EDGE('',*,*,#47846,.F.);
#63204=ORIENTED_EDGE('',*,*,#47850,.T.);
#63205=ORIENTED_EDGE('',*,*,#47851,.T.);
#63206=ORIENTED_EDGE('',*,*,#47852,.F.);
#63207=ORIENTED_EDGE('',*,*,#47853,.F.);
#63208=ORIENTED_EDGE('',*,*,#47854,.T.);
#63209=ORIENTED_EDGE('',*,*,#47855,.T.);
#63210=ORIENTED_EDGE('',*,*,#47856,.F.);
#63211=ORIENTED_EDGE('',*,*,#47851,.F.);
#63212=ORIENTED_EDGE('',*,*,#47857,.T.);
#63213=ORIENTED_EDGE('',*,*,#47858,.T.);
#63214=ORIENTED_EDGE('',*,*,#47859,.F.);
#63215=ORIENTED_EDGE('',*,*,#47855,.F.);
#63216=ORIENTED_EDGE('',*,*,#47860,.T.);
#63217=ORIENTED_EDGE('',*,*,#47853,.T.);
#63218=ORIENTED_EDGE('',*,*,#47861,.F.);
#63219=ORIENTED_EDGE('',*,*,#47858,.F.);
#63220=ORIENTED_EDGE('',*,*,#47862,.T.);
#63221=ORIENTED_EDGE('',*,*,#47863,.T.);
#63222=ORIENTED_EDGE('',*,*,#47864,.F.);
#63223=ORIENTED_EDGE('',*,*,#47865,.F.);
#63224=ORIENTED_EDGE('',*,*,#47866,.T.);
#63225=ORIENTED_EDGE('',*,*,#47867,.T.);
#63226=ORIENTED_EDGE('',*,*,#47868,.F.);
#63227=ORIENTED_EDGE('',*,*,#47863,.F.);
#63228=ORIENTED_EDGE('',*,*,#47869,.T.);
#63229=ORIENTED_EDGE('',*,*,#47870,.T.);
#63230=ORIENTED_EDGE('',*,*,#47871,.F.);
#63231=ORIENTED_EDGE('',*,*,#47867,.F.);
#63232=ORIENTED_EDGE('',*,*,#47872,.T.);
#63233=ORIENTED_EDGE('',*,*,#47865,.T.);
#63234=ORIENTED_EDGE('',*,*,#47873,.F.);
#63235=ORIENTED_EDGE('',*,*,#47870,.F.);
#63236=ORIENTED_EDGE('',*,*,#47874,.T.);
#63237=ORIENTED_EDGE('',*,*,#47875,.T.);
#63238=ORIENTED_EDGE('',*,*,#47876,.F.);
#63239=ORIENTED_EDGE('',*,*,#47877,.F.);
#63240=ORIENTED_EDGE('',*,*,#47878,.T.);
#63241=ORIENTED_EDGE('',*,*,#47879,.T.);
#63242=ORIENTED_EDGE('',*,*,#47880,.F.);
#63243=ORIENTED_EDGE('',*,*,#47875,.F.);
#63244=ORIENTED_EDGE('',*,*,#47881,.T.);
#63245=ORIENTED_EDGE('',*,*,#47882,.T.);
#63246=ORIENTED_EDGE('',*,*,#47883,.F.);
#63247=ORIENTED_EDGE('',*,*,#47879,.F.);
#63248=ORIENTED_EDGE('',*,*,#47884,.T.);
#63249=ORIENTED_EDGE('',*,*,#47877,.T.);
#63250=ORIENTED_EDGE('',*,*,#47885,.F.);
#63251=ORIENTED_EDGE('',*,*,#47882,.F.);
#63252=ORIENTED_EDGE('',*,*,#47886,.T.);
#63253=ORIENTED_EDGE('',*,*,#47887,.T.);
#63254=ORIENTED_EDGE('',*,*,#47888,.F.);
#63255=ORIENTED_EDGE('',*,*,#47889,.F.);
#63256=ORIENTED_EDGE('',*,*,#47890,.T.);
#63257=ORIENTED_EDGE('',*,*,#47891,.T.);
#63258=ORIENTED_EDGE('',*,*,#47892,.F.);
#63259=ORIENTED_EDGE('',*,*,#47887,.F.);
#63260=ORIENTED_EDGE('',*,*,#47893,.T.);
#63261=ORIENTED_EDGE('',*,*,#47894,.T.);
#63262=ORIENTED_EDGE('',*,*,#47895,.F.);
#63263=ORIENTED_EDGE('',*,*,#47891,.F.);
#63264=ORIENTED_EDGE('',*,*,#47896,.T.);
#63265=ORIENTED_EDGE('',*,*,#47889,.T.);
#63266=ORIENTED_EDGE('',*,*,#47897,.F.);
#63267=ORIENTED_EDGE('',*,*,#47894,.F.);
#63268=ORIENTED_EDGE('',*,*,#47898,.T.);
#63269=ORIENTED_EDGE('',*,*,#47899,.T.);
#63270=ORIENTED_EDGE('',*,*,#47900,.F.);
#63271=ORIENTED_EDGE('',*,*,#47901,.F.);
#63272=ORIENTED_EDGE('',*,*,#47902,.T.);
#63273=ORIENTED_EDGE('',*,*,#47903,.T.);
#63274=ORIENTED_EDGE('',*,*,#47904,.F.);
#63275=ORIENTED_EDGE('',*,*,#47899,.F.);
#63276=ORIENTED_EDGE('',*,*,#47905,.T.);
#63277=ORIENTED_EDGE('',*,*,#47906,.T.);
#63278=ORIENTED_EDGE('',*,*,#47907,.F.);
#63279=ORIENTED_EDGE('',*,*,#47903,.F.);
#63280=ORIENTED_EDGE('',*,*,#47908,.T.);
#63281=ORIENTED_EDGE('',*,*,#47901,.T.);
#63282=ORIENTED_EDGE('',*,*,#47909,.F.);
#63283=ORIENTED_EDGE('',*,*,#47906,.F.);
#63284=ORIENTED_EDGE('',*,*,#47910,.T.);
#63285=ORIENTED_EDGE('',*,*,#47911,.T.);
#63286=ORIENTED_EDGE('',*,*,#47912,.F.);
#63287=ORIENTED_EDGE('',*,*,#47913,.F.);
#63288=ORIENTED_EDGE('',*,*,#47914,.T.);
#63289=ORIENTED_EDGE('',*,*,#47915,.T.);
#63290=ORIENTED_EDGE('',*,*,#47916,.F.);
#63291=ORIENTED_EDGE('',*,*,#47911,.F.);
#63292=ORIENTED_EDGE('',*,*,#47917,.T.);
#63293=ORIENTED_EDGE('',*,*,#47918,.T.);
#63294=ORIENTED_EDGE('',*,*,#47919,.F.);
#63295=ORIENTED_EDGE('',*,*,#47915,.F.);
#63296=ORIENTED_EDGE('',*,*,#47920,.T.);
#63297=ORIENTED_EDGE('',*,*,#47913,.T.);
#63298=ORIENTED_EDGE('',*,*,#47921,.F.);
#63299=ORIENTED_EDGE('',*,*,#47918,.F.);
#63300=ORIENTED_EDGE('',*,*,#47922,.T.);
#63301=ORIENTED_EDGE('',*,*,#47923,.T.);
#63302=ORIENTED_EDGE('',*,*,#47924,.F.);
#63303=ORIENTED_EDGE('',*,*,#47925,.F.);
#63304=ORIENTED_EDGE('',*,*,#47926,.T.);
#63305=ORIENTED_EDGE('',*,*,#47927,.T.);
#63306=ORIENTED_EDGE('',*,*,#47928,.F.);
#63307=ORIENTED_EDGE('',*,*,#47923,.F.);
#63308=ORIENTED_EDGE('',*,*,#47929,.T.);
#63309=ORIENTED_EDGE('',*,*,#47930,.T.);
#63310=ORIENTED_EDGE('',*,*,#47931,.F.);
#63311=ORIENTED_EDGE('',*,*,#47927,.F.);
#63312=ORIENTED_EDGE('',*,*,#47932,.T.);
#63313=ORIENTED_EDGE('',*,*,#47925,.T.);
#63314=ORIENTED_EDGE('',*,*,#47933,.F.);
#63315=ORIENTED_EDGE('',*,*,#47930,.F.);
#63316=ORIENTED_EDGE('',*,*,#47934,.T.);
#63317=ORIENTED_EDGE('',*,*,#47935,.T.);
#63318=ORIENTED_EDGE('',*,*,#47936,.F.);
#63319=ORIENTED_EDGE('',*,*,#47937,.F.);
#63320=ORIENTED_EDGE('',*,*,#47938,.T.);
#63321=ORIENTED_EDGE('',*,*,#47939,.T.);
#63322=ORIENTED_EDGE('',*,*,#47940,.F.);
#63323=ORIENTED_EDGE('',*,*,#47935,.F.);
#63324=ORIENTED_EDGE('',*,*,#47941,.T.);
#63325=ORIENTED_EDGE('',*,*,#47942,.T.);
#63326=ORIENTED_EDGE('',*,*,#47943,.F.);
#63327=ORIENTED_EDGE('',*,*,#47939,.F.);
#63328=ORIENTED_EDGE('',*,*,#47944,.T.);
#63329=ORIENTED_EDGE('',*,*,#47937,.T.);
#63330=ORIENTED_EDGE('',*,*,#47945,.F.);
#63331=ORIENTED_EDGE('',*,*,#47942,.F.);
#63332=ORIENTED_EDGE('',*,*,#47946,.T.);
#63333=ORIENTED_EDGE('',*,*,#47947,.T.);
#63334=ORIENTED_EDGE('',*,*,#47948,.F.);
#63335=ORIENTED_EDGE('',*,*,#47949,.F.);
#63336=ORIENTED_EDGE('',*,*,#47950,.T.);
#63337=ORIENTED_EDGE('',*,*,#47951,.T.);
#63338=ORIENTED_EDGE('',*,*,#47952,.F.);
#63339=ORIENTED_EDGE('',*,*,#47947,.F.);
#63340=ORIENTED_EDGE('',*,*,#47953,.T.);
#63341=ORIENTED_EDGE('',*,*,#47954,.T.);
#63342=ORIENTED_EDGE('',*,*,#47955,.F.);
#63343=ORIENTED_EDGE('',*,*,#47951,.F.);
#63344=ORIENTED_EDGE('',*,*,#47956,.T.);
#63345=ORIENTED_EDGE('',*,*,#47949,.T.);
#63346=ORIENTED_EDGE('',*,*,#47957,.F.);
#63347=ORIENTED_EDGE('',*,*,#47954,.F.);
#63348=ORIENTED_EDGE('',*,*,#47958,.T.);
#63349=ORIENTED_EDGE('',*,*,#47959,.T.);
#63350=ORIENTED_EDGE('',*,*,#47960,.F.);
#63351=ORIENTED_EDGE('',*,*,#47961,.F.);
#63352=ORIENTED_EDGE('',*,*,#47962,.T.);
#63353=ORIENTED_EDGE('',*,*,#47963,.T.);
#63354=ORIENTED_EDGE('',*,*,#47964,.F.);
#63355=ORIENTED_EDGE('',*,*,#47959,.F.);
#63356=ORIENTED_EDGE('',*,*,#47965,.T.);
#63357=ORIENTED_EDGE('',*,*,#47966,.T.);
#63358=ORIENTED_EDGE('',*,*,#47967,.F.);
#63359=ORIENTED_EDGE('',*,*,#47963,.F.);
#63360=ORIENTED_EDGE('',*,*,#47968,.T.);
#63361=ORIENTED_EDGE('',*,*,#47961,.T.);
#63362=ORIENTED_EDGE('',*,*,#47969,.F.);
#63363=ORIENTED_EDGE('',*,*,#47966,.F.);
#63364=ORIENTED_EDGE('',*,*,#47970,.T.);
#63365=ORIENTED_EDGE('',*,*,#47971,.T.);
#63366=ORIENTED_EDGE('',*,*,#47972,.F.);
#63367=ORIENTED_EDGE('',*,*,#47973,.F.);
#63368=ORIENTED_EDGE('',*,*,#47974,.T.);
#63369=ORIENTED_EDGE('',*,*,#47975,.T.);
#63370=ORIENTED_EDGE('',*,*,#47976,.F.);
#63371=ORIENTED_EDGE('',*,*,#47971,.F.);
#63372=ORIENTED_EDGE('',*,*,#47977,.T.);
#63373=ORIENTED_EDGE('',*,*,#47978,.T.);
#63374=ORIENTED_EDGE('',*,*,#47979,.F.);
#63375=ORIENTED_EDGE('',*,*,#47975,.F.);
#63376=ORIENTED_EDGE('',*,*,#47980,.T.);
#63377=ORIENTED_EDGE('',*,*,#47973,.T.);
#63378=ORIENTED_EDGE('',*,*,#47981,.F.);
#63379=ORIENTED_EDGE('',*,*,#47978,.F.);
#63380=ORIENTED_EDGE('',*,*,#47982,.T.);
#63381=ORIENTED_EDGE('',*,*,#47983,.T.);
#63382=ORIENTED_EDGE('',*,*,#47984,.F.);
#63383=ORIENTED_EDGE('',*,*,#47985,.F.);
#63384=ORIENTED_EDGE('',*,*,#47986,.T.);
#63385=ORIENTED_EDGE('',*,*,#47987,.T.);
#63386=ORIENTED_EDGE('',*,*,#47988,.F.);
#63387=ORIENTED_EDGE('',*,*,#47983,.F.);
#63388=ORIENTED_EDGE('',*,*,#47989,.T.);
#63389=ORIENTED_EDGE('',*,*,#47990,.T.);
#63390=ORIENTED_EDGE('',*,*,#47991,.F.);
#63391=ORIENTED_EDGE('',*,*,#47987,.F.);
#63392=ORIENTED_EDGE('',*,*,#47992,.T.);
#63393=ORIENTED_EDGE('',*,*,#47985,.T.);
#63394=ORIENTED_EDGE('',*,*,#47993,.F.);
#63395=ORIENTED_EDGE('',*,*,#47990,.F.);
#63396=ORIENTED_EDGE('',*,*,#47994,.T.);
#63397=ORIENTED_EDGE('',*,*,#47995,.T.);
#63398=ORIENTED_EDGE('',*,*,#47996,.F.);
#63399=ORIENTED_EDGE('',*,*,#47997,.F.);
#63400=ORIENTED_EDGE('',*,*,#47998,.T.);
#63401=ORIENTED_EDGE('',*,*,#47999,.T.);
#63402=ORIENTED_EDGE('',*,*,#48000,.F.);
#63403=ORIENTED_EDGE('',*,*,#47995,.F.);
#63404=ORIENTED_EDGE('',*,*,#48001,.T.);
#63405=ORIENTED_EDGE('',*,*,#48002,.T.);
#63406=ORIENTED_EDGE('',*,*,#48003,.F.);
#63407=ORIENTED_EDGE('',*,*,#47999,.F.);
#63408=ORIENTED_EDGE('',*,*,#48004,.T.);
#63409=ORIENTED_EDGE('',*,*,#47997,.T.);
#63410=ORIENTED_EDGE('',*,*,#48005,.F.);
#63411=ORIENTED_EDGE('',*,*,#48002,.F.);
#63412=ORIENTED_EDGE('',*,*,#48006,.T.);
#63413=ORIENTED_EDGE('',*,*,#48007,.T.);
#63414=ORIENTED_EDGE('',*,*,#48008,.F.);
#63415=ORIENTED_EDGE('',*,*,#48009,.F.);
#63416=ORIENTED_EDGE('',*,*,#48010,.T.);
#63417=ORIENTED_EDGE('',*,*,#48011,.T.);
#63418=ORIENTED_EDGE('',*,*,#48012,.F.);
#63419=ORIENTED_EDGE('',*,*,#48007,.F.);
#63420=ORIENTED_EDGE('',*,*,#48013,.T.);
#63421=ORIENTED_EDGE('',*,*,#48014,.T.);
#63422=ORIENTED_EDGE('',*,*,#48015,.F.);
#63423=ORIENTED_EDGE('',*,*,#48011,.F.);
#63424=ORIENTED_EDGE('',*,*,#48016,.T.);
#63425=ORIENTED_EDGE('',*,*,#48009,.T.);
#63426=ORIENTED_EDGE('',*,*,#48017,.F.);
#63427=ORIENTED_EDGE('',*,*,#48014,.F.);
#63428=ORIENTED_EDGE('',*,*,#48018,.T.);
#63429=ORIENTED_EDGE('',*,*,#48019,.T.);
#63430=ORIENTED_EDGE('',*,*,#48020,.F.);
#63431=ORIENTED_EDGE('',*,*,#48021,.F.);
#63432=ORIENTED_EDGE('',*,*,#48022,.T.);
#63433=ORIENTED_EDGE('',*,*,#48023,.T.);
#63434=ORIENTED_EDGE('',*,*,#48024,.F.);
#63435=ORIENTED_EDGE('',*,*,#48019,.F.);
#63436=ORIENTED_EDGE('',*,*,#48025,.T.);
#63437=ORIENTED_EDGE('',*,*,#48026,.T.);
#63438=ORIENTED_EDGE('',*,*,#48027,.F.);
#63439=ORIENTED_EDGE('',*,*,#48023,.F.);
#63440=ORIENTED_EDGE('',*,*,#48028,.T.);
#63441=ORIENTED_EDGE('',*,*,#48021,.T.);
#63442=ORIENTED_EDGE('',*,*,#48029,.F.);
#63443=ORIENTED_EDGE('',*,*,#48026,.F.);
#63444=ORIENTED_EDGE('',*,*,#48030,.T.);
#63445=ORIENTED_EDGE('',*,*,#48031,.T.);
#63446=ORIENTED_EDGE('',*,*,#48032,.F.);
#63447=ORIENTED_EDGE('',*,*,#48033,.F.);
#63448=ORIENTED_EDGE('',*,*,#48034,.T.);
#63449=ORIENTED_EDGE('',*,*,#48035,.T.);
#63450=ORIENTED_EDGE('',*,*,#48036,.F.);
#63451=ORIENTED_EDGE('',*,*,#48031,.F.);
#63452=ORIENTED_EDGE('',*,*,#48037,.T.);
#63453=ORIENTED_EDGE('',*,*,#48038,.T.);
#63454=ORIENTED_EDGE('',*,*,#48039,.F.);
#63455=ORIENTED_EDGE('',*,*,#48035,.F.);
#63456=ORIENTED_EDGE('',*,*,#48040,.T.);
#63457=ORIENTED_EDGE('',*,*,#48033,.T.);
#63458=ORIENTED_EDGE('',*,*,#48041,.F.);
#63459=ORIENTED_EDGE('',*,*,#48038,.F.);
#63460=ORIENTED_EDGE('',*,*,#48042,.T.);
#63461=ORIENTED_EDGE('',*,*,#48043,.T.);
#63462=ORIENTED_EDGE('',*,*,#48044,.F.);
#63463=ORIENTED_EDGE('',*,*,#48045,.F.);
#63464=ORIENTED_EDGE('',*,*,#48046,.T.);
#63465=ORIENTED_EDGE('',*,*,#48047,.T.);
#63466=ORIENTED_EDGE('',*,*,#48048,.F.);
#63467=ORIENTED_EDGE('',*,*,#48043,.F.);
#63468=ORIENTED_EDGE('',*,*,#48049,.T.);
#63469=ORIENTED_EDGE('',*,*,#48050,.T.);
#63470=ORIENTED_EDGE('',*,*,#48051,.F.);
#63471=ORIENTED_EDGE('',*,*,#48047,.F.);
#63472=ORIENTED_EDGE('',*,*,#48052,.T.);
#63473=ORIENTED_EDGE('',*,*,#48045,.T.);
#63474=ORIENTED_EDGE('',*,*,#48053,.F.);
#63475=ORIENTED_EDGE('',*,*,#48050,.F.);
#63476=ORIENTED_EDGE('',*,*,#48054,.T.);
#63477=ORIENTED_EDGE('',*,*,#48055,.T.);
#63478=ORIENTED_EDGE('',*,*,#48056,.F.);
#63479=ORIENTED_EDGE('',*,*,#48057,.F.);
#63480=ORIENTED_EDGE('',*,*,#48058,.T.);
#63481=ORIENTED_EDGE('',*,*,#48059,.T.);
#63482=ORIENTED_EDGE('',*,*,#48060,.F.);
#63483=ORIENTED_EDGE('',*,*,#48055,.F.);
#63484=ORIENTED_EDGE('',*,*,#48061,.T.);
#63485=ORIENTED_EDGE('',*,*,#48062,.T.);
#63486=ORIENTED_EDGE('',*,*,#48063,.F.);
#63487=ORIENTED_EDGE('',*,*,#48059,.F.);
#63488=ORIENTED_EDGE('',*,*,#48064,.T.);
#63489=ORIENTED_EDGE('',*,*,#48057,.T.);
#63490=ORIENTED_EDGE('',*,*,#48065,.F.);
#63491=ORIENTED_EDGE('',*,*,#48062,.F.);
#63492=ORIENTED_EDGE('',*,*,#48066,.T.);
#63493=ORIENTED_EDGE('',*,*,#48067,.T.);
#63494=ORIENTED_EDGE('',*,*,#48068,.F.);
#63495=ORIENTED_EDGE('',*,*,#48069,.F.);
#63496=ORIENTED_EDGE('',*,*,#48070,.T.);
#63497=ORIENTED_EDGE('',*,*,#48071,.T.);
#63498=ORIENTED_EDGE('',*,*,#48072,.F.);
#63499=ORIENTED_EDGE('',*,*,#48067,.F.);
#63500=ORIENTED_EDGE('',*,*,#48073,.T.);
#63501=ORIENTED_EDGE('',*,*,#48074,.T.);
#63502=ORIENTED_EDGE('',*,*,#48075,.F.);
#63503=ORIENTED_EDGE('',*,*,#48071,.F.);
#63504=ORIENTED_EDGE('',*,*,#48076,.T.);
#63505=ORIENTED_EDGE('',*,*,#48069,.T.);
#63506=ORIENTED_EDGE('',*,*,#48077,.F.);
#63507=ORIENTED_EDGE('',*,*,#48074,.F.);
#63508=ORIENTED_EDGE('',*,*,#48078,.T.);
#63509=ORIENTED_EDGE('',*,*,#48079,.T.);
#63510=ORIENTED_EDGE('',*,*,#48080,.F.);
#63511=ORIENTED_EDGE('',*,*,#48081,.F.);
#63512=ORIENTED_EDGE('',*,*,#48082,.T.);
#63513=ORIENTED_EDGE('',*,*,#48083,.T.);
#63514=ORIENTED_EDGE('',*,*,#48084,.F.);
#63515=ORIENTED_EDGE('',*,*,#48079,.F.);
#63516=ORIENTED_EDGE('',*,*,#48085,.T.);
#63517=ORIENTED_EDGE('',*,*,#48086,.T.);
#63518=ORIENTED_EDGE('',*,*,#48087,.F.);
#63519=ORIENTED_EDGE('',*,*,#48083,.F.);
#63520=ORIENTED_EDGE('',*,*,#48088,.T.);
#63521=ORIENTED_EDGE('',*,*,#48081,.T.);
#63522=ORIENTED_EDGE('',*,*,#48089,.F.);
#63523=ORIENTED_EDGE('',*,*,#48086,.F.);
#63524=ORIENTED_EDGE('',*,*,#48090,.T.);
#63525=ORIENTED_EDGE('',*,*,#48091,.T.);
#63526=ORIENTED_EDGE('',*,*,#48092,.F.);
#63527=ORIENTED_EDGE('',*,*,#48093,.F.);
#63528=ORIENTED_EDGE('',*,*,#48094,.T.);
#63529=ORIENTED_EDGE('',*,*,#48095,.T.);
#63530=ORIENTED_EDGE('',*,*,#48096,.F.);
#63531=ORIENTED_EDGE('',*,*,#48091,.F.);
#63532=ORIENTED_EDGE('',*,*,#48097,.T.);
#63533=ORIENTED_EDGE('',*,*,#48098,.T.);
#63534=ORIENTED_EDGE('',*,*,#48099,.F.);
#63535=ORIENTED_EDGE('',*,*,#48095,.F.);
#63536=ORIENTED_EDGE('',*,*,#48100,.T.);
#63537=ORIENTED_EDGE('',*,*,#48093,.T.);
#63538=ORIENTED_EDGE('',*,*,#48101,.F.);
#63539=ORIENTED_EDGE('',*,*,#48098,.F.);
#63540=ORIENTED_EDGE('',*,*,#48102,.T.);
#63541=ORIENTED_EDGE('',*,*,#48103,.T.);
#63542=ORIENTED_EDGE('',*,*,#48104,.F.);
#63543=ORIENTED_EDGE('',*,*,#48105,.F.);
#63544=ORIENTED_EDGE('',*,*,#48106,.T.);
#63545=ORIENTED_EDGE('',*,*,#48107,.T.);
#63546=ORIENTED_EDGE('',*,*,#48108,.F.);
#63547=ORIENTED_EDGE('',*,*,#48103,.F.);
#63548=ORIENTED_EDGE('',*,*,#48109,.T.);
#63549=ORIENTED_EDGE('',*,*,#48110,.T.);
#63550=ORIENTED_EDGE('',*,*,#48111,.F.);
#63551=ORIENTED_EDGE('',*,*,#48107,.F.);
#63552=ORIENTED_EDGE('',*,*,#48112,.T.);
#63553=ORIENTED_EDGE('',*,*,#48105,.T.);
#63554=ORIENTED_EDGE('',*,*,#48113,.F.);
#63555=ORIENTED_EDGE('',*,*,#48110,.F.);
#63556=ORIENTED_EDGE('',*,*,#48114,.T.);
#63557=ORIENTED_EDGE('',*,*,#48115,.T.);
#63558=ORIENTED_EDGE('',*,*,#48116,.F.);
#63559=ORIENTED_EDGE('',*,*,#48117,.F.);
#63560=ORIENTED_EDGE('',*,*,#48118,.T.);
#63561=ORIENTED_EDGE('',*,*,#48119,.T.);
#63562=ORIENTED_EDGE('',*,*,#48120,.F.);
#63563=ORIENTED_EDGE('',*,*,#48115,.F.);
#63564=ORIENTED_EDGE('',*,*,#48121,.T.);
#63565=ORIENTED_EDGE('',*,*,#48122,.T.);
#63566=ORIENTED_EDGE('',*,*,#48123,.F.);
#63567=ORIENTED_EDGE('',*,*,#48119,.F.);
#63568=ORIENTED_EDGE('',*,*,#48124,.T.);
#63569=ORIENTED_EDGE('',*,*,#48117,.T.);
#63570=ORIENTED_EDGE('',*,*,#48125,.F.);
#63571=ORIENTED_EDGE('',*,*,#48122,.F.);
#63572=ORIENTED_EDGE('',*,*,#48126,.T.);
#63573=ORIENTED_EDGE('',*,*,#48127,.T.);
#63574=ORIENTED_EDGE('',*,*,#48128,.F.);
#63575=ORIENTED_EDGE('',*,*,#48129,.F.);
#63576=ORIENTED_EDGE('',*,*,#48130,.T.);
#63577=ORIENTED_EDGE('',*,*,#48131,.T.);
#63578=ORIENTED_EDGE('',*,*,#48132,.F.);
#63579=ORIENTED_EDGE('',*,*,#48127,.F.);
#63580=ORIENTED_EDGE('',*,*,#48133,.T.);
#63581=ORIENTED_EDGE('',*,*,#48134,.T.);
#63582=ORIENTED_EDGE('',*,*,#48135,.F.);
#63583=ORIENTED_EDGE('',*,*,#48131,.F.);
#63584=ORIENTED_EDGE('',*,*,#48136,.T.);
#63585=ORIENTED_EDGE('',*,*,#48129,.T.);
#63586=ORIENTED_EDGE('',*,*,#48137,.F.);
#63587=ORIENTED_EDGE('',*,*,#48134,.F.);
#63588=ORIENTED_EDGE('',*,*,#48138,.T.);
#63589=ORIENTED_EDGE('',*,*,#48139,.T.);
#63590=ORIENTED_EDGE('',*,*,#48140,.F.);
#63591=ORIENTED_EDGE('',*,*,#48141,.F.);
#63592=ORIENTED_EDGE('',*,*,#48142,.T.);
#63593=ORIENTED_EDGE('',*,*,#48143,.T.);
#63594=ORIENTED_EDGE('',*,*,#48144,.F.);
#63595=ORIENTED_EDGE('',*,*,#48139,.F.);
#63596=ORIENTED_EDGE('',*,*,#48145,.T.);
#63597=ORIENTED_EDGE('',*,*,#48146,.T.);
#63598=ORIENTED_EDGE('',*,*,#48147,.F.);
#63599=ORIENTED_EDGE('',*,*,#48143,.F.);
#63600=ORIENTED_EDGE('',*,*,#48148,.T.);
#63601=ORIENTED_EDGE('',*,*,#48141,.T.);
#63602=ORIENTED_EDGE('',*,*,#48149,.F.);
#63603=ORIENTED_EDGE('',*,*,#48146,.F.);
#63604=ORIENTED_EDGE('',*,*,#48150,.T.);
#63605=ORIENTED_EDGE('',*,*,#48151,.T.);
#63606=ORIENTED_EDGE('',*,*,#48152,.F.);
#63607=ORIENTED_EDGE('',*,*,#48153,.F.);
#63608=ORIENTED_EDGE('',*,*,#48154,.T.);
#63609=ORIENTED_EDGE('',*,*,#48155,.T.);
#63610=ORIENTED_EDGE('',*,*,#48156,.F.);
#63611=ORIENTED_EDGE('',*,*,#48151,.F.);
#63612=ORIENTED_EDGE('',*,*,#48157,.T.);
#63613=ORIENTED_EDGE('',*,*,#48158,.T.);
#63614=ORIENTED_EDGE('',*,*,#48159,.F.);
#63615=ORIENTED_EDGE('',*,*,#48155,.F.);
#63616=ORIENTED_EDGE('',*,*,#48160,.T.);
#63617=ORIENTED_EDGE('',*,*,#48153,.T.);
#63618=ORIENTED_EDGE('',*,*,#48161,.F.);
#63619=ORIENTED_EDGE('',*,*,#48158,.F.);
#63620=ORIENTED_EDGE('',*,*,#48162,.T.);
#63621=ORIENTED_EDGE('',*,*,#48163,.T.);
#63622=ORIENTED_EDGE('',*,*,#48164,.F.);
#63623=ORIENTED_EDGE('',*,*,#48165,.F.);
#63624=ORIENTED_EDGE('',*,*,#48166,.T.);
#63625=ORIENTED_EDGE('',*,*,#48167,.T.);
#63626=ORIENTED_EDGE('',*,*,#48168,.F.);
#63627=ORIENTED_EDGE('',*,*,#48163,.F.);
#63628=ORIENTED_EDGE('',*,*,#48169,.T.);
#63629=ORIENTED_EDGE('',*,*,#48170,.T.);
#63630=ORIENTED_EDGE('',*,*,#48171,.F.);
#63631=ORIENTED_EDGE('',*,*,#48167,.F.);
#63632=ORIENTED_EDGE('',*,*,#48172,.T.);
#63633=ORIENTED_EDGE('',*,*,#48165,.T.);
#63634=ORIENTED_EDGE('',*,*,#48173,.F.);
#63635=ORIENTED_EDGE('',*,*,#48170,.F.);
#63636=ORIENTED_EDGE('',*,*,#48174,.T.);
#63637=ORIENTED_EDGE('',*,*,#48175,.T.);
#63638=ORIENTED_EDGE('',*,*,#48176,.F.);
#63639=ORIENTED_EDGE('',*,*,#48177,.F.);
#63640=ORIENTED_EDGE('',*,*,#48178,.T.);
#63641=ORIENTED_EDGE('',*,*,#48179,.T.);
#63642=ORIENTED_EDGE('',*,*,#48180,.F.);
#63643=ORIENTED_EDGE('',*,*,#48175,.F.);
#63644=ORIENTED_EDGE('',*,*,#48181,.T.);
#63645=ORIENTED_EDGE('',*,*,#48182,.T.);
#63646=ORIENTED_EDGE('',*,*,#48183,.F.);
#63647=ORIENTED_EDGE('',*,*,#48179,.F.);
#63648=ORIENTED_EDGE('',*,*,#48184,.T.);
#63649=ORIENTED_EDGE('',*,*,#48177,.T.);
#63650=ORIENTED_EDGE('',*,*,#48185,.F.);
#63651=ORIENTED_EDGE('',*,*,#48182,.F.);
#63652=ORIENTED_EDGE('',*,*,#48186,.T.);
#63653=ORIENTED_EDGE('',*,*,#48187,.T.);
#63654=ORIENTED_EDGE('',*,*,#48188,.F.);
#63655=ORIENTED_EDGE('',*,*,#48189,.F.);
#63656=ORIENTED_EDGE('',*,*,#48190,.T.);
#63657=ORIENTED_EDGE('',*,*,#48191,.T.);
#63658=ORIENTED_EDGE('',*,*,#48192,.F.);
#63659=ORIENTED_EDGE('',*,*,#48187,.F.);
#63660=ORIENTED_EDGE('',*,*,#48193,.T.);
#63661=ORIENTED_EDGE('',*,*,#48194,.T.);
#63662=ORIENTED_EDGE('',*,*,#48195,.F.);
#63663=ORIENTED_EDGE('',*,*,#48191,.F.);
#63664=ORIENTED_EDGE('',*,*,#48196,.T.);
#63665=ORIENTED_EDGE('',*,*,#48189,.T.);
#63666=ORIENTED_EDGE('',*,*,#48197,.F.);
#63667=ORIENTED_EDGE('',*,*,#48194,.F.);
#63668=ORIENTED_EDGE('',*,*,#48198,.T.);
#63669=ORIENTED_EDGE('',*,*,#48199,.T.);
#63670=ORIENTED_EDGE('',*,*,#48200,.F.);
#63671=ORIENTED_EDGE('',*,*,#48201,.F.);
#63672=ORIENTED_EDGE('',*,*,#48202,.T.);
#63673=ORIENTED_EDGE('',*,*,#48203,.T.);
#63674=ORIENTED_EDGE('',*,*,#48204,.F.);
#63675=ORIENTED_EDGE('',*,*,#48199,.F.);
#63676=ORIENTED_EDGE('',*,*,#48205,.T.);
#63677=ORIENTED_EDGE('',*,*,#48206,.T.);
#63678=ORIENTED_EDGE('',*,*,#48207,.F.);
#63679=ORIENTED_EDGE('',*,*,#48203,.F.);
#63680=ORIENTED_EDGE('',*,*,#48208,.T.);
#63681=ORIENTED_EDGE('',*,*,#48201,.T.);
#63682=ORIENTED_EDGE('',*,*,#48209,.F.);
#63683=ORIENTED_EDGE('',*,*,#48206,.F.);
#63684=ORIENTED_EDGE('',*,*,#48210,.T.);
#63685=ORIENTED_EDGE('',*,*,#48211,.T.);
#63686=ORIENTED_EDGE('',*,*,#48212,.F.);
#63687=ORIENTED_EDGE('',*,*,#48213,.F.);
#63688=ORIENTED_EDGE('',*,*,#48214,.T.);
#63689=ORIENTED_EDGE('',*,*,#48215,.T.);
#63690=ORIENTED_EDGE('',*,*,#48216,.F.);
#63691=ORIENTED_EDGE('',*,*,#48211,.F.);
#63692=ORIENTED_EDGE('',*,*,#48217,.T.);
#63693=ORIENTED_EDGE('',*,*,#48218,.T.);
#63694=ORIENTED_EDGE('',*,*,#48219,.F.);
#63695=ORIENTED_EDGE('',*,*,#48215,.F.);
#63696=ORIENTED_EDGE('',*,*,#48220,.T.);
#63697=ORIENTED_EDGE('',*,*,#48213,.T.);
#63698=ORIENTED_EDGE('',*,*,#48221,.F.);
#63699=ORIENTED_EDGE('',*,*,#48218,.F.);
#63700=ORIENTED_EDGE('',*,*,#48222,.T.);
#63701=ORIENTED_EDGE('',*,*,#48223,.T.);
#63702=ORIENTED_EDGE('',*,*,#48224,.F.);
#63703=ORIENTED_EDGE('',*,*,#48225,.F.);
#63704=ORIENTED_EDGE('',*,*,#48226,.T.);
#63705=ORIENTED_EDGE('',*,*,#48227,.T.);
#63706=ORIENTED_EDGE('',*,*,#48228,.F.);
#63707=ORIENTED_EDGE('',*,*,#48223,.F.);
#63708=ORIENTED_EDGE('',*,*,#48229,.T.);
#63709=ORIENTED_EDGE('',*,*,#48230,.T.);
#63710=ORIENTED_EDGE('',*,*,#48231,.F.);
#63711=ORIENTED_EDGE('',*,*,#48227,.F.);
#63712=ORIENTED_EDGE('',*,*,#48232,.T.);
#63713=ORIENTED_EDGE('',*,*,#48225,.T.);
#63714=ORIENTED_EDGE('',*,*,#48233,.F.);
#63715=ORIENTED_EDGE('',*,*,#48230,.F.);
#63716=ORIENTED_EDGE('',*,*,#48234,.T.);
#63717=ORIENTED_EDGE('',*,*,#48235,.T.);
#63718=ORIENTED_EDGE('',*,*,#48236,.F.);
#63719=ORIENTED_EDGE('',*,*,#48237,.F.);
#63720=ORIENTED_EDGE('',*,*,#48238,.T.);
#63721=ORIENTED_EDGE('',*,*,#48239,.T.);
#63722=ORIENTED_EDGE('',*,*,#48240,.F.);
#63723=ORIENTED_EDGE('',*,*,#48235,.F.);
#63724=ORIENTED_EDGE('',*,*,#48241,.T.);
#63725=ORIENTED_EDGE('',*,*,#48242,.T.);
#63726=ORIENTED_EDGE('',*,*,#48243,.F.);
#63727=ORIENTED_EDGE('',*,*,#48239,.F.);
#63728=ORIENTED_EDGE('',*,*,#48244,.T.);
#63729=ORIENTED_EDGE('',*,*,#48237,.T.);
#63730=ORIENTED_EDGE('',*,*,#48245,.F.);
#63731=ORIENTED_EDGE('',*,*,#48242,.F.);
#63732=ORIENTED_EDGE('',*,*,#48246,.T.);
#63733=ORIENTED_EDGE('',*,*,#48247,.T.);
#63734=ORIENTED_EDGE('',*,*,#48248,.F.);
#63735=ORIENTED_EDGE('',*,*,#48249,.F.);
#63736=ORIENTED_EDGE('',*,*,#48250,.T.);
#63737=ORIENTED_EDGE('',*,*,#48251,.T.);
#63738=ORIENTED_EDGE('',*,*,#48252,.F.);
#63739=ORIENTED_EDGE('',*,*,#48247,.F.);
#63740=ORIENTED_EDGE('',*,*,#48253,.T.);
#63741=ORIENTED_EDGE('',*,*,#48254,.T.);
#63742=ORIENTED_EDGE('',*,*,#48255,.F.);
#63743=ORIENTED_EDGE('',*,*,#48251,.F.);
#63744=ORIENTED_EDGE('',*,*,#48256,.T.);
#63745=ORIENTED_EDGE('',*,*,#48249,.T.);
#63746=ORIENTED_EDGE('',*,*,#48257,.F.);
#63747=ORIENTED_EDGE('',*,*,#48254,.F.);
#63748=ORIENTED_EDGE('',*,*,#48258,.T.);
#63749=ORIENTED_EDGE('',*,*,#48259,.T.);
#63750=ORIENTED_EDGE('',*,*,#48260,.F.);
#63751=ORIENTED_EDGE('',*,*,#48261,.F.);
#63752=ORIENTED_EDGE('',*,*,#48262,.T.);
#63753=ORIENTED_EDGE('',*,*,#48263,.T.);
#63754=ORIENTED_EDGE('',*,*,#48264,.F.);
#63755=ORIENTED_EDGE('',*,*,#48259,.F.);
#63756=ORIENTED_EDGE('',*,*,#48265,.T.);
#63757=ORIENTED_EDGE('',*,*,#48266,.T.);
#63758=ORIENTED_EDGE('',*,*,#48267,.F.);
#63759=ORIENTED_EDGE('',*,*,#48263,.F.);
#63760=ORIENTED_EDGE('',*,*,#48268,.T.);
#63761=ORIENTED_EDGE('',*,*,#48261,.T.);
#63762=ORIENTED_EDGE('',*,*,#48269,.F.);
#63763=ORIENTED_EDGE('',*,*,#48266,.F.);
#63764=ORIENTED_EDGE('',*,*,#48270,.T.);
#63765=ORIENTED_EDGE('',*,*,#48271,.T.);
#63766=ORIENTED_EDGE('',*,*,#48272,.F.);
#63767=ORIENTED_EDGE('',*,*,#48273,.F.);
#63768=ORIENTED_EDGE('',*,*,#48274,.T.);
#63769=ORIENTED_EDGE('',*,*,#48275,.T.);
#63770=ORIENTED_EDGE('',*,*,#48276,.F.);
#63771=ORIENTED_EDGE('',*,*,#48271,.F.);
#63772=ORIENTED_EDGE('',*,*,#48277,.T.);
#63773=ORIENTED_EDGE('',*,*,#48278,.T.);
#63774=ORIENTED_EDGE('',*,*,#48279,.F.);
#63775=ORIENTED_EDGE('',*,*,#48275,.F.);
#63776=ORIENTED_EDGE('',*,*,#48280,.T.);
#63777=ORIENTED_EDGE('',*,*,#48273,.T.);
#63778=ORIENTED_EDGE('',*,*,#48281,.F.);
#63779=ORIENTED_EDGE('',*,*,#48278,.F.);
#63780=ORIENTED_EDGE('',*,*,#48282,.T.);
#63781=ORIENTED_EDGE('',*,*,#48283,.T.);
#63782=ORIENTED_EDGE('',*,*,#48284,.F.);
#63783=ORIENTED_EDGE('',*,*,#48285,.F.);
#63784=ORIENTED_EDGE('',*,*,#48286,.T.);
#63785=ORIENTED_EDGE('',*,*,#48287,.T.);
#63786=ORIENTED_EDGE('',*,*,#48288,.F.);
#63787=ORIENTED_EDGE('',*,*,#48283,.F.);
#63788=ORIENTED_EDGE('',*,*,#48289,.T.);
#63789=ORIENTED_EDGE('',*,*,#48290,.T.);
#63790=ORIENTED_EDGE('',*,*,#48291,.F.);
#63791=ORIENTED_EDGE('',*,*,#48287,.F.);
#63792=ORIENTED_EDGE('',*,*,#48292,.T.);
#63793=ORIENTED_EDGE('',*,*,#48285,.T.);
#63794=ORIENTED_EDGE('',*,*,#48293,.F.);
#63795=ORIENTED_EDGE('',*,*,#48290,.F.);
#63796=ORIENTED_EDGE('',*,*,#48294,.T.);
#63797=ORIENTED_EDGE('',*,*,#48295,.T.);
#63798=ORIENTED_EDGE('',*,*,#48296,.F.);
#63799=ORIENTED_EDGE('',*,*,#48297,.F.);
#63800=ORIENTED_EDGE('',*,*,#48298,.T.);
#63801=ORIENTED_EDGE('',*,*,#48299,.T.);
#63802=ORIENTED_EDGE('',*,*,#48300,.F.);
#63803=ORIENTED_EDGE('',*,*,#48295,.F.);
#63804=ORIENTED_EDGE('',*,*,#48301,.T.);
#63805=ORIENTED_EDGE('',*,*,#48302,.T.);
#63806=ORIENTED_EDGE('',*,*,#48303,.F.);
#63807=ORIENTED_EDGE('',*,*,#48299,.F.);
#63808=ORIENTED_EDGE('',*,*,#48304,.T.);
#63809=ORIENTED_EDGE('',*,*,#48297,.T.);
#63810=ORIENTED_EDGE('',*,*,#48305,.F.);
#63811=ORIENTED_EDGE('',*,*,#48302,.F.);
#63812=ORIENTED_EDGE('',*,*,#48306,.T.);
#63813=ORIENTED_EDGE('',*,*,#48307,.T.);
#63814=ORIENTED_EDGE('',*,*,#48308,.F.);
#63815=ORIENTED_EDGE('',*,*,#48309,.F.);
#63816=ORIENTED_EDGE('',*,*,#48310,.T.);
#63817=ORIENTED_EDGE('',*,*,#48311,.T.);
#63818=ORIENTED_EDGE('',*,*,#48312,.F.);
#63819=ORIENTED_EDGE('',*,*,#48307,.F.);
#63820=ORIENTED_EDGE('',*,*,#48313,.T.);
#63821=ORIENTED_EDGE('',*,*,#48314,.T.);
#63822=ORIENTED_EDGE('',*,*,#48315,.F.);
#63823=ORIENTED_EDGE('',*,*,#48311,.F.);
#63824=ORIENTED_EDGE('',*,*,#48316,.T.);
#63825=ORIENTED_EDGE('',*,*,#48309,.T.);
#63826=ORIENTED_EDGE('',*,*,#48317,.F.);
#63827=ORIENTED_EDGE('',*,*,#48314,.F.);
#63828=ORIENTED_EDGE('',*,*,#48318,.T.);
#63829=ORIENTED_EDGE('',*,*,#48319,.T.);
#63830=ORIENTED_EDGE('',*,*,#48320,.F.);
#63831=ORIENTED_EDGE('',*,*,#48321,.F.);
#63832=ORIENTED_EDGE('',*,*,#48322,.T.);
#63833=ORIENTED_EDGE('',*,*,#48323,.T.);
#63834=ORIENTED_EDGE('',*,*,#48324,.F.);
#63835=ORIENTED_EDGE('',*,*,#48319,.F.);
#63836=ORIENTED_EDGE('',*,*,#48325,.T.);
#63837=ORIENTED_EDGE('',*,*,#48326,.T.);
#63838=ORIENTED_EDGE('',*,*,#48327,.F.);
#63839=ORIENTED_EDGE('',*,*,#48323,.F.);
#63840=ORIENTED_EDGE('',*,*,#48328,.T.);
#63841=ORIENTED_EDGE('',*,*,#48321,.T.);
#63842=ORIENTED_EDGE('',*,*,#48329,.F.);
#63843=ORIENTED_EDGE('',*,*,#48326,.F.);
#63844=ORIENTED_EDGE('',*,*,#48330,.T.);
#63845=ORIENTED_EDGE('',*,*,#48331,.T.);
#63846=ORIENTED_EDGE('',*,*,#48332,.F.);
#63847=ORIENTED_EDGE('',*,*,#48333,.F.);
#63848=ORIENTED_EDGE('',*,*,#48334,.T.);
#63849=ORIENTED_EDGE('',*,*,#48335,.T.);
#63850=ORIENTED_EDGE('',*,*,#48336,.F.);
#63851=ORIENTED_EDGE('',*,*,#48331,.F.);
#63852=ORIENTED_EDGE('',*,*,#48337,.T.);
#63853=ORIENTED_EDGE('',*,*,#48338,.T.);
#63854=ORIENTED_EDGE('',*,*,#48339,.F.);
#63855=ORIENTED_EDGE('',*,*,#48335,.F.);
#63856=ORIENTED_EDGE('',*,*,#48340,.T.);
#63857=ORIENTED_EDGE('',*,*,#48333,.T.);
#63858=ORIENTED_EDGE('',*,*,#48341,.F.);
#63859=ORIENTED_EDGE('',*,*,#48338,.F.);
#63860=ORIENTED_EDGE('',*,*,#48342,.T.);
#63861=ORIENTED_EDGE('',*,*,#48343,.T.);
#63862=ORIENTED_EDGE('',*,*,#48344,.F.);
#63863=ORIENTED_EDGE('',*,*,#48345,.F.);
#63864=ORIENTED_EDGE('',*,*,#48346,.T.);
#63865=ORIENTED_EDGE('',*,*,#48347,.T.);
#63866=ORIENTED_EDGE('',*,*,#48348,.F.);
#63867=ORIENTED_EDGE('',*,*,#48343,.F.);
#63868=ORIENTED_EDGE('',*,*,#48349,.T.);
#63869=ORIENTED_EDGE('',*,*,#48350,.T.);
#63870=ORIENTED_EDGE('',*,*,#48351,.F.);
#63871=ORIENTED_EDGE('',*,*,#48347,.F.);
#63872=ORIENTED_EDGE('',*,*,#48352,.T.);
#63873=ORIENTED_EDGE('',*,*,#48345,.T.);
#63874=ORIENTED_EDGE('',*,*,#48353,.F.);
#63875=ORIENTED_EDGE('',*,*,#48350,.F.);
#63876=ORIENTED_EDGE('',*,*,#48354,.T.);
#63877=ORIENTED_EDGE('',*,*,#48355,.T.);
#63878=ORIENTED_EDGE('',*,*,#48356,.F.);
#63879=ORIENTED_EDGE('',*,*,#48357,.F.);
#63880=ORIENTED_EDGE('',*,*,#48358,.T.);
#63881=ORIENTED_EDGE('',*,*,#48359,.T.);
#63882=ORIENTED_EDGE('',*,*,#48360,.F.);
#63883=ORIENTED_EDGE('',*,*,#48355,.F.);
#63884=ORIENTED_EDGE('',*,*,#48361,.T.);
#63885=ORIENTED_EDGE('',*,*,#48362,.T.);
#63886=ORIENTED_EDGE('',*,*,#48363,.F.);
#63887=ORIENTED_EDGE('',*,*,#48359,.F.);
#63888=ORIENTED_EDGE('',*,*,#48364,.T.);
#63889=ORIENTED_EDGE('',*,*,#48357,.T.);
#63890=ORIENTED_EDGE('',*,*,#48365,.F.);
#63891=ORIENTED_EDGE('',*,*,#48362,.F.);
#63892=ORIENTED_EDGE('',*,*,#48366,.T.);
#63893=ORIENTED_EDGE('',*,*,#48367,.T.);
#63894=ORIENTED_EDGE('',*,*,#48368,.F.);
#63895=ORIENTED_EDGE('',*,*,#48369,.F.);
#63896=ORIENTED_EDGE('',*,*,#48370,.T.);
#63897=ORIENTED_EDGE('',*,*,#48371,.T.);
#63898=ORIENTED_EDGE('',*,*,#48372,.F.);
#63899=ORIENTED_EDGE('',*,*,#48367,.F.);
#63900=ORIENTED_EDGE('',*,*,#48373,.T.);
#63901=ORIENTED_EDGE('',*,*,#48374,.T.);
#63902=ORIENTED_EDGE('',*,*,#48375,.F.);
#63903=ORIENTED_EDGE('',*,*,#48371,.F.);
#63904=ORIENTED_EDGE('',*,*,#48376,.T.);
#63905=ORIENTED_EDGE('',*,*,#48369,.T.);
#63906=ORIENTED_EDGE('',*,*,#48377,.F.);
#63907=ORIENTED_EDGE('',*,*,#48374,.F.);
#63908=ORIENTED_EDGE('',*,*,#48378,.T.);
#63909=ORIENTED_EDGE('',*,*,#48379,.T.);
#63910=ORIENTED_EDGE('',*,*,#48380,.F.);
#63911=ORIENTED_EDGE('',*,*,#48381,.F.);
#63912=ORIENTED_EDGE('',*,*,#48382,.T.);
#63913=ORIENTED_EDGE('',*,*,#48383,.T.);
#63914=ORIENTED_EDGE('',*,*,#48384,.F.);
#63915=ORIENTED_EDGE('',*,*,#48379,.F.);
#63916=ORIENTED_EDGE('',*,*,#48385,.T.);
#63917=ORIENTED_EDGE('',*,*,#48386,.T.);
#63918=ORIENTED_EDGE('',*,*,#48387,.F.);
#63919=ORIENTED_EDGE('',*,*,#48383,.F.);
#63920=ORIENTED_EDGE('',*,*,#48388,.T.);
#63921=ORIENTED_EDGE('',*,*,#48381,.T.);
#63922=ORIENTED_EDGE('',*,*,#48389,.F.);
#63923=ORIENTED_EDGE('',*,*,#48386,.F.);
#63924=ORIENTED_EDGE('',*,*,#48390,.T.);
#63925=ORIENTED_EDGE('',*,*,#48391,.T.);
#63926=ORIENTED_EDGE('',*,*,#48392,.F.);
#63927=ORIENTED_EDGE('',*,*,#48393,.F.);
#63928=ORIENTED_EDGE('',*,*,#48394,.T.);
#63929=ORIENTED_EDGE('',*,*,#48395,.T.);
#63930=ORIENTED_EDGE('',*,*,#48396,.F.);
#63931=ORIENTED_EDGE('',*,*,#48391,.F.);
#63932=ORIENTED_EDGE('',*,*,#48397,.T.);
#63933=ORIENTED_EDGE('',*,*,#48398,.T.);
#63934=ORIENTED_EDGE('',*,*,#48399,.F.);
#63935=ORIENTED_EDGE('',*,*,#48395,.F.);
#63936=ORIENTED_EDGE('',*,*,#48400,.T.);
#63937=ORIENTED_EDGE('',*,*,#48393,.T.);
#63938=ORIENTED_EDGE('',*,*,#48401,.F.);
#63939=ORIENTED_EDGE('',*,*,#48398,.F.);
#63940=ORIENTED_EDGE('',*,*,#48402,.T.);
#63941=ORIENTED_EDGE('',*,*,#48403,.T.);
#63942=ORIENTED_EDGE('',*,*,#48404,.F.);
#63943=ORIENTED_EDGE('',*,*,#48405,.F.);
#63944=ORIENTED_EDGE('',*,*,#48406,.T.);
#63945=ORIENTED_EDGE('',*,*,#48407,.T.);
#63946=ORIENTED_EDGE('',*,*,#48408,.F.);
#63947=ORIENTED_EDGE('',*,*,#48403,.F.);
#63948=ORIENTED_EDGE('',*,*,#48409,.T.);
#63949=ORIENTED_EDGE('',*,*,#48410,.T.);
#63950=ORIENTED_EDGE('',*,*,#48411,.F.);
#63951=ORIENTED_EDGE('',*,*,#48407,.F.);
#63952=ORIENTED_EDGE('',*,*,#48412,.T.);
#63953=ORIENTED_EDGE('',*,*,#48405,.T.);
#63954=ORIENTED_EDGE('',*,*,#48413,.F.);
#63955=ORIENTED_EDGE('',*,*,#48410,.F.);
#63956=ORIENTED_EDGE('',*,*,#48414,.T.);
#63957=ORIENTED_EDGE('',*,*,#48415,.T.);
#63958=ORIENTED_EDGE('',*,*,#48416,.F.);
#63959=ORIENTED_EDGE('',*,*,#48417,.F.);
#63960=ORIENTED_EDGE('',*,*,#48418,.T.);
#63961=ORIENTED_EDGE('',*,*,#48419,.T.);
#63962=ORIENTED_EDGE('',*,*,#48420,.F.);
#63963=ORIENTED_EDGE('',*,*,#48415,.F.);
#63964=ORIENTED_EDGE('',*,*,#48421,.T.);
#63965=ORIENTED_EDGE('',*,*,#48422,.T.);
#63966=ORIENTED_EDGE('',*,*,#48423,.F.);
#63967=ORIENTED_EDGE('',*,*,#48419,.F.);
#63968=ORIENTED_EDGE('',*,*,#48424,.T.);
#63969=ORIENTED_EDGE('',*,*,#48417,.T.);
#63970=ORIENTED_EDGE('',*,*,#48425,.F.);
#63971=ORIENTED_EDGE('',*,*,#48422,.F.);
#63972=ORIENTED_EDGE('',*,*,#48426,.T.);
#63973=ORIENTED_EDGE('',*,*,#48427,.T.);
#63974=ORIENTED_EDGE('',*,*,#48428,.F.);
#63975=ORIENTED_EDGE('',*,*,#48429,.F.);
#63976=ORIENTED_EDGE('',*,*,#48430,.T.);
#63977=ORIENTED_EDGE('',*,*,#48431,.T.);
#63978=ORIENTED_EDGE('',*,*,#48432,.F.);
#63979=ORIENTED_EDGE('',*,*,#48427,.F.);
#63980=ORIENTED_EDGE('',*,*,#48433,.T.);
#63981=ORIENTED_EDGE('',*,*,#48434,.T.);
#63982=ORIENTED_EDGE('',*,*,#48435,.F.);
#63983=ORIENTED_EDGE('',*,*,#48431,.F.);
#63984=ORIENTED_EDGE('',*,*,#48436,.T.);
#63985=ORIENTED_EDGE('',*,*,#48429,.T.);
#63986=ORIENTED_EDGE('',*,*,#48437,.F.);
#63987=ORIENTED_EDGE('',*,*,#48434,.F.);
#63988=ORIENTED_EDGE('',*,*,#48438,.T.);
#63989=ORIENTED_EDGE('',*,*,#48439,.T.);
#63990=ORIENTED_EDGE('',*,*,#48440,.F.);
#63991=ORIENTED_EDGE('',*,*,#48441,.F.);
#63992=ORIENTED_EDGE('',*,*,#48442,.T.);
#63993=ORIENTED_EDGE('',*,*,#48443,.T.);
#63994=ORIENTED_EDGE('',*,*,#48444,.F.);
#63995=ORIENTED_EDGE('',*,*,#48439,.F.);
#63996=ORIENTED_EDGE('',*,*,#48445,.T.);
#63997=ORIENTED_EDGE('',*,*,#48446,.T.);
#63998=ORIENTED_EDGE('',*,*,#48447,.F.);
#63999=ORIENTED_EDGE('',*,*,#48443,.F.);
#64000=ORIENTED_EDGE('',*,*,#48448,.T.);
#64001=ORIENTED_EDGE('',*,*,#48441,.T.);
#64002=ORIENTED_EDGE('',*,*,#48449,.F.);
#64003=ORIENTED_EDGE('',*,*,#48446,.F.);
#64004=ORIENTED_EDGE('',*,*,#48450,.T.);
#64005=ORIENTED_EDGE('',*,*,#48451,.T.);
#64006=ORIENTED_EDGE('',*,*,#48452,.F.);
#64007=ORIENTED_EDGE('',*,*,#48453,.F.);
#64008=ORIENTED_EDGE('',*,*,#48454,.T.);
#64009=ORIENTED_EDGE('',*,*,#48455,.T.);
#64010=ORIENTED_EDGE('',*,*,#48456,.F.);
#64011=ORIENTED_EDGE('',*,*,#48451,.F.);
#64012=ORIENTED_EDGE('',*,*,#48457,.T.);
#64013=ORIENTED_EDGE('',*,*,#48458,.T.);
#64014=ORIENTED_EDGE('',*,*,#48459,.F.);
#64015=ORIENTED_EDGE('',*,*,#48455,.F.);
#64016=ORIENTED_EDGE('',*,*,#48460,.T.);
#64017=ORIENTED_EDGE('',*,*,#48453,.T.);
#64018=ORIENTED_EDGE('',*,*,#48461,.F.);
#64019=ORIENTED_EDGE('',*,*,#48458,.F.);
#64020=ORIENTED_EDGE('',*,*,#48462,.T.);
#64021=ORIENTED_EDGE('',*,*,#48463,.T.);
#64022=ORIENTED_EDGE('',*,*,#48464,.F.);
#64023=ORIENTED_EDGE('',*,*,#48465,.F.);
#64024=ORIENTED_EDGE('',*,*,#48466,.T.);
#64025=ORIENTED_EDGE('',*,*,#48467,.T.);
#64026=ORIENTED_EDGE('',*,*,#48468,.F.);
#64027=ORIENTED_EDGE('',*,*,#48463,.F.);
#64028=ORIENTED_EDGE('',*,*,#48469,.T.);
#64029=ORIENTED_EDGE('',*,*,#48470,.T.);
#64030=ORIENTED_EDGE('',*,*,#48471,.F.);
#64031=ORIENTED_EDGE('',*,*,#48467,.F.);
#64032=ORIENTED_EDGE('',*,*,#48472,.T.);
#64033=ORIENTED_EDGE('',*,*,#48465,.T.);
#64034=ORIENTED_EDGE('',*,*,#48473,.F.);
#64035=ORIENTED_EDGE('',*,*,#48470,.F.);
#64036=ORIENTED_EDGE('',*,*,#48474,.T.);
#64037=ORIENTED_EDGE('',*,*,#48475,.T.);
#64038=ORIENTED_EDGE('',*,*,#48476,.F.);
#64039=ORIENTED_EDGE('',*,*,#48477,.F.);
#64040=ORIENTED_EDGE('',*,*,#48478,.T.);
#64041=ORIENTED_EDGE('',*,*,#48479,.T.);
#64042=ORIENTED_EDGE('',*,*,#48480,.F.);
#64043=ORIENTED_EDGE('',*,*,#48475,.F.);
#64044=ORIENTED_EDGE('',*,*,#48481,.T.);
#64045=ORIENTED_EDGE('',*,*,#48482,.T.);
#64046=ORIENTED_EDGE('',*,*,#48483,.F.);
#64047=ORIENTED_EDGE('',*,*,#48479,.F.);
#64048=ORIENTED_EDGE('',*,*,#48484,.T.);
#64049=ORIENTED_EDGE('',*,*,#48477,.T.);
#64050=ORIENTED_EDGE('',*,*,#48485,.F.);
#64051=ORIENTED_EDGE('',*,*,#48482,.F.);
#64052=ORIENTED_EDGE('',*,*,#48486,.T.);
#64053=ORIENTED_EDGE('',*,*,#48487,.T.);
#64054=ORIENTED_EDGE('',*,*,#48488,.F.);
#64055=ORIENTED_EDGE('',*,*,#48489,.F.);
#64056=ORIENTED_EDGE('',*,*,#48490,.T.);
#64057=ORIENTED_EDGE('',*,*,#48491,.T.);
#64058=ORIENTED_EDGE('',*,*,#48492,.F.);
#64059=ORIENTED_EDGE('',*,*,#48487,.F.);
#64060=ORIENTED_EDGE('',*,*,#48493,.T.);
#64061=ORIENTED_EDGE('',*,*,#48494,.T.);
#64062=ORIENTED_EDGE('',*,*,#48495,.F.);
#64063=ORIENTED_EDGE('',*,*,#48491,.F.);
#64064=ORIENTED_EDGE('',*,*,#48496,.T.);
#64065=ORIENTED_EDGE('',*,*,#48489,.T.);
#64066=ORIENTED_EDGE('',*,*,#48497,.F.);
#64067=ORIENTED_EDGE('',*,*,#48494,.F.);
#64068=ORIENTED_EDGE('',*,*,#48498,.T.);
#64069=ORIENTED_EDGE('',*,*,#48499,.T.);
#64070=ORIENTED_EDGE('',*,*,#48500,.F.);
#64071=ORIENTED_EDGE('',*,*,#48501,.F.);
#64072=ORIENTED_EDGE('',*,*,#48502,.T.);
#64073=ORIENTED_EDGE('',*,*,#48503,.T.);
#64074=ORIENTED_EDGE('',*,*,#48504,.F.);
#64075=ORIENTED_EDGE('',*,*,#48499,.F.);
#64076=ORIENTED_EDGE('',*,*,#48505,.T.);
#64077=ORIENTED_EDGE('',*,*,#48506,.T.);
#64078=ORIENTED_EDGE('',*,*,#48507,.F.);
#64079=ORIENTED_EDGE('',*,*,#48503,.F.);
#64080=ORIENTED_EDGE('',*,*,#48508,.T.);
#64081=ORIENTED_EDGE('',*,*,#48501,.T.);
#64082=ORIENTED_EDGE('',*,*,#48509,.F.);
#64083=ORIENTED_EDGE('',*,*,#48506,.F.);
#64084=ORIENTED_EDGE('',*,*,#48510,.T.);
#64085=ORIENTED_EDGE('',*,*,#48511,.T.);
#64086=ORIENTED_EDGE('',*,*,#48512,.F.);
#64087=ORIENTED_EDGE('',*,*,#48513,.F.);
#64088=ORIENTED_EDGE('',*,*,#48514,.T.);
#64089=ORIENTED_EDGE('',*,*,#48515,.T.);
#64090=ORIENTED_EDGE('',*,*,#48516,.F.);
#64091=ORIENTED_EDGE('',*,*,#48511,.F.);
#64092=ORIENTED_EDGE('',*,*,#48517,.T.);
#64093=ORIENTED_EDGE('',*,*,#48518,.T.);
#64094=ORIENTED_EDGE('',*,*,#48519,.F.);
#64095=ORIENTED_EDGE('',*,*,#48515,.F.);
#64096=ORIENTED_EDGE('',*,*,#48520,.T.);
#64097=ORIENTED_EDGE('',*,*,#48513,.T.);
#64098=ORIENTED_EDGE('',*,*,#48521,.F.);
#64099=ORIENTED_EDGE('',*,*,#48518,.F.);
#64100=ORIENTED_EDGE('',*,*,#48522,.T.);
#64101=ORIENTED_EDGE('',*,*,#48523,.T.);
#64102=ORIENTED_EDGE('',*,*,#48524,.F.);
#64103=ORIENTED_EDGE('',*,*,#48525,.F.);
#64104=ORIENTED_EDGE('',*,*,#48526,.T.);
#64105=ORIENTED_EDGE('',*,*,#48527,.T.);
#64106=ORIENTED_EDGE('',*,*,#48528,.F.);
#64107=ORIENTED_EDGE('',*,*,#48523,.F.);
#64108=ORIENTED_EDGE('',*,*,#48529,.T.);
#64109=ORIENTED_EDGE('',*,*,#48530,.T.);
#64110=ORIENTED_EDGE('',*,*,#48531,.F.);
#64111=ORIENTED_EDGE('',*,*,#48527,.F.);
#64112=ORIENTED_EDGE('',*,*,#48532,.T.);
#64113=ORIENTED_EDGE('',*,*,#48525,.T.);
#64114=ORIENTED_EDGE('',*,*,#48533,.F.);
#64115=ORIENTED_EDGE('',*,*,#48530,.F.);
#64116=ORIENTED_EDGE('',*,*,#48534,.T.);
#64117=ORIENTED_EDGE('',*,*,#48535,.T.);
#64118=ORIENTED_EDGE('',*,*,#48536,.F.);
#64119=ORIENTED_EDGE('',*,*,#48537,.F.);
#64120=ORIENTED_EDGE('',*,*,#48538,.T.);
#64121=ORIENTED_EDGE('',*,*,#48539,.T.);
#64122=ORIENTED_EDGE('',*,*,#48540,.F.);
#64123=ORIENTED_EDGE('',*,*,#48535,.F.);
#64124=ORIENTED_EDGE('',*,*,#48541,.T.);
#64125=ORIENTED_EDGE('',*,*,#48542,.T.);
#64126=ORIENTED_EDGE('',*,*,#48543,.F.);
#64127=ORIENTED_EDGE('',*,*,#48539,.F.);
#64128=ORIENTED_EDGE('',*,*,#48544,.T.);
#64129=ORIENTED_EDGE('',*,*,#48537,.T.);
#64130=ORIENTED_EDGE('',*,*,#48545,.F.);
#64131=ORIENTED_EDGE('',*,*,#48542,.F.);
#64132=ORIENTED_EDGE('',*,*,#48546,.T.);
#64133=ORIENTED_EDGE('',*,*,#48547,.T.);
#64134=ORIENTED_EDGE('',*,*,#48548,.F.);
#64135=ORIENTED_EDGE('',*,*,#48549,.F.);
#64136=ORIENTED_EDGE('',*,*,#48550,.T.);
#64137=ORIENTED_EDGE('',*,*,#48551,.T.);
#64138=ORIENTED_EDGE('',*,*,#48552,.F.);
#64139=ORIENTED_EDGE('',*,*,#48547,.F.);
#64140=ORIENTED_EDGE('',*,*,#48553,.T.);
#64141=ORIENTED_EDGE('',*,*,#48554,.T.);
#64142=ORIENTED_EDGE('',*,*,#48555,.F.);
#64143=ORIENTED_EDGE('',*,*,#48551,.F.);
#64144=ORIENTED_EDGE('',*,*,#48556,.T.);
#64145=ORIENTED_EDGE('',*,*,#48549,.T.);
#64146=ORIENTED_EDGE('',*,*,#48557,.F.);
#64147=ORIENTED_EDGE('',*,*,#48554,.F.);
#64148=ORIENTED_EDGE('',*,*,#48558,.T.);
#64149=ORIENTED_EDGE('',*,*,#48559,.T.);
#64150=ORIENTED_EDGE('',*,*,#48560,.F.);
#64151=ORIENTED_EDGE('',*,*,#48561,.F.);
#64152=ORIENTED_EDGE('',*,*,#48562,.T.);
#64153=ORIENTED_EDGE('',*,*,#48563,.T.);
#64154=ORIENTED_EDGE('',*,*,#48564,.F.);
#64155=ORIENTED_EDGE('',*,*,#48559,.F.);
#64156=ORIENTED_EDGE('',*,*,#48565,.T.);
#64157=ORIENTED_EDGE('',*,*,#48566,.T.);
#64158=ORIENTED_EDGE('',*,*,#48567,.F.);
#64159=ORIENTED_EDGE('',*,*,#48563,.F.);
#64160=ORIENTED_EDGE('',*,*,#48568,.T.);
#64161=ORIENTED_EDGE('',*,*,#48561,.T.);
#64162=ORIENTED_EDGE('',*,*,#48569,.F.);
#64163=ORIENTED_EDGE('',*,*,#48566,.F.);
#64164=ORIENTED_EDGE('',*,*,#48570,.T.);
#64165=ORIENTED_EDGE('',*,*,#48571,.T.);
#64166=ORIENTED_EDGE('',*,*,#48572,.F.);
#64167=ORIENTED_EDGE('',*,*,#48573,.F.);
#64168=ORIENTED_EDGE('',*,*,#48574,.T.);
#64169=ORIENTED_EDGE('',*,*,#48575,.T.);
#64170=ORIENTED_EDGE('',*,*,#48576,.F.);
#64171=ORIENTED_EDGE('',*,*,#48571,.F.);
#64172=ORIENTED_EDGE('',*,*,#48577,.T.);
#64173=ORIENTED_EDGE('',*,*,#48578,.T.);
#64174=ORIENTED_EDGE('',*,*,#48579,.F.);
#64175=ORIENTED_EDGE('',*,*,#48575,.F.);
#64176=ORIENTED_EDGE('',*,*,#48580,.T.);
#64177=ORIENTED_EDGE('',*,*,#48573,.T.);
#64178=ORIENTED_EDGE('',*,*,#48581,.F.);
#64179=ORIENTED_EDGE('',*,*,#48578,.F.);
#64180=ORIENTED_EDGE('',*,*,#48582,.T.);
#64181=ORIENTED_EDGE('',*,*,#48583,.T.);
#64182=ORIENTED_EDGE('',*,*,#48584,.F.);
#64183=ORIENTED_EDGE('',*,*,#48585,.F.);
#64184=ORIENTED_EDGE('',*,*,#48586,.T.);
#64185=ORIENTED_EDGE('',*,*,#48587,.T.);
#64186=ORIENTED_EDGE('',*,*,#48588,.F.);
#64187=ORIENTED_EDGE('',*,*,#48583,.F.);
#64188=ORIENTED_EDGE('',*,*,#48589,.T.);
#64189=ORIENTED_EDGE('',*,*,#48590,.T.);
#64190=ORIENTED_EDGE('',*,*,#48591,.F.);
#64191=ORIENTED_EDGE('',*,*,#48587,.F.);
#64192=ORIENTED_EDGE('',*,*,#48592,.T.);
#64193=ORIENTED_EDGE('',*,*,#48585,.T.);
#64194=ORIENTED_EDGE('',*,*,#48593,.F.);
#64195=ORIENTED_EDGE('',*,*,#48590,.F.);
#64196=ORIENTED_EDGE('',*,*,#48594,.T.);
#64197=ORIENTED_EDGE('',*,*,#48595,.T.);
#64198=ORIENTED_EDGE('',*,*,#48596,.F.);
#64199=ORIENTED_EDGE('',*,*,#48597,.F.);
#64200=ORIENTED_EDGE('',*,*,#48598,.T.);
#64201=ORIENTED_EDGE('',*,*,#48599,.T.);
#64202=ORIENTED_EDGE('',*,*,#48600,.F.);
#64203=ORIENTED_EDGE('',*,*,#48595,.F.);
#64204=ORIENTED_EDGE('',*,*,#48601,.T.);
#64205=ORIENTED_EDGE('',*,*,#48602,.T.);
#64206=ORIENTED_EDGE('',*,*,#48603,.F.);
#64207=ORIENTED_EDGE('',*,*,#48599,.F.);
#64208=ORIENTED_EDGE('',*,*,#48604,.T.);
#64209=ORIENTED_EDGE('',*,*,#48597,.T.);
#64210=ORIENTED_EDGE('',*,*,#48605,.F.);
#64211=ORIENTED_EDGE('',*,*,#48602,.F.);
#64212=ORIENTED_EDGE('',*,*,#48606,.T.);
#64213=ORIENTED_EDGE('',*,*,#48607,.T.);
#64214=ORIENTED_EDGE('',*,*,#48608,.F.);
#64215=ORIENTED_EDGE('',*,*,#48609,.F.);
#64216=ORIENTED_EDGE('',*,*,#48610,.T.);
#64217=ORIENTED_EDGE('',*,*,#48611,.T.);
#64218=ORIENTED_EDGE('',*,*,#48612,.F.);
#64219=ORIENTED_EDGE('',*,*,#48607,.F.);
#64220=ORIENTED_EDGE('',*,*,#48613,.T.);
#64221=ORIENTED_EDGE('',*,*,#48614,.T.);
#64222=ORIENTED_EDGE('',*,*,#48615,.F.);
#64223=ORIENTED_EDGE('',*,*,#48611,.F.);
#64224=ORIENTED_EDGE('',*,*,#48616,.T.);
#64225=ORIENTED_EDGE('',*,*,#48609,.T.);
#64226=ORIENTED_EDGE('',*,*,#48617,.F.);
#64227=ORIENTED_EDGE('',*,*,#48614,.F.);
#64228=ORIENTED_EDGE('',*,*,#48618,.T.);
#64229=ORIENTED_EDGE('',*,*,#48619,.T.);
#64230=ORIENTED_EDGE('',*,*,#48620,.F.);
#64231=ORIENTED_EDGE('',*,*,#48621,.F.);
#64232=ORIENTED_EDGE('',*,*,#48622,.T.);
#64233=ORIENTED_EDGE('',*,*,#48623,.T.);
#64234=ORIENTED_EDGE('',*,*,#48624,.F.);
#64235=ORIENTED_EDGE('',*,*,#48619,.F.);
#64236=ORIENTED_EDGE('',*,*,#48625,.T.);
#64237=ORIENTED_EDGE('',*,*,#48626,.T.);
#64238=ORIENTED_EDGE('',*,*,#48627,.F.);
#64239=ORIENTED_EDGE('',*,*,#48623,.F.);
#64240=ORIENTED_EDGE('',*,*,#48628,.T.);
#64241=ORIENTED_EDGE('',*,*,#48621,.T.);
#64242=ORIENTED_EDGE('',*,*,#48629,.F.);
#64243=ORIENTED_EDGE('',*,*,#48626,.F.);
#64244=ORIENTED_EDGE('',*,*,#48630,.T.);
#64245=ORIENTED_EDGE('',*,*,#48631,.T.);
#64246=ORIENTED_EDGE('',*,*,#48632,.F.);
#64247=ORIENTED_EDGE('',*,*,#48633,.F.);
#64248=ORIENTED_EDGE('',*,*,#48634,.T.);
#64249=ORIENTED_EDGE('',*,*,#48635,.T.);
#64250=ORIENTED_EDGE('',*,*,#48636,.F.);
#64251=ORIENTED_EDGE('',*,*,#48631,.F.);
#64252=ORIENTED_EDGE('',*,*,#48637,.T.);
#64253=ORIENTED_EDGE('',*,*,#48638,.T.);
#64254=ORIENTED_EDGE('',*,*,#48639,.F.);
#64255=ORIENTED_EDGE('',*,*,#48635,.F.);
#64256=ORIENTED_EDGE('',*,*,#48640,.T.);
#64257=ORIENTED_EDGE('',*,*,#48633,.T.);
#64258=ORIENTED_EDGE('',*,*,#48641,.F.);
#64259=ORIENTED_EDGE('',*,*,#48638,.F.);
#64260=ORIENTED_EDGE('',*,*,#48642,.T.);
#64261=ORIENTED_EDGE('',*,*,#48643,.T.);
#64262=ORIENTED_EDGE('',*,*,#48644,.F.);
#64263=ORIENTED_EDGE('',*,*,#48645,.F.);
#64264=ORIENTED_EDGE('',*,*,#48646,.T.);
#64265=ORIENTED_EDGE('',*,*,#48647,.T.);
#64266=ORIENTED_EDGE('',*,*,#48648,.F.);
#64267=ORIENTED_EDGE('',*,*,#48643,.F.);
#64268=ORIENTED_EDGE('',*,*,#48649,.T.);
#64269=ORIENTED_EDGE('',*,*,#48650,.T.);
#64270=ORIENTED_EDGE('',*,*,#48651,.F.);
#64271=ORIENTED_EDGE('',*,*,#48647,.F.);
#64272=ORIENTED_EDGE('',*,*,#48652,.T.);
#64273=ORIENTED_EDGE('',*,*,#48645,.T.);
#64274=ORIENTED_EDGE('',*,*,#48653,.F.);
#64275=ORIENTED_EDGE('',*,*,#48650,.F.);
#64276=ORIENTED_EDGE('',*,*,#48654,.T.);
#64277=ORIENTED_EDGE('',*,*,#48655,.T.);
#64278=ORIENTED_EDGE('',*,*,#48656,.F.);
#64279=ORIENTED_EDGE('',*,*,#48657,.F.);
#64280=ORIENTED_EDGE('',*,*,#48658,.T.);
#64281=ORIENTED_EDGE('',*,*,#48659,.T.);
#64282=ORIENTED_EDGE('',*,*,#48660,.F.);
#64283=ORIENTED_EDGE('',*,*,#48655,.F.);
#64284=ORIENTED_EDGE('',*,*,#48661,.T.);
#64285=ORIENTED_EDGE('',*,*,#48662,.T.);
#64286=ORIENTED_EDGE('',*,*,#48663,.F.);
#64287=ORIENTED_EDGE('',*,*,#48659,.F.);
#64288=ORIENTED_EDGE('',*,*,#48664,.T.);
#64289=ORIENTED_EDGE('',*,*,#48657,.T.);
#64290=ORIENTED_EDGE('',*,*,#48665,.F.);
#64291=ORIENTED_EDGE('',*,*,#48662,.F.);
#64292=ORIENTED_EDGE('',*,*,#48666,.T.);
#64293=ORIENTED_EDGE('',*,*,#48667,.T.);
#64294=ORIENTED_EDGE('',*,*,#48668,.F.);
#64295=ORIENTED_EDGE('',*,*,#48669,.F.);
#64296=ORIENTED_EDGE('',*,*,#48670,.T.);
#64297=ORIENTED_EDGE('',*,*,#48671,.T.);
#64298=ORIENTED_EDGE('',*,*,#48672,.F.);
#64299=ORIENTED_EDGE('',*,*,#48667,.F.);
#64300=ORIENTED_EDGE('',*,*,#48673,.T.);
#64301=ORIENTED_EDGE('',*,*,#48674,.T.);
#64302=ORIENTED_EDGE('',*,*,#48675,.F.);
#64303=ORIENTED_EDGE('',*,*,#48671,.F.);
#64304=ORIENTED_EDGE('',*,*,#48676,.T.);
#64305=ORIENTED_EDGE('',*,*,#48669,.T.);
#64306=ORIENTED_EDGE('',*,*,#48677,.F.);
#64307=ORIENTED_EDGE('',*,*,#48674,.F.);
#64308=ORIENTED_EDGE('',*,*,#48678,.T.);
#64309=ORIENTED_EDGE('',*,*,#48679,.T.);
#64310=ORIENTED_EDGE('',*,*,#48680,.F.);
#64311=ORIENTED_EDGE('',*,*,#48681,.F.);
#64312=ORIENTED_EDGE('',*,*,#48682,.T.);
#64313=ORIENTED_EDGE('',*,*,#48683,.T.);
#64314=ORIENTED_EDGE('',*,*,#48684,.F.);
#64315=ORIENTED_EDGE('',*,*,#48679,.F.);
#64316=ORIENTED_EDGE('',*,*,#48685,.T.);
#64317=ORIENTED_EDGE('',*,*,#48686,.T.);
#64318=ORIENTED_EDGE('',*,*,#48687,.F.);
#64319=ORIENTED_EDGE('',*,*,#48683,.F.);
#64320=ORIENTED_EDGE('',*,*,#48688,.T.);
#64321=ORIENTED_EDGE('',*,*,#48681,.T.);
#64322=ORIENTED_EDGE('',*,*,#48689,.F.);
#64323=ORIENTED_EDGE('',*,*,#48686,.F.);
#64324=ORIENTED_EDGE('',*,*,#48690,.T.);
#64325=ORIENTED_EDGE('',*,*,#48691,.T.);
#64326=ORIENTED_EDGE('',*,*,#48692,.F.);
#64327=ORIENTED_EDGE('',*,*,#48693,.F.);
#64328=ORIENTED_EDGE('',*,*,#48694,.T.);
#64329=ORIENTED_EDGE('',*,*,#48695,.T.);
#64330=ORIENTED_EDGE('',*,*,#48696,.F.);
#64331=ORIENTED_EDGE('',*,*,#48691,.F.);
#64332=ORIENTED_EDGE('',*,*,#48697,.T.);
#64333=ORIENTED_EDGE('',*,*,#48698,.T.);
#64334=ORIENTED_EDGE('',*,*,#48699,.F.);
#64335=ORIENTED_EDGE('',*,*,#48695,.F.);
#64336=ORIENTED_EDGE('',*,*,#48700,.T.);
#64337=ORIENTED_EDGE('',*,*,#48693,.T.);
#64338=ORIENTED_EDGE('',*,*,#48701,.F.);
#64339=ORIENTED_EDGE('',*,*,#48698,.F.);
#64340=ORIENTED_EDGE('',*,*,#48702,.T.);
#64341=ORIENTED_EDGE('',*,*,#48703,.T.);
#64342=ORIENTED_EDGE('',*,*,#48704,.F.);
#64343=ORIENTED_EDGE('',*,*,#48705,.F.);
#64344=ORIENTED_EDGE('',*,*,#48706,.T.);
#64345=ORIENTED_EDGE('',*,*,#48707,.T.);
#64346=ORIENTED_EDGE('',*,*,#48708,.F.);
#64347=ORIENTED_EDGE('',*,*,#48703,.F.);
#64348=ORIENTED_EDGE('',*,*,#48709,.T.);
#64349=ORIENTED_EDGE('',*,*,#48710,.T.);
#64350=ORIENTED_EDGE('',*,*,#48711,.F.);
#64351=ORIENTED_EDGE('',*,*,#48707,.F.);
#64352=ORIENTED_EDGE('',*,*,#48712,.T.);
#64353=ORIENTED_EDGE('',*,*,#48705,.T.);
#64354=ORIENTED_EDGE('',*,*,#48713,.F.);
#64355=ORIENTED_EDGE('',*,*,#48710,.F.);
#64356=ORIENTED_EDGE('',*,*,#48714,.T.);
#64357=ORIENTED_EDGE('',*,*,#48715,.T.);
#64358=ORIENTED_EDGE('',*,*,#48716,.F.);
#64359=ORIENTED_EDGE('',*,*,#48717,.F.);
#64360=ORIENTED_EDGE('',*,*,#48718,.T.);
#64361=ORIENTED_EDGE('',*,*,#48719,.T.);
#64362=ORIENTED_EDGE('',*,*,#48720,.F.);
#64363=ORIENTED_EDGE('',*,*,#48715,.F.);
#64364=ORIENTED_EDGE('',*,*,#48721,.T.);
#64365=ORIENTED_EDGE('',*,*,#48722,.T.);
#64366=ORIENTED_EDGE('',*,*,#48723,.F.);
#64367=ORIENTED_EDGE('',*,*,#48719,.F.);
#64368=ORIENTED_EDGE('',*,*,#48724,.T.);
#64369=ORIENTED_EDGE('',*,*,#48717,.T.);
#64370=ORIENTED_EDGE('',*,*,#48725,.F.);
#64371=ORIENTED_EDGE('',*,*,#48722,.F.);
#64372=ORIENTED_EDGE('',*,*,#48726,.T.);
#64373=ORIENTED_EDGE('',*,*,#48727,.T.);
#64374=ORIENTED_EDGE('',*,*,#48728,.F.);
#64375=ORIENTED_EDGE('',*,*,#48729,.F.);
#64376=ORIENTED_EDGE('',*,*,#48730,.T.);
#64377=ORIENTED_EDGE('',*,*,#48731,.T.);
#64378=ORIENTED_EDGE('',*,*,#48732,.F.);
#64379=ORIENTED_EDGE('',*,*,#48727,.F.);
#64380=ORIENTED_EDGE('',*,*,#48733,.T.);
#64381=ORIENTED_EDGE('',*,*,#48734,.T.);
#64382=ORIENTED_EDGE('',*,*,#48735,.F.);
#64383=ORIENTED_EDGE('',*,*,#48731,.F.);
#64384=ORIENTED_EDGE('',*,*,#48736,.T.);
#64385=ORIENTED_EDGE('',*,*,#48729,.T.);
#64386=ORIENTED_EDGE('',*,*,#48737,.F.);
#64387=ORIENTED_EDGE('',*,*,#48734,.F.);
#64388=ORIENTED_EDGE('',*,*,#48738,.T.);
#64389=ORIENTED_EDGE('',*,*,#48739,.T.);
#64390=ORIENTED_EDGE('',*,*,#48740,.F.);
#64391=ORIENTED_EDGE('',*,*,#48741,.F.);
#64392=ORIENTED_EDGE('',*,*,#48742,.T.);
#64393=ORIENTED_EDGE('',*,*,#48743,.T.);
#64394=ORIENTED_EDGE('',*,*,#48744,.F.);
#64395=ORIENTED_EDGE('',*,*,#48739,.F.);
#64396=ORIENTED_EDGE('',*,*,#48745,.T.);
#64397=ORIENTED_EDGE('',*,*,#48746,.T.);
#64398=ORIENTED_EDGE('',*,*,#48747,.F.);
#64399=ORIENTED_EDGE('',*,*,#48743,.F.);
#64400=ORIENTED_EDGE('',*,*,#48748,.T.);
#64401=ORIENTED_EDGE('',*,*,#48741,.T.);
#64402=ORIENTED_EDGE('',*,*,#48749,.F.);
#64403=ORIENTED_EDGE('',*,*,#48746,.F.);
#64404=ORIENTED_EDGE('',*,*,#48750,.T.);
#64405=ORIENTED_EDGE('',*,*,#48751,.T.);
#64406=ORIENTED_EDGE('',*,*,#48752,.F.);
#64407=ORIENTED_EDGE('',*,*,#48753,.F.);
#64408=ORIENTED_EDGE('',*,*,#48754,.T.);
#64409=ORIENTED_EDGE('',*,*,#48755,.T.);
#64410=ORIENTED_EDGE('',*,*,#48756,.F.);
#64411=ORIENTED_EDGE('',*,*,#48751,.F.);
#64412=ORIENTED_EDGE('',*,*,#48757,.T.);
#64413=ORIENTED_EDGE('',*,*,#48758,.T.);
#64414=ORIENTED_EDGE('',*,*,#48759,.F.);
#64415=ORIENTED_EDGE('',*,*,#48755,.F.);
#64416=ORIENTED_EDGE('',*,*,#48760,.T.);
#64417=ORIENTED_EDGE('',*,*,#48753,.T.);
#64418=ORIENTED_EDGE('',*,*,#48761,.F.);
#64419=ORIENTED_EDGE('',*,*,#48758,.F.);
#64420=ORIENTED_EDGE('',*,*,#48762,.T.);
#64421=ORIENTED_EDGE('',*,*,#48763,.T.);
#64422=ORIENTED_EDGE('',*,*,#48764,.F.);
#64423=ORIENTED_EDGE('',*,*,#48765,.F.);
#64424=ORIENTED_EDGE('',*,*,#48766,.T.);
#64425=ORIENTED_EDGE('',*,*,#48767,.T.);
#64426=ORIENTED_EDGE('',*,*,#48768,.F.);
#64427=ORIENTED_EDGE('',*,*,#48763,.F.);
#64428=ORIENTED_EDGE('',*,*,#48769,.T.);
#64429=ORIENTED_EDGE('',*,*,#48770,.T.);
#64430=ORIENTED_EDGE('',*,*,#48771,.F.);
#64431=ORIENTED_EDGE('',*,*,#48767,.F.);
#64432=ORIENTED_EDGE('',*,*,#48772,.T.);
#64433=ORIENTED_EDGE('',*,*,#48765,.T.);
#64434=ORIENTED_EDGE('',*,*,#48773,.F.);
#64435=ORIENTED_EDGE('',*,*,#48770,.F.);
#64436=ORIENTED_EDGE('',*,*,#48774,.T.);
#64437=ORIENTED_EDGE('',*,*,#48775,.T.);
#64438=ORIENTED_EDGE('',*,*,#48776,.F.);
#64439=ORIENTED_EDGE('',*,*,#48777,.F.);
#64440=ORIENTED_EDGE('',*,*,#48778,.T.);
#64441=ORIENTED_EDGE('',*,*,#48779,.T.);
#64442=ORIENTED_EDGE('',*,*,#48780,.F.);
#64443=ORIENTED_EDGE('',*,*,#48775,.F.);
#64444=ORIENTED_EDGE('',*,*,#48781,.T.);
#64445=ORIENTED_EDGE('',*,*,#48782,.T.);
#64446=ORIENTED_EDGE('',*,*,#48783,.F.);
#64447=ORIENTED_EDGE('',*,*,#48779,.F.);
#64448=ORIENTED_EDGE('',*,*,#48784,.T.);
#64449=ORIENTED_EDGE('',*,*,#48777,.T.);
#64450=ORIENTED_EDGE('',*,*,#48785,.F.);
#64451=ORIENTED_EDGE('',*,*,#48782,.F.);
#64452=ORIENTED_EDGE('',*,*,#48786,.T.);
#64453=ORIENTED_EDGE('',*,*,#48787,.T.);
#64454=ORIENTED_EDGE('',*,*,#48788,.F.);
#64455=ORIENTED_EDGE('',*,*,#48789,.F.);
#64456=ORIENTED_EDGE('',*,*,#48790,.T.);
#64457=ORIENTED_EDGE('',*,*,#48791,.T.);
#64458=ORIENTED_EDGE('',*,*,#48792,.F.);
#64459=ORIENTED_EDGE('',*,*,#48787,.F.);
#64460=ORIENTED_EDGE('',*,*,#48793,.T.);
#64461=ORIENTED_EDGE('',*,*,#48794,.T.);
#64462=ORIENTED_EDGE('',*,*,#48795,.F.);
#64463=ORIENTED_EDGE('',*,*,#48791,.F.);
#64464=ORIENTED_EDGE('',*,*,#48796,.T.);
#64465=ORIENTED_EDGE('',*,*,#48789,.T.);
#64466=ORIENTED_EDGE('',*,*,#48797,.F.);
#64467=ORIENTED_EDGE('',*,*,#48794,.F.);
#64468=ORIENTED_EDGE('',*,*,#48798,.T.);
#64469=ORIENTED_EDGE('',*,*,#48799,.T.);
#64470=ORIENTED_EDGE('',*,*,#48800,.F.);
#64471=ORIENTED_EDGE('',*,*,#48801,.F.);
#64472=ORIENTED_EDGE('',*,*,#48802,.T.);
#64473=ORIENTED_EDGE('',*,*,#48803,.T.);
#64474=ORIENTED_EDGE('',*,*,#48804,.F.);
#64475=ORIENTED_EDGE('',*,*,#48799,.F.);
#64476=ORIENTED_EDGE('',*,*,#48805,.T.);
#64477=ORIENTED_EDGE('',*,*,#48806,.T.);
#64478=ORIENTED_EDGE('',*,*,#48807,.F.);
#64479=ORIENTED_EDGE('',*,*,#48803,.F.);
#64480=ORIENTED_EDGE('',*,*,#48808,.T.);
#64481=ORIENTED_EDGE('',*,*,#48801,.T.);
#64482=ORIENTED_EDGE('',*,*,#48809,.F.);
#64483=ORIENTED_EDGE('',*,*,#48806,.F.);
#64484=ORIENTED_EDGE('',*,*,#48810,.T.);
#64485=ORIENTED_EDGE('',*,*,#48811,.T.);
#64486=ORIENTED_EDGE('',*,*,#48812,.F.);
#64487=ORIENTED_EDGE('',*,*,#48813,.F.);
#64488=ORIENTED_EDGE('',*,*,#48814,.T.);
#64489=ORIENTED_EDGE('',*,*,#48815,.T.);
#64490=ORIENTED_EDGE('',*,*,#48816,.F.);
#64491=ORIENTED_EDGE('',*,*,#48811,.F.);
#64492=ORIENTED_EDGE('',*,*,#48817,.T.);
#64493=ORIENTED_EDGE('',*,*,#48818,.T.);
#64494=ORIENTED_EDGE('',*,*,#48819,.F.);
#64495=ORIENTED_EDGE('',*,*,#48815,.F.);
#64496=ORIENTED_EDGE('',*,*,#48820,.T.);
#64497=ORIENTED_EDGE('',*,*,#48813,.T.);
#64498=ORIENTED_EDGE('',*,*,#48821,.F.);
#64499=ORIENTED_EDGE('',*,*,#48818,.F.);
#64500=ORIENTED_EDGE('',*,*,#48822,.T.);
#64501=ORIENTED_EDGE('',*,*,#48823,.T.);
#64502=ORIENTED_EDGE('',*,*,#48824,.F.);
#64503=ORIENTED_EDGE('',*,*,#48825,.F.);
#64504=ORIENTED_EDGE('',*,*,#48826,.T.);
#64505=ORIENTED_EDGE('',*,*,#48827,.T.);
#64506=ORIENTED_EDGE('',*,*,#48828,.F.);
#64507=ORIENTED_EDGE('',*,*,#48823,.F.);
#64508=ORIENTED_EDGE('',*,*,#48829,.T.);
#64509=ORIENTED_EDGE('',*,*,#48830,.T.);
#64510=ORIENTED_EDGE('',*,*,#48831,.F.);
#64511=ORIENTED_EDGE('',*,*,#48827,.F.);
#64512=ORIENTED_EDGE('',*,*,#48832,.T.);
#64513=ORIENTED_EDGE('',*,*,#48825,.T.);
#64514=ORIENTED_EDGE('',*,*,#48833,.F.);
#64515=ORIENTED_EDGE('',*,*,#48830,.F.);
#64516=ORIENTED_EDGE('',*,*,#48834,.T.);
#64517=ORIENTED_EDGE('',*,*,#48835,.T.);
#64518=ORIENTED_EDGE('',*,*,#48836,.F.);
#64519=ORIENTED_EDGE('',*,*,#48837,.F.);
#64520=ORIENTED_EDGE('',*,*,#48838,.T.);
#64521=ORIENTED_EDGE('',*,*,#48839,.T.);
#64522=ORIENTED_EDGE('',*,*,#48840,.F.);
#64523=ORIENTED_EDGE('',*,*,#48835,.F.);
#64524=ORIENTED_EDGE('',*,*,#48841,.T.);
#64525=ORIENTED_EDGE('',*,*,#48842,.T.);
#64526=ORIENTED_EDGE('',*,*,#48843,.F.);
#64527=ORIENTED_EDGE('',*,*,#48839,.F.);
#64528=ORIENTED_EDGE('',*,*,#48844,.T.);
#64529=ORIENTED_EDGE('',*,*,#48837,.T.);
#64530=ORIENTED_EDGE('',*,*,#48845,.F.);
#64531=ORIENTED_EDGE('',*,*,#48842,.F.);
#64532=ORIENTED_EDGE('',*,*,#48846,.T.);
#64533=ORIENTED_EDGE('',*,*,#48847,.T.);
#64534=ORIENTED_EDGE('',*,*,#48848,.F.);
#64535=ORIENTED_EDGE('',*,*,#48849,.F.);
#64536=ORIENTED_EDGE('',*,*,#48850,.T.);
#64537=ORIENTED_EDGE('',*,*,#48851,.T.);
#64538=ORIENTED_EDGE('',*,*,#48852,.F.);
#64539=ORIENTED_EDGE('',*,*,#48847,.F.);
#64540=ORIENTED_EDGE('',*,*,#48853,.T.);
#64541=ORIENTED_EDGE('',*,*,#48854,.T.);
#64542=ORIENTED_EDGE('',*,*,#48855,.F.);
#64543=ORIENTED_EDGE('',*,*,#48851,.F.);
#64544=ORIENTED_EDGE('',*,*,#48856,.T.);
#64545=ORIENTED_EDGE('',*,*,#48849,.T.);
#64546=ORIENTED_EDGE('',*,*,#48857,.F.);
#64547=ORIENTED_EDGE('',*,*,#48854,.F.);
#64548=ORIENTED_EDGE('',*,*,#48858,.T.);
#64549=ORIENTED_EDGE('',*,*,#48859,.T.);
#64550=ORIENTED_EDGE('',*,*,#48860,.F.);
#64551=ORIENTED_EDGE('',*,*,#48861,.F.);
#64552=ORIENTED_EDGE('',*,*,#48862,.T.);
#64553=ORIENTED_EDGE('',*,*,#48863,.T.);
#64554=ORIENTED_EDGE('',*,*,#48864,.F.);
#64555=ORIENTED_EDGE('',*,*,#48859,.F.);
#64556=ORIENTED_EDGE('',*,*,#48865,.T.);
#64557=ORIENTED_EDGE('',*,*,#48866,.T.);
#64558=ORIENTED_EDGE('',*,*,#48867,.F.);
#64559=ORIENTED_EDGE('',*,*,#48863,.F.);
#64560=ORIENTED_EDGE('',*,*,#48868,.T.);
#64561=ORIENTED_EDGE('',*,*,#48861,.T.);
#64562=ORIENTED_EDGE('',*,*,#48869,.F.);
#64563=ORIENTED_EDGE('',*,*,#48866,.F.);
#64564=ORIENTED_EDGE('',*,*,#48870,.T.);
#64565=ORIENTED_EDGE('',*,*,#48871,.T.);
#64566=ORIENTED_EDGE('',*,*,#48872,.F.);
#64567=ORIENTED_EDGE('',*,*,#48873,.F.);
#64568=ORIENTED_EDGE('',*,*,#48874,.T.);
#64569=ORIENTED_EDGE('',*,*,#48875,.T.);
#64570=ORIENTED_EDGE('',*,*,#48876,.F.);
#64571=ORIENTED_EDGE('',*,*,#48871,.F.);
#64572=ORIENTED_EDGE('',*,*,#48877,.T.);
#64573=ORIENTED_EDGE('',*,*,#48878,.T.);
#64574=ORIENTED_EDGE('',*,*,#48879,.F.);
#64575=ORIENTED_EDGE('',*,*,#48875,.F.);
#64576=ORIENTED_EDGE('',*,*,#48880,.T.);
#64577=ORIENTED_EDGE('',*,*,#48873,.T.);
#64578=ORIENTED_EDGE('',*,*,#48881,.F.);
#64579=ORIENTED_EDGE('',*,*,#48878,.F.);
#64580=ORIENTED_EDGE('',*,*,#48882,.T.);
#64581=ORIENTED_EDGE('',*,*,#48883,.T.);
#64582=ORIENTED_EDGE('',*,*,#48884,.F.);
#64583=ORIENTED_EDGE('',*,*,#48885,.F.);
#64584=ORIENTED_EDGE('',*,*,#48886,.T.);
#64585=ORIENTED_EDGE('',*,*,#48887,.T.);
#64586=ORIENTED_EDGE('',*,*,#48888,.F.);
#64587=ORIENTED_EDGE('',*,*,#48883,.F.);
#64588=ORIENTED_EDGE('',*,*,#48889,.T.);
#64589=ORIENTED_EDGE('',*,*,#48890,.T.);
#64590=ORIENTED_EDGE('',*,*,#48891,.F.);
#64591=ORIENTED_EDGE('',*,*,#48887,.F.);
#64592=ORIENTED_EDGE('',*,*,#48892,.T.);
#64593=ORIENTED_EDGE('',*,*,#48885,.T.);
#64594=ORIENTED_EDGE('',*,*,#48893,.F.);
#64595=ORIENTED_EDGE('',*,*,#48890,.F.);
#64596=ORIENTED_EDGE('',*,*,#48894,.T.);
#64597=ORIENTED_EDGE('',*,*,#48895,.T.);
#64598=ORIENTED_EDGE('',*,*,#48896,.F.);
#64599=ORIENTED_EDGE('',*,*,#48897,.F.);
#64600=ORIENTED_EDGE('',*,*,#48898,.T.);
#64601=ORIENTED_EDGE('',*,*,#48899,.T.);
#64602=ORIENTED_EDGE('',*,*,#48900,.F.);
#64603=ORIENTED_EDGE('',*,*,#48895,.F.);
#64604=ORIENTED_EDGE('',*,*,#48901,.T.);
#64605=ORIENTED_EDGE('',*,*,#48902,.T.);
#64606=ORIENTED_EDGE('',*,*,#48903,.F.);
#64607=ORIENTED_EDGE('',*,*,#48899,.F.);
#64608=ORIENTED_EDGE('',*,*,#48904,.T.);
#64609=ORIENTED_EDGE('',*,*,#48897,.T.);
#64610=ORIENTED_EDGE('',*,*,#48905,.F.);
#64611=ORIENTED_EDGE('',*,*,#48902,.F.);
#64612=ORIENTED_EDGE('',*,*,#48906,.T.);
#64613=ORIENTED_EDGE('',*,*,#48907,.T.);
#64614=ORIENTED_EDGE('',*,*,#48908,.F.);
#64615=ORIENTED_EDGE('',*,*,#48909,.F.);
#64616=ORIENTED_EDGE('',*,*,#48910,.T.);
#64617=ORIENTED_EDGE('',*,*,#48911,.T.);
#64618=ORIENTED_EDGE('',*,*,#48912,.F.);
#64619=ORIENTED_EDGE('',*,*,#48907,.F.);
#64620=ORIENTED_EDGE('',*,*,#48913,.T.);
#64621=ORIENTED_EDGE('',*,*,#48914,.T.);
#64622=ORIENTED_EDGE('',*,*,#48915,.F.);
#64623=ORIENTED_EDGE('',*,*,#48911,.F.);
#64624=ORIENTED_EDGE('',*,*,#48916,.T.);
#64625=ORIENTED_EDGE('',*,*,#48909,.T.);
#64626=ORIENTED_EDGE('',*,*,#48917,.F.);
#64627=ORIENTED_EDGE('',*,*,#48914,.F.);
#64628=ORIENTED_EDGE('',*,*,#48918,.T.);
#64629=ORIENTED_EDGE('',*,*,#48919,.T.);
#64630=ORIENTED_EDGE('',*,*,#48920,.F.);
#64631=ORIENTED_EDGE('',*,*,#48921,.F.);
#64632=ORIENTED_EDGE('',*,*,#48922,.T.);
#64633=ORIENTED_EDGE('',*,*,#48923,.T.);
#64634=ORIENTED_EDGE('',*,*,#48924,.F.);
#64635=ORIENTED_EDGE('',*,*,#48919,.F.);
#64636=ORIENTED_EDGE('',*,*,#48925,.T.);
#64637=ORIENTED_EDGE('',*,*,#48926,.T.);
#64638=ORIENTED_EDGE('',*,*,#48927,.F.);
#64639=ORIENTED_EDGE('',*,*,#48923,.F.);
#64640=ORIENTED_EDGE('',*,*,#48928,.T.);
#64641=ORIENTED_EDGE('',*,*,#48921,.T.);
#64642=ORIENTED_EDGE('',*,*,#48929,.F.);
#64643=ORIENTED_EDGE('',*,*,#48926,.F.);
#64644=ORIENTED_EDGE('',*,*,#48930,.T.);
#64645=ORIENTED_EDGE('',*,*,#48931,.T.);
#64646=ORIENTED_EDGE('',*,*,#48932,.F.);
#64647=ORIENTED_EDGE('',*,*,#48933,.F.);
#64648=ORIENTED_EDGE('',*,*,#48934,.T.);
#64649=ORIENTED_EDGE('',*,*,#48935,.T.);
#64650=ORIENTED_EDGE('',*,*,#48936,.F.);
#64651=ORIENTED_EDGE('',*,*,#48931,.F.);
#64652=ORIENTED_EDGE('',*,*,#48937,.T.);
#64653=ORIENTED_EDGE('',*,*,#48938,.T.);
#64654=ORIENTED_EDGE('',*,*,#48939,.F.);
#64655=ORIENTED_EDGE('',*,*,#48935,.F.);
#64656=ORIENTED_EDGE('',*,*,#48940,.T.);
#64657=ORIENTED_EDGE('',*,*,#48933,.T.);
#64658=ORIENTED_EDGE('',*,*,#48941,.F.);
#64659=ORIENTED_EDGE('',*,*,#48938,.F.);
#64660=ORIENTED_EDGE('',*,*,#48942,.T.);
#64661=ORIENTED_EDGE('',*,*,#48943,.T.);
#64662=ORIENTED_EDGE('',*,*,#48944,.F.);
#64663=ORIENTED_EDGE('',*,*,#48945,.F.);
#64664=ORIENTED_EDGE('',*,*,#48946,.T.);
#64665=ORIENTED_EDGE('',*,*,#48947,.T.);
#64666=ORIENTED_EDGE('',*,*,#48948,.F.);
#64667=ORIENTED_EDGE('',*,*,#48943,.F.);
#64668=ORIENTED_EDGE('',*,*,#48949,.T.);
#64669=ORIENTED_EDGE('',*,*,#48950,.T.);
#64670=ORIENTED_EDGE('',*,*,#48951,.F.);
#64671=ORIENTED_EDGE('',*,*,#48947,.F.);
#64672=ORIENTED_EDGE('',*,*,#48952,.T.);
#64673=ORIENTED_EDGE('',*,*,#48945,.T.);
#64674=ORIENTED_EDGE('',*,*,#48953,.F.);
#64675=ORIENTED_EDGE('',*,*,#48950,.F.);
#64676=ORIENTED_EDGE('',*,*,#48954,.T.);
#64677=ORIENTED_EDGE('',*,*,#48955,.T.);
#64678=ORIENTED_EDGE('',*,*,#48956,.F.);
#64679=ORIENTED_EDGE('',*,*,#48957,.F.);
#64680=ORIENTED_EDGE('',*,*,#48958,.T.);
#64681=ORIENTED_EDGE('',*,*,#48959,.T.);
#64682=ORIENTED_EDGE('',*,*,#48960,.F.);
#64683=ORIENTED_EDGE('',*,*,#48955,.F.);
#64684=ORIENTED_EDGE('',*,*,#48961,.T.);
#64685=ORIENTED_EDGE('',*,*,#48962,.T.);
#64686=ORIENTED_EDGE('',*,*,#48963,.F.);
#64687=ORIENTED_EDGE('',*,*,#48959,.F.);
#64688=ORIENTED_EDGE('',*,*,#48964,.T.);
#64689=ORIENTED_EDGE('',*,*,#48957,.T.);
#64690=ORIENTED_EDGE('',*,*,#48965,.F.);
#64691=ORIENTED_EDGE('',*,*,#48962,.F.);
#64692=ORIENTED_EDGE('',*,*,#48966,.T.);
#64693=ORIENTED_EDGE('',*,*,#48967,.T.);
#64694=ORIENTED_EDGE('',*,*,#48968,.F.);
#64695=ORIENTED_EDGE('',*,*,#48969,.F.);
#64696=ORIENTED_EDGE('',*,*,#48970,.T.);
#64697=ORIENTED_EDGE('',*,*,#48971,.T.);
#64698=ORIENTED_EDGE('',*,*,#48972,.F.);
#64699=ORIENTED_EDGE('',*,*,#48967,.F.);
#64700=ORIENTED_EDGE('',*,*,#48973,.T.);
#64701=ORIENTED_EDGE('',*,*,#48974,.T.);
#64702=ORIENTED_EDGE('',*,*,#48975,.F.);
#64703=ORIENTED_EDGE('',*,*,#48971,.F.);
#64704=ORIENTED_EDGE('',*,*,#48976,.T.);
#64705=ORIENTED_EDGE('',*,*,#48969,.T.);
#64706=ORIENTED_EDGE('',*,*,#48977,.F.);
#64707=ORIENTED_EDGE('',*,*,#48974,.F.);
#64708=ORIENTED_EDGE('',*,*,#48978,.T.);
#64709=ORIENTED_EDGE('',*,*,#48979,.T.);
#64710=ORIENTED_EDGE('',*,*,#48980,.F.);
#64711=ORIENTED_EDGE('',*,*,#48981,.F.);
#64712=ORIENTED_EDGE('',*,*,#48982,.T.);
#64713=ORIENTED_EDGE('',*,*,#48983,.T.);
#64714=ORIENTED_EDGE('',*,*,#48984,.F.);
#64715=ORIENTED_EDGE('',*,*,#48979,.F.);
#64716=ORIENTED_EDGE('',*,*,#48985,.T.);
#64717=ORIENTED_EDGE('',*,*,#48986,.T.);
#64718=ORIENTED_EDGE('',*,*,#48987,.F.);
#64719=ORIENTED_EDGE('',*,*,#48983,.F.);
#64720=ORIENTED_EDGE('',*,*,#48988,.T.);
#64721=ORIENTED_EDGE('',*,*,#48981,.T.);
#64722=ORIENTED_EDGE('',*,*,#48989,.F.);
#64723=ORIENTED_EDGE('',*,*,#48986,.F.);
#64724=ORIENTED_EDGE('',*,*,#48990,.T.);
#64725=ORIENTED_EDGE('',*,*,#48991,.T.);
#64726=ORIENTED_EDGE('',*,*,#48992,.F.);
#64727=ORIENTED_EDGE('',*,*,#48993,.F.);
#64728=ORIENTED_EDGE('',*,*,#48994,.T.);
#64729=ORIENTED_EDGE('',*,*,#48995,.T.);
#64730=ORIENTED_EDGE('',*,*,#48996,.F.);
#64731=ORIENTED_EDGE('',*,*,#48991,.F.);
#64732=ORIENTED_EDGE('',*,*,#48997,.T.);
#64733=ORIENTED_EDGE('',*,*,#48998,.T.);
#64734=ORIENTED_EDGE('',*,*,#48999,.F.);
#64735=ORIENTED_EDGE('',*,*,#48995,.F.);
#64736=ORIENTED_EDGE('',*,*,#49000,.T.);
#64737=ORIENTED_EDGE('',*,*,#48993,.T.);
#64738=ORIENTED_EDGE('',*,*,#49001,.F.);
#64739=ORIENTED_EDGE('',*,*,#48998,.F.);
#64740=ORIENTED_EDGE('',*,*,#49002,.T.);
#64741=ORIENTED_EDGE('',*,*,#49003,.T.);
#64742=ORIENTED_EDGE('',*,*,#49004,.F.);
#64743=ORIENTED_EDGE('',*,*,#49005,.F.);
#64744=ORIENTED_EDGE('',*,*,#49006,.T.);
#64745=ORIENTED_EDGE('',*,*,#49007,.T.);
#64746=ORIENTED_EDGE('',*,*,#49008,.F.);
#64747=ORIENTED_EDGE('',*,*,#49003,.F.);
#64748=ORIENTED_EDGE('',*,*,#49009,.T.);
#64749=ORIENTED_EDGE('',*,*,#49010,.T.);
#64750=ORIENTED_EDGE('',*,*,#49011,.F.);
#64751=ORIENTED_EDGE('',*,*,#49007,.F.);
#64752=ORIENTED_EDGE('',*,*,#49012,.T.);
#64753=ORIENTED_EDGE('',*,*,#49005,.T.);
#64754=ORIENTED_EDGE('',*,*,#49013,.F.);
#64755=ORIENTED_EDGE('',*,*,#49010,.F.);
#64756=ORIENTED_EDGE('',*,*,#49014,.T.);
#64757=ORIENTED_EDGE('',*,*,#49015,.T.);
#64758=ORIENTED_EDGE('',*,*,#49016,.F.);
#64759=ORIENTED_EDGE('',*,*,#49017,.F.);
#64760=ORIENTED_EDGE('',*,*,#49018,.T.);
#64761=ORIENTED_EDGE('',*,*,#49019,.T.);
#64762=ORIENTED_EDGE('',*,*,#49020,.F.);
#64763=ORIENTED_EDGE('',*,*,#49015,.F.);
#64764=ORIENTED_EDGE('',*,*,#49021,.T.);
#64765=ORIENTED_EDGE('',*,*,#49022,.T.);
#64766=ORIENTED_EDGE('',*,*,#49023,.F.);
#64767=ORIENTED_EDGE('',*,*,#49019,.F.);
#64768=ORIENTED_EDGE('',*,*,#49024,.T.);
#64769=ORIENTED_EDGE('',*,*,#49017,.T.);
#64770=ORIENTED_EDGE('',*,*,#49025,.F.);
#64771=ORIENTED_EDGE('',*,*,#49022,.F.);
#64772=ORIENTED_EDGE('',*,*,#49026,.T.);
#64773=ORIENTED_EDGE('',*,*,#49027,.T.);
#64774=ORIENTED_EDGE('',*,*,#49028,.F.);
#64775=ORIENTED_EDGE('',*,*,#49029,.F.);
#64776=ORIENTED_EDGE('',*,*,#49030,.T.);
#64777=ORIENTED_EDGE('',*,*,#49031,.T.);
#64778=ORIENTED_EDGE('',*,*,#49032,.F.);
#64779=ORIENTED_EDGE('',*,*,#49027,.F.);
#64780=ORIENTED_EDGE('',*,*,#49033,.T.);
#64781=ORIENTED_EDGE('',*,*,#49034,.T.);
#64782=ORIENTED_EDGE('',*,*,#49035,.F.);
#64783=ORIENTED_EDGE('',*,*,#49031,.F.);
#64784=ORIENTED_EDGE('',*,*,#49036,.T.);
#64785=ORIENTED_EDGE('',*,*,#49029,.T.);
#64786=ORIENTED_EDGE('',*,*,#49037,.F.);
#64787=ORIENTED_EDGE('',*,*,#49034,.F.);
#64788=ORIENTED_EDGE('',*,*,#49038,.T.);
#64789=ORIENTED_EDGE('',*,*,#49039,.T.);
#64790=ORIENTED_EDGE('',*,*,#49040,.F.);
#64791=ORIENTED_EDGE('',*,*,#49041,.F.);
#64792=ORIENTED_EDGE('',*,*,#49042,.T.);
#64793=ORIENTED_EDGE('',*,*,#49043,.T.);
#64794=ORIENTED_EDGE('',*,*,#49044,.F.);
#64795=ORIENTED_EDGE('',*,*,#49039,.F.);
#64796=ORIENTED_EDGE('',*,*,#49045,.T.);
#64797=ORIENTED_EDGE('',*,*,#49046,.T.);
#64798=ORIENTED_EDGE('',*,*,#49047,.F.);
#64799=ORIENTED_EDGE('',*,*,#49043,.F.);
#64800=ORIENTED_EDGE('',*,*,#49048,.T.);
#64801=ORIENTED_EDGE('',*,*,#49041,.T.);
#64802=ORIENTED_EDGE('',*,*,#49049,.F.);
#64803=ORIENTED_EDGE('',*,*,#49046,.F.);
#64804=ORIENTED_EDGE('',*,*,#49050,.T.);
#64805=ORIENTED_EDGE('',*,*,#49051,.T.);
#64806=ORIENTED_EDGE('',*,*,#49052,.F.);
#64807=ORIENTED_EDGE('',*,*,#49053,.F.);
#64808=ORIENTED_EDGE('',*,*,#49054,.T.);
#64809=ORIENTED_EDGE('',*,*,#49055,.T.);
#64810=ORIENTED_EDGE('',*,*,#49056,.F.);
#64811=ORIENTED_EDGE('',*,*,#49051,.F.);
#64812=ORIENTED_EDGE('',*,*,#49057,.T.);
#64813=ORIENTED_EDGE('',*,*,#49058,.T.);
#64814=ORIENTED_EDGE('',*,*,#49059,.F.);
#64815=ORIENTED_EDGE('',*,*,#49055,.F.);
#64816=ORIENTED_EDGE('',*,*,#49060,.T.);
#64817=ORIENTED_EDGE('',*,*,#49053,.T.);
#64818=ORIENTED_EDGE('',*,*,#49061,.F.);
#64819=ORIENTED_EDGE('',*,*,#49058,.F.);
#64820=ORIENTED_EDGE('',*,*,#49062,.T.);
#64821=ORIENTED_EDGE('',*,*,#49063,.T.);
#64822=ORIENTED_EDGE('',*,*,#49064,.F.);
#64823=ORIENTED_EDGE('',*,*,#49065,.F.);
#64824=ORIENTED_EDGE('',*,*,#49066,.T.);
#64825=ORIENTED_EDGE('',*,*,#49067,.T.);
#64826=ORIENTED_EDGE('',*,*,#49068,.F.);
#64827=ORIENTED_EDGE('',*,*,#49063,.F.);
#64828=ORIENTED_EDGE('',*,*,#49069,.T.);
#64829=ORIENTED_EDGE('',*,*,#49070,.T.);
#64830=ORIENTED_EDGE('',*,*,#49071,.F.);
#64831=ORIENTED_EDGE('',*,*,#49067,.F.);
#64832=ORIENTED_EDGE('',*,*,#49072,.T.);
#64833=ORIENTED_EDGE('',*,*,#49065,.T.);
#64834=ORIENTED_EDGE('',*,*,#49073,.F.);
#64835=ORIENTED_EDGE('',*,*,#49070,.F.);
#64836=ORIENTED_EDGE('',*,*,#49074,.T.);
#64837=ORIENTED_EDGE('',*,*,#49075,.T.);
#64838=ORIENTED_EDGE('',*,*,#49076,.F.);
#64839=ORIENTED_EDGE('',*,*,#49077,.F.);
#64840=ORIENTED_EDGE('',*,*,#49078,.T.);
#64841=ORIENTED_EDGE('',*,*,#49079,.T.);
#64842=ORIENTED_EDGE('',*,*,#49080,.F.);
#64843=ORIENTED_EDGE('',*,*,#49075,.F.);
#64844=ORIENTED_EDGE('',*,*,#49081,.T.);
#64845=ORIENTED_EDGE('',*,*,#49082,.T.);
#64846=ORIENTED_EDGE('',*,*,#49083,.F.);
#64847=ORIENTED_EDGE('',*,*,#49079,.F.);
#64848=ORIENTED_EDGE('',*,*,#49084,.T.);
#64849=ORIENTED_EDGE('',*,*,#49077,.T.);
#64850=ORIENTED_EDGE('',*,*,#49085,.F.);
#64851=ORIENTED_EDGE('',*,*,#49082,.F.);
#64852=ORIENTED_EDGE('',*,*,#49086,.T.);
#64853=ORIENTED_EDGE('',*,*,#49087,.T.);
#64854=ORIENTED_EDGE('',*,*,#49088,.F.);
#64855=ORIENTED_EDGE('',*,*,#49089,.F.);
#64856=ORIENTED_EDGE('',*,*,#49090,.T.);
#64857=ORIENTED_EDGE('',*,*,#49091,.T.);
#64858=ORIENTED_EDGE('',*,*,#49092,.F.);
#64859=ORIENTED_EDGE('',*,*,#49087,.F.);
#64860=ORIENTED_EDGE('',*,*,#49093,.T.);
#64861=ORIENTED_EDGE('',*,*,#49094,.T.);
#64862=ORIENTED_EDGE('',*,*,#49095,.F.);
#64863=ORIENTED_EDGE('',*,*,#49091,.F.);
#64864=ORIENTED_EDGE('',*,*,#49096,.T.);
#64865=ORIENTED_EDGE('',*,*,#49089,.T.);
#64866=ORIENTED_EDGE('',*,*,#49097,.F.);
#64867=ORIENTED_EDGE('',*,*,#49094,.F.);
#64868=ORIENTED_EDGE('',*,*,#49098,.T.);
#64869=ORIENTED_EDGE('',*,*,#49099,.T.);
#64870=ORIENTED_EDGE('',*,*,#49100,.F.);
#64871=ORIENTED_EDGE('',*,*,#49101,.F.);
#64872=ORIENTED_EDGE('',*,*,#49102,.T.);
#64873=ORIENTED_EDGE('',*,*,#49103,.T.);
#64874=ORIENTED_EDGE('',*,*,#49104,.F.);
#64875=ORIENTED_EDGE('',*,*,#49099,.F.);
#64876=ORIENTED_EDGE('',*,*,#49105,.T.);
#64877=ORIENTED_EDGE('',*,*,#49106,.T.);
#64878=ORIENTED_EDGE('',*,*,#49107,.F.);
#64879=ORIENTED_EDGE('',*,*,#49103,.F.);
#64880=ORIENTED_EDGE('',*,*,#49108,.T.);
#64881=ORIENTED_EDGE('',*,*,#49101,.T.);
#64882=ORIENTED_EDGE('',*,*,#49109,.F.);
#64883=ORIENTED_EDGE('',*,*,#49106,.F.);
#64884=ORIENTED_EDGE('',*,*,#49110,.T.);
#64885=ORIENTED_EDGE('',*,*,#49111,.T.);
#64886=ORIENTED_EDGE('',*,*,#49112,.F.);
#64887=ORIENTED_EDGE('',*,*,#49113,.F.);
#64888=ORIENTED_EDGE('',*,*,#49114,.T.);
#64889=ORIENTED_EDGE('',*,*,#49115,.T.);
#64890=ORIENTED_EDGE('',*,*,#49116,.F.);
#64891=ORIENTED_EDGE('',*,*,#49111,.F.);
#64892=ORIENTED_EDGE('',*,*,#49117,.T.);
#64893=ORIENTED_EDGE('',*,*,#49118,.T.);
#64894=ORIENTED_EDGE('',*,*,#49119,.F.);
#64895=ORIENTED_EDGE('',*,*,#49115,.F.);
#64896=ORIENTED_EDGE('',*,*,#49120,.T.);
#64897=ORIENTED_EDGE('',*,*,#49113,.T.);
#64898=ORIENTED_EDGE('',*,*,#49121,.F.);
#64899=ORIENTED_EDGE('',*,*,#49118,.F.);
#64900=ORIENTED_EDGE('',*,*,#49122,.T.);
#64901=ORIENTED_EDGE('',*,*,#49123,.T.);
#64902=ORIENTED_EDGE('',*,*,#49124,.F.);
#64903=ORIENTED_EDGE('',*,*,#49125,.F.);
#64904=ORIENTED_EDGE('',*,*,#49126,.T.);
#64905=ORIENTED_EDGE('',*,*,#49127,.T.);
#64906=ORIENTED_EDGE('',*,*,#49128,.F.);
#64907=ORIENTED_EDGE('',*,*,#49123,.F.);
#64908=ORIENTED_EDGE('',*,*,#49129,.T.);
#64909=ORIENTED_EDGE('',*,*,#49130,.T.);
#64910=ORIENTED_EDGE('',*,*,#49131,.F.);
#64911=ORIENTED_EDGE('',*,*,#49127,.F.);
#64912=ORIENTED_EDGE('',*,*,#49132,.T.);
#64913=ORIENTED_EDGE('',*,*,#49125,.T.);
#64914=ORIENTED_EDGE('',*,*,#49133,.F.);
#64915=ORIENTED_EDGE('',*,*,#49130,.F.);
#64916=ORIENTED_EDGE('',*,*,#49134,.T.);
#64917=ORIENTED_EDGE('',*,*,#49135,.T.);
#64918=ORIENTED_EDGE('',*,*,#49136,.F.);
#64919=ORIENTED_EDGE('',*,*,#49137,.F.);
#64920=ORIENTED_EDGE('',*,*,#49138,.T.);
#64921=ORIENTED_EDGE('',*,*,#49139,.T.);
#64922=ORIENTED_EDGE('',*,*,#49140,.F.);
#64923=ORIENTED_EDGE('',*,*,#49135,.F.);
#64924=ORIENTED_EDGE('',*,*,#49141,.T.);
#64925=ORIENTED_EDGE('',*,*,#49142,.T.);
#64926=ORIENTED_EDGE('',*,*,#49143,.F.);
#64927=ORIENTED_EDGE('',*,*,#49139,.F.);
#64928=ORIENTED_EDGE('',*,*,#49144,.T.);
#64929=ORIENTED_EDGE('',*,*,#49137,.T.);
#64930=ORIENTED_EDGE('',*,*,#49145,.F.);
#64931=ORIENTED_EDGE('',*,*,#49142,.F.);
#64932=ORIENTED_EDGE('',*,*,#49146,.T.);
#64933=ORIENTED_EDGE('',*,*,#49147,.T.);
#64934=ORIENTED_EDGE('',*,*,#49148,.F.);
#64935=ORIENTED_EDGE('',*,*,#49149,.F.);
#64936=ORIENTED_EDGE('',*,*,#49150,.T.);
#64937=ORIENTED_EDGE('',*,*,#49151,.T.);
#64938=ORIENTED_EDGE('',*,*,#49152,.F.);
#64939=ORIENTED_EDGE('',*,*,#49147,.F.);
#64940=ORIENTED_EDGE('',*,*,#49153,.T.);
#64941=ORIENTED_EDGE('',*,*,#49154,.T.);
#64942=ORIENTED_EDGE('',*,*,#49155,.F.);
#64943=ORIENTED_EDGE('',*,*,#49151,.F.);
#64944=ORIENTED_EDGE('',*,*,#49156,.T.);
#64945=ORIENTED_EDGE('',*,*,#49149,.T.);
#64946=ORIENTED_EDGE('',*,*,#49157,.F.);
#64947=ORIENTED_EDGE('',*,*,#49154,.F.);
#64948=ORIENTED_EDGE('',*,*,#49158,.T.);
#64949=ORIENTED_EDGE('',*,*,#49159,.T.);
#64950=ORIENTED_EDGE('',*,*,#49160,.F.);
#64951=ORIENTED_EDGE('',*,*,#49161,.F.);
#64952=ORIENTED_EDGE('',*,*,#49162,.T.);
#64953=ORIENTED_EDGE('',*,*,#49163,.T.);
#64954=ORIENTED_EDGE('',*,*,#49164,.F.);
#64955=ORIENTED_EDGE('',*,*,#49159,.F.);
#64956=ORIENTED_EDGE('',*,*,#49165,.T.);
#64957=ORIENTED_EDGE('',*,*,#49166,.T.);
#64958=ORIENTED_EDGE('',*,*,#49167,.F.);
#64959=ORIENTED_EDGE('',*,*,#49163,.F.);
#64960=ORIENTED_EDGE('',*,*,#49168,.T.);
#64961=ORIENTED_EDGE('',*,*,#49161,.T.);
#64962=ORIENTED_EDGE('',*,*,#49169,.F.);
#64963=ORIENTED_EDGE('',*,*,#49166,.F.);
#64964=ORIENTED_EDGE('',*,*,#49170,.T.);
#64965=ORIENTED_EDGE('',*,*,#49171,.T.);
#64966=ORIENTED_EDGE('',*,*,#49172,.F.);
#64967=ORIENTED_EDGE('',*,*,#49173,.F.);
#64968=ORIENTED_EDGE('',*,*,#49174,.T.);
#64969=ORIENTED_EDGE('',*,*,#49175,.T.);
#64970=ORIENTED_EDGE('',*,*,#49176,.F.);
#64971=ORIENTED_EDGE('',*,*,#49171,.F.);
#64972=ORIENTED_EDGE('',*,*,#49177,.T.);
#64973=ORIENTED_EDGE('',*,*,#49178,.T.);
#64974=ORIENTED_EDGE('',*,*,#49179,.F.);
#64975=ORIENTED_EDGE('',*,*,#49175,.F.);
#64976=ORIENTED_EDGE('',*,*,#49180,.T.);
#64977=ORIENTED_EDGE('',*,*,#49173,.T.);
#64978=ORIENTED_EDGE('',*,*,#49181,.F.);
#64979=ORIENTED_EDGE('',*,*,#49178,.F.);
#64980=ORIENTED_EDGE('',*,*,#49182,.T.);
#64981=ORIENTED_EDGE('',*,*,#49183,.T.);
#64982=ORIENTED_EDGE('',*,*,#49184,.F.);
#64983=ORIENTED_EDGE('',*,*,#49185,.F.);
#64984=ORIENTED_EDGE('',*,*,#49186,.T.);
#64985=ORIENTED_EDGE('',*,*,#49187,.T.);
#64986=ORIENTED_EDGE('',*,*,#49188,.F.);
#64987=ORIENTED_EDGE('',*,*,#49183,.F.);
#64988=ORIENTED_EDGE('',*,*,#49189,.T.);
#64989=ORIENTED_EDGE('',*,*,#49190,.T.);
#64990=ORIENTED_EDGE('',*,*,#49191,.F.);
#64991=ORIENTED_EDGE('',*,*,#49187,.F.);
#64992=ORIENTED_EDGE('',*,*,#49192,.T.);
#64993=ORIENTED_EDGE('',*,*,#49185,.T.);
#64994=ORIENTED_EDGE('',*,*,#49193,.F.);
#64995=ORIENTED_EDGE('',*,*,#49190,.F.);
#64996=ORIENTED_EDGE('',*,*,#49194,.T.);
#64997=ORIENTED_EDGE('',*,*,#49195,.T.);
#64998=ORIENTED_EDGE('',*,*,#49196,.F.);
#64999=ORIENTED_EDGE('',*,*,#49197,.F.);
#65000=ORIENTED_EDGE('',*,*,#49198,.T.);
#65001=ORIENTED_EDGE('',*,*,#49199,.T.);
#65002=ORIENTED_EDGE('',*,*,#49200,.F.);
#65003=ORIENTED_EDGE('',*,*,#49195,.F.);
#65004=ORIENTED_EDGE('',*,*,#49201,.T.);
#65005=ORIENTED_EDGE('',*,*,#49202,.T.);
#65006=ORIENTED_EDGE('',*,*,#49203,.F.);
#65007=ORIENTED_EDGE('',*,*,#49199,.F.);
#65008=ORIENTED_EDGE('',*,*,#49204,.T.);
#65009=ORIENTED_EDGE('',*,*,#49197,.T.);
#65010=ORIENTED_EDGE('',*,*,#49205,.F.);
#65011=ORIENTED_EDGE('',*,*,#49202,.F.);
#65012=ORIENTED_EDGE('',*,*,#49206,.T.);
#65013=ORIENTED_EDGE('',*,*,#49207,.T.);
#65014=ORIENTED_EDGE('',*,*,#49208,.F.);
#65015=ORIENTED_EDGE('',*,*,#49209,.F.);
#65016=ORIENTED_EDGE('',*,*,#49210,.T.);
#65017=ORIENTED_EDGE('',*,*,#49211,.T.);
#65018=ORIENTED_EDGE('',*,*,#49212,.F.);
#65019=ORIENTED_EDGE('',*,*,#49207,.F.);
#65020=ORIENTED_EDGE('',*,*,#49213,.T.);
#65021=ORIENTED_EDGE('',*,*,#49214,.T.);
#65022=ORIENTED_EDGE('',*,*,#49215,.F.);
#65023=ORIENTED_EDGE('',*,*,#49211,.F.);
#65024=ORIENTED_EDGE('',*,*,#49216,.T.);
#65025=ORIENTED_EDGE('',*,*,#49209,.T.);
#65026=ORIENTED_EDGE('',*,*,#49217,.F.);
#65027=ORIENTED_EDGE('',*,*,#49214,.F.);
#65028=ORIENTED_EDGE('',*,*,#49218,.T.);
#65029=ORIENTED_EDGE('',*,*,#49219,.T.);
#65030=ORIENTED_EDGE('',*,*,#49220,.F.);
#65031=ORIENTED_EDGE('',*,*,#49221,.F.);
#65032=ORIENTED_EDGE('',*,*,#49222,.T.);
#65033=ORIENTED_EDGE('',*,*,#49223,.T.);
#65034=ORIENTED_EDGE('',*,*,#49224,.F.);
#65035=ORIENTED_EDGE('',*,*,#49219,.F.);
#65036=ORIENTED_EDGE('',*,*,#49225,.T.);
#65037=ORIENTED_EDGE('',*,*,#49226,.T.);
#65038=ORIENTED_EDGE('',*,*,#49227,.F.);
#65039=ORIENTED_EDGE('',*,*,#49223,.F.);
#65040=ORIENTED_EDGE('',*,*,#49228,.T.);
#65041=ORIENTED_EDGE('',*,*,#49221,.T.);
#65042=ORIENTED_EDGE('',*,*,#49229,.F.);
#65043=ORIENTED_EDGE('',*,*,#49226,.F.);
#65044=ORIENTED_EDGE('',*,*,#49230,.T.);
#65045=ORIENTED_EDGE('',*,*,#49231,.T.);
#65046=ORIENTED_EDGE('',*,*,#49232,.F.);
#65047=ORIENTED_EDGE('',*,*,#49233,.F.);
#65048=ORIENTED_EDGE('',*,*,#49234,.T.);
#65049=ORIENTED_EDGE('',*,*,#49235,.T.);
#65050=ORIENTED_EDGE('',*,*,#49236,.F.);
#65051=ORIENTED_EDGE('',*,*,#49231,.F.);
#65052=ORIENTED_EDGE('',*,*,#49237,.T.);
#65053=ORIENTED_EDGE('',*,*,#49238,.T.);
#65054=ORIENTED_EDGE('',*,*,#49239,.F.);
#65055=ORIENTED_EDGE('',*,*,#49235,.F.);
#65056=ORIENTED_EDGE('',*,*,#49240,.T.);
#65057=ORIENTED_EDGE('',*,*,#49233,.T.);
#65058=ORIENTED_EDGE('',*,*,#49241,.F.);
#65059=ORIENTED_EDGE('',*,*,#49238,.F.);
#65060=ORIENTED_EDGE('',*,*,#49242,.T.);
#65061=ORIENTED_EDGE('',*,*,#49243,.T.);
#65062=ORIENTED_EDGE('',*,*,#49244,.F.);
#65063=ORIENTED_EDGE('',*,*,#49245,.F.);
#65064=ORIENTED_EDGE('',*,*,#49246,.T.);
#65065=ORIENTED_EDGE('',*,*,#49247,.T.);
#65066=ORIENTED_EDGE('',*,*,#49248,.F.);
#65067=ORIENTED_EDGE('',*,*,#49243,.F.);
#65068=ORIENTED_EDGE('',*,*,#49249,.T.);
#65069=ORIENTED_EDGE('',*,*,#49250,.T.);
#65070=ORIENTED_EDGE('',*,*,#49251,.F.);
#65071=ORIENTED_EDGE('',*,*,#49247,.F.);
#65072=ORIENTED_EDGE('',*,*,#49252,.T.);
#65073=ORIENTED_EDGE('',*,*,#49245,.T.);
#65074=ORIENTED_EDGE('',*,*,#49253,.F.);
#65075=ORIENTED_EDGE('',*,*,#49250,.F.);
#65076=ORIENTED_EDGE('',*,*,#49254,.T.);
#65077=ORIENTED_EDGE('',*,*,#49255,.T.);
#65078=ORIENTED_EDGE('',*,*,#49256,.F.);
#65079=ORIENTED_EDGE('',*,*,#49257,.F.);
#65080=ORIENTED_EDGE('',*,*,#49258,.T.);
#65081=ORIENTED_EDGE('',*,*,#49259,.T.);
#65082=ORIENTED_EDGE('',*,*,#49260,.F.);
#65083=ORIENTED_EDGE('',*,*,#49255,.F.);
#65084=ORIENTED_EDGE('',*,*,#49261,.T.);
#65085=ORIENTED_EDGE('',*,*,#49262,.T.);
#65086=ORIENTED_EDGE('',*,*,#49263,.F.);
#65087=ORIENTED_EDGE('',*,*,#49259,.F.);
#65088=ORIENTED_EDGE('',*,*,#49264,.T.);
#65089=ORIENTED_EDGE('',*,*,#49257,.T.);
#65090=ORIENTED_EDGE('',*,*,#49265,.F.);
#65091=ORIENTED_EDGE('',*,*,#49262,.F.);
#65092=ORIENTED_EDGE('',*,*,#49266,.T.);
#65093=ORIENTED_EDGE('',*,*,#49267,.T.);
#65094=ORIENTED_EDGE('',*,*,#49268,.F.);
#65095=ORIENTED_EDGE('',*,*,#49269,.F.);
#65096=ORIENTED_EDGE('',*,*,#49270,.T.);
#65097=ORIENTED_EDGE('',*,*,#49271,.T.);
#65098=ORIENTED_EDGE('',*,*,#49272,.F.);
#65099=ORIENTED_EDGE('',*,*,#49267,.F.);
#65100=ORIENTED_EDGE('',*,*,#49273,.T.);
#65101=ORIENTED_EDGE('',*,*,#49274,.T.);
#65102=ORIENTED_EDGE('',*,*,#49275,.F.);
#65103=ORIENTED_EDGE('',*,*,#49271,.F.);
#65104=ORIENTED_EDGE('',*,*,#49276,.T.);
#65105=ORIENTED_EDGE('',*,*,#49269,.T.);
#65106=ORIENTED_EDGE('',*,*,#49277,.F.);
#65107=ORIENTED_EDGE('',*,*,#49274,.F.);
#65108=ORIENTED_EDGE('',*,*,#49278,.T.);
#65109=ORIENTED_EDGE('',*,*,#49279,.T.);
#65110=ORIENTED_EDGE('',*,*,#49280,.F.);
#65111=ORIENTED_EDGE('',*,*,#49281,.F.);
#65112=ORIENTED_EDGE('',*,*,#49282,.T.);
#65113=ORIENTED_EDGE('',*,*,#49283,.T.);
#65114=ORIENTED_EDGE('',*,*,#49284,.F.);
#65115=ORIENTED_EDGE('',*,*,#49279,.F.);
#65116=ORIENTED_EDGE('',*,*,#49285,.T.);
#65117=ORIENTED_EDGE('',*,*,#49286,.T.);
#65118=ORIENTED_EDGE('',*,*,#49287,.F.);
#65119=ORIENTED_EDGE('',*,*,#49283,.F.);
#65120=ORIENTED_EDGE('',*,*,#49288,.T.);
#65121=ORIENTED_EDGE('',*,*,#49281,.T.);
#65122=ORIENTED_EDGE('',*,*,#49289,.F.);
#65123=ORIENTED_EDGE('',*,*,#49286,.F.);
#65124=ORIENTED_EDGE('',*,*,#49290,.T.);
#65125=ORIENTED_EDGE('',*,*,#49291,.T.);
#65126=ORIENTED_EDGE('',*,*,#49292,.F.);
#65127=ORIENTED_EDGE('',*,*,#49293,.F.);
#65128=ORIENTED_EDGE('',*,*,#49294,.T.);
#65129=ORIENTED_EDGE('',*,*,#49295,.T.);
#65130=ORIENTED_EDGE('',*,*,#49296,.F.);
#65131=ORIENTED_EDGE('',*,*,#49291,.F.);
#65132=ORIENTED_EDGE('',*,*,#49297,.T.);
#65133=ORIENTED_EDGE('',*,*,#49298,.T.);
#65134=ORIENTED_EDGE('',*,*,#49299,.F.);
#65135=ORIENTED_EDGE('',*,*,#49295,.F.);
#65136=ORIENTED_EDGE('',*,*,#49300,.T.);
#65137=ORIENTED_EDGE('',*,*,#49293,.T.);
#65138=ORIENTED_EDGE('',*,*,#49301,.F.);
#65139=ORIENTED_EDGE('',*,*,#49298,.F.);
#65140=ORIENTED_EDGE('',*,*,#49302,.T.);
#65141=ORIENTED_EDGE('',*,*,#49303,.T.);
#65142=ORIENTED_EDGE('',*,*,#49304,.F.);
#65143=ORIENTED_EDGE('',*,*,#49305,.F.);
#65144=ORIENTED_EDGE('',*,*,#49306,.T.);
#65145=ORIENTED_EDGE('',*,*,#49307,.T.);
#65146=ORIENTED_EDGE('',*,*,#49308,.F.);
#65147=ORIENTED_EDGE('',*,*,#49303,.F.);
#65148=ORIENTED_EDGE('',*,*,#49309,.T.);
#65149=ORIENTED_EDGE('',*,*,#49310,.T.);
#65150=ORIENTED_EDGE('',*,*,#49311,.F.);
#65151=ORIENTED_EDGE('',*,*,#49307,.F.);
#65152=ORIENTED_EDGE('',*,*,#49312,.T.);
#65153=ORIENTED_EDGE('',*,*,#49305,.T.);
#65154=ORIENTED_EDGE('',*,*,#49313,.F.);
#65155=ORIENTED_EDGE('',*,*,#49310,.F.);
#65156=ORIENTED_EDGE('',*,*,#49314,.T.);
#65157=ORIENTED_EDGE('',*,*,#49315,.T.);
#65158=ORIENTED_EDGE('',*,*,#49316,.F.);
#65159=ORIENTED_EDGE('',*,*,#49317,.F.);
#65160=ORIENTED_EDGE('',*,*,#49318,.T.);
#65161=ORIENTED_EDGE('',*,*,#49319,.T.);
#65162=ORIENTED_EDGE('',*,*,#49320,.F.);
#65163=ORIENTED_EDGE('',*,*,#49315,.F.);
#65164=ORIENTED_EDGE('',*,*,#49321,.T.);
#65165=ORIENTED_EDGE('',*,*,#49322,.T.);
#65166=ORIENTED_EDGE('',*,*,#49323,.F.);
#65167=ORIENTED_EDGE('',*,*,#49319,.F.);
#65168=ORIENTED_EDGE('',*,*,#49324,.T.);
#65169=ORIENTED_EDGE('',*,*,#49317,.T.);
#65170=ORIENTED_EDGE('',*,*,#49325,.F.);
#65171=ORIENTED_EDGE('',*,*,#49322,.F.);
#65172=ORIENTED_EDGE('',*,*,#49326,.T.);
#65173=ORIENTED_EDGE('',*,*,#49327,.T.);
#65174=ORIENTED_EDGE('',*,*,#49328,.F.);
#65175=ORIENTED_EDGE('',*,*,#49329,.F.);
#65176=ORIENTED_EDGE('',*,*,#49330,.T.);
#65177=ORIENTED_EDGE('',*,*,#49331,.T.);
#65178=ORIENTED_EDGE('',*,*,#49332,.F.);
#65179=ORIENTED_EDGE('',*,*,#49327,.F.);
#65180=ORIENTED_EDGE('',*,*,#49333,.T.);
#65181=ORIENTED_EDGE('',*,*,#49334,.T.);
#65182=ORIENTED_EDGE('',*,*,#49335,.F.);
#65183=ORIENTED_EDGE('',*,*,#49331,.F.);
#65184=ORIENTED_EDGE('',*,*,#49336,.T.);
#65185=ORIENTED_EDGE('',*,*,#49329,.T.);
#65186=ORIENTED_EDGE('',*,*,#49337,.F.);
#65187=ORIENTED_EDGE('',*,*,#49334,.F.);
#65188=ORIENTED_EDGE('',*,*,#49338,.T.);
#65189=ORIENTED_EDGE('',*,*,#49339,.T.);
#65190=ORIENTED_EDGE('',*,*,#49340,.F.);
#65191=ORIENTED_EDGE('',*,*,#49341,.F.);
#65192=ORIENTED_EDGE('',*,*,#49342,.T.);
#65193=ORIENTED_EDGE('',*,*,#49343,.T.);
#65194=ORIENTED_EDGE('',*,*,#49344,.F.);
#65195=ORIENTED_EDGE('',*,*,#49339,.F.);
#65196=ORIENTED_EDGE('',*,*,#49345,.T.);
#65197=ORIENTED_EDGE('',*,*,#49346,.T.);
#65198=ORIENTED_EDGE('',*,*,#49347,.F.);
#65199=ORIENTED_EDGE('',*,*,#49343,.F.);
#65200=ORIENTED_EDGE('',*,*,#49348,.T.);
#65201=ORIENTED_EDGE('',*,*,#49341,.T.);
#65202=ORIENTED_EDGE('',*,*,#49349,.F.);
#65203=ORIENTED_EDGE('',*,*,#49346,.F.);
#65204=ORIENTED_EDGE('',*,*,#49350,.T.);
#65205=ORIENTED_EDGE('',*,*,#49351,.T.);
#65206=ORIENTED_EDGE('',*,*,#49352,.F.);
#65207=ORIENTED_EDGE('',*,*,#49353,.F.);
#65208=ORIENTED_EDGE('',*,*,#49354,.T.);
#65209=ORIENTED_EDGE('',*,*,#49355,.T.);
#65210=ORIENTED_EDGE('',*,*,#49356,.F.);
#65211=ORIENTED_EDGE('',*,*,#49351,.F.);
#65212=ORIENTED_EDGE('',*,*,#49357,.T.);
#65213=ORIENTED_EDGE('',*,*,#49358,.T.);
#65214=ORIENTED_EDGE('',*,*,#49359,.F.);
#65215=ORIENTED_EDGE('',*,*,#49355,.F.);
#65216=ORIENTED_EDGE('',*,*,#49360,.T.);
#65217=ORIENTED_EDGE('',*,*,#49353,.T.);
#65218=ORIENTED_EDGE('',*,*,#49361,.F.);
#65219=ORIENTED_EDGE('',*,*,#49358,.F.);
#65220=ORIENTED_EDGE('',*,*,#49362,.T.);
#65221=ORIENTED_EDGE('',*,*,#49363,.T.);
#65222=ORIENTED_EDGE('',*,*,#49364,.F.);
#65223=ORIENTED_EDGE('',*,*,#49365,.F.);
#65224=ORIENTED_EDGE('',*,*,#49366,.T.);
#65225=ORIENTED_EDGE('',*,*,#49367,.T.);
#65226=ORIENTED_EDGE('',*,*,#49368,.F.);
#65227=ORIENTED_EDGE('',*,*,#49363,.F.);
#65228=ORIENTED_EDGE('',*,*,#49369,.T.);
#65229=ORIENTED_EDGE('',*,*,#49370,.T.);
#65230=ORIENTED_EDGE('',*,*,#49371,.F.);
#65231=ORIENTED_EDGE('',*,*,#49367,.F.);
#65232=ORIENTED_EDGE('',*,*,#49372,.T.);
#65233=ORIENTED_EDGE('',*,*,#49365,.T.);
#65234=ORIENTED_EDGE('',*,*,#49373,.F.);
#65235=ORIENTED_EDGE('',*,*,#49370,.F.);
#65236=ORIENTED_EDGE('',*,*,#49374,.T.);
#65237=ORIENTED_EDGE('',*,*,#49375,.T.);
#65238=ORIENTED_EDGE('',*,*,#49376,.F.);
#65239=ORIENTED_EDGE('',*,*,#49377,.F.);
#65240=ORIENTED_EDGE('',*,*,#49378,.T.);
#65241=ORIENTED_EDGE('',*,*,#49379,.T.);
#65242=ORIENTED_EDGE('',*,*,#49380,.F.);
#65243=ORIENTED_EDGE('',*,*,#49375,.F.);
#65244=ORIENTED_EDGE('',*,*,#49381,.T.);
#65245=ORIENTED_EDGE('',*,*,#49382,.T.);
#65246=ORIENTED_EDGE('',*,*,#49383,.F.);
#65247=ORIENTED_EDGE('',*,*,#49379,.F.);
#65248=ORIENTED_EDGE('',*,*,#49384,.T.);
#65249=ORIENTED_EDGE('',*,*,#49377,.T.);
#65250=ORIENTED_EDGE('',*,*,#49385,.F.);
#65251=ORIENTED_EDGE('',*,*,#49382,.F.);
#65252=ORIENTED_EDGE('',*,*,#49386,.T.);
#65253=ORIENTED_EDGE('',*,*,#49387,.T.);
#65254=ORIENTED_EDGE('',*,*,#49388,.F.);
#65255=ORIENTED_EDGE('',*,*,#49389,.F.);
#65256=ORIENTED_EDGE('',*,*,#49390,.T.);
#65257=ORIENTED_EDGE('',*,*,#49391,.T.);
#65258=ORIENTED_EDGE('',*,*,#49392,.F.);
#65259=ORIENTED_EDGE('',*,*,#49387,.F.);
#65260=ORIENTED_EDGE('',*,*,#49393,.T.);
#65261=ORIENTED_EDGE('',*,*,#49394,.T.);
#65262=ORIENTED_EDGE('',*,*,#49395,.F.);
#65263=ORIENTED_EDGE('',*,*,#49391,.F.);
#65264=ORIENTED_EDGE('',*,*,#49396,.T.);
#65265=ORIENTED_EDGE('',*,*,#49389,.T.);
#65266=ORIENTED_EDGE('',*,*,#49397,.F.);
#65267=ORIENTED_EDGE('',*,*,#49394,.F.);
#65268=ORIENTED_EDGE('',*,*,#49398,.T.);
#65269=ORIENTED_EDGE('',*,*,#49399,.T.);
#65270=ORIENTED_EDGE('',*,*,#49400,.F.);
#65271=ORIENTED_EDGE('',*,*,#49401,.F.);
#65272=ORIENTED_EDGE('',*,*,#49402,.T.);
#65273=ORIENTED_EDGE('',*,*,#49403,.T.);
#65274=ORIENTED_EDGE('',*,*,#49404,.F.);
#65275=ORIENTED_EDGE('',*,*,#49399,.F.);
#65276=ORIENTED_EDGE('',*,*,#49405,.T.);
#65277=ORIENTED_EDGE('',*,*,#49406,.T.);
#65278=ORIENTED_EDGE('',*,*,#49407,.F.);
#65279=ORIENTED_EDGE('',*,*,#49403,.F.);
#65280=ORIENTED_EDGE('',*,*,#49408,.T.);
#65281=ORIENTED_EDGE('',*,*,#49401,.T.);
#65282=ORIENTED_EDGE('',*,*,#49409,.F.);
#65283=ORIENTED_EDGE('',*,*,#49406,.F.);
#65284=ORIENTED_EDGE('',*,*,#49410,.T.);
#65285=ORIENTED_EDGE('',*,*,#49411,.T.);
#65286=ORIENTED_EDGE('',*,*,#49412,.F.);
#65287=ORIENTED_EDGE('',*,*,#49413,.F.);
#65288=ORIENTED_EDGE('',*,*,#49414,.T.);
#65289=ORIENTED_EDGE('',*,*,#49415,.T.);
#65290=ORIENTED_EDGE('',*,*,#49416,.F.);
#65291=ORIENTED_EDGE('',*,*,#49411,.F.);
#65292=ORIENTED_EDGE('',*,*,#49417,.T.);
#65293=ORIENTED_EDGE('',*,*,#49418,.T.);
#65294=ORIENTED_EDGE('',*,*,#49419,.F.);
#65295=ORIENTED_EDGE('',*,*,#49415,.F.);
#65296=ORIENTED_EDGE('',*,*,#49420,.T.);
#65297=ORIENTED_EDGE('',*,*,#49413,.T.);
#65298=ORIENTED_EDGE('',*,*,#49421,.F.);
#65299=ORIENTED_EDGE('',*,*,#49418,.F.);
#65300=ORIENTED_EDGE('',*,*,#49422,.T.);
#65301=ORIENTED_EDGE('',*,*,#49423,.T.);
#65302=ORIENTED_EDGE('',*,*,#49424,.F.);
#65303=ORIENTED_EDGE('',*,*,#49425,.F.);
#65304=ORIENTED_EDGE('',*,*,#49426,.T.);
#65305=ORIENTED_EDGE('',*,*,#49427,.T.);
#65306=ORIENTED_EDGE('',*,*,#49428,.F.);
#65307=ORIENTED_EDGE('',*,*,#49423,.F.);
#65308=ORIENTED_EDGE('',*,*,#49429,.T.);
#65309=ORIENTED_EDGE('',*,*,#49430,.T.);
#65310=ORIENTED_EDGE('',*,*,#49431,.F.);
#65311=ORIENTED_EDGE('',*,*,#49427,.F.);
#65312=ORIENTED_EDGE('',*,*,#49432,.T.);
#65313=ORIENTED_EDGE('',*,*,#49425,.T.);
#65314=ORIENTED_EDGE('',*,*,#49433,.F.);
#65315=ORIENTED_EDGE('',*,*,#49430,.F.);
#65316=ORIENTED_EDGE('',*,*,#49434,.T.);
#65317=ORIENTED_EDGE('',*,*,#49435,.T.);
#65318=ORIENTED_EDGE('',*,*,#49436,.F.);
#65319=ORIENTED_EDGE('',*,*,#49437,.F.);
#65320=ORIENTED_EDGE('',*,*,#49438,.T.);
#65321=ORIENTED_EDGE('',*,*,#49439,.T.);
#65322=ORIENTED_EDGE('',*,*,#49440,.F.);
#65323=ORIENTED_EDGE('',*,*,#49435,.F.);
#65324=ORIENTED_EDGE('',*,*,#49441,.T.);
#65325=ORIENTED_EDGE('',*,*,#49442,.T.);
#65326=ORIENTED_EDGE('',*,*,#49443,.F.);
#65327=ORIENTED_EDGE('',*,*,#49439,.F.);
#65328=ORIENTED_EDGE('',*,*,#49444,.T.);
#65329=ORIENTED_EDGE('',*,*,#49437,.T.);
#65330=ORIENTED_EDGE('',*,*,#49445,.F.);
#65331=ORIENTED_EDGE('',*,*,#49442,.F.);
#65332=ORIENTED_EDGE('',*,*,#49446,.T.);
#65333=ORIENTED_EDGE('',*,*,#49447,.T.);
#65334=ORIENTED_EDGE('',*,*,#49448,.F.);
#65335=ORIENTED_EDGE('',*,*,#49449,.F.);
#65336=ORIENTED_EDGE('',*,*,#49450,.T.);
#65337=ORIENTED_EDGE('',*,*,#49451,.T.);
#65338=ORIENTED_EDGE('',*,*,#49452,.F.);
#65339=ORIENTED_EDGE('',*,*,#49447,.F.);
#65340=ORIENTED_EDGE('',*,*,#49453,.T.);
#65341=ORIENTED_EDGE('',*,*,#49454,.T.);
#65342=ORIENTED_EDGE('',*,*,#49455,.F.);
#65343=ORIENTED_EDGE('',*,*,#49451,.F.);
#65344=ORIENTED_EDGE('',*,*,#49456,.T.);
#65345=ORIENTED_EDGE('',*,*,#49449,.T.);
#65346=ORIENTED_EDGE('',*,*,#49457,.F.);
#65347=ORIENTED_EDGE('',*,*,#49454,.F.);
#65348=ORIENTED_EDGE('',*,*,#49458,.T.);
#65349=ORIENTED_EDGE('',*,*,#49459,.T.);
#65350=ORIENTED_EDGE('',*,*,#49460,.F.);
#65351=ORIENTED_EDGE('',*,*,#49461,.F.);
#65352=ORIENTED_EDGE('',*,*,#49462,.T.);
#65353=ORIENTED_EDGE('',*,*,#49463,.T.);
#65354=ORIENTED_EDGE('',*,*,#49464,.F.);
#65355=ORIENTED_EDGE('',*,*,#49459,.F.);
#65356=ORIENTED_EDGE('',*,*,#49465,.T.);
#65357=ORIENTED_EDGE('',*,*,#49466,.T.);
#65358=ORIENTED_EDGE('',*,*,#49467,.F.);
#65359=ORIENTED_EDGE('',*,*,#49463,.F.);
#65360=ORIENTED_EDGE('',*,*,#49468,.T.);
#65361=ORIENTED_EDGE('',*,*,#49461,.T.);
#65362=ORIENTED_EDGE('',*,*,#49469,.F.);
#65363=ORIENTED_EDGE('',*,*,#49466,.F.);
#65364=ORIENTED_EDGE('',*,*,#49470,.T.);
#65365=ORIENTED_EDGE('',*,*,#49471,.T.);
#65366=ORIENTED_EDGE('',*,*,#49472,.F.);
#65367=ORIENTED_EDGE('',*,*,#49473,.F.);
#65368=ORIENTED_EDGE('',*,*,#49474,.T.);
#65369=ORIENTED_EDGE('',*,*,#49475,.T.);
#65370=ORIENTED_EDGE('',*,*,#49476,.F.);
#65371=ORIENTED_EDGE('',*,*,#49471,.F.);
#65372=ORIENTED_EDGE('',*,*,#49477,.T.);
#65373=ORIENTED_EDGE('',*,*,#49478,.T.);
#65374=ORIENTED_EDGE('',*,*,#49479,.F.);
#65375=ORIENTED_EDGE('',*,*,#49475,.F.);
#65376=ORIENTED_EDGE('',*,*,#49480,.T.);
#65377=ORIENTED_EDGE('',*,*,#49473,.T.);
#65378=ORIENTED_EDGE('',*,*,#49481,.F.);
#65379=ORIENTED_EDGE('',*,*,#49478,.F.);
#65380=ORIENTED_EDGE('',*,*,#49482,.T.);
#65381=ORIENTED_EDGE('',*,*,#49483,.T.);
#65382=ORIENTED_EDGE('',*,*,#49484,.F.);
#65383=ORIENTED_EDGE('',*,*,#49485,.F.);
#65384=ORIENTED_EDGE('',*,*,#49486,.T.);
#65385=ORIENTED_EDGE('',*,*,#49487,.T.);
#65386=ORIENTED_EDGE('',*,*,#49488,.F.);
#65387=ORIENTED_EDGE('',*,*,#49483,.F.);
#65388=ORIENTED_EDGE('',*,*,#49489,.T.);
#65389=ORIENTED_EDGE('',*,*,#49490,.T.);
#65390=ORIENTED_EDGE('',*,*,#49491,.F.);
#65391=ORIENTED_EDGE('',*,*,#49487,.F.);
#65392=ORIENTED_EDGE('',*,*,#49492,.T.);
#65393=ORIENTED_EDGE('',*,*,#49485,.T.);
#65394=ORIENTED_EDGE('',*,*,#49493,.F.);
#65395=ORIENTED_EDGE('',*,*,#49490,.F.);
#65396=ORIENTED_EDGE('',*,*,#49494,.T.);
#65397=ORIENTED_EDGE('',*,*,#49495,.T.);
#65398=ORIENTED_EDGE('',*,*,#49496,.F.);
#65399=ORIENTED_EDGE('',*,*,#49497,.F.);
#65400=ORIENTED_EDGE('',*,*,#49498,.T.);
#65401=ORIENTED_EDGE('',*,*,#49499,.T.);
#65402=ORIENTED_EDGE('',*,*,#49500,.F.);
#65403=ORIENTED_EDGE('',*,*,#49495,.F.);
#65404=ORIENTED_EDGE('',*,*,#49501,.T.);
#65405=ORIENTED_EDGE('',*,*,#49502,.T.);
#65406=ORIENTED_EDGE('',*,*,#49503,.F.);
#65407=ORIENTED_EDGE('',*,*,#49499,.F.);
#65408=ORIENTED_EDGE('',*,*,#49504,.T.);
#65409=ORIENTED_EDGE('',*,*,#49497,.T.);
#65410=ORIENTED_EDGE('',*,*,#49505,.F.);
#65411=ORIENTED_EDGE('',*,*,#49502,.F.);
#65412=ORIENTED_EDGE('',*,*,#49506,.T.);
#65413=ORIENTED_EDGE('',*,*,#49507,.T.);
#65414=ORIENTED_EDGE('',*,*,#49508,.F.);
#65415=ORIENTED_EDGE('',*,*,#49509,.F.);
#65416=ORIENTED_EDGE('',*,*,#49510,.T.);
#65417=ORIENTED_EDGE('',*,*,#49511,.T.);
#65418=ORIENTED_EDGE('',*,*,#49512,.F.);
#65419=ORIENTED_EDGE('',*,*,#49507,.F.);
#65420=ORIENTED_EDGE('',*,*,#49513,.T.);
#65421=ORIENTED_EDGE('',*,*,#49514,.T.);
#65422=ORIENTED_EDGE('',*,*,#49515,.F.);
#65423=ORIENTED_EDGE('',*,*,#49511,.F.);
#65424=ORIENTED_EDGE('',*,*,#49516,.T.);
#65425=ORIENTED_EDGE('',*,*,#49509,.T.);
#65426=ORIENTED_EDGE('',*,*,#49517,.F.);
#65427=ORIENTED_EDGE('',*,*,#49514,.F.);
#65428=ORIENTED_EDGE('',*,*,#49518,.T.);
#65429=ORIENTED_EDGE('',*,*,#49519,.T.);
#65430=ORIENTED_EDGE('',*,*,#49520,.F.);
#65431=ORIENTED_EDGE('',*,*,#49521,.F.);
#65432=ORIENTED_EDGE('',*,*,#49522,.T.);
#65433=ORIENTED_EDGE('',*,*,#49523,.T.);
#65434=ORIENTED_EDGE('',*,*,#49524,.F.);
#65435=ORIENTED_EDGE('',*,*,#49519,.F.);
#65436=ORIENTED_EDGE('',*,*,#49525,.T.);
#65437=ORIENTED_EDGE('',*,*,#49526,.T.);
#65438=ORIENTED_EDGE('',*,*,#49527,.F.);
#65439=ORIENTED_EDGE('',*,*,#49523,.F.);
#65440=ORIENTED_EDGE('',*,*,#49528,.T.);
#65441=ORIENTED_EDGE('',*,*,#49521,.T.);
#65442=ORIENTED_EDGE('',*,*,#49529,.F.);
#65443=ORIENTED_EDGE('',*,*,#49526,.F.);
#65444=ORIENTED_EDGE('',*,*,#49530,.T.);
#65445=ORIENTED_EDGE('',*,*,#49531,.T.);
#65446=ORIENTED_EDGE('',*,*,#49532,.F.);
#65447=ORIENTED_EDGE('',*,*,#49533,.F.);
#65448=ORIENTED_EDGE('',*,*,#49534,.T.);
#65449=ORIENTED_EDGE('',*,*,#49535,.T.);
#65450=ORIENTED_EDGE('',*,*,#49536,.F.);
#65451=ORIENTED_EDGE('',*,*,#49531,.F.);
#65452=ORIENTED_EDGE('',*,*,#49537,.T.);
#65453=ORIENTED_EDGE('',*,*,#49538,.T.);
#65454=ORIENTED_EDGE('',*,*,#49539,.F.);
#65455=ORIENTED_EDGE('',*,*,#49535,.F.);
#65456=ORIENTED_EDGE('',*,*,#49540,.T.);
#65457=ORIENTED_EDGE('',*,*,#49533,.T.);
#65458=ORIENTED_EDGE('',*,*,#49541,.F.);
#65459=ORIENTED_EDGE('',*,*,#49538,.F.);
#65460=ORIENTED_EDGE('',*,*,#49542,.T.);
#65461=ORIENTED_EDGE('',*,*,#49543,.T.);
#65462=ORIENTED_EDGE('',*,*,#49544,.F.);
#65463=ORIENTED_EDGE('',*,*,#49545,.F.);
#65464=ORIENTED_EDGE('',*,*,#49546,.T.);
#65465=ORIENTED_EDGE('',*,*,#49547,.T.);
#65466=ORIENTED_EDGE('',*,*,#49548,.F.);
#65467=ORIENTED_EDGE('',*,*,#49543,.F.);
#65468=ORIENTED_EDGE('',*,*,#49549,.T.);
#65469=ORIENTED_EDGE('',*,*,#49550,.T.);
#65470=ORIENTED_EDGE('',*,*,#49551,.F.);
#65471=ORIENTED_EDGE('',*,*,#49547,.F.);
#65472=ORIENTED_EDGE('',*,*,#49552,.T.);
#65473=ORIENTED_EDGE('',*,*,#49545,.T.);
#65474=ORIENTED_EDGE('',*,*,#49553,.F.);
#65475=ORIENTED_EDGE('',*,*,#49550,.F.);
#65476=ORIENTED_EDGE('',*,*,#49554,.T.);
#65477=ORIENTED_EDGE('',*,*,#49555,.T.);
#65478=ORIENTED_EDGE('',*,*,#49556,.F.);
#65479=ORIENTED_EDGE('',*,*,#49557,.F.);
#65480=ORIENTED_EDGE('',*,*,#49558,.T.);
#65481=ORIENTED_EDGE('',*,*,#49559,.T.);
#65482=ORIENTED_EDGE('',*,*,#49560,.F.);
#65483=ORIENTED_EDGE('',*,*,#49555,.F.);
#65484=ORIENTED_EDGE('',*,*,#49561,.T.);
#65485=ORIENTED_EDGE('',*,*,#49562,.T.);
#65486=ORIENTED_EDGE('',*,*,#49563,.F.);
#65487=ORIENTED_EDGE('',*,*,#49559,.F.);
#65488=ORIENTED_EDGE('',*,*,#49564,.T.);
#65489=ORIENTED_EDGE('',*,*,#49557,.T.);
#65490=ORIENTED_EDGE('',*,*,#49565,.F.);
#65491=ORIENTED_EDGE('',*,*,#49562,.F.);
#65492=ORIENTED_EDGE('',*,*,#49566,.T.);
#65493=ORIENTED_EDGE('',*,*,#49567,.T.);
#65494=ORIENTED_EDGE('',*,*,#49568,.F.);
#65495=ORIENTED_EDGE('',*,*,#49569,.F.);
#65496=ORIENTED_EDGE('',*,*,#49570,.T.);
#65497=ORIENTED_EDGE('',*,*,#49571,.T.);
#65498=ORIENTED_EDGE('',*,*,#49572,.F.);
#65499=ORIENTED_EDGE('',*,*,#49567,.F.);
#65500=ORIENTED_EDGE('',*,*,#49573,.T.);
#65501=ORIENTED_EDGE('',*,*,#49574,.T.);
#65502=ORIENTED_EDGE('',*,*,#49575,.F.);
#65503=ORIENTED_EDGE('',*,*,#49571,.F.);
#65504=ORIENTED_EDGE('',*,*,#49576,.T.);
#65505=ORIENTED_EDGE('',*,*,#49569,.T.);
#65506=ORIENTED_EDGE('',*,*,#49577,.F.);
#65507=ORIENTED_EDGE('',*,*,#49574,.F.);
#65508=ORIENTED_EDGE('',*,*,#49578,.T.);
#65509=ORIENTED_EDGE('',*,*,#49579,.T.);
#65510=ORIENTED_EDGE('',*,*,#49580,.F.);
#65511=ORIENTED_EDGE('',*,*,#49581,.F.);
#65512=ORIENTED_EDGE('',*,*,#49582,.T.);
#65513=ORIENTED_EDGE('',*,*,#49583,.T.);
#65514=ORIENTED_EDGE('',*,*,#49584,.F.);
#65515=ORIENTED_EDGE('',*,*,#49579,.F.);
#65516=ORIENTED_EDGE('',*,*,#49585,.T.);
#65517=ORIENTED_EDGE('',*,*,#49586,.T.);
#65518=ORIENTED_EDGE('',*,*,#49587,.F.);
#65519=ORIENTED_EDGE('',*,*,#49583,.F.);
#65520=ORIENTED_EDGE('',*,*,#49588,.T.);
#65521=ORIENTED_EDGE('',*,*,#49581,.T.);
#65522=ORIENTED_EDGE('',*,*,#49589,.F.);
#65523=ORIENTED_EDGE('',*,*,#49586,.F.);
#65524=ORIENTED_EDGE('',*,*,#49590,.T.);
#65525=ORIENTED_EDGE('',*,*,#49591,.T.);
#65526=ORIENTED_EDGE('',*,*,#49592,.F.);
#65527=ORIENTED_EDGE('',*,*,#49593,.F.);
#65528=ORIENTED_EDGE('',*,*,#49594,.T.);
#65529=ORIENTED_EDGE('',*,*,#49595,.T.);
#65530=ORIENTED_EDGE('',*,*,#49596,.F.);
#65531=ORIENTED_EDGE('',*,*,#49591,.F.);
#65532=ORIENTED_EDGE('',*,*,#49597,.T.);
#65533=ORIENTED_EDGE('',*,*,#49598,.T.);
#65534=ORIENTED_EDGE('',*,*,#49599,.F.);
#65535=ORIENTED_EDGE('',*,*,#49595,.F.);
#65536=ORIENTED_EDGE('',*,*,#49600,.T.);
#65537=ORIENTED_EDGE('',*,*,#49593,.T.);
#65538=ORIENTED_EDGE('',*,*,#49601,.F.);
#65539=ORIENTED_EDGE('',*,*,#49598,.F.);
#65540=ORIENTED_EDGE('',*,*,#49602,.T.);
#65541=ORIENTED_EDGE('',*,*,#49603,.T.);
#65542=ORIENTED_EDGE('',*,*,#49604,.F.);
#65543=ORIENTED_EDGE('',*,*,#49605,.F.);
#65544=ORIENTED_EDGE('',*,*,#49606,.T.);
#65545=ORIENTED_EDGE('',*,*,#49607,.T.);
#65546=ORIENTED_EDGE('',*,*,#49608,.F.);
#65547=ORIENTED_EDGE('',*,*,#49603,.F.);
#65548=ORIENTED_EDGE('',*,*,#49609,.T.);
#65549=ORIENTED_EDGE('',*,*,#49610,.T.);
#65550=ORIENTED_EDGE('',*,*,#49611,.F.);
#65551=ORIENTED_EDGE('',*,*,#49607,.F.);
#65552=ORIENTED_EDGE('',*,*,#49612,.T.);
#65553=ORIENTED_EDGE('',*,*,#49605,.T.);
#65554=ORIENTED_EDGE('',*,*,#49613,.F.);
#65555=ORIENTED_EDGE('',*,*,#49610,.F.);
#65556=ORIENTED_EDGE('',*,*,#49614,.T.);
#65557=ORIENTED_EDGE('',*,*,#49615,.T.);
#65558=ORIENTED_EDGE('',*,*,#49616,.F.);
#65559=ORIENTED_EDGE('',*,*,#49617,.F.);
#65560=ORIENTED_EDGE('',*,*,#49618,.T.);
#65561=ORIENTED_EDGE('',*,*,#49619,.T.);
#65562=ORIENTED_EDGE('',*,*,#49620,.F.);
#65563=ORIENTED_EDGE('',*,*,#49615,.F.);
#65564=ORIENTED_EDGE('',*,*,#49621,.T.);
#65565=ORIENTED_EDGE('',*,*,#49622,.T.);
#65566=ORIENTED_EDGE('',*,*,#49623,.F.);
#65567=ORIENTED_EDGE('',*,*,#49619,.F.);
#65568=ORIENTED_EDGE('',*,*,#49624,.T.);
#65569=ORIENTED_EDGE('',*,*,#49617,.T.);
#65570=ORIENTED_EDGE('',*,*,#49625,.F.);
#65571=ORIENTED_EDGE('',*,*,#49622,.F.);
#65572=ORIENTED_EDGE('',*,*,#49626,.T.);
#65573=ORIENTED_EDGE('',*,*,#49627,.T.);
#65574=ORIENTED_EDGE('',*,*,#49628,.F.);
#65575=ORIENTED_EDGE('',*,*,#49629,.F.);
#65576=ORIENTED_EDGE('',*,*,#49630,.T.);
#65577=ORIENTED_EDGE('',*,*,#49631,.T.);
#65578=ORIENTED_EDGE('',*,*,#49632,.F.);
#65579=ORIENTED_EDGE('',*,*,#49627,.F.);
#65580=ORIENTED_EDGE('',*,*,#49633,.T.);
#65581=ORIENTED_EDGE('',*,*,#49634,.T.);
#65582=ORIENTED_EDGE('',*,*,#49635,.F.);
#65583=ORIENTED_EDGE('',*,*,#49631,.F.);
#65584=ORIENTED_EDGE('',*,*,#49636,.T.);
#65585=ORIENTED_EDGE('',*,*,#49629,.T.);
#65586=ORIENTED_EDGE('',*,*,#49637,.F.);
#65587=ORIENTED_EDGE('',*,*,#49634,.F.);
#65588=ORIENTED_EDGE('',*,*,#49638,.T.);
#65589=ORIENTED_EDGE('',*,*,#49639,.T.);
#65590=ORIENTED_EDGE('',*,*,#49640,.F.);
#65591=ORIENTED_EDGE('',*,*,#49641,.F.);
#65592=ORIENTED_EDGE('',*,*,#49642,.T.);
#65593=ORIENTED_EDGE('',*,*,#49643,.T.);
#65594=ORIENTED_EDGE('',*,*,#49644,.F.);
#65595=ORIENTED_EDGE('',*,*,#49639,.F.);
#65596=ORIENTED_EDGE('',*,*,#49645,.T.);
#65597=ORIENTED_EDGE('',*,*,#49646,.T.);
#65598=ORIENTED_EDGE('',*,*,#49647,.F.);
#65599=ORIENTED_EDGE('',*,*,#49643,.F.);
#65600=ORIENTED_EDGE('',*,*,#49648,.T.);
#65601=ORIENTED_EDGE('',*,*,#49641,.T.);
#65602=ORIENTED_EDGE('',*,*,#49649,.F.);
#65603=ORIENTED_EDGE('',*,*,#49646,.F.);
#65604=ORIENTED_EDGE('',*,*,#49650,.T.);
#65605=ORIENTED_EDGE('',*,*,#49651,.T.);
#65606=ORIENTED_EDGE('',*,*,#49652,.F.);
#65607=ORIENTED_EDGE('',*,*,#49653,.F.);
#65608=ORIENTED_EDGE('',*,*,#49654,.T.);
#65609=ORIENTED_EDGE('',*,*,#49655,.T.);
#65610=ORIENTED_EDGE('',*,*,#49656,.F.);
#65611=ORIENTED_EDGE('',*,*,#49651,.F.);
#65612=ORIENTED_EDGE('',*,*,#49657,.T.);
#65613=ORIENTED_EDGE('',*,*,#49658,.T.);
#65614=ORIENTED_EDGE('',*,*,#49659,.F.);
#65615=ORIENTED_EDGE('',*,*,#49655,.F.);
#65616=ORIENTED_EDGE('',*,*,#49660,.T.);
#65617=ORIENTED_EDGE('',*,*,#49653,.T.);
#65618=ORIENTED_EDGE('',*,*,#49661,.F.);
#65619=ORIENTED_EDGE('',*,*,#49658,.F.);
#65620=ORIENTED_EDGE('',*,*,#49662,.T.);
#65621=ORIENTED_EDGE('',*,*,#49663,.T.);
#65622=ORIENTED_EDGE('',*,*,#49664,.F.);
#65623=ORIENTED_EDGE('',*,*,#49665,.F.);
#65624=ORIENTED_EDGE('',*,*,#49666,.T.);
#65625=ORIENTED_EDGE('',*,*,#49667,.T.);
#65626=ORIENTED_EDGE('',*,*,#49668,.F.);
#65627=ORIENTED_EDGE('',*,*,#49663,.F.);
#65628=ORIENTED_EDGE('',*,*,#49669,.T.);
#65629=ORIENTED_EDGE('',*,*,#49670,.T.);
#65630=ORIENTED_EDGE('',*,*,#49671,.F.);
#65631=ORIENTED_EDGE('',*,*,#49667,.F.);
#65632=ORIENTED_EDGE('',*,*,#49672,.T.);
#65633=ORIENTED_EDGE('',*,*,#49665,.T.);
#65634=ORIENTED_EDGE('',*,*,#49673,.F.);
#65635=ORIENTED_EDGE('',*,*,#49670,.F.);
#65636=ORIENTED_EDGE('',*,*,#49674,.T.);
#65637=ORIENTED_EDGE('',*,*,#49675,.T.);
#65638=ORIENTED_EDGE('',*,*,#49676,.F.);
#65639=ORIENTED_EDGE('',*,*,#49677,.F.);
#65640=ORIENTED_EDGE('',*,*,#49678,.T.);
#65641=ORIENTED_EDGE('',*,*,#49679,.T.);
#65642=ORIENTED_EDGE('',*,*,#49680,.F.);
#65643=ORIENTED_EDGE('',*,*,#49675,.F.);
#65644=ORIENTED_EDGE('',*,*,#49681,.T.);
#65645=ORIENTED_EDGE('',*,*,#49682,.T.);
#65646=ORIENTED_EDGE('',*,*,#49683,.F.);
#65647=ORIENTED_EDGE('',*,*,#49679,.F.);
#65648=ORIENTED_EDGE('',*,*,#49684,.T.);
#65649=ORIENTED_EDGE('',*,*,#49677,.T.);
#65650=ORIENTED_EDGE('',*,*,#49685,.F.);
#65651=ORIENTED_EDGE('',*,*,#49682,.F.);
#65652=ORIENTED_EDGE('',*,*,#49686,.T.);
#65653=ORIENTED_EDGE('',*,*,#49687,.T.);
#65654=ORIENTED_EDGE('',*,*,#49688,.F.);
#65655=ORIENTED_EDGE('',*,*,#49689,.F.);
#65656=ORIENTED_EDGE('',*,*,#49690,.T.);
#65657=ORIENTED_EDGE('',*,*,#49691,.T.);
#65658=ORIENTED_EDGE('',*,*,#49692,.F.);
#65659=ORIENTED_EDGE('',*,*,#49687,.F.);
#65660=ORIENTED_EDGE('',*,*,#49693,.T.);
#65661=ORIENTED_EDGE('',*,*,#49694,.T.);
#65662=ORIENTED_EDGE('',*,*,#49695,.F.);
#65663=ORIENTED_EDGE('',*,*,#49691,.F.);
#65664=ORIENTED_EDGE('',*,*,#49696,.T.);
#65665=ORIENTED_EDGE('',*,*,#49689,.T.);
#65666=ORIENTED_EDGE('',*,*,#49697,.F.);
#65667=ORIENTED_EDGE('',*,*,#49694,.F.);
#65668=ORIENTED_EDGE('',*,*,#49698,.T.);
#65669=ORIENTED_EDGE('',*,*,#49699,.T.);
#65670=ORIENTED_EDGE('',*,*,#49700,.F.);
#65671=ORIENTED_EDGE('',*,*,#49701,.F.);
#65672=ORIENTED_EDGE('',*,*,#49702,.T.);
#65673=ORIENTED_EDGE('',*,*,#49703,.T.);
#65674=ORIENTED_EDGE('',*,*,#49704,.F.);
#65675=ORIENTED_EDGE('',*,*,#49699,.F.);
#65676=ORIENTED_EDGE('',*,*,#49705,.T.);
#65677=ORIENTED_EDGE('',*,*,#49706,.T.);
#65678=ORIENTED_EDGE('',*,*,#49707,.F.);
#65679=ORIENTED_EDGE('',*,*,#49703,.F.);
#65680=ORIENTED_EDGE('',*,*,#49708,.T.);
#65681=ORIENTED_EDGE('',*,*,#49701,.T.);
#65682=ORIENTED_EDGE('',*,*,#49709,.F.);
#65683=ORIENTED_EDGE('',*,*,#49706,.F.);
#65684=ORIENTED_EDGE('',*,*,#49710,.T.);
#65685=ORIENTED_EDGE('',*,*,#49711,.T.);
#65686=ORIENTED_EDGE('',*,*,#49712,.F.);
#65687=ORIENTED_EDGE('',*,*,#49713,.F.);
#65688=ORIENTED_EDGE('',*,*,#49714,.T.);
#65689=ORIENTED_EDGE('',*,*,#49715,.T.);
#65690=ORIENTED_EDGE('',*,*,#49716,.F.);
#65691=ORIENTED_EDGE('',*,*,#49711,.F.);
#65692=ORIENTED_EDGE('',*,*,#49717,.T.);
#65693=ORIENTED_EDGE('',*,*,#49718,.T.);
#65694=ORIENTED_EDGE('',*,*,#49719,.F.);
#65695=ORIENTED_EDGE('',*,*,#49715,.F.);
#65696=ORIENTED_EDGE('',*,*,#49720,.T.);
#65697=ORIENTED_EDGE('',*,*,#49713,.T.);
#65698=ORIENTED_EDGE('',*,*,#49721,.F.);
#65699=ORIENTED_EDGE('',*,*,#49718,.F.);
#65700=ORIENTED_EDGE('',*,*,#49722,.T.);
#65701=ORIENTED_EDGE('',*,*,#49723,.T.);
#65702=ORIENTED_EDGE('',*,*,#49724,.F.);
#65703=ORIENTED_EDGE('',*,*,#49725,.F.);
#65704=ORIENTED_EDGE('',*,*,#49726,.T.);
#65705=ORIENTED_EDGE('',*,*,#49727,.T.);
#65706=ORIENTED_EDGE('',*,*,#49728,.F.);
#65707=ORIENTED_EDGE('',*,*,#49723,.F.);
#65708=ORIENTED_EDGE('',*,*,#49729,.T.);
#65709=ORIENTED_EDGE('',*,*,#49730,.T.);
#65710=ORIENTED_EDGE('',*,*,#49731,.F.);
#65711=ORIENTED_EDGE('',*,*,#49727,.F.);
#65712=ORIENTED_EDGE('',*,*,#49732,.T.);
#65713=ORIENTED_EDGE('',*,*,#49725,.T.);
#65714=ORIENTED_EDGE('',*,*,#49733,.F.);
#65715=ORIENTED_EDGE('',*,*,#49730,.F.);
#65716=ORIENTED_EDGE('',*,*,#49734,.T.);
#65717=ORIENTED_EDGE('',*,*,#49735,.T.);
#65718=ORIENTED_EDGE('',*,*,#49736,.F.);
#65719=ORIENTED_EDGE('',*,*,#49737,.F.);
#65720=ORIENTED_EDGE('',*,*,#49738,.T.);
#65721=ORIENTED_EDGE('',*,*,#49739,.T.);
#65722=ORIENTED_EDGE('',*,*,#49740,.F.);
#65723=ORIENTED_EDGE('',*,*,#49735,.F.);
#65724=ORIENTED_EDGE('',*,*,#49741,.T.);
#65725=ORIENTED_EDGE('',*,*,#49742,.T.);
#65726=ORIENTED_EDGE('',*,*,#49743,.F.);
#65727=ORIENTED_EDGE('',*,*,#49739,.F.);
#65728=ORIENTED_EDGE('',*,*,#49744,.T.);
#65729=ORIENTED_EDGE('',*,*,#49737,.T.);
#65730=ORIENTED_EDGE('',*,*,#49745,.F.);
#65731=ORIENTED_EDGE('',*,*,#49742,.F.);
#65732=ORIENTED_EDGE('',*,*,#49746,.T.);
#65733=ORIENTED_EDGE('',*,*,#49747,.T.);
#65734=ORIENTED_EDGE('',*,*,#49748,.F.);
#65735=ORIENTED_EDGE('',*,*,#49749,.F.);
#65736=ORIENTED_EDGE('',*,*,#49750,.T.);
#65737=ORIENTED_EDGE('',*,*,#49751,.T.);
#65738=ORIENTED_EDGE('',*,*,#49752,.F.);
#65739=ORIENTED_EDGE('',*,*,#49747,.F.);
#65740=ORIENTED_EDGE('',*,*,#49753,.T.);
#65741=ORIENTED_EDGE('',*,*,#49754,.T.);
#65742=ORIENTED_EDGE('',*,*,#49755,.F.);
#65743=ORIENTED_EDGE('',*,*,#49751,.F.);
#65744=ORIENTED_EDGE('',*,*,#49756,.T.);
#65745=ORIENTED_EDGE('',*,*,#49749,.T.);
#65746=ORIENTED_EDGE('',*,*,#49757,.F.);
#65747=ORIENTED_EDGE('',*,*,#49754,.F.);
#65748=ORIENTED_EDGE('',*,*,#49758,.T.);
#65749=ORIENTED_EDGE('',*,*,#49759,.T.);
#65750=ORIENTED_EDGE('',*,*,#49760,.F.);
#65751=ORIENTED_EDGE('',*,*,#49761,.F.);
#65752=ORIENTED_EDGE('',*,*,#49762,.T.);
#65753=ORIENTED_EDGE('',*,*,#49763,.T.);
#65754=ORIENTED_EDGE('',*,*,#49764,.F.);
#65755=ORIENTED_EDGE('',*,*,#49759,.F.);
#65756=ORIENTED_EDGE('',*,*,#49765,.T.);
#65757=ORIENTED_EDGE('',*,*,#49766,.T.);
#65758=ORIENTED_EDGE('',*,*,#49767,.F.);
#65759=ORIENTED_EDGE('',*,*,#49763,.F.);
#65760=ORIENTED_EDGE('',*,*,#49768,.T.);
#65761=ORIENTED_EDGE('',*,*,#49761,.T.);
#65762=ORIENTED_EDGE('',*,*,#49769,.F.);
#65763=ORIENTED_EDGE('',*,*,#49766,.F.);
#65764=ORIENTED_EDGE('',*,*,#49770,.T.);
#65765=ORIENTED_EDGE('',*,*,#49771,.T.);
#65766=ORIENTED_EDGE('',*,*,#49772,.F.);
#65767=ORIENTED_EDGE('',*,*,#49773,.F.);
#65768=ORIENTED_EDGE('',*,*,#49774,.T.);
#65769=ORIENTED_EDGE('',*,*,#49775,.T.);
#65770=ORIENTED_EDGE('',*,*,#49776,.F.);
#65771=ORIENTED_EDGE('',*,*,#49771,.F.);
#65772=ORIENTED_EDGE('',*,*,#49777,.T.);
#65773=ORIENTED_EDGE('',*,*,#49778,.T.);
#65774=ORIENTED_EDGE('',*,*,#49779,.F.);
#65775=ORIENTED_EDGE('',*,*,#49775,.F.);
#65776=ORIENTED_EDGE('',*,*,#49780,.T.);
#65777=ORIENTED_EDGE('',*,*,#49773,.T.);
#65778=ORIENTED_EDGE('',*,*,#49781,.F.);
#65779=ORIENTED_EDGE('',*,*,#49778,.F.);
#65780=ORIENTED_EDGE('',*,*,#49782,.T.);
#65781=ORIENTED_EDGE('',*,*,#49783,.T.);
#65782=ORIENTED_EDGE('',*,*,#49784,.F.);
#65783=ORIENTED_EDGE('',*,*,#49785,.F.);
#65784=ORIENTED_EDGE('',*,*,#49786,.T.);
#65785=ORIENTED_EDGE('',*,*,#49787,.T.);
#65786=ORIENTED_EDGE('',*,*,#49788,.F.);
#65787=ORIENTED_EDGE('',*,*,#49783,.F.);
#65788=ORIENTED_EDGE('',*,*,#49789,.T.);
#65789=ORIENTED_EDGE('',*,*,#49790,.T.);
#65790=ORIENTED_EDGE('',*,*,#49791,.F.);
#65791=ORIENTED_EDGE('',*,*,#49787,.F.);
#65792=ORIENTED_EDGE('',*,*,#49792,.T.);
#65793=ORIENTED_EDGE('',*,*,#49785,.T.);
#65794=ORIENTED_EDGE('',*,*,#49793,.F.);
#65795=ORIENTED_EDGE('',*,*,#49790,.F.);
#65796=ORIENTED_EDGE('',*,*,#49794,.T.);
#65797=ORIENTED_EDGE('',*,*,#49795,.T.);
#65798=ORIENTED_EDGE('',*,*,#49796,.F.);
#65799=ORIENTED_EDGE('',*,*,#49797,.F.);
#65800=ORIENTED_EDGE('',*,*,#49798,.T.);
#65801=ORIENTED_EDGE('',*,*,#49799,.T.);
#65802=ORIENTED_EDGE('',*,*,#49800,.F.);
#65803=ORIENTED_EDGE('',*,*,#49795,.F.);
#65804=ORIENTED_EDGE('',*,*,#49801,.T.);
#65805=ORIENTED_EDGE('',*,*,#49802,.T.);
#65806=ORIENTED_EDGE('',*,*,#49803,.F.);
#65807=ORIENTED_EDGE('',*,*,#49799,.F.);
#65808=ORIENTED_EDGE('',*,*,#49804,.T.);
#65809=ORIENTED_EDGE('',*,*,#49797,.T.);
#65810=ORIENTED_EDGE('',*,*,#49805,.F.);
#65811=ORIENTED_EDGE('',*,*,#49802,.F.);
#65812=ORIENTED_EDGE('',*,*,#49806,.T.);
#65813=ORIENTED_EDGE('',*,*,#49807,.T.);
#65814=ORIENTED_EDGE('',*,*,#49808,.F.);
#65815=ORIENTED_EDGE('',*,*,#49809,.F.);
#65816=ORIENTED_EDGE('',*,*,#49810,.T.);
#65817=ORIENTED_EDGE('',*,*,#49811,.T.);
#65818=ORIENTED_EDGE('',*,*,#49812,.F.);
#65819=ORIENTED_EDGE('',*,*,#49807,.F.);
#65820=ORIENTED_EDGE('',*,*,#49813,.T.);
#65821=ORIENTED_EDGE('',*,*,#49814,.T.);
#65822=ORIENTED_EDGE('',*,*,#49815,.F.);
#65823=ORIENTED_EDGE('',*,*,#49811,.F.);
#65824=ORIENTED_EDGE('',*,*,#49816,.T.);
#65825=ORIENTED_EDGE('',*,*,#49809,.T.);
#65826=ORIENTED_EDGE('',*,*,#49817,.F.);
#65827=ORIENTED_EDGE('',*,*,#49814,.F.);
#65828=ORIENTED_EDGE('',*,*,#49818,.T.);
#65829=ORIENTED_EDGE('',*,*,#49819,.T.);
#65830=ORIENTED_EDGE('',*,*,#49820,.F.);
#65831=ORIENTED_EDGE('',*,*,#49821,.F.);
#65832=ORIENTED_EDGE('',*,*,#49822,.T.);
#65833=ORIENTED_EDGE('',*,*,#49823,.T.);
#65834=ORIENTED_EDGE('',*,*,#49824,.F.);
#65835=ORIENTED_EDGE('',*,*,#49819,.F.);
#65836=ORIENTED_EDGE('',*,*,#49825,.T.);
#65837=ORIENTED_EDGE('',*,*,#49826,.T.);
#65838=ORIENTED_EDGE('',*,*,#49827,.F.);
#65839=ORIENTED_EDGE('',*,*,#49823,.F.);
#65840=ORIENTED_EDGE('',*,*,#49828,.T.);
#65841=ORIENTED_EDGE('',*,*,#49821,.T.);
#65842=ORIENTED_EDGE('',*,*,#49829,.F.);
#65843=ORIENTED_EDGE('',*,*,#49826,.F.);
#65844=ORIENTED_EDGE('',*,*,#49830,.T.);
#65845=ORIENTED_EDGE('',*,*,#49831,.T.);
#65846=ORIENTED_EDGE('',*,*,#49832,.F.);
#65847=ORIENTED_EDGE('',*,*,#49833,.F.);
#65848=ORIENTED_EDGE('',*,*,#49834,.T.);
#65849=ORIENTED_EDGE('',*,*,#49835,.T.);
#65850=ORIENTED_EDGE('',*,*,#49836,.F.);
#65851=ORIENTED_EDGE('',*,*,#49831,.F.);
#65852=ORIENTED_EDGE('',*,*,#49837,.T.);
#65853=ORIENTED_EDGE('',*,*,#49838,.T.);
#65854=ORIENTED_EDGE('',*,*,#49839,.F.);
#65855=ORIENTED_EDGE('',*,*,#49835,.F.);
#65856=ORIENTED_EDGE('',*,*,#49840,.T.);
#65857=ORIENTED_EDGE('',*,*,#49833,.T.);
#65858=ORIENTED_EDGE('',*,*,#49841,.F.);
#65859=ORIENTED_EDGE('',*,*,#49838,.F.);
#65860=ORIENTED_EDGE('',*,*,#49842,.T.);
#65861=ORIENTED_EDGE('',*,*,#49843,.T.);
#65862=ORIENTED_EDGE('',*,*,#49844,.F.);
#65863=ORIENTED_EDGE('',*,*,#49845,.F.);
#65864=ORIENTED_EDGE('',*,*,#49846,.T.);
#65865=ORIENTED_EDGE('',*,*,#49847,.T.);
#65866=ORIENTED_EDGE('',*,*,#49848,.F.);
#65867=ORIENTED_EDGE('',*,*,#49843,.F.);
#65868=ORIENTED_EDGE('',*,*,#49849,.T.);
#65869=ORIENTED_EDGE('',*,*,#49850,.T.);
#65870=ORIENTED_EDGE('',*,*,#49851,.F.);
#65871=ORIENTED_EDGE('',*,*,#49847,.F.);
#65872=ORIENTED_EDGE('',*,*,#49852,.T.);
#65873=ORIENTED_EDGE('',*,*,#49845,.T.);
#65874=ORIENTED_EDGE('',*,*,#49853,.F.);
#65875=ORIENTED_EDGE('',*,*,#49850,.F.);
#65876=ORIENTED_EDGE('',*,*,#49854,.T.);
#65877=ORIENTED_EDGE('',*,*,#49855,.T.);
#65878=ORIENTED_EDGE('',*,*,#49856,.F.);
#65879=ORIENTED_EDGE('',*,*,#49857,.F.);
#65880=ORIENTED_EDGE('',*,*,#49858,.T.);
#65881=ORIENTED_EDGE('',*,*,#49859,.T.);
#65882=ORIENTED_EDGE('',*,*,#49860,.F.);
#65883=ORIENTED_EDGE('',*,*,#49855,.F.);
#65884=ORIENTED_EDGE('',*,*,#49861,.T.);
#65885=ORIENTED_EDGE('',*,*,#49862,.T.);
#65886=ORIENTED_EDGE('',*,*,#49863,.F.);
#65887=ORIENTED_EDGE('',*,*,#49859,.F.);
#65888=ORIENTED_EDGE('',*,*,#49864,.T.);
#65889=ORIENTED_EDGE('',*,*,#49857,.T.);
#65890=ORIENTED_EDGE('',*,*,#49865,.F.);
#65891=ORIENTED_EDGE('',*,*,#49862,.F.);
#65892=ORIENTED_EDGE('',*,*,#49866,.T.);
#65893=ORIENTED_EDGE('',*,*,#49867,.T.);
#65894=ORIENTED_EDGE('',*,*,#49868,.F.);
#65895=ORIENTED_EDGE('',*,*,#49869,.F.);
#65896=ORIENTED_EDGE('',*,*,#49870,.T.);
#65897=ORIENTED_EDGE('',*,*,#49871,.T.);
#65898=ORIENTED_EDGE('',*,*,#49872,.F.);
#65899=ORIENTED_EDGE('',*,*,#49867,.F.);
#65900=ORIENTED_EDGE('',*,*,#49873,.T.);
#65901=ORIENTED_EDGE('',*,*,#49874,.T.);
#65902=ORIENTED_EDGE('',*,*,#49875,.F.);
#65903=ORIENTED_EDGE('',*,*,#49871,.F.);
#65904=ORIENTED_EDGE('',*,*,#49876,.T.);
#65905=ORIENTED_EDGE('',*,*,#49869,.T.);
#65906=ORIENTED_EDGE('',*,*,#49877,.F.);
#65907=ORIENTED_EDGE('',*,*,#49874,.F.);
#65908=ORIENTED_EDGE('',*,*,#49878,.T.);
#65909=ORIENTED_EDGE('',*,*,#49879,.T.);
#65910=ORIENTED_EDGE('',*,*,#49880,.F.);
#65911=ORIENTED_EDGE('',*,*,#49881,.F.);
#65912=ORIENTED_EDGE('',*,*,#49882,.T.);
#65913=ORIENTED_EDGE('',*,*,#49883,.T.);
#65914=ORIENTED_EDGE('',*,*,#49884,.F.);
#65915=ORIENTED_EDGE('',*,*,#49879,.F.);
#65916=ORIENTED_EDGE('',*,*,#49885,.T.);
#65917=ORIENTED_EDGE('',*,*,#49886,.T.);
#65918=ORIENTED_EDGE('',*,*,#49887,.F.);
#65919=ORIENTED_EDGE('',*,*,#49883,.F.);
#65920=ORIENTED_EDGE('',*,*,#49888,.T.);
#65921=ORIENTED_EDGE('',*,*,#49881,.T.);
#65922=ORIENTED_EDGE('',*,*,#49889,.F.);
#65923=ORIENTED_EDGE('',*,*,#49886,.F.);
#65924=ORIENTED_EDGE('',*,*,#49890,.T.);
#65925=ORIENTED_EDGE('',*,*,#49891,.T.);
#65926=ORIENTED_EDGE('',*,*,#49892,.F.);
#65927=ORIENTED_EDGE('',*,*,#49893,.F.);
#65928=ORIENTED_EDGE('',*,*,#49894,.T.);
#65929=ORIENTED_EDGE('',*,*,#49895,.T.);
#65930=ORIENTED_EDGE('',*,*,#49896,.F.);
#65931=ORIENTED_EDGE('',*,*,#49891,.F.);
#65932=ORIENTED_EDGE('',*,*,#49897,.T.);
#65933=ORIENTED_EDGE('',*,*,#49898,.T.);
#65934=ORIENTED_EDGE('',*,*,#49899,.F.);
#65935=ORIENTED_EDGE('',*,*,#49895,.F.);
#65936=ORIENTED_EDGE('',*,*,#49900,.T.);
#65937=ORIENTED_EDGE('',*,*,#49893,.T.);
#65938=ORIENTED_EDGE('',*,*,#49901,.F.);
#65939=ORIENTED_EDGE('',*,*,#49898,.F.);
#65940=ORIENTED_EDGE('',*,*,#49902,.T.);
#65941=ORIENTED_EDGE('',*,*,#49903,.T.);
#65942=ORIENTED_EDGE('',*,*,#49904,.F.);
#65943=ORIENTED_EDGE('',*,*,#49905,.F.);
#65944=ORIENTED_EDGE('',*,*,#49906,.T.);
#65945=ORIENTED_EDGE('',*,*,#49907,.T.);
#65946=ORIENTED_EDGE('',*,*,#49908,.F.);
#65947=ORIENTED_EDGE('',*,*,#49903,.F.);
#65948=ORIENTED_EDGE('',*,*,#49909,.T.);
#65949=ORIENTED_EDGE('',*,*,#49910,.T.);
#65950=ORIENTED_EDGE('',*,*,#49911,.F.);
#65951=ORIENTED_EDGE('',*,*,#49907,.F.);
#65952=ORIENTED_EDGE('',*,*,#49912,.T.);
#65953=ORIENTED_EDGE('',*,*,#49905,.T.);
#65954=ORIENTED_EDGE('',*,*,#49913,.F.);
#65955=ORIENTED_EDGE('',*,*,#49910,.F.);
#65956=ORIENTED_EDGE('',*,*,#49914,.T.);
#65957=ORIENTED_EDGE('',*,*,#49915,.T.);
#65958=ORIENTED_EDGE('',*,*,#49916,.F.);
#65959=ORIENTED_EDGE('',*,*,#49917,.F.);
#65960=ORIENTED_EDGE('',*,*,#49918,.T.);
#65961=ORIENTED_EDGE('',*,*,#49919,.T.);
#65962=ORIENTED_EDGE('',*,*,#49920,.F.);
#65963=ORIENTED_EDGE('',*,*,#49915,.F.);
#65964=ORIENTED_EDGE('',*,*,#49921,.T.);
#65965=ORIENTED_EDGE('',*,*,#49922,.T.);
#65966=ORIENTED_EDGE('',*,*,#49923,.F.);
#65967=ORIENTED_EDGE('',*,*,#49919,.F.);
#65968=ORIENTED_EDGE('',*,*,#49924,.T.);
#65969=ORIENTED_EDGE('',*,*,#49917,.T.);
#65970=ORIENTED_EDGE('',*,*,#49925,.F.);
#65971=ORIENTED_EDGE('',*,*,#49922,.F.);
#65972=ORIENTED_EDGE('',*,*,#49926,.T.);
#65973=ORIENTED_EDGE('',*,*,#49927,.T.);
#65974=ORIENTED_EDGE('',*,*,#49928,.F.);
#65975=ORIENTED_EDGE('',*,*,#49929,.F.);
#65976=ORIENTED_EDGE('',*,*,#49930,.T.);
#65977=ORIENTED_EDGE('',*,*,#49931,.T.);
#65978=ORIENTED_EDGE('',*,*,#49932,.F.);
#65979=ORIENTED_EDGE('',*,*,#49927,.F.);
#65980=ORIENTED_EDGE('',*,*,#49933,.T.);
#65981=ORIENTED_EDGE('',*,*,#49934,.T.);
#65982=ORIENTED_EDGE('',*,*,#49935,.F.);
#65983=ORIENTED_EDGE('',*,*,#49931,.F.);
#65984=ORIENTED_EDGE('',*,*,#49936,.T.);
#65985=ORIENTED_EDGE('',*,*,#49929,.T.);
#65986=ORIENTED_EDGE('',*,*,#49937,.F.);
#65987=ORIENTED_EDGE('',*,*,#49934,.F.);
#65988=ORIENTED_EDGE('',*,*,#49938,.T.);
#65989=ORIENTED_EDGE('',*,*,#49939,.T.);
#65990=ORIENTED_EDGE('',*,*,#49940,.F.);
#65991=ORIENTED_EDGE('',*,*,#49941,.F.);
#65992=ORIENTED_EDGE('',*,*,#49942,.T.);
#65993=ORIENTED_EDGE('',*,*,#49943,.T.);
#65994=ORIENTED_EDGE('',*,*,#49944,.F.);
#65995=ORIENTED_EDGE('',*,*,#49939,.F.);
#65996=ORIENTED_EDGE('',*,*,#49945,.T.);
#65997=ORIENTED_EDGE('',*,*,#49946,.T.);
#65998=ORIENTED_EDGE('',*,*,#49947,.F.);
#65999=ORIENTED_EDGE('',*,*,#49943,.F.);
#66000=ORIENTED_EDGE('',*,*,#49948,.T.);
#66001=ORIENTED_EDGE('',*,*,#49941,.T.);
#66002=ORIENTED_EDGE('',*,*,#49949,.F.);
#66003=ORIENTED_EDGE('',*,*,#49946,.F.);
#66004=ORIENTED_EDGE('',*,*,#49950,.T.);
#66005=ORIENTED_EDGE('',*,*,#49951,.T.);
#66006=ORIENTED_EDGE('',*,*,#49952,.F.);
#66007=ORIENTED_EDGE('',*,*,#49953,.F.);
#66008=ORIENTED_EDGE('',*,*,#49954,.T.);
#66009=ORIENTED_EDGE('',*,*,#49955,.T.);
#66010=ORIENTED_EDGE('',*,*,#49956,.F.);
#66011=ORIENTED_EDGE('',*,*,#49951,.F.);
#66012=ORIENTED_EDGE('',*,*,#49957,.T.);
#66013=ORIENTED_EDGE('',*,*,#49958,.T.);
#66014=ORIENTED_EDGE('',*,*,#49959,.F.);
#66015=ORIENTED_EDGE('',*,*,#49955,.F.);
#66016=ORIENTED_EDGE('',*,*,#49960,.T.);
#66017=ORIENTED_EDGE('',*,*,#49953,.T.);
#66018=ORIENTED_EDGE('',*,*,#49961,.F.);
#66019=ORIENTED_EDGE('',*,*,#49958,.F.);
#66020=ORIENTED_EDGE('',*,*,#49962,.T.);
#66021=ORIENTED_EDGE('',*,*,#49963,.T.);
#66022=ORIENTED_EDGE('',*,*,#49964,.F.);
#66023=ORIENTED_EDGE('',*,*,#49965,.F.);
#66024=ORIENTED_EDGE('',*,*,#49966,.T.);
#66025=ORIENTED_EDGE('',*,*,#49967,.T.);
#66026=ORIENTED_EDGE('',*,*,#49968,.F.);
#66027=ORIENTED_EDGE('',*,*,#49963,.F.);
#66028=ORIENTED_EDGE('',*,*,#49969,.T.);
#66029=ORIENTED_EDGE('',*,*,#49970,.T.);
#66030=ORIENTED_EDGE('',*,*,#49971,.F.);
#66031=ORIENTED_EDGE('',*,*,#49967,.F.);
#66032=ORIENTED_EDGE('',*,*,#49972,.T.);
#66033=ORIENTED_EDGE('',*,*,#49965,.T.);
#66034=ORIENTED_EDGE('',*,*,#49973,.F.);
#66035=ORIENTED_EDGE('',*,*,#49970,.F.);
#66036=ORIENTED_EDGE('',*,*,#49974,.T.);
#66037=ORIENTED_EDGE('',*,*,#49975,.T.);
#66038=ORIENTED_EDGE('',*,*,#49976,.F.);
#66039=ORIENTED_EDGE('',*,*,#49977,.F.);
#66040=ORIENTED_EDGE('',*,*,#49978,.T.);
#66041=ORIENTED_EDGE('',*,*,#49979,.T.);
#66042=ORIENTED_EDGE('',*,*,#49980,.F.);
#66043=ORIENTED_EDGE('',*,*,#49975,.F.);
#66044=ORIENTED_EDGE('',*,*,#49981,.T.);
#66045=ORIENTED_EDGE('',*,*,#49982,.T.);
#66046=ORIENTED_EDGE('',*,*,#49983,.F.);
#66047=ORIENTED_EDGE('',*,*,#49979,.F.);
#66048=ORIENTED_EDGE('',*,*,#49984,.T.);
#66049=ORIENTED_EDGE('',*,*,#49977,.T.);
#66050=ORIENTED_EDGE('',*,*,#49985,.F.);
#66051=ORIENTED_EDGE('',*,*,#49982,.F.);
#66052=ORIENTED_EDGE('',*,*,#49986,.T.);
#66053=ORIENTED_EDGE('',*,*,#49987,.T.);
#66054=ORIENTED_EDGE('',*,*,#49988,.F.);
#66055=ORIENTED_EDGE('',*,*,#49989,.F.);
#66056=ORIENTED_EDGE('',*,*,#49990,.T.);
#66057=ORIENTED_EDGE('',*,*,#49991,.T.);
#66058=ORIENTED_EDGE('',*,*,#49992,.F.);
#66059=ORIENTED_EDGE('',*,*,#49987,.F.);
#66060=ORIENTED_EDGE('',*,*,#49993,.T.);
#66061=ORIENTED_EDGE('',*,*,#49994,.T.);
#66062=ORIENTED_EDGE('',*,*,#49995,.F.);
#66063=ORIENTED_EDGE('',*,*,#49991,.F.);
#66064=ORIENTED_EDGE('',*,*,#49996,.T.);
#66065=ORIENTED_EDGE('',*,*,#49989,.T.);
#66066=ORIENTED_EDGE('',*,*,#49997,.F.);
#66067=ORIENTED_EDGE('',*,*,#49994,.F.);
#66068=ORIENTED_EDGE('',*,*,#49998,.T.);
#66069=ORIENTED_EDGE('',*,*,#49999,.T.);
#66070=ORIENTED_EDGE('',*,*,#50000,.F.);
#66071=ORIENTED_EDGE('',*,*,#50001,.F.);
#66072=ORIENTED_EDGE('',*,*,#50002,.T.);
#66073=ORIENTED_EDGE('',*,*,#50003,.T.);
#66074=ORIENTED_EDGE('',*,*,#50004,.F.);
#66075=ORIENTED_EDGE('',*,*,#49999,.F.);
#66076=ORIENTED_EDGE('',*,*,#50005,.T.);
#66077=ORIENTED_EDGE('',*,*,#50006,.T.);
#66078=ORIENTED_EDGE('',*,*,#50007,.F.);
#66079=ORIENTED_EDGE('',*,*,#50003,.F.);
#66080=ORIENTED_EDGE('',*,*,#50008,.T.);
#66081=ORIENTED_EDGE('',*,*,#50001,.T.);
#66082=ORIENTED_EDGE('',*,*,#50009,.F.);
#66083=ORIENTED_EDGE('',*,*,#50006,.F.);
#66084=ORIENTED_EDGE('',*,*,#50010,.T.);
#66085=ORIENTED_EDGE('',*,*,#50011,.T.);
#66086=ORIENTED_EDGE('',*,*,#50012,.F.);
#66087=ORIENTED_EDGE('',*,*,#50013,.F.);
#66088=ORIENTED_EDGE('',*,*,#50014,.T.);
#66089=ORIENTED_EDGE('',*,*,#50015,.T.);
#66090=ORIENTED_EDGE('',*,*,#50016,.F.);
#66091=ORIENTED_EDGE('',*,*,#50011,.F.);
#66092=ORIENTED_EDGE('',*,*,#50017,.T.);
#66093=ORIENTED_EDGE('',*,*,#50018,.T.);
#66094=ORIENTED_EDGE('',*,*,#50019,.F.);
#66095=ORIENTED_EDGE('',*,*,#50015,.F.);
#66096=ORIENTED_EDGE('',*,*,#50020,.T.);
#66097=ORIENTED_EDGE('',*,*,#50013,.T.);
#66098=ORIENTED_EDGE('',*,*,#50021,.F.);
#66099=ORIENTED_EDGE('',*,*,#50018,.F.);
#66100=ORIENTED_EDGE('',*,*,#50022,.T.);
#66101=ORIENTED_EDGE('',*,*,#50023,.T.);
#66102=ORIENTED_EDGE('',*,*,#50024,.F.);
#66103=ORIENTED_EDGE('',*,*,#50025,.F.);
#66104=ORIENTED_EDGE('',*,*,#50026,.T.);
#66105=ORIENTED_EDGE('',*,*,#50027,.T.);
#66106=ORIENTED_EDGE('',*,*,#50028,.F.);
#66107=ORIENTED_EDGE('',*,*,#50023,.F.);
#66108=ORIENTED_EDGE('',*,*,#50029,.T.);
#66109=ORIENTED_EDGE('',*,*,#50030,.T.);
#66110=ORIENTED_EDGE('',*,*,#50031,.F.);
#66111=ORIENTED_EDGE('',*,*,#50027,.F.);
#66112=ORIENTED_EDGE('',*,*,#50032,.T.);
#66113=ORIENTED_EDGE('',*,*,#50025,.T.);
#66114=ORIENTED_EDGE('',*,*,#50033,.F.);
#66115=ORIENTED_EDGE('',*,*,#50030,.F.);
#66116=ORIENTED_EDGE('',*,*,#50034,.T.);
#66117=ORIENTED_EDGE('',*,*,#50035,.T.);
#66118=ORIENTED_EDGE('',*,*,#50036,.F.);
#66119=ORIENTED_EDGE('',*,*,#50037,.F.);
#66120=ORIENTED_EDGE('',*,*,#50038,.T.);
#66121=ORIENTED_EDGE('',*,*,#50039,.T.);
#66122=ORIENTED_EDGE('',*,*,#50040,.F.);
#66123=ORIENTED_EDGE('',*,*,#50035,.F.);
#66124=ORIENTED_EDGE('',*,*,#50041,.T.);
#66125=ORIENTED_EDGE('',*,*,#50042,.T.);
#66126=ORIENTED_EDGE('',*,*,#50043,.F.);
#66127=ORIENTED_EDGE('',*,*,#50039,.F.);
#66128=ORIENTED_EDGE('',*,*,#50044,.T.);
#66129=ORIENTED_EDGE('',*,*,#50037,.T.);
#66130=ORIENTED_EDGE('',*,*,#50045,.F.);
#66131=ORIENTED_EDGE('',*,*,#50042,.F.);
#66132=ORIENTED_EDGE('',*,*,#50046,.T.);
#66133=ORIENTED_EDGE('',*,*,#50047,.T.);
#66134=ORIENTED_EDGE('',*,*,#50048,.F.);
#66135=ORIENTED_EDGE('',*,*,#50049,.F.);
#66136=ORIENTED_EDGE('',*,*,#50050,.T.);
#66137=ORIENTED_EDGE('',*,*,#50051,.T.);
#66138=ORIENTED_EDGE('',*,*,#50052,.F.);
#66139=ORIENTED_EDGE('',*,*,#50047,.F.);
#66140=ORIENTED_EDGE('',*,*,#50053,.T.);
#66141=ORIENTED_EDGE('',*,*,#50054,.T.);
#66142=ORIENTED_EDGE('',*,*,#50055,.F.);
#66143=ORIENTED_EDGE('',*,*,#50051,.F.);
#66144=ORIENTED_EDGE('',*,*,#50056,.T.);
#66145=ORIENTED_EDGE('',*,*,#50049,.T.);
#66146=ORIENTED_EDGE('',*,*,#50057,.F.);
#66147=ORIENTED_EDGE('',*,*,#50054,.F.);
#66148=ORIENTED_EDGE('',*,*,#50058,.T.);
#66149=ORIENTED_EDGE('',*,*,#50059,.T.);
#66150=ORIENTED_EDGE('',*,*,#50060,.F.);
#66151=ORIENTED_EDGE('',*,*,#50061,.F.);
#66152=ORIENTED_EDGE('',*,*,#50062,.T.);
#66153=ORIENTED_EDGE('',*,*,#50063,.T.);
#66154=ORIENTED_EDGE('',*,*,#50064,.F.);
#66155=ORIENTED_EDGE('',*,*,#50059,.F.);
#66156=ORIENTED_EDGE('',*,*,#50065,.T.);
#66157=ORIENTED_EDGE('',*,*,#50066,.T.);
#66158=ORIENTED_EDGE('',*,*,#50067,.F.);
#66159=ORIENTED_EDGE('',*,*,#50063,.F.);
#66160=ORIENTED_EDGE('',*,*,#50068,.T.);
#66161=ORIENTED_EDGE('',*,*,#50061,.T.);
#66162=ORIENTED_EDGE('',*,*,#50069,.F.);
#66163=ORIENTED_EDGE('',*,*,#50066,.F.);
#66164=ORIENTED_EDGE('',*,*,#50070,.T.);
#66165=ORIENTED_EDGE('',*,*,#50071,.T.);
#66166=ORIENTED_EDGE('',*,*,#50072,.F.);
#66167=ORIENTED_EDGE('',*,*,#50073,.F.);
#66168=ORIENTED_EDGE('',*,*,#50074,.T.);
#66169=ORIENTED_EDGE('',*,*,#50075,.T.);
#66170=ORIENTED_EDGE('',*,*,#50076,.F.);
#66171=ORIENTED_EDGE('',*,*,#50071,.F.);
#66172=ORIENTED_EDGE('',*,*,#50077,.T.);
#66173=ORIENTED_EDGE('',*,*,#50078,.T.);
#66174=ORIENTED_EDGE('',*,*,#50079,.F.);
#66175=ORIENTED_EDGE('',*,*,#50075,.F.);
#66176=ORIENTED_EDGE('',*,*,#50080,.T.);
#66177=ORIENTED_EDGE('',*,*,#50073,.T.);
#66178=ORIENTED_EDGE('',*,*,#50081,.F.);
#66179=ORIENTED_EDGE('',*,*,#50078,.F.);
#66180=ORIENTED_EDGE('',*,*,#50082,.T.);
#66181=ORIENTED_EDGE('',*,*,#50083,.T.);
#66182=ORIENTED_EDGE('',*,*,#50084,.F.);
#66183=ORIENTED_EDGE('',*,*,#50085,.F.);
#66184=ORIENTED_EDGE('',*,*,#50086,.T.);
#66185=ORIENTED_EDGE('',*,*,#50087,.T.);
#66186=ORIENTED_EDGE('',*,*,#50088,.F.);
#66187=ORIENTED_EDGE('',*,*,#50083,.F.);
#66188=ORIENTED_EDGE('',*,*,#50089,.T.);
#66189=ORIENTED_EDGE('',*,*,#50090,.T.);
#66190=ORIENTED_EDGE('',*,*,#50091,.F.);
#66191=ORIENTED_EDGE('',*,*,#50087,.F.);
#66192=ORIENTED_EDGE('',*,*,#50092,.T.);
#66193=ORIENTED_EDGE('',*,*,#50085,.T.);
#66194=ORIENTED_EDGE('',*,*,#50093,.F.);
#66195=ORIENTED_EDGE('',*,*,#50090,.F.);
#66196=ORIENTED_EDGE('',*,*,#50094,.T.);
#66197=ORIENTED_EDGE('',*,*,#50095,.T.);
#66198=ORIENTED_EDGE('',*,*,#50096,.F.);
#66199=ORIENTED_EDGE('',*,*,#50097,.F.);
#66200=ORIENTED_EDGE('',*,*,#50098,.T.);
#66201=ORIENTED_EDGE('',*,*,#50099,.T.);
#66202=ORIENTED_EDGE('',*,*,#50100,.F.);
#66203=ORIENTED_EDGE('',*,*,#50095,.F.);
#66204=ORIENTED_EDGE('',*,*,#50101,.T.);
#66205=ORIENTED_EDGE('',*,*,#50102,.T.);
#66206=ORIENTED_EDGE('',*,*,#50103,.F.);
#66207=ORIENTED_EDGE('',*,*,#50099,.F.);
#66208=ORIENTED_EDGE('',*,*,#50104,.T.);
#66209=ORIENTED_EDGE('',*,*,#50097,.T.);
#66210=ORIENTED_EDGE('',*,*,#50105,.F.);
#66211=ORIENTED_EDGE('',*,*,#50102,.F.);
#66212=ORIENTED_EDGE('',*,*,#50106,.T.);
#66213=ORIENTED_EDGE('',*,*,#50107,.T.);
#66214=ORIENTED_EDGE('',*,*,#50108,.F.);
#66215=ORIENTED_EDGE('',*,*,#50109,.F.);
#66216=ORIENTED_EDGE('',*,*,#50110,.T.);
#66217=ORIENTED_EDGE('',*,*,#50111,.T.);
#66218=ORIENTED_EDGE('',*,*,#50112,.F.);
#66219=ORIENTED_EDGE('',*,*,#50107,.F.);
#66220=ORIENTED_EDGE('',*,*,#50113,.T.);
#66221=ORIENTED_EDGE('',*,*,#50114,.T.);
#66222=ORIENTED_EDGE('',*,*,#50115,.F.);
#66223=ORIENTED_EDGE('',*,*,#50111,.F.);
#66224=ORIENTED_EDGE('',*,*,#50116,.T.);
#66225=ORIENTED_EDGE('',*,*,#50109,.T.);
#66226=ORIENTED_EDGE('',*,*,#50117,.F.);
#66227=ORIENTED_EDGE('',*,*,#50114,.F.);
#66228=ORIENTED_EDGE('',*,*,#50118,.T.);
#66229=ORIENTED_EDGE('',*,*,#50119,.T.);
#66230=ORIENTED_EDGE('',*,*,#50120,.F.);
#66231=ORIENTED_EDGE('',*,*,#50121,.F.);
#66232=ORIENTED_EDGE('',*,*,#50122,.T.);
#66233=ORIENTED_EDGE('',*,*,#50123,.T.);
#66234=ORIENTED_EDGE('',*,*,#50124,.F.);
#66235=ORIENTED_EDGE('',*,*,#50119,.F.);
#66236=ORIENTED_EDGE('',*,*,#50125,.T.);
#66237=ORIENTED_EDGE('',*,*,#50126,.T.);
#66238=ORIENTED_EDGE('',*,*,#50127,.F.);
#66239=ORIENTED_EDGE('',*,*,#50123,.F.);
#66240=ORIENTED_EDGE('',*,*,#50128,.T.);
#66241=ORIENTED_EDGE('',*,*,#50121,.T.);
#66242=ORIENTED_EDGE('',*,*,#50129,.F.);
#66243=ORIENTED_EDGE('',*,*,#50126,.F.);
#66244=ORIENTED_EDGE('',*,*,#50130,.T.);
#66245=ORIENTED_EDGE('',*,*,#50131,.T.);
#66246=ORIENTED_EDGE('',*,*,#50132,.F.);
#66247=ORIENTED_EDGE('',*,*,#50133,.F.);
#66248=ORIENTED_EDGE('',*,*,#50134,.T.);
#66249=ORIENTED_EDGE('',*,*,#50135,.T.);
#66250=ORIENTED_EDGE('',*,*,#50136,.F.);
#66251=ORIENTED_EDGE('',*,*,#50131,.F.);
#66252=ORIENTED_EDGE('',*,*,#50137,.T.);
#66253=ORIENTED_EDGE('',*,*,#50138,.T.);
#66254=ORIENTED_EDGE('',*,*,#50139,.F.);
#66255=ORIENTED_EDGE('',*,*,#50135,.F.);
#66256=ORIENTED_EDGE('',*,*,#50140,.T.);
#66257=ORIENTED_EDGE('',*,*,#50133,.T.);
#66258=ORIENTED_EDGE('',*,*,#50141,.F.);
#66259=ORIENTED_EDGE('',*,*,#50138,.F.);
#66260=ORIENTED_EDGE('',*,*,#50142,.T.);
#66261=ORIENTED_EDGE('',*,*,#50143,.T.);
#66262=ORIENTED_EDGE('',*,*,#50144,.F.);
#66263=ORIENTED_EDGE('',*,*,#50145,.F.);
#66264=ORIENTED_EDGE('',*,*,#50146,.T.);
#66265=ORIENTED_EDGE('',*,*,#50147,.T.);
#66266=ORIENTED_EDGE('',*,*,#50148,.F.);
#66267=ORIENTED_EDGE('',*,*,#50143,.F.);
#66268=ORIENTED_EDGE('',*,*,#50149,.T.);
#66269=ORIENTED_EDGE('',*,*,#50150,.T.);
#66270=ORIENTED_EDGE('',*,*,#50151,.F.);
#66271=ORIENTED_EDGE('',*,*,#50147,.F.);
#66272=ORIENTED_EDGE('',*,*,#50152,.T.);
#66273=ORIENTED_EDGE('',*,*,#50145,.T.);
#66274=ORIENTED_EDGE('',*,*,#50153,.F.);
#66275=ORIENTED_EDGE('',*,*,#50150,.F.);
#66276=ORIENTED_EDGE('',*,*,#50154,.T.);
#66277=ORIENTED_EDGE('',*,*,#50155,.T.);
#66278=ORIENTED_EDGE('',*,*,#50156,.F.);
#66279=ORIENTED_EDGE('',*,*,#50157,.F.);
#66280=ORIENTED_EDGE('',*,*,#50158,.T.);
#66281=ORIENTED_EDGE('',*,*,#50159,.T.);
#66282=ORIENTED_EDGE('',*,*,#50160,.F.);
#66283=ORIENTED_EDGE('',*,*,#50155,.F.);
#66284=ORIENTED_EDGE('',*,*,#50161,.T.);
#66285=ORIENTED_EDGE('',*,*,#50162,.T.);
#66286=ORIENTED_EDGE('',*,*,#50163,.F.);
#66287=ORIENTED_EDGE('',*,*,#50159,.F.);
#66288=ORIENTED_EDGE('',*,*,#50164,.T.);
#66289=ORIENTED_EDGE('',*,*,#50157,.T.);
#66290=ORIENTED_EDGE('',*,*,#50165,.F.);
#66291=ORIENTED_EDGE('',*,*,#50162,.F.);
#66292=ORIENTED_EDGE('',*,*,#50166,.T.);
#66293=ORIENTED_EDGE('',*,*,#50167,.T.);
#66294=ORIENTED_EDGE('',*,*,#50168,.F.);
#66295=ORIENTED_EDGE('',*,*,#50169,.F.);
#66296=ORIENTED_EDGE('',*,*,#50170,.T.);
#66297=ORIENTED_EDGE('',*,*,#50171,.T.);
#66298=ORIENTED_EDGE('',*,*,#50172,.F.);
#66299=ORIENTED_EDGE('',*,*,#50167,.F.);
#66300=ORIENTED_EDGE('',*,*,#50173,.T.);
#66301=ORIENTED_EDGE('',*,*,#50174,.T.);
#66302=ORIENTED_EDGE('',*,*,#50175,.F.);
#66303=ORIENTED_EDGE('',*,*,#50171,.F.);
#66304=ORIENTED_EDGE('',*,*,#50176,.T.);
#66305=ORIENTED_EDGE('',*,*,#50169,.T.);
#66306=ORIENTED_EDGE('',*,*,#50177,.F.);
#66307=ORIENTED_EDGE('',*,*,#50174,.F.);
#66308=ORIENTED_EDGE('',*,*,#50178,.T.);
#66309=ORIENTED_EDGE('',*,*,#50179,.T.);
#66310=ORIENTED_EDGE('',*,*,#50180,.F.);
#66311=ORIENTED_EDGE('',*,*,#50181,.F.);
#66312=ORIENTED_EDGE('',*,*,#50182,.T.);
#66313=ORIENTED_EDGE('',*,*,#50183,.T.);
#66314=ORIENTED_EDGE('',*,*,#50184,.F.);
#66315=ORIENTED_EDGE('',*,*,#50179,.F.);
#66316=ORIENTED_EDGE('',*,*,#50185,.T.);
#66317=ORIENTED_EDGE('',*,*,#50186,.T.);
#66318=ORIENTED_EDGE('',*,*,#50187,.F.);
#66319=ORIENTED_EDGE('',*,*,#50183,.F.);
#66320=ORIENTED_EDGE('',*,*,#50188,.T.);
#66321=ORIENTED_EDGE('',*,*,#50181,.T.);
#66322=ORIENTED_EDGE('',*,*,#50189,.F.);
#66323=ORIENTED_EDGE('',*,*,#50186,.F.);
#66324=ORIENTED_EDGE('',*,*,#50190,.T.);
#66325=ORIENTED_EDGE('',*,*,#50191,.T.);
#66326=ORIENTED_EDGE('',*,*,#50192,.F.);
#66327=ORIENTED_EDGE('',*,*,#50193,.F.);
#66328=ORIENTED_EDGE('',*,*,#50194,.T.);
#66329=ORIENTED_EDGE('',*,*,#50195,.T.);
#66330=ORIENTED_EDGE('',*,*,#50196,.F.);
#66331=ORIENTED_EDGE('',*,*,#50191,.F.);
#66332=ORIENTED_EDGE('',*,*,#50197,.T.);
#66333=ORIENTED_EDGE('',*,*,#50198,.T.);
#66334=ORIENTED_EDGE('',*,*,#50199,.F.);
#66335=ORIENTED_EDGE('',*,*,#50195,.F.);
#66336=ORIENTED_EDGE('',*,*,#50200,.T.);
#66337=ORIENTED_EDGE('',*,*,#50193,.T.);
#66338=ORIENTED_EDGE('',*,*,#50201,.F.);
#66339=ORIENTED_EDGE('',*,*,#50198,.F.);
#66340=ORIENTED_EDGE('',*,*,#50202,.T.);
#66341=ORIENTED_EDGE('',*,*,#50203,.T.);
#66342=ORIENTED_EDGE('',*,*,#50204,.F.);
#66343=ORIENTED_EDGE('',*,*,#50205,.F.);
#66344=ORIENTED_EDGE('',*,*,#50206,.T.);
#66345=ORIENTED_EDGE('',*,*,#50207,.T.);
#66346=ORIENTED_EDGE('',*,*,#50208,.F.);
#66347=ORIENTED_EDGE('',*,*,#50203,.F.);
#66348=ORIENTED_EDGE('',*,*,#50209,.T.);
#66349=ORIENTED_EDGE('',*,*,#50210,.T.);
#66350=ORIENTED_EDGE('',*,*,#50211,.F.);
#66351=ORIENTED_EDGE('',*,*,#50207,.F.);
#66352=ORIENTED_EDGE('',*,*,#50212,.T.);
#66353=ORIENTED_EDGE('',*,*,#50205,.T.);
#66354=ORIENTED_EDGE('',*,*,#50213,.F.);
#66355=ORIENTED_EDGE('',*,*,#50210,.F.);
#66356=ORIENTED_EDGE('',*,*,#50214,.T.);
#66357=ORIENTED_EDGE('',*,*,#50215,.T.);
#66358=ORIENTED_EDGE('',*,*,#50216,.F.);
#66359=ORIENTED_EDGE('',*,*,#50217,.F.);
#66360=ORIENTED_EDGE('',*,*,#50218,.T.);
#66361=ORIENTED_EDGE('',*,*,#50219,.T.);
#66362=ORIENTED_EDGE('',*,*,#50220,.F.);
#66363=ORIENTED_EDGE('',*,*,#50215,.F.);
#66364=ORIENTED_EDGE('',*,*,#50221,.T.);
#66365=ORIENTED_EDGE('',*,*,#50222,.T.);
#66366=ORIENTED_EDGE('',*,*,#50223,.F.);
#66367=ORIENTED_EDGE('',*,*,#50219,.F.);
#66368=ORIENTED_EDGE('',*,*,#50224,.T.);
#66369=ORIENTED_EDGE('',*,*,#50217,.T.);
#66370=ORIENTED_EDGE('',*,*,#50225,.F.);
#66371=ORIENTED_EDGE('',*,*,#50222,.F.);
#66372=ORIENTED_EDGE('',*,*,#50226,.T.);
#66373=ORIENTED_EDGE('',*,*,#50227,.T.);
#66374=ORIENTED_EDGE('',*,*,#50228,.F.);
#66375=ORIENTED_EDGE('',*,*,#50229,.F.);
#66376=ORIENTED_EDGE('',*,*,#50230,.T.);
#66377=ORIENTED_EDGE('',*,*,#50231,.T.);
#66378=ORIENTED_EDGE('',*,*,#50232,.F.);
#66379=ORIENTED_EDGE('',*,*,#50227,.F.);
#66380=ORIENTED_EDGE('',*,*,#50233,.T.);
#66381=ORIENTED_EDGE('',*,*,#50234,.T.);
#66382=ORIENTED_EDGE('',*,*,#50235,.F.);
#66383=ORIENTED_EDGE('',*,*,#50231,.F.);
#66384=ORIENTED_EDGE('',*,*,#50236,.T.);
#66385=ORIENTED_EDGE('',*,*,#50229,.T.);
#66386=ORIENTED_EDGE('',*,*,#50237,.F.);
#66387=ORIENTED_EDGE('',*,*,#50234,.F.);
#66388=ORIENTED_EDGE('',*,*,#50238,.T.);
#66389=ORIENTED_EDGE('',*,*,#50239,.T.);
#66390=ORIENTED_EDGE('',*,*,#50240,.F.);
#66391=ORIENTED_EDGE('',*,*,#50241,.F.);
#66392=ORIENTED_EDGE('',*,*,#50242,.T.);
#66393=ORIENTED_EDGE('',*,*,#50243,.T.);
#66394=ORIENTED_EDGE('',*,*,#50244,.F.);
#66395=ORIENTED_EDGE('',*,*,#50239,.F.);
#66396=ORIENTED_EDGE('',*,*,#50245,.T.);
#66397=ORIENTED_EDGE('',*,*,#50246,.T.);
#66398=ORIENTED_EDGE('',*,*,#50247,.F.);
#66399=ORIENTED_EDGE('',*,*,#50243,.F.);
#66400=ORIENTED_EDGE('',*,*,#50248,.T.);
#66401=ORIENTED_EDGE('',*,*,#50241,.T.);
#66402=ORIENTED_EDGE('',*,*,#50249,.F.);
#66403=ORIENTED_EDGE('',*,*,#50246,.F.);
#66404=ORIENTED_EDGE('',*,*,#50250,.T.);
#66405=ORIENTED_EDGE('',*,*,#50251,.T.);
#66406=ORIENTED_EDGE('',*,*,#50252,.F.);
#66407=ORIENTED_EDGE('',*,*,#50253,.F.);
#66408=ORIENTED_EDGE('',*,*,#50254,.T.);
#66409=ORIENTED_EDGE('',*,*,#50255,.T.);
#66410=ORIENTED_EDGE('',*,*,#50256,.F.);
#66411=ORIENTED_EDGE('',*,*,#50251,.F.);
#66412=ORIENTED_EDGE('',*,*,#50257,.T.);
#66413=ORIENTED_EDGE('',*,*,#50258,.T.);
#66414=ORIENTED_EDGE('',*,*,#50259,.F.);
#66415=ORIENTED_EDGE('',*,*,#50255,.F.);
#66416=ORIENTED_EDGE('',*,*,#50260,.T.);
#66417=ORIENTED_EDGE('',*,*,#50253,.T.);
#66418=ORIENTED_EDGE('',*,*,#50261,.F.);
#66419=ORIENTED_EDGE('',*,*,#50258,.F.);
#66420=ORIENTED_EDGE('',*,*,#50262,.T.);
#66421=ORIENTED_EDGE('',*,*,#50263,.T.);
#66422=ORIENTED_EDGE('',*,*,#50264,.F.);
#66423=ORIENTED_EDGE('',*,*,#50265,.F.);
#66424=ORIENTED_EDGE('',*,*,#50266,.T.);
#66425=ORIENTED_EDGE('',*,*,#50267,.T.);
#66426=ORIENTED_EDGE('',*,*,#50268,.F.);
#66427=ORIENTED_EDGE('',*,*,#50263,.F.);
#66428=ORIENTED_EDGE('',*,*,#50269,.T.);
#66429=ORIENTED_EDGE('',*,*,#50270,.T.);
#66430=ORIENTED_EDGE('',*,*,#50271,.F.);
#66431=ORIENTED_EDGE('',*,*,#50267,.F.);
#66432=ORIENTED_EDGE('',*,*,#50272,.T.);
#66433=ORIENTED_EDGE('',*,*,#50265,.T.);
#66434=ORIENTED_EDGE('',*,*,#50273,.F.);
#66435=ORIENTED_EDGE('',*,*,#50270,.F.);
#66436=ORIENTED_EDGE('',*,*,#50274,.T.);
#66437=ORIENTED_EDGE('',*,*,#50275,.T.);
#66438=ORIENTED_EDGE('',*,*,#50276,.F.);
#66439=ORIENTED_EDGE('',*,*,#50277,.F.);
#66440=ORIENTED_EDGE('',*,*,#50278,.T.);
#66441=ORIENTED_EDGE('',*,*,#50279,.T.);
#66442=ORIENTED_EDGE('',*,*,#50280,.F.);
#66443=ORIENTED_EDGE('',*,*,#50275,.F.);
#66444=ORIENTED_EDGE('',*,*,#50281,.T.);
#66445=ORIENTED_EDGE('',*,*,#50282,.T.);
#66446=ORIENTED_EDGE('',*,*,#50283,.F.);
#66447=ORIENTED_EDGE('',*,*,#50279,.F.);
#66448=ORIENTED_EDGE('',*,*,#50284,.T.);
#66449=ORIENTED_EDGE('',*,*,#50277,.T.);
#66450=ORIENTED_EDGE('',*,*,#50285,.F.);
#66451=ORIENTED_EDGE('',*,*,#50282,.F.);
#66452=ORIENTED_EDGE('',*,*,#50286,.T.);
#66453=ORIENTED_EDGE('',*,*,#50287,.T.);
#66454=ORIENTED_EDGE('',*,*,#50288,.F.);
#66455=ORIENTED_EDGE('',*,*,#50289,.F.);
#66456=ORIENTED_EDGE('',*,*,#50290,.T.);
#66457=ORIENTED_EDGE('',*,*,#50291,.T.);
#66458=ORIENTED_EDGE('',*,*,#50292,.F.);
#66459=ORIENTED_EDGE('',*,*,#50287,.F.);
#66460=ORIENTED_EDGE('',*,*,#50293,.T.);
#66461=ORIENTED_EDGE('',*,*,#50294,.T.);
#66462=ORIENTED_EDGE('',*,*,#50295,.F.);
#66463=ORIENTED_EDGE('',*,*,#50291,.F.);
#66464=ORIENTED_EDGE('',*,*,#50296,.T.);
#66465=ORIENTED_EDGE('',*,*,#50289,.T.);
#66466=ORIENTED_EDGE('',*,*,#50297,.F.);
#66467=ORIENTED_EDGE('',*,*,#50294,.F.);
#66468=ORIENTED_EDGE('',*,*,#50298,.T.);
#66469=ORIENTED_EDGE('',*,*,#50299,.T.);
#66470=ORIENTED_EDGE('',*,*,#50300,.F.);
#66471=ORIENTED_EDGE('',*,*,#50301,.F.);
#66472=ORIENTED_EDGE('',*,*,#50302,.T.);
#66473=ORIENTED_EDGE('',*,*,#50303,.T.);
#66474=ORIENTED_EDGE('',*,*,#50304,.F.);
#66475=ORIENTED_EDGE('',*,*,#50299,.F.);
#66476=ORIENTED_EDGE('',*,*,#50305,.T.);
#66477=ORIENTED_EDGE('',*,*,#50306,.T.);
#66478=ORIENTED_EDGE('',*,*,#50307,.F.);
#66479=ORIENTED_EDGE('',*,*,#50303,.F.);
#66480=ORIENTED_EDGE('',*,*,#50308,.T.);
#66481=ORIENTED_EDGE('',*,*,#50301,.T.);
#66482=ORIENTED_EDGE('',*,*,#50309,.F.);
#66483=ORIENTED_EDGE('',*,*,#50306,.F.);
#66484=ORIENTED_EDGE('',*,*,#50310,.T.);
#66485=ORIENTED_EDGE('',*,*,#50311,.T.);
#66486=ORIENTED_EDGE('',*,*,#50312,.F.);
#66487=ORIENTED_EDGE('',*,*,#50313,.F.);
#66488=ORIENTED_EDGE('',*,*,#50314,.T.);
#66489=ORIENTED_EDGE('',*,*,#50315,.T.);
#66490=ORIENTED_EDGE('',*,*,#50316,.F.);
#66491=ORIENTED_EDGE('',*,*,#50311,.F.);
#66492=ORIENTED_EDGE('',*,*,#50317,.T.);
#66493=ORIENTED_EDGE('',*,*,#50318,.T.);
#66494=ORIENTED_EDGE('',*,*,#50319,.F.);
#66495=ORIENTED_EDGE('',*,*,#50315,.F.);
#66496=ORIENTED_EDGE('',*,*,#50320,.T.);
#66497=ORIENTED_EDGE('',*,*,#50313,.T.);
#66498=ORIENTED_EDGE('',*,*,#50321,.F.);
#66499=ORIENTED_EDGE('',*,*,#50318,.F.);
#66500=ORIENTED_EDGE('',*,*,#50322,.T.);
#66501=ORIENTED_EDGE('',*,*,#50323,.T.);
#66502=ORIENTED_EDGE('',*,*,#50324,.F.);
#66503=ORIENTED_EDGE('',*,*,#50325,.F.);
#66504=ORIENTED_EDGE('',*,*,#50326,.T.);
#66505=ORIENTED_EDGE('',*,*,#50327,.T.);
#66506=ORIENTED_EDGE('',*,*,#50328,.F.);
#66507=ORIENTED_EDGE('',*,*,#50323,.F.);
#66508=ORIENTED_EDGE('',*,*,#50329,.T.);
#66509=ORIENTED_EDGE('',*,*,#50330,.T.);
#66510=ORIENTED_EDGE('',*,*,#50331,.F.);
#66511=ORIENTED_EDGE('',*,*,#50327,.F.);
#66512=ORIENTED_EDGE('',*,*,#50332,.T.);
#66513=ORIENTED_EDGE('',*,*,#50325,.T.);
#66514=ORIENTED_EDGE('',*,*,#50333,.F.);
#66515=ORIENTED_EDGE('',*,*,#50330,.F.);
#66516=ORIENTED_EDGE('',*,*,#50334,.T.);
#66517=ORIENTED_EDGE('',*,*,#50335,.T.);
#66518=ORIENTED_EDGE('',*,*,#50336,.F.);
#66519=ORIENTED_EDGE('',*,*,#50337,.F.);
#66520=ORIENTED_EDGE('',*,*,#50338,.T.);
#66521=ORIENTED_EDGE('',*,*,#50339,.T.);
#66522=ORIENTED_EDGE('',*,*,#50340,.F.);
#66523=ORIENTED_EDGE('',*,*,#50335,.F.);
#66524=ORIENTED_EDGE('',*,*,#50341,.T.);
#66525=ORIENTED_EDGE('',*,*,#50342,.T.);
#66526=ORIENTED_EDGE('',*,*,#50343,.F.);
#66527=ORIENTED_EDGE('',*,*,#50339,.F.);
#66528=ORIENTED_EDGE('',*,*,#50344,.T.);
#66529=ORIENTED_EDGE('',*,*,#50337,.T.);
#66530=ORIENTED_EDGE('',*,*,#50345,.F.);
#66531=ORIENTED_EDGE('',*,*,#50342,.F.);
#66532=ORIENTED_EDGE('',*,*,#50346,.T.);
#66533=ORIENTED_EDGE('',*,*,#50347,.T.);
#66534=ORIENTED_EDGE('',*,*,#50348,.F.);
#66535=ORIENTED_EDGE('',*,*,#50349,.F.);
#66536=ORIENTED_EDGE('',*,*,#50350,.T.);
#66537=ORIENTED_EDGE('',*,*,#50351,.T.);
#66538=ORIENTED_EDGE('',*,*,#50352,.F.);
#66539=ORIENTED_EDGE('',*,*,#50347,.F.);
#66540=ORIENTED_EDGE('',*,*,#50353,.T.);
#66541=ORIENTED_EDGE('',*,*,#50354,.T.);
#66542=ORIENTED_EDGE('',*,*,#50355,.F.);
#66543=ORIENTED_EDGE('',*,*,#50351,.F.);
#66544=ORIENTED_EDGE('',*,*,#50356,.T.);
#66545=ORIENTED_EDGE('',*,*,#50349,.T.);
#66546=ORIENTED_EDGE('',*,*,#50357,.F.);
#66547=ORIENTED_EDGE('',*,*,#50354,.F.);
#66548=ORIENTED_EDGE('',*,*,#50358,.T.);
#66549=ORIENTED_EDGE('',*,*,#50359,.T.);
#66550=ORIENTED_EDGE('',*,*,#50360,.F.);
#66551=ORIENTED_EDGE('',*,*,#50361,.F.);
#66552=ORIENTED_EDGE('',*,*,#50362,.T.);
#66553=ORIENTED_EDGE('',*,*,#50363,.T.);
#66554=ORIENTED_EDGE('',*,*,#50364,.F.);
#66555=ORIENTED_EDGE('',*,*,#50359,.F.);
#66556=ORIENTED_EDGE('',*,*,#50365,.T.);
#66557=ORIENTED_EDGE('',*,*,#50366,.T.);
#66558=ORIENTED_EDGE('',*,*,#50367,.F.);
#66559=ORIENTED_EDGE('',*,*,#50363,.F.);
#66560=ORIENTED_EDGE('',*,*,#50368,.T.);
#66561=ORIENTED_EDGE('',*,*,#50361,.T.);
#66562=ORIENTED_EDGE('',*,*,#50369,.F.);
#66563=ORIENTED_EDGE('',*,*,#50366,.F.);
#66564=ORIENTED_EDGE('',*,*,#50370,.T.);
#66565=ORIENTED_EDGE('',*,*,#50371,.T.);
#66566=ORIENTED_EDGE('',*,*,#50372,.F.);
#66567=ORIENTED_EDGE('',*,*,#50373,.F.);
#66568=ORIENTED_EDGE('',*,*,#50374,.T.);
#66569=ORIENTED_EDGE('',*,*,#50375,.T.);
#66570=ORIENTED_EDGE('',*,*,#50376,.F.);
#66571=ORIENTED_EDGE('',*,*,#50371,.F.);
#66572=ORIENTED_EDGE('',*,*,#50377,.T.);
#66573=ORIENTED_EDGE('',*,*,#50378,.T.);
#66574=ORIENTED_EDGE('',*,*,#50379,.F.);
#66575=ORIENTED_EDGE('',*,*,#50375,.F.);
#66576=ORIENTED_EDGE('',*,*,#50380,.T.);
#66577=ORIENTED_EDGE('',*,*,#50373,.T.);
#66578=ORIENTED_EDGE('',*,*,#50381,.F.);
#66579=ORIENTED_EDGE('',*,*,#50378,.F.);
#66580=ORIENTED_EDGE('',*,*,#50382,.T.);
#66581=ORIENTED_EDGE('',*,*,#50383,.T.);
#66582=ORIENTED_EDGE('',*,*,#50384,.F.);
#66583=ORIENTED_EDGE('',*,*,#50385,.F.);
#66584=ORIENTED_EDGE('',*,*,#50386,.T.);
#66585=ORIENTED_EDGE('',*,*,#50387,.T.);
#66586=ORIENTED_EDGE('',*,*,#50388,.F.);
#66587=ORIENTED_EDGE('',*,*,#50383,.F.);
#66588=ORIENTED_EDGE('',*,*,#50389,.T.);
#66589=ORIENTED_EDGE('',*,*,#50390,.T.);
#66590=ORIENTED_EDGE('',*,*,#50391,.F.);
#66591=ORIENTED_EDGE('',*,*,#50387,.F.);
#66592=ORIENTED_EDGE('',*,*,#50392,.T.);
#66593=ORIENTED_EDGE('',*,*,#50385,.T.);
#66594=ORIENTED_EDGE('',*,*,#50393,.F.);
#66595=ORIENTED_EDGE('',*,*,#50390,.F.);
#66596=ORIENTED_EDGE('',*,*,#50394,.T.);
#66597=ORIENTED_EDGE('',*,*,#50395,.T.);
#66598=ORIENTED_EDGE('',*,*,#50396,.F.);
#66599=ORIENTED_EDGE('',*,*,#50397,.F.);
#66600=ORIENTED_EDGE('',*,*,#50398,.T.);
#66601=ORIENTED_EDGE('',*,*,#50399,.T.);
#66602=ORIENTED_EDGE('',*,*,#50400,.F.);
#66603=ORIENTED_EDGE('',*,*,#50395,.F.);
#66604=ORIENTED_EDGE('',*,*,#50401,.T.);
#66605=ORIENTED_EDGE('',*,*,#50402,.T.);
#66606=ORIENTED_EDGE('',*,*,#50403,.F.);
#66607=ORIENTED_EDGE('',*,*,#50399,.F.);
#66608=ORIENTED_EDGE('',*,*,#50404,.T.);
#66609=ORIENTED_EDGE('',*,*,#50397,.T.);
#66610=ORIENTED_EDGE('',*,*,#50405,.F.);
#66611=ORIENTED_EDGE('',*,*,#50402,.F.);
#66612=ORIENTED_EDGE('',*,*,#50406,.T.);
#66613=ORIENTED_EDGE('',*,*,#50407,.T.);
#66614=ORIENTED_EDGE('',*,*,#50408,.F.);
#66615=ORIENTED_EDGE('',*,*,#50409,.F.);
#66616=ORIENTED_EDGE('',*,*,#50410,.T.);
#66617=ORIENTED_EDGE('',*,*,#50411,.T.);
#66618=ORIENTED_EDGE('',*,*,#50412,.F.);
#66619=ORIENTED_EDGE('',*,*,#50407,.F.);
#66620=ORIENTED_EDGE('',*,*,#50413,.T.);
#66621=ORIENTED_EDGE('',*,*,#50414,.T.);
#66622=ORIENTED_EDGE('',*,*,#50415,.F.);
#66623=ORIENTED_EDGE('',*,*,#50411,.F.);
#66624=ORIENTED_EDGE('',*,*,#50416,.T.);
#66625=ORIENTED_EDGE('',*,*,#50409,.T.);
#66626=ORIENTED_EDGE('',*,*,#50417,.F.);
#66627=ORIENTED_EDGE('',*,*,#50414,.F.);
#66628=ORIENTED_EDGE('',*,*,#50418,.T.);
#66629=ORIENTED_EDGE('',*,*,#50419,.T.);
#66630=ORIENTED_EDGE('',*,*,#50420,.F.);
#66631=ORIENTED_EDGE('',*,*,#50421,.F.);
#66632=ORIENTED_EDGE('',*,*,#50422,.T.);
#66633=ORIENTED_EDGE('',*,*,#50423,.T.);
#66634=ORIENTED_EDGE('',*,*,#50424,.F.);
#66635=ORIENTED_EDGE('',*,*,#50419,.F.);
#66636=ORIENTED_EDGE('',*,*,#50425,.T.);
#66637=ORIENTED_EDGE('',*,*,#50426,.T.);
#66638=ORIENTED_EDGE('',*,*,#50427,.F.);
#66639=ORIENTED_EDGE('',*,*,#50423,.F.);
#66640=ORIENTED_EDGE('',*,*,#50428,.T.);
#66641=ORIENTED_EDGE('',*,*,#50421,.T.);
#66642=ORIENTED_EDGE('',*,*,#50429,.F.);
#66643=ORIENTED_EDGE('',*,*,#50426,.F.);
#66644=ORIENTED_EDGE('',*,*,#50430,.T.);
#66645=ORIENTED_EDGE('',*,*,#50431,.T.);
#66646=ORIENTED_EDGE('',*,*,#50432,.F.);
#66647=ORIENTED_EDGE('',*,*,#50433,.F.);
#66648=ORIENTED_EDGE('',*,*,#50434,.T.);
#66649=ORIENTED_EDGE('',*,*,#50435,.T.);
#66650=ORIENTED_EDGE('',*,*,#50436,.F.);
#66651=ORIENTED_EDGE('',*,*,#50431,.F.);
#66652=ORIENTED_EDGE('',*,*,#50437,.T.);
#66653=ORIENTED_EDGE('',*,*,#50438,.T.);
#66654=ORIENTED_EDGE('',*,*,#50439,.F.);
#66655=ORIENTED_EDGE('',*,*,#50435,.F.);
#66656=ORIENTED_EDGE('',*,*,#50440,.T.);
#66657=ORIENTED_EDGE('',*,*,#50433,.T.);
#66658=ORIENTED_EDGE('',*,*,#50441,.F.);
#66659=ORIENTED_EDGE('',*,*,#50438,.F.);
#66660=ORIENTED_EDGE('',*,*,#50442,.T.);
#66661=ORIENTED_EDGE('',*,*,#50443,.T.);
#66662=ORIENTED_EDGE('',*,*,#50444,.F.);
#66663=ORIENTED_EDGE('',*,*,#50445,.F.);
#66664=ORIENTED_EDGE('',*,*,#50446,.T.);
#66665=ORIENTED_EDGE('',*,*,#50447,.T.);
#66666=ORIENTED_EDGE('',*,*,#50448,.F.);
#66667=ORIENTED_EDGE('',*,*,#50443,.F.);
#66668=ORIENTED_EDGE('',*,*,#50449,.T.);
#66669=ORIENTED_EDGE('',*,*,#50450,.T.);
#66670=ORIENTED_EDGE('',*,*,#50451,.F.);
#66671=ORIENTED_EDGE('',*,*,#50447,.F.);
#66672=ORIENTED_EDGE('',*,*,#50452,.T.);
#66673=ORIENTED_EDGE('',*,*,#50445,.T.);
#66674=ORIENTED_EDGE('',*,*,#50453,.F.);
#66675=ORIENTED_EDGE('',*,*,#50450,.F.);
#66676=ORIENTED_EDGE('',*,*,#50454,.T.);
#66677=ORIENTED_EDGE('',*,*,#50455,.T.);
#66678=ORIENTED_EDGE('',*,*,#50456,.F.);
#66679=ORIENTED_EDGE('',*,*,#50457,.F.);
#66680=ORIENTED_EDGE('',*,*,#50458,.T.);
#66681=ORIENTED_EDGE('',*,*,#50459,.T.);
#66682=ORIENTED_EDGE('',*,*,#50460,.F.);
#66683=ORIENTED_EDGE('',*,*,#50455,.F.);
#66684=ORIENTED_EDGE('',*,*,#50461,.T.);
#66685=ORIENTED_EDGE('',*,*,#50462,.T.);
#66686=ORIENTED_EDGE('',*,*,#50463,.F.);
#66687=ORIENTED_EDGE('',*,*,#50459,.F.);
#66688=ORIENTED_EDGE('',*,*,#50464,.T.);
#66689=ORIENTED_EDGE('',*,*,#50457,.T.);
#66690=ORIENTED_EDGE('',*,*,#50465,.F.);
#66691=ORIENTED_EDGE('',*,*,#50462,.F.);
#66692=ORIENTED_EDGE('',*,*,#50466,.T.);
#66693=ORIENTED_EDGE('',*,*,#50467,.T.);
#66694=ORIENTED_EDGE('',*,*,#50468,.F.);
#66695=ORIENTED_EDGE('',*,*,#50469,.F.);
#66696=ORIENTED_EDGE('',*,*,#50470,.T.);
#66697=ORIENTED_EDGE('',*,*,#50471,.T.);
#66698=ORIENTED_EDGE('',*,*,#50472,.F.);
#66699=ORIENTED_EDGE('',*,*,#50467,.F.);
#66700=ORIENTED_EDGE('',*,*,#50473,.T.);
#66701=ORIENTED_EDGE('',*,*,#50474,.T.);
#66702=ORIENTED_EDGE('',*,*,#50475,.F.);
#66703=ORIENTED_EDGE('',*,*,#50471,.F.);
#66704=ORIENTED_EDGE('',*,*,#50476,.T.);
#66705=ORIENTED_EDGE('',*,*,#50469,.T.);
#66706=ORIENTED_EDGE('',*,*,#50477,.F.);
#66707=ORIENTED_EDGE('',*,*,#50474,.F.);
#66708=ORIENTED_EDGE('',*,*,#50478,.T.);
#66709=ORIENTED_EDGE('',*,*,#50479,.T.);
#66710=ORIENTED_EDGE('',*,*,#50480,.F.);
#66711=ORIENTED_EDGE('',*,*,#50481,.F.);
#66712=ORIENTED_EDGE('',*,*,#50482,.T.);
#66713=ORIENTED_EDGE('',*,*,#50483,.T.);
#66714=ORIENTED_EDGE('',*,*,#50484,.F.);
#66715=ORIENTED_EDGE('',*,*,#50479,.F.);
#66716=ORIENTED_EDGE('',*,*,#50485,.T.);
#66717=ORIENTED_EDGE('',*,*,#50486,.T.);
#66718=ORIENTED_EDGE('',*,*,#50487,.F.);
#66719=ORIENTED_EDGE('',*,*,#50483,.F.);
#66720=ORIENTED_EDGE('',*,*,#50488,.T.);
#66721=ORIENTED_EDGE('',*,*,#50481,.T.);
#66722=ORIENTED_EDGE('',*,*,#50489,.F.);
#66723=ORIENTED_EDGE('',*,*,#50486,.F.);
#66724=ORIENTED_EDGE('',*,*,#50490,.T.);
#66725=ORIENTED_EDGE('',*,*,#50491,.T.);
#66726=ORIENTED_EDGE('',*,*,#50492,.F.);
#66727=ORIENTED_EDGE('',*,*,#50493,.F.);
#66728=ORIENTED_EDGE('',*,*,#50494,.T.);
#66729=ORIENTED_EDGE('',*,*,#50495,.T.);
#66730=ORIENTED_EDGE('',*,*,#50496,.F.);
#66731=ORIENTED_EDGE('',*,*,#50491,.F.);
#66732=ORIENTED_EDGE('',*,*,#50497,.T.);
#66733=ORIENTED_EDGE('',*,*,#50498,.T.);
#66734=ORIENTED_EDGE('',*,*,#50499,.F.);
#66735=ORIENTED_EDGE('',*,*,#50495,.F.);
#66736=ORIENTED_EDGE('',*,*,#50500,.T.);
#66737=ORIENTED_EDGE('',*,*,#50493,.T.);
#66738=ORIENTED_EDGE('',*,*,#50501,.F.);
#66739=ORIENTED_EDGE('',*,*,#50498,.F.);
#66740=ORIENTED_EDGE('',*,*,#50502,.T.);
#66741=ORIENTED_EDGE('',*,*,#50503,.T.);
#66742=ORIENTED_EDGE('',*,*,#50504,.F.);
#66743=ORIENTED_EDGE('',*,*,#50505,.F.);
#66744=ORIENTED_EDGE('',*,*,#50506,.T.);
#66745=ORIENTED_EDGE('',*,*,#50507,.T.);
#66746=ORIENTED_EDGE('',*,*,#50508,.F.);
#66747=ORIENTED_EDGE('',*,*,#50503,.F.);
#66748=ORIENTED_EDGE('',*,*,#50509,.T.);
#66749=ORIENTED_EDGE('',*,*,#50510,.T.);
#66750=ORIENTED_EDGE('',*,*,#50511,.F.);
#66751=ORIENTED_EDGE('',*,*,#50507,.F.);
#66752=ORIENTED_EDGE('',*,*,#50512,.T.);
#66753=ORIENTED_EDGE('',*,*,#50505,.T.);
#66754=ORIENTED_EDGE('',*,*,#50513,.F.);
#66755=ORIENTED_EDGE('',*,*,#50510,.F.);
#66756=ORIENTED_EDGE('',*,*,#50514,.T.);
#66757=ORIENTED_EDGE('',*,*,#50515,.T.);
#66758=ORIENTED_EDGE('',*,*,#50516,.F.);
#66759=ORIENTED_EDGE('',*,*,#50517,.F.);
#66760=ORIENTED_EDGE('',*,*,#50518,.T.);
#66761=ORIENTED_EDGE('',*,*,#50519,.T.);
#66762=ORIENTED_EDGE('',*,*,#50520,.F.);
#66763=ORIENTED_EDGE('',*,*,#50515,.F.);
#66764=ORIENTED_EDGE('',*,*,#50521,.T.);
#66765=ORIENTED_EDGE('',*,*,#50522,.T.);
#66766=ORIENTED_EDGE('',*,*,#50523,.F.);
#66767=ORIENTED_EDGE('',*,*,#50519,.F.);
#66768=ORIENTED_EDGE('',*,*,#50524,.T.);
#66769=ORIENTED_EDGE('',*,*,#50517,.T.);
#66770=ORIENTED_EDGE('',*,*,#50525,.F.);
#66771=ORIENTED_EDGE('',*,*,#50522,.F.);
#66772=ORIENTED_EDGE('',*,*,#50526,.T.);
#66773=ORIENTED_EDGE('',*,*,#50527,.T.);
#66774=ORIENTED_EDGE('',*,*,#50528,.F.);
#66775=ORIENTED_EDGE('',*,*,#50529,.F.);
#66776=ORIENTED_EDGE('',*,*,#50530,.T.);
#66777=ORIENTED_EDGE('',*,*,#50531,.T.);
#66778=ORIENTED_EDGE('',*,*,#50532,.F.);
#66779=ORIENTED_EDGE('',*,*,#50527,.F.);
#66780=ORIENTED_EDGE('',*,*,#50533,.T.);
#66781=ORIENTED_EDGE('',*,*,#50534,.T.);
#66782=ORIENTED_EDGE('',*,*,#50535,.F.);
#66783=ORIENTED_EDGE('',*,*,#50531,.F.);
#66784=ORIENTED_EDGE('',*,*,#50536,.T.);
#66785=ORIENTED_EDGE('',*,*,#50529,.T.);
#66786=ORIENTED_EDGE('',*,*,#50537,.F.);
#66787=ORIENTED_EDGE('',*,*,#50534,.F.);
#66788=ORIENTED_EDGE('',*,*,#50538,.T.);
#66789=ORIENTED_EDGE('',*,*,#50539,.T.);
#66790=ORIENTED_EDGE('',*,*,#50540,.F.);
#66791=ORIENTED_EDGE('',*,*,#50541,.F.);
#66792=ORIENTED_EDGE('',*,*,#50542,.T.);
#66793=ORIENTED_EDGE('',*,*,#50543,.T.);
#66794=ORIENTED_EDGE('',*,*,#50544,.F.);
#66795=ORIENTED_EDGE('',*,*,#50539,.F.);
#66796=ORIENTED_EDGE('',*,*,#50545,.T.);
#66797=ORIENTED_EDGE('',*,*,#50546,.T.);
#66798=ORIENTED_EDGE('',*,*,#50547,.F.);
#66799=ORIENTED_EDGE('',*,*,#50543,.F.);
#66800=ORIENTED_EDGE('',*,*,#50548,.T.);
#66801=ORIENTED_EDGE('',*,*,#50541,.T.);
#66802=ORIENTED_EDGE('',*,*,#50549,.F.);
#66803=ORIENTED_EDGE('',*,*,#50546,.F.);
#66804=ORIENTED_EDGE('',*,*,#50550,.T.);
#66805=ORIENTED_EDGE('',*,*,#50551,.T.);
#66806=ORIENTED_EDGE('',*,*,#50552,.F.);
#66807=ORIENTED_EDGE('',*,*,#50553,.F.);
#66808=ORIENTED_EDGE('',*,*,#50554,.T.);
#66809=ORIENTED_EDGE('',*,*,#50555,.T.);
#66810=ORIENTED_EDGE('',*,*,#50556,.F.);
#66811=ORIENTED_EDGE('',*,*,#50551,.F.);
#66812=ORIENTED_EDGE('',*,*,#50557,.T.);
#66813=ORIENTED_EDGE('',*,*,#50558,.T.);
#66814=ORIENTED_EDGE('',*,*,#50559,.F.);
#66815=ORIENTED_EDGE('',*,*,#50555,.F.);
#66816=ORIENTED_EDGE('',*,*,#50560,.T.);
#66817=ORIENTED_EDGE('',*,*,#50553,.T.);
#66818=ORIENTED_EDGE('',*,*,#50561,.F.);
#66819=ORIENTED_EDGE('',*,*,#50558,.F.);
#66820=ORIENTED_EDGE('',*,*,#50562,.T.);
#66821=ORIENTED_EDGE('',*,*,#50563,.T.);
#66822=ORIENTED_EDGE('',*,*,#50564,.F.);
#66823=ORIENTED_EDGE('',*,*,#50565,.F.);
#66824=ORIENTED_EDGE('',*,*,#50566,.T.);
#66825=ORIENTED_EDGE('',*,*,#50567,.T.);
#66826=ORIENTED_EDGE('',*,*,#50568,.F.);
#66827=ORIENTED_EDGE('',*,*,#50563,.F.);
#66828=ORIENTED_EDGE('',*,*,#50569,.T.);
#66829=ORIENTED_EDGE('',*,*,#50570,.T.);
#66830=ORIENTED_EDGE('',*,*,#50571,.F.);
#66831=ORIENTED_EDGE('',*,*,#50567,.F.);
#66832=ORIENTED_EDGE('',*,*,#50572,.T.);
#66833=ORIENTED_EDGE('',*,*,#50565,.T.);
#66834=ORIENTED_EDGE('',*,*,#50573,.F.);
#66835=ORIENTED_EDGE('',*,*,#50570,.F.);
#66836=ORIENTED_EDGE('',*,*,#50574,.T.);
#66837=ORIENTED_EDGE('',*,*,#50575,.T.);
#66838=ORIENTED_EDGE('',*,*,#50576,.F.);
#66839=ORIENTED_EDGE('',*,*,#50577,.F.);
#66840=ORIENTED_EDGE('',*,*,#50578,.T.);
#66841=ORIENTED_EDGE('',*,*,#50579,.T.);
#66842=ORIENTED_EDGE('',*,*,#50580,.F.);
#66843=ORIENTED_EDGE('',*,*,#50575,.F.);
#66844=ORIENTED_EDGE('',*,*,#50581,.T.);
#66845=ORIENTED_EDGE('',*,*,#50582,.T.);
#66846=ORIENTED_EDGE('',*,*,#50583,.F.);
#66847=ORIENTED_EDGE('',*,*,#50579,.F.);
#66848=ORIENTED_EDGE('',*,*,#50584,.T.);
#66849=ORIENTED_EDGE('',*,*,#50577,.T.);
#66850=ORIENTED_EDGE('',*,*,#50585,.F.);
#66851=ORIENTED_EDGE('',*,*,#50582,.F.);
#66852=ORIENTED_EDGE('',*,*,#50586,.T.);
#66853=ORIENTED_EDGE('',*,*,#50587,.T.);
#66854=ORIENTED_EDGE('',*,*,#50588,.F.);
#66855=ORIENTED_EDGE('',*,*,#50589,.F.);
#66856=ORIENTED_EDGE('',*,*,#50590,.T.);
#66857=ORIENTED_EDGE('',*,*,#50591,.T.);
#66858=ORIENTED_EDGE('',*,*,#50592,.F.);
#66859=ORIENTED_EDGE('',*,*,#50587,.F.);
#66860=ORIENTED_EDGE('',*,*,#50593,.T.);
#66861=ORIENTED_EDGE('',*,*,#50594,.T.);
#66862=ORIENTED_EDGE('',*,*,#50595,.F.);
#66863=ORIENTED_EDGE('',*,*,#50591,.F.);
#66864=ORIENTED_EDGE('',*,*,#50596,.T.);
#66865=ORIENTED_EDGE('',*,*,#50589,.T.);
#66866=ORIENTED_EDGE('',*,*,#50597,.F.);
#66867=ORIENTED_EDGE('',*,*,#50594,.F.);
#66868=ORIENTED_EDGE('',*,*,#50598,.T.);
#66869=ORIENTED_EDGE('',*,*,#50599,.T.);
#66870=ORIENTED_EDGE('',*,*,#50600,.F.);
#66871=ORIENTED_EDGE('',*,*,#50601,.F.);
#66872=ORIENTED_EDGE('',*,*,#50602,.T.);
#66873=ORIENTED_EDGE('',*,*,#50603,.T.);
#66874=ORIENTED_EDGE('',*,*,#50604,.F.);
#66875=ORIENTED_EDGE('',*,*,#50599,.F.);
#66876=ORIENTED_EDGE('',*,*,#50605,.T.);
#66877=ORIENTED_EDGE('',*,*,#50606,.T.);
#66878=ORIENTED_EDGE('',*,*,#50607,.F.);
#66879=ORIENTED_EDGE('',*,*,#50603,.F.);
#66880=ORIENTED_EDGE('',*,*,#50608,.T.);
#66881=ORIENTED_EDGE('',*,*,#50601,.T.);
#66882=ORIENTED_EDGE('',*,*,#50609,.F.);
#66883=ORIENTED_EDGE('',*,*,#50606,.F.);
#66884=ORIENTED_EDGE('',*,*,#50610,.T.);
#66885=ORIENTED_EDGE('',*,*,#50611,.T.);
#66886=ORIENTED_EDGE('',*,*,#50612,.F.);
#66887=ORIENTED_EDGE('',*,*,#50613,.F.);
#66888=ORIENTED_EDGE('',*,*,#50614,.T.);
#66889=ORIENTED_EDGE('',*,*,#50615,.T.);
#66890=ORIENTED_EDGE('',*,*,#50616,.F.);
#66891=ORIENTED_EDGE('',*,*,#50611,.F.);
#66892=ORIENTED_EDGE('',*,*,#50617,.T.);
#66893=ORIENTED_EDGE('',*,*,#50618,.T.);
#66894=ORIENTED_EDGE('',*,*,#50619,.F.);
#66895=ORIENTED_EDGE('',*,*,#50615,.F.);
#66896=ORIENTED_EDGE('',*,*,#50620,.T.);
#66897=ORIENTED_EDGE('',*,*,#50613,.T.);
#66898=ORIENTED_EDGE('',*,*,#50621,.F.);
#66899=ORIENTED_EDGE('',*,*,#50618,.F.);
#66900=ORIENTED_EDGE('',*,*,#50622,.T.);
#66901=ORIENTED_EDGE('',*,*,#50623,.T.);
#66902=ORIENTED_EDGE('',*,*,#50624,.F.);
#66903=ORIENTED_EDGE('',*,*,#50625,.F.);
#66904=ORIENTED_EDGE('',*,*,#50626,.T.);
#66905=ORIENTED_EDGE('',*,*,#50627,.T.);
#66906=ORIENTED_EDGE('',*,*,#50628,.F.);
#66907=ORIENTED_EDGE('',*,*,#50623,.F.);
#66908=ORIENTED_EDGE('',*,*,#50629,.T.);
#66909=ORIENTED_EDGE('',*,*,#50630,.T.);
#66910=ORIENTED_EDGE('',*,*,#50631,.F.);
#66911=ORIENTED_EDGE('',*,*,#50627,.F.);
#66912=ORIENTED_EDGE('',*,*,#50632,.T.);
#66913=ORIENTED_EDGE('',*,*,#50625,.T.);
#66914=ORIENTED_EDGE('',*,*,#50633,.F.);
#66915=ORIENTED_EDGE('',*,*,#50630,.F.);
#66916=ORIENTED_EDGE('',*,*,#50634,.T.);
#66917=ORIENTED_EDGE('',*,*,#50635,.T.);
#66918=ORIENTED_EDGE('',*,*,#50636,.F.);
#66919=ORIENTED_EDGE('',*,*,#50637,.F.);
#66920=ORIENTED_EDGE('',*,*,#50638,.T.);
#66921=ORIENTED_EDGE('',*,*,#50639,.T.);
#66922=ORIENTED_EDGE('',*,*,#50640,.F.);
#66923=ORIENTED_EDGE('',*,*,#50635,.F.);
#66924=ORIENTED_EDGE('',*,*,#50641,.T.);
#66925=ORIENTED_EDGE('',*,*,#50642,.T.);
#66926=ORIENTED_EDGE('',*,*,#50643,.F.);
#66927=ORIENTED_EDGE('',*,*,#50639,.F.);
#66928=ORIENTED_EDGE('',*,*,#50644,.T.);
#66929=ORIENTED_EDGE('',*,*,#50637,.T.);
#66930=ORIENTED_EDGE('',*,*,#50645,.F.);
#66931=ORIENTED_EDGE('',*,*,#50642,.F.);
#66932=ORIENTED_EDGE('',*,*,#50646,.T.);
#66933=ORIENTED_EDGE('',*,*,#50647,.T.);
#66934=ORIENTED_EDGE('',*,*,#50648,.F.);
#66935=ORIENTED_EDGE('',*,*,#50649,.F.);
#66936=ORIENTED_EDGE('',*,*,#50650,.T.);
#66937=ORIENTED_EDGE('',*,*,#50651,.T.);
#66938=ORIENTED_EDGE('',*,*,#50652,.F.);
#66939=ORIENTED_EDGE('',*,*,#50647,.F.);
#66940=ORIENTED_EDGE('',*,*,#50653,.T.);
#66941=ORIENTED_EDGE('',*,*,#50654,.T.);
#66942=ORIENTED_EDGE('',*,*,#50655,.F.);
#66943=ORIENTED_EDGE('',*,*,#50651,.F.);
#66944=ORIENTED_EDGE('',*,*,#50656,.T.);
#66945=ORIENTED_EDGE('',*,*,#50649,.T.);
#66946=ORIENTED_EDGE('',*,*,#50657,.F.);
#66947=ORIENTED_EDGE('',*,*,#50654,.F.);
#66948=ORIENTED_EDGE('',*,*,#50658,.T.);
#66949=ORIENTED_EDGE('',*,*,#50659,.T.);
#66950=ORIENTED_EDGE('',*,*,#50660,.F.);
#66951=ORIENTED_EDGE('',*,*,#50661,.F.);
#66952=ORIENTED_EDGE('',*,*,#50662,.T.);
#66953=ORIENTED_EDGE('',*,*,#50663,.T.);
#66954=ORIENTED_EDGE('',*,*,#50664,.F.);
#66955=ORIENTED_EDGE('',*,*,#50659,.F.);
#66956=ORIENTED_EDGE('',*,*,#50665,.T.);
#66957=ORIENTED_EDGE('',*,*,#50666,.T.);
#66958=ORIENTED_EDGE('',*,*,#50667,.F.);
#66959=ORIENTED_EDGE('',*,*,#50663,.F.);
#66960=ORIENTED_EDGE('',*,*,#50668,.T.);
#66961=ORIENTED_EDGE('',*,*,#50661,.T.);
#66962=ORIENTED_EDGE('',*,*,#50669,.F.);
#66963=ORIENTED_EDGE('',*,*,#50666,.F.);
#66964=ORIENTED_EDGE('',*,*,#50670,.T.);
#66965=ORIENTED_EDGE('',*,*,#50671,.T.);
#66966=ORIENTED_EDGE('',*,*,#50672,.F.);
#66967=ORIENTED_EDGE('',*,*,#50673,.F.);
#66968=ORIENTED_EDGE('',*,*,#50674,.T.);
#66969=ORIENTED_EDGE('',*,*,#50675,.T.);
#66970=ORIENTED_EDGE('',*,*,#50676,.F.);
#66971=ORIENTED_EDGE('',*,*,#50671,.F.);
#66972=ORIENTED_EDGE('',*,*,#50677,.T.);
#66973=ORIENTED_EDGE('',*,*,#50678,.T.);
#66974=ORIENTED_EDGE('',*,*,#50679,.F.);
#66975=ORIENTED_EDGE('',*,*,#50675,.F.);
#66976=ORIENTED_EDGE('',*,*,#50680,.T.);
#66977=ORIENTED_EDGE('',*,*,#50673,.T.);
#66978=ORIENTED_EDGE('',*,*,#50681,.F.);
#66979=ORIENTED_EDGE('',*,*,#50678,.F.);
#66980=ORIENTED_EDGE('',*,*,#50682,.T.);
#66981=ORIENTED_EDGE('',*,*,#50683,.T.);
#66982=ORIENTED_EDGE('',*,*,#50684,.F.);
#66983=ORIENTED_EDGE('',*,*,#50685,.F.);
#66984=ORIENTED_EDGE('',*,*,#50686,.T.);
#66985=ORIENTED_EDGE('',*,*,#50687,.T.);
#66986=ORIENTED_EDGE('',*,*,#50688,.F.);
#66987=ORIENTED_EDGE('',*,*,#50683,.F.);
#66988=ORIENTED_EDGE('',*,*,#50689,.T.);
#66989=ORIENTED_EDGE('',*,*,#50690,.T.);
#66990=ORIENTED_EDGE('',*,*,#50691,.F.);
#66991=ORIENTED_EDGE('',*,*,#50687,.F.);
#66992=ORIENTED_EDGE('',*,*,#50692,.T.);
#66993=ORIENTED_EDGE('',*,*,#50685,.T.);
#66994=ORIENTED_EDGE('',*,*,#50693,.F.);
#66995=ORIENTED_EDGE('',*,*,#50690,.F.);
#66996=ORIENTED_EDGE('',*,*,#50694,.T.);
#66997=ORIENTED_EDGE('',*,*,#50695,.T.);
#66998=ORIENTED_EDGE('',*,*,#50696,.F.);
#66999=ORIENTED_EDGE('',*,*,#50697,.F.);
#67000=ORIENTED_EDGE('',*,*,#50698,.T.);
#67001=ORIENTED_EDGE('',*,*,#50699,.T.);
#67002=ORIENTED_EDGE('',*,*,#50700,.F.);
#67003=ORIENTED_EDGE('',*,*,#50695,.F.);
#67004=ORIENTED_EDGE('',*,*,#50701,.T.);
#67005=ORIENTED_EDGE('',*,*,#50702,.T.);
#67006=ORIENTED_EDGE('',*,*,#50703,.F.);
#67007=ORIENTED_EDGE('',*,*,#50699,.F.);
#67008=ORIENTED_EDGE('',*,*,#50704,.T.);
#67009=ORIENTED_EDGE('',*,*,#50697,.T.);
#67010=ORIENTED_EDGE('',*,*,#50705,.F.);
#67011=ORIENTED_EDGE('',*,*,#50702,.F.);
#67012=ORIENTED_EDGE('',*,*,#50706,.T.);
#67013=ORIENTED_EDGE('',*,*,#50707,.T.);
#67014=ORIENTED_EDGE('',*,*,#50708,.F.);
#67015=ORIENTED_EDGE('',*,*,#50709,.F.);
#67016=ORIENTED_EDGE('',*,*,#50710,.T.);
#67017=ORIENTED_EDGE('',*,*,#50711,.T.);
#67018=ORIENTED_EDGE('',*,*,#50712,.F.);
#67019=ORIENTED_EDGE('',*,*,#50707,.F.);
#67020=ORIENTED_EDGE('',*,*,#50713,.T.);
#67021=ORIENTED_EDGE('',*,*,#50714,.T.);
#67022=ORIENTED_EDGE('',*,*,#50715,.F.);
#67023=ORIENTED_EDGE('',*,*,#50711,.F.);
#67024=ORIENTED_EDGE('',*,*,#50716,.T.);
#67025=ORIENTED_EDGE('',*,*,#50709,.T.);
#67026=ORIENTED_EDGE('',*,*,#50717,.F.);
#67027=ORIENTED_EDGE('',*,*,#50714,.F.);
#67028=ORIENTED_EDGE('',*,*,#50718,.T.);
#67029=ORIENTED_EDGE('',*,*,#50719,.T.);
#67030=ORIENTED_EDGE('',*,*,#50720,.F.);
#67031=ORIENTED_EDGE('',*,*,#50721,.F.);
#67032=ORIENTED_EDGE('',*,*,#50722,.T.);
#67033=ORIENTED_EDGE('',*,*,#50723,.T.);
#67034=ORIENTED_EDGE('',*,*,#50724,.F.);
#67035=ORIENTED_EDGE('',*,*,#50719,.F.);
#67036=ORIENTED_EDGE('',*,*,#50725,.T.);
#67037=ORIENTED_EDGE('',*,*,#50726,.T.);
#67038=ORIENTED_EDGE('',*,*,#50727,.F.);
#67039=ORIENTED_EDGE('',*,*,#50723,.F.);
#67040=ORIENTED_EDGE('',*,*,#50728,.T.);
#67041=ORIENTED_EDGE('',*,*,#50721,.T.);
#67042=ORIENTED_EDGE('',*,*,#50729,.F.);
#67043=ORIENTED_EDGE('',*,*,#50726,.F.);
#67044=ORIENTED_EDGE('',*,*,#50730,.T.);
#67045=ORIENTED_EDGE('',*,*,#50731,.T.);
#67046=ORIENTED_EDGE('',*,*,#50732,.F.);
#67047=ORIENTED_EDGE('',*,*,#50733,.F.);
#67048=ORIENTED_EDGE('',*,*,#50734,.T.);
#67049=ORIENTED_EDGE('',*,*,#50735,.T.);
#67050=ORIENTED_EDGE('',*,*,#50736,.F.);
#67051=ORIENTED_EDGE('',*,*,#50731,.F.);
#67052=ORIENTED_EDGE('',*,*,#50737,.T.);
#67053=ORIENTED_EDGE('',*,*,#50738,.T.);
#67054=ORIENTED_EDGE('',*,*,#50739,.F.);
#67055=ORIENTED_EDGE('',*,*,#50735,.F.);
#67056=ORIENTED_EDGE('',*,*,#50740,.T.);
#67057=ORIENTED_EDGE('',*,*,#50733,.T.);
#67058=ORIENTED_EDGE('',*,*,#50741,.F.);
#67059=ORIENTED_EDGE('',*,*,#50738,.F.);
#67060=ORIENTED_EDGE('',*,*,#50742,.T.);
#67061=ORIENTED_EDGE('',*,*,#50743,.T.);
#67062=ORIENTED_EDGE('',*,*,#50744,.F.);
#67063=ORIENTED_EDGE('',*,*,#50745,.F.);
#67064=ORIENTED_EDGE('',*,*,#50746,.T.);
#67065=ORIENTED_EDGE('',*,*,#50747,.T.);
#67066=ORIENTED_EDGE('',*,*,#50748,.F.);
#67067=ORIENTED_EDGE('',*,*,#50743,.F.);
#67068=ORIENTED_EDGE('',*,*,#50749,.T.);
#67069=ORIENTED_EDGE('',*,*,#50750,.T.);
#67070=ORIENTED_EDGE('',*,*,#50751,.F.);
#67071=ORIENTED_EDGE('',*,*,#50747,.F.);
#67072=ORIENTED_EDGE('',*,*,#50752,.T.);
#67073=ORIENTED_EDGE('',*,*,#50745,.T.);
#67074=ORIENTED_EDGE('',*,*,#50753,.F.);
#67075=ORIENTED_EDGE('',*,*,#50750,.F.);
#67076=ORIENTED_EDGE('',*,*,#50754,.T.);
#67077=ORIENTED_EDGE('',*,*,#50755,.T.);
#67078=ORIENTED_EDGE('',*,*,#50756,.F.);
#67079=ORIENTED_EDGE('',*,*,#50757,.F.);
#67080=ORIENTED_EDGE('',*,*,#50758,.T.);
#67081=ORIENTED_EDGE('',*,*,#50759,.T.);
#67082=ORIENTED_EDGE('',*,*,#50760,.F.);
#67083=ORIENTED_EDGE('',*,*,#50755,.F.);
#67084=ORIENTED_EDGE('',*,*,#50761,.T.);
#67085=ORIENTED_EDGE('',*,*,#50762,.T.);
#67086=ORIENTED_EDGE('',*,*,#50763,.F.);
#67087=ORIENTED_EDGE('',*,*,#50759,.F.);
#67088=ORIENTED_EDGE('',*,*,#50764,.T.);
#67089=ORIENTED_EDGE('',*,*,#50757,.T.);
#67090=ORIENTED_EDGE('',*,*,#50765,.F.);
#67091=ORIENTED_EDGE('',*,*,#50762,.F.);
#67092=ORIENTED_EDGE('',*,*,#50766,.T.);
#67093=ORIENTED_EDGE('',*,*,#50767,.T.);
#67094=ORIENTED_EDGE('',*,*,#50768,.F.);
#67095=ORIENTED_EDGE('',*,*,#50769,.F.);
#67096=ORIENTED_EDGE('',*,*,#50770,.T.);
#67097=ORIENTED_EDGE('',*,*,#50771,.T.);
#67098=ORIENTED_EDGE('',*,*,#50772,.F.);
#67099=ORIENTED_EDGE('',*,*,#50767,.F.);
#67100=ORIENTED_EDGE('',*,*,#50773,.T.);
#67101=ORIENTED_EDGE('',*,*,#50774,.T.);
#67102=ORIENTED_EDGE('',*,*,#50775,.F.);
#67103=ORIENTED_EDGE('',*,*,#50771,.F.);
#67104=ORIENTED_EDGE('',*,*,#50776,.T.);
#67105=ORIENTED_EDGE('',*,*,#50769,.T.);
#67106=ORIENTED_EDGE('',*,*,#50777,.F.);
#67107=ORIENTED_EDGE('',*,*,#50774,.F.);
#67108=ORIENTED_EDGE('',*,*,#50778,.T.);
#67109=ORIENTED_EDGE('',*,*,#50779,.T.);
#67110=ORIENTED_EDGE('',*,*,#50780,.F.);
#67111=ORIENTED_EDGE('',*,*,#50781,.F.);
#67112=ORIENTED_EDGE('',*,*,#50782,.T.);
#67113=ORIENTED_EDGE('',*,*,#50783,.T.);
#67114=ORIENTED_EDGE('',*,*,#50784,.F.);
#67115=ORIENTED_EDGE('',*,*,#50779,.F.);
#67116=ORIENTED_EDGE('',*,*,#50785,.T.);
#67117=ORIENTED_EDGE('',*,*,#50786,.T.);
#67118=ORIENTED_EDGE('',*,*,#50787,.F.);
#67119=ORIENTED_EDGE('',*,*,#50783,.F.);
#67120=ORIENTED_EDGE('',*,*,#50788,.T.);
#67121=ORIENTED_EDGE('',*,*,#50781,.T.);
#67122=ORIENTED_EDGE('',*,*,#50789,.F.);
#67123=ORIENTED_EDGE('',*,*,#50786,.F.);
#67124=ORIENTED_EDGE('',*,*,#50790,.T.);
#67125=ORIENTED_EDGE('',*,*,#50791,.T.);
#67126=ORIENTED_EDGE('',*,*,#50792,.F.);
#67127=ORIENTED_EDGE('',*,*,#50793,.F.);
#67128=ORIENTED_EDGE('',*,*,#50794,.T.);
#67129=ORIENTED_EDGE('',*,*,#50795,.T.);
#67130=ORIENTED_EDGE('',*,*,#50796,.F.);
#67131=ORIENTED_EDGE('',*,*,#50791,.F.);
#67132=ORIENTED_EDGE('',*,*,#50797,.T.);
#67133=ORIENTED_EDGE('',*,*,#50798,.T.);
#67134=ORIENTED_EDGE('',*,*,#50799,.F.);
#67135=ORIENTED_EDGE('',*,*,#50795,.F.);
#67136=ORIENTED_EDGE('',*,*,#50800,.T.);
#67137=ORIENTED_EDGE('',*,*,#50793,.T.);
#67138=ORIENTED_EDGE('',*,*,#50801,.F.);
#67139=ORIENTED_EDGE('',*,*,#50798,.F.);
#67140=ORIENTED_EDGE('',*,*,#50802,.T.);
#67141=ORIENTED_EDGE('',*,*,#50803,.T.);
#67142=ORIENTED_EDGE('',*,*,#50804,.F.);
#67143=ORIENTED_EDGE('',*,*,#50805,.F.);
#67144=ORIENTED_EDGE('',*,*,#50806,.T.);
#67145=ORIENTED_EDGE('',*,*,#50807,.T.);
#67146=ORIENTED_EDGE('',*,*,#50808,.F.);
#67147=ORIENTED_EDGE('',*,*,#50803,.F.);
#67148=ORIENTED_EDGE('',*,*,#50809,.T.);
#67149=ORIENTED_EDGE('',*,*,#50810,.T.);
#67150=ORIENTED_EDGE('',*,*,#50811,.F.);
#67151=ORIENTED_EDGE('',*,*,#50807,.F.);
#67152=ORIENTED_EDGE('',*,*,#50812,.T.);
#67153=ORIENTED_EDGE('',*,*,#50805,.T.);
#67154=ORIENTED_EDGE('',*,*,#50813,.F.);
#67155=ORIENTED_EDGE('',*,*,#50810,.F.);
#67156=ORIENTED_EDGE('',*,*,#50814,.T.);
#67157=ORIENTED_EDGE('',*,*,#50815,.T.);
#67158=ORIENTED_EDGE('',*,*,#50816,.F.);
#67159=ORIENTED_EDGE('',*,*,#50817,.F.);
#67160=ORIENTED_EDGE('',*,*,#50818,.T.);
#67161=ORIENTED_EDGE('',*,*,#50819,.T.);
#67162=ORIENTED_EDGE('',*,*,#50820,.F.);
#67163=ORIENTED_EDGE('',*,*,#50815,.F.);
#67164=ORIENTED_EDGE('',*,*,#50821,.T.);
#67165=ORIENTED_EDGE('',*,*,#50822,.T.);
#67166=ORIENTED_EDGE('',*,*,#50823,.F.);
#67167=ORIENTED_EDGE('',*,*,#50819,.F.);
#67168=ORIENTED_EDGE('',*,*,#50824,.T.);
#67169=ORIENTED_EDGE('',*,*,#50817,.T.);
#67170=ORIENTED_EDGE('',*,*,#50825,.F.);
#67171=ORIENTED_EDGE('',*,*,#50822,.F.);
#67172=ORIENTED_EDGE('',*,*,#50826,.T.);
#67173=ORIENTED_EDGE('',*,*,#50827,.T.);
#67174=ORIENTED_EDGE('',*,*,#50828,.F.);
#67175=ORIENTED_EDGE('',*,*,#50829,.F.);
#67176=ORIENTED_EDGE('',*,*,#50830,.T.);
#67177=ORIENTED_EDGE('',*,*,#50831,.T.);
#67178=ORIENTED_EDGE('',*,*,#50832,.F.);
#67179=ORIENTED_EDGE('',*,*,#50827,.F.);
#67180=ORIENTED_EDGE('',*,*,#50833,.T.);
#67181=ORIENTED_EDGE('',*,*,#50834,.T.);
#67182=ORIENTED_EDGE('',*,*,#50835,.F.);
#67183=ORIENTED_EDGE('',*,*,#50831,.F.);
#67184=ORIENTED_EDGE('',*,*,#50836,.T.);
#67185=ORIENTED_EDGE('',*,*,#50829,.T.);
#67186=ORIENTED_EDGE('',*,*,#50837,.F.);
#67187=ORIENTED_EDGE('',*,*,#50834,.F.);
#67188=ORIENTED_EDGE('',*,*,#50838,.T.);
#67189=ORIENTED_EDGE('',*,*,#50839,.T.);
#67190=ORIENTED_EDGE('',*,*,#50840,.F.);
#67191=ORIENTED_EDGE('',*,*,#50841,.F.);
#67192=ORIENTED_EDGE('',*,*,#50842,.T.);
#67193=ORIENTED_EDGE('',*,*,#50843,.T.);
#67194=ORIENTED_EDGE('',*,*,#50844,.F.);
#67195=ORIENTED_EDGE('',*,*,#50839,.F.);
#67196=ORIENTED_EDGE('',*,*,#50845,.T.);
#67197=ORIENTED_EDGE('',*,*,#50846,.T.);
#67198=ORIENTED_EDGE('',*,*,#50847,.F.);
#67199=ORIENTED_EDGE('',*,*,#50843,.F.);
#67200=ORIENTED_EDGE('',*,*,#50848,.T.);
#67201=ORIENTED_EDGE('',*,*,#50841,.T.);
#67202=ORIENTED_EDGE('',*,*,#50849,.F.);
#67203=ORIENTED_EDGE('',*,*,#50846,.F.);
#67204=ORIENTED_EDGE('',*,*,#50850,.T.);
#67205=ORIENTED_EDGE('',*,*,#50851,.T.);
#67206=ORIENTED_EDGE('',*,*,#50852,.F.);
#67207=ORIENTED_EDGE('',*,*,#50853,.F.);
#67208=ORIENTED_EDGE('',*,*,#50854,.T.);
#67209=ORIENTED_EDGE('',*,*,#50855,.T.);
#67210=ORIENTED_EDGE('',*,*,#50856,.F.);
#67211=ORIENTED_EDGE('',*,*,#50851,.F.);
#67212=ORIENTED_EDGE('',*,*,#50857,.T.);
#67213=ORIENTED_EDGE('',*,*,#50858,.T.);
#67214=ORIENTED_EDGE('',*,*,#50859,.F.);
#67215=ORIENTED_EDGE('',*,*,#50855,.F.);
#67216=ORIENTED_EDGE('',*,*,#50860,.T.);
#67217=ORIENTED_EDGE('',*,*,#50853,.T.);
#67218=ORIENTED_EDGE('',*,*,#50861,.F.);
#67219=ORIENTED_EDGE('',*,*,#50858,.F.);
#67220=ORIENTED_EDGE('',*,*,#50862,.T.);
#67221=ORIENTED_EDGE('',*,*,#50863,.T.);
#67222=ORIENTED_EDGE('',*,*,#50864,.F.);
#67223=ORIENTED_EDGE('',*,*,#50865,.F.);
#67224=ORIENTED_EDGE('',*,*,#50866,.T.);
#67225=ORIENTED_EDGE('',*,*,#50867,.T.);
#67226=ORIENTED_EDGE('',*,*,#50868,.F.);
#67227=ORIENTED_EDGE('',*,*,#50863,.F.);
#67228=ORIENTED_EDGE('',*,*,#50869,.T.);
#67229=ORIENTED_EDGE('',*,*,#50870,.T.);
#67230=ORIENTED_EDGE('',*,*,#50871,.F.);
#67231=ORIENTED_EDGE('',*,*,#50867,.F.);
#67232=ORIENTED_EDGE('',*,*,#50872,.T.);
#67233=ORIENTED_EDGE('',*,*,#50865,.T.);
#67234=ORIENTED_EDGE('',*,*,#50873,.F.);
#67235=ORIENTED_EDGE('',*,*,#50870,.F.);
#67236=ORIENTED_EDGE('',*,*,#50874,.T.);
#67237=ORIENTED_EDGE('',*,*,#50875,.T.);
#67238=ORIENTED_EDGE('',*,*,#50876,.F.);
#67239=ORIENTED_EDGE('',*,*,#50877,.F.);
#67240=ORIENTED_EDGE('',*,*,#50878,.T.);
#67241=ORIENTED_EDGE('',*,*,#50879,.T.);
#67242=ORIENTED_EDGE('',*,*,#50880,.F.);
#67243=ORIENTED_EDGE('',*,*,#50875,.F.);
#67244=ORIENTED_EDGE('',*,*,#50881,.T.);
#67245=ORIENTED_EDGE('',*,*,#50882,.T.);
#67246=ORIENTED_EDGE('',*,*,#50883,.F.);
#67247=ORIENTED_EDGE('',*,*,#50879,.F.);
#67248=ORIENTED_EDGE('',*,*,#50884,.T.);
#67249=ORIENTED_EDGE('',*,*,#50877,.T.);
#67250=ORIENTED_EDGE('',*,*,#50885,.F.);
#67251=ORIENTED_EDGE('',*,*,#50882,.F.);
#67252=ORIENTED_EDGE('',*,*,#50886,.T.);
#67253=ORIENTED_EDGE('',*,*,#50887,.T.);
#67254=ORIENTED_EDGE('',*,*,#50888,.F.);
#67255=ORIENTED_EDGE('',*,*,#50889,.F.);
#67256=ORIENTED_EDGE('',*,*,#50890,.T.);
#67257=ORIENTED_EDGE('',*,*,#50891,.T.);
#67258=ORIENTED_EDGE('',*,*,#50892,.F.);
#67259=ORIENTED_EDGE('',*,*,#50887,.F.);
#67260=ORIENTED_EDGE('',*,*,#50893,.T.);
#67261=ORIENTED_EDGE('',*,*,#50894,.T.);
#67262=ORIENTED_EDGE('',*,*,#50895,.F.);
#67263=ORIENTED_EDGE('',*,*,#50891,.F.);
#67264=ORIENTED_EDGE('',*,*,#50896,.T.);
#67265=ORIENTED_EDGE('',*,*,#50889,.T.);
#67266=ORIENTED_EDGE('',*,*,#50897,.F.);
#67267=ORIENTED_EDGE('',*,*,#50894,.F.);
#67268=ORIENTED_EDGE('',*,*,#50898,.T.);
#67269=ORIENTED_EDGE('',*,*,#50899,.T.);
#67270=ORIENTED_EDGE('',*,*,#50900,.F.);
#67271=ORIENTED_EDGE('',*,*,#50901,.F.);
#67272=ORIENTED_EDGE('',*,*,#50902,.T.);
#67273=ORIENTED_EDGE('',*,*,#50903,.T.);
#67274=ORIENTED_EDGE('',*,*,#50904,.F.);
#67275=ORIENTED_EDGE('',*,*,#50899,.F.);
#67276=ORIENTED_EDGE('',*,*,#50905,.T.);
#67277=ORIENTED_EDGE('',*,*,#50906,.T.);
#67278=ORIENTED_EDGE('',*,*,#50907,.F.);
#67279=ORIENTED_EDGE('',*,*,#50903,.F.);
#67280=ORIENTED_EDGE('',*,*,#50908,.T.);
#67281=ORIENTED_EDGE('',*,*,#50901,.T.);
#67282=ORIENTED_EDGE('',*,*,#50909,.F.);
#67283=ORIENTED_EDGE('',*,*,#50906,.F.);
#67284=ORIENTED_EDGE('',*,*,#50910,.T.);
#67285=ORIENTED_EDGE('',*,*,#50911,.T.);
#67286=ORIENTED_EDGE('',*,*,#50912,.F.);
#67287=ORIENTED_EDGE('',*,*,#50913,.F.);
#67288=ORIENTED_EDGE('',*,*,#50914,.T.);
#67289=ORIENTED_EDGE('',*,*,#50915,.T.);
#67290=ORIENTED_EDGE('',*,*,#50916,.F.);
#67291=ORIENTED_EDGE('',*,*,#50911,.F.);
#67292=ORIENTED_EDGE('',*,*,#50917,.T.);
#67293=ORIENTED_EDGE('',*,*,#50918,.T.);
#67294=ORIENTED_EDGE('',*,*,#50919,.F.);
#67295=ORIENTED_EDGE('',*,*,#50915,.F.);
#67296=ORIENTED_EDGE('',*,*,#50920,.T.);
#67297=ORIENTED_EDGE('',*,*,#50913,.T.);
#67298=ORIENTED_EDGE('',*,*,#50921,.F.);
#67299=ORIENTED_EDGE('',*,*,#50918,.F.);
#67300=ORIENTED_EDGE('',*,*,#50922,.T.);
#67301=ORIENTED_EDGE('',*,*,#50923,.T.);
#67302=ORIENTED_EDGE('',*,*,#50924,.F.);
#67303=ORIENTED_EDGE('',*,*,#50925,.F.);
#67304=ORIENTED_EDGE('',*,*,#50926,.T.);
#67305=ORIENTED_EDGE('',*,*,#50927,.T.);
#67306=ORIENTED_EDGE('',*,*,#50928,.F.);
#67307=ORIENTED_EDGE('',*,*,#50923,.F.);
#67308=ORIENTED_EDGE('',*,*,#50929,.T.);
#67309=ORIENTED_EDGE('',*,*,#50930,.T.);
#67310=ORIENTED_EDGE('',*,*,#50931,.F.);
#67311=ORIENTED_EDGE('',*,*,#50927,.F.);
#67312=ORIENTED_EDGE('',*,*,#50932,.T.);
#67313=ORIENTED_EDGE('',*,*,#50925,.T.);
#67314=ORIENTED_EDGE('',*,*,#50933,.F.);
#67315=ORIENTED_EDGE('',*,*,#50930,.F.);
#67316=ORIENTED_EDGE('',*,*,#50934,.T.);
#67317=ORIENTED_EDGE('',*,*,#50935,.T.);
#67318=ORIENTED_EDGE('',*,*,#50936,.F.);
#67319=ORIENTED_EDGE('',*,*,#50937,.F.);
#67320=ORIENTED_EDGE('',*,*,#50938,.T.);
#67321=ORIENTED_EDGE('',*,*,#50939,.T.);
#67322=ORIENTED_EDGE('',*,*,#50940,.F.);
#67323=ORIENTED_EDGE('',*,*,#50935,.F.);
#67324=ORIENTED_EDGE('',*,*,#50941,.T.);
#67325=ORIENTED_EDGE('',*,*,#50942,.T.);
#67326=ORIENTED_EDGE('',*,*,#50943,.F.);
#67327=ORIENTED_EDGE('',*,*,#50939,.F.);
#67328=ORIENTED_EDGE('',*,*,#50944,.T.);
#67329=ORIENTED_EDGE('',*,*,#50937,.T.);
#67330=ORIENTED_EDGE('',*,*,#50945,.F.);
#67331=ORIENTED_EDGE('',*,*,#50942,.F.);
#67332=ORIENTED_EDGE('',*,*,#50946,.T.);
#67333=ORIENTED_EDGE('',*,*,#50947,.T.);
#67334=ORIENTED_EDGE('',*,*,#50948,.F.);
#67335=ORIENTED_EDGE('',*,*,#50949,.F.);
#67336=ORIENTED_EDGE('',*,*,#50950,.T.);
#67337=ORIENTED_EDGE('',*,*,#50951,.T.);
#67338=ORIENTED_EDGE('',*,*,#50952,.F.);
#67339=ORIENTED_EDGE('',*,*,#50947,.F.);
#67340=ORIENTED_EDGE('',*,*,#50953,.T.);
#67341=ORIENTED_EDGE('',*,*,#50954,.T.);
#67342=ORIENTED_EDGE('',*,*,#50955,.F.);
#67343=ORIENTED_EDGE('',*,*,#50951,.F.);
#67344=ORIENTED_EDGE('',*,*,#50956,.T.);
#67345=ORIENTED_EDGE('',*,*,#50949,.T.);
#67346=ORIENTED_EDGE('',*,*,#50957,.F.);
#67347=ORIENTED_EDGE('',*,*,#50954,.F.);
#67348=ORIENTED_EDGE('',*,*,#50958,.T.);
#67349=ORIENTED_EDGE('',*,*,#50959,.T.);
#67350=ORIENTED_EDGE('',*,*,#50960,.F.);
#67351=ORIENTED_EDGE('',*,*,#50961,.F.);
#67352=ORIENTED_EDGE('',*,*,#50962,.T.);
#67353=ORIENTED_EDGE('',*,*,#50963,.T.);
#67354=ORIENTED_EDGE('',*,*,#50964,.F.);
#67355=ORIENTED_EDGE('',*,*,#50959,.F.);
#67356=ORIENTED_EDGE('',*,*,#50965,.T.);
#67357=ORIENTED_EDGE('',*,*,#50966,.T.);
#67358=ORIENTED_EDGE('',*,*,#50967,.F.);
#67359=ORIENTED_EDGE('',*,*,#50963,.F.);
#67360=ORIENTED_EDGE('',*,*,#50968,.T.);
#67361=ORIENTED_EDGE('',*,*,#50961,.T.);
#67362=ORIENTED_EDGE('',*,*,#50969,.F.);
#67363=ORIENTED_EDGE('',*,*,#50966,.F.);
#67364=ORIENTED_EDGE('',*,*,#50970,.T.);
#67365=ORIENTED_EDGE('',*,*,#50971,.T.);
#67366=ORIENTED_EDGE('',*,*,#50972,.F.);
#67367=ORIENTED_EDGE('',*,*,#50973,.F.);
#67368=ORIENTED_EDGE('',*,*,#50974,.T.);
#67369=ORIENTED_EDGE('',*,*,#50975,.T.);
#67370=ORIENTED_EDGE('',*,*,#50976,.F.);
#67371=ORIENTED_EDGE('',*,*,#50971,.F.);
#67372=ORIENTED_EDGE('',*,*,#50977,.T.);
#67373=ORIENTED_EDGE('',*,*,#50978,.T.);
#67374=ORIENTED_EDGE('',*,*,#50979,.F.);
#67375=ORIENTED_EDGE('',*,*,#50975,.F.);
#67376=ORIENTED_EDGE('',*,*,#50980,.T.);
#67377=ORIENTED_EDGE('',*,*,#50973,.T.);
#67378=ORIENTED_EDGE('',*,*,#50981,.F.);
#67379=ORIENTED_EDGE('',*,*,#50978,.F.);
#67380=ORIENTED_EDGE('',*,*,#50982,.T.);
#67381=ORIENTED_EDGE('',*,*,#50983,.T.);
#67382=ORIENTED_EDGE('',*,*,#50984,.F.);
#67383=ORIENTED_EDGE('',*,*,#50985,.F.);
#67384=ORIENTED_EDGE('',*,*,#50986,.T.);
#67385=ORIENTED_EDGE('',*,*,#50987,.T.);
#67386=ORIENTED_EDGE('',*,*,#50988,.F.);
#67387=ORIENTED_EDGE('',*,*,#50983,.F.);
#67388=ORIENTED_EDGE('',*,*,#50989,.T.);
#67389=ORIENTED_EDGE('',*,*,#50990,.T.);
#67390=ORIENTED_EDGE('',*,*,#50991,.F.);
#67391=ORIENTED_EDGE('',*,*,#50987,.F.);
#67392=ORIENTED_EDGE('',*,*,#50992,.T.);
#67393=ORIENTED_EDGE('',*,*,#50985,.T.);
#67394=ORIENTED_EDGE('',*,*,#50993,.F.);
#67395=ORIENTED_EDGE('',*,*,#50990,.F.);
#67396=ORIENTED_EDGE('',*,*,#50994,.T.);
#67397=ORIENTED_EDGE('',*,*,#50995,.T.);
#67398=ORIENTED_EDGE('',*,*,#50996,.F.);
#67399=ORIENTED_EDGE('',*,*,#50997,.F.);
#67400=ORIENTED_EDGE('',*,*,#50998,.T.);
#67401=ORIENTED_EDGE('',*,*,#50999,.T.);
#67402=ORIENTED_EDGE('',*,*,#51000,.F.);
#67403=ORIENTED_EDGE('',*,*,#50995,.F.);
#67404=ORIENTED_EDGE('',*,*,#51001,.T.);
#67405=ORIENTED_EDGE('',*,*,#51002,.T.);
#67406=ORIENTED_EDGE('',*,*,#51003,.F.);
#67407=ORIENTED_EDGE('',*,*,#50999,.F.);
#67408=ORIENTED_EDGE('',*,*,#51004,.T.);
#67409=ORIENTED_EDGE('',*,*,#50997,.T.);
#67410=ORIENTED_EDGE('',*,*,#51005,.F.);
#67411=ORIENTED_EDGE('',*,*,#51002,.F.);
#67412=ORIENTED_EDGE('',*,*,#51006,.T.);
#67413=ORIENTED_EDGE('',*,*,#51007,.T.);
#67414=ORIENTED_EDGE('',*,*,#51008,.F.);
#67415=ORIENTED_EDGE('',*,*,#51009,.F.);
#67416=ORIENTED_EDGE('',*,*,#51010,.T.);
#67417=ORIENTED_EDGE('',*,*,#51011,.T.);
#67418=ORIENTED_EDGE('',*,*,#51012,.F.);
#67419=ORIENTED_EDGE('',*,*,#51007,.F.);
#67420=ORIENTED_EDGE('',*,*,#51013,.T.);
#67421=ORIENTED_EDGE('',*,*,#51014,.T.);
#67422=ORIENTED_EDGE('',*,*,#51015,.F.);
#67423=ORIENTED_EDGE('',*,*,#51011,.F.);
#67424=ORIENTED_EDGE('',*,*,#51016,.T.);
#67425=ORIENTED_EDGE('',*,*,#51009,.T.);
#67426=ORIENTED_EDGE('',*,*,#51017,.F.);
#67427=ORIENTED_EDGE('',*,*,#51014,.F.);
#67428=ORIENTED_EDGE('',*,*,#51018,.T.);
#67429=ORIENTED_EDGE('',*,*,#51019,.T.);
#67430=ORIENTED_EDGE('',*,*,#51020,.F.);
#67431=ORIENTED_EDGE('',*,*,#51021,.F.);
#67432=ORIENTED_EDGE('',*,*,#51022,.T.);
#67433=ORIENTED_EDGE('',*,*,#51023,.T.);
#67434=ORIENTED_EDGE('',*,*,#51024,.F.);
#67435=ORIENTED_EDGE('',*,*,#51019,.F.);
#67436=ORIENTED_EDGE('',*,*,#51025,.T.);
#67437=ORIENTED_EDGE('',*,*,#51026,.T.);
#67438=ORIENTED_EDGE('',*,*,#51027,.F.);
#67439=ORIENTED_EDGE('',*,*,#51023,.F.);
#67440=ORIENTED_EDGE('',*,*,#51028,.T.);
#67441=ORIENTED_EDGE('',*,*,#51021,.T.);
#67442=ORIENTED_EDGE('',*,*,#51029,.F.);
#67443=ORIENTED_EDGE('',*,*,#51026,.F.);
#67444=ORIENTED_EDGE('',*,*,#51030,.T.);
#67445=ORIENTED_EDGE('',*,*,#51031,.T.);
#67446=ORIENTED_EDGE('',*,*,#51032,.F.);
#67447=ORIENTED_EDGE('',*,*,#51033,.F.);
#67448=ORIENTED_EDGE('',*,*,#51034,.T.);
#67449=ORIENTED_EDGE('',*,*,#51035,.T.);
#67450=ORIENTED_EDGE('',*,*,#51036,.F.);
#67451=ORIENTED_EDGE('',*,*,#51031,.F.);
#67452=ORIENTED_EDGE('',*,*,#51037,.T.);
#67453=ORIENTED_EDGE('',*,*,#51038,.T.);
#67454=ORIENTED_EDGE('',*,*,#51039,.F.);
#67455=ORIENTED_EDGE('',*,*,#51035,.F.);
#67456=ORIENTED_EDGE('',*,*,#51040,.T.);
#67457=ORIENTED_EDGE('',*,*,#51033,.T.);
#67458=ORIENTED_EDGE('',*,*,#51041,.F.);
#67459=ORIENTED_EDGE('',*,*,#51038,.F.);
#67460=ORIENTED_EDGE('',*,*,#51042,.T.);
#67461=ORIENTED_EDGE('',*,*,#51043,.T.);
#67462=ORIENTED_EDGE('',*,*,#51044,.F.);
#67463=ORIENTED_EDGE('',*,*,#51045,.F.);
#67464=ORIENTED_EDGE('',*,*,#51046,.T.);
#67465=ORIENTED_EDGE('',*,*,#51047,.T.);
#67466=ORIENTED_EDGE('',*,*,#51048,.F.);
#67467=ORIENTED_EDGE('',*,*,#51043,.F.);
#67468=ORIENTED_EDGE('',*,*,#51049,.T.);
#67469=ORIENTED_EDGE('',*,*,#51050,.T.);
#67470=ORIENTED_EDGE('',*,*,#51051,.F.);
#67471=ORIENTED_EDGE('',*,*,#51047,.F.);
#67472=ORIENTED_EDGE('',*,*,#51052,.T.);
#67473=ORIENTED_EDGE('',*,*,#51045,.T.);
#67474=ORIENTED_EDGE('',*,*,#51053,.F.);
#67475=ORIENTED_EDGE('',*,*,#51050,.F.);
#67476=ORIENTED_EDGE('',*,*,#51054,.T.);
#67477=ORIENTED_EDGE('',*,*,#51055,.T.);
#67478=ORIENTED_EDGE('',*,*,#51056,.F.);
#67479=ORIENTED_EDGE('',*,*,#51057,.F.);
#67480=ORIENTED_EDGE('',*,*,#51058,.T.);
#67481=ORIENTED_EDGE('',*,*,#51059,.T.);
#67482=ORIENTED_EDGE('',*,*,#51060,.F.);
#67483=ORIENTED_EDGE('',*,*,#51055,.F.);
#67484=ORIENTED_EDGE('',*,*,#51061,.T.);
#67485=ORIENTED_EDGE('',*,*,#51062,.T.);
#67486=ORIENTED_EDGE('',*,*,#51063,.F.);
#67487=ORIENTED_EDGE('',*,*,#51059,.F.);
#67488=ORIENTED_EDGE('',*,*,#51064,.T.);
#67489=ORIENTED_EDGE('',*,*,#51057,.T.);
#67490=ORIENTED_EDGE('',*,*,#51065,.F.);
#67491=ORIENTED_EDGE('',*,*,#51062,.F.);
#67492=ORIENTED_EDGE('',*,*,#51066,.T.);
#67493=ORIENTED_EDGE('',*,*,#51067,.T.);
#67494=ORIENTED_EDGE('',*,*,#51068,.F.);
#67495=ORIENTED_EDGE('',*,*,#51069,.F.);
#67496=ORIENTED_EDGE('',*,*,#51070,.T.);
#67497=ORIENTED_EDGE('',*,*,#51071,.T.);
#67498=ORIENTED_EDGE('',*,*,#51072,.F.);
#67499=ORIENTED_EDGE('',*,*,#51067,.F.);
#67500=ORIENTED_EDGE('',*,*,#51073,.T.);
#67501=ORIENTED_EDGE('',*,*,#51074,.T.);
#67502=ORIENTED_EDGE('',*,*,#51075,.F.);
#67503=ORIENTED_EDGE('',*,*,#51071,.F.);
#67504=ORIENTED_EDGE('',*,*,#51076,.T.);
#67505=ORIENTED_EDGE('',*,*,#51069,.T.);
#67506=ORIENTED_EDGE('',*,*,#51077,.F.);
#67507=ORIENTED_EDGE('',*,*,#51074,.F.);
#67508=ORIENTED_EDGE('',*,*,#51078,.T.);
#67509=ORIENTED_EDGE('',*,*,#51079,.T.);
#67510=ORIENTED_EDGE('',*,*,#51080,.F.);
#67511=ORIENTED_EDGE('',*,*,#51081,.F.);
#67512=ORIENTED_EDGE('',*,*,#51082,.T.);
#67513=ORIENTED_EDGE('',*,*,#51083,.T.);
#67514=ORIENTED_EDGE('',*,*,#51084,.F.);
#67515=ORIENTED_EDGE('',*,*,#51079,.F.);
#67516=ORIENTED_EDGE('',*,*,#51085,.T.);
#67517=ORIENTED_EDGE('',*,*,#51086,.T.);
#67518=ORIENTED_EDGE('',*,*,#51087,.F.);
#67519=ORIENTED_EDGE('',*,*,#51083,.F.);
#67520=ORIENTED_EDGE('',*,*,#51088,.T.);
#67521=ORIENTED_EDGE('',*,*,#51081,.T.);
#67522=ORIENTED_EDGE('',*,*,#51089,.F.);
#67523=ORIENTED_EDGE('',*,*,#51086,.F.);
#67524=ORIENTED_EDGE('',*,*,#51090,.T.);
#67525=ORIENTED_EDGE('',*,*,#51091,.T.);
#67526=ORIENTED_EDGE('',*,*,#51092,.F.);
#67527=ORIENTED_EDGE('',*,*,#51093,.F.);
#67528=ORIENTED_EDGE('',*,*,#51094,.T.);
#67529=ORIENTED_EDGE('',*,*,#51095,.T.);
#67530=ORIENTED_EDGE('',*,*,#51096,.F.);
#67531=ORIENTED_EDGE('',*,*,#51091,.F.);
#67532=ORIENTED_EDGE('',*,*,#51097,.T.);
#67533=ORIENTED_EDGE('',*,*,#51098,.T.);
#67534=ORIENTED_EDGE('',*,*,#51099,.F.);
#67535=ORIENTED_EDGE('',*,*,#51095,.F.);
#67536=ORIENTED_EDGE('',*,*,#51100,.T.);
#67537=ORIENTED_EDGE('',*,*,#51093,.T.);
#67538=ORIENTED_EDGE('',*,*,#51101,.F.);
#67539=ORIENTED_EDGE('',*,*,#51098,.F.);
#67540=ORIENTED_EDGE('',*,*,#51102,.T.);
#67541=ORIENTED_EDGE('',*,*,#51103,.T.);
#67542=ORIENTED_EDGE('',*,*,#51104,.F.);
#67543=ORIENTED_EDGE('',*,*,#51105,.F.);
#67544=ORIENTED_EDGE('',*,*,#51106,.T.);
#67545=ORIENTED_EDGE('',*,*,#51107,.T.);
#67546=ORIENTED_EDGE('',*,*,#51108,.F.);
#67547=ORIENTED_EDGE('',*,*,#51103,.F.);
#67548=ORIENTED_EDGE('',*,*,#51109,.T.);
#67549=ORIENTED_EDGE('',*,*,#51110,.T.);
#67550=ORIENTED_EDGE('',*,*,#51111,.F.);
#67551=ORIENTED_EDGE('',*,*,#51107,.F.);
#67552=ORIENTED_EDGE('',*,*,#51112,.T.);
#67553=ORIENTED_EDGE('',*,*,#51105,.T.);
#67554=ORIENTED_EDGE('',*,*,#51113,.F.);
#67555=ORIENTED_EDGE('',*,*,#51110,.F.);
#67556=ORIENTED_EDGE('',*,*,#51114,.T.);
#67557=ORIENTED_EDGE('',*,*,#51115,.T.);
#67558=ORIENTED_EDGE('',*,*,#51116,.F.);
#67559=ORIENTED_EDGE('',*,*,#51117,.F.);
#67560=ORIENTED_EDGE('',*,*,#51118,.T.);
#67561=ORIENTED_EDGE('',*,*,#51119,.T.);
#67562=ORIENTED_EDGE('',*,*,#51120,.F.);
#67563=ORIENTED_EDGE('',*,*,#51115,.F.);
#67564=ORIENTED_EDGE('',*,*,#51121,.T.);
#67565=ORIENTED_EDGE('',*,*,#51122,.T.);
#67566=ORIENTED_EDGE('',*,*,#51123,.F.);
#67567=ORIENTED_EDGE('',*,*,#51119,.F.);
#67568=ORIENTED_EDGE('',*,*,#51124,.T.);
#67569=ORIENTED_EDGE('',*,*,#51117,.T.);
#67570=ORIENTED_EDGE('',*,*,#51125,.F.);
#67571=ORIENTED_EDGE('',*,*,#51122,.F.);
#67572=ORIENTED_EDGE('',*,*,#51126,.T.);
#67573=ORIENTED_EDGE('',*,*,#51127,.T.);
#67574=ORIENTED_EDGE('',*,*,#51128,.F.);
#67575=ORIENTED_EDGE('',*,*,#51129,.F.);
#67576=ORIENTED_EDGE('',*,*,#51130,.T.);
#67577=ORIENTED_EDGE('',*,*,#51131,.T.);
#67578=ORIENTED_EDGE('',*,*,#51132,.F.);
#67579=ORIENTED_EDGE('',*,*,#51127,.F.);
#67580=ORIENTED_EDGE('',*,*,#51133,.T.);
#67581=ORIENTED_EDGE('',*,*,#51134,.T.);
#67582=ORIENTED_EDGE('',*,*,#51135,.F.);
#67583=ORIENTED_EDGE('',*,*,#51131,.F.);
#67584=ORIENTED_EDGE('',*,*,#51136,.T.);
#67585=ORIENTED_EDGE('',*,*,#51129,.T.);
#67586=ORIENTED_EDGE('',*,*,#51137,.F.);
#67587=ORIENTED_EDGE('',*,*,#51134,.F.);
#67588=ORIENTED_EDGE('',*,*,#51138,.T.);
#67589=ORIENTED_EDGE('',*,*,#51139,.T.);
#67590=ORIENTED_EDGE('',*,*,#51140,.F.);
#67591=ORIENTED_EDGE('',*,*,#51141,.F.);
#67592=ORIENTED_EDGE('',*,*,#51142,.T.);
#67593=ORIENTED_EDGE('',*,*,#51143,.T.);
#67594=ORIENTED_EDGE('',*,*,#51144,.F.);
#67595=ORIENTED_EDGE('',*,*,#51139,.F.);
#67596=ORIENTED_EDGE('',*,*,#51145,.T.);
#67597=ORIENTED_EDGE('',*,*,#51146,.T.);
#67598=ORIENTED_EDGE('',*,*,#51147,.F.);
#67599=ORIENTED_EDGE('',*,*,#51143,.F.);
#67600=ORIENTED_EDGE('',*,*,#51148,.T.);
#67601=ORIENTED_EDGE('',*,*,#51141,.T.);
#67602=ORIENTED_EDGE('',*,*,#51149,.F.);
#67603=ORIENTED_EDGE('',*,*,#51146,.F.);
#67604=ORIENTED_EDGE('',*,*,#51150,.T.);
#67605=ORIENTED_EDGE('',*,*,#51151,.T.);
#67606=ORIENTED_EDGE('',*,*,#51152,.F.);
#67607=ORIENTED_EDGE('',*,*,#51153,.F.);
#67608=ORIENTED_EDGE('',*,*,#51154,.T.);
#67609=ORIENTED_EDGE('',*,*,#51155,.T.);
#67610=ORIENTED_EDGE('',*,*,#51156,.F.);
#67611=ORIENTED_EDGE('',*,*,#51151,.F.);
#67612=ORIENTED_EDGE('',*,*,#51157,.T.);
#67613=ORIENTED_EDGE('',*,*,#51158,.T.);
#67614=ORIENTED_EDGE('',*,*,#51159,.F.);
#67615=ORIENTED_EDGE('',*,*,#51155,.F.);
#67616=ORIENTED_EDGE('',*,*,#51160,.T.);
#67617=ORIENTED_EDGE('',*,*,#51153,.T.);
#67618=ORIENTED_EDGE('',*,*,#51161,.F.);
#67619=ORIENTED_EDGE('',*,*,#51158,.F.);
#67620=ORIENTED_EDGE('',*,*,#51162,.T.);
#67621=ORIENTED_EDGE('',*,*,#51163,.T.);
#67622=ORIENTED_EDGE('',*,*,#51164,.F.);
#67623=ORIENTED_EDGE('',*,*,#51165,.F.);
#67624=ORIENTED_EDGE('',*,*,#51166,.T.);
#67625=ORIENTED_EDGE('',*,*,#51167,.T.);
#67626=ORIENTED_EDGE('',*,*,#51168,.F.);
#67627=ORIENTED_EDGE('',*,*,#51163,.F.);
#67628=ORIENTED_EDGE('',*,*,#51169,.T.);
#67629=ORIENTED_EDGE('',*,*,#51170,.T.);
#67630=ORIENTED_EDGE('',*,*,#51171,.F.);
#67631=ORIENTED_EDGE('',*,*,#51167,.F.);
#67632=ORIENTED_EDGE('',*,*,#51172,.T.);
#67633=ORIENTED_EDGE('',*,*,#51165,.T.);
#67634=ORIENTED_EDGE('',*,*,#51173,.F.);
#67635=ORIENTED_EDGE('',*,*,#51170,.F.);
#67636=ORIENTED_EDGE('',*,*,#51174,.T.);
#67637=ORIENTED_EDGE('',*,*,#51175,.T.);
#67638=ORIENTED_EDGE('',*,*,#51176,.F.);
#67639=ORIENTED_EDGE('',*,*,#51177,.F.);
#67640=ORIENTED_EDGE('',*,*,#51178,.T.);
#67641=ORIENTED_EDGE('',*,*,#51179,.T.);
#67642=ORIENTED_EDGE('',*,*,#51180,.F.);
#67643=ORIENTED_EDGE('',*,*,#51175,.F.);
#67644=ORIENTED_EDGE('',*,*,#51181,.T.);
#67645=ORIENTED_EDGE('',*,*,#51182,.T.);
#67646=ORIENTED_EDGE('',*,*,#51183,.F.);
#67647=ORIENTED_EDGE('',*,*,#51179,.F.);
#67648=ORIENTED_EDGE('',*,*,#51184,.T.);
#67649=ORIENTED_EDGE('',*,*,#51177,.T.);
#67650=ORIENTED_EDGE('',*,*,#51185,.F.);
#67651=ORIENTED_EDGE('',*,*,#51182,.F.);
#67652=ORIENTED_EDGE('',*,*,#51186,.T.);
#67653=ORIENTED_EDGE('',*,*,#51187,.T.);
#67654=ORIENTED_EDGE('',*,*,#51188,.F.);
#67655=ORIENTED_EDGE('',*,*,#51189,.F.);
#67656=ORIENTED_EDGE('',*,*,#51190,.T.);
#67657=ORIENTED_EDGE('',*,*,#51191,.T.);
#67658=ORIENTED_EDGE('',*,*,#51192,.F.);
#67659=ORIENTED_EDGE('',*,*,#51187,.F.);
#67660=ORIENTED_EDGE('',*,*,#51193,.T.);
#67661=ORIENTED_EDGE('',*,*,#51194,.T.);
#67662=ORIENTED_EDGE('',*,*,#51195,.F.);
#67663=ORIENTED_EDGE('',*,*,#51191,.F.);
#67664=ORIENTED_EDGE('',*,*,#51196,.T.);
#67665=ORIENTED_EDGE('',*,*,#51189,.T.);
#67666=ORIENTED_EDGE('',*,*,#51197,.F.);
#67667=ORIENTED_EDGE('',*,*,#51194,.F.);
#67668=ORIENTED_EDGE('',*,*,#51198,.T.);
#67669=ORIENTED_EDGE('',*,*,#51199,.T.);
#67670=ORIENTED_EDGE('',*,*,#51200,.F.);
#67671=ORIENTED_EDGE('',*,*,#51201,.F.);
#67672=ORIENTED_EDGE('',*,*,#51202,.T.);
#67673=ORIENTED_EDGE('',*,*,#51203,.T.);
#67674=ORIENTED_EDGE('',*,*,#51204,.F.);
#67675=ORIENTED_EDGE('',*,*,#51199,.F.);
#67676=ORIENTED_EDGE('',*,*,#51205,.T.);
#67677=ORIENTED_EDGE('',*,*,#51206,.T.);
#67678=ORIENTED_EDGE('',*,*,#51207,.F.);
#67679=ORIENTED_EDGE('',*,*,#51203,.F.);
#67680=ORIENTED_EDGE('',*,*,#51208,.T.);
#67681=ORIENTED_EDGE('',*,*,#51201,.T.);
#67682=ORIENTED_EDGE('',*,*,#51209,.F.);
#67683=ORIENTED_EDGE('',*,*,#51206,.F.);
#67684=ORIENTED_EDGE('',*,*,#51210,.T.);
#67685=ORIENTED_EDGE('',*,*,#51211,.T.);
#67686=ORIENTED_EDGE('',*,*,#51212,.F.);
#67687=ORIENTED_EDGE('',*,*,#51213,.F.);
#67688=ORIENTED_EDGE('',*,*,#51214,.T.);
#67689=ORIENTED_EDGE('',*,*,#51215,.T.);
#67690=ORIENTED_EDGE('',*,*,#51216,.F.);
#67691=ORIENTED_EDGE('',*,*,#51211,.F.);
#67692=ORIENTED_EDGE('',*,*,#51217,.T.);
#67693=ORIENTED_EDGE('',*,*,#51218,.T.);
#67694=ORIENTED_EDGE('',*,*,#51219,.F.);
#67695=ORIENTED_EDGE('',*,*,#51215,.F.);
#67696=ORIENTED_EDGE('',*,*,#51220,.T.);
#67697=ORIENTED_EDGE('',*,*,#51213,.T.);
#67698=ORIENTED_EDGE('',*,*,#51221,.F.);
#67699=ORIENTED_EDGE('',*,*,#51218,.F.);
#67700=ORIENTED_EDGE('',*,*,#51222,.T.);
#67701=ORIENTED_EDGE('',*,*,#51223,.T.);
#67702=ORIENTED_EDGE('',*,*,#51224,.F.);
#67703=ORIENTED_EDGE('',*,*,#51225,.F.);
#67704=ORIENTED_EDGE('',*,*,#51226,.T.);
#67705=ORIENTED_EDGE('',*,*,#51227,.T.);
#67706=ORIENTED_EDGE('',*,*,#51228,.F.);
#67707=ORIENTED_EDGE('',*,*,#51223,.F.);
#67708=ORIENTED_EDGE('',*,*,#51229,.T.);
#67709=ORIENTED_EDGE('',*,*,#51230,.T.);
#67710=ORIENTED_EDGE('',*,*,#51231,.F.);
#67711=ORIENTED_EDGE('',*,*,#51227,.F.);
#67712=ORIENTED_EDGE('',*,*,#51232,.T.);
#67713=ORIENTED_EDGE('',*,*,#51225,.T.);
#67714=ORIENTED_EDGE('',*,*,#51233,.F.);
#67715=ORIENTED_EDGE('',*,*,#51230,.F.);
#67716=ORIENTED_EDGE('',*,*,#51234,.T.);
#67717=ORIENTED_EDGE('',*,*,#51235,.T.);
#67718=ORIENTED_EDGE('',*,*,#51236,.F.);
#67719=ORIENTED_EDGE('',*,*,#51237,.F.);
#67720=ORIENTED_EDGE('',*,*,#51238,.T.);
#67721=ORIENTED_EDGE('',*,*,#51239,.T.);
#67722=ORIENTED_EDGE('',*,*,#51240,.F.);
#67723=ORIENTED_EDGE('',*,*,#51235,.F.);
#67724=ORIENTED_EDGE('',*,*,#51241,.T.);
#67725=ORIENTED_EDGE('',*,*,#51242,.T.);
#67726=ORIENTED_EDGE('',*,*,#51243,.F.);
#67727=ORIENTED_EDGE('',*,*,#51239,.F.);
#67728=ORIENTED_EDGE('',*,*,#51244,.T.);
#67729=ORIENTED_EDGE('',*,*,#51237,.T.);
#67730=ORIENTED_EDGE('',*,*,#51245,.F.);
#67731=ORIENTED_EDGE('',*,*,#51242,.F.);
#67732=ORIENTED_EDGE('',*,*,#51246,.T.);
#67733=ORIENTED_EDGE('',*,*,#51247,.T.);
#67734=ORIENTED_EDGE('',*,*,#51248,.F.);
#67735=ORIENTED_EDGE('',*,*,#51249,.F.);
#67736=ORIENTED_EDGE('',*,*,#51250,.T.);
#67737=ORIENTED_EDGE('',*,*,#51251,.T.);
#67738=ORIENTED_EDGE('',*,*,#51252,.F.);
#67739=ORIENTED_EDGE('',*,*,#51247,.F.);
#67740=ORIENTED_EDGE('',*,*,#51253,.T.);
#67741=ORIENTED_EDGE('',*,*,#51254,.T.);
#67742=ORIENTED_EDGE('',*,*,#51255,.F.);
#67743=ORIENTED_EDGE('',*,*,#51251,.F.);
#67744=ORIENTED_EDGE('',*,*,#51256,.T.);
#67745=ORIENTED_EDGE('',*,*,#51249,.T.);
#67746=ORIENTED_EDGE('',*,*,#51257,.F.);
#67747=ORIENTED_EDGE('',*,*,#51254,.F.);
#67748=ORIENTED_EDGE('',*,*,#51258,.T.);
#67749=ORIENTED_EDGE('',*,*,#51259,.T.);
#67750=ORIENTED_EDGE('',*,*,#51260,.F.);
#67751=ORIENTED_EDGE('',*,*,#51261,.F.);
#67752=ORIENTED_EDGE('',*,*,#51262,.T.);
#67753=ORIENTED_EDGE('',*,*,#51263,.T.);
#67754=ORIENTED_EDGE('',*,*,#51264,.F.);
#67755=ORIENTED_EDGE('',*,*,#51259,.F.);
#67756=ORIENTED_EDGE('',*,*,#51265,.T.);
#67757=ORIENTED_EDGE('',*,*,#51266,.T.);
#67758=ORIENTED_EDGE('',*,*,#51267,.F.);
#67759=ORIENTED_EDGE('',*,*,#51263,.F.);
#67760=ORIENTED_EDGE('',*,*,#51268,.T.);
#67761=ORIENTED_EDGE('',*,*,#51261,.T.);
#67762=ORIENTED_EDGE('',*,*,#51269,.F.);
#67763=ORIENTED_EDGE('',*,*,#51266,.F.);
#67764=ORIENTED_EDGE('',*,*,#51270,.T.);
#67765=ORIENTED_EDGE('',*,*,#51271,.T.);
#67766=ORIENTED_EDGE('',*,*,#51272,.F.);
#67767=ORIENTED_EDGE('',*,*,#51273,.F.);
#67768=ORIENTED_EDGE('',*,*,#51274,.T.);
#67769=ORIENTED_EDGE('',*,*,#51275,.T.);
#67770=ORIENTED_EDGE('',*,*,#51276,.F.);
#67771=ORIENTED_EDGE('',*,*,#51271,.F.);
#67772=ORIENTED_EDGE('',*,*,#51277,.T.);
#67773=ORIENTED_EDGE('',*,*,#51278,.T.);
#67774=ORIENTED_EDGE('',*,*,#51279,.F.);
#67775=ORIENTED_EDGE('',*,*,#51275,.F.);
#67776=ORIENTED_EDGE('',*,*,#51280,.T.);
#67777=ORIENTED_EDGE('',*,*,#51273,.T.);
#67778=ORIENTED_EDGE('',*,*,#51281,.F.);
#67779=ORIENTED_EDGE('',*,*,#51278,.F.);
#67780=ORIENTED_EDGE('',*,*,#51282,.T.);
#67781=ORIENTED_EDGE('',*,*,#51283,.T.);
#67782=ORIENTED_EDGE('',*,*,#51284,.F.);
#67783=ORIENTED_EDGE('',*,*,#51285,.F.);
#67784=ORIENTED_EDGE('',*,*,#51286,.T.);
#67785=ORIENTED_EDGE('',*,*,#51287,.T.);
#67786=ORIENTED_EDGE('',*,*,#51288,.F.);
#67787=ORIENTED_EDGE('',*,*,#51283,.F.);
#67788=ORIENTED_EDGE('',*,*,#51289,.T.);
#67789=ORIENTED_EDGE('',*,*,#51290,.T.);
#67790=ORIENTED_EDGE('',*,*,#51291,.F.);
#67791=ORIENTED_EDGE('',*,*,#51287,.F.);
#67792=ORIENTED_EDGE('',*,*,#51292,.T.);
#67793=ORIENTED_EDGE('',*,*,#51285,.T.);
#67794=ORIENTED_EDGE('',*,*,#51293,.F.);
#67795=ORIENTED_EDGE('',*,*,#51290,.F.);
#67796=ORIENTED_EDGE('',*,*,#51294,.T.);
#67797=ORIENTED_EDGE('',*,*,#51295,.T.);
#67798=ORIENTED_EDGE('',*,*,#51296,.F.);
#67799=ORIENTED_EDGE('',*,*,#51297,.F.);
#67800=ORIENTED_EDGE('',*,*,#51298,.T.);
#67801=ORIENTED_EDGE('',*,*,#51299,.T.);
#67802=ORIENTED_EDGE('',*,*,#51300,.F.);
#67803=ORIENTED_EDGE('',*,*,#51295,.F.);
#67804=ORIENTED_EDGE('',*,*,#51301,.T.);
#67805=ORIENTED_EDGE('',*,*,#51302,.T.);
#67806=ORIENTED_EDGE('',*,*,#51303,.F.);
#67807=ORIENTED_EDGE('',*,*,#51299,.F.);
#67808=ORIENTED_EDGE('',*,*,#51304,.T.);
#67809=ORIENTED_EDGE('',*,*,#51297,.T.);
#67810=ORIENTED_EDGE('',*,*,#51305,.F.);
#67811=ORIENTED_EDGE('',*,*,#51302,.F.);
#67812=ORIENTED_EDGE('',*,*,#51306,.T.);
#67813=ORIENTED_EDGE('',*,*,#51307,.T.);
#67814=ORIENTED_EDGE('',*,*,#51308,.F.);
#67815=ORIENTED_EDGE('',*,*,#51309,.F.);
#67816=ORIENTED_EDGE('',*,*,#51310,.T.);
#67817=ORIENTED_EDGE('',*,*,#51311,.T.);
#67818=ORIENTED_EDGE('',*,*,#51312,.F.);
#67819=ORIENTED_EDGE('',*,*,#51307,.F.);
#67820=ORIENTED_EDGE('',*,*,#51313,.T.);
#67821=ORIENTED_EDGE('',*,*,#51314,.T.);
#67822=ORIENTED_EDGE('',*,*,#51315,.F.);
#67823=ORIENTED_EDGE('',*,*,#51311,.F.);
#67824=ORIENTED_EDGE('',*,*,#51316,.T.);
#67825=ORIENTED_EDGE('',*,*,#51309,.T.);
#67826=ORIENTED_EDGE('',*,*,#51317,.F.);
#67827=ORIENTED_EDGE('',*,*,#51314,.F.);
#67828=ORIENTED_EDGE('',*,*,#51318,.T.);
#67829=ORIENTED_EDGE('',*,*,#51319,.T.);
#67830=ORIENTED_EDGE('',*,*,#51320,.F.);
#67831=ORIENTED_EDGE('',*,*,#51321,.F.);
#67832=ORIENTED_EDGE('',*,*,#51322,.T.);
#67833=ORIENTED_EDGE('',*,*,#51323,.T.);
#67834=ORIENTED_EDGE('',*,*,#51324,.F.);
#67835=ORIENTED_EDGE('',*,*,#51319,.F.);
#67836=ORIENTED_EDGE('',*,*,#51325,.T.);
#67837=ORIENTED_EDGE('',*,*,#51326,.T.);
#67838=ORIENTED_EDGE('',*,*,#51327,.F.);
#67839=ORIENTED_EDGE('',*,*,#51323,.F.);
#67840=ORIENTED_EDGE('',*,*,#51328,.T.);
#67841=ORIENTED_EDGE('',*,*,#51321,.T.);
#67842=ORIENTED_EDGE('',*,*,#51329,.F.);
#67843=ORIENTED_EDGE('',*,*,#51326,.F.);
#67844=ORIENTED_EDGE('',*,*,#51330,.T.);
#67845=ORIENTED_EDGE('',*,*,#51331,.T.);
#67846=ORIENTED_EDGE('',*,*,#51332,.F.);
#67847=ORIENTED_EDGE('',*,*,#51333,.F.);
#67848=ORIENTED_EDGE('',*,*,#51334,.T.);
#67849=ORIENTED_EDGE('',*,*,#51335,.T.);
#67850=ORIENTED_EDGE('',*,*,#51336,.F.);
#67851=ORIENTED_EDGE('',*,*,#51331,.F.);
#67852=ORIENTED_EDGE('',*,*,#51337,.T.);
#67853=ORIENTED_EDGE('',*,*,#51338,.T.);
#67854=ORIENTED_EDGE('',*,*,#51339,.F.);
#67855=ORIENTED_EDGE('',*,*,#51335,.F.);
#67856=ORIENTED_EDGE('',*,*,#51340,.T.);
#67857=ORIENTED_EDGE('',*,*,#51333,.T.);
#67858=ORIENTED_EDGE('',*,*,#51341,.F.);
#67859=ORIENTED_EDGE('',*,*,#51338,.F.);
#67860=ORIENTED_EDGE('',*,*,#51342,.T.);
#67861=ORIENTED_EDGE('',*,*,#51343,.T.);
#67862=ORIENTED_EDGE('',*,*,#51344,.F.);
#67863=ORIENTED_EDGE('',*,*,#51345,.F.);
#67864=ORIENTED_EDGE('',*,*,#51346,.T.);
#67865=ORIENTED_EDGE('',*,*,#51347,.T.);
#67866=ORIENTED_EDGE('',*,*,#51348,.F.);
#67867=ORIENTED_EDGE('',*,*,#51343,.F.);
#67868=ORIENTED_EDGE('',*,*,#51349,.T.);
#67869=ORIENTED_EDGE('',*,*,#51350,.T.);
#67870=ORIENTED_EDGE('',*,*,#51351,.F.);
#67871=ORIENTED_EDGE('',*,*,#51347,.F.);
#67872=ORIENTED_EDGE('',*,*,#51352,.T.);
#67873=ORIENTED_EDGE('',*,*,#51345,.T.);
#67874=ORIENTED_EDGE('',*,*,#51353,.F.);
#67875=ORIENTED_EDGE('',*,*,#51350,.F.);
#67876=ORIENTED_EDGE('',*,*,#51354,.T.);
#67877=ORIENTED_EDGE('',*,*,#51355,.T.);
#67878=ORIENTED_EDGE('',*,*,#51356,.F.);
#67879=ORIENTED_EDGE('',*,*,#51357,.F.);
#67880=ORIENTED_EDGE('',*,*,#51358,.T.);
#67881=ORIENTED_EDGE('',*,*,#51359,.T.);
#67882=ORIENTED_EDGE('',*,*,#51360,.F.);
#67883=ORIENTED_EDGE('',*,*,#51355,.F.);
#67884=ORIENTED_EDGE('',*,*,#51361,.T.);
#67885=ORIENTED_EDGE('',*,*,#51362,.T.);
#67886=ORIENTED_EDGE('',*,*,#51363,.F.);
#67887=ORIENTED_EDGE('',*,*,#51359,.F.);
#67888=ORIENTED_EDGE('',*,*,#51364,.T.);
#67889=ORIENTED_EDGE('',*,*,#51357,.T.);
#67890=ORIENTED_EDGE('',*,*,#51365,.F.);
#67891=ORIENTED_EDGE('',*,*,#51362,.F.);
#67892=ORIENTED_EDGE('',*,*,#51366,.T.);
#67893=ORIENTED_EDGE('',*,*,#51367,.T.);
#67894=ORIENTED_EDGE('',*,*,#51368,.F.);
#67895=ORIENTED_EDGE('',*,*,#51369,.F.);
#67896=ORIENTED_EDGE('',*,*,#51370,.T.);
#67897=ORIENTED_EDGE('',*,*,#51371,.T.);
#67898=ORIENTED_EDGE('',*,*,#51372,.F.);
#67899=ORIENTED_EDGE('',*,*,#51367,.F.);
#67900=ORIENTED_EDGE('',*,*,#51373,.T.);
#67901=ORIENTED_EDGE('',*,*,#51374,.T.);
#67902=ORIENTED_EDGE('',*,*,#51375,.F.);
#67903=ORIENTED_EDGE('',*,*,#51371,.F.);
#67904=ORIENTED_EDGE('',*,*,#51376,.T.);
#67905=ORIENTED_EDGE('',*,*,#51369,.T.);
#67906=ORIENTED_EDGE('',*,*,#51377,.F.);
#67907=ORIENTED_EDGE('',*,*,#51374,.F.);
#67908=ORIENTED_EDGE('',*,*,#51378,.T.);
#67909=ORIENTED_EDGE('',*,*,#51379,.T.);
#67910=ORIENTED_EDGE('',*,*,#51380,.F.);
#67911=ORIENTED_EDGE('',*,*,#51381,.F.);
#67912=ORIENTED_EDGE('',*,*,#51382,.T.);
#67913=ORIENTED_EDGE('',*,*,#51383,.T.);
#67914=ORIENTED_EDGE('',*,*,#51384,.F.);
#67915=ORIENTED_EDGE('',*,*,#51379,.F.);
#67916=ORIENTED_EDGE('',*,*,#51385,.T.);
#67917=ORIENTED_EDGE('',*,*,#51386,.T.);
#67918=ORIENTED_EDGE('',*,*,#51387,.F.);
#67919=ORIENTED_EDGE('',*,*,#51383,.F.);
#67920=ORIENTED_EDGE('',*,*,#51388,.T.);
#67921=ORIENTED_EDGE('',*,*,#51381,.T.);
#67922=ORIENTED_EDGE('',*,*,#51389,.F.);
#67923=ORIENTED_EDGE('',*,*,#51386,.F.);
#67924=ORIENTED_EDGE('',*,*,#51390,.T.);
#67925=ORIENTED_EDGE('',*,*,#51391,.T.);
#67926=ORIENTED_EDGE('',*,*,#51392,.F.);
#67927=ORIENTED_EDGE('',*,*,#51393,.F.);
#67928=ORIENTED_EDGE('',*,*,#51394,.T.);
#67929=ORIENTED_EDGE('',*,*,#51395,.T.);
#67930=ORIENTED_EDGE('',*,*,#51396,.F.);
#67931=ORIENTED_EDGE('',*,*,#51391,.F.);
#67932=ORIENTED_EDGE('',*,*,#51397,.T.);
#67933=ORIENTED_EDGE('',*,*,#51398,.T.);
#67934=ORIENTED_EDGE('',*,*,#51399,.F.);
#67935=ORIENTED_EDGE('',*,*,#51395,.F.);
#67936=ORIENTED_EDGE('',*,*,#51400,.T.);
#67937=ORIENTED_EDGE('',*,*,#51393,.T.);
#67938=ORIENTED_EDGE('',*,*,#51401,.F.);
#67939=ORIENTED_EDGE('',*,*,#51398,.F.);
#67940=ORIENTED_EDGE('',*,*,#51402,.T.);
#67941=ORIENTED_EDGE('',*,*,#51403,.T.);
#67942=ORIENTED_EDGE('',*,*,#51404,.F.);
#67943=ORIENTED_EDGE('',*,*,#51405,.F.);
#67944=ORIENTED_EDGE('',*,*,#51406,.T.);
#67945=ORIENTED_EDGE('',*,*,#51407,.T.);
#67946=ORIENTED_EDGE('',*,*,#51408,.F.);
#67947=ORIENTED_EDGE('',*,*,#51403,.F.);
#67948=ORIENTED_EDGE('',*,*,#51409,.T.);
#67949=ORIENTED_EDGE('',*,*,#51410,.T.);
#67950=ORIENTED_EDGE('',*,*,#51411,.F.);
#67951=ORIENTED_EDGE('',*,*,#51407,.F.);
#67952=ORIENTED_EDGE('',*,*,#51412,.T.);
#67953=ORIENTED_EDGE('',*,*,#51405,.T.);
#67954=ORIENTED_EDGE('',*,*,#51413,.F.);
#67955=ORIENTED_EDGE('',*,*,#51410,.F.);
#67956=ORIENTED_EDGE('',*,*,#51414,.T.);
#67957=ORIENTED_EDGE('',*,*,#51415,.T.);
#67958=ORIENTED_EDGE('',*,*,#51416,.F.);
#67959=ORIENTED_EDGE('',*,*,#51417,.F.);
#67960=ORIENTED_EDGE('',*,*,#51418,.T.);
#67961=ORIENTED_EDGE('',*,*,#51419,.T.);
#67962=ORIENTED_EDGE('',*,*,#51420,.F.);
#67963=ORIENTED_EDGE('',*,*,#51415,.F.);
#67964=ORIENTED_EDGE('',*,*,#51421,.T.);
#67965=ORIENTED_EDGE('',*,*,#51422,.T.);
#67966=ORIENTED_EDGE('',*,*,#51423,.F.);
#67967=ORIENTED_EDGE('',*,*,#51419,.F.);
#67968=ORIENTED_EDGE('',*,*,#51424,.T.);
#67969=ORIENTED_EDGE('',*,*,#51417,.T.);
#67970=ORIENTED_EDGE('',*,*,#51425,.F.);
#67971=ORIENTED_EDGE('',*,*,#51422,.F.);
#67972=ORIENTED_EDGE('',*,*,#51426,.T.);
#67973=ORIENTED_EDGE('',*,*,#51427,.T.);
#67974=ORIENTED_EDGE('',*,*,#51428,.F.);
#67975=ORIENTED_EDGE('',*,*,#51429,.F.);
#67976=ORIENTED_EDGE('',*,*,#51430,.T.);
#67977=ORIENTED_EDGE('',*,*,#51431,.T.);
#67978=ORIENTED_EDGE('',*,*,#51432,.F.);
#67979=ORIENTED_EDGE('',*,*,#51427,.F.);
#67980=ORIENTED_EDGE('',*,*,#51433,.T.);
#67981=ORIENTED_EDGE('',*,*,#51434,.T.);
#67982=ORIENTED_EDGE('',*,*,#51435,.F.);
#67983=ORIENTED_EDGE('',*,*,#51431,.F.);
#67984=ORIENTED_EDGE('',*,*,#51436,.T.);
#67985=ORIENTED_EDGE('',*,*,#51429,.T.);
#67986=ORIENTED_EDGE('',*,*,#51437,.F.);
#67987=ORIENTED_EDGE('',*,*,#51434,.F.);
#67988=ORIENTED_EDGE('',*,*,#51438,.T.);
#67989=ORIENTED_EDGE('',*,*,#51439,.T.);
#67990=ORIENTED_EDGE('',*,*,#51440,.F.);
#67991=ORIENTED_EDGE('',*,*,#51441,.F.);
#67992=ORIENTED_EDGE('',*,*,#51442,.T.);
#67993=ORIENTED_EDGE('',*,*,#51443,.T.);
#67994=ORIENTED_EDGE('',*,*,#51444,.F.);
#67995=ORIENTED_EDGE('',*,*,#51439,.F.);
#67996=ORIENTED_EDGE('',*,*,#51445,.T.);
#67997=ORIENTED_EDGE('',*,*,#51446,.T.);
#67998=ORIENTED_EDGE('',*,*,#51447,.F.);
#67999=ORIENTED_EDGE('',*,*,#51443,.F.);
#68000=ORIENTED_EDGE('',*,*,#51448,.T.);
#68001=ORIENTED_EDGE('',*,*,#51441,.T.);
#68002=ORIENTED_EDGE('',*,*,#51449,.F.);
#68003=ORIENTED_EDGE('',*,*,#51446,.F.);
#68004=ORIENTED_EDGE('',*,*,#51450,.T.);
#68005=ORIENTED_EDGE('',*,*,#51451,.T.);
#68006=ORIENTED_EDGE('',*,*,#51452,.F.);
#68007=ORIENTED_EDGE('',*,*,#51453,.F.);
#68008=ORIENTED_EDGE('',*,*,#51454,.T.);
#68009=ORIENTED_EDGE('',*,*,#51455,.T.);
#68010=ORIENTED_EDGE('',*,*,#51456,.F.);
#68011=ORIENTED_EDGE('',*,*,#51451,.F.);
#68012=ORIENTED_EDGE('',*,*,#51457,.T.);
#68013=ORIENTED_EDGE('',*,*,#51458,.T.);
#68014=ORIENTED_EDGE('',*,*,#51459,.F.);
#68015=ORIENTED_EDGE('',*,*,#51455,.F.);
#68016=ORIENTED_EDGE('',*,*,#51460,.T.);
#68017=ORIENTED_EDGE('',*,*,#51453,.T.);
#68018=ORIENTED_EDGE('',*,*,#51461,.F.);
#68019=ORIENTED_EDGE('',*,*,#51458,.F.);
#68020=ORIENTED_EDGE('',*,*,#51462,.T.);
#68021=ORIENTED_EDGE('',*,*,#51463,.T.);
#68022=ORIENTED_EDGE('',*,*,#51464,.F.);
#68023=ORIENTED_EDGE('',*,*,#51465,.F.);
#68024=ORIENTED_EDGE('',*,*,#51466,.T.);
#68025=ORIENTED_EDGE('',*,*,#51467,.T.);
#68026=ORIENTED_EDGE('',*,*,#51468,.F.);
#68027=ORIENTED_EDGE('',*,*,#51463,.F.);
#68028=ORIENTED_EDGE('',*,*,#51469,.T.);
#68029=ORIENTED_EDGE('',*,*,#51470,.T.);
#68030=ORIENTED_EDGE('',*,*,#51471,.F.);
#68031=ORIENTED_EDGE('',*,*,#51467,.F.);
#68032=ORIENTED_EDGE('',*,*,#51472,.T.);
#68033=ORIENTED_EDGE('',*,*,#51465,.T.);
#68034=ORIENTED_EDGE('',*,*,#51473,.F.);
#68035=ORIENTED_EDGE('',*,*,#51470,.F.);
#68036=ORIENTED_EDGE('',*,*,#51474,.T.);
#68037=ORIENTED_EDGE('',*,*,#51475,.T.);
#68038=ORIENTED_EDGE('',*,*,#51476,.F.);
#68039=ORIENTED_EDGE('',*,*,#51477,.F.);
#68040=ORIENTED_EDGE('',*,*,#51478,.T.);
#68041=ORIENTED_EDGE('',*,*,#51479,.T.);
#68042=ORIENTED_EDGE('',*,*,#51480,.F.);
#68043=ORIENTED_EDGE('',*,*,#51475,.F.);
#68044=ORIENTED_EDGE('',*,*,#51481,.T.);
#68045=ORIENTED_EDGE('',*,*,#51482,.T.);
#68046=ORIENTED_EDGE('',*,*,#51483,.F.);
#68047=ORIENTED_EDGE('',*,*,#51479,.F.);
#68048=ORIENTED_EDGE('',*,*,#51484,.T.);
#68049=ORIENTED_EDGE('',*,*,#51477,.T.);
#68050=ORIENTED_EDGE('',*,*,#51485,.F.);
#68051=ORIENTED_EDGE('',*,*,#51482,.F.);
#68052=ORIENTED_EDGE('',*,*,#51486,.T.);
#68053=ORIENTED_EDGE('',*,*,#51487,.T.);
#68054=ORIENTED_EDGE('',*,*,#51488,.F.);
#68055=ORIENTED_EDGE('',*,*,#51489,.F.);
#68056=ORIENTED_EDGE('',*,*,#51490,.T.);
#68057=ORIENTED_EDGE('',*,*,#51491,.T.);
#68058=ORIENTED_EDGE('',*,*,#51492,.F.);
#68059=ORIENTED_EDGE('',*,*,#51487,.F.);
#68060=ORIENTED_EDGE('',*,*,#51493,.T.);
#68061=ORIENTED_EDGE('',*,*,#51494,.T.);
#68062=ORIENTED_EDGE('',*,*,#51495,.F.);
#68063=ORIENTED_EDGE('',*,*,#51491,.F.);
#68064=ORIENTED_EDGE('',*,*,#51496,.T.);
#68065=ORIENTED_EDGE('',*,*,#51489,.T.);
#68066=ORIENTED_EDGE('',*,*,#51497,.F.);
#68067=ORIENTED_EDGE('',*,*,#51494,.F.);
#68068=ORIENTED_EDGE('',*,*,#51498,.T.);
#68069=ORIENTED_EDGE('',*,*,#51499,.T.);
#68070=ORIENTED_EDGE('',*,*,#51500,.F.);
#68071=ORIENTED_EDGE('',*,*,#51501,.F.);
#68072=ORIENTED_EDGE('',*,*,#51502,.T.);
#68073=ORIENTED_EDGE('',*,*,#51503,.T.);
#68074=ORIENTED_EDGE('',*,*,#51504,.F.);
#68075=ORIENTED_EDGE('',*,*,#51499,.F.);
#68076=ORIENTED_EDGE('',*,*,#51505,.T.);
#68077=ORIENTED_EDGE('',*,*,#51506,.T.);
#68078=ORIENTED_EDGE('',*,*,#51507,.F.);
#68079=ORIENTED_EDGE('',*,*,#51503,.F.);
#68080=ORIENTED_EDGE('',*,*,#51508,.T.);
#68081=ORIENTED_EDGE('',*,*,#51501,.T.);
#68082=ORIENTED_EDGE('',*,*,#51509,.F.);
#68083=ORIENTED_EDGE('',*,*,#51506,.F.);
#68084=ORIENTED_EDGE('',*,*,#51510,.T.);
#68085=ORIENTED_EDGE('',*,*,#51511,.T.);
#68086=ORIENTED_EDGE('',*,*,#51512,.F.);
#68087=ORIENTED_EDGE('',*,*,#51513,.F.);
#68088=ORIENTED_EDGE('',*,*,#51514,.T.);
#68089=ORIENTED_EDGE('',*,*,#51515,.T.);
#68090=ORIENTED_EDGE('',*,*,#51516,.F.);
#68091=ORIENTED_EDGE('',*,*,#51511,.F.);
#68092=ORIENTED_EDGE('',*,*,#51517,.T.);
#68093=ORIENTED_EDGE('',*,*,#51518,.T.);
#68094=ORIENTED_EDGE('',*,*,#51519,.F.);
#68095=ORIENTED_EDGE('',*,*,#51515,.F.);
#68096=ORIENTED_EDGE('',*,*,#51520,.T.);
#68097=ORIENTED_EDGE('',*,*,#51513,.T.);
#68098=ORIENTED_EDGE('',*,*,#51521,.F.);
#68099=ORIENTED_EDGE('',*,*,#51518,.F.);
#68100=ORIENTED_EDGE('',*,*,#51522,.T.);
#68101=ORIENTED_EDGE('',*,*,#51523,.T.);
#68102=ORIENTED_EDGE('',*,*,#51524,.F.);
#68103=ORIENTED_EDGE('',*,*,#51525,.F.);
#68104=ORIENTED_EDGE('',*,*,#51526,.T.);
#68105=ORIENTED_EDGE('',*,*,#51527,.T.);
#68106=ORIENTED_EDGE('',*,*,#51528,.F.);
#68107=ORIENTED_EDGE('',*,*,#51523,.F.);
#68108=ORIENTED_EDGE('',*,*,#51529,.T.);
#68109=ORIENTED_EDGE('',*,*,#51530,.T.);
#68110=ORIENTED_EDGE('',*,*,#51531,.F.);
#68111=ORIENTED_EDGE('',*,*,#51527,.F.);
#68112=ORIENTED_EDGE('',*,*,#51532,.T.);
#68113=ORIENTED_EDGE('',*,*,#51525,.T.);
#68114=ORIENTED_EDGE('',*,*,#51533,.F.);
#68115=ORIENTED_EDGE('',*,*,#51530,.F.);
#68116=ORIENTED_EDGE('',*,*,#51534,.T.);
#68117=ORIENTED_EDGE('',*,*,#51535,.T.);
#68118=ORIENTED_EDGE('',*,*,#51536,.F.);
#68119=ORIENTED_EDGE('',*,*,#51537,.F.);
#68120=ORIENTED_EDGE('',*,*,#51538,.T.);
#68121=ORIENTED_EDGE('',*,*,#51539,.T.);
#68122=ORIENTED_EDGE('',*,*,#51540,.F.);
#68123=ORIENTED_EDGE('',*,*,#51535,.F.);
#68124=ORIENTED_EDGE('',*,*,#51541,.T.);
#68125=ORIENTED_EDGE('',*,*,#51542,.T.);
#68126=ORIENTED_EDGE('',*,*,#51543,.F.);
#68127=ORIENTED_EDGE('',*,*,#51539,.F.);
#68128=ORIENTED_EDGE('',*,*,#51544,.T.);
#68129=ORIENTED_EDGE('',*,*,#51537,.T.);
#68130=ORIENTED_EDGE('',*,*,#51545,.F.);
#68131=ORIENTED_EDGE('',*,*,#51542,.F.);
#68132=ORIENTED_EDGE('',*,*,#51546,.T.);
#68133=ORIENTED_EDGE('',*,*,#51547,.T.);
#68134=ORIENTED_EDGE('',*,*,#51548,.F.);
#68135=ORIENTED_EDGE('',*,*,#51549,.F.);
#68136=ORIENTED_EDGE('',*,*,#51550,.T.);
#68137=ORIENTED_EDGE('',*,*,#51551,.T.);
#68138=ORIENTED_EDGE('',*,*,#51552,.F.);
#68139=ORIENTED_EDGE('',*,*,#51547,.F.);
#68140=ORIENTED_EDGE('',*,*,#51553,.T.);
#68141=ORIENTED_EDGE('',*,*,#51554,.T.);
#68142=ORIENTED_EDGE('',*,*,#51555,.F.);
#68143=ORIENTED_EDGE('',*,*,#51551,.F.);
#68144=ORIENTED_EDGE('',*,*,#51556,.T.);
#68145=ORIENTED_EDGE('',*,*,#51549,.T.);
#68146=ORIENTED_EDGE('',*,*,#51557,.F.);
#68147=ORIENTED_EDGE('',*,*,#51554,.F.);
#68148=ORIENTED_EDGE('',*,*,#51558,.T.);
#68149=ORIENTED_EDGE('',*,*,#51559,.T.);
#68150=ORIENTED_EDGE('',*,*,#51560,.F.);
#68151=ORIENTED_EDGE('',*,*,#51561,.F.);
#68152=ORIENTED_EDGE('',*,*,#51562,.T.);
#68153=ORIENTED_EDGE('',*,*,#51563,.T.);
#68154=ORIENTED_EDGE('',*,*,#51564,.F.);
#68155=ORIENTED_EDGE('',*,*,#51559,.F.);
#68156=ORIENTED_EDGE('',*,*,#51565,.T.);
#68157=ORIENTED_EDGE('',*,*,#51566,.T.);
#68158=ORIENTED_EDGE('',*,*,#51567,.F.);
#68159=ORIENTED_EDGE('',*,*,#51563,.F.);
#68160=ORIENTED_EDGE('',*,*,#51568,.T.);
#68161=ORIENTED_EDGE('',*,*,#51561,.T.);
#68162=ORIENTED_EDGE('',*,*,#51569,.F.);
#68163=ORIENTED_EDGE('',*,*,#51566,.F.);
#68164=ORIENTED_EDGE('',*,*,#51570,.T.);
#68165=ORIENTED_EDGE('',*,*,#51571,.T.);
#68166=ORIENTED_EDGE('',*,*,#51572,.F.);
#68167=ORIENTED_EDGE('',*,*,#51573,.F.);
#68168=ORIENTED_EDGE('',*,*,#51574,.T.);
#68169=ORIENTED_EDGE('',*,*,#51575,.T.);
#68170=ORIENTED_EDGE('',*,*,#51576,.F.);
#68171=ORIENTED_EDGE('',*,*,#51571,.F.);
#68172=ORIENTED_EDGE('',*,*,#51577,.T.);
#68173=ORIENTED_EDGE('',*,*,#51578,.T.);
#68174=ORIENTED_EDGE('',*,*,#51579,.F.);
#68175=ORIENTED_EDGE('',*,*,#51575,.F.);
#68176=ORIENTED_EDGE('',*,*,#51580,.T.);
#68177=ORIENTED_EDGE('',*,*,#51573,.T.);
#68178=ORIENTED_EDGE('',*,*,#51581,.F.);
#68179=ORIENTED_EDGE('',*,*,#51578,.F.);
#68180=ORIENTED_EDGE('',*,*,#51582,.T.);
#68181=ORIENTED_EDGE('',*,*,#51583,.T.);
#68182=ORIENTED_EDGE('',*,*,#51584,.F.);
#68183=ORIENTED_EDGE('',*,*,#51585,.F.);
#68184=ORIENTED_EDGE('',*,*,#51586,.T.);
#68185=ORIENTED_EDGE('',*,*,#51587,.T.);
#68186=ORIENTED_EDGE('',*,*,#51588,.F.);
#68187=ORIENTED_EDGE('',*,*,#51583,.F.);
#68188=ORIENTED_EDGE('',*,*,#51589,.T.);
#68189=ORIENTED_EDGE('',*,*,#51590,.T.);
#68190=ORIENTED_EDGE('',*,*,#51591,.F.);
#68191=ORIENTED_EDGE('',*,*,#51587,.F.);
#68192=ORIENTED_EDGE('',*,*,#51592,.T.);
#68193=ORIENTED_EDGE('',*,*,#51585,.T.);
#68194=ORIENTED_EDGE('',*,*,#51593,.F.);
#68195=ORIENTED_EDGE('',*,*,#51590,.F.);
#68196=ORIENTED_EDGE('',*,*,#51594,.T.);
#68197=ORIENTED_EDGE('',*,*,#51595,.T.);
#68198=ORIENTED_EDGE('',*,*,#51596,.F.);
#68199=ORIENTED_EDGE('',*,*,#51597,.F.);
#68200=ORIENTED_EDGE('',*,*,#51598,.T.);
#68201=ORIENTED_EDGE('',*,*,#51599,.T.);
#68202=ORIENTED_EDGE('',*,*,#51600,.F.);
#68203=ORIENTED_EDGE('',*,*,#51595,.F.);
#68204=ORIENTED_EDGE('',*,*,#51601,.T.);
#68205=ORIENTED_EDGE('',*,*,#51602,.T.);
#68206=ORIENTED_EDGE('',*,*,#51603,.F.);
#68207=ORIENTED_EDGE('',*,*,#51599,.F.);
#68208=ORIENTED_EDGE('',*,*,#51604,.T.);
#68209=ORIENTED_EDGE('',*,*,#51597,.T.);
#68210=ORIENTED_EDGE('',*,*,#51605,.F.);
#68211=ORIENTED_EDGE('',*,*,#51602,.F.);
#68212=ORIENTED_EDGE('',*,*,#51606,.T.);
#68213=ORIENTED_EDGE('',*,*,#51607,.T.);
#68214=ORIENTED_EDGE('',*,*,#51608,.F.);
#68215=ORIENTED_EDGE('',*,*,#51609,.F.);
#68216=ORIENTED_EDGE('',*,*,#51610,.T.);
#68217=ORIENTED_EDGE('',*,*,#51611,.T.);
#68218=ORIENTED_EDGE('',*,*,#51612,.F.);
#68219=ORIENTED_EDGE('',*,*,#51607,.F.);
#68220=ORIENTED_EDGE('',*,*,#51613,.T.);
#68221=ORIENTED_EDGE('',*,*,#51614,.T.);
#68222=ORIENTED_EDGE('',*,*,#51615,.F.);
#68223=ORIENTED_EDGE('',*,*,#51611,.F.);
#68224=ORIENTED_EDGE('',*,*,#51616,.T.);
#68225=ORIENTED_EDGE('',*,*,#51609,.T.);
#68226=ORIENTED_EDGE('',*,*,#51617,.F.);
#68227=ORIENTED_EDGE('',*,*,#51614,.F.);
#68228=ORIENTED_EDGE('',*,*,#51618,.T.);
#68229=ORIENTED_EDGE('',*,*,#51619,.T.);
#68230=ORIENTED_EDGE('',*,*,#51620,.F.);
#68231=ORIENTED_EDGE('',*,*,#51621,.F.);
#68232=ORIENTED_EDGE('',*,*,#51622,.T.);
#68233=ORIENTED_EDGE('',*,*,#51623,.T.);
#68234=ORIENTED_EDGE('',*,*,#51624,.F.);
#68235=ORIENTED_EDGE('',*,*,#51619,.F.);
#68236=ORIENTED_EDGE('',*,*,#51625,.T.);
#68237=ORIENTED_EDGE('',*,*,#51626,.T.);
#68238=ORIENTED_EDGE('',*,*,#51627,.F.);
#68239=ORIENTED_EDGE('',*,*,#51623,.F.);
#68240=ORIENTED_EDGE('',*,*,#51628,.T.);
#68241=ORIENTED_EDGE('',*,*,#51621,.T.);
#68242=ORIENTED_EDGE('',*,*,#51629,.F.);
#68243=ORIENTED_EDGE('',*,*,#51626,.F.);
#68244=ORIENTED_EDGE('',*,*,#51630,.T.);
#68245=ORIENTED_EDGE('',*,*,#51631,.T.);
#68246=ORIENTED_EDGE('',*,*,#51632,.F.);
#68247=ORIENTED_EDGE('',*,*,#51633,.F.);
#68248=ORIENTED_EDGE('',*,*,#51634,.T.);
#68249=ORIENTED_EDGE('',*,*,#51635,.T.);
#68250=ORIENTED_EDGE('',*,*,#51636,.F.);
#68251=ORIENTED_EDGE('',*,*,#51631,.F.);
#68252=ORIENTED_EDGE('',*,*,#51637,.T.);
#68253=ORIENTED_EDGE('',*,*,#51638,.T.);
#68254=ORIENTED_EDGE('',*,*,#51639,.F.);
#68255=ORIENTED_EDGE('',*,*,#51635,.F.);
#68256=ORIENTED_EDGE('',*,*,#51640,.T.);
#68257=ORIENTED_EDGE('',*,*,#51633,.T.);
#68258=ORIENTED_EDGE('',*,*,#51641,.F.);
#68259=ORIENTED_EDGE('',*,*,#51638,.F.);
#68260=ORIENTED_EDGE('',*,*,#51642,.T.);
#68261=ORIENTED_EDGE('',*,*,#51643,.T.);
#68262=ORIENTED_EDGE('',*,*,#51644,.F.);
#68263=ORIENTED_EDGE('',*,*,#51645,.F.);
#68264=ORIENTED_EDGE('',*,*,#51646,.T.);
#68265=ORIENTED_EDGE('',*,*,#51647,.T.);
#68266=ORIENTED_EDGE('',*,*,#51648,.F.);
#68267=ORIENTED_EDGE('',*,*,#51643,.F.);
#68268=ORIENTED_EDGE('',*,*,#51649,.T.);
#68269=ORIENTED_EDGE('',*,*,#51650,.T.);
#68270=ORIENTED_EDGE('',*,*,#51651,.F.);
#68271=ORIENTED_EDGE('',*,*,#51647,.F.);
#68272=ORIENTED_EDGE('',*,*,#51652,.T.);
#68273=ORIENTED_EDGE('',*,*,#51645,.T.);
#68274=ORIENTED_EDGE('',*,*,#51653,.F.);
#68275=ORIENTED_EDGE('',*,*,#51650,.F.);
#68276=ORIENTED_EDGE('',*,*,#51654,.T.);
#68277=ORIENTED_EDGE('',*,*,#51655,.T.);
#68278=ORIENTED_EDGE('',*,*,#51656,.F.);
#68279=ORIENTED_EDGE('',*,*,#51657,.F.);
#68280=ORIENTED_EDGE('',*,*,#51658,.T.);
#68281=ORIENTED_EDGE('',*,*,#51659,.T.);
#68282=ORIENTED_EDGE('',*,*,#51660,.F.);
#68283=ORIENTED_EDGE('',*,*,#51655,.F.);
#68284=ORIENTED_EDGE('',*,*,#51661,.T.);
#68285=ORIENTED_EDGE('',*,*,#51662,.T.);
#68286=ORIENTED_EDGE('',*,*,#51663,.F.);
#68287=ORIENTED_EDGE('',*,*,#51659,.F.);
#68288=ORIENTED_EDGE('',*,*,#51664,.T.);
#68289=ORIENTED_EDGE('',*,*,#51657,.T.);
#68290=ORIENTED_EDGE('',*,*,#51665,.F.);
#68291=ORIENTED_EDGE('',*,*,#51662,.F.);
#68292=ORIENTED_EDGE('',*,*,#51666,.T.);
#68293=ORIENTED_EDGE('',*,*,#51667,.T.);
#68294=ORIENTED_EDGE('',*,*,#51668,.F.);
#68295=ORIENTED_EDGE('',*,*,#51669,.F.);
#68296=ORIENTED_EDGE('',*,*,#51670,.T.);
#68297=ORIENTED_EDGE('',*,*,#51671,.T.);
#68298=ORIENTED_EDGE('',*,*,#51672,.F.);
#68299=ORIENTED_EDGE('',*,*,#51667,.F.);
#68300=ORIENTED_EDGE('',*,*,#51673,.T.);
#68301=ORIENTED_EDGE('',*,*,#51674,.T.);
#68302=ORIENTED_EDGE('',*,*,#51675,.F.);
#68303=ORIENTED_EDGE('',*,*,#51671,.F.);
#68304=ORIENTED_EDGE('',*,*,#51676,.T.);
#68305=ORIENTED_EDGE('',*,*,#51669,.T.);
#68306=ORIENTED_EDGE('',*,*,#51677,.F.);
#68307=ORIENTED_EDGE('',*,*,#51674,.F.);
#68308=ORIENTED_EDGE('',*,*,#51678,.T.);
#68309=ORIENTED_EDGE('',*,*,#51679,.T.);
#68310=ORIENTED_EDGE('',*,*,#51680,.F.);
#68311=ORIENTED_EDGE('',*,*,#51681,.F.);
#68312=ORIENTED_EDGE('',*,*,#51682,.T.);
#68313=ORIENTED_EDGE('',*,*,#51683,.T.);
#68314=ORIENTED_EDGE('',*,*,#51684,.F.);
#68315=ORIENTED_EDGE('',*,*,#51679,.F.);
#68316=ORIENTED_EDGE('',*,*,#51685,.T.);
#68317=ORIENTED_EDGE('',*,*,#51686,.T.);
#68318=ORIENTED_EDGE('',*,*,#51687,.F.);
#68319=ORIENTED_EDGE('',*,*,#51683,.F.);
#68320=ORIENTED_EDGE('',*,*,#51688,.T.);
#68321=ORIENTED_EDGE('',*,*,#51681,.T.);
#68322=ORIENTED_EDGE('',*,*,#51689,.F.);
#68323=ORIENTED_EDGE('',*,*,#51686,.F.);
#68324=ORIENTED_EDGE('',*,*,#51690,.T.);
#68325=ORIENTED_EDGE('',*,*,#51691,.T.);
#68326=ORIENTED_EDGE('',*,*,#51692,.F.);
#68327=ORIENTED_EDGE('',*,*,#51693,.F.);
#68328=ORIENTED_EDGE('',*,*,#51694,.T.);
#68329=ORIENTED_EDGE('',*,*,#51695,.T.);
#68330=ORIENTED_EDGE('',*,*,#51696,.F.);
#68331=ORIENTED_EDGE('',*,*,#51691,.F.);
#68332=ORIENTED_EDGE('',*,*,#51697,.T.);
#68333=ORIENTED_EDGE('',*,*,#51698,.T.);
#68334=ORIENTED_EDGE('',*,*,#51699,.F.);
#68335=ORIENTED_EDGE('',*,*,#51695,.F.);
#68336=ORIENTED_EDGE('',*,*,#51700,.T.);
#68337=ORIENTED_EDGE('',*,*,#51693,.T.);
#68338=ORIENTED_EDGE('',*,*,#51701,.F.);
#68339=ORIENTED_EDGE('',*,*,#51698,.F.);
#68340=ORIENTED_EDGE('',*,*,#51702,.T.);
#68341=ORIENTED_EDGE('',*,*,#51703,.T.);
#68342=ORIENTED_EDGE('',*,*,#51704,.F.);
#68343=ORIENTED_EDGE('',*,*,#51705,.F.);
#68344=ORIENTED_EDGE('',*,*,#51706,.T.);
#68345=ORIENTED_EDGE('',*,*,#51707,.T.);
#68346=ORIENTED_EDGE('',*,*,#51708,.F.);
#68347=ORIENTED_EDGE('',*,*,#51703,.F.);
#68348=ORIENTED_EDGE('',*,*,#51709,.T.);
#68349=ORIENTED_EDGE('',*,*,#51710,.T.);
#68350=ORIENTED_EDGE('',*,*,#51711,.F.);
#68351=ORIENTED_EDGE('',*,*,#51707,.F.);
#68352=ORIENTED_EDGE('',*,*,#51712,.T.);
#68353=ORIENTED_EDGE('',*,*,#51705,.T.);
#68354=ORIENTED_EDGE('',*,*,#51713,.F.);
#68355=ORIENTED_EDGE('',*,*,#51710,.F.);
#68356=ORIENTED_EDGE('',*,*,#51714,.T.);
#68357=ORIENTED_EDGE('',*,*,#51715,.T.);
#68358=ORIENTED_EDGE('',*,*,#51716,.F.);
#68359=ORIENTED_EDGE('',*,*,#51717,.F.);
#68360=ORIENTED_EDGE('',*,*,#51718,.T.);
#68361=ORIENTED_EDGE('',*,*,#51719,.T.);
#68362=ORIENTED_EDGE('',*,*,#51720,.F.);
#68363=ORIENTED_EDGE('',*,*,#51715,.F.);
#68364=ORIENTED_EDGE('',*,*,#51721,.T.);
#68365=ORIENTED_EDGE('',*,*,#51722,.T.);
#68366=ORIENTED_EDGE('',*,*,#51723,.F.);
#68367=ORIENTED_EDGE('',*,*,#51719,.F.);
#68368=ORIENTED_EDGE('',*,*,#51724,.T.);
#68369=ORIENTED_EDGE('',*,*,#51717,.T.);
#68370=ORIENTED_EDGE('',*,*,#51725,.F.);
#68371=ORIENTED_EDGE('',*,*,#51722,.F.);
#68372=ORIENTED_EDGE('',*,*,#51726,.T.);
#68373=ORIENTED_EDGE('',*,*,#51727,.T.);
#68374=ORIENTED_EDGE('',*,*,#51728,.F.);
#68375=ORIENTED_EDGE('',*,*,#51729,.F.);
#68376=ORIENTED_EDGE('',*,*,#51730,.T.);
#68377=ORIENTED_EDGE('',*,*,#51731,.T.);
#68378=ORIENTED_EDGE('',*,*,#51732,.F.);
#68379=ORIENTED_EDGE('',*,*,#51727,.F.);
#68380=ORIENTED_EDGE('',*,*,#51733,.T.);
#68381=ORIENTED_EDGE('',*,*,#51734,.T.);
#68382=ORIENTED_EDGE('',*,*,#51735,.F.);
#68383=ORIENTED_EDGE('',*,*,#51731,.F.);
#68384=ORIENTED_EDGE('',*,*,#51736,.T.);
#68385=ORIENTED_EDGE('',*,*,#51729,.T.);
#68386=ORIENTED_EDGE('',*,*,#51737,.F.);
#68387=ORIENTED_EDGE('',*,*,#51734,.F.);
#68388=ORIENTED_EDGE('',*,*,#51738,.T.);
#68389=ORIENTED_EDGE('',*,*,#51739,.T.);
#68390=ORIENTED_EDGE('',*,*,#51740,.F.);
#68391=ORIENTED_EDGE('',*,*,#51741,.F.);
#68392=ORIENTED_EDGE('',*,*,#51742,.T.);
#68393=ORIENTED_EDGE('',*,*,#51743,.T.);
#68394=ORIENTED_EDGE('',*,*,#51744,.F.);
#68395=ORIENTED_EDGE('',*,*,#51739,.F.);
#68396=ORIENTED_EDGE('',*,*,#51745,.T.);
#68397=ORIENTED_EDGE('',*,*,#51746,.T.);
#68398=ORIENTED_EDGE('',*,*,#51747,.F.);
#68399=ORIENTED_EDGE('',*,*,#51743,.F.);
#68400=ORIENTED_EDGE('',*,*,#51748,.T.);
#68401=ORIENTED_EDGE('',*,*,#51741,.T.);
#68402=ORIENTED_EDGE('',*,*,#51749,.F.);
#68403=ORIENTED_EDGE('',*,*,#51746,.F.);
#68404=ORIENTED_EDGE('',*,*,#51750,.T.);
#68405=ORIENTED_EDGE('',*,*,#51751,.T.);
#68406=ORIENTED_EDGE('',*,*,#51752,.F.);
#68407=ORIENTED_EDGE('',*,*,#51753,.F.);
#68408=ORIENTED_EDGE('',*,*,#51754,.T.);
#68409=ORIENTED_EDGE('',*,*,#51755,.T.);
#68410=ORIENTED_EDGE('',*,*,#51756,.F.);
#68411=ORIENTED_EDGE('',*,*,#51751,.F.);
#68412=ORIENTED_EDGE('',*,*,#51757,.T.);
#68413=ORIENTED_EDGE('',*,*,#51758,.T.);
#68414=ORIENTED_EDGE('',*,*,#51759,.F.);
#68415=ORIENTED_EDGE('',*,*,#51755,.F.);
#68416=ORIENTED_EDGE('',*,*,#51760,.T.);
#68417=ORIENTED_EDGE('',*,*,#51753,.T.);
#68418=ORIENTED_EDGE('',*,*,#51761,.F.);
#68419=ORIENTED_EDGE('',*,*,#51758,.F.);
#68420=ORIENTED_EDGE('',*,*,#51762,.T.);
#68421=ORIENTED_EDGE('',*,*,#51763,.T.);
#68422=ORIENTED_EDGE('',*,*,#51764,.F.);
#68423=ORIENTED_EDGE('',*,*,#51765,.F.);
#68424=ORIENTED_EDGE('',*,*,#51766,.T.);
#68425=ORIENTED_EDGE('',*,*,#51767,.T.);
#68426=ORIENTED_EDGE('',*,*,#51768,.F.);
#68427=ORIENTED_EDGE('',*,*,#51763,.F.);
#68428=ORIENTED_EDGE('',*,*,#51769,.T.);
#68429=ORIENTED_EDGE('',*,*,#51770,.T.);
#68430=ORIENTED_EDGE('',*,*,#51771,.F.);
#68431=ORIENTED_EDGE('',*,*,#51767,.F.);
#68432=ORIENTED_EDGE('',*,*,#51772,.T.);
#68433=ORIENTED_EDGE('',*,*,#51765,.T.);
#68434=ORIENTED_EDGE('',*,*,#51773,.F.);
#68435=ORIENTED_EDGE('',*,*,#51770,.F.);
#68436=ORIENTED_EDGE('',*,*,#51774,.T.);
#68437=ORIENTED_EDGE('',*,*,#51775,.T.);
#68438=ORIENTED_EDGE('',*,*,#51776,.F.);
#68439=ORIENTED_EDGE('',*,*,#51777,.F.);
#68440=ORIENTED_EDGE('',*,*,#51778,.T.);
#68441=ORIENTED_EDGE('',*,*,#51779,.T.);
#68442=ORIENTED_EDGE('',*,*,#51780,.F.);
#68443=ORIENTED_EDGE('',*,*,#51775,.F.);
#68444=ORIENTED_EDGE('',*,*,#51781,.T.);
#68445=ORIENTED_EDGE('',*,*,#51782,.T.);
#68446=ORIENTED_EDGE('',*,*,#51783,.F.);
#68447=ORIENTED_EDGE('',*,*,#51779,.F.);
#68448=ORIENTED_EDGE('',*,*,#51784,.T.);
#68449=ORIENTED_EDGE('',*,*,#51777,.T.);
#68450=ORIENTED_EDGE('',*,*,#51785,.F.);
#68451=ORIENTED_EDGE('',*,*,#51782,.F.);
#68452=ORIENTED_EDGE('',*,*,#51786,.T.);
#68453=ORIENTED_EDGE('',*,*,#51787,.T.);
#68454=ORIENTED_EDGE('',*,*,#51788,.F.);
#68455=ORIENTED_EDGE('',*,*,#51789,.F.);
#68456=ORIENTED_EDGE('',*,*,#51790,.T.);
#68457=ORIENTED_EDGE('',*,*,#51791,.T.);
#68458=ORIENTED_EDGE('',*,*,#51792,.F.);
#68459=ORIENTED_EDGE('',*,*,#51787,.F.);
#68460=ORIENTED_EDGE('',*,*,#51793,.T.);
#68461=ORIENTED_EDGE('',*,*,#51794,.T.);
#68462=ORIENTED_EDGE('',*,*,#51795,.F.);
#68463=ORIENTED_EDGE('',*,*,#51791,.F.);
#68464=ORIENTED_EDGE('',*,*,#51796,.T.);
#68465=ORIENTED_EDGE('',*,*,#51789,.T.);
#68466=ORIENTED_EDGE('',*,*,#51797,.F.);
#68467=ORIENTED_EDGE('',*,*,#51794,.F.);
#68468=ORIENTED_EDGE('',*,*,#51798,.T.);
#68469=ORIENTED_EDGE('',*,*,#51799,.T.);
#68470=ORIENTED_EDGE('',*,*,#51800,.F.);
#68471=ORIENTED_EDGE('',*,*,#51801,.F.);
#68472=ORIENTED_EDGE('',*,*,#51802,.T.);
#68473=ORIENTED_EDGE('',*,*,#51803,.T.);
#68474=ORIENTED_EDGE('',*,*,#51804,.F.);
#68475=ORIENTED_EDGE('',*,*,#51799,.F.);
#68476=ORIENTED_EDGE('',*,*,#51805,.T.);
#68477=ORIENTED_EDGE('',*,*,#51806,.T.);
#68478=ORIENTED_EDGE('',*,*,#51807,.F.);
#68479=ORIENTED_EDGE('',*,*,#51803,.F.);
#68480=ORIENTED_EDGE('',*,*,#51808,.T.);
#68481=ORIENTED_EDGE('',*,*,#51801,.T.);
#68482=ORIENTED_EDGE('',*,*,#51809,.F.);
#68483=ORIENTED_EDGE('',*,*,#51806,.F.);
#68484=ORIENTED_EDGE('',*,*,#51810,.T.);
#68485=ORIENTED_EDGE('',*,*,#51811,.T.);
#68486=ORIENTED_EDGE('',*,*,#51812,.F.);
#68487=ORIENTED_EDGE('',*,*,#51813,.F.);
#68488=ORIENTED_EDGE('',*,*,#51814,.T.);
#68489=ORIENTED_EDGE('',*,*,#51815,.T.);
#68490=ORIENTED_EDGE('',*,*,#51816,.F.);
#68491=ORIENTED_EDGE('',*,*,#51811,.F.);
#68492=ORIENTED_EDGE('',*,*,#51817,.T.);
#68493=ORIENTED_EDGE('',*,*,#51818,.T.);
#68494=ORIENTED_EDGE('',*,*,#51819,.F.);
#68495=ORIENTED_EDGE('',*,*,#51815,.F.);
#68496=ORIENTED_EDGE('',*,*,#51820,.T.);
#68497=ORIENTED_EDGE('',*,*,#51813,.T.);
#68498=ORIENTED_EDGE('',*,*,#51821,.F.);
#68499=ORIENTED_EDGE('',*,*,#51818,.F.);
#68500=ORIENTED_EDGE('',*,*,#51822,.T.);
#68501=ORIENTED_EDGE('',*,*,#51823,.T.);
#68502=ORIENTED_EDGE('',*,*,#51824,.F.);
#68503=ORIENTED_EDGE('',*,*,#51825,.F.);
#68504=ORIENTED_EDGE('',*,*,#51826,.T.);
#68505=ORIENTED_EDGE('',*,*,#51827,.T.);
#68506=ORIENTED_EDGE('',*,*,#51828,.F.);
#68507=ORIENTED_EDGE('',*,*,#51823,.F.);
#68508=ORIENTED_EDGE('',*,*,#51829,.T.);
#68509=ORIENTED_EDGE('',*,*,#51830,.T.);
#68510=ORIENTED_EDGE('',*,*,#51831,.F.);
#68511=ORIENTED_EDGE('',*,*,#51827,.F.);
#68512=ORIENTED_EDGE('',*,*,#51832,.T.);
#68513=ORIENTED_EDGE('',*,*,#51825,.T.);
#68514=ORIENTED_EDGE('',*,*,#51833,.F.);
#68515=ORIENTED_EDGE('',*,*,#51830,.F.);
#68516=ORIENTED_EDGE('',*,*,#51834,.T.);
#68517=ORIENTED_EDGE('',*,*,#51835,.T.);
#68518=ORIENTED_EDGE('',*,*,#51836,.F.);
#68519=ORIENTED_EDGE('',*,*,#51837,.F.);
#68520=ORIENTED_EDGE('',*,*,#51838,.T.);
#68521=ORIENTED_EDGE('',*,*,#51839,.T.);
#68522=ORIENTED_EDGE('',*,*,#51840,.F.);
#68523=ORIENTED_EDGE('',*,*,#51835,.F.);
#68524=ORIENTED_EDGE('',*,*,#51841,.T.);
#68525=ORIENTED_EDGE('',*,*,#51842,.T.);
#68526=ORIENTED_EDGE('',*,*,#51843,.F.);
#68527=ORIENTED_EDGE('',*,*,#51839,.F.);
#68528=ORIENTED_EDGE('',*,*,#51844,.T.);
#68529=ORIENTED_EDGE('',*,*,#51837,.T.);
#68530=ORIENTED_EDGE('',*,*,#51845,.F.);
#68531=ORIENTED_EDGE('',*,*,#51842,.F.);
#68532=ORIENTED_EDGE('',*,*,#51846,.T.);
#68533=ORIENTED_EDGE('',*,*,#51847,.T.);
#68534=ORIENTED_EDGE('',*,*,#51848,.F.);
#68535=ORIENTED_EDGE('',*,*,#51849,.F.);
#68536=ORIENTED_EDGE('',*,*,#51850,.T.);
#68537=ORIENTED_EDGE('',*,*,#51851,.T.);
#68538=ORIENTED_EDGE('',*,*,#51852,.F.);
#68539=ORIENTED_EDGE('',*,*,#51847,.F.);
#68540=ORIENTED_EDGE('',*,*,#51853,.T.);
#68541=ORIENTED_EDGE('',*,*,#51854,.T.);
#68542=ORIENTED_EDGE('',*,*,#51855,.F.);
#68543=ORIENTED_EDGE('',*,*,#51851,.F.);
#68544=ORIENTED_EDGE('',*,*,#51856,.T.);
#68545=ORIENTED_EDGE('',*,*,#51849,.T.);
#68546=ORIENTED_EDGE('',*,*,#51857,.F.);
#68547=ORIENTED_EDGE('',*,*,#51854,.F.);
#68548=ORIENTED_EDGE('',*,*,#51858,.T.);
#68549=ORIENTED_EDGE('',*,*,#51859,.T.);
#68550=ORIENTED_EDGE('',*,*,#51860,.F.);
#68551=ORIENTED_EDGE('',*,*,#51861,.F.);
#68552=ORIENTED_EDGE('',*,*,#51862,.T.);
#68553=ORIENTED_EDGE('',*,*,#51863,.T.);
#68554=ORIENTED_EDGE('',*,*,#51864,.F.);
#68555=ORIENTED_EDGE('',*,*,#51859,.F.);
#68556=ORIENTED_EDGE('',*,*,#51865,.T.);
#68557=ORIENTED_EDGE('',*,*,#51866,.T.);
#68558=ORIENTED_EDGE('',*,*,#51867,.F.);
#68559=ORIENTED_EDGE('',*,*,#51863,.F.);
#68560=ORIENTED_EDGE('',*,*,#51868,.T.);
#68561=ORIENTED_EDGE('',*,*,#51861,.T.);
#68562=ORIENTED_EDGE('',*,*,#51869,.F.);
#68563=ORIENTED_EDGE('',*,*,#51866,.F.);
#68564=ORIENTED_EDGE('',*,*,#51870,.T.);
#68565=ORIENTED_EDGE('',*,*,#51871,.T.);
#68566=ORIENTED_EDGE('',*,*,#51872,.F.);
#68567=ORIENTED_EDGE('',*,*,#51873,.F.);
#68568=ORIENTED_EDGE('',*,*,#51874,.T.);
#68569=ORIENTED_EDGE('',*,*,#51875,.T.);
#68570=ORIENTED_EDGE('',*,*,#51876,.F.);
#68571=ORIENTED_EDGE('',*,*,#51871,.F.);
#68572=ORIENTED_EDGE('',*,*,#51877,.T.);
#68573=ORIENTED_EDGE('',*,*,#51878,.T.);
#68574=ORIENTED_EDGE('',*,*,#51879,.F.);
#68575=ORIENTED_EDGE('',*,*,#51875,.F.);
#68576=ORIENTED_EDGE('',*,*,#51880,.T.);
#68577=ORIENTED_EDGE('',*,*,#51873,.T.);
#68578=ORIENTED_EDGE('',*,*,#51881,.F.);
#68579=ORIENTED_EDGE('',*,*,#51878,.F.);
#68580=ORIENTED_EDGE('',*,*,#51882,.T.);
#68581=ORIENTED_EDGE('',*,*,#51883,.T.);
#68582=ORIENTED_EDGE('',*,*,#51884,.F.);
#68583=ORIENTED_EDGE('',*,*,#51885,.F.);
#68584=ORIENTED_EDGE('',*,*,#51886,.T.);
#68585=ORIENTED_EDGE('',*,*,#51887,.T.);
#68586=ORIENTED_EDGE('',*,*,#51888,.F.);
#68587=ORIENTED_EDGE('',*,*,#51883,.F.);
#68588=ORIENTED_EDGE('',*,*,#51889,.T.);
#68589=ORIENTED_EDGE('',*,*,#51890,.T.);
#68590=ORIENTED_EDGE('',*,*,#51891,.F.);
#68591=ORIENTED_EDGE('',*,*,#51887,.F.);
#68592=ORIENTED_EDGE('',*,*,#51892,.T.);
#68593=ORIENTED_EDGE('',*,*,#51885,.T.);
#68594=ORIENTED_EDGE('',*,*,#51893,.F.);
#68595=ORIENTED_EDGE('',*,*,#51890,.F.);
#68596=ORIENTED_EDGE('',*,*,#51894,.T.);
#68597=ORIENTED_EDGE('',*,*,#51895,.T.);
#68598=ORIENTED_EDGE('',*,*,#51896,.F.);
#68599=ORIENTED_EDGE('',*,*,#51897,.F.);
#68600=ORIENTED_EDGE('',*,*,#51898,.T.);
#68601=ORIENTED_EDGE('',*,*,#51899,.T.);
#68602=ORIENTED_EDGE('',*,*,#51900,.F.);
#68603=ORIENTED_EDGE('',*,*,#51895,.F.);
#68604=ORIENTED_EDGE('',*,*,#51901,.T.);
#68605=ORIENTED_EDGE('',*,*,#51902,.T.);
#68606=ORIENTED_EDGE('',*,*,#51903,.F.);
#68607=ORIENTED_EDGE('',*,*,#51899,.F.);
#68608=ORIENTED_EDGE('',*,*,#51904,.T.);
#68609=ORIENTED_EDGE('',*,*,#51897,.T.);
#68610=ORIENTED_EDGE('',*,*,#51905,.F.);
#68611=ORIENTED_EDGE('',*,*,#51902,.F.);
#68612=ORIENTED_EDGE('',*,*,#51906,.T.);
#68613=ORIENTED_EDGE('',*,*,#51907,.T.);
#68614=ORIENTED_EDGE('',*,*,#51908,.F.);
#68615=ORIENTED_EDGE('',*,*,#51909,.F.);
#68616=ORIENTED_EDGE('',*,*,#51910,.T.);
#68617=ORIENTED_EDGE('',*,*,#51911,.T.);
#68618=ORIENTED_EDGE('',*,*,#51912,.F.);
#68619=ORIENTED_EDGE('',*,*,#51907,.F.);
#68620=ORIENTED_EDGE('',*,*,#51913,.T.);
#68621=ORIENTED_EDGE('',*,*,#51914,.T.);
#68622=ORIENTED_EDGE('',*,*,#51915,.F.);
#68623=ORIENTED_EDGE('',*,*,#51911,.F.);
#68624=ORIENTED_EDGE('',*,*,#51916,.T.);
#68625=ORIENTED_EDGE('',*,*,#51909,.T.);
#68626=ORIENTED_EDGE('',*,*,#51917,.F.);
#68627=ORIENTED_EDGE('',*,*,#51914,.F.);
#68628=ORIENTED_EDGE('',*,*,#51918,.T.);
#68629=ORIENTED_EDGE('',*,*,#51919,.T.);
#68630=ORIENTED_EDGE('',*,*,#51920,.F.);
#68631=ORIENTED_EDGE('',*,*,#51921,.F.);
#68632=ORIENTED_EDGE('',*,*,#51922,.T.);
#68633=ORIENTED_EDGE('',*,*,#51923,.T.);
#68634=ORIENTED_EDGE('',*,*,#51924,.F.);
#68635=ORIENTED_EDGE('',*,*,#51919,.F.);
#68636=ORIENTED_EDGE('',*,*,#51925,.T.);
#68637=ORIENTED_EDGE('',*,*,#51926,.T.);
#68638=ORIENTED_EDGE('',*,*,#51927,.F.);
#68639=ORIENTED_EDGE('',*,*,#51923,.F.);
#68640=ORIENTED_EDGE('',*,*,#51928,.T.);
#68641=ORIENTED_EDGE('',*,*,#51921,.T.);
#68642=ORIENTED_EDGE('',*,*,#51929,.F.);
#68643=ORIENTED_EDGE('',*,*,#51926,.F.);
#68644=ORIENTED_EDGE('',*,*,#51930,.T.);
#68645=ORIENTED_EDGE('',*,*,#51931,.T.);
#68646=ORIENTED_EDGE('',*,*,#51932,.F.);
#68647=ORIENTED_EDGE('',*,*,#51933,.F.);
#68648=ORIENTED_EDGE('',*,*,#51934,.T.);
#68649=ORIENTED_EDGE('',*,*,#51935,.T.);
#68650=ORIENTED_EDGE('',*,*,#51936,.F.);
#68651=ORIENTED_EDGE('',*,*,#51931,.F.);
#68652=ORIENTED_EDGE('',*,*,#51937,.T.);
#68653=ORIENTED_EDGE('',*,*,#51938,.T.);
#68654=ORIENTED_EDGE('',*,*,#51939,.F.);
#68655=ORIENTED_EDGE('',*,*,#51935,.F.);
#68656=ORIENTED_EDGE('',*,*,#51940,.T.);
#68657=ORIENTED_EDGE('',*,*,#51933,.T.);
#68658=ORIENTED_EDGE('',*,*,#51941,.F.);
#68659=ORIENTED_EDGE('',*,*,#51938,.F.);
#68660=ORIENTED_EDGE('',*,*,#51942,.T.);
#68661=ORIENTED_EDGE('',*,*,#51943,.T.);
#68662=ORIENTED_EDGE('',*,*,#51944,.F.);
#68663=ORIENTED_EDGE('',*,*,#51945,.F.);
#68664=ORIENTED_EDGE('',*,*,#51946,.T.);
#68665=ORIENTED_EDGE('',*,*,#51947,.T.);
#68666=ORIENTED_EDGE('',*,*,#51948,.F.);
#68667=ORIENTED_EDGE('',*,*,#51943,.F.);
#68668=ORIENTED_EDGE('',*,*,#51949,.T.);
#68669=ORIENTED_EDGE('',*,*,#51950,.T.);
#68670=ORIENTED_EDGE('',*,*,#51951,.F.);
#68671=ORIENTED_EDGE('',*,*,#51947,.F.);
#68672=ORIENTED_EDGE('',*,*,#51952,.T.);
#68673=ORIENTED_EDGE('',*,*,#51945,.T.);
#68674=ORIENTED_EDGE('',*,*,#51953,.F.);
#68675=ORIENTED_EDGE('',*,*,#51950,.F.);
#68676=ORIENTED_EDGE('',*,*,#51954,.T.);
#68677=ORIENTED_EDGE('',*,*,#51955,.T.);
#68678=ORIENTED_EDGE('',*,*,#51956,.F.);
#68679=ORIENTED_EDGE('',*,*,#51957,.F.);
#68680=ORIENTED_EDGE('',*,*,#51958,.T.);
#68681=ORIENTED_EDGE('',*,*,#51959,.T.);
#68682=ORIENTED_EDGE('',*,*,#51960,.F.);
#68683=ORIENTED_EDGE('',*,*,#51955,.F.);
#68684=ORIENTED_EDGE('',*,*,#51961,.T.);
#68685=ORIENTED_EDGE('',*,*,#51962,.T.);
#68686=ORIENTED_EDGE('',*,*,#51963,.F.);
#68687=ORIENTED_EDGE('',*,*,#51959,.F.);
#68688=ORIENTED_EDGE('',*,*,#51964,.T.);
#68689=ORIENTED_EDGE('',*,*,#51957,.T.);
#68690=ORIENTED_EDGE('',*,*,#51965,.F.);
#68691=ORIENTED_EDGE('',*,*,#51962,.F.);
#68692=ORIENTED_EDGE('',*,*,#51966,.T.);
#68693=ORIENTED_EDGE('',*,*,#43453,.T.);
#68694=ORIENTED_EDGE('',*,*,#43496,.F.);
#68695=ORIENTED_EDGE('',*,*,#43498,.T.);
#68696=ORIENTED_EDGE('',*,*,#46736,.T.);
#68697=ORIENTED_EDGE('',*,*,#46740,.T.);
#68698=ORIENTED_EDGE('',*,*,#46743,.T.);
#68699=ORIENTED_EDGE('',*,*,#46745,.T.);
#68700=ORIENTED_EDGE('',*,*,#46748,.T.);
#68701=ORIENTED_EDGE('',*,*,#46752,.T.);
#68702=ORIENTED_EDGE('',*,*,#46755,.T.);
#68703=ORIENTED_EDGE('',*,*,#46757,.T.);
#68704=ORIENTED_EDGE('',*,*,#46760,.T.);
#68705=ORIENTED_EDGE('',*,*,#46764,.T.);
#68706=ORIENTED_EDGE('',*,*,#46767,.T.);
#68707=ORIENTED_EDGE('',*,*,#46769,.T.);
#68708=ORIENTED_EDGE('',*,*,#46772,.T.);
#68709=ORIENTED_EDGE('',*,*,#46776,.T.);
#68710=ORIENTED_EDGE('',*,*,#46779,.T.);
#68711=ORIENTED_EDGE('',*,*,#46781,.T.);
#68712=ORIENTED_EDGE('',*,*,#46784,.T.);
#68713=ORIENTED_EDGE('',*,*,#46788,.T.);
#68714=ORIENTED_EDGE('',*,*,#46791,.T.);
#68715=ORIENTED_EDGE('',*,*,#46793,.T.);
#68716=ORIENTED_EDGE('',*,*,#46796,.T.);
#68717=ORIENTED_EDGE('',*,*,#46800,.T.);
#68718=ORIENTED_EDGE('',*,*,#46803,.T.);
#68719=ORIENTED_EDGE('',*,*,#46805,.T.);
#68720=ORIENTED_EDGE('',*,*,#46808,.T.);
#68721=ORIENTED_EDGE('',*,*,#46812,.T.);
#68722=ORIENTED_EDGE('',*,*,#46815,.T.);
#68723=ORIENTED_EDGE('',*,*,#46817,.T.);
#68724=ORIENTED_EDGE('',*,*,#46820,.T.);
#68725=ORIENTED_EDGE('',*,*,#46824,.T.);
#68726=ORIENTED_EDGE('',*,*,#46827,.T.);
#68727=ORIENTED_EDGE('',*,*,#46829,.T.);
#68728=ORIENTED_EDGE('',*,*,#46832,.T.);
#68729=ORIENTED_EDGE('',*,*,#46836,.T.);
#68730=ORIENTED_EDGE('',*,*,#46839,.T.);
#68731=ORIENTED_EDGE('',*,*,#46841,.T.);
#68732=ORIENTED_EDGE('',*,*,#46844,.T.);
#68733=ORIENTED_EDGE('',*,*,#46848,.T.);
#68734=ORIENTED_EDGE('',*,*,#46851,.T.);
#68735=ORIENTED_EDGE('',*,*,#46853,.T.);
#68736=ORIENTED_EDGE('',*,*,#46856,.T.);
#68737=ORIENTED_EDGE('',*,*,#46860,.T.);
#68738=ORIENTED_EDGE('',*,*,#46863,.T.);
#68739=ORIENTED_EDGE('',*,*,#46865,.T.);
#68740=ORIENTED_EDGE('',*,*,#46868,.T.);
#68741=ORIENTED_EDGE('',*,*,#46872,.T.);
#68742=ORIENTED_EDGE('',*,*,#46875,.T.);
#68743=ORIENTED_EDGE('',*,*,#46877,.T.);
#68744=ORIENTED_EDGE('',*,*,#46880,.T.);
#68745=ORIENTED_EDGE('',*,*,#46884,.T.);
#68746=ORIENTED_EDGE('',*,*,#46887,.T.);
#68747=ORIENTED_EDGE('',*,*,#46889,.T.);
#68748=ORIENTED_EDGE('',*,*,#46892,.T.);
#68749=ORIENTED_EDGE('',*,*,#46896,.T.);
#68750=ORIENTED_EDGE('',*,*,#46899,.T.);
#68751=ORIENTED_EDGE('',*,*,#46901,.T.);
#68752=ORIENTED_EDGE('',*,*,#46904,.T.);
#68753=ORIENTED_EDGE('',*,*,#46908,.T.);
#68754=ORIENTED_EDGE('',*,*,#46911,.T.);
#68755=ORIENTED_EDGE('',*,*,#46913,.T.);
#68756=ORIENTED_EDGE('',*,*,#46916,.T.);
#68757=ORIENTED_EDGE('',*,*,#46920,.T.);
#68758=ORIENTED_EDGE('',*,*,#46923,.T.);
#68759=ORIENTED_EDGE('',*,*,#46925,.T.);
#68760=ORIENTED_EDGE('',*,*,#46928,.T.);
#68761=ORIENTED_EDGE('',*,*,#46932,.T.);
#68762=ORIENTED_EDGE('',*,*,#46935,.T.);
#68763=ORIENTED_EDGE('',*,*,#46937,.T.);
#68764=ORIENTED_EDGE('',*,*,#46940,.T.);
#68765=ORIENTED_EDGE('',*,*,#46944,.T.);
#68766=ORIENTED_EDGE('',*,*,#46947,.T.);
#68767=ORIENTED_EDGE('',*,*,#46949,.T.);
#68768=ORIENTED_EDGE('',*,*,#46952,.T.);
#68769=ORIENTED_EDGE('',*,*,#46956,.T.);
#68770=ORIENTED_EDGE('',*,*,#46959,.T.);
#68771=ORIENTED_EDGE('',*,*,#46961,.T.);
#68772=ORIENTED_EDGE('',*,*,#46964,.T.);
#68773=ORIENTED_EDGE('',*,*,#46968,.T.);
#68774=ORIENTED_EDGE('',*,*,#46971,.T.);
#68775=ORIENTED_EDGE('',*,*,#46973,.T.);
#68776=ORIENTED_EDGE('',*,*,#46976,.T.);
#68777=ORIENTED_EDGE('',*,*,#46980,.T.);
#68778=ORIENTED_EDGE('',*,*,#46983,.T.);
#68779=ORIENTED_EDGE('',*,*,#46985,.T.);
#68780=ORIENTED_EDGE('',*,*,#46988,.T.);
#68781=ORIENTED_EDGE('',*,*,#46992,.T.);
#68782=ORIENTED_EDGE('',*,*,#46995,.T.);
#68783=ORIENTED_EDGE('',*,*,#46997,.T.);
#68784=ORIENTED_EDGE('',*,*,#47000,.T.);
#68785=ORIENTED_EDGE('',*,*,#47004,.T.);
#68786=ORIENTED_EDGE('',*,*,#47007,.T.);
#68787=ORIENTED_EDGE('',*,*,#47009,.T.);
#68788=ORIENTED_EDGE('',*,*,#47012,.T.);
#68789=ORIENTED_EDGE('',*,*,#47016,.T.);
#68790=ORIENTED_EDGE('',*,*,#47019,.T.);
#68791=ORIENTED_EDGE('',*,*,#47021,.T.);
#68792=ORIENTED_EDGE('',*,*,#47024,.T.);
#68793=ORIENTED_EDGE('',*,*,#47028,.T.);
#68794=ORIENTED_EDGE('',*,*,#47031,.T.);
#68795=ORIENTED_EDGE('',*,*,#47033,.T.);
#68796=ORIENTED_EDGE('',*,*,#47036,.T.);
#68797=ORIENTED_EDGE('',*,*,#47040,.T.);
#68798=ORIENTED_EDGE('',*,*,#47043,.T.);
#68799=ORIENTED_EDGE('',*,*,#47045,.T.);
#68800=ORIENTED_EDGE('',*,*,#47048,.T.);
#68801=ORIENTED_EDGE('',*,*,#47052,.T.);
#68802=ORIENTED_EDGE('',*,*,#47055,.T.);
#68803=ORIENTED_EDGE('',*,*,#47057,.T.);
#68804=ORIENTED_EDGE('',*,*,#47060,.T.);
#68805=ORIENTED_EDGE('',*,*,#47064,.T.);
#68806=ORIENTED_EDGE('',*,*,#47067,.T.);
#68807=ORIENTED_EDGE('',*,*,#47069,.T.);
#68808=ORIENTED_EDGE('',*,*,#47072,.T.);
#68809=ORIENTED_EDGE('',*,*,#47076,.T.);
#68810=ORIENTED_EDGE('',*,*,#47079,.T.);
#68811=ORIENTED_EDGE('',*,*,#47081,.T.);
#68812=ORIENTED_EDGE('',*,*,#47084,.T.);
#68813=ORIENTED_EDGE('',*,*,#47088,.T.);
#68814=ORIENTED_EDGE('',*,*,#47091,.T.);
#68815=ORIENTED_EDGE('',*,*,#47093,.T.);
#68816=ORIENTED_EDGE('',*,*,#47096,.T.);
#68817=ORIENTED_EDGE('',*,*,#47100,.T.);
#68818=ORIENTED_EDGE('',*,*,#47103,.T.);
#68819=ORIENTED_EDGE('',*,*,#47105,.T.);
#68820=ORIENTED_EDGE('',*,*,#47108,.T.);
#68821=ORIENTED_EDGE('',*,*,#47112,.T.);
#68822=ORIENTED_EDGE('',*,*,#47115,.T.);
#68823=ORIENTED_EDGE('',*,*,#47117,.T.);
#68824=ORIENTED_EDGE('',*,*,#47120,.T.);
#68825=ORIENTED_EDGE('',*,*,#47124,.T.);
#68826=ORIENTED_EDGE('',*,*,#47127,.T.);
#68827=ORIENTED_EDGE('',*,*,#47129,.T.);
#68828=ORIENTED_EDGE('',*,*,#47132,.T.);
#68829=ORIENTED_EDGE('',*,*,#47136,.T.);
#68830=ORIENTED_EDGE('',*,*,#47139,.T.);
#68831=ORIENTED_EDGE('',*,*,#47141,.T.);
#68832=ORIENTED_EDGE('',*,*,#47144,.T.);
#68833=ORIENTED_EDGE('',*,*,#47148,.T.);
#68834=ORIENTED_EDGE('',*,*,#47151,.T.);
#68835=ORIENTED_EDGE('',*,*,#47153,.T.);
#68836=ORIENTED_EDGE('',*,*,#47156,.T.);
#68837=ORIENTED_EDGE('',*,*,#47160,.T.);
#68838=ORIENTED_EDGE('',*,*,#47163,.T.);
#68839=ORIENTED_EDGE('',*,*,#47165,.T.);
#68840=ORIENTED_EDGE('',*,*,#47168,.T.);
#68841=ORIENTED_EDGE('',*,*,#47172,.T.);
#68842=ORIENTED_EDGE('',*,*,#47175,.T.);
#68843=ORIENTED_EDGE('',*,*,#47177,.T.);
#68844=ORIENTED_EDGE('',*,*,#47180,.T.);
#68845=ORIENTED_EDGE('',*,*,#47184,.T.);
#68846=ORIENTED_EDGE('',*,*,#47187,.T.);
#68847=ORIENTED_EDGE('',*,*,#47189,.T.);
#68848=ORIENTED_EDGE('',*,*,#47192,.T.);
#68849=ORIENTED_EDGE('',*,*,#47196,.T.);
#68850=ORIENTED_EDGE('',*,*,#47199,.T.);
#68851=ORIENTED_EDGE('',*,*,#47201,.T.);
#68852=ORIENTED_EDGE('',*,*,#47204,.T.);
#68853=ORIENTED_EDGE('',*,*,#47208,.T.);
#68854=ORIENTED_EDGE('',*,*,#47211,.T.);
#68855=ORIENTED_EDGE('',*,*,#47213,.T.);
#68856=ORIENTED_EDGE('',*,*,#47216,.T.);
#68857=ORIENTED_EDGE('',*,*,#47220,.T.);
#68858=ORIENTED_EDGE('',*,*,#47223,.T.);
#68859=ORIENTED_EDGE('',*,*,#47225,.T.);
#68860=ORIENTED_EDGE('',*,*,#47228,.T.);
#68861=ORIENTED_EDGE('',*,*,#47232,.T.);
#68862=ORIENTED_EDGE('',*,*,#47235,.T.);
#68863=ORIENTED_EDGE('',*,*,#47237,.T.);
#68864=ORIENTED_EDGE('',*,*,#47240,.T.);
#68865=ORIENTED_EDGE('',*,*,#47244,.T.);
#68866=ORIENTED_EDGE('',*,*,#47247,.T.);
#68867=ORIENTED_EDGE('',*,*,#47249,.T.);
#68868=ORIENTED_EDGE('',*,*,#47252,.T.);
#68869=ORIENTED_EDGE('',*,*,#47256,.T.);
#68870=ORIENTED_EDGE('',*,*,#47259,.T.);
#68871=ORIENTED_EDGE('',*,*,#47261,.T.);
#68872=ORIENTED_EDGE('',*,*,#47264,.T.);
#68873=ORIENTED_EDGE('',*,*,#47268,.T.);
#68874=ORIENTED_EDGE('',*,*,#47271,.T.);
#68875=ORIENTED_EDGE('',*,*,#47273,.T.);
#68876=ORIENTED_EDGE('',*,*,#47276,.T.);
#68877=ORIENTED_EDGE('',*,*,#47280,.T.);
#68878=ORIENTED_EDGE('',*,*,#47283,.T.);
#68879=ORIENTED_EDGE('',*,*,#47285,.T.);
#68880=ORIENTED_EDGE('',*,*,#47288,.T.);
#68881=ORIENTED_EDGE('',*,*,#47292,.T.);
#68882=ORIENTED_EDGE('',*,*,#47295,.T.);
#68883=ORIENTED_EDGE('',*,*,#47297,.T.);
#68884=ORIENTED_EDGE('',*,*,#47300,.T.);
#68885=ORIENTED_EDGE('',*,*,#47304,.T.);
#68886=ORIENTED_EDGE('',*,*,#47307,.T.);
#68887=ORIENTED_EDGE('',*,*,#47309,.T.);
#68888=ORIENTED_EDGE('',*,*,#47312,.T.);
#68889=ORIENTED_EDGE('',*,*,#47316,.T.);
#68890=ORIENTED_EDGE('',*,*,#47319,.T.);
#68891=ORIENTED_EDGE('',*,*,#47321,.T.);
#68892=ORIENTED_EDGE('',*,*,#47324,.T.);
#68893=ORIENTED_EDGE('',*,*,#47328,.T.);
#68894=ORIENTED_EDGE('',*,*,#47331,.T.);
#68895=ORIENTED_EDGE('',*,*,#47333,.T.);
#68896=ORIENTED_EDGE('',*,*,#47336,.T.);
#68897=ORIENTED_EDGE('',*,*,#47340,.T.);
#68898=ORIENTED_EDGE('',*,*,#47343,.T.);
#68899=ORIENTED_EDGE('',*,*,#47345,.T.);
#68900=ORIENTED_EDGE('',*,*,#47348,.T.);
#68901=ORIENTED_EDGE('',*,*,#47352,.T.);
#68902=ORIENTED_EDGE('',*,*,#47355,.T.);
#68903=ORIENTED_EDGE('',*,*,#47357,.T.);
#68904=ORIENTED_EDGE('',*,*,#47360,.T.);
#68905=ORIENTED_EDGE('',*,*,#47364,.T.);
#68906=ORIENTED_EDGE('',*,*,#47367,.T.);
#68907=ORIENTED_EDGE('',*,*,#47369,.T.);
#68908=ORIENTED_EDGE('',*,*,#47372,.T.);
#68909=ORIENTED_EDGE('',*,*,#47376,.T.);
#68910=ORIENTED_EDGE('',*,*,#47379,.T.);
#68911=ORIENTED_EDGE('',*,*,#47381,.T.);
#68912=ORIENTED_EDGE('',*,*,#47384,.T.);
#68913=ORIENTED_EDGE('',*,*,#47388,.T.);
#68914=ORIENTED_EDGE('',*,*,#47391,.T.);
#68915=ORIENTED_EDGE('',*,*,#47393,.T.);
#68916=ORIENTED_EDGE('',*,*,#47396,.T.);
#68917=ORIENTED_EDGE('',*,*,#47400,.T.);
#68918=ORIENTED_EDGE('',*,*,#47403,.T.);
#68919=ORIENTED_EDGE('',*,*,#47405,.T.);
#68920=ORIENTED_EDGE('',*,*,#47408,.T.);
#68921=ORIENTED_EDGE('',*,*,#47412,.T.);
#68922=ORIENTED_EDGE('',*,*,#47415,.T.);
#68923=ORIENTED_EDGE('',*,*,#47417,.T.);
#68924=ORIENTED_EDGE('',*,*,#47420,.T.);
#68925=ORIENTED_EDGE('',*,*,#47424,.T.);
#68926=ORIENTED_EDGE('',*,*,#47427,.T.);
#68927=ORIENTED_EDGE('',*,*,#47429,.T.);
#68928=ORIENTED_EDGE('',*,*,#47432,.T.);
#68929=ORIENTED_EDGE('',*,*,#47436,.T.);
#68930=ORIENTED_EDGE('',*,*,#47439,.T.);
#68931=ORIENTED_EDGE('',*,*,#47441,.T.);
#68932=ORIENTED_EDGE('',*,*,#47444,.T.);
#68933=ORIENTED_EDGE('',*,*,#47448,.T.);
#68934=ORIENTED_EDGE('',*,*,#47451,.T.);
#68935=ORIENTED_EDGE('',*,*,#47453,.T.);
#68936=ORIENTED_EDGE('',*,*,#47456,.T.);
#68937=ORIENTED_EDGE('',*,*,#47460,.T.);
#68938=ORIENTED_EDGE('',*,*,#47463,.T.);
#68939=ORIENTED_EDGE('',*,*,#47465,.T.);
#68940=ORIENTED_EDGE('',*,*,#47468,.T.);
#68941=ORIENTED_EDGE('',*,*,#47472,.T.);
#68942=ORIENTED_EDGE('',*,*,#47475,.T.);
#68943=ORIENTED_EDGE('',*,*,#47477,.T.);
#68944=ORIENTED_EDGE('',*,*,#47480,.T.);
#68945=ORIENTED_EDGE('',*,*,#47484,.T.);
#68946=ORIENTED_EDGE('',*,*,#47487,.T.);
#68947=ORIENTED_EDGE('',*,*,#47489,.T.);
#68948=ORIENTED_EDGE('',*,*,#47492,.T.);
#68949=ORIENTED_EDGE('',*,*,#47496,.T.);
#68950=ORIENTED_EDGE('',*,*,#47499,.T.);
#68951=ORIENTED_EDGE('',*,*,#47501,.T.);
#68952=ORIENTED_EDGE('',*,*,#47504,.T.);
#68953=ORIENTED_EDGE('',*,*,#47508,.T.);
#68954=ORIENTED_EDGE('',*,*,#47511,.T.);
#68955=ORIENTED_EDGE('',*,*,#47513,.T.);
#68956=ORIENTED_EDGE('',*,*,#47516,.T.);
#68957=ORIENTED_EDGE('',*,*,#47520,.T.);
#68958=ORIENTED_EDGE('',*,*,#47523,.T.);
#68959=ORIENTED_EDGE('',*,*,#47525,.T.);
#68960=ORIENTED_EDGE('',*,*,#47528,.T.);
#68961=ORIENTED_EDGE('',*,*,#47532,.T.);
#68962=ORIENTED_EDGE('',*,*,#47535,.T.);
#68963=ORIENTED_EDGE('',*,*,#47537,.T.);
#68964=ORIENTED_EDGE('',*,*,#47540,.T.);
#68965=ORIENTED_EDGE('',*,*,#47544,.T.);
#68966=ORIENTED_EDGE('',*,*,#47547,.T.);
#68967=ORIENTED_EDGE('',*,*,#47549,.T.);
#68968=ORIENTED_EDGE('',*,*,#47552,.T.);
#68969=ORIENTED_EDGE('',*,*,#47556,.T.);
#68970=ORIENTED_EDGE('',*,*,#47559,.T.);
#68971=ORIENTED_EDGE('',*,*,#47561,.T.);
#68972=ORIENTED_EDGE('',*,*,#47564,.T.);
#68973=ORIENTED_EDGE('',*,*,#47568,.T.);
#68974=ORIENTED_EDGE('',*,*,#47571,.T.);
#68975=ORIENTED_EDGE('',*,*,#47573,.T.);
#68976=ORIENTED_EDGE('',*,*,#47576,.T.);
#68977=ORIENTED_EDGE('',*,*,#47580,.T.);
#68978=ORIENTED_EDGE('',*,*,#47583,.T.);
#68979=ORIENTED_EDGE('',*,*,#47585,.T.);
#68980=ORIENTED_EDGE('',*,*,#47588,.T.);
#68981=ORIENTED_EDGE('',*,*,#47592,.T.);
#68982=ORIENTED_EDGE('',*,*,#47595,.T.);
#68983=ORIENTED_EDGE('',*,*,#47597,.T.);
#68984=ORIENTED_EDGE('',*,*,#47600,.T.);
#68985=ORIENTED_EDGE('',*,*,#47604,.T.);
#68986=ORIENTED_EDGE('',*,*,#47607,.T.);
#68987=ORIENTED_EDGE('',*,*,#47609,.T.);
#68988=ORIENTED_EDGE('',*,*,#47612,.T.);
#68989=ORIENTED_EDGE('',*,*,#47616,.T.);
#68990=ORIENTED_EDGE('',*,*,#47619,.T.);
#68991=ORIENTED_EDGE('',*,*,#47621,.T.);
#68992=ORIENTED_EDGE('',*,*,#47624,.T.);
#68993=ORIENTED_EDGE('',*,*,#47628,.T.);
#68994=ORIENTED_EDGE('',*,*,#47631,.T.);
#68995=ORIENTED_EDGE('',*,*,#47633,.T.);
#68996=ORIENTED_EDGE('',*,*,#47636,.T.);
#68997=ORIENTED_EDGE('',*,*,#47640,.T.);
#68998=ORIENTED_EDGE('',*,*,#47643,.T.);
#68999=ORIENTED_EDGE('',*,*,#47645,.T.);
#69000=ORIENTED_EDGE('',*,*,#47648,.T.);
#69001=ORIENTED_EDGE('',*,*,#47652,.T.);
#69002=ORIENTED_EDGE('',*,*,#47655,.T.);
#69003=ORIENTED_EDGE('',*,*,#47657,.T.);
#69004=ORIENTED_EDGE('',*,*,#47660,.T.);
#69005=ORIENTED_EDGE('',*,*,#47664,.T.);
#69006=ORIENTED_EDGE('',*,*,#47667,.T.);
#69007=ORIENTED_EDGE('',*,*,#47669,.T.);
#69008=ORIENTED_EDGE('',*,*,#47672,.T.);
#69009=ORIENTED_EDGE('',*,*,#47676,.T.);
#69010=ORIENTED_EDGE('',*,*,#47679,.T.);
#69011=ORIENTED_EDGE('',*,*,#47681,.T.);
#69012=ORIENTED_EDGE('',*,*,#47684,.T.);
#69013=ORIENTED_EDGE('',*,*,#47688,.T.);
#69014=ORIENTED_EDGE('',*,*,#47691,.T.);
#69015=ORIENTED_EDGE('',*,*,#47693,.T.);
#69016=ORIENTED_EDGE('',*,*,#47696,.T.);
#69017=ORIENTED_EDGE('',*,*,#47700,.T.);
#69018=ORIENTED_EDGE('',*,*,#47703,.T.);
#69019=ORIENTED_EDGE('',*,*,#47705,.T.);
#69020=ORIENTED_EDGE('',*,*,#47708,.T.);
#69021=ORIENTED_EDGE('',*,*,#47712,.T.);
#69022=ORIENTED_EDGE('',*,*,#47715,.T.);
#69023=ORIENTED_EDGE('',*,*,#47717,.T.);
#69024=ORIENTED_EDGE('',*,*,#47720,.T.);
#69025=ORIENTED_EDGE('',*,*,#47724,.T.);
#69026=ORIENTED_EDGE('',*,*,#47727,.T.);
#69027=ORIENTED_EDGE('',*,*,#47729,.T.);
#69028=ORIENTED_EDGE('',*,*,#47732,.T.);
#69029=ORIENTED_EDGE('',*,*,#47736,.T.);
#69030=ORIENTED_EDGE('',*,*,#47739,.T.);
#69031=ORIENTED_EDGE('',*,*,#47741,.T.);
#69032=ORIENTED_EDGE('',*,*,#47744,.T.);
#69033=ORIENTED_EDGE('',*,*,#47748,.T.);
#69034=ORIENTED_EDGE('',*,*,#47751,.T.);
#69035=ORIENTED_EDGE('',*,*,#47753,.T.);
#69036=ORIENTED_EDGE('',*,*,#47756,.T.);
#69037=ORIENTED_EDGE('',*,*,#47760,.T.);
#69038=ORIENTED_EDGE('',*,*,#47763,.T.);
#69039=ORIENTED_EDGE('',*,*,#47765,.T.);
#69040=ORIENTED_EDGE('',*,*,#47768,.T.);
#69041=ORIENTED_EDGE('',*,*,#47772,.T.);
#69042=ORIENTED_EDGE('',*,*,#47775,.T.);
#69043=ORIENTED_EDGE('',*,*,#47777,.T.);
#69044=ORIENTED_EDGE('',*,*,#47780,.T.);
#69045=ORIENTED_EDGE('',*,*,#47784,.T.);
#69046=ORIENTED_EDGE('',*,*,#47787,.T.);
#69047=ORIENTED_EDGE('',*,*,#47789,.T.);
#69048=ORIENTED_EDGE('',*,*,#47792,.T.);
#69049=ORIENTED_EDGE('',*,*,#47796,.T.);
#69050=ORIENTED_EDGE('',*,*,#47799,.T.);
#69051=ORIENTED_EDGE('',*,*,#47801,.T.);
#69052=ORIENTED_EDGE('',*,*,#47804,.T.);
#69053=ORIENTED_EDGE('',*,*,#47808,.T.);
#69054=ORIENTED_EDGE('',*,*,#47811,.T.);
#69055=ORIENTED_EDGE('',*,*,#47813,.T.);
#69056=ORIENTED_EDGE('',*,*,#47816,.T.);
#69057=ORIENTED_EDGE('',*,*,#47820,.T.);
#69058=ORIENTED_EDGE('',*,*,#47823,.T.);
#69059=ORIENTED_EDGE('',*,*,#47825,.T.);
#69060=ORIENTED_EDGE('',*,*,#47828,.T.);
#69061=ORIENTED_EDGE('',*,*,#47832,.T.);
#69062=ORIENTED_EDGE('',*,*,#47835,.T.);
#69063=ORIENTED_EDGE('',*,*,#47837,.T.);
#69064=ORIENTED_EDGE('',*,*,#47840,.T.);
#69065=ORIENTED_EDGE('',*,*,#47844,.T.);
#69066=ORIENTED_EDGE('',*,*,#47847,.T.);
#69067=ORIENTED_EDGE('',*,*,#47849,.T.);
#69068=ORIENTED_EDGE('',*,*,#47852,.T.);
#69069=ORIENTED_EDGE('',*,*,#47856,.T.);
#69070=ORIENTED_EDGE('',*,*,#47859,.T.);
#69071=ORIENTED_EDGE('',*,*,#47861,.T.);
#69072=ORIENTED_EDGE('',*,*,#47864,.T.);
#69073=ORIENTED_EDGE('',*,*,#47868,.T.);
#69074=ORIENTED_EDGE('',*,*,#47871,.T.);
#69075=ORIENTED_EDGE('',*,*,#47873,.T.);
#69076=ORIENTED_EDGE('',*,*,#47876,.T.);
#69077=ORIENTED_EDGE('',*,*,#47880,.T.);
#69078=ORIENTED_EDGE('',*,*,#47883,.T.);
#69079=ORIENTED_EDGE('',*,*,#47885,.T.);
#69080=ORIENTED_EDGE('',*,*,#47888,.T.);
#69081=ORIENTED_EDGE('',*,*,#47892,.T.);
#69082=ORIENTED_EDGE('',*,*,#47895,.T.);
#69083=ORIENTED_EDGE('',*,*,#47897,.T.);
#69084=ORIENTED_EDGE('',*,*,#47900,.T.);
#69085=ORIENTED_EDGE('',*,*,#47904,.T.);
#69086=ORIENTED_EDGE('',*,*,#47907,.T.);
#69087=ORIENTED_EDGE('',*,*,#47909,.T.);
#69088=ORIENTED_EDGE('',*,*,#47912,.T.);
#69089=ORIENTED_EDGE('',*,*,#47916,.T.);
#69090=ORIENTED_EDGE('',*,*,#47919,.T.);
#69091=ORIENTED_EDGE('',*,*,#47921,.T.);
#69092=ORIENTED_EDGE('',*,*,#47924,.T.);
#69093=ORIENTED_EDGE('',*,*,#47928,.T.);
#69094=ORIENTED_EDGE('',*,*,#47931,.T.);
#69095=ORIENTED_EDGE('',*,*,#47933,.T.);
#69096=ORIENTED_EDGE('',*,*,#47936,.T.);
#69097=ORIENTED_EDGE('',*,*,#47940,.T.);
#69098=ORIENTED_EDGE('',*,*,#47943,.T.);
#69099=ORIENTED_EDGE('',*,*,#47945,.T.);
#69100=ORIENTED_EDGE('',*,*,#47948,.T.);
#69101=ORIENTED_EDGE('',*,*,#47952,.T.);
#69102=ORIENTED_EDGE('',*,*,#47955,.T.);
#69103=ORIENTED_EDGE('',*,*,#47957,.T.);
#69104=ORIENTED_EDGE('',*,*,#47960,.T.);
#69105=ORIENTED_EDGE('',*,*,#47964,.T.);
#69106=ORIENTED_EDGE('',*,*,#47967,.T.);
#69107=ORIENTED_EDGE('',*,*,#47969,.T.);
#69108=ORIENTED_EDGE('',*,*,#47972,.T.);
#69109=ORIENTED_EDGE('',*,*,#47976,.T.);
#69110=ORIENTED_EDGE('',*,*,#47979,.T.);
#69111=ORIENTED_EDGE('',*,*,#47981,.T.);
#69112=ORIENTED_EDGE('',*,*,#47984,.T.);
#69113=ORIENTED_EDGE('',*,*,#47988,.T.);
#69114=ORIENTED_EDGE('',*,*,#47991,.T.);
#69115=ORIENTED_EDGE('',*,*,#47993,.T.);
#69116=ORIENTED_EDGE('',*,*,#47996,.T.);
#69117=ORIENTED_EDGE('',*,*,#48000,.T.);
#69118=ORIENTED_EDGE('',*,*,#48003,.T.);
#69119=ORIENTED_EDGE('',*,*,#48005,.T.);
#69120=ORIENTED_EDGE('',*,*,#48008,.T.);
#69121=ORIENTED_EDGE('',*,*,#48012,.T.);
#69122=ORIENTED_EDGE('',*,*,#48015,.T.);
#69123=ORIENTED_EDGE('',*,*,#48017,.T.);
#69124=ORIENTED_EDGE('',*,*,#48020,.T.);
#69125=ORIENTED_EDGE('',*,*,#48024,.T.);
#69126=ORIENTED_EDGE('',*,*,#48027,.T.);
#69127=ORIENTED_EDGE('',*,*,#48029,.T.);
#69128=ORIENTED_EDGE('',*,*,#48032,.T.);
#69129=ORIENTED_EDGE('',*,*,#48036,.T.);
#69130=ORIENTED_EDGE('',*,*,#48039,.T.);
#69131=ORIENTED_EDGE('',*,*,#48041,.T.);
#69132=ORIENTED_EDGE('',*,*,#48044,.T.);
#69133=ORIENTED_EDGE('',*,*,#48048,.T.);
#69134=ORIENTED_EDGE('',*,*,#48051,.T.);
#69135=ORIENTED_EDGE('',*,*,#48053,.T.);
#69136=ORIENTED_EDGE('',*,*,#48056,.T.);
#69137=ORIENTED_EDGE('',*,*,#48060,.T.);
#69138=ORIENTED_EDGE('',*,*,#48063,.T.);
#69139=ORIENTED_EDGE('',*,*,#48065,.T.);
#69140=ORIENTED_EDGE('',*,*,#48068,.T.);
#69141=ORIENTED_EDGE('',*,*,#48072,.T.);
#69142=ORIENTED_EDGE('',*,*,#48075,.T.);
#69143=ORIENTED_EDGE('',*,*,#48077,.T.);
#69144=ORIENTED_EDGE('',*,*,#48080,.T.);
#69145=ORIENTED_EDGE('',*,*,#48084,.T.);
#69146=ORIENTED_EDGE('',*,*,#48087,.T.);
#69147=ORIENTED_EDGE('',*,*,#48089,.T.);
#69148=ORIENTED_EDGE('',*,*,#48092,.T.);
#69149=ORIENTED_EDGE('',*,*,#48096,.T.);
#69150=ORIENTED_EDGE('',*,*,#48099,.T.);
#69151=ORIENTED_EDGE('',*,*,#48101,.T.);
#69152=ORIENTED_EDGE('',*,*,#48104,.T.);
#69153=ORIENTED_EDGE('',*,*,#48108,.T.);
#69154=ORIENTED_EDGE('',*,*,#48111,.T.);
#69155=ORIENTED_EDGE('',*,*,#48113,.T.);
#69156=ORIENTED_EDGE('',*,*,#48116,.T.);
#69157=ORIENTED_EDGE('',*,*,#48120,.T.);
#69158=ORIENTED_EDGE('',*,*,#48123,.T.);
#69159=ORIENTED_EDGE('',*,*,#48125,.T.);
#69160=ORIENTED_EDGE('',*,*,#48128,.T.);
#69161=ORIENTED_EDGE('',*,*,#48132,.T.);
#69162=ORIENTED_EDGE('',*,*,#48135,.T.);
#69163=ORIENTED_EDGE('',*,*,#48137,.T.);
#69164=ORIENTED_EDGE('',*,*,#48140,.T.);
#69165=ORIENTED_EDGE('',*,*,#48144,.T.);
#69166=ORIENTED_EDGE('',*,*,#48147,.T.);
#69167=ORIENTED_EDGE('',*,*,#48149,.T.);
#69168=ORIENTED_EDGE('',*,*,#48152,.T.);
#69169=ORIENTED_EDGE('',*,*,#48156,.T.);
#69170=ORIENTED_EDGE('',*,*,#48159,.T.);
#69171=ORIENTED_EDGE('',*,*,#48161,.T.);
#69172=ORIENTED_EDGE('',*,*,#48164,.T.);
#69173=ORIENTED_EDGE('',*,*,#48168,.T.);
#69174=ORIENTED_EDGE('',*,*,#48171,.T.);
#69175=ORIENTED_EDGE('',*,*,#48173,.T.);
#69176=ORIENTED_EDGE('',*,*,#48176,.T.);
#69177=ORIENTED_EDGE('',*,*,#48180,.T.);
#69178=ORIENTED_EDGE('',*,*,#48183,.T.);
#69179=ORIENTED_EDGE('',*,*,#48185,.T.);
#69180=ORIENTED_EDGE('',*,*,#48188,.T.);
#69181=ORIENTED_EDGE('',*,*,#48192,.T.);
#69182=ORIENTED_EDGE('',*,*,#48195,.T.);
#69183=ORIENTED_EDGE('',*,*,#48197,.T.);
#69184=ORIENTED_EDGE('',*,*,#48200,.T.);
#69185=ORIENTED_EDGE('',*,*,#48204,.T.);
#69186=ORIENTED_EDGE('',*,*,#48207,.T.);
#69187=ORIENTED_EDGE('',*,*,#48209,.T.);
#69188=ORIENTED_EDGE('',*,*,#48212,.T.);
#69189=ORIENTED_EDGE('',*,*,#48216,.T.);
#69190=ORIENTED_EDGE('',*,*,#48219,.T.);
#69191=ORIENTED_EDGE('',*,*,#48221,.T.);
#69192=ORIENTED_EDGE('',*,*,#48224,.T.);
#69193=ORIENTED_EDGE('',*,*,#48228,.T.);
#69194=ORIENTED_EDGE('',*,*,#48231,.T.);
#69195=ORIENTED_EDGE('',*,*,#48233,.T.);
#69196=ORIENTED_EDGE('',*,*,#48236,.T.);
#69197=ORIENTED_EDGE('',*,*,#48240,.T.);
#69198=ORIENTED_EDGE('',*,*,#48243,.T.);
#69199=ORIENTED_EDGE('',*,*,#48245,.T.);
#69200=ORIENTED_EDGE('',*,*,#48248,.T.);
#69201=ORIENTED_EDGE('',*,*,#48252,.T.);
#69202=ORIENTED_EDGE('',*,*,#48255,.T.);
#69203=ORIENTED_EDGE('',*,*,#48257,.T.);
#69204=ORIENTED_EDGE('',*,*,#48260,.T.);
#69205=ORIENTED_EDGE('',*,*,#48264,.T.);
#69206=ORIENTED_EDGE('',*,*,#48267,.T.);
#69207=ORIENTED_EDGE('',*,*,#48269,.T.);
#69208=ORIENTED_EDGE('',*,*,#48272,.T.);
#69209=ORIENTED_EDGE('',*,*,#48276,.T.);
#69210=ORIENTED_EDGE('',*,*,#48279,.T.);
#69211=ORIENTED_EDGE('',*,*,#48281,.T.);
#69212=ORIENTED_EDGE('',*,*,#48284,.T.);
#69213=ORIENTED_EDGE('',*,*,#48288,.T.);
#69214=ORIENTED_EDGE('',*,*,#48291,.T.);
#69215=ORIENTED_EDGE('',*,*,#48293,.T.);
#69216=ORIENTED_EDGE('',*,*,#48296,.T.);
#69217=ORIENTED_EDGE('',*,*,#48300,.T.);
#69218=ORIENTED_EDGE('',*,*,#48303,.T.);
#69219=ORIENTED_EDGE('',*,*,#48305,.T.);
#69220=ORIENTED_EDGE('',*,*,#48308,.T.);
#69221=ORIENTED_EDGE('',*,*,#48312,.T.);
#69222=ORIENTED_EDGE('',*,*,#48315,.T.);
#69223=ORIENTED_EDGE('',*,*,#48317,.T.);
#69224=ORIENTED_EDGE('',*,*,#48320,.T.);
#69225=ORIENTED_EDGE('',*,*,#48324,.T.);
#69226=ORIENTED_EDGE('',*,*,#48327,.T.);
#69227=ORIENTED_EDGE('',*,*,#48329,.T.);
#69228=ORIENTED_EDGE('',*,*,#48332,.T.);
#69229=ORIENTED_EDGE('',*,*,#48336,.T.);
#69230=ORIENTED_EDGE('',*,*,#48339,.T.);
#69231=ORIENTED_EDGE('',*,*,#48341,.T.);
#69232=ORIENTED_EDGE('',*,*,#48344,.T.);
#69233=ORIENTED_EDGE('',*,*,#48348,.T.);
#69234=ORIENTED_EDGE('',*,*,#48351,.T.);
#69235=ORIENTED_EDGE('',*,*,#48353,.T.);
#69236=ORIENTED_EDGE('',*,*,#48356,.T.);
#69237=ORIENTED_EDGE('',*,*,#48360,.T.);
#69238=ORIENTED_EDGE('',*,*,#48363,.T.);
#69239=ORIENTED_EDGE('',*,*,#48365,.T.);
#69240=ORIENTED_EDGE('',*,*,#48368,.T.);
#69241=ORIENTED_EDGE('',*,*,#48372,.T.);
#69242=ORIENTED_EDGE('',*,*,#48375,.T.);
#69243=ORIENTED_EDGE('',*,*,#48377,.T.);
#69244=ORIENTED_EDGE('',*,*,#48380,.T.);
#69245=ORIENTED_EDGE('',*,*,#48384,.T.);
#69246=ORIENTED_EDGE('',*,*,#48387,.T.);
#69247=ORIENTED_EDGE('',*,*,#48389,.T.);
#69248=ORIENTED_EDGE('',*,*,#48392,.T.);
#69249=ORIENTED_EDGE('',*,*,#48396,.T.);
#69250=ORIENTED_EDGE('',*,*,#48399,.T.);
#69251=ORIENTED_EDGE('',*,*,#48401,.T.);
#69252=ORIENTED_EDGE('',*,*,#48404,.T.);
#69253=ORIENTED_EDGE('',*,*,#48408,.T.);
#69254=ORIENTED_EDGE('',*,*,#48411,.T.);
#69255=ORIENTED_EDGE('',*,*,#48413,.T.);
#69256=ORIENTED_EDGE('',*,*,#48416,.T.);
#69257=ORIENTED_EDGE('',*,*,#48420,.T.);
#69258=ORIENTED_EDGE('',*,*,#48423,.T.);
#69259=ORIENTED_EDGE('',*,*,#48425,.T.);
#69260=ORIENTED_EDGE('',*,*,#48428,.T.);
#69261=ORIENTED_EDGE('',*,*,#48432,.T.);
#69262=ORIENTED_EDGE('',*,*,#48435,.T.);
#69263=ORIENTED_EDGE('',*,*,#48437,.T.);
#69264=ORIENTED_EDGE('',*,*,#48440,.T.);
#69265=ORIENTED_EDGE('',*,*,#48444,.T.);
#69266=ORIENTED_EDGE('',*,*,#48447,.T.);
#69267=ORIENTED_EDGE('',*,*,#48449,.T.);
#69268=ORIENTED_EDGE('',*,*,#48452,.T.);
#69269=ORIENTED_EDGE('',*,*,#48456,.T.);
#69270=ORIENTED_EDGE('',*,*,#48459,.T.);
#69271=ORIENTED_EDGE('',*,*,#48461,.T.);
#69272=ORIENTED_EDGE('',*,*,#48464,.T.);
#69273=ORIENTED_EDGE('',*,*,#48468,.T.);
#69274=ORIENTED_EDGE('',*,*,#48471,.T.);
#69275=ORIENTED_EDGE('',*,*,#48473,.T.);
#69276=ORIENTED_EDGE('',*,*,#48476,.T.);
#69277=ORIENTED_EDGE('',*,*,#48480,.T.);
#69278=ORIENTED_EDGE('',*,*,#48483,.T.);
#69279=ORIENTED_EDGE('',*,*,#48485,.T.);
#69280=ORIENTED_EDGE('',*,*,#48488,.T.);
#69281=ORIENTED_EDGE('',*,*,#48492,.T.);
#69282=ORIENTED_EDGE('',*,*,#48495,.T.);
#69283=ORIENTED_EDGE('',*,*,#48497,.T.);
#69284=ORIENTED_EDGE('',*,*,#48500,.T.);
#69285=ORIENTED_EDGE('',*,*,#48504,.T.);
#69286=ORIENTED_EDGE('',*,*,#48507,.T.);
#69287=ORIENTED_EDGE('',*,*,#48509,.T.);
#69288=ORIENTED_EDGE('',*,*,#48512,.T.);
#69289=ORIENTED_EDGE('',*,*,#48516,.T.);
#69290=ORIENTED_EDGE('',*,*,#48519,.T.);
#69291=ORIENTED_EDGE('',*,*,#48521,.T.);
#69292=ORIENTED_EDGE('',*,*,#48524,.T.);
#69293=ORIENTED_EDGE('',*,*,#48528,.T.);
#69294=ORIENTED_EDGE('',*,*,#48531,.T.);
#69295=ORIENTED_EDGE('',*,*,#48533,.T.);
#69296=ORIENTED_EDGE('',*,*,#48536,.T.);
#69297=ORIENTED_EDGE('',*,*,#48540,.T.);
#69298=ORIENTED_EDGE('',*,*,#48543,.T.);
#69299=ORIENTED_EDGE('',*,*,#48545,.T.);
#69300=ORIENTED_EDGE('',*,*,#48548,.T.);
#69301=ORIENTED_EDGE('',*,*,#48552,.T.);
#69302=ORIENTED_EDGE('',*,*,#48555,.T.);
#69303=ORIENTED_EDGE('',*,*,#48557,.T.);
#69304=ORIENTED_EDGE('',*,*,#48560,.T.);
#69305=ORIENTED_EDGE('',*,*,#48564,.T.);
#69306=ORIENTED_EDGE('',*,*,#48567,.T.);
#69307=ORIENTED_EDGE('',*,*,#48569,.T.);
#69308=ORIENTED_EDGE('',*,*,#48572,.T.);
#69309=ORIENTED_EDGE('',*,*,#48576,.T.);
#69310=ORIENTED_EDGE('',*,*,#48579,.T.);
#69311=ORIENTED_EDGE('',*,*,#48581,.T.);
#69312=ORIENTED_EDGE('',*,*,#48584,.T.);
#69313=ORIENTED_EDGE('',*,*,#48588,.T.);
#69314=ORIENTED_EDGE('',*,*,#48591,.T.);
#69315=ORIENTED_EDGE('',*,*,#48593,.T.);
#69316=ORIENTED_EDGE('',*,*,#48596,.T.);
#69317=ORIENTED_EDGE('',*,*,#48600,.T.);
#69318=ORIENTED_EDGE('',*,*,#48603,.T.);
#69319=ORIENTED_EDGE('',*,*,#48605,.T.);
#69320=ORIENTED_EDGE('',*,*,#48608,.T.);
#69321=ORIENTED_EDGE('',*,*,#48612,.T.);
#69322=ORIENTED_EDGE('',*,*,#48615,.T.);
#69323=ORIENTED_EDGE('',*,*,#48617,.T.);
#69324=ORIENTED_EDGE('',*,*,#48620,.T.);
#69325=ORIENTED_EDGE('',*,*,#48624,.T.);
#69326=ORIENTED_EDGE('',*,*,#48627,.T.);
#69327=ORIENTED_EDGE('',*,*,#48629,.T.);
#69328=ORIENTED_EDGE('',*,*,#48632,.T.);
#69329=ORIENTED_EDGE('',*,*,#48636,.T.);
#69330=ORIENTED_EDGE('',*,*,#48639,.T.);
#69331=ORIENTED_EDGE('',*,*,#48641,.T.);
#69332=ORIENTED_EDGE('',*,*,#48644,.T.);
#69333=ORIENTED_EDGE('',*,*,#48648,.T.);
#69334=ORIENTED_EDGE('',*,*,#48651,.T.);
#69335=ORIENTED_EDGE('',*,*,#48653,.T.);
#69336=ORIENTED_EDGE('',*,*,#48656,.T.);
#69337=ORIENTED_EDGE('',*,*,#48660,.T.);
#69338=ORIENTED_EDGE('',*,*,#48663,.T.);
#69339=ORIENTED_EDGE('',*,*,#48665,.T.);
#69340=ORIENTED_EDGE('',*,*,#48668,.T.);
#69341=ORIENTED_EDGE('',*,*,#48672,.T.);
#69342=ORIENTED_EDGE('',*,*,#48675,.T.);
#69343=ORIENTED_EDGE('',*,*,#48677,.T.);
#69344=ORIENTED_EDGE('',*,*,#48680,.T.);
#69345=ORIENTED_EDGE('',*,*,#48684,.T.);
#69346=ORIENTED_EDGE('',*,*,#48687,.T.);
#69347=ORIENTED_EDGE('',*,*,#48689,.T.);
#69348=ORIENTED_EDGE('',*,*,#48692,.T.);
#69349=ORIENTED_EDGE('',*,*,#48696,.T.);
#69350=ORIENTED_EDGE('',*,*,#48699,.T.);
#69351=ORIENTED_EDGE('',*,*,#48701,.T.);
#69352=ORIENTED_EDGE('',*,*,#48704,.T.);
#69353=ORIENTED_EDGE('',*,*,#48708,.T.);
#69354=ORIENTED_EDGE('',*,*,#48711,.T.);
#69355=ORIENTED_EDGE('',*,*,#48713,.T.);
#69356=ORIENTED_EDGE('',*,*,#48716,.T.);
#69357=ORIENTED_EDGE('',*,*,#48720,.T.);
#69358=ORIENTED_EDGE('',*,*,#48723,.T.);
#69359=ORIENTED_EDGE('',*,*,#48725,.T.);
#69360=ORIENTED_EDGE('',*,*,#48728,.T.);
#69361=ORIENTED_EDGE('',*,*,#48732,.T.);
#69362=ORIENTED_EDGE('',*,*,#48735,.T.);
#69363=ORIENTED_EDGE('',*,*,#48737,.T.);
#69364=ORIENTED_EDGE('',*,*,#48740,.T.);
#69365=ORIENTED_EDGE('',*,*,#48744,.T.);
#69366=ORIENTED_EDGE('',*,*,#48747,.T.);
#69367=ORIENTED_EDGE('',*,*,#48749,.T.);
#69368=ORIENTED_EDGE('',*,*,#48752,.T.);
#69369=ORIENTED_EDGE('',*,*,#48756,.T.);
#69370=ORIENTED_EDGE('',*,*,#48759,.T.);
#69371=ORIENTED_EDGE('',*,*,#48761,.T.);
#69372=ORIENTED_EDGE('',*,*,#48764,.T.);
#69373=ORIENTED_EDGE('',*,*,#48768,.T.);
#69374=ORIENTED_EDGE('',*,*,#48771,.T.);
#69375=ORIENTED_EDGE('',*,*,#48773,.T.);
#69376=ORIENTED_EDGE('',*,*,#48776,.T.);
#69377=ORIENTED_EDGE('',*,*,#48780,.T.);
#69378=ORIENTED_EDGE('',*,*,#48783,.T.);
#69379=ORIENTED_EDGE('',*,*,#48785,.T.);
#69380=ORIENTED_EDGE('',*,*,#48788,.T.);
#69381=ORIENTED_EDGE('',*,*,#48792,.T.);
#69382=ORIENTED_EDGE('',*,*,#48795,.T.);
#69383=ORIENTED_EDGE('',*,*,#48797,.T.);
#69384=ORIENTED_EDGE('',*,*,#48800,.T.);
#69385=ORIENTED_EDGE('',*,*,#48804,.T.);
#69386=ORIENTED_EDGE('',*,*,#48807,.T.);
#69387=ORIENTED_EDGE('',*,*,#48809,.T.);
#69388=ORIENTED_EDGE('',*,*,#48812,.T.);
#69389=ORIENTED_EDGE('',*,*,#48816,.T.);
#69390=ORIENTED_EDGE('',*,*,#48819,.T.);
#69391=ORIENTED_EDGE('',*,*,#48821,.T.);
#69392=ORIENTED_EDGE('',*,*,#48824,.T.);
#69393=ORIENTED_EDGE('',*,*,#48828,.T.);
#69394=ORIENTED_EDGE('',*,*,#48831,.T.);
#69395=ORIENTED_EDGE('',*,*,#48833,.T.);
#69396=ORIENTED_EDGE('',*,*,#48836,.T.);
#69397=ORIENTED_EDGE('',*,*,#48840,.T.);
#69398=ORIENTED_EDGE('',*,*,#48843,.T.);
#69399=ORIENTED_EDGE('',*,*,#48845,.T.);
#69400=ORIENTED_EDGE('',*,*,#48848,.T.);
#69401=ORIENTED_EDGE('',*,*,#48852,.T.);
#69402=ORIENTED_EDGE('',*,*,#48855,.T.);
#69403=ORIENTED_EDGE('',*,*,#48857,.T.);
#69404=ORIENTED_EDGE('',*,*,#48860,.T.);
#69405=ORIENTED_EDGE('',*,*,#48864,.T.);
#69406=ORIENTED_EDGE('',*,*,#48867,.T.);
#69407=ORIENTED_EDGE('',*,*,#48869,.T.);
#69408=ORIENTED_EDGE('',*,*,#48872,.T.);
#69409=ORIENTED_EDGE('',*,*,#48876,.T.);
#69410=ORIENTED_EDGE('',*,*,#48879,.T.);
#69411=ORIENTED_EDGE('',*,*,#48881,.T.);
#69412=ORIENTED_EDGE('',*,*,#48884,.T.);
#69413=ORIENTED_EDGE('',*,*,#48888,.T.);
#69414=ORIENTED_EDGE('',*,*,#48891,.T.);
#69415=ORIENTED_EDGE('',*,*,#48893,.T.);
#69416=ORIENTED_EDGE('',*,*,#48896,.T.);
#69417=ORIENTED_EDGE('',*,*,#48900,.T.);
#69418=ORIENTED_EDGE('',*,*,#48903,.T.);
#69419=ORIENTED_EDGE('',*,*,#48905,.T.);
#69420=ORIENTED_EDGE('',*,*,#48908,.T.);
#69421=ORIENTED_EDGE('',*,*,#48912,.T.);
#69422=ORIENTED_EDGE('',*,*,#48915,.T.);
#69423=ORIENTED_EDGE('',*,*,#48917,.T.);
#69424=ORIENTED_EDGE('',*,*,#48920,.T.);
#69425=ORIENTED_EDGE('',*,*,#48924,.T.);
#69426=ORIENTED_EDGE('',*,*,#48927,.T.);
#69427=ORIENTED_EDGE('',*,*,#48929,.T.);
#69428=ORIENTED_EDGE('',*,*,#48932,.T.);
#69429=ORIENTED_EDGE('',*,*,#48936,.T.);
#69430=ORIENTED_EDGE('',*,*,#48939,.T.);
#69431=ORIENTED_EDGE('',*,*,#48941,.T.);
#69432=ORIENTED_EDGE('',*,*,#48944,.T.);
#69433=ORIENTED_EDGE('',*,*,#48948,.T.);
#69434=ORIENTED_EDGE('',*,*,#48951,.T.);
#69435=ORIENTED_EDGE('',*,*,#48953,.T.);
#69436=ORIENTED_EDGE('',*,*,#48956,.T.);
#69437=ORIENTED_EDGE('',*,*,#48960,.T.);
#69438=ORIENTED_EDGE('',*,*,#48963,.T.);
#69439=ORIENTED_EDGE('',*,*,#48965,.T.);
#69440=ORIENTED_EDGE('',*,*,#48968,.T.);
#69441=ORIENTED_EDGE('',*,*,#48972,.T.);
#69442=ORIENTED_EDGE('',*,*,#48975,.T.);
#69443=ORIENTED_EDGE('',*,*,#48977,.T.);
#69444=ORIENTED_EDGE('',*,*,#48980,.T.);
#69445=ORIENTED_EDGE('',*,*,#48984,.T.);
#69446=ORIENTED_EDGE('',*,*,#48987,.T.);
#69447=ORIENTED_EDGE('',*,*,#48989,.T.);
#69448=ORIENTED_EDGE('',*,*,#48992,.T.);
#69449=ORIENTED_EDGE('',*,*,#48996,.T.);
#69450=ORIENTED_EDGE('',*,*,#48999,.T.);
#69451=ORIENTED_EDGE('',*,*,#49001,.T.);
#69452=ORIENTED_EDGE('',*,*,#49004,.T.);
#69453=ORIENTED_EDGE('',*,*,#49008,.T.);
#69454=ORIENTED_EDGE('',*,*,#49011,.T.);
#69455=ORIENTED_EDGE('',*,*,#49013,.T.);
#69456=ORIENTED_EDGE('',*,*,#49016,.T.);
#69457=ORIENTED_EDGE('',*,*,#49020,.T.);
#69458=ORIENTED_EDGE('',*,*,#49023,.T.);
#69459=ORIENTED_EDGE('',*,*,#49025,.T.);
#69460=ORIENTED_EDGE('',*,*,#49028,.T.);
#69461=ORIENTED_EDGE('',*,*,#49032,.T.);
#69462=ORIENTED_EDGE('',*,*,#49035,.T.);
#69463=ORIENTED_EDGE('',*,*,#49037,.T.);
#69464=ORIENTED_EDGE('',*,*,#49040,.T.);
#69465=ORIENTED_EDGE('',*,*,#49044,.T.);
#69466=ORIENTED_EDGE('',*,*,#49047,.T.);
#69467=ORIENTED_EDGE('',*,*,#49049,.T.);
#69468=ORIENTED_EDGE('',*,*,#49052,.T.);
#69469=ORIENTED_EDGE('',*,*,#49056,.T.);
#69470=ORIENTED_EDGE('',*,*,#49059,.T.);
#69471=ORIENTED_EDGE('',*,*,#49061,.T.);
#69472=ORIENTED_EDGE('',*,*,#49064,.T.);
#69473=ORIENTED_EDGE('',*,*,#49068,.T.);
#69474=ORIENTED_EDGE('',*,*,#49071,.T.);
#69475=ORIENTED_EDGE('',*,*,#49073,.T.);
#69476=ORIENTED_EDGE('',*,*,#49076,.T.);
#69477=ORIENTED_EDGE('',*,*,#49080,.T.);
#69478=ORIENTED_EDGE('',*,*,#49083,.T.);
#69479=ORIENTED_EDGE('',*,*,#49085,.T.);
#69480=ORIENTED_EDGE('',*,*,#49088,.T.);
#69481=ORIENTED_EDGE('',*,*,#49092,.T.);
#69482=ORIENTED_EDGE('',*,*,#49095,.T.);
#69483=ORIENTED_EDGE('',*,*,#49097,.T.);
#69484=ORIENTED_EDGE('',*,*,#49100,.T.);
#69485=ORIENTED_EDGE('',*,*,#49104,.T.);
#69486=ORIENTED_EDGE('',*,*,#49107,.T.);
#69487=ORIENTED_EDGE('',*,*,#49109,.T.);
#69488=ORIENTED_EDGE('',*,*,#49112,.T.);
#69489=ORIENTED_EDGE('',*,*,#49116,.T.);
#69490=ORIENTED_EDGE('',*,*,#49119,.T.);
#69491=ORIENTED_EDGE('',*,*,#49121,.T.);
#69492=ORIENTED_EDGE('',*,*,#49124,.T.);
#69493=ORIENTED_EDGE('',*,*,#49128,.T.);
#69494=ORIENTED_EDGE('',*,*,#49131,.T.);
#69495=ORIENTED_EDGE('',*,*,#49133,.T.);
#69496=ORIENTED_EDGE('',*,*,#49136,.T.);
#69497=ORIENTED_EDGE('',*,*,#49140,.T.);
#69498=ORIENTED_EDGE('',*,*,#49143,.T.);
#69499=ORIENTED_EDGE('',*,*,#49145,.T.);
#69500=ORIENTED_EDGE('',*,*,#49148,.T.);
#69501=ORIENTED_EDGE('',*,*,#49152,.T.);
#69502=ORIENTED_EDGE('',*,*,#49155,.T.);
#69503=ORIENTED_EDGE('',*,*,#49157,.T.);
#69504=ORIENTED_EDGE('',*,*,#49160,.T.);
#69505=ORIENTED_EDGE('',*,*,#49164,.T.);
#69506=ORIENTED_EDGE('',*,*,#49167,.T.);
#69507=ORIENTED_EDGE('',*,*,#49169,.T.);
#69508=ORIENTED_EDGE('',*,*,#49172,.T.);
#69509=ORIENTED_EDGE('',*,*,#49176,.T.);
#69510=ORIENTED_EDGE('',*,*,#49179,.T.);
#69511=ORIENTED_EDGE('',*,*,#49181,.T.);
#69512=ORIENTED_EDGE('',*,*,#49184,.T.);
#69513=ORIENTED_EDGE('',*,*,#49188,.T.);
#69514=ORIENTED_EDGE('',*,*,#49191,.T.);
#69515=ORIENTED_EDGE('',*,*,#49193,.T.);
#69516=ORIENTED_EDGE('',*,*,#49196,.T.);
#69517=ORIENTED_EDGE('',*,*,#49200,.T.);
#69518=ORIENTED_EDGE('',*,*,#49203,.T.);
#69519=ORIENTED_EDGE('',*,*,#49205,.T.);
#69520=ORIENTED_EDGE('',*,*,#49208,.T.);
#69521=ORIENTED_EDGE('',*,*,#49212,.T.);
#69522=ORIENTED_EDGE('',*,*,#49215,.T.);
#69523=ORIENTED_EDGE('',*,*,#49217,.T.);
#69524=ORIENTED_EDGE('',*,*,#49220,.T.);
#69525=ORIENTED_EDGE('',*,*,#49224,.T.);
#69526=ORIENTED_EDGE('',*,*,#49227,.T.);
#69527=ORIENTED_EDGE('',*,*,#49229,.T.);
#69528=ORIENTED_EDGE('',*,*,#49232,.T.);
#69529=ORIENTED_EDGE('',*,*,#49236,.T.);
#69530=ORIENTED_EDGE('',*,*,#49239,.T.);
#69531=ORIENTED_EDGE('',*,*,#49241,.T.);
#69532=ORIENTED_EDGE('',*,*,#49244,.T.);
#69533=ORIENTED_EDGE('',*,*,#49248,.T.);
#69534=ORIENTED_EDGE('',*,*,#49251,.T.);
#69535=ORIENTED_EDGE('',*,*,#49253,.T.);
#69536=ORIENTED_EDGE('',*,*,#49256,.T.);
#69537=ORIENTED_EDGE('',*,*,#49260,.T.);
#69538=ORIENTED_EDGE('',*,*,#49263,.T.);
#69539=ORIENTED_EDGE('',*,*,#49265,.T.);
#69540=ORIENTED_EDGE('',*,*,#49268,.T.);
#69541=ORIENTED_EDGE('',*,*,#49272,.T.);
#69542=ORIENTED_EDGE('',*,*,#49275,.T.);
#69543=ORIENTED_EDGE('',*,*,#49277,.T.);
#69544=ORIENTED_EDGE('',*,*,#49280,.T.);
#69545=ORIENTED_EDGE('',*,*,#49284,.T.);
#69546=ORIENTED_EDGE('',*,*,#49287,.T.);
#69547=ORIENTED_EDGE('',*,*,#49289,.T.);
#69548=ORIENTED_EDGE('',*,*,#49292,.T.);
#69549=ORIENTED_EDGE('',*,*,#49296,.T.);
#69550=ORIENTED_EDGE('',*,*,#49299,.T.);
#69551=ORIENTED_EDGE('',*,*,#49301,.T.);
#69552=ORIENTED_EDGE('',*,*,#49304,.T.);
#69553=ORIENTED_EDGE('',*,*,#49308,.T.);
#69554=ORIENTED_EDGE('',*,*,#49311,.T.);
#69555=ORIENTED_EDGE('',*,*,#49313,.T.);
#69556=ORIENTED_EDGE('',*,*,#49316,.T.);
#69557=ORIENTED_EDGE('',*,*,#49320,.T.);
#69558=ORIENTED_EDGE('',*,*,#49323,.T.);
#69559=ORIENTED_EDGE('',*,*,#49325,.T.);
#69560=ORIENTED_EDGE('',*,*,#49328,.T.);
#69561=ORIENTED_EDGE('',*,*,#49332,.T.);
#69562=ORIENTED_EDGE('',*,*,#49335,.T.);
#69563=ORIENTED_EDGE('',*,*,#49337,.T.);
#69564=ORIENTED_EDGE('',*,*,#49340,.T.);
#69565=ORIENTED_EDGE('',*,*,#49344,.T.);
#69566=ORIENTED_EDGE('',*,*,#49347,.T.);
#69567=ORIENTED_EDGE('',*,*,#49349,.T.);
#69568=ORIENTED_EDGE('',*,*,#49352,.T.);
#69569=ORIENTED_EDGE('',*,*,#49356,.T.);
#69570=ORIENTED_EDGE('',*,*,#49359,.T.);
#69571=ORIENTED_EDGE('',*,*,#49361,.T.);
#69572=ORIENTED_EDGE('',*,*,#49364,.T.);
#69573=ORIENTED_EDGE('',*,*,#49368,.T.);
#69574=ORIENTED_EDGE('',*,*,#49371,.T.);
#69575=ORIENTED_EDGE('',*,*,#49373,.T.);
#69576=ORIENTED_EDGE('',*,*,#49376,.T.);
#69577=ORIENTED_EDGE('',*,*,#49380,.T.);
#69578=ORIENTED_EDGE('',*,*,#49383,.T.);
#69579=ORIENTED_EDGE('',*,*,#49385,.T.);
#69580=ORIENTED_EDGE('',*,*,#49388,.T.);
#69581=ORIENTED_EDGE('',*,*,#49392,.T.);
#69582=ORIENTED_EDGE('',*,*,#49395,.T.);
#69583=ORIENTED_EDGE('',*,*,#49397,.T.);
#69584=ORIENTED_EDGE('',*,*,#49400,.T.);
#69585=ORIENTED_EDGE('',*,*,#49404,.T.);
#69586=ORIENTED_EDGE('',*,*,#49407,.T.);
#69587=ORIENTED_EDGE('',*,*,#49409,.T.);
#69588=ORIENTED_EDGE('',*,*,#49412,.T.);
#69589=ORIENTED_EDGE('',*,*,#49416,.T.);
#69590=ORIENTED_EDGE('',*,*,#49419,.T.);
#69591=ORIENTED_EDGE('',*,*,#49421,.T.);
#69592=ORIENTED_EDGE('',*,*,#49424,.T.);
#69593=ORIENTED_EDGE('',*,*,#49428,.T.);
#69594=ORIENTED_EDGE('',*,*,#49431,.T.);
#69595=ORIENTED_EDGE('',*,*,#49433,.T.);
#69596=ORIENTED_EDGE('',*,*,#49436,.T.);
#69597=ORIENTED_EDGE('',*,*,#49440,.T.);
#69598=ORIENTED_EDGE('',*,*,#49443,.T.);
#69599=ORIENTED_EDGE('',*,*,#49445,.T.);
#69600=ORIENTED_EDGE('',*,*,#49448,.T.);
#69601=ORIENTED_EDGE('',*,*,#49452,.T.);
#69602=ORIENTED_EDGE('',*,*,#49455,.T.);
#69603=ORIENTED_EDGE('',*,*,#49457,.T.);
#69604=ORIENTED_EDGE('',*,*,#49460,.T.);
#69605=ORIENTED_EDGE('',*,*,#49464,.T.);
#69606=ORIENTED_EDGE('',*,*,#49467,.T.);
#69607=ORIENTED_EDGE('',*,*,#49469,.T.);
#69608=ORIENTED_EDGE('',*,*,#49472,.T.);
#69609=ORIENTED_EDGE('',*,*,#49476,.T.);
#69610=ORIENTED_EDGE('',*,*,#49479,.T.);
#69611=ORIENTED_EDGE('',*,*,#49481,.T.);
#69612=ORIENTED_EDGE('',*,*,#49484,.T.);
#69613=ORIENTED_EDGE('',*,*,#49488,.T.);
#69614=ORIENTED_EDGE('',*,*,#49491,.T.);
#69615=ORIENTED_EDGE('',*,*,#49493,.T.);
#69616=ORIENTED_EDGE('',*,*,#49496,.T.);
#69617=ORIENTED_EDGE('',*,*,#49500,.T.);
#69618=ORIENTED_EDGE('',*,*,#49503,.T.);
#69619=ORIENTED_EDGE('',*,*,#49505,.T.);
#69620=ORIENTED_EDGE('',*,*,#49508,.T.);
#69621=ORIENTED_EDGE('',*,*,#49512,.T.);
#69622=ORIENTED_EDGE('',*,*,#49515,.T.);
#69623=ORIENTED_EDGE('',*,*,#49517,.T.);
#69624=ORIENTED_EDGE('',*,*,#49520,.T.);
#69625=ORIENTED_EDGE('',*,*,#49524,.T.);
#69626=ORIENTED_EDGE('',*,*,#49527,.T.);
#69627=ORIENTED_EDGE('',*,*,#49529,.T.);
#69628=ORIENTED_EDGE('',*,*,#49532,.T.);
#69629=ORIENTED_EDGE('',*,*,#49536,.T.);
#69630=ORIENTED_EDGE('',*,*,#49539,.T.);
#69631=ORIENTED_EDGE('',*,*,#49541,.T.);
#69632=ORIENTED_EDGE('',*,*,#49544,.T.);
#69633=ORIENTED_EDGE('',*,*,#49548,.T.);
#69634=ORIENTED_EDGE('',*,*,#49551,.T.);
#69635=ORIENTED_EDGE('',*,*,#49553,.T.);
#69636=ORIENTED_EDGE('',*,*,#49556,.T.);
#69637=ORIENTED_EDGE('',*,*,#49560,.T.);
#69638=ORIENTED_EDGE('',*,*,#49563,.T.);
#69639=ORIENTED_EDGE('',*,*,#49565,.T.);
#69640=ORIENTED_EDGE('',*,*,#49568,.T.);
#69641=ORIENTED_EDGE('',*,*,#49572,.T.);
#69642=ORIENTED_EDGE('',*,*,#49575,.T.);
#69643=ORIENTED_EDGE('',*,*,#49577,.T.);
#69644=ORIENTED_EDGE('',*,*,#49580,.T.);
#69645=ORIENTED_EDGE('',*,*,#49584,.T.);
#69646=ORIENTED_EDGE('',*,*,#49587,.T.);
#69647=ORIENTED_EDGE('',*,*,#49589,.T.);
#69648=ORIENTED_EDGE('',*,*,#49592,.T.);
#69649=ORIENTED_EDGE('',*,*,#49596,.T.);
#69650=ORIENTED_EDGE('',*,*,#49599,.T.);
#69651=ORIENTED_EDGE('',*,*,#49601,.T.);
#69652=ORIENTED_EDGE('',*,*,#49604,.T.);
#69653=ORIENTED_EDGE('',*,*,#49608,.T.);
#69654=ORIENTED_EDGE('',*,*,#49611,.T.);
#69655=ORIENTED_EDGE('',*,*,#49613,.T.);
#69656=ORIENTED_EDGE('',*,*,#49616,.T.);
#69657=ORIENTED_EDGE('',*,*,#49620,.T.);
#69658=ORIENTED_EDGE('',*,*,#49623,.T.);
#69659=ORIENTED_EDGE('',*,*,#49625,.T.);
#69660=ORIENTED_EDGE('',*,*,#49628,.T.);
#69661=ORIENTED_EDGE('',*,*,#49632,.T.);
#69662=ORIENTED_EDGE('',*,*,#49635,.T.);
#69663=ORIENTED_EDGE('',*,*,#49637,.T.);
#69664=ORIENTED_EDGE('',*,*,#49640,.T.);
#69665=ORIENTED_EDGE('',*,*,#49644,.T.);
#69666=ORIENTED_EDGE('',*,*,#49647,.T.);
#69667=ORIENTED_EDGE('',*,*,#49649,.T.);
#69668=ORIENTED_EDGE('',*,*,#49652,.T.);
#69669=ORIENTED_EDGE('',*,*,#49656,.T.);
#69670=ORIENTED_EDGE('',*,*,#49659,.T.);
#69671=ORIENTED_EDGE('',*,*,#49661,.T.);
#69672=ORIENTED_EDGE('',*,*,#49664,.T.);
#69673=ORIENTED_EDGE('',*,*,#49668,.T.);
#69674=ORIENTED_EDGE('',*,*,#49671,.T.);
#69675=ORIENTED_EDGE('',*,*,#49673,.T.);
#69676=ORIENTED_EDGE('',*,*,#49676,.T.);
#69677=ORIENTED_EDGE('',*,*,#49680,.T.);
#69678=ORIENTED_EDGE('',*,*,#49683,.T.);
#69679=ORIENTED_EDGE('',*,*,#49685,.T.);
#69680=ORIENTED_EDGE('',*,*,#49688,.T.);
#69681=ORIENTED_EDGE('',*,*,#49692,.T.);
#69682=ORIENTED_EDGE('',*,*,#49695,.T.);
#69683=ORIENTED_EDGE('',*,*,#49697,.T.);
#69684=ORIENTED_EDGE('',*,*,#49700,.T.);
#69685=ORIENTED_EDGE('',*,*,#49704,.T.);
#69686=ORIENTED_EDGE('',*,*,#49707,.T.);
#69687=ORIENTED_EDGE('',*,*,#49709,.T.);
#69688=ORIENTED_EDGE('',*,*,#49712,.T.);
#69689=ORIENTED_EDGE('',*,*,#49716,.T.);
#69690=ORIENTED_EDGE('',*,*,#49719,.T.);
#69691=ORIENTED_EDGE('',*,*,#49721,.T.);
#69692=ORIENTED_EDGE('',*,*,#49724,.T.);
#69693=ORIENTED_EDGE('',*,*,#49728,.T.);
#69694=ORIENTED_EDGE('',*,*,#49731,.T.);
#69695=ORIENTED_EDGE('',*,*,#49733,.T.);
#69696=ORIENTED_EDGE('',*,*,#49736,.T.);
#69697=ORIENTED_EDGE('',*,*,#49740,.T.);
#69698=ORIENTED_EDGE('',*,*,#49743,.T.);
#69699=ORIENTED_EDGE('',*,*,#49745,.T.);
#69700=ORIENTED_EDGE('',*,*,#49748,.T.);
#69701=ORIENTED_EDGE('',*,*,#49752,.T.);
#69702=ORIENTED_EDGE('',*,*,#49755,.T.);
#69703=ORIENTED_EDGE('',*,*,#49757,.T.);
#69704=ORIENTED_EDGE('',*,*,#49760,.T.);
#69705=ORIENTED_EDGE('',*,*,#49764,.T.);
#69706=ORIENTED_EDGE('',*,*,#49767,.T.);
#69707=ORIENTED_EDGE('',*,*,#49769,.T.);
#69708=ORIENTED_EDGE('',*,*,#49772,.T.);
#69709=ORIENTED_EDGE('',*,*,#49776,.T.);
#69710=ORIENTED_EDGE('',*,*,#49779,.T.);
#69711=ORIENTED_EDGE('',*,*,#49781,.T.);
#69712=ORIENTED_EDGE('',*,*,#49784,.T.);
#69713=ORIENTED_EDGE('',*,*,#49788,.T.);
#69714=ORIENTED_EDGE('',*,*,#49791,.T.);
#69715=ORIENTED_EDGE('',*,*,#49793,.T.);
#69716=ORIENTED_EDGE('',*,*,#49796,.T.);
#69717=ORIENTED_EDGE('',*,*,#49800,.T.);
#69718=ORIENTED_EDGE('',*,*,#49803,.T.);
#69719=ORIENTED_EDGE('',*,*,#49805,.T.);
#69720=ORIENTED_EDGE('',*,*,#49808,.T.);
#69721=ORIENTED_EDGE('',*,*,#49812,.T.);
#69722=ORIENTED_EDGE('',*,*,#49815,.T.);
#69723=ORIENTED_EDGE('',*,*,#49817,.T.);
#69724=ORIENTED_EDGE('',*,*,#49820,.T.);
#69725=ORIENTED_EDGE('',*,*,#49824,.T.);
#69726=ORIENTED_EDGE('',*,*,#49827,.T.);
#69727=ORIENTED_EDGE('',*,*,#49829,.T.);
#69728=ORIENTED_EDGE('',*,*,#49832,.T.);
#69729=ORIENTED_EDGE('',*,*,#49836,.T.);
#69730=ORIENTED_EDGE('',*,*,#49839,.T.);
#69731=ORIENTED_EDGE('',*,*,#49841,.T.);
#69732=ORIENTED_EDGE('',*,*,#49844,.T.);
#69733=ORIENTED_EDGE('',*,*,#49848,.T.);
#69734=ORIENTED_EDGE('',*,*,#49851,.T.);
#69735=ORIENTED_EDGE('',*,*,#49853,.T.);
#69736=ORIENTED_EDGE('',*,*,#49856,.T.);
#69737=ORIENTED_EDGE('',*,*,#49860,.T.);
#69738=ORIENTED_EDGE('',*,*,#49863,.T.);
#69739=ORIENTED_EDGE('',*,*,#49865,.T.);
#69740=ORIENTED_EDGE('',*,*,#49868,.T.);
#69741=ORIENTED_EDGE('',*,*,#49872,.T.);
#69742=ORIENTED_EDGE('',*,*,#49875,.T.);
#69743=ORIENTED_EDGE('',*,*,#49877,.T.);
#69744=ORIENTED_EDGE('',*,*,#49880,.T.);
#69745=ORIENTED_EDGE('',*,*,#49884,.T.);
#69746=ORIENTED_EDGE('',*,*,#49887,.T.);
#69747=ORIENTED_EDGE('',*,*,#49889,.T.);
#69748=ORIENTED_EDGE('',*,*,#49892,.T.);
#69749=ORIENTED_EDGE('',*,*,#49896,.T.);
#69750=ORIENTED_EDGE('',*,*,#49899,.T.);
#69751=ORIENTED_EDGE('',*,*,#49901,.T.);
#69752=ORIENTED_EDGE('',*,*,#49904,.T.);
#69753=ORIENTED_EDGE('',*,*,#49908,.T.);
#69754=ORIENTED_EDGE('',*,*,#49911,.T.);
#69755=ORIENTED_EDGE('',*,*,#49913,.T.);
#69756=ORIENTED_EDGE('',*,*,#49916,.T.);
#69757=ORIENTED_EDGE('',*,*,#49920,.T.);
#69758=ORIENTED_EDGE('',*,*,#49923,.T.);
#69759=ORIENTED_EDGE('',*,*,#49925,.T.);
#69760=ORIENTED_EDGE('',*,*,#49928,.T.);
#69761=ORIENTED_EDGE('',*,*,#49932,.T.);
#69762=ORIENTED_EDGE('',*,*,#49935,.T.);
#69763=ORIENTED_EDGE('',*,*,#49937,.T.);
#69764=ORIENTED_EDGE('',*,*,#49940,.T.);
#69765=ORIENTED_EDGE('',*,*,#49944,.T.);
#69766=ORIENTED_EDGE('',*,*,#49947,.T.);
#69767=ORIENTED_EDGE('',*,*,#49949,.T.);
#69768=ORIENTED_EDGE('',*,*,#49952,.T.);
#69769=ORIENTED_EDGE('',*,*,#49956,.T.);
#69770=ORIENTED_EDGE('',*,*,#49959,.T.);
#69771=ORIENTED_EDGE('',*,*,#49961,.T.);
#69772=ORIENTED_EDGE('',*,*,#49964,.T.);
#69773=ORIENTED_EDGE('',*,*,#49968,.T.);
#69774=ORIENTED_EDGE('',*,*,#49971,.T.);
#69775=ORIENTED_EDGE('',*,*,#49973,.T.);
#69776=ORIENTED_EDGE('',*,*,#49976,.T.);
#69777=ORIENTED_EDGE('',*,*,#49980,.T.);
#69778=ORIENTED_EDGE('',*,*,#49983,.T.);
#69779=ORIENTED_EDGE('',*,*,#49985,.T.);
#69780=ORIENTED_EDGE('',*,*,#49988,.T.);
#69781=ORIENTED_EDGE('',*,*,#49992,.T.);
#69782=ORIENTED_EDGE('',*,*,#49995,.T.);
#69783=ORIENTED_EDGE('',*,*,#49997,.T.);
#69784=ORIENTED_EDGE('',*,*,#50000,.T.);
#69785=ORIENTED_EDGE('',*,*,#50004,.T.);
#69786=ORIENTED_EDGE('',*,*,#50007,.T.);
#69787=ORIENTED_EDGE('',*,*,#50009,.T.);
#69788=ORIENTED_EDGE('',*,*,#50012,.T.);
#69789=ORIENTED_EDGE('',*,*,#50016,.T.);
#69790=ORIENTED_EDGE('',*,*,#50019,.T.);
#69791=ORIENTED_EDGE('',*,*,#50021,.T.);
#69792=ORIENTED_EDGE('',*,*,#50024,.T.);
#69793=ORIENTED_EDGE('',*,*,#50028,.T.);
#69794=ORIENTED_EDGE('',*,*,#50031,.T.);
#69795=ORIENTED_EDGE('',*,*,#50033,.T.);
#69796=ORIENTED_EDGE('',*,*,#50036,.T.);
#69797=ORIENTED_EDGE('',*,*,#50040,.T.);
#69798=ORIENTED_EDGE('',*,*,#50043,.T.);
#69799=ORIENTED_EDGE('',*,*,#50045,.T.);
#69800=ORIENTED_EDGE('',*,*,#50048,.T.);
#69801=ORIENTED_EDGE('',*,*,#50052,.T.);
#69802=ORIENTED_EDGE('',*,*,#50055,.T.);
#69803=ORIENTED_EDGE('',*,*,#50057,.T.);
#69804=ORIENTED_EDGE('',*,*,#50060,.T.);
#69805=ORIENTED_EDGE('',*,*,#50064,.T.);
#69806=ORIENTED_EDGE('',*,*,#50067,.T.);
#69807=ORIENTED_EDGE('',*,*,#50069,.T.);
#69808=ORIENTED_EDGE('',*,*,#50072,.T.);
#69809=ORIENTED_EDGE('',*,*,#50076,.T.);
#69810=ORIENTED_EDGE('',*,*,#50079,.T.);
#69811=ORIENTED_EDGE('',*,*,#50081,.T.);
#69812=ORIENTED_EDGE('',*,*,#50084,.T.);
#69813=ORIENTED_EDGE('',*,*,#50088,.T.);
#69814=ORIENTED_EDGE('',*,*,#50091,.T.);
#69815=ORIENTED_EDGE('',*,*,#50093,.T.);
#69816=ORIENTED_EDGE('',*,*,#50096,.T.);
#69817=ORIENTED_EDGE('',*,*,#50100,.T.);
#69818=ORIENTED_EDGE('',*,*,#50103,.T.);
#69819=ORIENTED_EDGE('',*,*,#50105,.T.);
#69820=ORIENTED_EDGE('',*,*,#50108,.T.);
#69821=ORIENTED_EDGE('',*,*,#50112,.T.);
#69822=ORIENTED_EDGE('',*,*,#50115,.T.);
#69823=ORIENTED_EDGE('',*,*,#50117,.T.);
#69824=ORIENTED_EDGE('',*,*,#50120,.T.);
#69825=ORIENTED_EDGE('',*,*,#50124,.T.);
#69826=ORIENTED_EDGE('',*,*,#50127,.T.);
#69827=ORIENTED_EDGE('',*,*,#50129,.T.);
#69828=ORIENTED_EDGE('',*,*,#50132,.T.);
#69829=ORIENTED_EDGE('',*,*,#50136,.T.);
#69830=ORIENTED_EDGE('',*,*,#50139,.T.);
#69831=ORIENTED_EDGE('',*,*,#50141,.T.);
#69832=ORIENTED_EDGE('',*,*,#50144,.T.);
#69833=ORIENTED_EDGE('',*,*,#50148,.T.);
#69834=ORIENTED_EDGE('',*,*,#50151,.T.);
#69835=ORIENTED_EDGE('',*,*,#50153,.T.);
#69836=ORIENTED_EDGE('',*,*,#50156,.T.);
#69837=ORIENTED_EDGE('',*,*,#50160,.T.);
#69838=ORIENTED_EDGE('',*,*,#50163,.T.);
#69839=ORIENTED_EDGE('',*,*,#50165,.T.);
#69840=ORIENTED_EDGE('',*,*,#50168,.T.);
#69841=ORIENTED_EDGE('',*,*,#50172,.T.);
#69842=ORIENTED_EDGE('',*,*,#50175,.T.);
#69843=ORIENTED_EDGE('',*,*,#50177,.T.);
#69844=ORIENTED_EDGE('',*,*,#50180,.T.);
#69845=ORIENTED_EDGE('',*,*,#50184,.T.);
#69846=ORIENTED_EDGE('',*,*,#50187,.T.);
#69847=ORIENTED_EDGE('',*,*,#50189,.T.);
#69848=ORIENTED_EDGE('',*,*,#50192,.T.);
#69849=ORIENTED_EDGE('',*,*,#50196,.T.);
#69850=ORIENTED_EDGE('',*,*,#50199,.T.);
#69851=ORIENTED_EDGE('',*,*,#50201,.T.);
#69852=ORIENTED_EDGE('',*,*,#50204,.T.);
#69853=ORIENTED_EDGE('',*,*,#50208,.T.);
#69854=ORIENTED_EDGE('',*,*,#50211,.T.);
#69855=ORIENTED_EDGE('',*,*,#50213,.T.);
#69856=ORIENTED_EDGE('',*,*,#50216,.T.);
#69857=ORIENTED_EDGE('',*,*,#50220,.T.);
#69858=ORIENTED_EDGE('',*,*,#50223,.T.);
#69859=ORIENTED_EDGE('',*,*,#50225,.T.);
#69860=ORIENTED_EDGE('',*,*,#50228,.T.);
#69861=ORIENTED_EDGE('',*,*,#50232,.T.);
#69862=ORIENTED_EDGE('',*,*,#50235,.T.);
#69863=ORIENTED_EDGE('',*,*,#50237,.T.);
#69864=ORIENTED_EDGE('',*,*,#50240,.T.);
#69865=ORIENTED_EDGE('',*,*,#50244,.T.);
#69866=ORIENTED_EDGE('',*,*,#50247,.T.);
#69867=ORIENTED_EDGE('',*,*,#50249,.T.);
#69868=ORIENTED_EDGE('',*,*,#50252,.T.);
#69869=ORIENTED_EDGE('',*,*,#50256,.T.);
#69870=ORIENTED_EDGE('',*,*,#50259,.T.);
#69871=ORIENTED_EDGE('',*,*,#50261,.T.);
#69872=ORIENTED_EDGE('',*,*,#50264,.T.);
#69873=ORIENTED_EDGE('',*,*,#50268,.T.);
#69874=ORIENTED_EDGE('',*,*,#50271,.T.);
#69875=ORIENTED_EDGE('',*,*,#50273,.T.);
#69876=ORIENTED_EDGE('',*,*,#50276,.T.);
#69877=ORIENTED_EDGE('',*,*,#50280,.T.);
#69878=ORIENTED_EDGE('',*,*,#50283,.T.);
#69879=ORIENTED_EDGE('',*,*,#50285,.T.);
#69880=ORIENTED_EDGE('',*,*,#50288,.T.);
#69881=ORIENTED_EDGE('',*,*,#50292,.T.);
#69882=ORIENTED_EDGE('',*,*,#50295,.T.);
#69883=ORIENTED_EDGE('',*,*,#50297,.T.);
#69884=ORIENTED_EDGE('',*,*,#50300,.T.);
#69885=ORIENTED_EDGE('',*,*,#50304,.T.);
#69886=ORIENTED_EDGE('',*,*,#50307,.T.);
#69887=ORIENTED_EDGE('',*,*,#50309,.T.);
#69888=ORIENTED_EDGE('',*,*,#50312,.T.);
#69889=ORIENTED_EDGE('',*,*,#50316,.T.);
#69890=ORIENTED_EDGE('',*,*,#50319,.T.);
#69891=ORIENTED_EDGE('',*,*,#50321,.T.);
#69892=ORIENTED_EDGE('',*,*,#50324,.T.);
#69893=ORIENTED_EDGE('',*,*,#50328,.T.);
#69894=ORIENTED_EDGE('',*,*,#50331,.T.);
#69895=ORIENTED_EDGE('',*,*,#50333,.T.);
#69896=ORIENTED_EDGE('',*,*,#50336,.T.);
#69897=ORIENTED_EDGE('',*,*,#50340,.T.);
#69898=ORIENTED_EDGE('',*,*,#50343,.T.);
#69899=ORIENTED_EDGE('',*,*,#50345,.T.);
#69900=ORIENTED_EDGE('',*,*,#50348,.T.);
#69901=ORIENTED_EDGE('',*,*,#50352,.T.);
#69902=ORIENTED_EDGE('',*,*,#50355,.T.);
#69903=ORIENTED_EDGE('',*,*,#50357,.T.);
#69904=ORIENTED_EDGE('',*,*,#50360,.T.);
#69905=ORIENTED_EDGE('',*,*,#50364,.T.);
#69906=ORIENTED_EDGE('',*,*,#50367,.T.);
#69907=ORIENTED_EDGE('',*,*,#50369,.T.);
#69908=ORIENTED_EDGE('',*,*,#50372,.T.);
#69909=ORIENTED_EDGE('',*,*,#50376,.T.);
#69910=ORIENTED_EDGE('',*,*,#50379,.T.);
#69911=ORIENTED_EDGE('',*,*,#50381,.T.);
#69912=ORIENTED_EDGE('',*,*,#50384,.T.);
#69913=ORIENTED_EDGE('',*,*,#50388,.T.);
#69914=ORIENTED_EDGE('',*,*,#50391,.T.);
#69915=ORIENTED_EDGE('',*,*,#50393,.T.);
#69916=ORIENTED_EDGE('',*,*,#50396,.T.);
#69917=ORIENTED_EDGE('',*,*,#50400,.T.);
#69918=ORIENTED_EDGE('',*,*,#50403,.T.);
#69919=ORIENTED_EDGE('',*,*,#50405,.T.);
#69920=ORIENTED_EDGE('',*,*,#50408,.T.);
#69921=ORIENTED_EDGE('',*,*,#50412,.T.);
#69922=ORIENTED_EDGE('',*,*,#50415,.T.);
#69923=ORIENTED_EDGE('',*,*,#50417,.T.);
#69924=ORIENTED_EDGE('',*,*,#50420,.T.);
#69925=ORIENTED_EDGE('',*,*,#50424,.T.);
#69926=ORIENTED_EDGE('',*,*,#50427,.T.);
#69927=ORIENTED_EDGE('',*,*,#50429,.T.);
#69928=ORIENTED_EDGE('',*,*,#50432,.T.);
#69929=ORIENTED_EDGE('',*,*,#50436,.T.);
#69930=ORIENTED_EDGE('',*,*,#50439,.T.);
#69931=ORIENTED_EDGE('',*,*,#50441,.T.);
#69932=ORIENTED_EDGE('',*,*,#50444,.T.);
#69933=ORIENTED_EDGE('',*,*,#50448,.T.);
#69934=ORIENTED_EDGE('',*,*,#50451,.T.);
#69935=ORIENTED_EDGE('',*,*,#50453,.T.);
#69936=ORIENTED_EDGE('',*,*,#50456,.T.);
#69937=ORIENTED_EDGE('',*,*,#50460,.T.);
#69938=ORIENTED_EDGE('',*,*,#50463,.T.);
#69939=ORIENTED_EDGE('',*,*,#50465,.T.);
#69940=ORIENTED_EDGE('',*,*,#50468,.T.);
#69941=ORIENTED_EDGE('',*,*,#50472,.T.);
#69942=ORIENTED_EDGE('',*,*,#50475,.T.);
#69943=ORIENTED_EDGE('',*,*,#50477,.T.);
#69944=ORIENTED_EDGE('',*,*,#50480,.T.);
#69945=ORIENTED_EDGE('',*,*,#50484,.T.);
#69946=ORIENTED_EDGE('',*,*,#50487,.T.);
#69947=ORIENTED_EDGE('',*,*,#50489,.T.);
#69948=ORIENTED_EDGE('',*,*,#50492,.T.);
#69949=ORIENTED_EDGE('',*,*,#50496,.T.);
#69950=ORIENTED_EDGE('',*,*,#50499,.T.);
#69951=ORIENTED_EDGE('',*,*,#50501,.T.);
#69952=ORIENTED_EDGE('',*,*,#50504,.T.);
#69953=ORIENTED_EDGE('',*,*,#50508,.T.);
#69954=ORIENTED_EDGE('',*,*,#50511,.T.);
#69955=ORIENTED_EDGE('',*,*,#50513,.T.);
#69956=ORIENTED_EDGE('',*,*,#50516,.T.);
#69957=ORIENTED_EDGE('',*,*,#50520,.T.);
#69958=ORIENTED_EDGE('',*,*,#50523,.T.);
#69959=ORIENTED_EDGE('',*,*,#50525,.T.);
#69960=ORIENTED_EDGE('',*,*,#50528,.T.);
#69961=ORIENTED_EDGE('',*,*,#50532,.T.);
#69962=ORIENTED_EDGE('',*,*,#50535,.T.);
#69963=ORIENTED_EDGE('',*,*,#50537,.T.);
#69964=ORIENTED_EDGE('',*,*,#50540,.T.);
#69965=ORIENTED_EDGE('',*,*,#50544,.T.);
#69966=ORIENTED_EDGE('',*,*,#50547,.T.);
#69967=ORIENTED_EDGE('',*,*,#50549,.T.);
#69968=ORIENTED_EDGE('',*,*,#50552,.T.);
#69969=ORIENTED_EDGE('',*,*,#50556,.T.);
#69970=ORIENTED_EDGE('',*,*,#50559,.T.);
#69971=ORIENTED_EDGE('',*,*,#50561,.T.);
#69972=ORIENTED_EDGE('',*,*,#50564,.T.);
#69973=ORIENTED_EDGE('',*,*,#50568,.T.);
#69974=ORIENTED_EDGE('',*,*,#50571,.T.);
#69975=ORIENTED_EDGE('',*,*,#50573,.T.);
#69976=ORIENTED_EDGE('',*,*,#50576,.T.);
#69977=ORIENTED_EDGE('',*,*,#50580,.T.);
#69978=ORIENTED_EDGE('',*,*,#50583,.T.);
#69979=ORIENTED_EDGE('',*,*,#50585,.T.);
#69980=ORIENTED_EDGE('',*,*,#50588,.T.);
#69981=ORIENTED_EDGE('',*,*,#50592,.T.);
#69982=ORIENTED_EDGE('',*,*,#50595,.T.);
#69983=ORIENTED_EDGE('',*,*,#50597,.T.);
#69984=ORIENTED_EDGE('',*,*,#50600,.T.);
#69985=ORIENTED_EDGE('',*,*,#50604,.T.);
#69986=ORIENTED_EDGE('',*,*,#50607,.T.);
#69987=ORIENTED_EDGE('',*,*,#50609,.T.);
#69988=ORIENTED_EDGE('',*,*,#50612,.T.);
#69989=ORIENTED_EDGE('',*,*,#50616,.T.);
#69990=ORIENTED_EDGE('',*,*,#50619,.T.);
#69991=ORIENTED_EDGE('',*,*,#50621,.T.);
#69992=ORIENTED_EDGE('',*,*,#50624,.T.);
#69993=ORIENTED_EDGE('',*,*,#50628,.T.);
#69994=ORIENTED_EDGE('',*,*,#50631,.T.);
#69995=ORIENTED_EDGE('',*,*,#50633,.T.);
#69996=ORIENTED_EDGE('',*,*,#50636,.T.);
#69997=ORIENTED_EDGE('',*,*,#50640,.T.);
#69998=ORIENTED_EDGE('',*,*,#50643,.T.);
#69999=ORIENTED_EDGE('',*,*,#50645,.T.);
#70000=ORIENTED_EDGE('',*,*,#50648,.T.);
#70001=ORIENTED_EDGE('',*,*,#50652,.T.);
#70002=ORIENTED_EDGE('',*,*,#50655,.T.);
#70003=ORIENTED_EDGE('',*,*,#50657,.T.);
#70004=ORIENTED_EDGE('',*,*,#50660,.T.);
#70005=ORIENTED_EDGE('',*,*,#50664,.T.);
#70006=ORIENTED_EDGE('',*,*,#50667,.T.);
#70007=ORIENTED_EDGE('',*,*,#50669,.T.);
#70008=ORIENTED_EDGE('',*,*,#50672,.T.);
#70009=ORIENTED_EDGE('',*,*,#50676,.T.);
#70010=ORIENTED_EDGE('',*,*,#50679,.T.);
#70011=ORIENTED_EDGE('',*,*,#50681,.T.);
#70012=ORIENTED_EDGE('',*,*,#50684,.T.);
#70013=ORIENTED_EDGE('',*,*,#50688,.T.);
#70014=ORIENTED_EDGE('',*,*,#50691,.T.);
#70015=ORIENTED_EDGE('',*,*,#50693,.T.);
#70016=ORIENTED_EDGE('',*,*,#50696,.T.);
#70017=ORIENTED_EDGE('',*,*,#50700,.T.);
#70018=ORIENTED_EDGE('',*,*,#50703,.T.);
#70019=ORIENTED_EDGE('',*,*,#50705,.T.);
#70020=ORIENTED_EDGE('',*,*,#50708,.T.);
#70021=ORIENTED_EDGE('',*,*,#50712,.T.);
#70022=ORIENTED_EDGE('',*,*,#50715,.T.);
#70023=ORIENTED_EDGE('',*,*,#50717,.T.);
#70024=ORIENTED_EDGE('',*,*,#50720,.T.);
#70025=ORIENTED_EDGE('',*,*,#50724,.T.);
#70026=ORIENTED_EDGE('',*,*,#50727,.T.);
#70027=ORIENTED_EDGE('',*,*,#50729,.T.);
#70028=ORIENTED_EDGE('',*,*,#50732,.T.);
#70029=ORIENTED_EDGE('',*,*,#50736,.T.);
#70030=ORIENTED_EDGE('',*,*,#50739,.T.);
#70031=ORIENTED_EDGE('',*,*,#50741,.T.);
#70032=ORIENTED_EDGE('',*,*,#50744,.T.);
#70033=ORIENTED_EDGE('',*,*,#50748,.T.);
#70034=ORIENTED_EDGE('',*,*,#50751,.T.);
#70035=ORIENTED_EDGE('',*,*,#50753,.T.);
#70036=ORIENTED_EDGE('',*,*,#50756,.T.);
#70037=ORIENTED_EDGE('',*,*,#50760,.T.);
#70038=ORIENTED_EDGE('',*,*,#50763,.T.);
#70039=ORIENTED_EDGE('',*,*,#50765,.T.);
#70040=ORIENTED_EDGE('',*,*,#50768,.T.);
#70041=ORIENTED_EDGE('',*,*,#50772,.T.);
#70042=ORIENTED_EDGE('',*,*,#50775,.T.);
#70043=ORIENTED_EDGE('',*,*,#50777,.T.);
#70044=ORIENTED_EDGE('',*,*,#50780,.T.);
#70045=ORIENTED_EDGE('',*,*,#50784,.T.);
#70046=ORIENTED_EDGE('',*,*,#50787,.T.);
#70047=ORIENTED_EDGE('',*,*,#50789,.T.);
#70048=ORIENTED_EDGE('',*,*,#50792,.T.);
#70049=ORIENTED_EDGE('',*,*,#50796,.T.);
#70050=ORIENTED_EDGE('',*,*,#50799,.T.);
#70051=ORIENTED_EDGE('',*,*,#50801,.T.);
#70052=ORIENTED_EDGE('',*,*,#50804,.T.);
#70053=ORIENTED_EDGE('',*,*,#50808,.T.);
#70054=ORIENTED_EDGE('',*,*,#50811,.T.);
#70055=ORIENTED_EDGE('',*,*,#50813,.T.);
#70056=ORIENTED_EDGE('',*,*,#50816,.T.);
#70057=ORIENTED_EDGE('',*,*,#50820,.T.);
#70058=ORIENTED_EDGE('',*,*,#50823,.T.);
#70059=ORIENTED_EDGE('',*,*,#50825,.T.);
#70060=ORIENTED_EDGE('',*,*,#50828,.T.);
#70061=ORIENTED_EDGE('',*,*,#50832,.T.);
#70062=ORIENTED_EDGE('',*,*,#50835,.T.);
#70063=ORIENTED_EDGE('',*,*,#50837,.T.);
#70064=ORIENTED_EDGE('',*,*,#50840,.T.);
#70065=ORIENTED_EDGE('',*,*,#50844,.T.);
#70066=ORIENTED_EDGE('',*,*,#50847,.T.);
#70067=ORIENTED_EDGE('',*,*,#50849,.T.);
#70068=ORIENTED_EDGE('',*,*,#50852,.T.);
#70069=ORIENTED_EDGE('',*,*,#50856,.T.);
#70070=ORIENTED_EDGE('',*,*,#50859,.T.);
#70071=ORIENTED_EDGE('',*,*,#50861,.T.);
#70072=ORIENTED_EDGE('',*,*,#50864,.T.);
#70073=ORIENTED_EDGE('',*,*,#50868,.T.);
#70074=ORIENTED_EDGE('',*,*,#50871,.T.);
#70075=ORIENTED_EDGE('',*,*,#50873,.T.);
#70076=ORIENTED_EDGE('',*,*,#50876,.T.);
#70077=ORIENTED_EDGE('',*,*,#50880,.T.);
#70078=ORIENTED_EDGE('',*,*,#50883,.T.);
#70079=ORIENTED_EDGE('',*,*,#50885,.T.);
#70080=ORIENTED_EDGE('',*,*,#50888,.T.);
#70081=ORIENTED_EDGE('',*,*,#50892,.T.);
#70082=ORIENTED_EDGE('',*,*,#50895,.T.);
#70083=ORIENTED_EDGE('',*,*,#50897,.T.);
#70084=ORIENTED_EDGE('',*,*,#50900,.T.);
#70085=ORIENTED_EDGE('',*,*,#50904,.T.);
#70086=ORIENTED_EDGE('',*,*,#50907,.T.);
#70087=ORIENTED_EDGE('',*,*,#50909,.T.);
#70088=ORIENTED_EDGE('',*,*,#50912,.T.);
#70089=ORIENTED_EDGE('',*,*,#50916,.T.);
#70090=ORIENTED_EDGE('',*,*,#50919,.T.);
#70091=ORIENTED_EDGE('',*,*,#50921,.T.);
#70092=ORIENTED_EDGE('',*,*,#50924,.T.);
#70093=ORIENTED_EDGE('',*,*,#50928,.T.);
#70094=ORIENTED_EDGE('',*,*,#50931,.T.);
#70095=ORIENTED_EDGE('',*,*,#50933,.T.);
#70096=ORIENTED_EDGE('',*,*,#50936,.T.);
#70097=ORIENTED_EDGE('',*,*,#50940,.T.);
#70098=ORIENTED_EDGE('',*,*,#50943,.T.);
#70099=ORIENTED_EDGE('',*,*,#50945,.T.);
#70100=ORIENTED_EDGE('',*,*,#50948,.T.);
#70101=ORIENTED_EDGE('',*,*,#50952,.T.);
#70102=ORIENTED_EDGE('',*,*,#50955,.T.);
#70103=ORIENTED_EDGE('',*,*,#50957,.T.);
#70104=ORIENTED_EDGE('',*,*,#50960,.T.);
#70105=ORIENTED_EDGE('',*,*,#50964,.T.);
#70106=ORIENTED_EDGE('',*,*,#50967,.T.);
#70107=ORIENTED_EDGE('',*,*,#50969,.T.);
#70108=ORIENTED_EDGE('',*,*,#50972,.T.);
#70109=ORIENTED_EDGE('',*,*,#50976,.T.);
#70110=ORIENTED_EDGE('',*,*,#50979,.T.);
#70111=ORIENTED_EDGE('',*,*,#50981,.T.);
#70112=ORIENTED_EDGE('',*,*,#50984,.T.);
#70113=ORIENTED_EDGE('',*,*,#50988,.T.);
#70114=ORIENTED_EDGE('',*,*,#50991,.T.);
#70115=ORIENTED_EDGE('',*,*,#50993,.T.);
#70116=ORIENTED_EDGE('',*,*,#50996,.T.);
#70117=ORIENTED_EDGE('',*,*,#51000,.T.);
#70118=ORIENTED_EDGE('',*,*,#51003,.T.);
#70119=ORIENTED_EDGE('',*,*,#51005,.T.);
#70120=ORIENTED_EDGE('',*,*,#51008,.T.);
#70121=ORIENTED_EDGE('',*,*,#51012,.T.);
#70122=ORIENTED_EDGE('',*,*,#51015,.T.);
#70123=ORIENTED_EDGE('',*,*,#51017,.T.);
#70124=ORIENTED_EDGE('',*,*,#51020,.T.);
#70125=ORIENTED_EDGE('',*,*,#51024,.T.);
#70126=ORIENTED_EDGE('',*,*,#51027,.T.);
#70127=ORIENTED_EDGE('',*,*,#51029,.T.);
#70128=ORIENTED_EDGE('',*,*,#51032,.T.);
#70129=ORIENTED_EDGE('',*,*,#51036,.T.);
#70130=ORIENTED_EDGE('',*,*,#51039,.T.);
#70131=ORIENTED_EDGE('',*,*,#51041,.T.);
#70132=ORIENTED_EDGE('',*,*,#51044,.T.);
#70133=ORIENTED_EDGE('',*,*,#51048,.T.);
#70134=ORIENTED_EDGE('',*,*,#51051,.T.);
#70135=ORIENTED_EDGE('',*,*,#51053,.T.);
#70136=ORIENTED_EDGE('',*,*,#51056,.T.);
#70137=ORIENTED_EDGE('',*,*,#51060,.T.);
#70138=ORIENTED_EDGE('',*,*,#51063,.T.);
#70139=ORIENTED_EDGE('',*,*,#51065,.T.);
#70140=ORIENTED_EDGE('',*,*,#51068,.T.);
#70141=ORIENTED_EDGE('',*,*,#51072,.T.);
#70142=ORIENTED_EDGE('',*,*,#51075,.T.);
#70143=ORIENTED_EDGE('',*,*,#51077,.T.);
#70144=ORIENTED_EDGE('',*,*,#51080,.T.);
#70145=ORIENTED_EDGE('',*,*,#51084,.T.);
#70146=ORIENTED_EDGE('',*,*,#51087,.T.);
#70147=ORIENTED_EDGE('',*,*,#51089,.T.);
#70148=ORIENTED_EDGE('',*,*,#51092,.T.);
#70149=ORIENTED_EDGE('',*,*,#51096,.T.);
#70150=ORIENTED_EDGE('',*,*,#51099,.T.);
#70151=ORIENTED_EDGE('',*,*,#51101,.T.);
#70152=ORIENTED_EDGE('',*,*,#51104,.T.);
#70153=ORIENTED_EDGE('',*,*,#51108,.T.);
#70154=ORIENTED_EDGE('',*,*,#51111,.T.);
#70155=ORIENTED_EDGE('',*,*,#51113,.T.);
#70156=ORIENTED_EDGE('',*,*,#51116,.T.);
#70157=ORIENTED_EDGE('',*,*,#51120,.T.);
#70158=ORIENTED_EDGE('',*,*,#51123,.T.);
#70159=ORIENTED_EDGE('',*,*,#51125,.T.);
#70160=ORIENTED_EDGE('',*,*,#51128,.T.);
#70161=ORIENTED_EDGE('',*,*,#51132,.T.);
#70162=ORIENTED_EDGE('',*,*,#51135,.T.);
#70163=ORIENTED_EDGE('',*,*,#51137,.T.);
#70164=ORIENTED_EDGE('',*,*,#51140,.T.);
#70165=ORIENTED_EDGE('',*,*,#51144,.T.);
#70166=ORIENTED_EDGE('',*,*,#51147,.T.);
#70167=ORIENTED_EDGE('',*,*,#51149,.T.);
#70168=ORIENTED_EDGE('',*,*,#51152,.T.);
#70169=ORIENTED_EDGE('',*,*,#51156,.T.);
#70170=ORIENTED_EDGE('',*,*,#51159,.T.);
#70171=ORIENTED_EDGE('',*,*,#51161,.T.);
#70172=ORIENTED_EDGE('',*,*,#51164,.T.);
#70173=ORIENTED_EDGE('',*,*,#51168,.T.);
#70174=ORIENTED_EDGE('',*,*,#51171,.T.);
#70175=ORIENTED_EDGE('',*,*,#51173,.T.);
#70176=ORIENTED_EDGE('',*,*,#51176,.T.);
#70177=ORIENTED_EDGE('',*,*,#51180,.T.);
#70178=ORIENTED_EDGE('',*,*,#51183,.T.);
#70179=ORIENTED_EDGE('',*,*,#51185,.T.);
#70180=ORIENTED_EDGE('',*,*,#51188,.T.);
#70181=ORIENTED_EDGE('',*,*,#51192,.T.);
#70182=ORIENTED_EDGE('',*,*,#51195,.T.);
#70183=ORIENTED_EDGE('',*,*,#51197,.T.);
#70184=ORIENTED_EDGE('',*,*,#51200,.T.);
#70185=ORIENTED_EDGE('',*,*,#51204,.T.);
#70186=ORIENTED_EDGE('',*,*,#51207,.T.);
#70187=ORIENTED_EDGE('',*,*,#51209,.T.);
#70188=ORIENTED_EDGE('',*,*,#51212,.T.);
#70189=ORIENTED_EDGE('',*,*,#51216,.T.);
#70190=ORIENTED_EDGE('',*,*,#51219,.T.);
#70191=ORIENTED_EDGE('',*,*,#51221,.T.);
#70192=ORIENTED_EDGE('',*,*,#51224,.T.);
#70193=ORIENTED_EDGE('',*,*,#51228,.T.);
#70194=ORIENTED_EDGE('',*,*,#51231,.T.);
#70195=ORIENTED_EDGE('',*,*,#51233,.T.);
#70196=ORIENTED_EDGE('',*,*,#51236,.T.);
#70197=ORIENTED_EDGE('',*,*,#51240,.T.);
#70198=ORIENTED_EDGE('',*,*,#51243,.T.);
#70199=ORIENTED_EDGE('',*,*,#51245,.T.);
#70200=ORIENTED_EDGE('',*,*,#51248,.T.);
#70201=ORIENTED_EDGE('',*,*,#51252,.T.);
#70202=ORIENTED_EDGE('',*,*,#51255,.T.);
#70203=ORIENTED_EDGE('',*,*,#51257,.T.);
#70204=ORIENTED_EDGE('',*,*,#51260,.T.);
#70205=ORIENTED_EDGE('',*,*,#51264,.T.);
#70206=ORIENTED_EDGE('',*,*,#51267,.T.);
#70207=ORIENTED_EDGE('',*,*,#51269,.T.);
#70208=ORIENTED_EDGE('',*,*,#51272,.T.);
#70209=ORIENTED_EDGE('',*,*,#51276,.T.);
#70210=ORIENTED_EDGE('',*,*,#51279,.T.);
#70211=ORIENTED_EDGE('',*,*,#51281,.T.);
#70212=ORIENTED_EDGE('',*,*,#51284,.T.);
#70213=ORIENTED_EDGE('',*,*,#51288,.T.);
#70214=ORIENTED_EDGE('',*,*,#51291,.T.);
#70215=ORIENTED_EDGE('',*,*,#51293,.T.);
#70216=ORIENTED_EDGE('',*,*,#51296,.T.);
#70217=ORIENTED_EDGE('',*,*,#51300,.T.);
#70218=ORIENTED_EDGE('',*,*,#51303,.T.);
#70219=ORIENTED_EDGE('',*,*,#51305,.T.);
#70220=ORIENTED_EDGE('',*,*,#51308,.T.);
#70221=ORIENTED_EDGE('',*,*,#51312,.T.);
#70222=ORIENTED_EDGE('',*,*,#51315,.T.);
#70223=ORIENTED_EDGE('',*,*,#51317,.T.);
#70224=ORIENTED_EDGE('',*,*,#51320,.T.);
#70225=ORIENTED_EDGE('',*,*,#51324,.T.);
#70226=ORIENTED_EDGE('',*,*,#51327,.T.);
#70227=ORIENTED_EDGE('',*,*,#51329,.T.);
#70228=ORIENTED_EDGE('',*,*,#51332,.T.);
#70229=ORIENTED_EDGE('',*,*,#51336,.T.);
#70230=ORIENTED_EDGE('',*,*,#51339,.T.);
#70231=ORIENTED_EDGE('',*,*,#51341,.T.);
#70232=ORIENTED_EDGE('',*,*,#51344,.T.);
#70233=ORIENTED_EDGE('',*,*,#51348,.T.);
#70234=ORIENTED_EDGE('',*,*,#51351,.T.);
#70235=ORIENTED_EDGE('',*,*,#51353,.T.);
#70236=ORIENTED_EDGE('',*,*,#51356,.T.);
#70237=ORIENTED_EDGE('',*,*,#51360,.T.);
#70238=ORIENTED_EDGE('',*,*,#51363,.T.);
#70239=ORIENTED_EDGE('',*,*,#51365,.T.);
#70240=ORIENTED_EDGE('',*,*,#51368,.T.);
#70241=ORIENTED_EDGE('',*,*,#51372,.T.);
#70242=ORIENTED_EDGE('',*,*,#51375,.T.);
#70243=ORIENTED_EDGE('',*,*,#51377,.T.);
#70244=ORIENTED_EDGE('',*,*,#51380,.T.);
#70245=ORIENTED_EDGE('',*,*,#51384,.T.);
#70246=ORIENTED_EDGE('',*,*,#51387,.T.);
#70247=ORIENTED_EDGE('',*,*,#51389,.T.);
#70248=ORIENTED_EDGE('',*,*,#51392,.T.);
#70249=ORIENTED_EDGE('',*,*,#51396,.T.);
#70250=ORIENTED_EDGE('',*,*,#51399,.T.);
#70251=ORIENTED_EDGE('',*,*,#51401,.T.);
#70252=ORIENTED_EDGE('',*,*,#51404,.T.);
#70253=ORIENTED_EDGE('',*,*,#51408,.T.);
#70254=ORIENTED_EDGE('',*,*,#51411,.T.);
#70255=ORIENTED_EDGE('',*,*,#51413,.T.);
#70256=ORIENTED_EDGE('',*,*,#51416,.T.);
#70257=ORIENTED_EDGE('',*,*,#51420,.T.);
#70258=ORIENTED_EDGE('',*,*,#51423,.T.);
#70259=ORIENTED_EDGE('',*,*,#51425,.T.);
#70260=ORIENTED_EDGE('',*,*,#51428,.T.);
#70261=ORIENTED_EDGE('',*,*,#51432,.T.);
#70262=ORIENTED_EDGE('',*,*,#51435,.T.);
#70263=ORIENTED_EDGE('',*,*,#51437,.T.);
#70264=ORIENTED_EDGE('',*,*,#51440,.T.);
#70265=ORIENTED_EDGE('',*,*,#51444,.T.);
#70266=ORIENTED_EDGE('',*,*,#51447,.T.);
#70267=ORIENTED_EDGE('',*,*,#51449,.T.);
#70268=ORIENTED_EDGE('',*,*,#51452,.T.);
#70269=ORIENTED_EDGE('',*,*,#51456,.T.);
#70270=ORIENTED_EDGE('',*,*,#51459,.T.);
#70271=ORIENTED_EDGE('',*,*,#51461,.T.);
#70272=ORIENTED_EDGE('',*,*,#51464,.T.);
#70273=ORIENTED_EDGE('',*,*,#51468,.T.);
#70274=ORIENTED_EDGE('',*,*,#51471,.T.);
#70275=ORIENTED_EDGE('',*,*,#51473,.T.);
#70276=ORIENTED_EDGE('',*,*,#51476,.T.);
#70277=ORIENTED_EDGE('',*,*,#51480,.T.);
#70278=ORIENTED_EDGE('',*,*,#51483,.T.);
#70279=ORIENTED_EDGE('',*,*,#51485,.T.);
#70280=ORIENTED_EDGE('',*,*,#51488,.T.);
#70281=ORIENTED_EDGE('',*,*,#51492,.T.);
#70282=ORIENTED_EDGE('',*,*,#51495,.T.);
#70283=ORIENTED_EDGE('',*,*,#51497,.T.);
#70284=ORIENTED_EDGE('',*,*,#51500,.T.);
#70285=ORIENTED_EDGE('',*,*,#51504,.T.);
#70286=ORIENTED_EDGE('',*,*,#51507,.T.);
#70287=ORIENTED_EDGE('',*,*,#51509,.T.);
#70288=ORIENTED_EDGE('',*,*,#51512,.T.);
#70289=ORIENTED_EDGE('',*,*,#51516,.T.);
#70290=ORIENTED_EDGE('',*,*,#51519,.T.);
#70291=ORIENTED_EDGE('',*,*,#51521,.T.);
#70292=ORIENTED_EDGE('',*,*,#51524,.T.);
#70293=ORIENTED_EDGE('',*,*,#51528,.T.);
#70294=ORIENTED_EDGE('',*,*,#51531,.T.);
#70295=ORIENTED_EDGE('',*,*,#51533,.T.);
#70296=ORIENTED_EDGE('',*,*,#51536,.T.);
#70297=ORIENTED_EDGE('',*,*,#51540,.T.);
#70298=ORIENTED_EDGE('',*,*,#51543,.T.);
#70299=ORIENTED_EDGE('',*,*,#51545,.T.);
#70300=ORIENTED_EDGE('',*,*,#51548,.T.);
#70301=ORIENTED_EDGE('',*,*,#51552,.T.);
#70302=ORIENTED_EDGE('',*,*,#51555,.T.);
#70303=ORIENTED_EDGE('',*,*,#51557,.T.);
#70304=ORIENTED_EDGE('',*,*,#51560,.T.);
#70305=ORIENTED_EDGE('',*,*,#51564,.T.);
#70306=ORIENTED_EDGE('',*,*,#51567,.T.);
#70307=ORIENTED_EDGE('',*,*,#51569,.T.);
#70308=ORIENTED_EDGE('',*,*,#51572,.T.);
#70309=ORIENTED_EDGE('',*,*,#51576,.T.);
#70310=ORIENTED_EDGE('',*,*,#51579,.T.);
#70311=ORIENTED_EDGE('',*,*,#51581,.T.);
#70312=ORIENTED_EDGE('',*,*,#51584,.T.);
#70313=ORIENTED_EDGE('',*,*,#51588,.T.);
#70314=ORIENTED_EDGE('',*,*,#51591,.T.);
#70315=ORIENTED_EDGE('',*,*,#51593,.T.);
#70316=ORIENTED_EDGE('',*,*,#51596,.T.);
#70317=ORIENTED_EDGE('',*,*,#51600,.T.);
#70318=ORIENTED_EDGE('',*,*,#51603,.T.);
#70319=ORIENTED_EDGE('',*,*,#51605,.T.);
#70320=ORIENTED_EDGE('',*,*,#51608,.T.);
#70321=ORIENTED_EDGE('',*,*,#51612,.T.);
#70322=ORIENTED_EDGE('',*,*,#51615,.T.);
#70323=ORIENTED_EDGE('',*,*,#51617,.T.);
#70324=ORIENTED_EDGE('',*,*,#51620,.T.);
#70325=ORIENTED_EDGE('',*,*,#51624,.T.);
#70326=ORIENTED_EDGE('',*,*,#51627,.T.);
#70327=ORIENTED_EDGE('',*,*,#51629,.T.);
#70328=ORIENTED_EDGE('',*,*,#51632,.T.);
#70329=ORIENTED_EDGE('',*,*,#51636,.T.);
#70330=ORIENTED_EDGE('',*,*,#51639,.T.);
#70331=ORIENTED_EDGE('',*,*,#51641,.T.);
#70332=ORIENTED_EDGE('',*,*,#51644,.T.);
#70333=ORIENTED_EDGE('',*,*,#51648,.T.);
#70334=ORIENTED_EDGE('',*,*,#51651,.T.);
#70335=ORIENTED_EDGE('',*,*,#51653,.T.);
#70336=ORIENTED_EDGE('',*,*,#51656,.T.);
#70337=ORIENTED_EDGE('',*,*,#51660,.T.);
#70338=ORIENTED_EDGE('',*,*,#51663,.T.);
#70339=ORIENTED_EDGE('',*,*,#51665,.T.);
#70340=ORIENTED_EDGE('',*,*,#51668,.T.);
#70341=ORIENTED_EDGE('',*,*,#51672,.T.);
#70342=ORIENTED_EDGE('',*,*,#51675,.T.);
#70343=ORIENTED_EDGE('',*,*,#51677,.T.);
#70344=ORIENTED_EDGE('',*,*,#51680,.T.);
#70345=ORIENTED_EDGE('',*,*,#51684,.T.);
#70346=ORIENTED_EDGE('',*,*,#51687,.T.);
#70347=ORIENTED_EDGE('',*,*,#51689,.T.);
#70348=ORIENTED_EDGE('',*,*,#51692,.T.);
#70349=ORIENTED_EDGE('',*,*,#51696,.T.);
#70350=ORIENTED_EDGE('',*,*,#51699,.T.);
#70351=ORIENTED_EDGE('',*,*,#51701,.T.);
#70352=ORIENTED_EDGE('',*,*,#51704,.T.);
#70353=ORIENTED_EDGE('',*,*,#51708,.T.);
#70354=ORIENTED_EDGE('',*,*,#51711,.T.);
#70355=ORIENTED_EDGE('',*,*,#51713,.T.);
#70356=ORIENTED_EDGE('',*,*,#51716,.T.);
#70357=ORIENTED_EDGE('',*,*,#51720,.T.);
#70358=ORIENTED_EDGE('',*,*,#51723,.T.);
#70359=ORIENTED_EDGE('',*,*,#51725,.T.);
#70360=ORIENTED_EDGE('',*,*,#51728,.T.);
#70361=ORIENTED_EDGE('',*,*,#51732,.T.);
#70362=ORIENTED_EDGE('',*,*,#51735,.T.);
#70363=ORIENTED_EDGE('',*,*,#51737,.T.);
#70364=ORIENTED_EDGE('',*,*,#51740,.T.);
#70365=ORIENTED_EDGE('',*,*,#51744,.T.);
#70366=ORIENTED_EDGE('',*,*,#51747,.T.);
#70367=ORIENTED_EDGE('',*,*,#51749,.T.);
#70368=ORIENTED_EDGE('',*,*,#51752,.T.);
#70369=ORIENTED_EDGE('',*,*,#51756,.T.);
#70370=ORIENTED_EDGE('',*,*,#51759,.T.);
#70371=ORIENTED_EDGE('',*,*,#51761,.T.);
#70372=ORIENTED_EDGE('',*,*,#51764,.T.);
#70373=ORIENTED_EDGE('',*,*,#51768,.T.);
#70374=ORIENTED_EDGE('',*,*,#51771,.T.);
#70375=ORIENTED_EDGE('',*,*,#51773,.T.);
#70376=ORIENTED_EDGE('',*,*,#51776,.T.);
#70377=ORIENTED_EDGE('',*,*,#51780,.T.);
#70378=ORIENTED_EDGE('',*,*,#51783,.T.);
#70379=ORIENTED_EDGE('',*,*,#51785,.T.);
#70380=ORIENTED_EDGE('',*,*,#51788,.T.);
#70381=ORIENTED_EDGE('',*,*,#51792,.T.);
#70382=ORIENTED_EDGE('',*,*,#51795,.T.);
#70383=ORIENTED_EDGE('',*,*,#51797,.T.);
#70384=ORIENTED_EDGE('',*,*,#51800,.T.);
#70385=ORIENTED_EDGE('',*,*,#51804,.T.);
#70386=ORIENTED_EDGE('',*,*,#51807,.T.);
#70387=ORIENTED_EDGE('',*,*,#51809,.T.);
#70388=ORIENTED_EDGE('',*,*,#51812,.T.);
#70389=ORIENTED_EDGE('',*,*,#51816,.T.);
#70390=ORIENTED_EDGE('',*,*,#51819,.T.);
#70391=ORIENTED_EDGE('',*,*,#51821,.T.);
#70392=ORIENTED_EDGE('',*,*,#51824,.T.);
#70393=ORIENTED_EDGE('',*,*,#51828,.T.);
#70394=ORIENTED_EDGE('',*,*,#51831,.T.);
#70395=ORIENTED_EDGE('',*,*,#51833,.T.);
#70396=ORIENTED_EDGE('',*,*,#51836,.T.);
#70397=ORIENTED_EDGE('',*,*,#51840,.T.);
#70398=ORIENTED_EDGE('',*,*,#51843,.T.);
#70399=ORIENTED_EDGE('',*,*,#51845,.T.);
#70400=ORIENTED_EDGE('',*,*,#51848,.T.);
#70401=ORIENTED_EDGE('',*,*,#51852,.T.);
#70402=ORIENTED_EDGE('',*,*,#51855,.T.);
#70403=ORIENTED_EDGE('',*,*,#51857,.T.);
#70404=ORIENTED_EDGE('',*,*,#51860,.T.);
#70405=ORIENTED_EDGE('',*,*,#51864,.T.);
#70406=ORIENTED_EDGE('',*,*,#51867,.T.);
#70407=ORIENTED_EDGE('',*,*,#51869,.T.);
#70408=ORIENTED_EDGE('',*,*,#51872,.T.);
#70409=ORIENTED_EDGE('',*,*,#51876,.T.);
#70410=ORIENTED_EDGE('',*,*,#51879,.T.);
#70411=ORIENTED_EDGE('',*,*,#51881,.T.);
#70412=ORIENTED_EDGE('',*,*,#51884,.T.);
#70413=ORIENTED_EDGE('',*,*,#51888,.T.);
#70414=ORIENTED_EDGE('',*,*,#51891,.T.);
#70415=ORIENTED_EDGE('',*,*,#51893,.T.);
#70416=ORIENTED_EDGE('',*,*,#51896,.T.);
#70417=ORIENTED_EDGE('',*,*,#51900,.T.);
#70418=ORIENTED_EDGE('',*,*,#51903,.T.);
#70419=ORIENTED_EDGE('',*,*,#51905,.T.);
#70420=ORIENTED_EDGE('',*,*,#51908,.T.);
#70421=ORIENTED_EDGE('',*,*,#51912,.T.);
#70422=ORIENTED_EDGE('',*,*,#51915,.T.);
#70423=ORIENTED_EDGE('',*,*,#51917,.T.);
#70424=ORIENTED_EDGE('',*,*,#51920,.T.);
#70425=ORIENTED_EDGE('',*,*,#51924,.T.);
#70426=ORIENTED_EDGE('',*,*,#51927,.T.);
#70427=ORIENTED_EDGE('',*,*,#51929,.T.);
#70428=ORIENTED_EDGE('',*,*,#51932,.T.);
#70429=ORIENTED_EDGE('',*,*,#51936,.T.);
#70430=ORIENTED_EDGE('',*,*,#51939,.T.);
#70431=ORIENTED_EDGE('',*,*,#51941,.T.);
#70432=ORIENTED_EDGE('',*,*,#51944,.T.);
#70433=ORIENTED_EDGE('',*,*,#51948,.T.);
#70434=ORIENTED_EDGE('',*,*,#51951,.T.);
#70435=ORIENTED_EDGE('',*,*,#51953,.T.);
#70436=ORIENTED_EDGE('',*,*,#51956,.T.);
#70437=ORIENTED_EDGE('',*,*,#51960,.T.);
#70438=ORIENTED_EDGE('',*,*,#51963,.T.);
#70439=ORIENTED_EDGE('',*,*,#51965,.T.);
#70440=ORIENTED_EDGE('',*,*,#51967,.T.);
#70441=ORIENTED_EDGE('',*,*,#51968,.T.);
#70442=ORIENTED_EDGE('',*,*,#51969,.T.);
#70443=ORIENTED_EDGE('',*,*,#51970,.T.);
#70444=ORIENTED_EDGE('',*,*,#51971,.T.);
#70445=ORIENTED_EDGE('',*,*,#51967,.F.);
#70446=ORIENTED_EDGE('',*,*,#51972,.F.);
#70447=ORIENTED_EDGE('',*,*,#51973,.T.);
#70448=ORIENTED_EDGE('',*,*,#51974,.T.);
#70449=ORIENTED_EDGE('',*,*,#51968,.F.);
#70450=ORIENTED_EDGE('',*,*,#51971,.F.);
#70451=ORIENTED_EDGE('',*,*,#51975,.T.);
#70452=ORIENTED_EDGE('',*,*,#51976,.T.);
#70453=ORIENTED_EDGE('',*,*,#51969,.F.);
#70454=ORIENTED_EDGE('',*,*,#51974,.F.);
#70455=ORIENTED_EDGE('',*,*,#51977,.T.);
#70456=ORIENTED_EDGE('',*,*,#51972,.T.);
#70457=ORIENTED_EDGE('',*,*,#51970,.F.);
#70458=ORIENTED_EDGE('',*,*,#51976,.F.);
#70459=ORIENTED_EDGE('',*,*,#51978,.T.);
#70460=ORIENTED_EDGE('',*,*,#43493,.F.);
#70461=ORIENTED_EDGE('',*,*,#46744,.F.);
#70462=ORIENTED_EDGE('',*,*,#46741,.F.);
#70463=ORIENTED_EDGE('',*,*,#46738,.F.);
#70464=ORIENTED_EDGE('',*,*,#46746,.F.);
#70465=ORIENTED_EDGE('',*,*,#46756,.F.);
#70466=ORIENTED_EDGE('',*,*,#46753,.F.);
#70467=ORIENTED_EDGE('',*,*,#46750,.F.);
#70468=ORIENTED_EDGE('',*,*,#46758,.F.);
#70469=ORIENTED_EDGE('',*,*,#46768,.F.);
#70470=ORIENTED_EDGE('',*,*,#46765,.F.);
#70471=ORIENTED_EDGE('',*,*,#46762,.F.);
#70472=ORIENTED_EDGE('',*,*,#46770,.F.);
#70473=ORIENTED_EDGE('',*,*,#46780,.F.);
#70474=ORIENTED_EDGE('',*,*,#46777,.F.);
#70475=ORIENTED_EDGE('',*,*,#46774,.F.);
#70476=ORIENTED_EDGE('',*,*,#46782,.F.);
#70477=ORIENTED_EDGE('',*,*,#46792,.F.);
#70478=ORIENTED_EDGE('',*,*,#46789,.F.);
#70479=ORIENTED_EDGE('',*,*,#46786,.F.);
#70480=ORIENTED_EDGE('',*,*,#46794,.F.);
#70481=ORIENTED_EDGE('',*,*,#46804,.F.);
#70482=ORIENTED_EDGE('',*,*,#46801,.F.);
#70483=ORIENTED_EDGE('',*,*,#46798,.F.);
#70484=ORIENTED_EDGE('',*,*,#46806,.F.);
#70485=ORIENTED_EDGE('',*,*,#46816,.F.);
#70486=ORIENTED_EDGE('',*,*,#46813,.F.);
#70487=ORIENTED_EDGE('',*,*,#46810,.F.);
#70488=ORIENTED_EDGE('',*,*,#46818,.F.);
#70489=ORIENTED_EDGE('',*,*,#46828,.F.);
#70490=ORIENTED_EDGE('',*,*,#46825,.F.);
#70491=ORIENTED_EDGE('',*,*,#46822,.F.);
#70492=ORIENTED_EDGE('',*,*,#46830,.F.);
#70493=ORIENTED_EDGE('',*,*,#46840,.F.);
#70494=ORIENTED_EDGE('',*,*,#46837,.F.);
#70495=ORIENTED_EDGE('',*,*,#46834,.F.);
#70496=ORIENTED_EDGE('',*,*,#46842,.F.);
#70497=ORIENTED_EDGE('',*,*,#46852,.F.);
#70498=ORIENTED_EDGE('',*,*,#46849,.F.);
#70499=ORIENTED_EDGE('',*,*,#46846,.F.);
#70500=ORIENTED_EDGE('',*,*,#46854,.F.);
#70501=ORIENTED_EDGE('',*,*,#46864,.F.);
#70502=ORIENTED_EDGE('',*,*,#46861,.F.);
#70503=ORIENTED_EDGE('',*,*,#46858,.F.);
#70504=ORIENTED_EDGE('',*,*,#46866,.F.);
#70505=ORIENTED_EDGE('',*,*,#46876,.F.);
#70506=ORIENTED_EDGE('',*,*,#46873,.F.);
#70507=ORIENTED_EDGE('',*,*,#46870,.F.);
#70508=ORIENTED_EDGE('',*,*,#46878,.F.);
#70509=ORIENTED_EDGE('',*,*,#46888,.F.);
#70510=ORIENTED_EDGE('',*,*,#46885,.F.);
#70511=ORIENTED_EDGE('',*,*,#46882,.F.);
#70512=ORIENTED_EDGE('',*,*,#46890,.F.);
#70513=ORIENTED_EDGE('',*,*,#46900,.F.);
#70514=ORIENTED_EDGE('',*,*,#46897,.F.);
#70515=ORIENTED_EDGE('',*,*,#46894,.F.);
#70516=ORIENTED_EDGE('',*,*,#46902,.F.);
#70517=ORIENTED_EDGE('',*,*,#46912,.F.);
#70518=ORIENTED_EDGE('',*,*,#46909,.F.);
#70519=ORIENTED_EDGE('',*,*,#46906,.F.);
#70520=ORIENTED_EDGE('',*,*,#46914,.F.);
#70521=ORIENTED_EDGE('',*,*,#46924,.F.);
#70522=ORIENTED_EDGE('',*,*,#46921,.F.);
#70523=ORIENTED_EDGE('',*,*,#46918,.F.);
#70524=ORIENTED_EDGE('',*,*,#46926,.F.);
#70525=ORIENTED_EDGE('',*,*,#46936,.F.);
#70526=ORIENTED_EDGE('',*,*,#46933,.F.);
#70527=ORIENTED_EDGE('',*,*,#46930,.F.);
#70528=ORIENTED_EDGE('',*,*,#46938,.F.);
#70529=ORIENTED_EDGE('',*,*,#46948,.F.);
#70530=ORIENTED_EDGE('',*,*,#46945,.F.);
#70531=ORIENTED_EDGE('',*,*,#46942,.F.);
#70532=ORIENTED_EDGE('',*,*,#46950,.F.);
#70533=ORIENTED_EDGE('',*,*,#46960,.F.);
#70534=ORIENTED_EDGE('',*,*,#46957,.F.);
#70535=ORIENTED_EDGE('',*,*,#46954,.F.);
#70536=ORIENTED_EDGE('',*,*,#46962,.F.);
#70537=ORIENTED_EDGE('',*,*,#46972,.F.);
#70538=ORIENTED_EDGE('',*,*,#46969,.F.);
#70539=ORIENTED_EDGE('',*,*,#46966,.F.);
#70540=ORIENTED_EDGE('',*,*,#46974,.F.);
#70541=ORIENTED_EDGE('',*,*,#46984,.F.);
#70542=ORIENTED_EDGE('',*,*,#46981,.F.);
#70543=ORIENTED_EDGE('',*,*,#46978,.F.);
#70544=ORIENTED_EDGE('',*,*,#46986,.F.);
#70545=ORIENTED_EDGE('',*,*,#46996,.F.);
#70546=ORIENTED_EDGE('',*,*,#46993,.F.);
#70547=ORIENTED_EDGE('',*,*,#46990,.F.);
#70548=ORIENTED_EDGE('',*,*,#46998,.F.);
#70549=ORIENTED_EDGE('',*,*,#47008,.F.);
#70550=ORIENTED_EDGE('',*,*,#47005,.F.);
#70551=ORIENTED_EDGE('',*,*,#47002,.F.);
#70552=ORIENTED_EDGE('',*,*,#47010,.F.);
#70553=ORIENTED_EDGE('',*,*,#47020,.F.);
#70554=ORIENTED_EDGE('',*,*,#47017,.F.);
#70555=ORIENTED_EDGE('',*,*,#47014,.F.);
#70556=ORIENTED_EDGE('',*,*,#47022,.F.);
#70557=ORIENTED_EDGE('',*,*,#47032,.F.);
#70558=ORIENTED_EDGE('',*,*,#47029,.F.);
#70559=ORIENTED_EDGE('',*,*,#47026,.F.);
#70560=ORIENTED_EDGE('',*,*,#47034,.F.);
#70561=ORIENTED_EDGE('',*,*,#47044,.F.);
#70562=ORIENTED_EDGE('',*,*,#47041,.F.);
#70563=ORIENTED_EDGE('',*,*,#47038,.F.);
#70564=ORIENTED_EDGE('',*,*,#47046,.F.);
#70565=ORIENTED_EDGE('',*,*,#47056,.F.);
#70566=ORIENTED_EDGE('',*,*,#47053,.F.);
#70567=ORIENTED_EDGE('',*,*,#47050,.F.);
#70568=ORIENTED_EDGE('',*,*,#47058,.F.);
#70569=ORIENTED_EDGE('',*,*,#47068,.F.);
#70570=ORIENTED_EDGE('',*,*,#47065,.F.);
#70571=ORIENTED_EDGE('',*,*,#47062,.F.);
#70572=ORIENTED_EDGE('',*,*,#47070,.F.);
#70573=ORIENTED_EDGE('',*,*,#47080,.F.);
#70574=ORIENTED_EDGE('',*,*,#47077,.F.);
#70575=ORIENTED_EDGE('',*,*,#47074,.F.);
#70576=ORIENTED_EDGE('',*,*,#47082,.F.);
#70577=ORIENTED_EDGE('',*,*,#47092,.F.);
#70578=ORIENTED_EDGE('',*,*,#47089,.F.);
#70579=ORIENTED_EDGE('',*,*,#47086,.F.);
#70580=ORIENTED_EDGE('',*,*,#47094,.F.);
#70581=ORIENTED_EDGE('',*,*,#47104,.F.);
#70582=ORIENTED_EDGE('',*,*,#47101,.F.);
#70583=ORIENTED_EDGE('',*,*,#47098,.F.);
#70584=ORIENTED_EDGE('',*,*,#47106,.F.);
#70585=ORIENTED_EDGE('',*,*,#47116,.F.);
#70586=ORIENTED_EDGE('',*,*,#47113,.F.);
#70587=ORIENTED_EDGE('',*,*,#47110,.F.);
#70588=ORIENTED_EDGE('',*,*,#47118,.F.);
#70589=ORIENTED_EDGE('',*,*,#47128,.F.);
#70590=ORIENTED_EDGE('',*,*,#47125,.F.);
#70591=ORIENTED_EDGE('',*,*,#47122,.F.);
#70592=ORIENTED_EDGE('',*,*,#47130,.F.);
#70593=ORIENTED_EDGE('',*,*,#47140,.F.);
#70594=ORIENTED_EDGE('',*,*,#47137,.F.);
#70595=ORIENTED_EDGE('',*,*,#47134,.F.);
#70596=ORIENTED_EDGE('',*,*,#47142,.F.);
#70597=ORIENTED_EDGE('',*,*,#47152,.F.);
#70598=ORIENTED_EDGE('',*,*,#47149,.F.);
#70599=ORIENTED_EDGE('',*,*,#47146,.F.);
#70600=ORIENTED_EDGE('',*,*,#47154,.F.);
#70601=ORIENTED_EDGE('',*,*,#47164,.F.);
#70602=ORIENTED_EDGE('',*,*,#47161,.F.);
#70603=ORIENTED_EDGE('',*,*,#47158,.F.);
#70604=ORIENTED_EDGE('',*,*,#47166,.F.);
#70605=ORIENTED_EDGE('',*,*,#47176,.F.);
#70606=ORIENTED_EDGE('',*,*,#47173,.F.);
#70607=ORIENTED_EDGE('',*,*,#47170,.F.);
#70608=ORIENTED_EDGE('',*,*,#47178,.F.);
#70609=ORIENTED_EDGE('',*,*,#47188,.F.);
#70610=ORIENTED_EDGE('',*,*,#47185,.F.);
#70611=ORIENTED_EDGE('',*,*,#47182,.F.);
#70612=ORIENTED_EDGE('',*,*,#47190,.F.);
#70613=ORIENTED_EDGE('',*,*,#47200,.F.);
#70614=ORIENTED_EDGE('',*,*,#47197,.F.);
#70615=ORIENTED_EDGE('',*,*,#47194,.F.);
#70616=ORIENTED_EDGE('',*,*,#47202,.F.);
#70617=ORIENTED_EDGE('',*,*,#47212,.F.);
#70618=ORIENTED_EDGE('',*,*,#47209,.F.);
#70619=ORIENTED_EDGE('',*,*,#47206,.F.);
#70620=ORIENTED_EDGE('',*,*,#47214,.F.);
#70621=ORIENTED_EDGE('',*,*,#47224,.F.);
#70622=ORIENTED_EDGE('',*,*,#47221,.F.);
#70623=ORIENTED_EDGE('',*,*,#47218,.F.);
#70624=ORIENTED_EDGE('',*,*,#47226,.F.);
#70625=ORIENTED_EDGE('',*,*,#47236,.F.);
#70626=ORIENTED_EDGE('',*,*,#47233,.F.);
#70627=ORIENTED_EDGE('',*,*,#47230,.F.);
#70628=ORIENTED_EDGE('',*,*,#47238,.F.);
#70629=ORIENTED_EDGE('',*,*,#47248,.F.);
#70630=ORIENTED_EDGE('',*,*,#47245,.F.);
#70631=ORIENTED_EDGE('',*,*,#47242,.F.);
#70632=ORIENTED_EDGE('',*,*,#47250,.F.);
#70633=ORIENTED_EDGE('',*,*,#47260,.F.);
#70634=ORIENTED_EDGE('',*,*,#47257,.F.);
#70635=ORIENTED_EDGE('',*,*,#47254,.F.);
#70636=ORIENTED_EDGE('',*,*,#47262,.F.);
#70637=ORIENTED_EDGE('',*,*,#47272,.F.);
#70638=ORIENTED_EDGE('',*,*,#47269,.F.);
#70639=ORIENTED_EDGE('',*,*,#47266,.F.);
#70640=ORIENTED_EDGE('',*,*,#47274,.F.);
#70641=ORIENTED_EDGE('',*,*,#47284,.F.);
#70642=ORIENTED_EDGE('',*,*,#47281,.F.);
#70643=ORIENTED_EDGE('',*,*,#47278,.F.);
#70644=ORIENTED_EDGE('',*,*,#47286,.F.);
#70645=ORIENTED_EDGE('',*,*,#47296,.F.);
#70646=ORIENTED_EDGE('',*,*,#47293,.F.);
#70647=ORIENTED_EDGE('',*,*,#47290,.F.);
#70648=ORIENTED_EDGE('',*,*,#47298,.F.);
#70649=ORIENTED_EDGE('',*,*,#47308,.F.);
#70650=ORIENTED_EDGE('',*,*,#47305,.F.);
#70651=ORIENTED_EDGE('',*,*,#47302,.F.);
#70652=ORIENTED_EDGE('',*,*,#47310,.F.);
#70653=ORIENTED_EDGE('',*,*,#47320,.F.);
#70654=ORIENTED_EDGE('',*,*,#47317,.F.);
#70655=ORIENTED_EDGE('',*,*,#47314,.F.);
#70656=ORIENTED_EDGE('',*,*,#47322,.F.);
#70657=ORIENTED_EDGE('',*,*,#47332,.F.);
#70658=ORIENTED_EDGE('',*,*,#47329,.F.);
#70659=ORIENTED_EDGE('',*,*,#47326,.F.);
#70660=ORIENTED_EDGE('',*,*,#47334,.F.);
#70661=ORIENTED_EDGE('',*,*,#47344,.F.);
#70662=ORIENTED_EDGE('',*,*,#47341,.F.);
#70663=ORIENTED_EDGE('',*,*,#47338,.F.);
#70664=ORIENTED_EDGE('',*,*,#47346,.F.);
#70665=ORIENTED_EDGE('',*,*,#47356,.F.);
#70666=ORIENTED_EDGE('',*,*,#47353,.F.);
#70667=ORIENTED_EDGE('',*,*,#47350,.F.);
#70668=ORIENTED_EDGE('',*,*,#47358,.F.);
#70669=ORIENTED_EDGE('',*,*,#47368,.F.);
#70670=ORIENTED_EDGE('',*,*,#47365,.F.);
#70671=ORIENTED_EDGE('',*,*,#47362,.F.);
#70672=ORIENTED_EDGE('',*,*,#47370,.F.);
#70673=ORIENTED_EDGE('',*,*,#47380,.F.);
#70674=ORIENTED_EDGE('',*,*,#47377,.F.);
#70675=ORIENTED_EDGE('',*,*,#47374,.F.);
#70676=ORIENTED_EDGE('',*,*,#47382,.F.);
#70677=ORIENTED_EDGE('',*,*,#47392,.F.);
#70678=ORIENTED_EDGE('',*,*,#47389,.F.);
#70679=ORIENTED_EDGE('',*,*,#47386,.F.);
#70680=ORIENTED_EDGE('',*,*,#47394,.F.);
#70681=ORIENTED_EDGE('',*,*,#47404,.F.);
#70682=ORIENTED_EDGE('',*,*,#47401,.F.);
#70683=ORIENTED_EDGE('',*,*,#47398,.F.);
#70684=ORIENTED_EDGE('',*,*,#47406,.F.);
#70685=ORIENTED_EDGE('',*,*,#47416,.F.);
#70686=ORIENTED_EDGE('',*,*,#47413,.F.);
#70687=ORIENTED_EDGE('',*,*,#47410,.F.);
#70688=ORIENTED_EDGE('',*,*,#47418,.F.);
#70689=ORIENTED_EDGE('',*,*,#47428,.F.);
#70690=ORIENTED_EDGE('',*,*,#47425,.F.);
#70691=ORIENTED_EDGE('',*,*,#47422,.F.);
#70692=ORIENTED_EDGE('',*,*,#47430,.F.);
#70693=ORIENTED_EDGE('',*,*,#47440,.F.);
#70694=ORIENTED_EDGE('',*,*,#47437,.F.);
#70695=ORIENTED_EDGE('',*,*,#47434,.F.);
#70696=ORIENTED_EDGE('',*,*,#47442,.F.);
#70697=ORIENTED_EDGE('',*,*,#47452,.F.);
#70698=ORIENTED_EDGE('',*,*,#47449,.F.);
#70699=ORIENTED_EDGE('',*,*,#47446,.F.);
#70700=ORIENTED_EDGE('',*,*,#47454,.F.);
#70701=ORIENTED_EDGE('',*,*,#47464,.F.);
#70702=ORIENTED_EDGE('',*,*,#47461,.F.);
#70703=ORIENTED_EDGE('',*,*,#47458,.F.);
#70704=ORIENTED_EDGE('',*,*,#47466,.F.);
#70705=ORIENTED_EDGE('',*,*,#47476,.F.);
#70706=ORIENTED_EDGE('',*,*,#47473,.F.);
#70707=ORIENTED_EDGE('',*,*,#47470,.F.);
#70708=ORIENTED_EDGE('',*,*,#47478,.F.);
#70709=ORIENTED_EDGE('',*,*,#47488,.F.);
#70710=ORIENTED_EDGE('',*,*,#47485,.F.);
#70711=ORIENTED_EDGE('',*,*,#47482,.F.);
#70712=ORIENTED_EDGE('',*,*,#47490,.F.);
#70713=ORIENTED_EDGE('',*,*,#47500,.F.);
#70714=ORIENTED_EDGE('',*,*,#47497,.F.);
#70715=ORIENTED_EDGE('',*,*,#47494,.F.);
#70716=ORIENTED_EDGE('',*,*,#47502,.F.);
#70717=ORIENTED_EDGE('',*,*,#47512,.F.);
#70718=ORIENTED_EDGE('',*,*,#47509,.F.);
#70719=ORIENTED_EDGE('',*,*,#47506,.F.);
#70720=ORIENTED_EDGE('',*,*,#47514,.F.);
#70721=ORIENTED_EDGE('',*,*,#47524,.F.);
#70722=ORIENTED_EDGE('',*,*,#47521,.F.);
#70723=ORIENTED_EDGE('',*,*,#47518,.F.);
#70724=ORIENTED_EDGE('',*,*,#47526,.F.);
#70725=ORIENTED_EDGE('',*,*,#47536,.F.);
#70726=ORIENTED_EDGE('',*,*,#47533,.F.);
#70727=ORIENTED_EDGE('',*,*,#47530,.F.);
#70728=ORIENTED_EDGE('',*,*,#47538,.F.);
#70729=ORIENTED_EDGE('',*,*,#47548,.F.);
#70730=ORIENTED_EDGE('',*,*,#47545,.F.);
#70731=ORIENTED_EDGE('',*,*,#47542,.F.);
#70732=ORIENTED_EDGE('',*,*,#47550,.F.);
#70733=ORIENTED_EDGE('',*,*,#47560,.F.);
#70734=ORIENTED_EDGE('',*,*,#47557,.F.);
#70735=ORIENTED_EDGE('',*,*,#47554,.F.);
#70736=ORIENTED_EDGE('',*,*,#47562,.F.);
#70737=ORIENTED_EDGE('',*,*,#47572,.F.);
#70738=ORIENTED_EDGE('',*,*,#47569,.F.);
#70739=ORIENTED_EDGE('',*,*,#47566,.F.);
#70740=ORIENTED_EDGE('',*,*,#47574,.F.);
#70741=ORIENTED_EDGE('',*,*,#47584,.F.);
#70742=ORIENTED_EDGE('',*,*,#47581,.F.);
#70743=ORIENTED_EDGE('',*,*,#47578,.F.);
#70744=ORIENTED_EDGE('',*,*,#47586,.F.);
#70745=ORIENTED_EDGE('',*,*,#47596,.F.);
#70746=ORIENTED_EDGE('',*,*,#47593,.F.);
#70747=ORIENTED_EDGE('',*,*,#47590,.F.);
#70748=ORIENTED_EDGE('',*,*,#47598,.F.);
#70749=ORIENTED_EDGE('',*,*,#47608,.F.);
#70750=ORIENTED_EDGE('',*,*,#47605,.F.);
#70751=ORIENTED_EDGE('',*,*,#47602,.F.);
#70752=ORIENTED_EDGE('',*,*,#47610,.F.);
#70753=ORIENTED_EDGE('',*,*,#47620,.F.);
#70754=ORIENTED_EDGE('',*,*,#47617,.F.);
#70755=ORIENTED_EDGE('',*,*,#47614,.F.);
#70756=ORIENTED_EDGE('',*,*,#47622,.F.);
#70757=ORIENTED_EDGE('',*,*,#47632,.F.);
#70758=ORIENTED_EDGE('',*,*,#47629,.F.);
#70759=ORIENTED_EDGE('',*,*,#47626,.F.);
#70760=ORIENTED_EDGE('',*,*,#47634,.F.);
#70761=ORIENTED_EDGE('',*,*,#47644,.F.);
#70762=ORIENTED_EDGE('',*,*,#47641,.F.);
#70763=ORIENTED_EDGE('',*,*,#47638,.F.);
#70764=ORIENTED_EDGE('',*,*,#47646,.F.);
#70765=ORIENTED_EDGE('',*,*,#47656,.F.);
#70766=ORIENTED_EDGE('',*,*,#47653,.F.);
#70767=ORIENTED_EDGE('',*,*,#47650,.F.);
#70768=ORIENTED_EDGE('',*,*,#47658,.F.);
#70769=ORIENTED_EDGE('',*,*,#47668,.F.);
#70770=ORIENTED_EDGE('',*,*,#47665,.F.);
#70771=ORIENTED_EDGE('',*,*,#47662,.F.);
#70772=ORIENTED_EDGE('',*,*,#47670,.F.);
#70773=ORIENTED_EDGE('',*,*,#47680,.F.);
#70774=ORIENTED_EDGE('',*,*,#47677,.F.);
#70775=ORIENTED_EDGE('',*,*,#47674,.F.);
#70776=ORIENTED_EDGE('',*,*,#47682,.F.);
#70777=ORIENTED_EDGE('',*,*,#47692,.F.);
#70778=ORIENTED_EDGE('',*,*,#47689,.F.);
#70779=ORIENTED_EDGE('',*,*,#47686,.F.);
#70780=ORIENTED_EDGE('',*,*,#47694,.F.);
#70781=ORIENTED_EDGE('',*,*,#47704,.F.);
#70782=ORIENTED_EDGE('',*,*,#47701,.F.);
#70783=ORIENTED_EDGE('',*,*,#47698,.F.);
#70784=ORIENTED_EDGE('',*,*,#47706,.F.);
#70785=ORIENTED_EDGE('',*,*,#47716,.F.);
#70786=ORIENTED_EDGE('',*,*,#47713,.F.);
#70787=ORIENTED_EDGE('',*,*,#47710,.F.);
#70788=ORIENTED_EDGE('',*,*,#47718,.F.);
#70789=ORIENTED_EDGE('',*,*,#47728,.F.);
#70790=ORIENTED_EDGE('',*,*,#47725,.F.);
#70791=ORIENTED_EDGE('',*,*,#47722,.F.);
#70792=ORIENTED_EDGE('',*,*,#47730,.F.);
#70793=ORIENTED_EDGE('',*,*,#47740,.F.);
#70794=ORIENTED_EDGE('',*,*,#47737,.F.);
#70795=ORIENTED_EDGE('',*,*,#47734,.F.);
#70796=ORIENTED_EDGE('',*,*,#47742,.F.);
#70797=ORIENTED_EDGE('',*,*,#47752,.F.);
#70798=ORIENTED_EDGE('',*,*,#47749,.F.);
#70799=ORIENTED_EDGE('',*,*,#47746,.F.);
#70800=ORIENTED_EDGE('',*,*,#47754,.F.);
#70801=ORIENTED_EDGE('',*,*,#47764,.F.);
#70802=ORIENTED_EDGE('',*,*,#47761,.F.);
#70803=ORIENTED_EDGE('',*,*,#47758,.F.);
#70804=ORIENTED_EDGE('',*,*,#47766,.F.);
#70805=ORIENTED_EDGE('',*,*,#47776,.F.);
#70806=ORIENTED_EDGE('',*,*,#47773,.F.);
#70807=ORIENTED_EDGE('',*,*,#47770,.F.);
#70808=ORIENTED_EDGE('',*,*,#47778,.F.);
#70809=ORIENTED_EDGE('',*,*,#47788,.F.);
#70810=ORIENTED_EDGE('',*,*,#47785,.F.);
#70811=ORIENTED_EDGE('',*,*,#47782,.F.);
#70812=ORIENTED_EDGE('',*,*,#47790,.F.);
#70813=ORIENTED_EDGE('',*,*,#47800,.F.);
#70814=ORIENTED_EDGE('',*,*,#47797,.F.);
#70815=ORIENTED_EDGE('',*,*,#47794,.F.);
#70816=ORIENTED_EDGE('',*,*,#47802,.F.);
#70817=ORIENTED_EDGE('',*,*,#47812,.F.);
#70818=ORIENTED_EDGE('',*,*,#47809,.F.);
#70819=ORIENTED_EDGE('',*,*,#47806,.F.);
#70820=ORIENTED_EDGE('',*,*,#47814,.F.);
#70821=ORIENTED_EDGE('',*,*,#47824,.F.);
#70822=ORIENTED_EDGE('',*,*,#47821,.F.);
#70823=ORIENTED_EDGE('',*,*,#47818,.F.);
#70824=ORIENTED_EDGE('',*,*,#47826,.F.);
#70825=ORIENTED_EDGE('',*,*,#47836,.F.);
#70826=ORIENTED_EDGE('',*,*,#47833,.F.);
#70827=ORIENTED_EDGE('',*,*,#47830,.F.);
#70828=ORIENTED_EDGE('',*,*,#47838,.F.);
#70829=ORIENTED_EDGE('',*,*,#47848,.F.);
#70830=ORIENTED_EDGE('',*,*,#47845,.F.);
#70831=ORIENTED_EDGE('',*,*,#47842,.F.);
#70832=ORIENTED_EDGE('',*,*,#47850,.F.);
#70833=ORIENTED_EDGE('',*,*,#47860,.F.);
#70834=ORIENTED_EDGE('',*,*,#47857,.F.);
#70835=ORIENTED_EDGE('',*,*,#47854,.F.);
#70836=ORIENTED_EDGE('',*,*,#47862,.F.);
#70837=ORIENTED_EDGE('',*,*,#47872,.F.);
#70838=ORIENTED_EDGE('',*,*,#47869,.F.);
#70839=ORIENTED_EDGE('',*,*,#47866,.F.);
#70840=ORIENTED_EDGE('',*,*,#47874,.F.);
#70841=ORIENTED_EDGE('',*,*,#47884,.F.);
#70842=ORIENTED_EDGE('',*,*,#47881,.F.);
#70843=ORIENTED_EDGE('',*,*,#47878,.F.);
#70844=ORIENTED_EDGE('',*,*,#47886,.F.);
#70845=ORIENTED_EDGE('',*,*,#47896,.F.);
#70846=ORIENTED_EDGE('',*,*,#47893,.F.);
#70847=ORIENTED_EDGE('',*,*,#47890,.F.);
#70848=ORIENTED_EDGE('',*,*,#47898,.F.);
#70849=ORIENTED_EDGE('',*,*,#47908,.F.);
#70850=ORIENTED_EDGE('',*,*,#47905,.F.);
#70851=ORIENTED_EDGE('',*,*,#47902,.F.);
#70852=ORIENTED_EDGE('',*,*,#47910,.F.);
#70853=ORIENTED_EDGE('',*,*,#47920,.F.);
#70854=ORIENTED_EDGE('',*,*,#47917,.F.);
#70855=ORIENTED_EDGE('',*,*,#47914,.F.);
#70856=ORIENTED_EDGE('',*,*,#47922,.F.);
#70857=ORIENTED_EDGE('',*,*,#47932,.F.);
#70858=ORIENTED_EDGE('',*,*,#47929,.F.);
#70859=ORIENTED_EDGE('',*,*,#47926,.F.);
#70860=ORIENTED_EDGE('',*,*,#47934,.F.);
#70861=ORIENTED_EDGE('',*,*,#47944,.F.);
#70862=ORIENTED_EDGE('',*,*,#47941,.F.);
#70863=ORIENTED_EDGE('',*,*,#47938,.F.);
#70864=ORIENTED_EDGE('',*,*,#47946,.F.);
#70865=ORIENTED_EDGE('',*,*,#47956,.F.);
#70866=ORIENTED_EDGE('',*,*,#47953,.F.);
#70867=ORIENTED_EDGE('',*,*,#47950,.F.);
#70868=ORIENTED_EDGE('',*,*,#47958,.F.);
#70869=ORIENTED_EDGE('',*,*,#47968,.F.);
#70870=ORIENTED_EDGE('',*,*,#47965,.F.);
#70871=ORIENTED_EDGE('',*,*,#47962,.F.);
#70872=ORIENTED_EDGE('',*,*,#47970,.F.);
#70873=ORIENTED_EDGE('',*,*,#47980,.F.);
#70874=ORIENTED_EDGE('',*,*,#47977,.F.);
#70875=ORIENTED_EDGE('',*,*,#47974,.F.);
#70876=ORIENTED_EDGE('',*,*,#47982,.F.);
#70877=ORIENTED_EDGE('',*,*,#47992,.F.);
#70878=ORIENTED_EDGE('',*,*,#47989,.F.);
#70879=ORIENTED_EDGE('',*,*,#47986,.F.);
#70880=ORIENTED_EDGE('',*,*,#47994,.F.);
#70881=ORIENTED_EDGE('',*,*,#48004,.F.);
#70882=ORIENTED_EDGE('',*,*,#48001,.F.);
#70883=ORIENTED_EDGE('',*,*,#47998,.F.);
#70884=ORIENTED_EDGE('',*,*,#48006,.F.);
#70885=ORIENTED_EDGE('',*,*,#48016,.F.);
#70886=ORIENTED_EDGE('',*,*,#48013,.F.);
#70887=ORIENTED_EDGE('',*,*,#48010,.F.);
#70888=ORIENTED_EDGE('',*,*,#48018,.F.);
#70889=ORIENTED_EDGE('',*,*,#48028,.F.);
#70890=ORIENTED_EDGE('',*,*,#48025,.F.);
#70891=ORIENTED_EDGE('',*,*,#48022,.F.);
#70892=ORIENTED_EDGE('',*,*,#48030,.F.);
#70893=ORIENTED_EDGE('',*,*,#48040,.F.);
#70894=ORIENTED_EDGE('',*,*,#48037,.F.);
#70895=ORIENTED_EDGE('',*,*,#48034,.F.);
#70896=ORIENTED_EDGE('',*,*,#48042,.F.);
#70897=ORIENTED_EDGE('',*,*,#48052,.F.);
#70898=ORIENTED_EDGE('',*,*,#48049,.F.);
#70899=ORIENTED_EDGE('',*,*,#48046,.F.);
#70900=ORIENTED_EDGE('',*,*,#48054,.F.);
#70901=ORIENTED_EDGE('',*,*,#48064,.F.);
#70902=ORIENTED_EDGE('',*,*,#48061,.F.);
#70903=ORIENTED_EDGE('',*,*,#48058,.F.);
#70904=ORIENTED_EDGE('',*,*,#48066,.F.);
#70905=ORIENTED_EDGE('',*,*,#48076,.F.);
#70906=ORIENTED_EDGE('',*,*,#48073,.F.);
#70907=ORIENTED_EDGE('',*,*,#48070,.F.);
#70908=ORIENTED_EDGE('',*,*,#48078,.F.);
#70909=ORIENTED_EDGE('',*,*,#48088,.F.);
#70910=ORIENTED_EDGE('',*,*,#48085,.F.);
#70911=ORIENTED_EDGE('',*,*,#48082,.F.);
#70912=ORIENTED_EDGE('',*,*,#48090,.F.);
#70913=ORIENTED_EDGE('',*,*,#48100,.F.);
#70914=ORIENTED_EDGE('',*,*,#48097,.F.);
#70915=ORIENTED_EDGE('',*,*,#48094,.F.);
#70916=ORIENTED_EDGE('',*,*,#48102,.F.);
#70917=ORIENTED_EDGE('',*,*,#48112,.F.);
#70918=ORIENTED_EDGE('',*,*,#48109,.F.);
#70919=ORIENTED_EDGE('',*,*,#48106,.F.);
#70920=ORIENTED_EDGE('',*,*,#48114,.F.);
#70921=ORIENTED_EDGE('',*,*,#48124,.F.);
#70922=ORIENTED_EDGE('',*,*,#48121,.F.);
#70923=ORIENTED_EDGE('',*,*,#48118,.F.);
#70924=ORIENTED_EDGE('',*,*,#48126,.F.);
#70925=ORIENTED_EDGE('',*,*,#48136,.F.);
#70926=ORIENTED_EDGE('',*,*,#48133,.F.);
#70927=ORIENTED_EDGE('',*,*,#48130,.F.);
#70928=ORIENTED_EDGE('',*,*,#48138,.F.);
#70929=ORIENTED_EDGE('',*,*,#48148,.F.);
#70930=ORIENTED_EDGE('',*,*,#48145,.F.);
#70931=ORIENTED_EDGE('',*,*,#48142,.F.);
#70932=ORIENTED_EDGE('',*,*,#48150,.F.);
#70933=ORIENTED_EDGE('',*,*,#48160,.F.);
#70934=ORIENTED_EDGE('',*,*,#48157,.F.);
#70935=ORIENTED_EDGE('',*,*,#48154,.F.);
#70936=ORIENTED_EDGE('',*,*,#48162,.F.);
#70937=ORIENTED_EDGE('',*,*,#48172,.F.);
#70938=ORIENTED_EDGE('',*,*,#48169,.F.);
#70939=ORIENTED_EDGE('',*,*,#48166,.F.);
#70940=ORIENTED_EDGE('',*,*,#48174,.F.);
#70941=ORIENTED_EDGE('',*,*,#48184,.F.);
#70942=ORIENTED_EDGE('',*,*,#48181,.F.);
#70943=ORIENTED_EDGE('',*,*,#48178,.F.);
#70944=ORIENTED_EDGE('',*,*,#48186,.F.);
#70945=ORIENTED_EDGE('',*,*,#48196,.F.);
#70946=ORIENTED_EDGE('',*,*,#48193,.F.);
#70947=ORIENTED_EDGE('',*,*,#48190,.F.);
#70948=ORIENTED_EDGE('',*,*,#48198,.F.);
#70949=ORIENTED_EDGE('',*,*,#48208,.F.);
#70950=ORIENTED_EDGE('',*,*,#48205,.F.);
#70951=ORIENTED_EDGE('',*,*,#48202,.F.);
#70952=ORIENTED_EDGE('',*,*,#48210,.F.);
#70953=ORIENTED_EDGE('',*,*,#48220,.F.);
#70954=ORIENTED_EDGE('',*,*,#48217,.F.);
#70955=ORIENTED_EDGE('',*,*,#48214,.F.);
#70956=ORIENTED_EDGE('',*,*,#48222,.F.);
#70957=ORIENTED_EDGE('',*,*,#48232,.F.);
#70958=ORIENTED_EDGE('',*,*,#48229,.F.);
#70959=ORIENTED_EDGE('',*,*,#48226,.F.);
#70960=ORIENTED_EDGE('',*,*,#48234,.F.);
#70961=ORIENTED_EDGE('',*,*,#48244,.F.);
#70962=ORIENTED_EDGE('',*,*,#48241,.F.);
#70963=ORIENTED_EDGE('',*,*,#48238,.F.);
#70964=ORIENTED_EDGE('',*,*,#48246,.F.);
#70965=ORIENTED_EDGE('',*,*,#48256,.F.);
#70966=ORIENTED_EDGE('',*,*,#48253,.F.);
#70967=ORIENTED_EDGE('',*,*,#48250,.F.);
#70968=ORIENTED_EDGE('',*,*,#48258,.F.);
#70969=ORIENTED_EDGE('',*,*,#48268,.F.);
#70970=ORIENTED_EDGE('',*,*,#48265,.F.);
#70971=ORIENTED_EDGE('',*,*,#48262,.F.);
#70972=ORIENTED_EDGE('',*,*,#48270,.F.);
#70973=ORIENTED_EDGE('',*,*,#48280,.F.);
#70974=ORIENTED_EDGE('',*,*,#48277,.F.);
#70975=ORIENTED_EDGE('',*,*,#48274,.F.);
#70976=ORIENTED_EDGE('',*,*,#48282,.F.);
#70977=ORIENTED_EDGE('',*,*,#48292,.F.);
#70978=ORIENTED_EDGE('',*,*,#48289,.F.);
#70979=ORIENTED_EDGE('',*,*,#48286,.F.);
#70980=ORIENTED_EDGE('',*,*,#48294,.F.);
#70981=ORIENTED_EDGE('',*,*,#48304,.F.);
#70982=ORIENTED_EDGE('',*,*,#48301,.F.);
#70983=ORIENTED_EDGE('',*,*,#48298,.F.);
#70984=ORIENTED_EDGE('',*,*,#48306,.F.);
#70985=ORIENTED_EDGE('',*,*,#48316,.F.);
#70986=ORIENTED_EDGE('',*,*,#48313,.F.);
#70987=ORIENTED_EDGE('',*,*,#48310,.F.);
#70988=ORIENTED_EDGE('',*,*,#48318,.F.);
#70989=ORIENTED_EDGE('',*,*,#48328,.F.);
#70990=ORIENTED_EDGE('',*,*,#48325,.F.);
#70991=ORIENTED_EDGE('',*,*,#48322,.F.);
#70992=ORIENTED_EDGE('',*,*,#48330,.F.);
#70993=ORIENTED_EDGE('',*,*,#48340,.F.);
#70994=ORIENTED_EDGE('',*,*,#48337,.F.);
#70995=ORIENTED_EDGE('',*,*,#48334,.F.);
#70996=ORIENTED_EDGE('',*,*,#48342,.F.);
#70997=ORIENTED_EDGE('',*,*,#48352,.F.);
#70998=ORIENTED_EDGE('',*,*,#48349,.F.);
#70999=ORIENTED_EDGE('',*,*,#48346,.F.);
#71000=ORIENTED_EDGE('',*,*,#48354,.F.);
#71001=ORIENTED_EDGE('',*,*,#48364,.F.);
#71002=ORIENTED_EDGE('',*,*,#48361,.F.);
#71003=ORIENTED_EDGE('',*,*,#48358,.F.);
#71004=ORIENTED_EDGE('',*,*,#48366,.F.);
#71005=ORIENTED_EDGE('',*,*,#48376,.F.);
#71006=ORIENTED_EDGE('',*,*,#48373,.F.);
#71007=ORIENTED_EDGE('',*,*,#48370,.F.);
#71008=ORIENTED_EDGE('',*,*,#48378,.F.);
#71009=ORIENTED_EDGE('',*,*,#48388,.F.);
#71010=ORIENTED_EDGE('',*,*,#48385,.F.);
#71011=ORIENTED_EDGE('',*,*,#48382,.F.);
#71012=ORIENTED_EDGE('',*,*,#48390,.F.);
#71013=ORIENTED_EDGE('',*,*,#48400,.F.);
#71014=ORIENTED_EDGE('',*,*,#48397,.F.);
#71015=ORIENTED_EDGE('',*,*,#48394,.F.);
#71016=ORIENTED_EDGE('',*,*,#48402,.F.);
#71017=ORIENTED_EDGE('',*,*,#48412,.F.);
#71018=ORIENTED_EDGE('',*,*,#48409,.F.);
#71019=ORIENTED_EDGE('',*,*,#48406,.F.);
#71020=ORIENTED_EDGE('',*,*,#48414,.F.);
#71021=ORIENTED_EDGE('',*,*,#48424,.F.);
#71022=ORIENTED_EDGE('',*,*,#48421,.F.);
#71023=ORIENTED_EDGE('',*,*,#48418,.F.);
#71024=ORIENTED_EDGE('',*,*,#48426,.F.);
#71025=ORIENTED_EDGE('',*,*,#48436,.F.);
#71026=ORIENTED_EDGE('',*,*,#48433,.F.);
#71027=ORIENTED_EDGE('',*,*,#48430,.F.);
#71028=ORIENTED_EDGE('',*,*,#48438,.F.);
#71029=ORIENTED_EDGE('',*,*,#48448,.F.);
#71030=ORIENTED_EDGE('',*,*,#48445,.F.);
#71031=ORIENTED_EDGE('',*,*,#48442,.F.);
#71032=ORIENTED_EDGE('',*,*,#48450,.F.);
#71033=ORIENTED_EDGE('',*,*,#48460,.F.);
#71034=ORIENTED_EDGE('',*,*,#48457,.F.);
#71035=ORIENTED_EDGE('',*,*,#48454,.F.);
#71036=ORIENTED_EDGE('',*,*,#48462,.F.);
#71037=ORIENTED_EDGE('',*,*,#48472,.F.);
#71038=ORIENTED_EDGE('',*,*,#48469,.F.);
#71039=ORIENTED_EDGE('',*,*,#48466,.F.);
#71040=ORIENTED_EDGE('',*,*,#48474,.F.);
#71041=ORIENTED_EDGE('',*,*,#48484,.F.);
#71042=ORIENTED_EDGE('',*,*,#48481,.F.);
#71043=ORIENTED_EDGE('',*,*,#48478,.F.);
#71044=ORIENTED_EDGE('',*,*,#48486,.F.);
#71045=ORIENTED_EDGE('',*,*,#48496,.F.);
#71046=ORIENTED_EDGE('',*,*,#48493,.F.);
#71047=ORIENTED_EDGE('',*,*,#48490,.F.);
#71048=ORIENTED_EDGE('',*,*,#48498,.F.);
#71049=ORIENTED_EDGE('',*,*,#48508,.F.);
#71050=ORIENTED_EDGE('',*,*,#48505,.F.);
#71051=ORIENTED_EDGE('',*,*,#48502,.F.);
#71052=ORIENTED_EDGE('',*,*,#48510,.F.);
#71053=ORIENTED_EDGE('',*,*,#48520,.F.);
#71054=ORIENTED_EDGE('',*,*,#48517,.F.);
#71055=ORIENTED_EDGE('',*,*,#48514,.F.);
#71056=ORIENTED_EDGE('',*,*,#48522,.F.);
#71057=ORIENTED_EDGE('',*,*,#48532,.F.);
#71058=ORIENTED_EDGE('',*,*,#48529,.F.);
#71059=ORIENTED_EDGE('',*,*,#48526,.F.);
#71060=ORIENTED_EDGE('',*,*,#48534,.F.);
#71061=ORIENTED_EDGE('',*,*,#48544,.F.);
#71062=ORIENTED_EDGE('',*,*,#48541,.F.);
#71063=ORIENTED_EDGE('',*,*,#48538,.F.);
#71064=ORIENTED_EDGE('',*,*,#48546,.F.);
#71065=ORIENTED_EDGE('',*,*,#48556,.F.);
#71066=ORIENTED_EDGE('',*,*,#48553,.F.);
#71067=ORIENTED_EDGE('',*,*,#48550,.F.);
#71068=ORIENTED_EDGE('',*,*,#48558,.F.);
#71069=ORIENTED_EDGE('',*,*,#48568,.F.);
#71070=ORIENTED_EDGE('',*,*,#48565,.F.);
#71071=ORIENTED_EDGE('',*,*,#48562,.F.);
#71072=ORIENTED_EDGE('',*,*,#48570,.F.);
#71073=ORIENTED_EDGE('',*,*,#48580,.F.);
#71074=ORIENTED_EDGE('',*,*,#48577,.F.);
#71075=ORIENTED_EDGE('',*,*,#48574,.F.);
#71076=ORIENTED_EDGE('',*,*,#48582,.F.);
#71077=ORIENTED_EDGE('',*,*,#48592,.F.);
#71078=ORIENTED_EDGE('',*,*,#48589,.F.);
#71079=ORIENTED_EDGE('',*,*,#48586,.F.);
#71080=ORIENTED_EDGE('',*,*,#48594,.F.);
#71081=ORIENTED_EDGE('',*,*,#48604,.F.);
#71082=ORIENTED_EDGE('',*,*,#48601,.F.);
#71083=ORIENTED_EDGE('',*,*,#48598,.F.);
#71084=ORIENTED_EDGE('',*,*,#48606,.F.);
#71085=ORIENTED_EDGE('',*,*,#48616,.F.);
#71086=ORIENTED_EDGE('',*,*,#48613,.F.);
#71087=ORIENTED_EDGE('',*,*,#48610,.F.);
#71088=ORIENTED_EDGE('',*,*,#48618,.F.);
#71089=ORIENTED_EDGE('',*,*,#48628,.F.);
#71090=ORIENTED_EDGE('',*,*,#48625,.F.);
#71091=ORIENTED_EDGE('',*,*,#48622,.F.);
#71092=ORIENTED_EDGE('',*,*,#48630,.F.);
#71093=ORIENTED_EDGE('',*,*,#48640,.F.);
#71094=ORIENTED_EDGE('',*,*,#48637,.F.);
#71095=ORIENTED_EDGE('',*,*,#48634,.F.);
#71096=ORIENTED_EDGE('',*,*,#48642,.F.);
#71097=ORIENTED_EDGE('',*,*,#48652,.F.);
#71098=ORIENTED_EDGE('',*,*,#48649,.F.);
#71099=ORIENTED_EDGE('',*,*,#48646,.F.);
#71100=ORIENTED_EDGE('',*,*,#48654,.F.);
#71101=ORIENTED_EDGE('',*,*,#48664,.F.);
#71102=ORIENTED_EDGE('',*,*,#48661,.F.);
#71103=ORIENTED_EDGE('',*,*,#48658,.F.);
#71104=ORIENTED_EDGE('',*,*,#48666,.F.);
#71105=ORIENTED_EDGE('',*,*,#48676,.F.);
#71106=ORIENTED_EDGE('',*,*,#48673,.F.);
#71107=ORIENTED_EDGE('',*,*,#48670,.F.);
#71108=ORIENTED_EDGE('',*,*,#48678,.F.);
#71109=ORIENTED_EDGE('',*,*,#48688,.F.);
#71110=ORIENTED_EDGE('',*,*,#48685,.F.);
#71111=ORIENTED_EDGE('',*,*,#48682,.F.);
#71112=ORIENTED_EDGE('',*,*,#48690,.F.);
#71113=ORIENTED_EDGE('',*,*,#48700,.F.);
#71114=ORIENTED_EDGE('',*,*,#48697,.F.);
#71115=ORIENTED_EDGE('',*,*,#48694,.F.);
#71116=ORIENTED_EDGE('',*,*,#48702,.F.);
#71117=ORIENTED_EDGE('',*,*,#48712,.F.);
#71118=ORIENTED_EDGE('',*,*,#48709,.F.);
#71119=ORIENTED_EDGE('',*,*,#48706,.F.);
#71120=ORIENTED_EDGE('',*,*,#48714,.F.);
#71121=ORIENTED_EDGE('',*,*,#48724,.F.);
#71122=ORIENTED_EDGE('',*,*,#48721,.F.);
#71123=ORIENTED_EDGE('',*,*,#48718,.F.);
#71124=ORIENTED_EDGE('',*,*,#48726,.F.);
#71125=ORIENTED_EDGE('',*,*,#48736,.F.);
#71126=ORIENTED_EDGE('',*,*,#48733,.F.);
#71127=ORIENTED_EDGE('',*,*,#48730,.F.);
#71128=ORIENTED_EDGE('',*,*,#48738,.F.);
#71129=ORIENTED_EDGE('',*,*,#48748,.F.);
#71130=ORIENTED_EDGE('',*,*,#48745,.F.);
#71131=ORIENTED_EDGE('',*,*,#48742,.F.);
#71132=ORIENTED_EDGE('',*,*,#48750,.F.);
#71133=ORIENTED_EDGE('',*,*,#48760,.F.);
#71134=ORIENTED_EDGE('',*,*,#48757,.F.);
#71135=ORIENTED_EDGE('',*,*,#48754,.F.);
#71136=ORIENTED_EDGE('',*,*,#48762,.F.);
#71137=ORIENTED_EDGE('',*,*,#48772,.F.);
#71138=ORIENTED_EDGE('',*,*,#48769,.F.);
#71139=ORIENTED_EDGE('',*,*,#48766,.F.);
#71140=ORIENTED_EDGE('',*,*,#48774,.F.);
#71141=ORIENTED_EDGE('',*,*,#48784,.F.);
#71142=ORIENTED_EDGE('',*,*,#48781,.F.);
#71143=ORIENTED_EDGE('',*,*,#48778,.F.);
#71144=ORIENTED_EDGE('',*,*,#48786,.F.);
#71145=ORIENTED_EDGE('',*,*,#48796,.F.);
#71146=ORIENTED_EDGE('',*,*,#48793,.F.);
#71147=ORIENTED_EDGE('',*,*,#48790,.F.);
#71148=ORIENTED_EDGE('',*,*,#48798,.F.);
#71149=ORIENTED_EDGE('',*,*,#48808,.F.);
#71150=ORIENTED_EDGE('',*,*,#48805,.F.);
#71151=ORIENTED_EDGE('',*,*,#48802,.F.);
#71152=ORIENTED_EDGE('',*,*,#48810,.F.);
#71153=ORIENTED_EDGE('',*,*,#48820,.F.);
#71154=ORIENTED_EDGE('',*,*,#48817,.F.);
#71155=ORIENTED_EDGE('',*,*,#48814,.F.);
#71156=ORIENTED_EDGE('',*,*,#48822,.F.);
#71157=ORIENTED_EDGE('',*,*,#48832,.F.);
#71158=ORIENTED_EDGE('',*,*,#48829,.F.);
#71159=ORIENTED_EDGE('',*,*,#48826,.F.);
#71160=ORIENTED_EDGE('',*,*,#48834,.F.);
#71161=ORIENTED_EDGE('',*,*,#48844,.F.);
#71162=ORIENTED_EDGE('',*,*,#48841,.F.);
#71163=ORIENTED_EDGE('',*,*,#48838,.F.);
#71164=ORIENTED_EDGE('',*,*,#48846,.F.);
#71165=ORIENTED_EDGE('',*,*,#48856,.F.);
#71166=ORIENTED_EDGE('',*,*,#48853,.F.);
#71167=ORIENTED_EDGE('',*,*,#48850,.F.);
#71168=ORIENTED_EDGE('',*,*,#48858,.F.);
#71169=ORIENTED_EDGE('',*,*,#48868,.F.);
#71170=ORIENTED_EDGE('',*,*,#48865,.F.);
#71171=ORIENTED_EDGE('',*,*,#48862,.F.);
#71172=ORIENTED_EDGE('',*,*,#48870,.F.);
#71173=ORIENTED_EDGE('',*,*,#48880,.F.);
#71174=ORIENTED_EDGE('',*,*,#48877,.F.);
#71175=ORIENTED_EDGE('',*,*,#48874,.F.);
#71176=ORIENTED_EDGE('',*,*,#48882,.F.);
#71177=ORIENTED_EDGE('',*,*,#48892,.F.);
#71178=ORIENTED_EDGE('',*,*,#48889,.F.);
#71179=ORIENTED_EDGE('',*,*,#48886,.F.);
#71180=ORIENTED_EDGE('',*,*,#48894,.F.);
#71181=ORIENTED_EDGE('',*,*,#48904,.F.);
#71182=ORIENTED_EDGE('',*,*,#48901,.F.);
#71183=ORIENTED_EDGE('',*,*,#48898,.F.);
#71184=ORIENTED_EDGE('',*,*,#48906,.F.);
#71185=ORIENTED_EDGE('',*,*,#48916,.F.);
#71186=ORIENTED_EDGE('',*,*,#48913,.F.);
#71187=ORIENTED_EDGE('',*,*,#48910,.F.);
#71188=ORIENTED_EDGE('',*,*,#48918,.F.);
#71189=ORIENTED_EDGE('',*,*,#48928,.F.);
#71190=ORIENTED_EDGE('',*,*,#48925,.F.);
#71191=ORIENTED_EDGE('',*,*,#48922,.F.);
#71192=ORIENTED_EDGE('',*,*,#48930,.F.);
#71193=ORIENTED_EDGE('',*,*,#48940,.F.);
#71194=ORIENTED_EDGE('',*,*,#48937,.F.);
#71195=ORIENTED_EDGE('',*,*,#48934,.F.);
#71196=ORIENTED_EDGE('',*,*,#48942,.F.);
#71197=ORIENTED_EDGE('',*,*,#48952,.F.);
#71198=ORIENTED_EDGE('',*,*,#48949,.F.);
#71199=ORIENTED_EDGE('',*,*,#48946,.F.);
#71200=ORIENTED_EDGE('',*,*,#48954,.F.);
#71201=ORIENTED_EDGE('',*,*,#48964,.F.);
#71202=ORIENTED_EDGE('',*,*,#48961,.F.);
#71203=ORIENTED_EDGE('',*,*,#48958,.F.);
#71204=ORIENTED_EDGE('',*,*,#48966,.F.);
#71205=ORIENTED_EDGE('',*,*,#48976,.F.);
#71206=ORIENTED_EDGE('',*,*,#48973,.F.);
#71207=ORIENTED_EDGE('',*,*,#48970,.F.);
#71208=ORIENTED_EDGE('',*,*,#48978,.F.);
#71209=ORIENTED_EDGE('',*,*,#48988,.F.);
#71210=ORIENTED_EDGE('',*,*,#48985,.F.);
#71211=ORIENTED_EDGE('',*,*,#48982,.F.);
#71212=ORIENTED_EDGE('',*,*,#48990,.F.);
#71213=ORIENTED_EDGE('',*,*,#49000,.F.);
#71214=ORIENTED_EDGE('',*,*,#48997,.F.);
#71215=ORIENTED_EDGE('',*,*,#48994,.F.);
#71216=ORIENTED_EDGE('',*,*,#49002,.F.);
#71217=ORIENTED_EDGE('',*,*,#49012,.F.);
#71218=ORIENTED_EDGE('',*,*,#49009,.F.);
#71219=ORIENTED_EDGE('',*,*,#49006,.F.);
#71220=ORIENTED_EDGE('',*,*,#49014,.F.);
#71221=ORIENTED_EDGE('',*,*,#49024,.F.);
#71222=ORIENTED_EDGE('',*,*,#49021,.F.);
#71223=ORIENTED_EDGE('',*,*,#49018,.F.);
#71224=ORIENTED_EDGE('',*,*,#49026,.F.);
#71225=ORIENTED_EDGE('',*,*,#49036,.F.);
#71226=ORIENTED_EDGE('',*,*,#49033,.F.);
#71227=ORIENTED_EDGE('',*,*,#49030,.F.);
#71228=ORIENTED_EDGE('',*,*,#49038,.F.);
#71229=ORIENTED_EDGE('',*,*,#49048,.F.);
#71230=ORIENTED_EDGE('',*,*,#49045,.F.);
#71231=ORIENTED_EDGE('',*,*,#49042,.F.);
#71232=ORIENTED_EDGE('',*,*,#49050,.F.);
#71233=ORIENTED_EDGE('',*,*,#49060,.F.);
#71234=ORIENTED_EDGE('',*,*,#49057,.F.);
#71235=ORIENTED_EDGE('',*,*,#49054,.F.);
#71236=ORIENTED_EDGE('',*,*,#49062,.F.);
#71237=ORIENTED_EDGE('',*,*,#49072,.F.);
#71238=ORIENTED_EDGE('',*,*,#49069,.F.);
#71239=ORIENTED_EDGE('',*,*,#49066,.F.);
#71240=ORIENTED_EDGE('',*,*,#49074,.F.);
#71241=ORIENTED_EDGE('',*,*,#49084,.F.);
#71242=ORIENTED_EDGE('',*,*,#49081,.F.);
#71243=ORIENTED_EDGE('',*,*,#49078,.F.);
#71244=ORIENTED_EDGE('',*,*,#49086,.F.);
#71245=ORIENTED_EDGE('',*,*,#49096,.F.);
#71246=ORIENTED_EDGE('',*,*,#49093,.F.);
#71247=ORIENTED_EDGE('',*,*,#49090,.F.);
#71248=ORIENTED_EDGE('',*,*,#49098,.F.);
#71249=ORIENTED_EDGE('',*,*,#49108,.F.);
#71250=ORIENTED_EDGE('',*,*,#49105,.F.);
#71251=ORIENTED_EDGE('',*,*,#49102,.F.);
#71252=ORIENTED_EDGE('',*,*,#49110,.F.);
#71253=ORIENTED_EDGE('',*,*,#49120,.F.);
#71254=ORIENTED_EDGE('',*,*,#49117,.F.);
#71255=ORIENTED_EDGE('',*,*,#49114,.F.);
#71256=ORIENTED_EDGE('',*,*,#49122,.F.);
#71257=ORIENTED_EDGE('',*,*,#49132,.F.);
#71258=ORIENTED_EDGE('',*,*,#49129,.F.);
#71259=ORIENTED_EDGE('',*,*,#49126,.F.);
#71260=ORIENTED_EDGE('',*,*,#49134,.F.);
#71261=ORIENTED_EDGE('',*,*,#49144,.F.);
#71262=ORIENTED_EDGE('',*,*,#49141,.F.);
#71263=ORIENTED_EDGE('',*,*,#49138,.F.);
#71264=ORIENTED_EDGE('',*,*,#49146,.F.);
#71265=ORIENTED_EDGE('',*,*,#49156,.F.);
#71266=ORIENTED_EDGE('',*,*,#49153,.F.);
#71267=ORIENTED_EDGE('',*,*,#49150,.F.);
#71268=ORIENTED_EDGE('',*,*,#49158,.F.);
#71269=ORIENTED_EDGE('',*,*,#49168,.F.);
#71270=ORIENTED_EDGE('',*,*,#49165,.F.);
#71271=ORIENTED_EDGE('',*,*,#49162,.F.);
#71272=ORIENTED_EDGE('',*,*,#49170,.F.);
#71273=ORIENTED_EDGE('',*,*,#49180,.F.);
#71274=ORIENTED_EDGE('',*,*,#49177,.F.);
#71275=ORIENTED_EDGE('',*,*,#49174,.F.);
#71276=ORIENTED_EDGE('',*,*,#49182,.F.);
#71277=ORIENTED_EDGE('',*,*,#49192,.F.);
#71278=ORIENTED_EDGE('',*,*,#49189,.F.);
#71279=ORIENTED_EDGE('',*,*,#49186,.F.);
#71280=ORIENTED_EDGE('',*,*,#49194,.F.);
#71281=ORIENTED_EDGE('',*,*,#49204,.F.);
#71282=ORIENTED_EDGE('',*,*,#49201,.F.);
#71283=ORIENTED_EDGE('',*,*,#49198,.F.);
#71284=ORIENTED_EDGE('',*,*,#49206,.F.);
#71285=ORIENTED_EDGE('',*,*,#49216,.F.);
#71286=ORIENTED_EDGE('',*,*,#49213,.F.);
#71287=ORIENTED_EDGE('',*,*,#49210,.F.);
#71288=ORIENTED_EDGE('',*,*,#49218,.F.);
#71289=ORIENTED_EDGE('',*,*,#49228,.F.);
#71290=ORIENTED_EDGE('',*,*,#49225,.F.);
#71291=ORIENTED_EDGE('',*,*,#49222,.F.);
#71292=ORIENTED_EDGE('',*,*,#49230,.F.);
#71293=ORIENTED_EDGE('',*,*,#49240,.F.);
#71294=ORIENTED_EDGE('',*,*,#49237,.F.);
#71295=ORIENTED_EDGE('',*,*,#49234,.F.);
#71296=ORIENTED_EDGE('',*,*,#49242,.F.);
#71297=ORIENTED_EDGE('',*,*,#49252,.F.);
#71298=ORIENTED_EDGE('',*,*,#49249,.F.);
#71299=ORIENTED_EDGE('',*,*,#49246,.F.);
#71300=ORIENTED_EDGE('',*,*,#49254,.F.);
#71301=ORIENTED_EDGE('',*,*,#49264,.F.);
#71302=ORIENTED_EDGE('',*,*,#49261,.F.);
#71303=ORIENTED_EDGE('',*,*,#49258,.F.);
#71304=ORIENTED_EDGE('',*,*,#49266,.F.);
#71305=ORIENTED_EDGE('',*,*,#49276,.F.);
#71306=ORIENTED_EDGE('',*,*,#49273,.F.);
#71307=ORIENTED_EDGE('',*,*,#49270,.F.);
#71308=ORIENTED_EDGE('',*,*,#49278,.F.);
#71309=ORIENTED_EDGE('',*,*,#49288,.F.);
#71310=ORIENTED_EDGE('',*,*,#49285,.F.);
#71311=ORIENTED_EDGE('',*,*,#49282,.F.);
#71312=ORIENTED_EDGE('',*,*,#49290,.F.);
#71313=ORIENTED_EDGE('',*,*,#49300,.F.);
#71314=ORIENTED_EDGE('',*,*,#49297,.F.);
#71315=ORIENTED_EDGE('',*,*,#49294,.F.);
#71316=ORIENTED_EDGE('',*,*,#49302,.F.);
#71317=ORIENTED_EDGE('',*,*,#49312,.F.);
#71318=ORIENTED_EDGE('',*,*,#49309,.F.);
#71319=ORIENTED_EDGE('',*,*,#49306,.F.);
#71320=ORIENTED_EDGE('',*,*,#49314,.F.);
#71321=ORIENTED_EDGE('',*,*,#49324,.F.);
#71322=ORIENTED_EDGE('',*,*,#49321,.F.);
#71323=ORIENTED_EDGE('',*,*,#49318,.F.);
#71324=ORIENTED_EDGE('',*,*,#49326,.F.);
#71325=ORIENTED_EDGE('',*,*,#49336,.F.);
#71326=ORIENTED_EDGE('',*,*,#49333,.F.);
#71327=ORIENTED_EDGE('',*,*,#49330,.F.);
#71328=ORIENTED_EDGE('',*,*,#49338,.F.);
#71329=ORIENTED_EDGE('',*,*,#49348,.F.);
#71330=ORIENTED_EDGE('',*,*,#49345,.F.);
#71331=ORIENTED_EDGE('',*,*,#49342,.F.);
#71332=ORIENTED_EDGE('',*,*,#49350,.F.);
#71333=ORIENTED_EDGE('',*,*,#49360,.F.);
#71334=ORIENTED_EDGE('',*,*,#49357,.F.);
#71335=ORIENTED_EDGE('',*,*,#49354,.F.);
#71336=ORIENTED_EDGE('',*,*,#49362,.F.);
#71337=ORIENTED_EDGE('',*,*,#49372,.F.);
#71338=ORIENTED_EDGE('',*,*,#49369,.F.);
#71339=ORIENTED_EDGE('',*,*,#49366,.F.);
#71340=ORIENTED_EDGE('',*,*,#49374,.F.);
#71341=ORIENTED_EDGE('',*,*,#49384,.F.);
#71342=ORIENTED_EDGE('',*,*,#49381,.F.);
#71343=ORIENTED_EDGE('',*,*,#49378,.F.);
#71344=ORIENTED_EDGE('',*,*,#49386,.F.);
#71345=ORIENTED_EDGE('',*,*,#49396,.F.);
#71346=ORIENTED_EDGE('',*,*,#49393,.F.);
#71347=ORIENTED_EDGE('',*,*,#49390,.F.);
#71348=ORIENTED_EDGE('',*,*,#49398,.F.);
#71349=ORIENTED_EDGE('',*,*,#49408,.F.);
#71350=ORIENTED_EDGE('',*,*,#49405,.F.);
#71351=ORIENTED_EDGE('',*,*,#49402,.F.);
#71352=ORIENTED_EDGE('',*,*,#49410,.F.);
#71353=ORIENTED_EDGE('',*,*,#49420,.F.);
#71354=ORIENTED_EDGE('',*,*,#49417,.F.);
#71355=ORIENTED_EDGE('',*,*,#49414,.F.);
#71356=ORIENTED_EDGE('',*,*,#49422,.F.);
#71357=ORIENTED_EDGE('',*,*,#49432,.F.);
#71358=ORIENTED_EDGE('',*,*,#49429,.F.);
#71359=ORIENTED_EDGE('',*,*,#49426,.F.);
#71360=ORIENTED_EDGE('',*,*,#49434,.F.);
#71361=ORIENTED_EDGE('',*,*,#49444,.F.);
#71362=ORIENTED_EDGE('',*,*,#49441,.F.);
#71363=ORIENTED_EDGE('',*,*,#49438,.F.);
#71364=ORIENTED_EDGE('',*,*,#49446,.F.);
#71365=ORIENTED_EDGE('',*,*,#49456,.F.);
#71366=ORIENTED_EDGE('',*,*,#49453,.F.);
#71367=ORIENTED_EDGE('',*,*,#49450,.F.);
#71368=ORIENTED_EDGE('',*,*,#49458,.F.);
#71369=ORIENTED_EDGE('',*,*,#49468,.F.);
#71370=ORIENTED_EDGE('',*,*,#49465,.F.);
#71371=ORIENTED_EDGE('',*,*,#49462,.F.);
#71372=ORIENTED_EDGE('',*,*,#49470,.F.);
#71373=ORIENTED_EDGE('',*,*,#49480,.F.);
#71374=ORIENTED_EDGE('',*,*,#49477,.F.);
#71375=ORIENTED_EDGE('',*,*,#49474,.F.);
#71376=ORIENTED_EDGE('',*,*,#49482,.F.);
#71377=ORIENTED_EDGE('',*,*,#49492,.F.);
#71378=ORIENTED_EDGE('',*,*,#49489,.F.);
#71379=ORIENTED_EDGE('',*,*,#49486,.F.);
#71380=ORIENTED_EDGE('',*,*,#49494,.F.);
#71381=ORIENTED_EDGE('',*,*,#49504,.F.);
#71382=ORIENTED_EDGE('',*,*,#49501,.F.);
#71383=ORIENTED_EDGE('',*,*,#49498,.F.);
#71384=ORIENTED_EDGE('',*,*,#49506,.F.);
#71385=ORIENTED_EDGE('',*,*,#49516,.F.);
#71386=ORIENTED_EDGE('',*,*,#49513,.F.);
#71387=ORIENTED_EDGE('',*,*,#49510,.F.);
#71388=ORIENTED_EDGE('',*,*,#49518,.F.);
#71389=ORIENTED_EDGE('',*,*,#49528,.F.);
#71390=ORIENTED_EDGE('',*,*,#49525,.F.);
#71391=ORIENTED_EDGE('',*,*,#49522,.F.);
#71392=ORIENTED_EDGE('',*,*,#49530,.F.);
#71393=ORIENTED_EDGE('',*,*,#49540,.F.);
#71394=ORIENTED_EDGE('',*,*,#49537,.F.);
#71395=ORIENTED_EDGE('',*,*,#49534,.F.);
#71396=ORIENTED_EDGE('',*,*,#49542,.F.);
#71397=ORIENTED_EDGE('',*,*,#49552,.F.);
#71398=ORIENTED_EDGE('',*,*,#49549,.F.);
#71399=ORIENTED_EDGE('',*,*,#49546,.F.);
#71400=ORIENTED_EDGE('',*,*,#49554,.F.);
#71401=ORIENTED_EDGE('',*,*,#49564,.F.);
#71402=ORIENTED_EDGE('',*,*,#49561,.F.);
#71403=ORIENTED_EDGE('',*,*,#49558,.F.);
#71404=ORIENTED_EDGE('',*,*,#49566,.F.);
#71405=ORIENTED_EDGE('',*,*,#49576,.F.);
#71406=ORIENTED_EDGE('',*,*,#49573,.F.);
#71407=ORIENTED_EDGE('',*,*,#49570,.F.);
#71408=ORIENTED_EDGE('',*,*,#49578,.F.);
#71409=ORIENTED_EDGE('',*,*,#49588,.F.);
#71410=ORIENTED_EDGE('',*,*,#49585,.F.);
#71411=ORIENTED_EDGE('',*,*,#49582,.F.);
#71412=ORIENTED_EDGE('',*,*,#49590,.F.);
#71413=ORIENTED_EDGE('',*,*,#49600,.F.);
#71414=ORIENTED_EDGE('',*,*,#49597,.F.);
#71415=ORIENTED_EDGE('',*,*,#49594,.F.);
#71416=ORIENTED_EDGE('',*,*,#49602,.F.);
#71417=ORIENTED_EDGE('',*,*,#49612,.F.);
#71418=ORIENTED_EDGE('',*,*,#49609,.F.);
#71419=ORIENTED_EDGE('',*,*,#49606,.F.);
#71420=ORIENTED_EDGE('',*,*,#49614,.F.);
#71421=ORIENTED_EDGE('',*,*,#49624,.F.);
#71422=ORIENTED_EDGE('',*,*,#49621,.F.);
#71423=ORIENTED_EDGE('',*,*,#49618,.F.);
#71424=ORIENTED_EDGE('',*,*,#49626,.F.);
#71425=ORIENTED_EDGE('',*,*,#49636,.F.);
#71426=ORIENTED_EDGE('',*,*,#49633,.F.);
#71427=ORIENTED_EDGE('',*,*,#49630,.F.);
#71428=ORIENTED_EDGE('',*,*,#49638,.F.);
#71429=ORIENTED_EDGE('',*,*,#49648,.F.);
#71430=ORIENTED_EDGE('',*,*,#49645,.F.);
#71431=ORIENTED_EDGE('',*,*,#49642,.F.);
#71432=ORIENTED_EDGE('',*,*,#49650,.F.);
#71433=ORIENTED_EDGE('',*,*,#49660,.F.);
#71434=ORIENTED_EDGE('',*,*,#49657,.F.);
#71435=ORIENTED_EDGE('',*,*,#49654,.F.);
#71436=ORIENTED_EDGE('',*,*,#49662,.F.);
#71437=ORIENTED_EDGE('',*,*,#49672,.F.);
#71438=ORIENTED_EDGE('',*,*,#49669,.F.);
#71439=ORIENTED_EDGE('',*,*,#49666,.F.);
#71440=ORIENTED_EDGE('',*,*,#49674,.F.);
#71441=ORIENTED_EDGE('',*,*,#49684,.F.);
#71442=ORIENTED_EDGE('',*,*,#49681,.F.);
#71443=ORIENTED_EDGE('',*,*,#49678,.F.);
#71444=ORIENTED_EDGE('',*,*,#49686,.F.);
#71445=ORIENTED_EDGE('',*,*,#49696,.F.);
#71446=ORIENTED_EDGE('',*,*,#49693,.F.);
#71447=ORIENTED_EDGE('',*,*,#49690,.F.);
#71448=ORIENTED_EDGE('',*,*,#49698,.F.);
#71449=ORIENTED_EDGE('',*,*,#49708,.F.);
#71450=ORIENTED_EDGE('',*,*,#49705,.F.);
#71451=ORIENTED_EDGE('',*,*,#49702,.F.);
#71452=ORIENTED_EDGE('',*,*,#49710,.F.);
#71453=ORIENTED_EDGE('',*,*,#49720,.F.);
#71454=ORIENTED_EDGE('',*,*,#49717,.F.);
#71455=ORIENTED_EDGE('',*,*,#49714,.F.);
#71456=ORIENTED_EDGE('',*,*,#49722,.F.);
#71457=ORIENTED_EDGE('',*,*,#49732,.F.);
#71458=ORIENTED_EDGE('',*,*,#49729,.F.);
#71459=ORIENTED_EDGE('',*,*,#49726,.F.);
#71460=ORIENTED_EDGE('',*,*,#49734,.F.);
#71461=ORIENTED_EDGE('',*,*,#49744,.F.);
#71462=ORIENTED_EDGE('',*,*,#49741,.F.);
#71463=ORIENTED_EDGE('',*,*,#49738,.F.);
#71464=ORIENTED_EDGE('',*,*,#49746,.F.);
#71465=ORIENTED_EDGE('',*,*,#49756,.F.);
#71466=ORIENTED_EDGE('',*,*,#49753,.F.);
#71467=ORIENTED_EDGE('',*,*,#49750,.F.);
#71468=ORIENTED_EDGE('',*,*,#49758,.F.);
#71469=ORIENTED_EDGE('',*,*,#49768,.F.);
#71470=ORIENTED_EDGE('',*,*,#49765,.F.);
#71471=ORIENTED_EDGE('',*,*,#49762,.F.);
#71472=ORIENTED_EDGE('',*,*,#49770,.F.);
#71473=ORIENTED_EDGE('',*,*,#49780,.F.);
#71474=ORIENTED_EDGE('',*,*,#49777,.F.);
#71475=ORIENTED_EDGE('',*,*,#49774,.F.);
#71476=ORIENTED_EDGE('',*,*,#49782,.F.);
#71477=ORIENTED_EDGE('',*,*,#49792,.F.);
#71478=ORIENTED_EDGE('',*,*,#49789,.F.);
#71479=ORIENTED_EDGE('',*,*,#49786,.F.);
#71480=ORIENTED_EDGE('',*,*,#49794,.F.);
#71481=ORIENTED_EDGE('',*,*,#49804,.F.);
#71482=ORIENTED_EDGE('',*,*,#49801,.F.);
#71483=ORIENTED_EDGE('',*,*,#49798,.F.);
#71484=ORIENTED_EDGE('',*,*,#49806,.F.);
#71485=ORIENTED_EDGE('',*,*,#49816,.F.);
#71486=ORIENTED_EDGE('',*,*,#49813,.F.);
#71487=ORIENTED_EDGE('',*,*,#49810,.F.);
#71488=ORIENTED_EDGE('',*,*,#49818,.F.);
#71489=ORIENTED_EDGE('',*,*,#49828,.F.);
#71490=ORIENTED_EDGE('',*,*,#49825,.F.);
#71491=ORIENTED_EDGE('',*,*,#49822,.F.);
#71492=ORIENTED_EDGE('',*,*,#49830,.F.);
#71493=ORIENTED_EDGE('',*,*,#49840,.F.);
#71494=ORIENTED_EDGE('',*,*,#49837,.F.);
#71495=ORIENTED_EDGE('',*,*,#49834,.F.);
#71496=ORIENTED_EDGE('',*,*,#49842,.F.);
#71497=ORIENTED_EDGE('',*,*,#49852,.F.);
#71498=ORIENTED_EDGE('',*,*,#49849,.F.);
#71499=ORIENTED_EDGE('',*,*,#49846,.F.);
#71500=ORIENTED_EDGE('',*,*,#49854,.F.);
#71501=ORIENTED_EDGE('',*,*,#49864,.F.);
#71502=ORIENTED_EDGE('',*,*,#49861,.F.);
#71503=ORIENTED_EDGE('',*,*,#49858,.F.);
#71504=ORIENTED_EDGE('',*,*,#49866,.F.);
#71505=ORIENTED_EDGE('',*,*,#49876,.F.);
#71506=ORIENTED_EDGE('',*,*,#49873,.F.);
#71507=ORIENTED_EDGE('',*,*,#49870,.F.);
#71508=ORIENTED_EDGE('',*,*,#49878,.F.);
#71509=ORIENTED_EDGE('',*,*,#49888,.F.);
#71510=ORIENTED_EDGE('',*,*,#49885,.F.);
#71511=ORIENTED_EDGE('',*,*,#49882,.F.);
#71512=ORIENTED_EDGE('',*,*,#49890,.F.);
#71513=ORIENTED_EDGE('',*,*,#49900,.F.);
#71514=ORIENTED_EDGE('',*,*,#49897,.F.);
#71515=ORIENTED_EDGE('',*,*,#49894,.F.);
#71516=ORIENTED_EDGE('',*,*,#49902,.F.);
#71517=ORIENTED_EDGE('',*,*,#49912,.F.);
#71518=ORIENTED_EDGE('',*,*,#49909,.F.);
#71519=ORIENTED_EDGE('',*,*,#49906,.F.);
#71520=ORIENTED_EDGE('',*,*,#49914,.F.);
#71521=ORIENTED_EDGE('',*,*,#49924,.F.);
#71522=ORIENTED_EDGE('',*,*,#49921,.F.);
#71523=ORIENTED_EDGE('',*,*,#49918,.F.);
#71524=ORIENTED_EDGE('',*,*,#49926,.F.);
#71525=ORIENTED_EDGE('',*,*,#49936,.F.);
#71526=ORIENTED_EDGE('',*,*,#49933,.F.);
#71527=ORIENTED_EDGE('',*,*,#49930,.F.);
#71528=ORIENTED_EDGE('',*,*,#49938,.F.);
#71529=ORIENTED_EDGE('',*,*,#49948,.F.);
#71530=ORIENTED_EDGE('',*,*,#49945,.F.);
#71531=ORIENTED_EDGE('',*,*,#49942,.F.);
#71532=ORIENTED_EDGE('',*,*,#49950,.F.);
#71533=ORIENTED_EDGE('',*,*,#49960,.F.);
#71534=ORIENTED_EDGE('',*,*,#49957,.F.);
#71535=ORIENTED_EDGE('',*,*,#49954,.F.);
#71536=ORIENTED_EDGE('',*,*,#49962,.F.);
#71537=ORIENTED_EDGE('',*,*,#49972,.F.);
#71538=ORIENTED_EDGE('',*,*,#49969,.F.);
#71539=ORIENTED_EDGE('',*,*,#49966,.F.);
#71540=ORIENTED_EDGE('',*,*,#49974,.F.);
#71541=ORIENTED_EDGE('',*,*,#49984,.F.);
#71542=ORIENTED_EDGE('',*,*,#49981,.F.);
#71543=ORIENTED_EDGE('',*,*,#49978,.F.);
#71544=ORIENTED_EDGE('',*,*,#49986,.F.);
#71545=ORIENTED_EDGE('',*,*,#49996,.F.);
#71546=ORIENTED_EDGE('',*,*,#49993,.F.);
#71547=ORIENTED_EDGE('',*,*,#49990,.F.);
#71548=ORIENTED_EDGE('',*,*,#49998,.F.);
#71549=ORIENTED_EDGE('',*,*,#50008,.F.);
#71550=ORIENTED_EDGE('',*,*,#50005,.F.);
#71551=ORIENTED_EDGE('',*,*,#50002,.F.);
#71552=ORIENTED_EDGE('',*,*,#50010,.F.);
#71553=ORIENTED_EDGE('',*,*,#50020,.F.);
#71554=ORIENTED_EDGE('',*,*,#50017,.F.);
#71555=ORIENTED_EDGE('',*,*,#50014,.F.);
#71556=ORIENTED_EDGE('',*,*,#50022,.F.);
#71557=ORIENTED_EDGE('',*,*,#50032,.F.);
#71558=ORIENTED_EDGE('',*,*,#50029,.F.);
#71559=ORIENTED_EDGE('',*,*,#50026,.F.);
#71560=ORIENTED_EDGE('',*,*,#50034,.F.);
#71561=ORIENTED_EDGE('',*,*,#50044,.F.);
#71562=ORIENTED_EDGE('',*,*,#50041,.F.);
#71563=ORIENTED_EDGE('',*,*,#50038,.F.);
#71564=ORIENTED_EDGE('',*,*,#50046,.F.);
#71565=ORIENTED_EDGE('',*,*,#50056,.F.);
#71566=ORIENTED_EDGE('',*,*,#50053,.F.);
#71567=ORIENTED_EDGE('',*,*,#50050,.F.);
#71568=ORIENTED_EDGE('',*,*,#50058,.F.);
#71569=ORIENTED_EDGE('',*,*,#50068,.F.);
#71570=ORIENTED_EDGE('',*,*,#50065,.F.);
#71571=ORIENTED_EDGE('',*,*,#50062,.F.);
#71572=ORIENTED_EDGE('',*,*,#50070,.F.);
#71573=ORIENTED_EDGE('',*,*,#50080,.F.);
#71574=ORIENTED_EDGE('',*,*,#50077,.F.);
#71575=ORIENTED_EDGE('',*,*,#50074,.F.);
#71576=ORIENTED_EDGE('',*,*,#50082,.F.);
#71577=ORIENTED_EDGE('',*,*,#50092,.F.);
#71578=ORIENTED_EDGE('',*,*,#50089,.F.);
#71579=ORIENTED_EDGE('',*,*,#50086,.F.);
#71580=ORIENTED_EDGE('',*,*,#50094,.F.);
#71581=ORIENTED_EDGE('',*,*,#50104,.F.);
#71582=ORIENTED_EDGE('',*,*,#50101,.F.);
#71583=ORIENTED_EDGE('',*,*,#50098,.F.);
#71584=ORIENTED_EDGE('',*,*,#50106,.F.);
#71585=ORIENTED_EDGE('',*,*,#50116,.F.);
#71586=ORIENTED_EDGE('',*,*,#50113,.F.);
#71587=ORIENTED_EDGE('',*,*,#50110,.F.);
#71588=ORIENTED_EDGE('',*,*,#50118,.F.);
#71589=ORIENTED_EDGE('',*,*,#50128,.F.);
#71590=ORIENTED_EDGE('',*,*,#50125,.F.);
#71591=ORIENTED_EDGE('',*,*,#50122,.F.);
#71592=ORIENTED_EDGE('',*,*,#50130,.F.);
#71593=ORIENTED_EDGE('',*,*,#50140,.F.);
#71594=ORIENTED_EDGE('',*,*,#50137,.F.);
#71595=ORIENTED_EDGE('',*,*,#50134,.F.);
#71596=ORIENTED_EDGE('',*,*,#50142,.F.);
#71597=ORIENTED_EDGE('',*,*,#50152,.F.);
#71598=ORIENTED_EDGE('',*,*,#50149,.F.);
#71599=ORIENTED_EDGE('',*,*,#50146,.F.);
#71600=ORIENTED_EDGE('',*,*,#50154,.F.);
#71601=ORIENTED_EDGE('',*,*,#50164,.F.);
#71602=ORIENTED_EDGE('',*,*,#50161,.F.);
#71603=ORIENTED_EDGE('',*,*,#50158,.F.);
#71604=ORIENTED_EDGE('',*,*,#50166,.F.);
#71605=ORIENTED_EDGE('',*,*,#50176,.F.);
#71606=ORIENTED_EDGE('',*,*,#50173,.F.);
#71607=ORIENTED_EDGE('',*,*,#50170,.F.);
#71608=ORIENTED_EDGE('',*,*,#50178,.F.);
#71609=ORIENTED_EDGE('',*,*,#50188,.F.);
#71610=ORIENTED_EDGE('',*,*,#50185,.F.);
#71611=ORIENTED_EDGE('',*,*,#50182,.F.);
#71612=ORIENTED_EDGE('',*,*,#50190,.F.);
#71613=ORIENTED_EDGE('',*,*,#50200,.F.);
#71614=ORIENTED_EDGE('',*,*,#50197,.F.);
#71615=ORIENTED_EDGE('',*,*,#50194,.F.);
#71616=ORIENTED_EDGE('',*,*,#50202,.F.);
#71617=ORIENTED_EDGE('',*,*,#50212,.F.);
#71618=ORIENTED_EDGE('',*,*,#50209,.F.);
#71619=ORIENTED_EDGE('',*,*,#50206,.F.);
#71620=ORIENTED_EDGE('',*,*,#50214,.F.);
#71621=ORIENTED_EDGE('',*,*,#50224,.F.);
#71622=ORIENTED_EDGE('',*,*,#50221,.F.);
#71623=ORIENTED_EDGE('',*,*,#50218,.F.);
#71624=ORIENTED_EDGE('',*,*,#50226,.F.);
#71625=ORIENTED_EDGE('',*,*,#50236,.F.);
#71626=ORIENTED_EDGE('',*,*,#50233,.F.);
#71627=ORIENTED_EDGE('',*,*,#50230,.F.);
#71628=ORIENTED_EDGE('',*,*,#50238,.F.);
#71629=ORIENTED_EDGE('',*,*,#50248,.F.);
#71630=ORIENTED_EDGE('',*,*,#50245,.F.);
#71631=ORIENTED_EDGE('',*,*,#50242,.F.);
#71632=ORIENTED_EDGE('',*,*,#50250,.F.);
#71633=ORIENTED_EDGE('',*,*,#50260,.F.);
#71634=ORIENTED_EDGE('',*,*,#50257,.F.);
#71635=ORIENTED_EDGE('',*,*,#50254,.F.);
#71636=ORIENTED_EDGE('',*,*,#50262,.F.);
#71637=ORIENTED_EDGE('',*,*,#50272,.F.);
#71638=ORIENTED_EDGE('',*,*,#50269,.F.);
#71639=ORIENTED_EDGE('',*,*,#50266,.F.);
#71640=ORIENTED_EDGE('',*,*,#50274,.F.);
#71641=ORIENTED_EDGE('',*,*,#50284,.F.);
#71642=ORIENTED_EDGE('',*,*,#50281,.F.);
#71643=ORIENTED_EDGE('',*,*,#50278,.F.);
#71644=ORIENTED_EDGE('',*,*,#50286,.F.);
#71645=ORIENTED_EDGE('',*,*,#50296,.F.);
#71646=ORIENTED_EDGE('',*,*,#50293,.F.);
#71647=ORIENTED_EDGE('',*,*,#50290,.F.);
#71648=ORIENTED_EDGE('',*,*,#50298,.F.);
#71649=ORIENTED_EDGE('',*,*,#50308,.F.);
#71650=ORIENTED_EDGE('',*,*,#50305,.F.);
#71651=ORIENTED_EDGE('',*,*,#50302,.F.);
#71652=ORIENTED_EDGE('',*,*,#50310,.F.);
#71653=ORIENTED_EDGE('',*,*,#50320,.F.);
#71654=ORIENTED_EDGE('',*,*,#50317,.F.);
#71655=ORIENTED_EDGE('',*,*,#50314,.F.);
#71656=ORIENTED_EDGE('',*,*,#50322,.F.);
#71657=ORIENTED_EDGE('',*,*,#50332,.F.);
#71658=ORIENTED_EDGE('',*,*,#50329,.F.);
#71659=ORIENTED_EDGE('',*,*,#50326,.F.);
#71660=ORIENTED_EDGE('',*,*,#50334,.F.);
#71661=ORIENTED_EDGE('',*,*,#50344,.F.);
#71662=ORIENTED_EDGE('',*,*,#50341,.F.);
#71663=ORIENTED_EDGE('',*,*,#50338,.F.);
#71664=ORIENTED_EDGE('',*,*,#50346,.F.);
#71665=ORIENTED_EDGE('',*,*,#50356,.F.);
#71666=ORIENTED_EDGE('',*,*,#50353,.F.);
#71667=ORIENTED_EDGE('',*,*,#50350,.F.);
#71668=ORIENTED_EDGE('',*,*,#50358,.F.);
#71669=ORIENTED_EDGE('',*,*,#50368,.F.);
#71670=ORIENTED_EDGE('',*,*,#50365,.F.);
#71671=ORIENTED_EDGE('',*,*,#50362,.F.);
#71672=ORIENTED_EDGE('',*,*,#50370,.F.);
#71673=ORIENTED_EDGE('',*,*,#50380,.F.);
#71674=ORIENTED_EDGE('',*,*,#50377,.F.);
#71675=ORIENTED_EDGE('',*,*,#50374,.F.);
#71676=ORIENTED_EDGE('',*,*,#50382,.F.);
#71677=ORIENTED_EDGE('',*,*,#50392,.F.);
#71678=ORIENTED_EDGE('',*,*,#50389,.F.);
#71679=ORIENTED_EDGE('',*,*,#50386,.F.);
#71680=ORIENTED_EDGE('',*,*,#50394,.F.);
#71681=ORIENTED_EDGE('',*,*,#50404,.F.);
#71682=ORIENTED_EDGE('',*,*,#50401,.F.);
#71683=ORIENTED_EDGE('',*,*,#50398,.F.);
#71684=ORIENTED_EDGE('',*,*,#50406,.F.);
#71685=ORIENTED_EDGE('',*,*,#50416,.F.);
#71686=ORIENTED_EDGE('',*,*,#50413,.F.);
#71687=ORIENTED_EDGE('',*,*,#50410,.F.);
#71688=ORIENTED_EDGE('',*,*,#50418,.F.);
#71689=ORIENTED_EDGE('',*,*,#50428,.F.);
#71690=ORIENTED_EDGE('',*,*,#50425,.F.);
#71691=ORIENTED_EDGE('',*,*,#50422,.F.);
#71692=ORIENTED_EDGE('',*,*,#50430,.F.);
#71693=ORIENTED_EDGE('',*,*,#50440,.F.);
#71694=ORIENTED_EDGE('',*,*,#50437,.F.);
#71695=ORIENTED_EDGE('',*,*,#50434,.F.);
#71696=ORIENTED_EDGE('',*,*,#50442,.F.);
#71697=ORIENTED_EDGE('',*,*,#50452,.F.);
#71698=ORIENTED_EDGE('',*,*,#50449,.F.);
#71699=ORIENTED_EDGE('',*,*,#50446,.F.);
#71700=ORIENTED_EDGE('',*,*,#50454,.F.);
#71701=ORIENTED_EDGE('',*,*,#50464,.F.);
#71702=ORIENTED_EDGE('',*,*,#50461,.F.);
#71703=ORIENTED_EDGE('',*,*,#50458,.F.);
#71704=ORIENTED_EDGE('',*,*,#50466,.F.);
#71705=ORIENTED_EDGE('',*,*,#50476,.F.);
#71706=ORIENTED_EDGE('',*,*,#50473,.F.);
#71707=ORIENTED_EDGE('',*,*,#50470,.F.);
#71708=ORIENTED_EDGE('',*,*,#50478,.F.);
#71709=ORIENTED_EDGE('',*,*,#50488,.F.);
#71710=ORIENTED_EDGE('',*,*,#50485,.F.);
#71711=ORIENTED_EDGE('',*,*,#50482,.F.);
#71712=ORIENTED_EDGE('',*,*,#50490,.F.);
#71713=ORIENTED_EDGE('',*,*,#50500,.F.);
#71714=ORIENTED_EDGE('',*,*,#50497,.F.);
#71715=ORIENTED_EDGE('',*,*,#50494,.F.);
#71716=ORIENTED_EDGE('',*,*,#50502,.F.);
#71717=ORIENTED_EDGE('',*,*,#50512,.F.);
#71718=ORIENTED_EDGE('',*,*,#50509,.F.);
#71719=ORIENTED_EDGE('',*,*,#50506,.F.);
#71720=ORIENTED_EDGE('',*,*,#50514,.F.);
#71721=ORIENTED_EDGE('',*,*,#50524,.F.);
#71722=ORIENTED_EDGE('',*,*,#50521,.F.);
#71723=ORIENTED_EDGE('',*,*,#50518,.F.);
#71724=ORIENTED_EDGE('',*,*,#50526,.F.);
#71725=ORIENTED_EDGE('',*,*,#50536,.F.);
#71726=ORIENTED_EDGE('',*,*,#50533,.F.);
#71727=ORIENTED_EDGE('',*,*,#50530,.F.);
#71728=ORIENTED_EDGE('',*,*,#50538,.F.);
#71729=ORIENTED_EDGE('',*,*,#50548,.F.);
#71730=ORIENTED_EDGE('',*,*,#50545,.F.);
#71731=ORIENTED_EDGE('',*,*,#50542,.F.);
#71732=ORIENTED_EDGE('',*,*,#50550,.F.);
#71733=ORIENTED_EDGE('',*,*,#50560,.F.);
#71734=ORIENTED_EDGE('',*,*,#50557,.F.);
#71735=ORIENTED_EDGE('',*,*,#50554,.F.);
#71736=ORIENTED_EDGE('',*,*,#50562,.F.);
#71737=ORIENTED_EDGE('',*,*,#50572,.F.);
#71738=ORIENTED_EDGE('',*,*,#50569,.F.);
#71739=ORIENTED_EDGE('',*,*,#50566,.F.);
#71740=ORIENTED_EDGE('',*,*,#50574,.F.);
#71741=ORIENTED_EDGE('',*,*,#50584,.F.);
#71742=ORIENTED_EDGE('',*,*,#50581,.F.);
#71743=ORIENTED_EDGE('',*,*,#50578,.F.);
#71744=ORIENTED_EDGE('',*,*,#50586,.F.);
#71745=ORIENTED_EDGE('',*,*,#50596,.F.);
#71746=ORIENTED_EDGE('',*,*,#50593,.F.);
#71747=ORIENTED_EDGE('',*,*,#50590,.F.);
#71748=ORIENTED_EDGE('',*,*,#50598,.F.);
#71749=ORIENTED_EDGE('',*,*,#50608,.F.);
#71750=ORIENTED_EDGE('',*,*,#50605,.F.);
#71751=ORIENTED_EDGE('',*,*,#50602,.F.);
#71752=ORIENTED_EDGE('',*,*,#50610,.F.);
#71753=ORIENTED_EDGE('',*,*,#50620,.F.);
#71754=ORIENTED_EDGE('',*,*,#50617,.F.);
#71755=ORIENTED_EDGE('',*,*,#50614,.F.);
#71756=ORIENTED_EDGE('',*,*,#50622,.F.);
#71757=ORIENTED_EDGE('',*,*,#50632,.F.);
#71758=ORIENTED_EDGE('',*,*,#50629,.F.);
#71759=ORIENTED_EDGE('',*,*,#50626,.F.);
#71760=ORIENTED_EDGE('',*,*,#50634,.F.);
#71761=ORIENTED_EDGE('',*,*,#50644,.F.);
#71762=ORIENTED_EDGE('',*,*,#50641,.F.);
#71763=ORIENTED_EDGE('',*,*,#50638,.F.);
#71764=ORIENTED_EDGE('',*,*,#50646,.F.);
#71765=ORIENTED_EDGE('',*,*,#50656,.F.);
#71766=ORIENTED_EDGE('',*,*,#50653,.F.);
#71767=ORIENTED_EDGE('',*,*,#50650,.F.);
#71768=ORIENTED_EDGE('',*,*,#50658,.F.);
#71769=ORIENTED_EDGE('',*,*,#50668,.F.);
#71770=ORIENTED_EDGE('',*,*,#50665,.F.);
#71771=ORIENTED_EDGE('',*,*,#50662,.F.);
#71772=ORIENTED_EDGE('',*,*,#50670,.F.);
#71773=ORIENTED_EDGE('',*,*,#50680,.F.);
#71774=ORIENTED_EDGE('',*,*,#50677,.F.);
#71775=ORIENTED_EDGE('',*,*,#50674,.F.);
#71776=ORIENTED_EDGE('',*,*,#50682,.F.);
#71777=ORIENTED_EDGE('',*,*,#50692,.F.);
#71778=ORIENTED_EDGE('',*,*,#50689,.F.);
#71779=ORIENTED_EDGE('',*,*,#50686,.F.);
#71780=ORIENTED_EDGE('',*,*,#50694,.F.);
#71781=ORIENTED_EDGE('',*,*,#50704,.F.);
#71782=ORIENTED_EDGE('',*,*,#50701,.F.);
#71783=ORIENTED_EDGE('',*,*,#50698,.F.);
#71784=ORIENTED_EDGE('',*,*,#50706,.F.);
#71785=ORIENTED_EDGE('',*,*,#50716,.F.);
#71786=ORIENTED_EDGE('',*,*,#50713,.F.);
#71787=ORIENTED_EDGE('',*,*,#50710,.F.);
#71788=ORIENTED_EDGE('',*,*,#50718,.F.);
#71789=ORIENTED_EDGE('',*,*,#50728,.F.);
#71790=ORIENTED_EDGE('',*,*,#50725,.F.);
#71791=ORIENTED_EDGE('',*,*,#50722,.F.);
#71792=ORIENTED_EDGE('',*,*,#50730,.F.);
#71793=ORIENTED_EDGE('',*,*,#50740,.F.);
#71794=ORIENTED_EDGE('',*,*,#50737,.F.);
#71795=ORIENTED_EDGE('',*,*,#50734,.F.);
#71796=ORIENTED_EDGE('',*,*,#50742,.F.);
#71797=ORIENTED_EDGE('',*,*,#50752,.F.);
#71798=ORIENTED_EDGE('',*,*,#50749,.F.);
#71799=ORIENTED_EDGE('',*,*,#50746,.F.);
#71800=ORIENTED_EDGE('',*,*,#50754,.F.);
#71801=ORIENTED_EDGE('',*,*,#50764,.F.);
#71802=ORIENTED_EDGE('',*,*,#50761,.F.);
#71803=ORIENTED_EDGE('',*,*,#50758,.F.);
#71804=ORIENTED_EDGE('',*,*,#50766,.F.);
#71805=ORIENTED_EDGE('',*,*,#50776,.F.);
#71806=ORIENTED_EDGE('',*,*,#50773,.F.);
#71807=ORIENTED_EDGE('',*,*,#50770,.F.);
#71808=ORIENTED_EDGE('',*,*,#50778,.F.);
#71809=ORIENTED_EDGE('',*,*,#50788,.F.);
#71810=ORIENTED_EDGE('',*,*,#50785,.F.);
#71811=ORIENTED_EDGE('',*,*,#50782,.F.);
#71812=ORIENTED_EDGE('',*,*,#50790,.F.);
#71813=ORIENTED_EDGE('',*,*,#50800,.F.);
#71814=ORIENTED_EDGE('',*,*,#50797,.F.);
#71815=ORIENTED_EDGE('',*,*,#50794,.F.);
#71816=ORIENTED_EDGE('',*,*,#50802,.F.);
#71817=ORIENTED_EDGE('',*,*,#50812,.F.);
#71818=ORIENTED_EDGE('',*,*,#50809,.F.);
#71819=ORIENTED_EDGE('',*,*,#50806,.F.);
#71820=ORIENTED_EDGE('',*,*,#50814,.F.);
#71821=ORIENTED_EDGE('',*,*,#50824,.F.);
#71822=ORIENTED_EDGE('',*,*,#50821,.F.);
#71823=ORIENTED_EDGE('',*,*,#50818,.F.);
#71824=ORIENTED_EDGE('',*,*,#50826,.F.);
#71825=ORIENTED_EDGE('',*,*,#50836,.F.);
#71826=ORIENTED_EDGE('',*,*,#50833,.F.);
#71827=ORIENTED_EDGE('',*,*,#50830,.F.);
#71828=ORIENTED_EDGE('',*,*,#50838,.F.);
#71829=ORIENTED_EDGE('',*,*,#50848,.F.);
#71830=ORIENTED_EDGE('',*,*,#50845,.F.);
#71831=ORIENTED_EDGE('',*,*,#50842,.F.);
#71832=ORIENTED_EDGE('',*,*,#50850,.F.);
#71833=ORIENTED_EDGE('',*,*,#50860,.F.);
#71834=ORIENTED_EDGE('',*,*,#50857,.F.);
#71835=ORIENTED_EDGE('',*,*,#50854,.F.);
#71836=ORIENTED_EDGE('',*,*,#50862,.F.);
#71837=ORIENTED_EDGE('',*,*,#50872,.F.);
#71838=ORIENTED_EDGE('',*,*,#50869,.F.);
#71839=ORIENTED_EDGE('',*,*,#50866,.F.);
#71840=ORIENTED_EDGE('',*,*,#50874,.F.);
#71841=ORIENTED_EDGE('',*,*,#50884,.F.);
#71842=ORIENTED_EDGE('',*,*,#50881,.F.);
#71843=ORIENTED_EDGE('',*,*,#50878,.F.);
#71844=ORIENTED_EDGE('',*,*,#50886,.F.);
#71845=ORIENTED_EDGE('',*,*,#50896,.F.);
#71846=ORIENTED_EDGE('',*,*,#50893,.F.);
#71847=ORIENTED_EDGE('',*,*,#50890,.F.);
#71848=ORIENTED_EDGE('',*,*,#50898,.F.);
#71849=ORIENTED_EDGE('',*,*,#50908,.F.);
#71850=ORIENTED_EDGE('',*,*,#50905,.F.);
#71851=ORIENTED_EDGE('',*,*,#50902,.F.);
#71852=ORIENTED_EDGE('',*,*,#50910,.F.);
#71853=ORIENTED_EDGE('',*,*,#50920,.F.);
#71854=ORIENTED_EDGE('',*,*,#50917,.F.);
#71855=ORIENTED_EDGE('',*,*,#50914,.F.);
#71856=ORIENTED_EDGE('',*,*,#50922,.F.);
#71857=ORIENTED_EDGE('',*,*,#50932,.F.);
#71858=ORIENTED_EDGE('',*,*,#50929,.F.);
#71859=ORIENTED_EDGE('',*,*,#50926,.F.);
#71860=ORIENTED_EDGE('',*,*,#50934,.F.);
#71861=ORIENTED_EDGE('',*,*,#50944,.F.);
#71862=ORIENTED_EDGE('',*,*,#50941,.F.);
#71863=ORIENTED_EDGE('',*,*,#50938,.F.);
#71864=ORIENTED_EDGE('',*,*,#50946,.F.);
#71865=ORIENTED_EDGE('',*,*,#50956,.F.);
#71866=ORIENTED_EDGE('',*,*,#50953,.F.);
#71867=ORIENTED_EDGE('',*,*,#50950,.F.);
#71868=ORIENTED_EDGE('',*,*,#50958,.F.);
#71869=ORIENTED_EDGE('',*,*,#50968,.F.);
#71870=ORIENTED_EDGE('',*,*,#50965,.F.);
#71871=ORIENTED_EDGE('',*,*,#50962,.F.);
#71872=ORIENTED_EDGE('',*,*,#50970,.F.);
#71873=ORIENTED_EDGE('',*,*,#50980,.F.);
#71874=ORIENTED_EDGE('',*,*,#50977,.F.);
#71875=ORIENTED_EDGE('',*,*,#50974,.F.);
#71876=ORIENTED_EDGE('',*,*,#50982,.F.);
#71877=ORIENTED_EDGE('',*,*,#50992,.F.);
#71878=ORIENTED_EDGE('',*,*,#50989,.F.);
#71879=ORIENTED_EDGE('',*,*,#50986,.F.);
#71880=ORIENTED_EDGE('',*,*,#50994,.F.);
#71881=ORIENTED_EDGE('',*,*,#51004,.F.);
#71882=ORIENTED_EDGE('',*,*,#51001,.F.);
#71883=ORIENTED_EDGE('',*,*,#50998,.F.);
#71884=ORIENTED_EDGE('',*,*,#51006,.F.);
#71885=ORIENTED_EDGE('',*,*,#51016,.F.);
#71886=ORIENTED_EDGE('',*,*,#51013,.F.);
#71887=ORIENTED_EDGE('',*,*,#51010,.F.);
#71888=ORIENTED_EDGE('',*,*,#51018,.F.);
#71889=ORIENTED_EDGE('',*,*,#51028,.F.);
#71890=ORIENTED_EDGE('',*,*,#51025,.F.);
#71891=ORIENTED_EDGE('',*,*,#51022,.F.);
#71892=ORIENTED_EDGE('',*,*,#51030,.F.);
#71893=ORIENTED_EDGE('',*,*,#51040,.F.);
#71894=ORIENTED_EDGE('',*,*,#51037,.F.);
#71895=ORIENTED_EDGE('',*,*,#51034,.F.);
#71896=ORIENTED_EDGE('',*,*,#51042,.F.);
#71897=ORIENTED_EDGE('',*,*,#51052,.F.);
#71898=ORIENTED_EDGE('',*,*,#51049,.F.);
#71899=ORIENTED_EDGE('',*,*,#51046,.F.);
#71900=ORIENTED_EDGE('',*,*,#51054,.F.);
#71901=ORIENTED_EDGE('',*,*,#51064,.F.);
#71902=ORIENTED_EDGE('',*,*,#51061,.F.);
#71903=ORIENTED_EDGE('',*,*,#51058,.F.);
#71904=ORIENTED_EDGE('',*,*,#51066,.F.);
#71905=ORIENTED_EDGE('',*,*,#51076,.F.);
#71906=ORIENTED_EDGE('',*,*,#51073,.F.);
#71907=ORIENTED_EDGE('',*,*,#51070,.F.);
#71908=ORIENTED_EDGE('',*,*,#51078,.F.);
#71909=ORIENTED_EDGE('',*,*,#51088,.F.);
#71910=ORIENTED_EDGE('',*,*,#51085,.F.);
#71911=ORIENTED_EDGE('',*,*,#51082,.F.);
#71912=ORIENTED_EDGE('',*,*,#51090,.F.);
#71913=ORIENTED_EDGE('',*,*,#51100,.F.);
#71914=ORIENTED_EDGE('',*,*,#51097,.F.);
#71915=ORIENTED_EDGE('',*,*,#51094,.F.);
#71916=ORIENTED_EDGE('',*,*,#51102,.F.);
#71917=ORIENTED_EDGE('',*,*,#51112,.F.);
#71918=ORIENTED_EDGE('',*,*,#51109,.F.);
#71919=ORIENTED_EDGE('',*,*,#51106,.F.);
#71920=ORIENTED_EDGE('',*,*,#51114,.F.);
#71921=ORIENTED_EDGE('',*,*,#51124,.F.);
#71922=ORIENTED_EDGE('',*,*,#51121,.F.);
#71923=ORIENTED_EDGE('',*,*,#51118,.F.);
#71924=ORIENTED_EDGE('',*,*,#51126,.F.);
#71925=ORIENTED_EDGE('',*,*,#51136,.F.);
#71926=ORIENTED_EDGE('',*,*,#51133,.F.);
#71927=ORIENTED_EDGE('',*,*,#51130,.F.);
#71928=ORIENTED_EDGE('',*,*,#51138,.F.);
#71929=ORIENTED_EDGE('',*,*,#51148,.F.);
#71930=ORIENTED_EDGE('',*,*,#51145,.F.);
#71931=ORIENTED_EDGE('',*,*,#51142,.F.);
#71932=ORIENTED_EDGE('',*,*,#51150,.F.);
#71933=ORIENTED_EDGE('',*,*,#51160,.F.);
#71934=ORIENTED_EDGE('',*,*,#51157,.F.);
#71935=ORIENTED_EDGE('',*,*,#51154,.F.);
#71936=ORIENTED_EDGE('',*,*,#51162,.F.);
#71937=ORIENTED_EDGE('',*,*,#51172,.F.);
#71938=ORIENTED_EDGE('',*,*,#51169,.F.);
#71939=ORIENTED_EDGE('',*,*,#51166,.F.);
#71940=ORIENTED_EDGE('',*,*,#51174,.F.);
#71941=ORIENTED_EDGE('',*,*,#51184,.F.);
#71942=ORIENTED_EDGE('',*,*,#51181,.F.);
#71943=ORIENTED_EDGE('',*,*,#51178,.F.);
#71944=ORIENTED_EDGE('',*,*,#51186,.F.);
#71945=ORIENTED_EDGE('',*,*,#51196,.F.);
#71946=ORIENTED_EDGE('',*,*,#51193,.F.);
#71947=ORIENTED_EDGE('',*,*,#51190,.F.);
#71948=ORIENTED_EDGE('',*,*,#51198,.F.);
#71949=ORIENTED_EDGE('',*,*,#51208,.F.);
#71950=ORIENTED_EDGE('',*,*,#51205,.F.);
#71951=ORIENTED_EDGE('',*,*,#51202,.F.);
#71952=ORIENTED_EDGE('',*,*,#51210,.F.);
#71953=ORIENTED_EDGE('',*,*,#51220,.F.);
#71954=ORIENTED_EDGE('',*,*,#51217,.F.);
#71955=ORIENTED_EDGE('',*,*,#51214,.F.);
#71956=ORIENTED_EDGE('',*,*,#51222,.F.);
#71957=ORIENTED_EDGE('',*,*,#51232,.F.);
#71958=ORIENTED_EDGE('',*,*,#51229,.F.);
#71959=ORIENTED_EDGE('',*,*,#51226,.F.);
#71960=ORIENTED_EDGE('',*,*,#51234,.F.);
#71961=ORIENTED_EDGE('',*,*,#51244,.F.);
#71962=ORIENTED_EDGE('',*,*,#51241,.F.);
#71963=ORIENTED_EDGE('',*,*,#51238,.F.);
#71964=ORIENTED_EDGE('',*,*,#51246,.F.);
#71965=ORIENTED_EDGE('',*,*,#51256,.F.);
#71966=ORIENTED_EDGE('',*,*,#51253,.F.);
#71967=ORIENTED_EDGE('',*,*,#51250,.F.);
#71968=ORIENTED_EDGE('',*,*,#51258,.F.);
#71969=ORIENTED_EDGE('',*,*,#51268,.F.);
#71970=ORIENTED_EDGE('',*,*,#51265,.F.);
#71971=ORIENTED_EDGE('',*,*,#51262,.F.);
#71972=ORIENTED_EDGE('',*,*,#51270,.F.);
#71973=ORIENTED_EDGE('',*,*,#51280,.F.);
#71974=ORIENTED_EDGE('',*,*,#51277,.F.);
#71975=ORIENTED_EDGE('',*,*,#51274,.F.);
#71976=ORIENTED_EDGE('',*,*,#51282,.F.);
#71977=ORIENTED_EDGE('',*,*,#51292,.F.);
#71978=ORIENTED_EDGE('',*,*,#51289,.F.);
#71979=ORIENTED_EDGE('',*,*,#51286,.F.);
#71980=ORIENTED_EDGE('',*,*,#51294,.F.);
#71981=ORIENTED_EDGE('',*,*,#51304,.F.);
#71982=ORIENTED_EDGE('',*,*,#51301,.F.);
#71983=ORIENTED_EDGE('',*,*,#51298,.F.);
#71984=ORIENTED_EDGE('',*,*,#51306,.F.);
#71985=ORIENTED_EDGE('',*,*,#51316,.F.);
#71986=ORIENTED_EDGE('',*,*,#51313,.F.);
#71987=ORIENTED_EDGE('',*,*,#51310,.F.);
#71988=ORIENTED_EDGE('',*,*,#51318,.F.);
#71989=ORIENTED_EDGE('',*,*,#51328,.F.);
#71990=ORIENTED_EDGE('',*,*,#51325,.F.);
#71991=ORIENTED_EDGE('',*,*,#51322,.F.);
#71992=ORIENTED_EDGE('',*,*,#51330,.F.);
#71993=ORIENTED_EDGE('',*,*,#51340,.F.);
#71994=ORIENTED_EDGE('',*,*,#51337,.F.);
#71995=ORIENTED_EDGE('',*,*,#51334,.F.);
#71996=ORIENTED_EDGE('',*,*,#51342,.F.);
#71997=ORIENTED_EDGE('',*,*,#51352,.F.);
#71998=ORIENTED_EDGE('',*,*,#51349,.F.);
#71999=ORIENTED_EDGE('',*,*,#51346,.F.);
#72000=ORIENTED_EDGE('',*,*,#51354,.F.);
#72001=ORIENTED_EDGE('',*,*,#51364,.F.);
#72002=ORIENTED_EDGE('',*,*,#51361,.F.);
#72003=ORIENTED_EDGE('',*,*,#51358,.F.);
#72004=ORIENTED_EDGE('',*,*,#51366,.F.);
#72005=ORIENTED_EDGE('',*,*,#51376,.F.);
#72006=ORIENTED_EDGE('',*,*,#51373,.F.);
#72007=ORIENTED_EDGE('',*,*,#51370,.F.);
#72008=ORIENTED_EDGE('',*,*,#51378,.F.);
#72009=ORIENTED_EDGE('',*,*,#51388,.F.);
#72010=ORIENTED_EDGE('',*,*,#51385,.F.);
#72011=ORIENTED_EDGE('',*,*,#51382,.F.);
#72012=ORIENTED_EDGE('',*,*,#51390,.F.);
#72013=ORIENTED_EDGE('',*,*,#51400,.F.);
#72014=ORIENTED_EDGE('',*,*,#51397,.F.);
#72015=ORIENTED_EDGE('',*,*,#51394,.F.);
#72016=ORIENTED_EDGE('',*,*,#51402,.F.);
#72017=ORIENTED_EDGE('',*,*,#51412,.F.);
#72018=ORIENTED_EDGE('',*,*,#51409,.F.);
#72019=ORIENTED_EDGE('',*,*,#51406,.F.);
#72020=ORIENTED_EDGE('',*,*,#51414,.F.);
#72021=ORIENTED_EDGE('',*,*,#51424,.F.);
#72022=ORIENTED_EDGE('',*,*,#51421,.F.);
#72023=ORIENTED_EDGE('',*,*,#51418,.F.);
#72024=ORIENTED_EDGE('',*,*,#51426,.F.);
#72025=ORIENTED_EDGE('',*,*,#51436,.F.);
#72026=ORIENTED_EDGE('',*,*,#51433,.F.);
#72027=ORIENTED_EDGE('',*,*,#51430,.F.);
#72028=ORIENTED_EDGE('',*,*,#51438,.F.);
#72029=ORIENTED_EDGE('',*,*,#51448,.F.);
#72030=ORIENTED_EDGE('',*,*,#51445,.F.);
#72031=ORIENTED_EDGE('',*,*,#51442,.F.);
#72032=ORIENTED_EDGE('',*,*,#51450,.F.);
#72033=ORIENTED_EDGE('',*,*,#51460,.F.);
#72034=ORIENTED_EDGE('',*,*,#51457,.F.);
#72035=ORIENTED_EDGE('',*,*,#51454,.F.);
#72036=ORIENTED_EDGE('',*,*,#51462,.F.);
#72037=ORIENTED_EDGE('',*,*,#51472,.F.);
#72038=ORIENTED_EDGE('',*,*,#51469,.F.);
#72039=ORIENTED_EDGE('',*,*,#51466,.F.);
#72040=ORIENTED_EDGE('',*,*,#51474,.F.);
#72041=ORIENTED_EDGE('',*,*,#51484,.F.);
#72042=ORIENTED_EDGE('',*,*,#51481,.F.);
#72043=ORIENTED_EDGE('',*,*,#51478,.F.);
#72044=ORIENTED_EDGE('',*,*,#51486,.F.);
#72045=ORIENTED_EDGE('',*,*,#51496,.F.);
#72046=ORIENTED_EDGE('',*,*,#51493,.F.);
#72047=ORIENTED_EDGE('',*,*,#51490,.F.);
#72048=ORIENTED_EDGE('',*,*,#51498,.F.);
#72049=ORIENTED_EDGE('',*,*,#51508,.F.);
#72050=ORIENTED_EDGE('',*,*,#51505,.F.);
#72051=ORIENTED_EDGE('',*,*,#51502,.F.);
#72052=ORIENTED_EDGE('',*,*,#51510,.F.);
#72053=ORIENTED_EDGE('',*,*,#51520,.F.);
#72054=ORIENTED_EDGE('',*,*,#51517,.F.);
#72055=ORIENTED_EDGE('',*,*,#51514,.F.);
#72056=ORIENTED_EDGE('',*,*,#51522,.F.);
#72057=ORIENTED_EDGE('',*,*,#51532,.F.);
#72058=ORIENTED_EDGE('',*,*,#51529,.F.);
#72059=ORIENTED_EDGE('',*,*,#51526,.F.);
#72060=ORIENTED_EDGE('',*,*,#51534,.F.);
#72061=ORIENTED_EDGE('',*,*,#51544,.F.);
#72062=ORIENTED_EDGE('',*,*,#51541,.F.);
#72063=ORIENTED_EDGE('',*,*,#51538,.F.);
#72064=ORIENTED_EDGE('',*,*,#51546,.F.);
#72065=ORIENTED_EDGE('',*,*,#51556,.F.);
#72066=ORIENTED_EDGE('',*,*,#51553,.F.);
#72067=ORIENTED_EDGE('',*,*,#51550,.F.);
#72068=ORIENTED_EDGE('',*,*,#51558,.F.);
#72069=ORIENTED_EDGE('',*,*,#51568,.F.);
#72070=ORIENTED_EDGE('',*,*,#51565,.F.);
#72071=ORIENTED_EDGE('',*,*,#51562,.F.);
#72072=ORIENTED_EDGE('',*,*,#51570,.F.);
#72073=ORIENTED_EDGE('',*,*,#51580,.F.);
#72074=ORIENTED_EDGE('',*,*,#51577,.F.);
#72075=ORIENTED_EDGE('',*,*,#51574,.F.);
#72076=ORIENTED_EDGE('',*,*,#51582,.F.);
#72077=ORIENTED_EDGE('',*,*,#51592,.F.);
#72078=ORIENTED_EDGE('',*,*,#51589,.F.);
#72079=ORIENTED_EDGE('',*,*,#51586,.F.);
#72080=ORIENTED_EDGE('',*,*,#51594,.F.);
#72081=ORIENTED_EDGE('',*,*,#51604,.F.);
#72082=ORIENTED_EDGE('',*,*,#51601,.F.);
#72083=ORIENTED_EDGE('',*,*,#51598,.F.);
#72084=ORIENTED_EDGE('',*,*,#51606,.F.);
#72085=ORIENTED_EDGE('',*,*,#51616,.F.);
#72086=ORIENTED_EDGE('',*,*,#51613,.F.);
#72087=ORIENTED_EDGE('',*,*,#51610,.F.);
#72088=ORIENTED_EDGE('',*,*,#51618,.F.);
#72089=ORIENTED_EDGE('',*,*,#51628,.F.);
#72090=ORIENTED_EDGE('',*,*,#51625,.F.);
#72091=ORIENTED_EDGE('',*,*,#51622,.F.);
#72092=ORIENTED_EDGE('',*,*,#51630,.F.);
#72093=ORIENTED_EDGE('',*,*,#51640,.F.);
#72094=ORIENTED_EDGE('',*,*,#51637,.F.);
#72095=ORIENTED_EDGE('',*,*,#51634,.F.);
#72096=ORIENTED_EDGE('',*,*,#51642,.F.);
#72097=ORIENTED_EDGE('',*,*,#51652,.F.);
#72098=ORIENTED_EDGE('',*,*,#51649,.F.);
#72099=ORIENTED_EDGE('',*,*,#51646,.F.);
#72100=ORIENTED_EDGE('',*,*,#51654,.F.);
#72101=ORIENTED_EDGE('',*,*,#51664,.F.);
#72102=ORIENTED_EDGE('',*,*,#51661,.F.);
#72103=ORIENTED_EDGE('',*,*,#51658,.F.);
#72104=ORIENTED_EDGE('',*,*,#51666,.F.);
#72105=ORIENTED_EDGE('',*,*,#51676,.F.);
#72106=ORIENTED_EDGE('',*,*,#51673,.F.);
#72107=ORIENTED_EDGE('',*,*,#51670,.F.);
#72108=ORIENTED_EDGE('',*,*,#51678,.F.);
#72109=ORIENTED_EDGE('',*,*,#51688,.F.);
#72110=ORIENTED_EDGE('',*,*,#51685,.F.);
#72111=ORIENTED_EDGE('',*,*,#51682,.F.);
#72112=ORIENTED_EDGE('',*,*,#51690,.F.);
#72113=ORIENTED_EDGE('',*,*,#51700,.F.);
#72114=ORIENTED_EDGE('',*,*,#51697,.F.);
#72115=ORIENTED_EDGE('',*,*,#51694,.F.);
#72116=ORIENTED_EDGE('',*,*,#51702,.F.);
#72117=ORIENTED_EDGE('',*,*,#51712,.F.);
#72118=ORIENTED_EDGE('',*,*,#51709,.F.);
#72119=ORIENTED_EDGE('',*,*,#51706,.F.);
#72120=ORIENTED_EDGE('',*,*,#51714,.F.);
#72121=ORIENTED_EDGE('',*,*,#51724,.F.);
#72122=ORIENTED_EDGE('',*,*,#51721,.F.);
#72123=ORIENTED_EDGE('',*,*,#51718,.F.);
#72124=ORIENTED_EDGE('',*,*,#51726,.F.);
#72125=ORIENTED_EDGE('',*,*,#51736,.F.);
#72126=ORIENTED_EDGE('',*,*,#51733,.F.);
#72127=ORIENTED_EDGE('',*,*,#51730,.F.);
#72128=ORIENTED_EDGE('',*,*,#51738,.F.);
#72129=ORIENTED_EDGE('',*,*,#51748,.F.);
#72130=ORIENTED_EDGE('',*,*,#51745,.F.);
#72131=ORIENTED_EDGE('',*,*,#51742,.F.);
#72132=ORIENTED_EDGE('',*,*,#51750,.F.);
#72133=ORIENTED_EDGE('',*,*,#51760,.F.);
#72134=ORIENTED_EDGE('',*,*,#51757,.F.);
#72135=ORIENTED_EDGE('',*,*,#51754,.F.);
#72136=ORIENTED_EDGE('',*,*,#51762,.F.);
#72137=ORIENTED_EDGE('',*,*,#51772,.F.);
#72138=ORIENTED_EDGE('',*,*,#51769,.F.);
#72139=ORIENTED_EDGE('',*,*,#51766,.F.);
#72140=ORIENTED_EDGE('',*,*,#51774,.F.);
#72141=ORIENTED_EDGE('',*,*,#51784,.F.);
#72142=ORIENTED_EDGE('',*,*,#51781,.F.);
#72143=ORIENTED_EDGE('',*,*,#51778,.F.);
#72144=ORIENTED_EDGE('',*,*,#51786,.F.);
#72145=ORIENTED_EDGE('',*,*,#51796,.F.);
#72146=ORIENTED_EDGE('',*,*,#51793,.F.);
#72147=ORIENTED_EDGE('',*,*,#51790,.F.);
#72148=ORIENTED_EDGE('',*,*,#51798,.F.);
#72149=ORIENTED_EDGE('',*,*,#51808,.F.);
#72150=ORIENTED_EDGE('',*,*,#51805,.F.);
#72151=ORIENTED_EDGE('',*,*,#51802,.F.);
#72152=ORIENTED_EDGE('',*,*,#51810,.F.);
#72153=ORIENTED_EDGE('',*,*,#51820,.F.);
#72154=ORIENTED_EDGE('',*,*,#51817,.F.);
#72155=ORIENTED_EDGE('',*,*,#51814,.F.);
#72156=ORIENTED_EDGE('',*,*,#51822,.F.);
#72157=ORIENTED_EDGE('',*,*,#51832,.F.);
#72158=ORIENTED_EDGE('',*,*,#51829,.F.);
#72159=ORIENTED_EDGE('',*,*,#51826,.F.);
#72160=ORIENTED_EDGE('',*,*,#51834,.F.);
#72161=ORIENTED_EDGE('',*,*,#51844,.F.);
#72162=ORIENTED_EDGE('',*,*,#51841,.F.);
#72163=ORIENTED_EDGE('',*,*,#51838,.F.);
#72164=ORIENTED_EDGE('',*,*,#51846,.F.);
#72165=ORIENTED_EDGE('',*,*,#51856,.F.);
#72166=ORIENTED_EDGE('',*,*,#51853,.F.);
#72167=ORIENTED_EDGE('',*,*,#51850,.F.);
#72168=ORIENTED_EDGE('',*,*,#51858,.F.);
#72169=ORIENTED_EDGE('',*,*,#51868,.F.);
#72170=ORIENTED_EDGE('',*,*,#51865,.F.);
#72171=ORIENTED_EDGE('',*,*,#51862,.F.);
#72172=ORIENTED_EDGE('',*,*,#51870,.F.);
#72173=ORIENTED_EDGE('',*,*,#51880,.F.);
#72174=ORIENTED_EDGE('',*,*,#51877,.F.);
#72175=ORIENTED_EDGE('',*,*,#51874,.F.);
#72176=ORIENTED_EDGE('',*,*,#51882,.F.);
#72177=ORIENTED_EDGE('',*,*,#51892,.F.);
#72178=ORIENTED_EDGE('',*,*,#51889,.F.);
#72179=ORIENTED_EDGE('',*,*,#51886,.F.);
#72180=ORIENTED_EDGE('',*,*,#51894,.F.);
#72181=ORIENTED_EDGE('',*,*,#51904,.F.);
#72182=ORIENTED_EDGE('',*,*,#51901,.F.);
#72183=ORIENTED_EDGE('',*,*,#51898,.F.);
#72184=ORIENTED_EDGE('',*,*,#51906,.F.);
#72185=ORIENTED_EDGE('',*,*,#51916,.F.);
#72186=ORIENTED_EDGE('',*,*,#51913,.F.);
#72187=ORIENTED_EDGE('',*,*,#51910,.F.);
#72188=ORIENTED_EDGE('',*,*,#51918,.F.);
#72189=ORIENTED_EDGE('',*,*,#51928,.F.);
#72190=ORIENTED_EDGE('',*,*,#51925,.F.);
#72191=ORIENTED_EDGE('',*,*,#51922,.F.);
#72192=ORIENTED_EDGE('',*,*,#51930,.F.);
#72193=ORIENTED_EDGE('',*,*,#51940,.F.);
#72194=ORIENTED_EDGE('',*,*,#51937,.F.);
#72195=ORIENTED_EDGE('',*,*,#51934,.F.);
#72196=ORIENTED_EDGE('',*,*,#51942,.F.);
#72197=ORIENTED_EDGE('',*,*,#51952,.F.);
#72198=ORIENTED_EDGE('',*,*,#51949,.F.);
#72199=ORIENTED_EDGE('',*,*,#51946,.F.);
#72200=ORIENTED_EDGE('',*,*,#51954,.F.);
#72201=ORIENTED_EDGE('',*,*,#51964,.F.);
#72202=ORIENTED_EDGE('',*,*,#51961,.F.);
#72203=ORIENTED_EDGE('',*,*,#51958,.F.);
#72204=ORIENTED_EDGE('',*,*,#51966,.F.);
#72205=ORIENTED_EDGE('',*,*,#51977,.F.);
#72206=ORIENTED_EDGE('',*,*,#51975,.F.);
#72207=ORIENTED_EDGE('',*,*,#51973,.F.);
#72208=ORIENTED_EDGE('',*,*,#51978,.F.);
#72209=ORIENTED_EDGE('',*,*,#43491,.F.);
#72210=ORIENTED_EDGE('',*,*,#43495,.T.);
#72211=ORIENTED_EDGE('',*,*,#43486,.F.);
#72212=ORIENTED_EDGE('',*,*,#43470,.F.);
#72213=ORIENTED_EDGE('',*,*,#43456,.T.);
#72214=ORIENTED_EDGE('',*,*,#51979,.T.);
#72215=ORIENTED_EDGE('',*,*,#43462,.T.);
#72216=ORIENTED_EDGE('',*,*,#43468,.F.);
#72217=ORIENTED_EDGE('',*,*,#43482,.F.);
#72218=ORIENTED_EDGE('',*,*,#51980,.T.);
#72219=ORIENTED_EDGE('',*,*,#43458,.F.);
#72220=ORIENTED_EDGE('',*,*,#43472,.T.);
#72221=ORIENTED_EDGE('',*,*,#43485,.T.);
#72222=ORIENTED_EDGE('',*,*,#51981,.F.);
#72223=ORIENTED_EDGE('',*,*,#43483,.T.);
#72224=ORIENTED_EDGE('',*,*,#43469,.T.);
#72225=ORIENTED_EDGE('',*,*,#43460,.F.);
#72226=ORIENTED_EDGE('',*,*,#51982,.F.);
#72227=ORIENTED_EDGE('',*,*,#43487,.F.);
#72228=ORIENTED_EDGE('',*,*,#51979,.F.);
#72229=ORIENTED_EDGE('',*,*,#43459,.F.);
#72230=ORIENTED_EDGE('',*,*,#51981,.T.);
#72231=ORIENTED_EDGE('',*,*,#43463,.F.);
#72232=ORIENTED_EDGE('',*,*,#51980,.F.);
#72233=ORIENTED_EDGE('',*,*,#43484,.F.);
#72234=ORIENTED_EDGE('',*,*,#51982,.T.);
#72235=ORIENTED_EDGE('',*,*,#43489,.T.);
#72236=ORIENTED_EDGE('',*,*,#43447,.T.);
#72237=ORIENTED_EDGE('',*,*,#43466,.F.);
#72238=ORIENTED_EDGE('',*,*,#51983,.F.);
#72239=ORIENTED_EDGE('',*,*,#51984,.F.);
#72240=ORIENTED_EDGE('',*,*,#43449,.F.);
#72241=ORIENTED_EDGE('',*,*,#43455,.F.);
#72242=ORIENTED_EDGE('',*,*,#43443,.T.);
#72243=ORIENTED_EDGE('',*,*,#43480,.T.);
#72244=ORIENTED_EDGE('',*,*,#43477,.T.);
#72245=ORIENTED_EDGE('',*,*,#43464,.T.);
#72246=ORIENTED_EDGE('',*,*,#43445,.F.);
#72247=ORIENTED_EDGE('',*,*,#43488,.F.);
#72248=ORIENTED_EDGE('',*,*,#51985,.T.);
#72249=ORIENTED_EDGE('',*,*,#43441,.F.);
#72250=ORIENTED_EDGE('',*,*,#43454,.T.);
#72251=ORIENTED_EDGE('',*,*,#43451,.T.);
#72252=ORIENTED_EDGE('',*,*,#51986,.T.);
#72253=ORIENTED_EDGE('',*,*,#43475,.F.);
#72254=ORIENTED_EDGE('',*,*,#43481,.F.);
#72255=ORIENTED_EDGE('',*,*,#43465,.F.);
#72256=ORIENTED_EDGE('',*,*,#51985,.F.);
#72257=ORIENTED_EDGE('',*,*,#43490,.F.);
#72258=ORIENTED_EDGE('',*,*,#51983,.T.);
#72259=ORIENTED_EDGE('',*,*,#51986,.F.);
#72260=ORIENTED_EDGE('',*,*,#43450,.F.);
#72261=ORIENTED_EDGE('',*,*,#51984,.T.);
#72262=ORIENTED_EDGE('',*,*,#43476,.F.);
#72263=ORIENTED_EDGE('',*,*,#43434,.F.);
#72264=ORIENTED_EDGE('',*,*,#51987,.T.);
#72265=ORIENTED_EDGE('',*,*,#51987,.F.);
#72266=ORIENTED_EDGE('',*,*,#51988,.F.);
#72267=ORIENTED_EDGE('',*,*,#51989,.F.);
#72268=ORIENTED_EDGE('',*,*,#51990,.F.);
#72269=ORIENTED_EDGE('',*,*,#51991,.F.);
#72270=ORIENTED_EDGE('',*,*,#45129,.F.);
#72271=ORIENTED_EDGE('',*,*,#45133,.F.);
#72272=ORIENTED_EDGE('',*,*,#45136,.F.);
#72273=ORIENTED_EDGE('',*,*,#45138,.F.);
#72274=ORIENTED_EDGE('',*,*,#45117,.F.);
#72275=ORIENTED_EDGE('',*,*,#45121,.F.);
#72276=ORIENTED_EDGE('',*,*,#45124,.F.);
#72277=ORIENTED_EDGE('',*,*,#45126,.F.);
#72278=ORIENTED_EDGE('',*,*,#45105,.F.);
#72279=ORIENTED_EDGE('',*,*,#45109,.F.);
#72280=ORIENTED_EDGE('',*,*,#45112,.F.);
#72281=ORIENTED_EDGE('',*,*,#45114,.F.);
#72282=ORIENTED_EDGE('',*,*,#45093,.F.);
#72283=ORIENTED_EDGE('',*,*,#45097,.F.);
#72284=ORIENTED_EDGE('',*,*,#45100,.F.);
#72285=ORIENTED_EDGE('',*,*,#45102,.F.);
#72286=ORIENTED_EDGE('',*,*,#45081,.F.);
#72287=ORIENTED_EDGE('',*,*,#45085,.F.);
#72288=ORIENTED_EDGE('',*,*,#45088,.F.);
#72289=ORIENTED_EDGE('',*,*,#45090,.F.);
#72290=ORIENTED_EDGE('',*,*,#45069,.F.);
#72291=ORIENTED_EDGE('',*,*,#45073,.F.);
#72292=ORIENTED_EDGE('',*,*,#45076,.F.);
#72293=ORIENTED_EDGE('',*,*,#45078,.F.);
#72294=ORIENTED_EDGE('',*,*,#45057,.F.);
#72295=ORIENTED_EDGE('',*,*,#45061,.F.);
#72296=ORIENTED_EDGE('',*,*,#45064,.F.);
#72297=ORIENTED_EDGE('',*,*,#45066,.F.);
#72298=ORIENTED_EDGE('',*,*,#45045,.F.);
#72299=ORIENTED_EDGE('',*,*,#45049,.F.);
#72300=ORIENTED_EDGE('',*,*,#45052,.F.);
#72301=ORIENTED_EDGE('',*,*,#45054,.F.);
#72302=ORIENTED_EDGE('',*,*,#45033,.F.);
#72303=ORIENTED_EDGE('',*,*,#45037,.F.);
#72304=ORIENTED_EDGE('',*,*,#45040,.F.);
#72305=ORIENTED_EDGE('',*,*,#45042,.F.);
#72306=ORIENTED_EDGE('',*,*,#45021,.F.);
#72307=ORIENTED_EDGE('',*,*,#45025,.F.);
#72308=ORIENTED_EDGE('',*,*,#45028,.F.);
#72309=ORIENTED_EDGE('',*,*,#45030,.F.);
#72310=ORIENTED_EDGE('',*,*,#45009,.F.);
#72311=ORIENTED_EDGE('',*,*,#45013,.F.);
#72312=ORIENTED_EDGE('',*,*,#45016,.F.);
#72313=ORIENTED_EDGE('',*,*,#45018,.F.);
#72314=ORIENTED_EDGE('',*,*,#44997,.F.);
#72315=ORIENTED_EDGE('',*,*,#45001,.F.);
#72316=ORIENTED_EDGE('',*,*,#45004,.F.);
#72317=ORIENTED_EDGE('',*,*,#45006,.F.);
#72318=ORIENTED_EDGE('',*,*,#44985,.F.);
#72319=ORIENTED_EDGE('',*,*,#44989,.F.);
#72320=ORIENTED_EDGE('',*,*,#44992,.F.);
#72321=ORIENTED_EDGE('',*,*,#44994,.F.);
#72322=ORIENTED_EDGE('',*,*,#44973,.F.);
#72323=ORIENTED_EDGE('',*,*,#44977,.F.);
#72324=ORIENTED_EDGE('',*,*,#44980,.F.);
#72325=ORIENTED_EDGE('',*,*,#44982,.F.);
#72326=ORIENTED_EDGE('',*,*,#44961,.F.);
#72327=ORIENTED_EDGE('',*,*,#44965,.F.);
#72328=ORIENTED_EDGE('',*,*,#44968,.F.);
#72329=ORIENTED_EDGE('',*,*,#44970,.F.);
#72330=ORIENTED_EDGE('',*,*,#44949,.F.);
#72331=ORIENTED_EDGE('',*,*,#44953,.F.);
#72332=ORIENTED_EDGE('',*,*,#44956,.F.);
#72333=ORIENTED_EDGE('',*,*,#44958,.F.);
#72334=ORIENTED_EDGE('',*,*,#44937,.F.);
#72335=ORIENTED_EDGE('',*,*,#44941,.F.);
#72336=ORIENTED_EDGE('',*,*,#44944,.F.);
#72337=ORIENTED_EDGE('',*,*,#44946,.F.);
#72338=ORIENTED_EDGE('',*,*,#44925,.F.);
#72339=ORIENTED_EDGE('',*,*,#44929,.F.);
#72340=ORIENTED_EDGE('',*,*,#44932,.F.);
#72341=ORIENTED_EDGE('',*,*,#44934,.F.);
#72342=ORIENTED_EDGE('',*,*,#44913,.F.);
#72343=ORIENTED_EDGE('',*,*,#44917,.F.);
#72344=ORIENTED_EDGE('',*,*,#44920,.F.);
#72345=ORIENTED_EDGE('',*,*,#44922,.F.);
#72346=ORIENTED_EDGE('',*,*,#44901,.F.);
#72347=ORIENTED_EDGE('',*,*,#44905,.F.);
#72348=ORIENTED_EDGE('',*,*,#44908,.F.);
#72349=ORIENTED_EDGE('',*,*,#44910,.F.);
#72350=ORIENTED_EDGE('',*,*,#44889,.F.);
#72351=ORIENTED_EDGE('',*,*,#44893,.F.);
#72352=ORIENTED_EDGE('',*,*,#44896,.F.);
#72353=ORIENTED_EDGE('',*,*,#44898,.F.);
#72354=ORIENTED_EDGE('',*,*,#44877,.F.);
#72355=ORIENTED_EDGE('',*,*,#44881,.F.);
#72356=ORIENTED_EDGE('',*,*,#44884,.F.);
#72357=ORIENTED_EDGE('',*,*,#44886,.F.);
#72358=ORIENTED_EDGE('',*,*,#44865,.F.);
#72359=ORIENTED_EDGE('',*,*,#44869,.F.);
#72360=ORIENTED_EDGE('',*,*,#44872,.F.);
#72361=ORIENTED_EDGE('',*,*,#44874,.F.);
#72362=ORIENTED_EDGE('',*,*,#44853,.F.);
#72363=ORIENTED_EDGE('',*,*,#44857,.F.);
#72364=ORIENTED_EDGE('',*,*,#44860,.F.);
#72365=ORIENTED_EDGE('',*,*,#44862,.F.);
#72366=ORIENTED_EDGE('',*,*,#44841,.F.);
#72367=ORIENTED_EDGE('',*,*,#44845,.F.);
#72368=ORIENTED_EDGE('',*,*,#44848,.F.);
#72369=ORIENTED_EDGE('',*,*,#44850,.F.);
#72370=ORIENTED_EDGE('',*,*,#44829,.F.);
#72371=ORIENTED_EDGE('',*,*,#44833,.F.);
#72372=ORIENTED_EDGE('',*,*,#44836,.F.);
#72373=ORIENTED_EDGE('',*,*,#44838,.F.);
#72374=ORIENTED_EDGE('',*,*,#44817,.F.);
#72375=ORIENTED_EDGE('',*,*,#44821,.F.);
#72376=ORIENTED_EDGE('',*,*,#44824,.F.);
#72377=ORIENTED_EDGE('',*,*,#44826,.F.);
#72378=ORIENTED_EDGE('',*,*,#44805,.F.);
#72379=ORIENTED_EDGE('',*,*,#44809,.F.);
#72380=ORIENTED_EDGE('',*,*,#44812,.F.);
#72381=ORIENTED_EDGE('',*,*,#44814,.F.);
#72382=ORIENTED_EDGE('',*,*,#44793,.F.);
#72383=ORIENTED_EDGE('',*,*,#44797,.F.);
#72384=ORIENTED_EDGE('',*,*,#44800,.F.);
#72385=ORIENTED_EDGE('',*,*,#44802,.F.);
#72386=ORIENTED_EDGE('',*,*,#44781,.F.);
#72387=ORIENTED_EDGE('',*,*,#44785,.F.);
#72388=ORIENTED_EDGE('',*,*,#44788,.F.);
#72389=ORIENTED_EDGE('',*,*,#44790,.F.);
#72390=ORIENTED_EDGE('',*,*,#44769,.F.);
#72391=ORIENTED_EDGE('',*,*,#44773,.F.);
#72392=ORIENTED_EDGE('',*,*,#44776,.F.);
#72393=ORIENTED_EDGE('',*,*,#44778,.F.);
#72394=ORIENTED_EDGE('',*,*,#44757,.F.);
#72395=ORIENTED_EDGE('',*,*,#44761,.F.);
#72396=ORIENTED_EDGE('',*,*,#44764,.F.);
#72397=ORIENTED_EDGE('',*,*,#44766,.F.);
#72398=ORIENTED_EDGE('',*,*,#44745,.F.);
#72399=ORIENTED_EDGE('',*,*,#44749,.F.);
#72400=ORIENTED_EDGE('',*,*,#44752,.F.);
#72401=ORIENTED_EDGE('',*,*,#44754,.F.);
#72402=ORIENTED_EDGE('',*,*,#44733,.F.);
#72403=ORIENTED_EDGE('',*,*,#44737,.F.);
#72404=ORIENTED_EDGE('',*,*,#44740,.F.);
#72405=ORIENTED_EDGE('',*,*,#44742,.F.);
#72406=ORIENTED_EDGE('',*,*,#44721,.F.);
#72407=ORIENTED_EDGE('',*,*,#44725,.F.);
#72408=ORIENTED_EDGE('',*,*,#44728,.F.);
#72409=ORIENTED_EDGE('',*,*,#44730,.F.);
#72410=ORIENTED_EDGE('',*,*,#44709,.F.);
#72411=ORIENTED_EDGE('',*,*,#44713,.F.);
#72412=ORIENTED_EDGE('',*,*,#44716,.F.);
#72413=ORIENTED_EDGE('',*,*,#44718,.F.);
#72414=ORIENTED_EDGE('',*,*,#44697,.F.);
#72415=ORIENTED_EDGE('',*,*,#44701,.F.);
#72416=ORIENTED_EDGE('',*,*,#44704,.F.);
#72417=ORIENTED_EDGE('',*,*,#44706,.F.);
#72418=ORIENTED_EDGE('',*,*,#44685,.F.);
#72419=ORIENTED_EDGE('',*,*,#44689,.F.);
#72420=ORIENTED_EDGE('',*,*,#44692,.F.);
#72421=ORIENTED_EDGE('',*,*,#44694,.F.);
#72422=ORIENTED_EDGE('',*,*,#44673,.F.);
#72423=ORIENTED_EDGE('',*,*,#44677,.F.);
#72424=ORIENTED_EDGE('',*,*,#44680,.F.);
#72425=ORIENTED_EDGE('',*,*,#44682,.F.);
#72426=ORIENTED_EDGE('',*,*,#44661,.F.);
#72427=ORIENTED_EDGE('',*,*,#44665,.F.);
#72428=ORIENTED_EDGE('',*,*,#44668,.F.);
#72429=ORIENTED_EDGE('',*,*,#44670,.F.);
#72430=ORIENTED_EDGE('',*,*,#44649,.F.);
#72431=ORIENTED_EDGE('',*,*,#44653,.F.);
#72432=ORIENTED_EDGE('',*,*,#44656,.F.);
#72433=ORIENTED_EDGE('',*,*,#44658,.F.);
#72434=ORIENTED_EDGE('',*,*,#44637,.F.);
#72435=ORIENTED_EDGE('',*,*,#44641,.F.);
#72436=ORIENTED_EDGE('',*,*,#44644,.F.);
#72437=ORIENTED_EDGE('',*,*,#44646,.F.);
#72438=ORIENTED_EDGE('',*,*,#44625,.F.);
#72439=ORIENTED_EDGE('',*,*,#44629,.F.);
#72440=ORIENTED_EDGE('',*,*,#44632,.F.);
#72441=ORIENTED_EDGE('',*,*,#44634,.F.);
#72442=ORIENTED_EDGE('',*,*,#44613,.F.);
#72443=ORIENTED_EDGE('',*,*,#44617,.F.);
#72444=ORIENTED_EDGE('',*,*,#44620,.F.);
#72445=ORIENTED_EDGE('',*,*,#44622,.F.);
#72446=ORIENTED_EDGE('',*,*,#44601,.F.);
#72447=ORIENTED_EDGE('',*,*,#44605,.F.);
#72448=ORIENTED_EDGE('',*,*,#44608,.F.);
#72449=ORIENTED_EDGE('',*,*,#44610,.F.);
#72450=ORIENTED_EDGE('',*,*,#44589,.F.);
#72451=ORIENTED_EDGE('',*,*,#44593,.F.);
#72452=ORIENTED_EDGE('',*,*,#44596,.F.);
#72453=ORIENTED_EDGE('',*,*,#44598,.F.);
#72454=ORIENTED_EDGE('',*,*,#44577,.F.);
#72455=ORIENTED_EDGE('',*,*,#44581,.F.);
#72456=ORIENTED_EDGE('',*,*,#44584,.F.);
#72457=ORIENTED_EDGE('',*,*,#44586,.F.);
#72458=ORIENTED_EDGE('',*,*,#44565,.F.);
#72459=ORIENTED_EDGE('',*,*,#44569,.F.);
#72460=ORIENTED_EDGE('',*,*,#44572,.F.);
#72461=ORIENTED_EDGE('',*,*,#44574,.F.);
#72462=ORIENTED_EDGE('',*,*,#44553,.F.);
#72463=ORIENTED_EDGE('',*,*,#44557,.F.);
#72464=ORIENTED_EDGE('',*,*,#44560,.F.);
#72465=ORIENTED_EDGE('',*,*,#44562,.F.);
#72466=ORIENTED_EDGE('',*,*,#44541,.F.);
#72467=ORIENTED_EDGE('',*,*,#44545,.F.);
#72468=ORIENTED_EDGE('',*,*,#44548,.F.);
#72469=ORIENTED_EDGE('',*,*,#44550,.F.);
#72470=ORIENTED_EDGE('',*,*,#44529,.F.);
#72471=ORIENTED_EDGE('',*,*,#44533,.F.);
#72472=ORIENTED_EDGE('',*,*,#44536,.F.);
#72473=ORIENTED_EDGE('',*,*,#44538,.F.);
#72474=ORIENTED_EDGE('',*,*,#44517,.F.);
#72475=ORIENTED_EDGE('',*,*,#44521,.F.);
#72476=ORIENTED_EDGE('',*,*,#44524,.F.);
#72477=ORIENTED_EDGE('',*,*,#44526,.F.);
#72478=ORIENTED_EDGE('',*,*,#44505,.F.);
#72479=ORIENTED_EDGE('',*,*,#44509,.F.);
#72480=ORIENTED_EDGE('',*,*,#44512,.F.);
#72481=ORIENTED_EDGE('',*,*,#44514,.F.);
#72482=ORIENTED_EDGE('',*,*,#44493,.F.);
#72483=ORIENTED_EDGE('',*,*,#44497,.F.);
#72484=ORIENTED_EDGE('',*,*,#44500,.F.);
#72485=ORIENTED_EDGE('',*,*,#44502,.F.);
#72486=ORIENTED_EDGE('',*,*,#44481,.F.);
#72487=ORIENTED_EDGE('',*,*,#44485,.F.);
#72488=ORIENTED_EDGE('',*,*,#44488,.F.);
#72489=ORIENTED_EDGE('',*,*,#44490,.F.);
#72490=ORIENTED_EDGE('',*,*,#44469,.F.);
#72491=ORIENTED_EDGE('',*,*,#44473,.F.);
#72492=ORIENTED_EDGE('',*,*,#44476,.F.);
#72493=ORIENTED_EDGE('',*,*,#44478,.F.);
#72494=ORIENTED_EDGE('',*,*,#44457,.F.);
#72495=ORIENTED_EDGE('',*,*,#44461,.F.);
#72496=ORIENTED_EDGE('',*,*,#44464,.F.);
#72497=ORIENTED_EDGE('',*,*,#44466,.F.);
#72498=ORIENTED_EDGE('',*,*,#44445,.F.);
#72499=ORIENTED_EDGE('',*,*,#44449,.F.);
#72500=ORIENTED_EDGE('',*,*,#44452,.F.);
#72501=ORIENTED_EDGE('',*,*,#44454,.F.);
#72502=ORIENTED_EDGE('',*,*,#44433,.F.);
#72503=ORIENTED_EDGE('',*,*,#44437,.F.);
#72504=ORIENTED_EDGE('',*,*,#44440,.F.);
#72505=ORIENTED_EDGE('',*,*,#44442,.F.);
#72506=ORIENTED_EDGE('',*,*,#44421,.F.);
#72507=ORIENTED_EDGE('',*,*,#44425,.F.);
#72508=ORIENTED_EDGE('',*,*,#44428,.F.);
#72509=ORIENTED_EDGE('',*,*,#44430,.F.);
#72510=ORIENTED_EDGE('',*,*,#44409,.F.);
#72511=ORIENTED_EDGE('',*,*,#44413,.F.);
#72512=ORIENTED_EDGE('',*,*,#44416,.F.);
#72513=ORIENTED_EDGE('',*,*,#44418,.F.);
#72514=ORIENTED_EDGE('',*,*,#44397,.F.);
#72515=ORIENTED_EDGE('',*,*,#44401,.F.);
#72516=ORIENTED_EDGE('',*,*,#44404,.F.);
#72517=ORIENTED_EDGE('',*,*,#44406,.F.);
#72518=ORIENTED_EDGE('',*,*,#44385,.F.);
#72519=ORIENTED_EDGE('',*,*,#44389,.F.);
#72520=ORIENTED_EDGE('',*,*,#44392,.F.);
#72521=ORIENTED_EDGE('',*,*,#44394,.F.);
#72522=ORIENTED_EDGE('',*,*,#44373,.F.);
#72523=ORIENTED_EDGE('',*,*,#44377,.F.);
#72524=ORIENTED_EDGE('',*,*,#44380,.F.);
#72525=ORIENTED_EDGE('',*,*,#44382,.F.);
#72526=ORIENTED_EDGE('',*,*,#44361,.F.);
#72527=ORIENTED_EDGE('',*,*,#44365,.F.);
#72528=ORIENTED_EDGE('',*,*,#44368,.F.);
#72529=ORIENTED_EDGE('',*,*,#44370,.F.);
#72530=ORIENTED_EDGE('',*,*,#44349,.F.);
#72531=ORIENTED_EDGE('',*,*,#44353,.F.);
#72532=ORIENTED_EDGE('',*,*,#44356,.F.);
#72533=ORIENTED_EDGE('',*,*,#44358,.F.);
#72534=ORIENTED_EDGE('',*,*,#44337,.F.);
#72535=ORIENTED_EDGE('',*,*,#44341,.F.);
#72536=ORIENTED_EDGE('',*,*,#44344,.F.);
#72537=ORIENTED_EDGE('',*,*,#44346,.F.);
#72538=ORIENTED_EDGE('',*,*,#44325,.F.);
#72539=ORIENTED_EDGE('',*,*,#44329,.F.);
#72540=ORIENTED_EDGE('',*,*,#44332,.F.);
#72541=ORIENTED_EDGE('',*,*,#44334,.F.);
#72542=ORIENTED_EDGE('',*,*,#44313,.F.);
#72543=ORIENTED_EDGE('',*,*,#44317,.F.);
#72544=ORIENTED_EDGE('',*,*,#44320,.F.);
#72545=ORIENTED_EDGE('',*,*,#44322,.F.);
#72546=ORIENTED_EDGE('',*,*,#44301,.F.);
#72547=ORIENTED_EDGE('',*,*,#44305,.F.);
#72548=ORIENTED_EDGE('',*,*,#44308,.F.);
#72549=ORIENTED_EDGE('',*,*,#44310,.F.);
#72550=ORIENTED_EDGE('',*,*,#44296,.F.);
#72551=ORIENTED_EDGE('',*,*,#44286,.F.);
#72552=ORIENTED_EDGE('',*,*,#44290,.F.);
#72553=ORIENTED_EDGE('',*,*,#44294,.F.);
#72554=ORIENTED_EDGE('',*,*,#44299,.F.);
#72555=ORIENTED_EDGE('',*,*,#44281,.F.);
#72556=ORIENTED_EDGE('',*,*,#44271,.F.);
#72557=ORIENTED_EDGE('',*,*,#44275,.F.);
#72558=ORIENTED_EDGE('',*,*,#44279,.F.);
#72559=ORIENTED_EDGE('',*,*,#44284,.F.);
#72560=ORIENTED_EDGE('',*,*,#44259,.F.);
#72561=ORIENTED_EDGE('',*,*,#44263,.F.);
#72562=ORIENTED_EDGE('',*,*,#44266,.F.);
#72563=ORIENTED_EDGE('',*,*,#44268,.F.);
#72564=ORIENTED_EDGE('',*,*,#44247,.F.);
#72565=ORIENTED_EDGE('',*,*,#44251,.F.);
#72566=ORIENTED_EDGE('',*,*,#44254,.F.);
#72567=ORIENTED_EDGE('',*,*,#44256,.F.);
#72568=ORIENTED_EDGE('',*,*,#44235,.F.);
#72569=ORIENTED_EDGE('',*,*,#44239,.F.);
#72570=ORIENTED_EDGE('',*,*,#44242,.F.);
#72571=ORIENTED_EDGE('',*,*,#44244,.F.);
#72572=ORIENTED_EDGE('',*,*,#44223,.F.);
#72573=ORIENTED_EDGE('',*,*,#44227,.F.);
#72574=ORIENTED_EDGE('',*,*,#44230,.F.);
#72575=ORIENTED_EDGE('',*,*,#44232,.F.);
#72576=ORIENTED_EDGE('',*,*,#44211,.F.);
#72577=ORIENTED_EDGE('',*,*,#44215,.F.);
#72578=ORIENTED_EDGE('',*,*,#44218,.F.);
#72579=ORIENTED_EDGE('',*,*,#44220,.F.);
#72580=ORIENTED_EDGE('',*,*,#44199,.F.);
#72581=ORIENTED_EDGE('',*,*,#44203,.F.);
#72582=ORIENTED_EDGE('',*,*,#44206,.F.);
#72583=ORIENTED_EDGE('',*,*,#44208,.F.);
#72584=ORIENTED_EDGE('',*,*,#44187,.F.);
#72585=ORIENTED_EDGE('',*,*,#44191,.F.);
#72586=ORIENTED_EDGE('',*,*,#44194,.F.);
#72587=ORIENTED_EDGE('',*,*,#44196,.F.);
#72588=ORIENTED_EDGE('',*,*,#44175,.F.);
#72589=ORIENTED_EDGE('',*,*,#44179,.F.);
#72590=ORIENTED_EDGE('',*,*,#44182,.F.);
#72591=ORIENTED_EDGE('',*,*,#44184,.F.);
#72592=ORIENTED_EDGE('',*,*,#44163,.F.);
#72593=ORIENTED_EDGE('',*,*,#44167,.F.);
#72594=ORIENTED_EDGE('',*,*,#44170,.F.);
#72595=ORIENTED_EDGE('',*,*,#44172,.F.);
#72596=ORIENTED_EDGE('',*,*,#44151,.F.);
#72597=ORIENTED_EDGE('',*,*,#44155,.F.);
#72598=ORIENTED_EDGE('',*,*,#44158,.F.);
#72599=ORIENTED_EDGE('',*,*,#44160,.F.);
#72600=ORIENTED_EDGE('',*,*,#44139,.F.);
#72601=ORIENTED_EDGE('',*,*,#44143,.F.);
#72602=ORIENTED_EDGE('',*,*,#44146,.F.);
#72603=ORIENTED_EDGE('',*,*,#44137,.F.);
#72604=ORIENTED_EDGE('',*,*,#44148,.F.);
#72605=ORIENTED_EDGE('',*,*,#44124,.F.);
#72606=ORIENTED_EDGE('',*,*,#44128,.F.);
#72607=ORIENTED_EDGE('',*,*,#44131,.F.);
#72608=ORIENTED_EDGE('',*,*,#44133,.F.);
#72609=ORIENTED_EDGE('',*,*,#44112,.F.);
#72610=ORIENTED_EDGE('',*,*,#44116,.F.);
#72611=ORIENTED_EDGE('',*,*,#44119,.F.);
#72612=ORIENTED_EDGE('',*,*,#44121,.F.);
#72613=ORIENTED_EDGE('',*,*,#44100,.F.);
#72614=ORIENTED_EDGE('',*,*,#44104,.F.);
#72615=ORIENTED_EDGE('',*,*,#44107,.F.);
#72616=ORIENTED_EDGE('',*,*,#44109,.F.);
#72617=ORIENTED_EDGE('',*,*,#44088,.F.);
#72618=ORIENTED_EDGE('',*,*,#44092,.F.);
#72619=ORIENTED_EDGE('',*,*,#44095,.F.);
#72620=ORIENTED_EDGE('',*,*,#44097,.F.);
#72621=ORIENTED_EDGE('',*,*,#44076,.F.);
#72622=ORIENTED_EDGE('',*,*,#44080,.F.);
#72623=ORIENTED_EDGE('',*,*,#44083,.F.);
#72624=ORIENTED_EDGE('',*,*,#44085,.F.);
#72625=ORIENTED_EDGE('',*,*,#44064,.F.);
#72626=ORIENTED_EDGE('',*,*,#44068,.F.);
#72627=ORIENTED_EDGE('',*,*,#44071,.F.);
#72628=ORIENTED_EDGE('',*,*,#44073,.F.);
#72629=ORIENTED_EDGE('',*,*,#44052,.F.);
#72630=ORIENTED_EDGE('',*,*,#44056,.F.);
#72631=ORIENTED_EDGE('',*,*,#44059,.F.);
#72632=ORIENTED_EDGE('',*,*,#44061,.F.);
#72633=ORIENTED_EDGE('',*,*,#44040,.F.);
#72634=ORIENTED_EDGE('',*,*,#44044,.F.);
#72635=ORIENTED_EDGE('',*,*,#44047,.F.);
#72636=ORIENTED_EDGE('',*,*,#44049,.F.);
#72637=ORIENTED_EDGE('',*,*,#44028,.F.);
#72638=ORIENTED_EDGE('',*,*,#44032,.F.);
#72639=ORIENTED_EDGE('',*,*,#44035,.F.);
#72640=ORIENTED_EDGE('',*,*,#44037,.F.);
#72641=ORIENTED_EDGE('',*,*,#44016,.F.);
#72642=ORIENTED_EDGE('',*,*,#44020,.F.);
#72643=ORIENTED_EDGE('',*,*,#44023,.F.);
#72644=ORIENTED_EDGE('',*,*,#44025,.F.);
#72645=ORIENTED_EDGE('',*,*,#44011,.F.);
#72646=ORIENTED_EDGE('',*,*,#44001,.F.);
#72647=ORIENTED_EDGE('',*,*,#44006,.F.);
#72648=ORIENTED_EDGE('',*,*,#44014,.F.);
#72649=ORIENTED_EDGE('',*,*,#43996,.F.);
#72650=ORIENTED_EDGE('',*,*,#43986,.F.);
#72651=ORIENTED_EDGE('',*,*,#43991,.F.);
#72652=ORIENTED_EDGE('',*,*,#43999,.F.);
#72653=ORIENTED_EDGE('',*,*,#43974,.F.);
#72654=ORIENTED_EDGE('',*,*,#43978,.F.);
#72655=ORIENTED_EDGE('',*,*,#43981,.F.);
#72656=ORIENTED_EDGE('',*,*,#43983,.F.);
#72657=ORIENTED_EDGE('',*,*,#43962,.F.);
#72658=ORIENTED_EDGE('',*,*,#43966,.F.);
#72659=ORIENTED_EDGE('',*,*,#43969,.F.);
#72660=ORIENTED_EDGE('',*,*,#43971,.F.);
#72661=ORIENTED_EDGE('',*,*,#43950,.F.);
#72662=ORIENTED_EDGE('',*,*,#43954,.F.);
#72663=ORIENTED_EDGE('',*,*,#43957,.F.);
#72664=ORIENTED_EDGE('',*,*,#43959,.F.);
#72665=ORIENTED_EDGE('',*,*,#43938,.F.);
#72666=ORIENTED_EDGE('',*,*,#43942,.F.);
#72667=ORIENTED_EDGE('',*,*,#43945,.F.);
#72668=ORIENTED_EDGE('',*,*,#43947,.F.);
#72669=ORIENTED_EDGE('',*,*,#43926,.F.);
#72670=ORIENTED_EDGE('',*,*,#43930,.F.);
#72671=ORIENTED_EDGE('',*,*,#43933,.F.);
#72672=ORIENTED_EDGE('',*,*,#43935,.F.);
#72673=ORIENTED_EDGE('',*,*,#43914,.F.);
#72674=ORIENTED_EDGE('',*,*,#43918,.F.);
#72675=ORIENTED_EDGE('',*,*,#43921,.F.);
#72676=ORIENTED_EDGE('',*,*,#43923,.F.);
#72677=ORIENTED_EDGE('',*,*,#43902,.F.);
#72678=ORIENTED_EDGE('',*,*,#43906,.F.);
#72679=ORIENTED_EDGE('',*,*,#43909,.F.);
#72680=ORIENTED_EDGE('',*,*,#43911,.F.);
#72681=ORIENTED_EDGE('',*,*,#43890,.F.);
#72682=ORIENTED_EDGE('',*,*,#43894,.F.);
#72683=ORIENTED_EDGE('',*,*,#43897,.F.);
#72684=ORIENTED_EDGE('',*,*,#43899,.F.);
#72685=ORIENTED_EDGE('',*,*,#43885,.F.);
#72686=ORIENTED_EDGE('',*,*,#43875,.F.);
#72687=ORIENTED_EDGE('',*,*,#43880,.F.);
#72688=ORIENTED_EDGE('',*,*,#43888,.F.);
#72689=ORIENTED_EDGE('',*,*,#43871,.F.);
#72690=ORIENTED_EDGE('',*,*,#43861,.F.);
#72691=ORIENTED_EDGE('',*,*,#43865,.F.);
#72692=ORIENTED_EDGE('',*,*,#43867,.F.);
#72693=ORIENTED_EDGE('',*,*,#43873,.F.);
#72694=ORIENTED_EDGE('',*,*,#43848,.F.);
#72695=ORIENTED_EDGE('',*,*,#43852,.F.);
#72696=ORIENTED_EDGE('',*,*,#43855,.F.);
#72697=ORIENTED_EDGE('',*,*,#43857,.F.);
#72698=ORIENTED_EDGE('',*,*,#43836,.F.);
#72699=ORIENTED_EDGE('',*,*,#43840,.F.);
#72700=ORIENTED_EDGE('',*,*,#43843,.F.);
#72701=ORIENTED_EDGE('',*,*,#43845,.F.);
#72702=ORIENTED_EDGE('',*,*,#43824,.F.);
#72703=ORIENTED_EDGE('',*,*,#43828,.F.);
#72704=ORIENTED_EDGE('',*,*,#43831,.F.);
#72705=ORIENTED_EDGE('',*,*,#43833,.F.);
#72706=ORIENTED_EDGE('',*,*,#43812,.F.);
#72707=ORIENTED_EDGE('',*,*,#43816,.F.);
#72708=ORIENTED_EDGE('',*,*,#43819,.F.);
#72709=ORIENTED_EDGE('',*,*,#43821,.F.);
#72710=ORIENTED_EDGE('',*,*,#43800,.F.);
#72711=ORIENTED_EDGE('',*,*,#43804,.F.);
#72712=ORIENTED_EDGE('',*,*,#43807,.F.);
#72713=ORIENTED_EDGE('',*,*,#43809,.F.);
#72714=ORIENTED_EDGE('',*,*,#43788,.F.);
#72715=ORIENTED_EDGE('',*,*,#43792,.F.);
#72716=ORIENTED_EDGE('',*,*,#43795,.F.);
#72717=ORIENTED_EDGE('',*,*,#43797,.F.);
#72718=ORIENTED_EDGE('',*,*,#43783,.F.);
#72719=ORIENTED_EDGE('',*,*,#43773,.F.);
#72720=ORIENTED_EDGE('',*,*,#43778,.F.);
#72721=ORIENTED_EDGE('',*,*,#43786,.F.);
#72722=ORIENTED_EDGE('',*,*,#43768,.F.);
#72723=ORIENTED_EDGE('',*,*,#43758,.F.);
#72724=ORIENTED_EDGE('',*,*,#43763,.F.);
#72725=ORIENTED_EDGE('',*,*,#43771,.F.);
#72726=ORIENTED_EDGE('',*,*,#43753,.F.);
#72727=ORIENTED_EDGE('',*,*,#43743,.F.);
#72728=ORIENTED_EDGE('',*,*,#43748,.F.);
#72729=ORIENTED_EDGE('',*,*,#43756,.F.);
#72730=ORIENTED_EDGE('',*,*,#43738,.F.);
#72731=ORIENTED_EDGE('',*,*,#43728,.F.);
#72732=ORIENTED_EDGE('',*,*,#43733,.F.);
#72733=ORIENTED_EDGE('',*,*,#43741,.F.);
#72734=ORIENTED_EDGE('',*,*,#43716,.F.);
#72735=ORIENTED_EDGE('',*,*,#43720,.F.);
#72736=ORIENTED_EDGE('',*,*,#43723,.F.);
#72737=ORIENTED_EDGE('',*,*,#43725,.F.);
#72738=ORIENTED_EDGE('',*,*,#43711,.F.);
#72739=ORIENTED_EDGE('',*,*,#43701,.F.);
#72740=ORIENTED_EDGE('',*,*,#43705,.F.);
#72741=ORIENTED_EDGE('',*,*,#43709,.F.);
#72742=ORIENTED_EDGE('',*,*,#43714,.F.);
#72743=ORIENTED_EDGE('',*,*,#43696,.F.);
#72744=ORIENTED_EDGE('',*,*,#43686,.F.);
#72745=ORIENTED_EDGE('',*,*,#43691,.F.);
#72746=ORIENTED_EDGE('',*,*,#43699,.F.);
#72747=ORIENTED_EDGE('',*,*,#43681,.F.);
#72748=ORIENTED_EDGE('',*,*,#43671,.F.);
#72749=ORIENTED_EDGE('',*,*,#43676,.F.);
#72750=ORIENTED_EDGE('',*,*,#43684,.F.);
#72751=ORIENTED_EDGE('',*,*,#43667,.F.);
#72752=ORIENTED_EDGE('',*,*,#43664,.F.);
#72753=ORIENTED_EDGE('',*,*,#43659,.F.);
#72754=ORIENTED_EDGE('',*,*,#43669,.F.);
#72755=ORIENTED_EDGE('',*,*,#43644,.F.);
#72756=ORIENTED_EDGE('',*,*,#43648,.F.);
#72757=ORIENTED_EDGE('',*,*,#43651,.F.);
#72758=ORIENTED_EDGE('',*,*,#43653,.F.);
#72759=ORIENTED_EDGE('',*,*,#43632,.F.);
#72760=ORIENTED_EDGE('',*,*,#43636,.F.);
#72761=ORIENTED_EDGE('',*,*,#43639,.F.);
#72762=ORIENTED_EDGE('',*,*,#43641,.F.);
#72763=ORIENTED_EDGE('',*,*,#43620,.F.);
#72764=ORIENTED_EDGE('',*,*,#43624,.F.);
#72765=ORIENTED_EDGE('',*,*,#43627,.F.);
#72766=ORIENTED_EDGE('',*,*,#43629,.F.);
#72767=ORIENTED_EDGE('',*,*,#43608,.F.);
#72768=ORIENTED_EDGE('',*,*,#43612,.F.);
#72769=ORIENTED_EDGE('',*,*,#43615,.F.);
#72770=ORIENTED_EDGE('',*,*,#43617,.F.);
#72771=ORIENTED_EDGE('',*,*,#43603,.F.);
#72772=ORIENTED_EDGE('',*,*,#43594,.F.);
#72773=ORIENTED_EDGE('',*,*,#43606,.F.);
#72774=ORIENTED_EDGE('',*,*,#43590,.F.);
#72775=ORIENTED_EDGE('',*,*,#43587,.F.);
#72776=ORIENTED_EDGE('',*,*,#43582,.F.);
#72777=ORIENTED_EDGE('',*,*,#43592,.F.);
#72778=ORIENTED_EDGE('',*,*,#43575,.F.);
#72779=ORIENTED_EDGE('',*,*,#43572,.F.);
#72780=ORIENTED_EDGE('',*,*,#43568,.F.);
#72781=ORIENTED_EDGE('',*,*,#43577,.F.);
#72782=ORIENTED_EDGE('',*,*,#45141,.F.);
#72783=ORIENTED_EDGE('',*,*,#45146,.F.);
#72784=ORIENTED_EDGE('',*,*,#45153,.F.);
#72785=ORIENTED_EDGE('',*,*,#45165,.F.);
#72786=ORIENTED_EDGE('',*,*,#45155,.F.);
#72787=ORIENTED_EDGE('',*,*,#45160,.F.);
#72788=ORIENTED_EDGE('',*,*,#45168,.F.);
#72789=ORIENTED_EDGE('',*,*,#45180,.F.);
#72790=ORIENTED_EDGE('',*,*,#45170,.F.);
#72791=ORIENTED_EDGE('',*,*,#45175,.F.);
#72792=ORIENTED_EDGE('',*,*,#45183,.F.);
#72793=ORIENTED_EDGE('',*,*,#45195,.F.);
#72794=ORIENTED_EDGE('',*,*,#45185,.F.);
#72795=ORIENTED_EDGE('',*,*,#45190,.F.);
#72796=ORIENTED_EDGE('',*,*,#45198,.F.);
#72797=ORIENTED_EDGE('',*,*,#45210,.F.);
#72798=ORIENTED_EDGE('',*,*,#45200,.F.);
#72799=ORIENTED_EDGE('',*,*,#45205,.F.);
#72800=ORIENTED_EDGE('',*,*,#45213,.F.);
#72801=ORIENTED_EDGE('',*,*,#45225,.F.);
#72802=ORIENTED_EDGE('',*,*,#45216,.F.);
#72803=ORIENTED_EDGE('',*,*,#45228,.F.);
#72804=ORIENTED_EDGE('',*,*,#45240,.F.);
#72805=ORIENTED_EDGE('',*,*,#45231,.F.);
#72806=ORIENTED_EDGE('',*,*,#45243,.F.);
#72807=ORIENTED_EDGE('',*,*,#45255,.F.);
#72808=ORIENTED_EDGE('',*,*,#45245,.F.);
#72809=ORIENTED_EDGE('',*,*,#45250,.F.);
#72810=ORIENTED_EDGE('',*,*,#45258,.F.);
#72811=ORIENTED_EDGE('',*,*,#45270,.F.);
#72812=ORIENTED_EDGE('',*,*,#45260,.F.);
#72813=ORIENTED_EDGE('',*,*,#45265,.F.);
#72814=ORIENTED_EDGE('',*,*,#45273,.F.);
#72815=ORIENTED_EDGE('',*,*,#45285,.F.);
#72816=ORIENTED_EDGE('',*,*,#45275,.F.);
#72817=ORIENTED_EDGE('',*,*,#45280,.F.);
#72818=ORIENTED_EDGE('',*,*,#45288,.F.);
#72819=ORIENTED_EDGE('',*,*,#45290,.F.);
#72820=ORIENTED_EDGE('',*,*,#45294,.F.);
#72821=ORIENTED_EDGE('',*,*,#45297,.F.);
#72822=ORIENTED_EDGE('',*,*,#45299,.F.);
#72823=ORIENTED_EDGE('',*,*,#45302,.F.);
#72824=ORIENTED_EDGE('',*,*,#45306,.F.);
#72825=ORIENTED_EDGE('',*,*,#45309,.F.);
#72826=ORIENTED_EDGE('',*,*,#45311,.F.);
#72827=ORIENTED_EDGE('',*,*,#45314,.F.);
#72828=ORIENTED_EDGE('',*,*,#45318,.F.);
#72829=ORIENTED_EDGE('',*,*,#45321,.F.);
#72830=ORIENTED_EDGE('',*,*,#45323,.F.);
#72831=ORIENTED_EDGE('',*,*,#45326,.F.);
#72832=ORIENTED_EDGE('',*,*,#45330,.F.);
#72833=ORIENTED_EDGE('',*,*,#45333,.F.);
#72834=ORIENTED_EDGE('',*,*,#45335,.F.);
#72835=ORIENTED_EDGE('',*,*,#45338,.F.);
#72836=ORIENTED_EDGE('',*,*,#45342,.F.);
#72837=ORIENTED_EDGE('',*,*,#45345,.F.);
#72838=ORIENTED_EDGE('',*,*,#45347,.F.);
#72839=ORIENTED_EDGE('',*,*,#45350,.F.);
#72840=ORIENTED_EDGE('',*,*,#45354,.F.);
#72841=ORIENTED_EDGE('',*,*,#45357,.F.);
#72842=ORIENTED_EDGE('',*,*,#45359,.F.);
#72843=ORIENTED_EDGE('',*,*,#45362,.F.);
#72844=ORIENTED_EDGE('',*,*,#45366,.F.);
#72845=ORIENTED_EDGE('',*,*,#45369,.F.);
#72846=ORIENTED_EDGE('',*,*,#45371,.F.);
#72847=ORIENTED_EDGE('',*,*,#45374,.F.);
#72848=ORIENTED_EDGE('',*,*,#45378,.F.);
#72849=ORIENTED_EDGE('',*,*,#45381,.F.);
#72850=ORIENTED_EDGE('',*,*,#45383,.F.);
#72851=ORIENTED_EDGE('',*,*,#45396,.F.);
#72852=ORIENTED_EDGE('',*,*,#45387,.F.);
#72853=ORIENTED_EDGE('',*,*,#45399,.F.);
#72854=ORIENTED_EDGE('',*,*,#45411,.F.);
#72855=ORIENTED_EDGE('',*,*,#45402,.F.);
#72856=ORIENTED_EDGE('',*,*,#45414,.F.);
#72857=ORIENTED_EDGE('',*,*,#45416,.F.);
#72858=ORIENTED_EDGE('',*,*,#45420,.F.);
#72859=ORIENTED_EDGE('',*,*,#45423,.F.);
#72860=ORIENTED_EDGE('',*,*,#45425,.F.);
#72861=ORIENTED_EDGE('',*,*,#45428,.F.);
#72862=ORIENTED_EDGE('',*,*,#45432,.F.);
#72863=ORIENTED_EDGE('',*,*,#45435,.F.);
#72864=ORIENTED_EDGE('',*,*,#45437,.F.);
#72865=ORIENTED_EDGE('',*,*,#45440,.F.);
#72866=ORIENTED_EDGE('',*,*,#45444,.F.);
#72867=ORIENTED_EDGE('',*,*,#45447,.F.);
#72868=ORIENTED_EDGE('',*,*,#45449,.F.);
#72869=ORIENTED_EDGE('',*,*,#45452,.F.);
#72870=ORIENTED_EDGE('',*,*,#45456,.F.);
#72871=ORIENTED_EDGE('',*,*,#45459,.F.);
#72872=ORIENTED_EDGE('',*,*,#45461,.F.);
#72873=ORIENTED_EDGE('',*,*,#45474,.F.);
#72874=ORIENTED_EDGE('',*,*,#45464,.F.);
#72875=ORIENTED_EDGE('',*,*,#45468,.F.);
#72876=ORIENTED_EDGE('',*,*,#45472,.F.);
#72877=ORIENTED_EDGE('',*,*,#45477,.F.);
#72878=ORIENTED_EDGE('',*,*,#45489,.F.);
#72879=ORIENTED_EDGE('',*,*,#45479,.F.);
#72880=ORIENTED_EDGE('',*,*,#45484,.F.);
#72881=ORIENTED_EDGE('',*,*,#45492,.F.);
#72882=ORIENTED_EDGE('',*,*,#45504,.F.);
#72883=ORIENTED_EDGE('',*,*,#45494,.F.);
#72884=ORIENTED_EDGE('',*,*,#45499,.F.);
#72885=ORIENTED_EDGE('',*,*,#45507,.F.);
#72886=ORIENTED_EDGE('',*,*,#45519,.F.);
#72887=ORIENTED_EDGE('',*,*,#45509,.F.);
#72888=ORIENTED_EDGE('',*,*,#45513,.F.);
#72889=ORIENTED_EDGE('',*,*,#45517,.F.);
#72890=ORIENTED_EDGE('',*,*,#45522,.F.);
#72891=ORIENTED_EDGE('',*,*,#45524,.F.);
#72892=ORIENTED_EDGE('',*,*,#45528,.F.);
#72893=ORIENTED_EDGE('',*,*,#45531,.F.);
#72894=ORIENTED_EDGE('',*,*,#45533,.F.);
#72895=ORIENTED_EDGE('',*,*,#45536,.F.);
#72896=ORIENTED_EDGE('',*,*,#45540,.F.);
#72897=ORIENTED_EDGE('',*,*,#45543,.F.);
#72898=ORIENTED_EDGE('',*,*,#45545,.F.);
#72899=ORIENTED_EDGE('',*,*,#45548,.F.);
#72900=ORIENTED_EDGE('',*,*,#45552,.F.);
#72901=ORIENTED_EDGE('',*,*,#45555,.F.);
#72902=ORIENTED_EDGE('',*,*,#45557,.F.);
#72903=ORIENTED_EDGE('',*,*,#45560,.F.);
#72904=ORIENTED_EDGE('',*,*,#45564,.F.);
#72905=ORIENTED_EDGE('',*,*,#45567,.F.);
#72906=ORIENTED_EDGE('',*,*,#45569,.F.);
#72907=ORIENTED_EDGE('',*,*,#45572,.F.);
#72908=ORIENTED_EDGE('',*,*,#45576,.F.);
#72909=ORIENTED_EDGE('',*,*,#45579,.F.);
#72910=ORIENTED_EDGE('',*,*,#45581,.F.);
#72911=ORIENTED_EDGE('',*,*,#45584,.F.);
#72912=ORIENTED_EDGE('',*,*,#45588,.F.);
#72913=ORIENTED_EDGE('',*,*,#45591,.F.);
#72914=ORIENTED_EDGE('',*,*,#45593,.F.);
#72915=ORIENTED_EDGE('',*,*,#45596,.F.);
#72916=ORIENTED_EDGE('',*,*,#45600,.F.);
#72917=ORIENTED_EDGE('',*,*,#45603,.F.);
#72918=ORIENTED_EDGE('',*,*,#45605,.F.);
#72919=ORIENTED_EDGE('',*,*,#45608,.F.);
#72920=ORIENTED_EDGE('',*,*,#45612,.F.);
#72921=ORIENTED_EDGE('',*,*,#45615,.F.);
#72922=ORIENTED_EDGE('',*,*,#45617,.F.);
#72923=ORIENTED_EDGE('',*,*,#45620,.F.);
#72924=ORIENTED_EDGE('',*,*,#45624,.F.);
#72925=ORIENTED_EDGE('',*,*,#45627,.F.);
#72926=ORIENTED_EDGE('',*,*,#45629,.F.);
#72927=ORIENTED_EDGE('',*,*,#45632,.F.);
#72928=ORIENTED_EDGE('',*,*,#45636,.F.);
#72929=ORIENTED_EDGE('',*,*,#45639,.F.);
#72930=ORIENTED_EDGE('',*,*,#45641,.F.);
#72931=ORIENTED_EDGE('',*,*,#45654,.F.);
#72932=ORIENTED_EDGE('',*,*,#45644,.F.);
#72933=ORIENTED_EDGE('',*,*,#45648,.F.);
#72934=ORIENTED_EDGE('',*,*,#45652,.F.);
#72935=ORIENTED_EDGE('',*,*,#45657,.F.);
#72936=ORIENTED_EDGE('',*,*,#45669,.F.);
#72937=ORIENTED_EDGE('',*,*,#45659,.F.);
#72938=ORIENTED_EDGE('',*,*,#45663,.F.);
#72939=ORIENTED_EDGE('',*,*,#45667,.F.);
#72940=ORIENTED_EDGE('',*,*,#45672,.F.);
#72941=ORIENTED_EDGE('',*,*,#45674,.F.);
#72942=ORIENTED_EDGE('',*,*,#45678,.F.);
#72943=ORIENTED_EDGE('',*,*,#45681,.F.);
#72944=ORIENTED_EDGE('',*,*,#45683,.F.);
#72945=ORIENTED_EDGE('',*,*,#45686,.F.);
#72946=ORIENTED_EDGE('',*,*,#45690,.F.);
#72947=ORIENTED_EDGE('',*,*,#45693,.F.);
#72948=ORIENTED_EDGE('',*,*,#45695,.F.);
#72949=ORIENTED_EDGE('',*,*,#45698,.F.);
#72950=ORIENTED_EDGE('',*,*,#45702,.F.);
#72951=ORIENTED_EDGE('',*,*,#45705,.F.);
#72952=ORIENTED_EDGE('',*,*,#45707,.F.);
#72953=ORIENTED_EDGE('',*,*,#45710,.F.);
#72954=ORIENTED_EDGE('',*,*,#45714,.F.);
#72955=ORIENTED_EDGE('',*,*,#45717,.F.);
#72956=ORIENTED_EDGE('',*,*,#45719,.F.);
#72957=ORIENTED_EDGE('',*,*,#45722,.F.);
#72958=ORIENTED_EDGE('',*,*,#45726,.F.);
#72959=ORIENTED_EDGE('',*,*,#45729,.F.);
#72960=ORIENTED_EDGE('',*,*,#45731,.F.);
#72961=ORIENTED_EDGE('',*,*,#45734,.F.);
#72962=ORIENTED_EDGE('',*,*,#45738,.F.);
#72963=ORIENTED_EDGE('',*,*,#45741,.F.);
#72964=ORIENTED_EDGE('',*,*,#45743,.F.);
#72965=ORIENTED_EDGE('',*,*,#45746,.F.);
#72966=ORIENTED_EDGE('',*,*,#45750,.F.);
#72967=ORIENTED_EDGE('',*,*,#45753,.F.);
#72968=ORIENTED_EDGE('',*,*,#45755,.F.);
#72969=ORIENTED_EDGE('',*,*,#45758,.F.);
#72970=ORIENTED_EDGE('',*,*,#45762,.F.);
#72971=ORIENTED_EDGE('',*,*,#45765,.F.);
#72972=ORIENTED_EDGE('',*,*,#45767,.F.);
#72973=ORIENTED_EDGE('',*,*,#45770,.F.);
#72974=ORIENTED_EDGE('',*,*,#45774,.F.);
#72975=ORIENTED_EDGE('',*,*,#45777,.F.);
#72976=ORIENTED_EDGE('',*,*,#45779,.F.);
#72977=ORIENTED_EDGE('',*,*,#45792,.F.);
#72978=ORIENTED_EDGE('',*,*,#45782,.F.);
#72979=ORIENTED_EDGE('',*,*,#45787,.F.);
#72980=ORIENTED_EDGE('',*,*,#45795,.F.);
#72981=ORIENTED_EDGE('',*,*,#45807,.F.);
#72982=ORIENTED_EDGE('',*,*,#45797,.F.);
#72983=ORIENTED_EDGE('',*,*,#45801,.F.);
#72984=ORIENTED_EDGE('',*,*,#45805,.F.);
#72985=ORIENTED_EDGE('',*,*,#45810,.F.);
#72986=ORIENTED_EDGE('',*,*,#45812,.F.);
#72987=ORIENTED_EDGE('',*,*,#45816,.F.);
#72988=ORIENTED_EDGE('',*,*,#45819,.F.);
#72989=ORIENTED_EDGE('',*,*,#45821,.F.);
#72990=ORIENTED_EDGE('',*,*,#45824,.F.);
#72991=ORIENTED_EDGE('',*,*,#45828,.F.);
#72992=ORIENTED_EDGE('',*,*,#45831,.F.);
#72993=ORIENTED_EDGE('',*,*,#45833,.F.);
#72994=ORIENTED_EDGE('',*,*,#45836,.F.);
#72995=ORIENTED_EDGE('',*,*,#45840,.F.);
#72996=ORIENTED_EDGE('',*,*,#45843,.F.);
#72997=ORIENTED_EDGE('',*,*,#45845,.F.);
#72998=ORIENTED_EDGE('',*,*,#45848,.F.);
#72999=ORIENTED_EDGE('',*,*,#45852,.F.);
#73000=ORIENTED_EDGE('',*,*,#45855,.F.);
#73001=ORIENTED_EDGE('',*,*,#45857,.F.);
#73002=ORIENTED_EDGE('',*,*,#45860,.F.);
#73003=ORIENTED_EDGE('',*,*,#45864,.F.);
#73004=ORIENTED_EDGE('',*,*,#45867,.F.);
#73005=ORIENTED_EDGE('',*,*,#45869,.F.);
#73006=ORIENTED_EDGE('',*,*,#45872,.F.);
#73007=ORIENTED_EDGE('',*,*,#45876,.F.);
#73008=ORIENTED_EDGE('',*,*,#45879,.F.);
#73009=ORIENTED_EDGE('',*,*,#45881,.F.);
#73010=ORIENTED_EDGE('',*,*,#45884,.F.);
#73011=ORIENTED_EDGE('',*,*,#45888,.F.);
#73012=ORIENTED_EDGE('',*,*,#45891,.F.);
#73013=ORIENTED_EDGE('',*,*,#45893,.F.);
#73014=ORIENTED_EDGE('',*,*,#45896,.F.);
#73015=ORIENTED_EDGE('',*,*,#45900,.F.);
#73016=ORIENTED_EDGE('',*,*,#45903,.F.);
#73017=ORIENTED_EDGE('',*,*,#45905,.F.);
#73018=ORIENTED_EDGE('',*,*,#45908,.F.);
#73019=ORIENTED_EDGE('',*,*,#45912,.F.);
#73020=ORIENTED_EDGE('',*,*,#45915,.F.);
#73021=ORIENTED_EDGE('',*,*,#45917,.F.);
#73022=ORIENTED_EDGE('',*,*,#45920,.F.);
#73023=ORIENTED_EDGE('',*,*,#45924,.F.);
#73024=ORIENTED_EDGE('',*,*,#45927,.F.);
#73025=ORIENTED_EDGE('',*,*,#45929,.F.);
#73026=ORIENTED_EDGE('',*,*,#45932,.F.);
#73027=ORIENTED_EDGE('',*,*,#45936,.F.);
#73028=ORIENTED_EDGE('',*,*,#45939,.F.);
#73029=ORIENTED_EDGE('',*,*,#45941,.F.);
#73030=ORIENTED_EDGE('',*,*,#45944,.F.);
#73031=ORIENTED_EDGE('',*,*,#45948,.F.);
#73032=ORIENTED_EDGE('',*,*,#45951,.F.);
#73033=ORIENTED_EDGE('',*,*,#45953,.F.);
#73034=ORIENTED_EDGE('',*,*,#45956,.F.);
#73035=ORIENTED_EDGE('',*,*,#45960,.F.);
#73036=ORIENTED_EDGE('',*,*,#45963,.F.);
#73037=ORIENTED_EDGE('',*,*,#45965,.F.);
#73038=ORIENTED_EDGE('',*,*,#45968,.F.);
#73039=ORIENTED_EDGE('',*,*,#45972,.F.);
#73040=ORIENTED_EDGE('',*,*,#45975,.F.);
#73041=ORIENTED_EDGE('',*,*,#45977,.F.);
#73042=ORIENTED_EDGE('',*,*,#45980,.F.);
#73043=ORIENTED_EDGE('',*,*,#45984,.F.);
#73044=ORIENTED_EDGE('',*,*,#45987,.F.);
#73045=ORIENTED_EDGE('',*,*,#45989,.F.);
#73046=ORIENTED_EDGE('',*,*,#45992,.F.);
#73047=ORIENTED_EDGE('',*,*,#45996,.F.);
#73048=ORIENTED_EDGE('',*,*,#45999,.F.);
#73049=ORIENTED_EDGE('',*,*,#46001,.F.);
#73050=ORIENTED_EDGE('',*,*,#46004,.F.);
#73051=ORIENTED_EDGE('',*,*,#46008,.F.);
#73052=ORIENTED_EDGE('',*,*,#46011,.F.);
#73053=ORIENTED_EDGE('',*,*,#46013,.F.);
#73054=ORIENTED_EDGE('',*,*,#46016,.F.);
#73055=ORIENTED_EDGE('',*,*,#46020,.F.);
#73056=ORIENTED_EDGE('',*,*,#46023,.F.);
#73057=ORIENTED_EDGE('',*,*,#46025,.F.);
#73058=ORIENTED_EDGE('',*,*,#46028,.F.);
#73059=ORIENTED_EDGE('',*,*,#46032,.F.);
#73060=ORIENTED_EDGE('',*,*,#46035,.F.);
#73061=ORIENTED_EDGE('',*,*,#46037,.F.);
#73062=ORIENTED_EDGE('',*,*,#46040,.F.);
#73063=ORIENTED_EDGE('',*,*,#46044,.F.);
#73064=ORIENTED_EDGE('',*,*,#46047,.F.);
#73065=ORIENTED_EDGE('',*,*,#46049,.F.);
#73066=ORIENTED_EDGE('',*,*,#46052,.F.);
#73067=ORIENTED_EDGE('',*,*,#46056,.F.);
#73068=ORIENTED_EDGE('',*,*,#46059,.F.);
#73069=ORIENTED_EDGE('',*,*,#46061,.F.);
#73070=ORIENTED_EDGE('',*,*,#46064,.F.);
#73071=ORIENTED_EDGE('',*,*,#46068,.F.);
#73072=ORIENTED_EDGE('',*,*,#46071,.F.);
#73073=ORIENTED_EDGE('',*,*,#46073,.F.);
#73074=ORIENTED_EDGE('',*,*,#46076,.F.);
#73075=ORIENTED_EDGE('',*,*,#46080,.F.);
#73076=ORIENTED_EDGE('',*,*,#46083,.F.);
#73077=ORIENTED_EDGE('',*,*,#46085,.F.);
#73078=ORIENTED_EDGE('',*,*,#46088,.F.);
#73079=ORIENTED_EDGE('',*,*,#46092,.F.);
#73080=ORIENTED_EDGE('',*,*,#46095,.F.);
#73081=ORIENTED_EDGE('',*,*,#46097,.F.);
#73082=ORIENTED_EDGE('',*,*,#46100,.F.);
#73083=ORIENTED_EDGE('',*,*,#46104,.F.);
#73084=ORIENTED_EDGE('',*,*,#46107,.F.);
#73085=ORIENTED_EDGE('',*,*,#46109,.F.);
#73086=ORIENTED_EDGE('',*,*,#46112,.F.);
#73087=ORIENTED_EDGE('',*,*,#46116,.F.);
#73088=ORIENTED_EDGE('',*,*,#46119,.F.);
#73089=ORIENTED_EDGE('',*,*,#46121,.F.);
#73090=ORIENTED_EDGE('',*,*,#46124,.F.);
#73091=ORIENTED_EDGE('',*,*,#46128,.F.);
#73092=ORIENTED_EDGE('',*,*,#46131,.F.);
#73093=ORIENTED_EDGE('',*,*,#46133,.F.);
#73094=ORIENTED_EDGE('',*,*,#46136,.F.);
#73095=ORIENTED_EDGE('',*,*,#46140,.F.);
#73096=ORIENTED_EDGE('',*,*,#46143,.F.);
#73097=ORIENTED_EDGE('',*,*,#46145,.F.);
#73098=ORIENTED_EDGE('',*,*,#46148,.F.);
#73099=ORIENTED_EDGE('',*,*,#46152,.F.);
#73100=ORIENTED_EDGE('',*,*,#46155,.F.);
#73101=ORIENTED_EDGE('',*,*,#46157,.F.);
#73102=ORIENTED_EDGE('',*,*,#46160,.F.);
#73103=ORIENTED_EDGE('',*,*,#46164,.F.);
#73104=ORIENTED_EDGE('',*,*,#46167,.F.);
#73105=ORIENTED_EDGE('',*,*,#46169,.F.);
#73106=ORIENTED_EDGE('',*,*,#46172,.F.);
#73107=ORIENTED_EDGE('',*,*,#46176,.F.);
#73108=ORIENTED_EDGE('',*,*,#46179,.F.);
#73109=ORIENTED_EDGE('',*,*,#46181,.F.);
#73110=ORIENTED_EDGE('',*,*,#46184,.F.);
#73111=ORIENTED_EDGE('',*,*,#46188,.F.);
#73112=ORIENTED_EDGE('',*,*,#46191,.F.);
#73113=ORIENTED_EDGE('',*,*,#46193,.F.);
#73114=ORIENTED_EDGE('',*,*,#46196,.F.);
#73115=ORIENTED_EDGE('',*,*,#46200,.F.);
#73116=ORIENTED_EDGE('',*,*,#46203,.F.);
#73117=ORIENTED_EDGE('',*,*,#46205,.F.);
#73118=ORIENTED_EDGE('',*,*,#46208,.F.);
#73119=ORIENTED_EDGE('',*,*,#46212,.F.);
#73120=ORIENTED_EDGE('',*,*,#46215,.F.);
#73121=ORIENTED_EDGE('',*,*,#46217,.F.);
#73122=ORIENTED_EDGE('',*,*,#46220,.F.);
#73123=ORIENTED_EDGE('',*,*,#46224,.F.);
#73124=ORIENTED_EDGE('',*,*,#46227,.F.);
#73125=ORIENTED_EDGE('',*,*,#46229,.F.);
#73126=ORIENTED_EDGE('',*,*,#46232,.F.);
#73127=ORIENTED_EDGE('',*,*,#46236,.F.);
#73128=ORIENTED_EDGE('',*,*,#46239,.F.);
#73129=ORIENTED_EDGE('',*,*,#46241,.F.);
#73130=ORIENTED_EDGE('',*,*,#46244,.F.);
#73131=ORIENTED_EDGE('',*,*,#46248,.F.);
#73132=ORIENTED_EDGE('',*,*,#46251,.F.);
#73133=ORIENTED_EDGE('',*,*,#46253,.F.);
#73134=ORIENTED_EDGE('',*,*,#46256,.F.);
#73135=ORIENTED_EDGE('',*,*,#46260,.F.);
#73136=ORIENTED_EDGE('',*,*,#46263,.F.);
#73137=ORIENTED_EDGE('',*,*,#46265,.F.);
#73138=ORIENTED_EDGE('',*,*,#46268,.F.);
#73139=ORIENTED_EDGE('',*,*,#46272,.F.);
#73140=ORIENTED_EDGE('',*,*,#46275,.F.);
#73141=ORIENTED_EDGE('',*,*,#46277,.F.);
#73142=ORIENTED_EDGE('',*,*,#46280,.F.);
#73143=ORIENTED_EDGE('',*,*,#46284,.F.);
#73144=ORIENTED_EDGE('',*,*,#46287,.F.);
#73145=ORIENTED_EDGE('',*,*,#46289,.F.);
#73146=ORIENTED_EDGE('',*,*,#46292,.F.);
#73147=ORIENTED_EDGE('',*,*,#46296,.F.);
#73148=ORIENTED_EDGE('',*,*,#46299,.F.);
#73149=ORIENTED_EDGE('',*,*,#46301,.F.);
#73150=ORIENTED_EDGE('',*,*,#46304,.F.);
#73151=ORIENTED_EDGE('',*,*,#46308,.F.);
#73152=ORIENTED_EDGE('',*,*,#46311,.F.);
#73153=ORIENTED_EDGE('',*,*,#46313,.F.);
#73154=ORIENTED_EDGE('',*,*,#46316,.F.);
#73155=ORIENTED_EDGE('',*,*,#46320,.F.);
#73156=ORIENTED_EDGE('',*,*,#46323,.F.);
#73157=ORIENTED_EDGE('',*,*,#46325,.F.);
#73158=ORIENTED_EDGE('',*,*,#46328,.F.);
#73159=ORIENTED_EDGE('',*,*,#46332,.F.);
#73160=ORIENTED_EDGE('',*,*,#46335,.F.);
#73161=ORIENTED_EDGE('',*,*,#46337,.F.);
#73162=ORIENTED_EDGE('',*,*,#46340,.F.);
#73163=ORIENTED_EDGE('',*,*,#46344,.F.);
#73164=ORIENTED_EDGE('',*,*,#46347,.F.);
#73165=ORIENTED_EDGE('',*,*,#46349,.F.);
#73166=ORIENTED_EDGE('',*,*,#46352,.F.);
#73167=ORIENTED_EDGE('',*,*,#46356,.F.);
#73168=ORIENTED_EDGE('',*,*,#46359,.F.);
#73169=ORIENTED_EDGE('',*,*,#46361,.F.);
#73170=ORIENTED_EDGE('',*,*,#46364,.F.);
#73171=ORIENTED_EDGE('',*,*,#46368,.F.);
#73172=ORIENTED_EDGE('',*,*,#46371,.F.);
#73173=ORIENTED_EDGE('',*,*,#46373,.F.);
#73174=ORIENTED_EDGE('',*,*,#46376,.F.);
#73175=ORIENTED_EDGE('',*,*,#46380,.F.);
#73176=ORIENTED_EDGE('',*,*,#46383,.F.);
#73177=ORIENTED_EDGE('',*,*,#46385,.F.);
#73178=ORIENTED_EDGE('',*,*,#46388,.F.);
#73179=ORIENTED_EDGE('',*,*,#46392,.F.);
#73180=ORIENTED_EDGE('',*,*,#46395,.F.);
#73181=ORIENTED_EDGE('',*,*,#46397,.F.);
#73182=ORIENTED_EDGE('',*,*,#46400,.F.);
#73183=ORIENTED_EDGE('',*,*,#46404,.F.);
#73184=ORIENTED_EDGE('',*,*,#46407,.F.);
#73185=ORIENTED_EDGE('',*,*,#46409,.F.);
#73186=ORIENTED_EDGE('',*,*,#46412,.F.);
#73187=ORIENTED_EDGE('',*,*,#46416,.F.);
#73188=ORIENTED_EDGE('',*,*,#46419,.F.);
#73189=ORIENTED_EDGE('',*,*,#46421,.F.);
#73190=ORIENTED_EDGE('',*,*,#46424,.F.);
#73191=ORIENTED_EDGE('',*,*,#46428,.F.);
#73192=ORIENTED_EDGE('',*,*,#46431,.F.);
#73193=ORIENTED_EDGE('',*,*,#46433,.F.);
#73194=ORIENTED_EDGE('',*,*,#46436,.F.);
#73195=ORIENTED_EDGE('',*,*,#46440,.F.);
#73196=ORIENTED_EDGE('',*,*,#46443,.F.);
#73197=ORIENTED_EDGE('',*,*,#46445,.F.);
#73198=ORIENTED_EDGE('',*,*,#46448,.F.);
#73199=ORIENTED_EDGE('',*,*,#46452,.F.);
#73200=ORIENTED_EDGE('',*,*,#46455,.F.);
#73201=ORIENTED_EDGE('',*,*,#46457,.F.);
#73202=ORIENTED_EDGE('',*,*,#46460,.F.);
#73203=ORIENTED_EDGE('',*,*,#46464,.F.);
#73204=ORIENTED_EDGE('',*,*,#46467,.F.);
#73205=ORIENTED_EDGE('',*,*,#46469,.F.);
#73206=ORIENTED_EDGE('',*,*,#46472,.F.);
#73207=ORIENTED_EDGE('',*,*,#46476,.F.);
#73208=ORIENTED_EDGE('',*,*,#46479,.F.);
#73209=ORIENTED_EDGE('',*,*,#46481,.F.);
#73210=ORIENTED_EDGE('',*,*,#46484,.F.);
#73211=ORIENTED_EDGE('',*,*,#46488,.F.);
#73212=ORIENTED_EDGE('',*,*,#46491,.F.);
#73213=ORIENTED_EDGE('',*,*,#46493,.F.);
#73214=ORIENTED_EDGE('',*,*,#46496,.F.);
#73215=ORIENTED_EDGE('',*,*,#46500,.F.);
#73216=ORIENTED_EDGE('',*,*,#46503,.F.);
#73217=ORIENTED_EDGE('',*,*,#46505,.F.);
#73218=ORIENTED_EDGE('',*,*,#46508,.F.);
#73219=ORIENTED_EDGE('',*,*,#46512,.F.);
#73220=ORIENTED_EDGE('',*,*,#46515,.F.);
#73221=ORIENTED_EDGE('',*,*,#46517,.F.);
#73222=ORIENTED_EDGE('',*,*,#46520,.F.);
#73223=ORIENTED_EDGE('',*,*,#46524,.F.);
#73224=ORIENTED_EDGE('',*,*,#46527,.F.);
#73225=ORIENTED_EDGE('',*,*,#46529,.F.);
#73226=ORIENTED_EDGE('',*,*,#46532,.F.);
#73227=ORIENTED_EDGE('',*,*,#46536,.F.);
#73228=ORIENTED_EDGE('',*,*,#46539,.F.);
#73229=ORIENTED_EDGE('',*,*,#46541,.F.);
#73230=ORIENTED_EDGE('',*,*,#46544,.F.);
#73231=ORIENTED_EDGE('',*,*,#46548,.F.);
#73232=ORIENTED_EDGE('',*,*,#46551,.F.);
#73233=ORIENTED_EDGE('',*,*,#46553,.F.);
#73234=ORIENTED_EDGE('',*,*,#46556,.F.);
#73235=ORIENTED_EDGE('',*,*,#46560,.F.);
#73236=ORIENTED_EDGE('',*,*,#46563,.F.);
#73237=ORIENTED_EDGE('',*,*,#46565,.F.);
#73238=ORIENTED_EDGE('',*,*,#46568,.F.);
#73239=ORIENTED_EDGE('',*,*,#46572,.F.);
#73240=ORIENTED_EDGE('',*,*,#46575,.F.);
#73241=ORIENTED_EDGE('',*,*,#46577,.F.);
#73242=ORIENTED_EDGE('',*,*,#46580,.F.);
#73243=ORIENTED_EDGE('',*,*,#46584,.F.);
#73244=ORIENTED_EDGE('',*,*,#46587,.F.);
#73245=ORIENTED_EDGE('',*,*,#46589,.F.);
#73246=ORIENTED_EDGE('',*,*,#46592,.F.);
#73247=ORIENTED_EDGE('',*,*,#46596,.F.);
#73248=ORIENTED_EDGE('',*,*,#46599,.F.);
#73249=ORIENTED_EDGE('',*,*,#46601,.F.);
#73250=ORIENTED_EDGE('',*,*,#46604,.F.);
#73251=ORIENTED_EDGE('',*,*,#46608,.F.);
#73252=ORIENTED_EDGE('',*,*,#46611,.F.);
#73253=ORIENTED_EDGE('',*,*,#46613,.F.);
#73254=ORIENTED_EDGE('',*,*,#46616,.F.);
#73255=ORIENTED_EDGE('',*,*,#46620,.F.);
#73256=ORIENTED_EDGE('',*,*,#46623,.F.);
#73257=ORIENTED_EDGE('',*,*,#46625,.F.);
#73258=ORIENTED_EDGE('',*,*,#46628,.F.);
#73259=ORIENTED_EDGE('',*,*,#46632,.F.);
#73260=ORIENTED_EDGE('',*,*,#46635,.F.);
#73261=ORIENTED_EDGE('',*,*,#46637,.F.);
#73262=ORIENTED_EDGE('',*,*,#46640,.F.);
#73263=ORIENTED_EDGE('',*,*,#46644,.F.);
#73264=ORIENTED_EDGE('',*,*,#46647,.F.);
#73265=ORIENTED_EDGE('',*,*,#46649,.F.);
#73266=ORIENTED_EDGE('',*,*,#46652,.F.);
#73267=ORIENTED_EDGE('',*,*,#46656,.F.);
#73268=ORIENTED_EDGE('',*,*,#46659,.F.);
#73269=ORIENTED_EDGE('',*,*,#46661,.F.);
#73270=ORIENTED_EDGE('',*,*,#46664,.F.);
#73271=ORIENTED_EDGE('',*,*,#46668,.F.);
#73272=ORIENTED_EDGE('',*,*,#46671,.F.);
#73273=ORIENTED_EDGE('',*,*,#46673,.F.);
#73274=ORIENTED_EDGE('',*,*,#46676,.F.);
#73275=ORIENTED_EDGE('',*,*,#46680,.F.);
#73276=ORIENTED_EDGE('',*,*,#46683,.F.);
#73277=ORIENTED_EDGE('',*,*,#46685,.F.);
#73278=ORIENTED_EDGE('',*,*,#46688,.F.);
#73279=ORIENTED_EDGE('',*,*,#46692,.F.);
#73280=ORIENTED_EDGE('',*,*,#46695,.F.);
#73281=ORIENTED_EDGE('',*,*,#46697,.F.);
#73282=ORIENTED_EDGE('',*,*,#46700,.F.);
#73283=ORIENTED_EDGE('',*,*,#46704,.F.);
#73284=ORIENTED_EDGE('',*,*,#46707,.F.);
#73285=ORIENTED_EDGE('',*,*,#46709,.F.);
#73286=ORIENTED_EDGE('',*,*,#46712,.F.);
#73287=ORIENTED_EDGE('',*,*,#46716,.F.);
#73288=ORIENTED_EDGE('',*,*,#46719,.F.);
#73289=ORIENTED_EDGE('',*,*,#46721,.F.);
#73290=ORIENTED_EDGE('',*,*,#46724,.F.);
#73291=ORIENTED_EDGE('',*,*,#46728,.F.);
#73292=ORIENTED_EDGE('',*,*,#46731,.F.);
#73293=ORIENTED_EDGE('',*,*,#46733,.F.);
#73294=ORIENTED_EDGE('',*,*,#51992,.F.);
#73295=ORIENTED_EDGE('',*,*,#51988,.T.);
#73296=ORIENTED_EDGE('',*,*,#51993,.T.);
#73297=ORIENTED_EDGE('',*,*,#51994,.F.);
#73298=ORIENTED_EDGE('',*,*,#51995,.F.);
#73299=ORIENTED_EDGE('',*,*,#51989,.T.);
#73300=ORIENTED_EDGE('',*,*,#51992,.T.);
#73301=ORIENTED_EDGE('',*,*,#51996,.F.);
#73302=ORIENTED_EDGE('',*,*,#51997,.F.);
#73303=ORIENTED_EDGE('',*,*,#51990,.T.);
#73304=ORIENTED_EDGE('',*,*,#51995,.T.);
#73305=ORIENTED_EDGE('',*,*,#51998,.F.);
#73306=ORIENTED_EDGE('',*,*,#51993,.F.);
#73307=ORIENTED_EDGE('',*,*,#51991,.T.);
#73308=ORIENTED_EDGE('',*,*,#51997,.T.);
#73309=ORIENTED_EDGE('',*,*,#51999,.F.);
#73310=ORIENTED_EDGE('',*,*,#52000,.T.);
#73311=ORIENTED_EDGE('',*,*,#46732,.T.);
#73312=ORIENTED_EDGE('',*,*,#46729,.T.);
#73313=ORIENTED_EDGE('',*,*,#46726,.T.);
#73314=ORIENTED_EDGE('',*,*,#46734,.T.);
#73315=ORIENTED_EDGE('',*,*,#46720,.T.);
#73316=ORIENTED_EDGE('',*,*,#46717,.T.);
#73317=ORIENTED_EDGE('',*,*,#46714,.T.);
#73318=ORIENTED_EDGE('',*,*,#46722,.T.);
#73319=ORIENTED_EDGE('',*,*,#46708,.T.);
#73320=ORIENTED_EDGE('',*,*,#46705,.T.);
#73321=ORIENTED_EDGE('',*,*,#46702,.T.);
#73322=ORIENTED_EDGE('',*,*,#46710,.T.);
#73323=ORIENTED_EDGE('',*,*,#46696,.T.);
#73324=ORIENTED_EDGE('',*,*,#46693,.T.);
#73325=ORIENTED_EDGE('',*,*,#46690,.T.);
#73326=ORIENTED_EDGE('',*,*,#46698,.T.);
#73327=ORIENTED_EDGE('',*,*,#46684,.T.);
#73328=ORIENTED_EDGE('',*,*,#46681,.T.);
#73329=ORIENTED_EDGE('',*,*,#46678,.T.);
#73330=ORIENTED_EDGE('',*,*,#46686,.T.);
#73331=ORIENTED_EDGE('',*,*,#46672,.T.);
#73332=ORIENTED_EDGE('',*,*,#46669,.T.);
#73333=ORIENTED_EDGE('',*,*,#46666,.T.);
#73334=ORIENTED_EDGE('',*,*,#46674,.T.);
#73335=ORIENTED_EDGE('',*,*,#46660,.T.);
#73336=ORIENTED_EDGE('',*,*,#46657,.T.);
#73337=ORIENTED_EDGE('',*,*,#46654,.T.);
#73338=ORIENTED_EDGE('',*,*,#46662,.T.);
#73339=ORIENTED_EDGE('',*,*,#46648,.T.);
#73340=ORIENTED_EDGE('',*,*,#46645,.T.);
#73341=ORIENTED_EDGE('',*,*,#46642,.T.);
#73342=ORIENTED_EDGE('',*,*,#46650,.T.);
#73343=ORIENTED_EDGE('',*,*,#46636,.T.);
#73344=ORIENTED_EDGE('',*,*,#46633,.T.);
#73345=ORIENTED_EDGE('',*,*,#46630,.T.);
#73346=ORIENTED_EDGE('',*,*,#46638,.T.);
#73347=ORIENTED_EDGE('',*,*,#46624,.T.);
#73348=ORIENTED_EDGE('',*,*,#46621,.T.);
#73349=ORIENTED_EDGE('',*,*,#46618,.T.);
#73350=ORIENTED_EDGE('',*,*,#46626,.T.);
#73351=ORIENTED_EDGE('',*,*,#46612,.T.);
#73352=ORIENTED_EDGE('',*,*,#46609,.T.);
#73353=ORIENTED_EDGE('',*,*,#46606,.T.);
#73354=ORIENTED_EDGE('',*,*,#46614,.T.);
#73355=ORIENTED_EDGE('',*,*,#46600,.T.);
#73356=ORIENTED_EDGE('',*,*,#46597,.T.);
#73357=ORIENTED_EDGE('',*,*,#46594,.T.);
#73358=ORIENTED_EDGE('',*,*,#46602,.T.);
#73359=ORIENTED_EDGE('',*,*,#46588,.T.);
#73360=ORIENTED_EDGE('',*,*,#46585,.T.);
#73361=ORIENTED_EDGE('',*,*,#46582,.T.);
#73362=ORIENTED_EDGE('',*,*,#46590,.T.);
#73363=ORIENTED_EDGE('',*,*,#46576,.T.);
#73364=ORIENTED_EDGE('',*,*,#46573,.T.);
#73365=ORIENTED_EDGE('',*,*,#46570,.T.);
#73366=ORIENTED_EDGE('',*,*,#46578,.T.);
#73367=ORIENTED_EDGE('',*,*,#46564,.T.);
#73368=ORIENTED_EDGE('',*,*,#46561,.T.);
#73369=ORIENTED_EDGE('',*,*,#46558,.T.);
#73370=ORIENTED_EDGE('',*,*,#46566,.T.);
#73371=ORIENTED_EDGE('',*,*,#46552,.T.);
#73372=ORIENTED_EDGE('',*,*,#46549,.T.);
#73373=ORIENTED_EDGE('',*,*,#46546,.T.);
#73374=ORIENTED_EDGE('',*,*,#46554,.T.);
#73375=ORIENTED_EDGE('',*,*,#46540,.T.);
#73376=ORIENTED_EDGE('',*,*,#46537,.T.);
#73377=ORIENTED_EDGE('',*,*,#46534,.T.);
#73378=ORIENTED_EDGE('',*,*,#46542,.T.);
#73379=ORIENTED_EDGE('',*,*,#46528,.T.);
#73380=ORIENTED_EDGE('',*,*,#46525,.T.);
#73381=ORIENTED_EDGE('',*,*,#46522,.T.);
#73382=ORIENTED_EDGE('',*,*,#46530,.T.);
#73383=ORIENTED_EDGE('',*,*,#46516,.T.);
#73384=ORIENTED_EDGE('',*,*,#46513,.T.);
#73385=ORIENTED_EDGE('',*,*,#46510,.T.);
#73386=ORIENTED_EDGE('',*,*,#46518,.T.);
#73387=ORIENTED_EDGE('',*,*,#46504,.T.);
#73388=ORIENTED_EDGE('',*,*,#46501,.T.);
#73389=ORIENTED_EDGE('',*,*,#46498,.T.);
#73390=ORIENTED_EDGE('',*,*,#46506,.T.);
#73391=ORIENTED_EDGE('',*,*,#46492,.T.);
#73392=ORIENTED_EDGE('',*,*,#46489,.T.);
#73393=ORIENTED_EDGE('',*,*,#46486,.T.);
#73394=ORIENTED_EDGE('',*,*,#46494,.T.);
#73395=ORIENTED_EDGE('',*,*,#46480,.T.);
#73396=ORIENTED_EDGE('',*,*,#46477,.T.);
#73397=ORIENTED_EDGE('',*,*,#46474,.T.);
#73398=ORIENTED_EDGE('',*,*,#46482,.T.);
#73399=ORIENTED_EDGE('',*,*,#46468,.T.);
#73400=ORIENTED_EDGE('',*,*,#46465,.T.);
#73401=ORIENTED_EDGE('',*,*,#46462,.T.);
#73402=ORIENTED_EDGE('',*,*,#46470,.T.);
#73403=ORIENTED_EDGE('',*,*,#46456,.T.);
#73404=ORIENTED_EDGE('',*,*,#46453,.T.);
#73405=ORIENTED_EDGE('',*,*,#46450,.T.);
#73406=ORIENTED_EDGE('',*,*,#46458,.T.);
#73407=ORIENTED_EDGE('',*,*,#46441,.T.);
#73408=ORIENTED_EDGE('',*,*,#46438,.T.);
#73409=ORIENTED_EDGE('',*,*,#46446,.T.);
#73410=ORIENTED_EDGE('',*,*,#46444,.T.);
#73411=ORIENTED_EDGE('',*,*,#46432,.T.);
#73412=ORIENTED_EDGE('',*,*,#46429,.T.);
#73413=ORIENTED_EDGE('',*,*,#46426,.T.);
#73414=ORIENTED_EDGE('',*,*,#46434,.T.);
#73415=ORIENTED_EDGE('',*,*,#46420,.T.);
#73416=ORIENTED_EDGE('',*,*,#46417,.T.);
#73417=ORIENTED_EDGE('',*,*,#46414,.T.);
#73418=ORIENTED_EDGE('',*,*,#46422,.T.);
#73419=ORIENTED_EDGE('',*,*,#46408,.T.);
#73420=ORIENTED_EDGE('',*,*,#46405,.T.);
#73421=ORIENTED_EDGE('',*,*,#46402,.T.);
#73422=ORIENTED_EDGE('',*,*,#46410,.T.);
#73423=ORIENTED_EDGE('',*,*,#46396,.T.);
#73424=ORIENTED_EDGE('',*,*,#46393,.T.);
#73425=ORIENTED_EDGE('',*,*,#46390,.T.);
#73426=ORIENTED_EDGE('',*,*,#46398,.T.);
#73427=ORIENTED_EDGE('',*,*,#46384,.T.);
#73428=ORIENTED_EDGE('',*,*,#46381,.T.);
#73429=ORIENTED_EDGE('',*,*,#46378,.T.);
#73430=ORIENTED_EDGE('',*,*,#46386,.T.);
#73431=ORIENTED_EDGE('',*,*,#46372,.T.);
#73432=ORIENTED_EDGE('',*,*,#46369,.T.);
#73433=ORIENTED_EDGE('',*,*,#46366,.T.);
#73434=ORIENTED_EDGE('',*,*,#46374,.T.);
#73435=ORIENTED_EDGE('',*,*,#46360,.T.);
#73436=ORIENTED_EDGE('',*,*,#46357,.T.);
#73437=ORIENTED_EDGE('',*,*,#46354,.T.);
#73438=ORIENTED_EDGE('',*,*,#46362,.T.);
#73439=ORIENTED_EDGE('',*,*,#46348,.T.);
#73440=ORIENTED_EDGE('',*,*,#46345,.T.);
#73441=ORIENTED_EDGE('',*,*,#46342,.T.);
#73442=ORIENTED_EDGE('',*,*,#46350,.T.);
#73443=ORIENTED_EDGE('',*,*,#46336,.T.);
#73444=ORIENTED_EDGE('',*,*,#46333,.T.);
#73445=ORIENTED_EDGE('',*,*,#46330,.T.);
#73446=ORIENTED_EDGE('',*,*,#46338,.T.);
#73447=ORIENTED_EDGE('',*,*,#46324,.T.);
#73448=ORIENTED_EDGE('',*,*,#46321,.T.);
#73449=ORIENTED_EDGE('',*,*,#46318,.T.);
#73450=ORIENTED_EDGE('',*,*,#46326,.T.);
#73451=ORIENTED_EDGE('',*,*,#46312,.T.);
#73452=ORIENTED_EDGE('',*,*,#46309,.T.);
#73453=ORIENTED_EDGE('',*,*,#46306,.T.);
#73454=ORIENTED_EDGE('',*,*,#46314,.T.);
#73455=ORIENTED_EDGE('',*,*,#46300,.T.);
#73456=ORIENTED_EDGE('',*,*,#46297,.T.);
#73457=ORIENTED_EDGE('',*,*,#46294,.T.);
#73458=ORIENTED_EDGE('',*,*,#46302,.T.);
#73459=ORIENTED_EDGE('',*,*,#46288,.T.);
#73460=ORIENTED_EDGE('',*,*,#46285,.T.);
#73461=ORIENTED_EDGE('',*,*,#46282,.T.);
#73462=ORIENTED_EDGE('',*,*,#46290,.T.);
#73463=ORIENTED_EDGE('',*,*,#46276,.T.);
#73464=ORIENTED_EDGE('',*,*,#46273,.T.);
#73465=ORIENTED_EDGE('',*,*,#46270,.T.);
#73466=ORIENTED_EDGE('',*,*,#46278,.T.);
#73467=ORIENTED_EDGE('',*,*,#46264,.T.);
#73468=ORIENTED_EDGE('',*,*,#46261,.T.);
#73469=ORIENTED_EDGE('',*,*,#46258,.T.);
#73470=ORIENTED_EDGE('',*,*,#46266,.T.);
#73471=ORIENTED_EDGE('',*,*,#46252,.T.);
#73472=ORIENTED_EDGE('',*,*,#46249,.T.);
#73473=ORIENTED_EDGE('',*,*,#46246,.T.);
#73474=ORIENTED_EDGE('',*,*,#46254,.T.);
#73475=ORIENTED_EDGE('',*,*,#46240,.T.);
#73476=ORIENTED_EDGE('',*,*,#46237,.T.);
#73477=ORIENTED_EDGE('',*,*,#46234,.T.);
#73478=ORIENTED_EDGE('',*,*,#46242,.T.);
#73479=ORIENTED_EDGE('',*,*,#46228,.T.);
#73480=ORIENTED_EDGE('',*,*,#46225,.T.);
#73481=ORIENTED_EDGE('',*,*,#46222,.T.);
#73482=ORIENTED_EDGE('',*,*,#46230,.T.);
#73483=ORIENTED_EDGE('',*,*,#46216,.T.);
#73484=ORIENTED_EDGE('',*,*,#46213,.T.);
#73485=ORIENTED_EDGE('',*,*,#46210,.T.);
#73486=ORIENTED_EDGE('',*,*,#46218,.T.);
#73487=ORIENTED_EDGE('',*,*,#46204,.T.);
#73488=ORIENTED_EDGE('',*,*,#46201,.T.);
#73489=ORIENTED_EDGE('',*,*,#46198,.T.);
#73490=ORIENTED_EDGE('',*,*,#46206,.T.);
#73491=ORIENTED_EDGE('',*,*,#46192,.T.);
#73492=ORIENTED_EDGE('',*,*,#46189,.T.);
#73493=ORIENTED_EDGE('',*,*,#46186,.T.);
#73494=ORIENTED_EDGE('',*,*,#46194,.T.);
#73495=ORIENTED_EDGE('',*,*,#46180,.T.);
#73496=ORIENTED_EDGE('',*,*,#46177,.T.);
#73497=ORIENTED_EDGE('',*,*,#46174,.T.);
#73498=ORIENTED_EDGE('',*,*,#46182,.T.);
#73499=ORIENTED_EDGE('',*,*,#46168,.T.);
#73500=ORIENTED_EDGE('',*,*,#46165,.T.);
#73501=ORIENTED_EDGE('',*,*,#46162,.T.);
#73502=ORIENTED_EDGE('',*,*,#46170,.T.);
#73503=ORIENTED_EDGE('',*,*,#46156,.T.);
#73504=ORIENTED_EDGE('',*,*,#46153,.T.);
#73505=ORIENTED_EDGE('',*,*,#46150,.T.);
#73506=ORIENTED_EDGE('',*,*,#46158,.T.);
#73507=ORIENTED_EDGE('',*,*,#46144,.T.);
#73508=ORIENTED_EDGE('',*,*,#46141,.T.);
#73509=ORIENTED_EDGE('',*,*,#46138,.T.);
#73510=ORIENTED_EDGE('',*,*,#46146,.T.);
#73511=ORIENTED_EDGE('',*,*,#46132,.T.);
#73512=ORIENTED_EDGE('',*,*,#46129,.T.);
#73513=ORIENTED_EDGE('',*,*,#46126,.T.);
#73514=ORIENTED_EDGE('',*,*,#46134,.T.);
#73515=ORIENTED_EDGE('',*,*,#46120,.T.);
#73516=ORIENTED_EDGE('',*,*,#46117,.T.);
#73517=ORIENTED_EDGE('',*,*,#46114,.T.);
#73518=ORIENTED_EDGE('',*,*,#46122,.T.);
#73519=ORIENTED_EDGE('',*,*,#46108,.T.);
#73520=ORIENTED_EDGE('',*,*,#46105,.T.);
#73521=ORIENTED_EDGE('',*,*,#46102,.T.);
#73522=ORIENTED_EDGE('',*,*,#46110,.T.);
#73523=ORIENTED_EDGE('',*,*,#46096,.T.);
#73524=ORIENTED_EDGE('',*,*,#46093,.T.);
#73525=ORIENTED_EDGE('',*,*,#46090,.T.);
#73526=ORIENTED_EDGE('',*,*,#46098,.T.);
#73527=ORIENTED_EDGE('',*,*,#46084,.T.);
#73528=ORIENTED_EDGE('',*,*,#46081,.T.);
#73529=ORIENTED_EDGE('',*,*,#46078,.T.);
#73530=ORIENTED_EDGE('',*,*,#46086,.T.);
#73531=ORIENTED_EDGE('',*,*,#46072,.T.);
#73532=ORIENTED_EDGE('',*,*,#46069,.T.);
#73533=ORIENTED_EDGE('',*,*,#46066,.T.);
#73534=ORIENTED_EDGE('',*,*,#46074,.T.);
#73535=ORIENTED_EDGE('',*,*,#46060,.T.);
#73536=ORIENTED_EDGE('',*,*,#46057,.T.);
#73537=ORIENTED_EDGE('',*,*,#46054,.T.);
#73538=ORIENTED_EDGE('',*,*,#46062,.T.);
#73539=ORIENTED_EDGE('',*,*,#46048,.T.);
#73540=ORIENTED_EDGE('',*,*,#46045,.T.);
#73541=ORIENTED_EDGE('',*,*,#46042,.T.);
#73542=ORIENTED_EDGE('',*,*,#46050,.T.);
#73543=ORIENTED_EDGE('',*,*,#46036,.T.);
#73544=ORIENTED_EDGE('',*,*,#46033,.T.);
#73545=ORIENTED_EDGE('',*,*,#46030,.T.);
#73546=ORIENTED_EDGE('',*,*,#46038,.T.);
#73547=ORIENTED_EDGE('',*,*,#46024,.T.);
#73548=ORIENTED_EDGE('',*,*,#46021,.T.);
#73549=ORIENTED_EDGE('',*,*,#46018,.T.);
#73550=ORIENTED_EDGE('',*,*,#46026,.T.);
#73551=ORIENTED_EDGE('',*,*,#46012,.T.);
#73552=ORIENTED_EDGE('',*,*,#46009,.T.);
#73553=ORIENTED_EDGE('',*,*,#46006,.T.);
#73554=ORIENTED_EDGE('',*,*,#46014,.T.);
#73555=ORIENTED_EDGE('',*,*,#46000,.T.);
#73556=ORIENTED_EDGE('',*,*,#45997,.T.);
#73557=ORIENTED_EDGE('',*,*,#45994,.T.);
#73558=ORIENTED_EDGE('',*,*,#46002,.T.);
#73559=ORIENTED_EDGE('',*,*,#45988,.T.);
#73560=ORIENTED_EDGE('',*,*,#45985,.T.);
#73561=ORIENTED_EDGE('',*,*,#45982,.T.);
#73562=ORIENTED_EDGE('',*,*,#45990,.T.);
#73563=ORIENTED_EDGE('',*,*,#45976,.T.);
#73564=ORIENTED_EDGE('',*,*,#45973,.T.);
#73565=ORIENTED_EDGE('',*,*,#45970,.T.);
#73566=ORIENTED_EDGE('',*,*,#45978,.T.);
#73567=ORIENTED_EDGE('',*,*,#45964,.T.);
#73568=ORIENTED_EDGE('',*,*,#45961,.T.);
#73569=ORIENTED_EDGE('',*,*,#45958,.T.);
#73570=ORIENTED_EDGE('',*,*,#45966,.T.);
#73571=ORIENTED_EDGE('',*,*,#45952,.T.);
#73572=ORIENTED_EDGE('',*,*,#45949,.T.);
#73573=ORIENTED_EDGE('',*,*,#45946,.T.);
#73574=ORIENTED_EDGE('',*,*,#45954,.T.);
#73575=ORIENTED_EDGE('',*,*,#45940,.T.);
#73576=ORIENTED_EDGE('',*,*,#45937,.T.);
#73577=ORIENTED_EDGE('',*,*,#45934,.T.);
#73578=ORIENTED_EDGE('',*,*,#45942,.T.);
#73579=ORIENTED_EDGE('',*,*,#45928,.T.);
#73580=ORIENTED_EDGE('',*,*,#45925,.T.);
#73581=ORIENTED_EDGE('',*,*,#45922,.T.);
#73582=ORIENTED_EDGE('',*,*,#45930,.T.);
#73583=ORIENTED_EDGE('',*,*,#45916,.T.);
#73584=ORIENTED_EDGE('',*,*,#45913,.T.);
#73585=ORIENTED_EDGE('',*,*,#45910,.T.);
#73586=ORIENTED_EDGE('',*,*,#45918,.T.);
#73587=ORIENTED_EDGE('',*,*,#45904,.T.);
#73588=ORIENTED_EDGE('',*,*,#45901,.T.);
#73589=ORIENTED_EDGE('',*,*,#45898,.T.);
#73590=ORIENTED_EDGE('',*,*,#45906,.T.);
#73591=ORIENTED_EDGE('',*,*,#45892,.T.);
#73592=ORIENTED_EDGE('',*,*,#45889,.T.);
#73593=ORIENTED_EDGE('',*,*,#45886,.T.);
#73594=ORIENTED_EDGE('',*,*,#45894,.T.);
#73595=ORIENTED_EDGE('',*,*,#45880,.T.);
#73596=ORIENTED_EDGE('',*,*,#45877,.T.);
#73597=ORIENTED_EDGE('',*,*,#45874,.T.);
#73598=ORIENTED_EDGE('',*,*,#45882,.T.);
#73599=ORIENTED_EDGE('',*,*,#45868,.T.);
#73600=ORIENTED_EDGE('',*,*,#45865,.T.);
#73601=ORIENTED_EDGE('',*,*,#45862,.T.);
#73602=ORIENTED_EDGE('',*,*,#45870,.T.);
#73603=ORIENTED_EDGE('',*,*,#45856,.T.);
#73604=ORIENTED_EDGE('',*,*,#45853,.T.);
#73605=ORIENTED_EDGE('',*,*,#45850,.T.);
#73606=ORIENTED_EDGE('',*,*,#45858,.T.);
#73607=ORIENTED_EDGE('',*,*,#45844,.T.);
#73608=ORIENTED_EDGE('',*,*,#45841,.T.);
#73609=ORIENTED_EDGE('',*,*,#45838,.T.);
#73610=ORIENTED_EDGE('',*,*,#45846,.T.);
#73611=ORIENTED_EDGE('',*,*,#45832,.T.);
#73612=ORIENTED_EDGE('',*,*,#45829,.T.);
#73613=ORIENTED_EDGE('',*,*,#45826,.T.);
#73614=ORIENTED_EDGE('',*,*,#45834,.T.);
#73615=ORIENTED_EDGE('',*,*,#45820,.T.);
#73616=ORIENTED_EDGE('',*,*,#45817,.T.);
#73617=ORIENTED_EDGE('',*,*,#45814,.T.);
#73618=ORIENTED_EDGE('',*,*,#45822,.T.);
#73619=ORIENTED_EDGE('',*,*,#45799,.T.);
#73620=ORIENTED_EDGE('',*,*,#45809,.T.);
#73621=ORIENTED_EDGE('',*,*,#45806,.T.);
#73622=ORIENTED_EDGE('',*,*,#45802,.T.);
#73623=ORIENTED_EDGE('',*,*,#45794,.T.);
#73624=ORIENTED_EDGE('',*,*,#45791,.T.);
#73625=ORIENTED_EDGE('',*,*,#45788,.T.);
#73626=ORIENTED_EDGE('',*,*,#45784,.T.);
#73627=ORIENTED_EDGE('',*,*,#45778,.T.);
#73628=ORIENTED_EDGE('',*,*,#45775,.T.);
#73629=ORIENTED_EDGE('',*,*,#45772,.T.);
#73630=ORIENTED_EDGE('',*,*,#45780,.T.);
#73631=ORIENTED_EDGE('',*,*,#45766,.T.);
#73632=ORIENTED_EDGE('',*,*,#45763,.T.);
#73633=ORIENTED_EDGE('',*,*,#45760,.T.);
#73634=ORIENTED_EDGE('',*,*,#45768,.T.);
#73635=ORIENTED_EDGE('',*,*,#45754,.T.);
#73636=ORIENTED_EDGE('',*,*,#45751,.T.);
#73637=ORIENTED_EDGE('',*,*,#45748,.T.);
#73638=ORIENTED_EDGE('',*,*,#45756,.T.);
#73639=ORIENTED_EDGE('',*,*,#45742,.T.);
#73640=ORIENTED_EDGE('',*,*,#45739,.T.);
#73641=ORIENTED_EDGE('',*,*,#45736,.T.);
#73642=ORIENTED_EDGE('',*,*,#45744,.T.);
#73643=ORIENTED_EDGE('',*,*,#45730,.T.);
#73644=ORIENTED_EDGE('',*,*,#45727,.T.);
#73645=ORIENTED_EDGE('',*,*,#45724,.T.);
#73646=ORIENTED_EDGE('',*,*,#45732,.T.);
#73647=ORIENTED_EDGE('',*,*,#45718,.T.);
#73648=ORIENTED_EDGE('',*,*,#45715,.T.);
#73649=ORIENTED_EDGE('',*,*,#45712,.T.);
#73650=ORIENTED_EDGE('',*,*,#45720,.T.);
#73651=ORIENTED_EDGE('',*,*,#45706,.T.);
#73652=ORIENTED_EDGE('',*,*,#45703,.T.);
#73653=ORIENTED_EDGE('',*,*,#45700,.T.);
#73654=ORIENTED_EDGE('',*,*,#45708,.T.);
#73655=ORIENTED_EDGE('',*,*,#45694,.T.);
#73656=ORIENTED_EDGE('',*,*,#45691,.T.);
#73657=ORIENTED_EDGE('',*,*,#45688,.T.);
#73658=ORIENTED_EDGE('',*,*,#45696,.T.);
#73659=ORIENTED_EDGE('',*,*,#45682,.T.);
#73660=ORIENTED_EDGE('',*,*,#45679,.T.);
#73661=ORIENTED_EDGE('',*,*,#45676,.T.);
#73662=ORIENTED_EDGE('',*,*,#45684,.T.);
#73663=ORIENTED_EDGE('',*,*,#45664,.T.);
#73664=ORIENTED_EDGE('',*,*,#45661,.T.);
#73665=ORIENTED_EDGE('',*,*,#45671,.T.);
#73666=ORIENTED_EDGE('',*,*,#45668,.T.);
#73667=ORIENTED_EDGE('',*,*,#45649,.T.);
#73668=ORIENTED_EDGE('',*,*,#45646,.T.);
#73669=ORIENTED_EDGE('',*,*,#45656,.T.);
#73670=ORIENTED_EDGE('',*,*,#45653,.T.);
#73671=ORIENTED_EDGE('',*,*,#45640,.T.);
#73672=ORIENTED_EDGE('',*,*,#45637,.T.);
#73673=ORIENTED_EDGE('',*,*,#45634,.T.);
#73674=ORIENTED_EDGE('',*,*,#45642,.T.);
#73675=ORIENTED_EDGE('',*,*,#45628,.T.);
#73676=ORIENTED_EDGE('',*,*,#45625,.T.);
#73677=ORIENTED_EDGE('',*,*,#45622,.T.);
#73678=ORIENTED_EDGE('',*,*,#45630,.T.);
#73679=ORIENTED_EDGE('',*,*,#45616,.T.);
#73680=ORIENTED_EDGE('',*,*,#45613,.T.);
#73681=ORIENTED_EDGE('',*,*,#45610,.T.);
#73682=ORIENTED_EDGE('',*,*,#45618,.T.);
#73683=ORIENTED_EDGE('',*,*,#45604,.T.);
#73684=ORIENTED_EDGE('',*,*,#45601,.T.);
#73685=ORIENTED_EDGE('',*,*,#45598,.T.);
#73686=ORIENTED_EDGE('',*,*,#45606,.T.);
#73687=ORIENTED_EDGE('',*,*,#45592,.T.);
#73688=ORIENTED_EDGE('',*,*,#45589,.T.);
#73689=ORIENTED_EDGE('',*,*,#45586,.T.);
#73690=ORIENTED_EDGE('',*,*,#45594,.T.);
#73691=ORIENTED_EDGE('',*,*,#45580,.T.);
#73692=ORIENTED_EDGE('',*,*,#45577,.T.);
#73693=ORIENTED_EDGE('',*,*,#45574,.T.);
#73694=ORIENTED_EDGE('',*,*,#45582,.T.);
#73695=ORIENTED_EDGE('',*,*,#45568,.T.);
#73696=ORIENTED_EDGE('',*,*,#45565,.T.);
#73697=ORIENTED_EDGE('',*,*,#45562,.T.);
#73698=ORIENTED_EDGE('',*,*,#45570,.T.);
#73699=ORIENTED_EDGE('',*,*,#45556,.T.);
#73700=ORIENTED_EDGE('',*,*,#45553,.T.);
#73701=ORIENTED_EDGE('',*,*,#45550,.T.);
#73702=ORIENTED_EDGE('',*,*,#45558,.T.);
#73703=ORIENTED_EDGE('',*,*,#45544,.T.);
#73704=ORIENTED_EDGE('',*,*,#45541,.T.);
#73705=ORIENTED_EDGE('',*,*,#45538,.T.);
#73706=ORIENTED_EDGE('',*,*,#45546,.T.);
#73707=ORIENTED_EDGE('',*,*,#45532,.T.);
#73708=ORIENTED_EDGE('',*,*,#45529,.T.);
#73709=ORIENTED_EDGE('',*,*,#45526,.T.);
#73710=ORIENTED_EDGE('',*,*,#45534,.T.);
#73711=ORIENTED_EDGE('',*,*,#45511,.T.);
#73712=ORIENTED_EDGE('',*,*,#45521,.T.);
#73713=ORIENTED_EDGE('',*,*,#45518,.T.);
#73714=ORIENTED_EDGE('',*,*,#45514,.T.);
#73715=ORIENTED_EDGE('',*,*,#45506,.T.);
#73716=ORIENTED_EDGE('',*,*,#45503,.T.);
#73717=ORIENTED_EDGE('',*,*,#45500,.T.);
#73718=ORIENTED_EDGE('',*,*,#45496,.T.);
#73719=ORIENTED_EDGE('',*,*,#45491,.T.);
#73720=ORIENTED_EDGE('',*,*,#45488,.T.);
#73721=ORIENTED_EDGE('',*,*,#45485,.T.);
#73722=ORIENTED_EDGE('',*,*,#45481,.T.);
#73723=ORIENTED_EDGE('',*,*,#45466,.T.);
#73724=ORIENTED_EDGE('',*,*,#45476,.T.);
#73725=ORIENTED_EDGE('',*,*,#45473,.T.);
#73726=ORIENTED_EDGE('',*,*,#45469,.T.);
#73727=ORIENTED_EDGE('',*,*,#45460,.T.);
#73728=ORIENTED_EDGE('',*,*,#45457,.T.);
#73729=ORIENTED_EDGE('',*,*,#45454,.T.);
#73730=ORIENTED_EDGE('',*,*,#45462,.T.);
#73731=ORIENTED_EDGE('',*,*,#45448,.T.);
#73732=ORIENTED_EDGE('',*,*,#45445,.T.);
#73733=ORIENTED_EDGE('',*,*,#45442,.T.);
#73734=ORIENTED_EDGE('',*,*,#45450,.T.);
#73735=ORIENTED_EDGE('',*,*,#45436,.T.);
#73736=ORIENTED_EDGE('',*,*,#45433,.T.);
#73737=ORIENTED_EDGE('',*,*,#45430,.T.);
#73738=ORIENTED_EDGE('',*,*,#45438,.T.);
#73739=ORIENTED_EDGE('',*,*,#45421,.T.);
#73740=ORIENTED_EDGE('',*,*,#45418,.T.);
#73741=ORIENTED_EDGE('',*,*,#45426,.T.);
#73742=ORIENTED_EDGE('',*,*,#45424,.T.);
#73743=ORIENTED_EDGE('',*,*,#45404,.T.);
#73744=ORIENTED_EDGE('',*,*,#45413,.T.);
#73745=ORIENTED_EDGE('',*,*,#45410,.T.);
#73746=ORIENTED_EDGE('',*,*,#45407,.T.);
#73747=ORIENTED_EDGE('',*,*,#45389,.T.);
#73748=ORIENTED_EDGE('',*,*,#45398,.T.);
#73749=ORIENTED_EDGE('',*,*,#45395,.T.);
#73750=ORIENTED_EDGE('',*,*,#45392,.T.);
#73751=ORIENTED_EDGE('',*,*,#45382,.T.);
#73752=ORIENTED_EDGE('',*,*,#45379,.T.);
#73753=ORIENTED_EDGE('',*,*,#45376,.T.);
#73754=ORIENTED_EDGE('',*,*,#45384,.T.);
#73755=ORIENTED_EDGE('',*,*,#45370,.T.);
#73756=ORIENTED_EDGE('',*,*,#45367,.T.);
#73757=ORIENTED_EDGE('',*,*,#45364,.T.);
#73758=ORIENTED_EDGE('',*,*,#45372,.T.);
#73759=ORIENTED_EDGE('',*,*,#45358,.T.);
#73760=ORIENTED_EDGE('',*,*,#45355,.T.);
#73761=ORIENTED_EDGE('',*,*,#45352,.T.);
#73762=ORIENTED_EDGE('',*,*,#45360,.T.);
#73763=ORIENTED_EDGE('',*,*,#45346,.T.);
#73764=ORIENTED_EDGE('',*,*,#45343,.T.);
#73765=ORIENTED_EDGE('',*,*,#45340,.T.);
#73766=ORIENTED_EDGE('',*,*,#45348,.T.);
#73767=ORIENTED_EDGE('',*,*,#45334,.T.);
#73768=ORIENTED_EDGE('',*,*,#45331,.T.);
#73769=ORIENTED_EDGE('',*,*,#45328,.T.);
#73770=ORIENTED_EDGE('',*,*,#45336,.T.);
#73771=ORIENTED_EDGE('',*,*,#45322,.T.);
#73772=ORIENTED_EDGE('',*,*,#45319,.T.);
#73773=ORIENTED_EDGE('',*,*,#45316,.T.);
#73774=ORIENTED_EDGE('',*,*,#45324,.T.);
#73775=ORIENTED_EDGE('',*,*,#45310,.T.);
#73776=ORIENTED_EDGE('',*,*,#45307,.T.);
#73777=ORIENTED_EDGE('',*,*,#45304,.T.);
#73778=ORIENTED_EDGE('',*,*,#45312,.T.);
#73779=ORIENTED_EDGE('',*,*,#45298,.T.);
#73780=ORIENTED_EDGE('',*,*,#45295,.T.);
#73781=ORIENTED_EDGE('',*,*,#45292,.T.);
#73782=ORIENTED_EDGE('',*,*,#45300,.T.);
#73783=ORIENTED_EDGE('',*,*,#45277,.T.);
#73784=ORIENTED_EDGE('',*,*,#45287,.T.);
#73785=ORIENTED_EDGE('',*,*,#45284,.T.);
#73786=ORIENTED_EDGE('',*,*,#45281,.T.);
#73787=ORIENTED_EDGE('',*,*,#45266,.T.);
#73788=ORIENTED_EDGE('',*,*,#45262,.T.);
#73789=ORIENTED_EDGE('',*,*,#45272,.T.);
#73790=ORIENTED_EDGE('',*,*,#45269,.T.);
#73791=ORIENTED_EDGE('',*,*,#45251,.T.);
#73792=ORIENTED_EDGE('',*,*,#45247,.T.);
#73793=ORIENTED_EDGE('',*,*,#45257,.T.);
#73794=ORIENTED_EDGE('',*,*,#45254,.T.);
#73795=ORIENTED_EDGE('',*,*,#45233,.T.);
#73796=ORIENTED_EDGE('',*,*,#45242,.T.);
#73797=ORIENTED_EDGE('',*,*,#45239,.T.);
#73798=ORIENTED_EDGE('',*,*,#45236,.T.);
#73799=ORIENTED_EDGE('',*,*,#45218,.T.);
#73800=ORIENTED_EDGE('',*,*,#45227,.T.);
#73801=ORIENTED_EDGE('',*,*,#45224,.T.);
#73802=ORIENTED_EDGE('',*,*,#45221,.T.);
#73803=ORIENTED_EDGE('',*,*,#45202,.T.);
#73804=ORIENTED_EDGE('',*,*,#45212,.T.);
#73805=ORIENTED_EDGE('',*,*,#45209,.T.);
#73806=ORIENTED_EDGE('',*,*,#45206,.T.);
#73807=ORIENTED_EDGE('',*,*,#45187,.T.);
#73808=ORIENTED_EDGE('',*,*,#45197,.T.);
#73809=ORIENTED_EDGE('',*,*,#45194,.T.);
#73810=ORIENTED_EDGE('',*,*,#45191,.T.);
#73811=ORIENTED_EDGE('',*,*,#45172,.T.);
#73812=ORIENTED_EDGE('',*,*,#45182,.T.);
#73813=ORIENTED_EDGE('',*,*,#45179,.T.);
#73814=ORIENTED_EDGE('',*,*,#45176,.T.);
#73815=ORIENTED_EDGE('',*,*,#45157,.T.);
#73816=ORIENTED_EDGE('',*,*,#45167,.T.);
#73817=ORIENTED_EDGE('',*,*,#45164,.T.);
#73818=ORIENTED_EDGE('',*,*,#45161,.T.);
#73819=ORIENTED_EDGE('',*,*,#45143,.T.);
#73820=ORIENTED_EDGE('',*,*,#45152,.T.);
#73821=ORIENTED_EDGE('',*,*,#45150,.T.);
#73822=ORIENTED_EDGE('',*,*,#45147,.T.);
#73823=ORIENTED_EDGE('',*,*,#43570,.T.);
#73824=ORIENTED_EDGE('',*,*,#43571,.T.);
#73825=ORIENTED_EDGE('',*,*,#43574,.T.);
#73826=ORIENTED_EDGE('',*,*,#43563,.T.);
#73827=ORIENTED_EDGE('',*,*,#43584,.T.);
#73828=ORIENTED_EDGE('',*,*,#43586,.T.);
#73829=ORIENTED_EDGE('',*,*,#43589,.T.);
#73830=ORIENTED_EDGE('',*,*,#43578,.T.);
#73831=ORIENTED_EDGE('',*,*,#43599,.T.);
#73832=ORIENTED_EDGE('',*,*,#43596,.T.);
#73833=ORIENTED_EDGE('',*,*,#43605,.T.);
#73834=ORIENTED_EDGE('',*,*,#43602,.T.);
#73835=ORIENTED_EDGE('',*,*,#43616,.T.);
#73836=ORIENTED_EDGE('',*,*,#43613,.T.);
#73837=ORIENTED_EDGE('',*,*,#43610,.T.);
#73838=ORIENTED_EDGE('',*,*,#43618,.T.);
#73839=ORIENTED_EDGE('',*,*,#43628,.T.);
#73840=ORIENTED_EDGE('',*,*,#43625,.T.);
#73841=ORIENTED_EDGE('',*,*,#43622,.T.);
#73842=ORIENTED_EDGE('',*,*,#43630,.T.);
#73843=ORIENTED_EDGE('',*,*,#43640,.T.);
#73844=ORIENTED_EDGE('',*,*,#43637,.T.);
#73845=ORIENTED_EDGE('',*,*,#43634,.T.);
#73846=ORIENTED_EDGE('',*,*,#43642,.T.);
#73847=ORIENTED_EDGE('',*,*,#43649,.T.);
#73848=ORIENTED_EDGE('',*,*,#43646,.T.);
#73849=ORIENTED_EDGE('',*,*,#43654,.T.);
#73850=ORIENTED_EDGE('',*,*,#43652,.T.);
#73851=ORIENTED_EDGE('',*,*,#43661,.T.);
#73852=ORIENTED_EDGE('',*,*,#43663,.T.);
#73853=ORIENTED_EDGE('',*,*,#43666,.T.);
#73854=ORIENTED_EDGE('',*,*,#43655,.T.);
#73855=ORIENTED_EDGE('',*,*,#43680,.T.);
#73856=ORIENTED_EDGE('',*,*,#43677,.T.);
#73857=ORIENTED_EDGE('',*,*,#43673,.T.);
#73858=ORIENTED_EDGE('',*,*,#43683,.T.);
#73859=ORIENTED_EDGE('',*,*,#43695,.T.);
#73860=ORIENTED_EDGE('',*,*,#43692,.T.);
#73861=ORIENTED_EDGE('',*,*,#43688,.T.);
#73862=ORIENTED_EDGE('',*,*,#43698,.T.);
#73863=ORIENTED_EDGE('',*,*,#43710,.T.);
#73864=ORIENTED_EDGE('',*,*,#43706,.T.);
#73865=ORIENTED_EDGE('',*,*,#43703,.T.);
#73866=ORIENTED_EDGE('',*,*,#43713,.T.);
#73867=ORIENTED_EDGE('',*,*,#43724,.T.);
#73868=ORIENTED_EDGE('',*,*,#43721,.T.);
#73869=ORIENTED_EDGE('',*,*,#43718,.T.);
#73870=ORIENTED_EDGE('',*,*,#43726,.T.);
#73871=ORIENTED_EDGE('',*,*,#43737,.T.);
#73872=ORIENTED_EDGE('',*,*,#43734,.T.);
#73873=ORIENTED_EDGE('',*,*,#43730,.T.);
#73874=ORIENTED_EDGE('',*,*,#43740,.T.);
#73875=ORIENTED_EDGE('',*,*,#43752,.T.);
#73876=ORIENTED_EDGE('',*,*,#43749,.T.);
#73877=ORIENTED_EDGE('',*,*,#43745,.T.);
#73878=ORIENTED_EDGE('',*,*,#43755,.T.);
#73879=ORIENTED_EDGE('',*,*,#43770,.T.);
#73880=ORIENTED_EDGE('',*,*,#43767,.T.);
#73881=ORIENTED_EDGE('',*,*,#43764,.T.);
#73882=ORIENTED_EDGE('',*,*,#43760,.T.);
#73883=ORIENTED_EDGE('',*,*,#43785,.T.);
#73884=ORIENTED_EDGE('',*,*,#43782,.T.);
#73885=ORIENTED_EDGE('',*,*,#43779,.T.);
#73886=ORIENTED_EDGE('',*,*,#43775,.T.);
#73887=ORIENTED_EDGE('',*,*,#43796,.T.);
#73888=ORIENTED_EDGE('',*,*,#43793,.T.);
#73889=ORIENTED_EDGE('',*,*,#43790,.T.);
#73890=ORIENTED_EDGE('',*,*,#43798,.T.);
#73891=ORIENTED_EDGE('',*,*,#43808,.T.);
#73892=ORIENTED_EDGE('',*,*,#43805,.T.);
#73893=ORIENTED_EDGE('',*,*,#43802,.T.);
#73894=ORIENTED_EDGE('',*,*,#43810,.T.);
#73895=ORIENTED_EDGE('',*,*,#43820,.T.);
#73896=ORIENTED_EDGE('',*,*,#43817,.T.);
#73897=ORIENTED_EDGE('',*,*,#43814,.T.);
#73898=ORIENTED_EDGE('',*,*,#43822,.T.);
#73899=ORIENTED_EDGE('',*,*,#43832,.T.);
#73900=ORIENTED_EDGE('',*,*,#43829,.T.);
#73901=ORIENTED_EDGE('',*,*,#43826,.T.);
#73902=ORIENTED_EDGE('',*,*,#43834,.T.);
#73903=ORIENTED_EDGE('',*,*,#43844,.T.);
#73904=ORIENTED_EDGE('',*,*,#43841,.T.);
#73905=ORIENTED_EDGE('',*,*,#43838,.T.);
#73906=ORIENTED_EDGE('',*,*,#43846,.T.);
#73907=ORIENTED_EDGE('',*,*,#43856,.T.);
#73908=ORIENTED_EDGE('',*,*,#43853,.T.);
#73909=ORIENTED_EDGE('',*,*,#43850,.T.);
#73910=ORIENTED_EDGE('',*,*,#43858,.T.);
#73911=ORIENTED_EDGE('',*,*,#43868,.T.);
#73912=ORIENTED_EDGE('',*,*,#43863,.T.);
#73913=ORIENTED_EDGE('',*,*,#43859,.T.);
#73914=ORIENTED_EDGE('',*,*,#43870,.T.);
#73915=ORIENTED_EDGE('',*,*,#43884,.T.);
#73916=ORIENTED_EDGE('',*,*,#43881,.T.);
#73917=ORIENTED_EDGE('',*,*,#43877,.T.);
#73918=ORIENTED_EDGE('',*,*,#43887,.T.);
#73919=ORIENTED_EDGE('',*,*,#43898,.T.);
#73920=ORIENTED_EDGE('',*,*,#43895,.T.);
#73921=ORIENTED_EDGE('',*,*,#43892,.T.);
#73922=ORIENTED_EDGE('',*,*,#43900,.T.);
#73923=ORIENTED_EDGE('',*,*,#43910,.T.);
#73924=ORIENTED_EDGE('',*,*,#43907,.T.);
#73925=ORIENTED_EDGE('',*,*,#43904,.T.);
#73926=ORIENTED_EDGE('',*,*,#43912,.T.);
#73927=ORIENTED_EDGE('',*,*,#43922,.T.);
#73928=ORIENTED_EDGE('',*,*,#43919,.T.);
#73929=ORIENTED_EDGE('',*,*,#43916,.T.);
#73930=ORIENTED_EDGE('',*,*,#43924,.T.);
#73931=ORIENTED_EDGE('',*,*,#43934,.T.);
#73932=ORIENTED_EDGE('',*,*,#43931,.T.);
#73933=ORIENTED_EDGE('',*,*,#43928,.T.);
#73934=ORIENTED_EDGE('',*,*,#43936,.T.);
#73935=ORIENTED_EDGE('',*,*,#43946,.T.);
#73936=ORIENTED_EDGE('',*,*,#43943,.T.);
#73937=ORIENTED_EDGE('',*,*,#43940,.T.);
#73938=ORIENTED_EDGE('',*,*,#43948,.T.);
#73939=ORIENTED_EDGE('',*,*,#43958,.T.);
#73940=ORIENTED_EDGE('',*,*,#43955,.T.);
#73941=ORIENTED_EDGE('',*,*,#43952,.T.);
#73942=ORIENTED_EDGE('',*,*,#43960,.T.);
#73943=ORIENTED_EDGE('',*,*,#43970,.T.);
#73944=ORIENTED_EDGE('',*,*,#43967,.T.);
#73945=ORIENTED_EDGE('',*,*,#43964,.T.);
#73946=ORIENTED_EDGE('',*,*,#43972,.T.);
#73947=ORIENTED_EDGE('',*,*,#43982,.T.);
#73948=ORIENTED_EDGE('',*,*,#43979,.T.);
#73949=ORIENTED_EDGE('',*,*,#43976,.T.);
#73950=ORIENTED_EDGE('',*,*,#43984,.T.);
#73951=ORIENTED_EDGE('',*,*,#43995,.T.);
#73952=ORIENTED_EDGE('',*,*,#43992,.T.);
#73953=ORIENTED_EDGE('',*,*,#43988,.T.);
#73954=ORIENTED_EDGE('',*,*,#43998,.T.);
#73955=ORIENTED_EDGE('',*,*,#44013,.T.);
#73956=ORIENTED_EDGE('',*,*,#44010,.T.);
#73957=ORIENTED_EDGE('',*,*,#44007,.T.);
#73958=ORIENTED_EDGE('',*,*,#44003,.T.);
#73959=ORIENTED_EDGE('',*,*,#44024,.T.);
#73960=ORIENTED_EDGE('',*,*,#44021,.T.);
#73961=ORIENTED_EDGE('',*,*,#44018,.T.);
#73962=ORIENTED_EDGE('',*,*,#44026,.T.);
#73963=ORIENTED_EDGE('',*,*,#44036,.T.);
#73964=ORIENTED_EDGE('',*,*,#44033,.T.);
#73965=ORIENTED_EDGE('',*,*,#44030,.T.);
#73966=ORIENTED_EDGE('',*,*,#44038,.T.);
#73967=ORIENTED_EDGE('',*,*,#44048,.T.);
#73968=ORIENTED_EDGE('',*,*,#44045,.T.);
#73969=ORIENTED_EDGE('',*,*,#44042,.T.);
#73970=ORIENTED_EDGE('',*,*,#44050,.T.);
#73971=ORIENTED_EDGE('',*,*,#44060,.T.);
#73972=ORIENTED_EDGE('',*,*,#44057,.T.);
#73973=ORIENTED_EDGE('',*,*,#44054,.T.);
#73974=ORIENTED_EDGE('',*,*,#44062,.T.);
#73975=ORIENTED_EDGE('',*,*,#44072,.T.);
#73976=ORIENTED_EDGE('',*,*,#44069,.T.);
#73977=ORIENTED_EDGE('',*,*,#44066,.T.);
#73978=ORIENTED_EDGE('',*,*,#44074,.T.);
#73979=ORIENTED_EDGE('',*,*,#44084,.T.);
#73980=ORIENTED_EDGE('',*,*,#44081,.T.);
#73981=ORIENTED_EDGE('',*,*,#44078,.T.);
#73982=ORIENTED_EDGE('',*,*,#44086,.T.);
#73983=ORIENTED_EDGE('',*,*,#44096,.T.);
#73984=ORIENTED_EDGE('',*,*,#44093,.T.);
#73985=ORIENTED_EDGE('',*,*,#44090,.T.);
#73986=ORIENTED_EDGE('',*,*,#44098,.T.);
#73987=ORIENTED_EDGE('',*,*,#44108,.T.);
#73988=ORIENTED_EDGE('',*,*,#44105,.T.);
#73989=ORIENTED_EDGE('',*,*,#44102,.T.);
#73990=ORIENTED_EDGE('',*,*,#44110,.T.);
#73991=ORIENTED_EDGE('',*,*,#44120,.T.);
#73992=ORIENTED_EDGE('',*,*,#44117,.T.);
#73993=ORIENTED_EDGE('',*,*,#44114,.T.);
#73994=ORIENTED_EDGE('',*,*,#44122,.T.);
#73995=ORIENTED_EDGE('',*,*,#44132,.T.);
#73996=ORIENTED_EDGE('',*,*,#44129,.T.);
#73997=ORIENTED_EDGE('',*,*,#44126,.T.);
#73998=ORIENTED_EDGE('',*,*,#44134,.T.);
#73999=ORIENTED_EDGE('',*,*,#44147,.T.);
#74000=ORIENTED_EDGE('',*,*,#44144,.T.);
#74001=ORIENTED_EDGE('',*,*,#44141,.T.);
#74002=ORIENTED_EDGE('',*,*,#44149,.T.);
#74003=ORIENTED_EDGE('',*,*,#44159,.T.);
#74004=ORIENTED_EDGE('',*,*,#44156,.T.);
#74005=ORIENTED_EDGE('',*,*,#44153,.T.);
#74006=ORIENTED_EDGE('',*,*,#44161,.T.);
#74007=ORIENTED_EDGE('',*,*,#44171,.T.);
#74008=ORIENTED_EDGE('',*,*,#44168,.T.);
#74009=ORIENTED_EDGE('',*,*,#44165,.T.);
#74010=ORIENTED_EDGE('',*,*,#44173,.T.);
#74011=ORIENTED_EDGE('',*,*,#44183,.T.);
#74012=ORIENTED_EDGE('',*,*,#44180,.T.);
#74013=ORIENTED_EDGE('',*,*,#44177,.T.);
#74014=ORIENTED_EDGE('',*,*,#44185,.T.);
#74015=ORIENTED_EDGE('',*,*,#44195,.T.);
#74016=ORIENTED_EDGE('',*,*,#44192,.T.);
#74017=ORIENTED_EDGE('',*,*,#44189,.T.);
#74018=ORIENTED_EDGE('',*,*,#44197,.T.);
#74019=ORIENTED_EDGE('',*,*,#44207,.T.);
#74020=ORIENTED_EDGE('',*,*,#44204,.T.);
#74021=ORIENTED_EDGE('',*,*,#44201,.T.);
#74022=ORIENTED_EDGE('',*,*,#44209,.T.);
#74023=ORIENTED_EDGE('',*,*,#44219,.T.);
#74024=ORIENTED_EDGE('',*,*,#44216,.T.);
#74025=ORIENTED_EDGE('',*,*,#44213,.T.);
#74026=ORIENTED_EDGE('',*,*,#44221,.T.);
#74027=ORIENTED_EDGE('',*,*,#44231,.T.);
#74028=ORIENTED_EDGE('',*,*,#44228,.T.);
#74029=ORIENTED_EDGE('',*,*,#44225,.T.);
#74030=ORIENTED_EDGE('',*,*,#44233,.T.);
#74031=ORIENTED_EDGE('',*,*,#44243,.T.);
#74032=ORIENTED_EDGE('',*,*,#44240,.T.);
#74033=ORIENTED_EDGE('',*,*,#44237,.T.);
#74034=ORIENTED_EDGE('',*,*,#44245,.T.);
#74035=ORIENTED_EDGE('',*,*,#44255,.T.);
#74036=ORIENTED_EDGE('',*,*,#44252,.T.);
#74037=ORIENTED_EDGE('',*,*,#44249,.T.);
#74038=ORIENTED_EDGE('',*,*,#44257,.T.);
#74039=ORIENTED_EDGE('',*,*,#44267,.T.);
#74040=ORIENTED_EDGE('',*,*,#44264,.T.);
#74041=ORIENTED_EDGE('',*,*,#44261,.T.);
#74042=ORIENTED_EDGE('',*,*,#44269,.T.);
#74043=ORIENTED_EDGE('',*,*,#44283,.T.);
#74044=ORIENTED_EDGE('',*,*,#44280,.T.);
#74045=ORIENTED_EDGE('',*,*,#44276,.T.);
#74046=ORIENTED_EDGE('',*,*,#44273,.T.);
#74047=ORIENTED_EDGE('',*,*,#44298,.T.);
#74048=ORIENTED_EDGE('',*,*,#44295,.T.);
#74049=ORIENTED_EDGE('',*,*,#44291,.T.);
#74050=ORIENTED_EDGE('',*,*,#44288,.T.);
#74051=ORIENTED_EDGE('',*,*,#44309,.T.);
#74052=ORIENTED_EDGE('',*,*,#44306,.T.);
#74053=ORIENTED_EDGE('',*,*,#44303,.T.);
#74054=ORIENTED_EDGE('',*,*,#44311,.T.);
#74055=ORIENTED_EDGE('',*,*,#44321,.T.);
#74056=ORIENTED_EDGE('',*,*,#44318,.T.);
#74057=ORIENTED_EDGE('',*,*,#44315,.T.);
#74058=ORIENTED_EDGE('',*,*,#44323,.T.);
#74059=ORIENTED_EDGE('',*,*,#44333,.T.);
#74060=ORIENTED_EDGE('',*,*,#44330,.T.);
#74061=ORIENTED_EDGE('',*,*,#44327,.T.);
#74062=ORIENTED_EDGE('',*,*,#44335,.T.);
#74063=ORIENTED_EDGE('',*,*,#44345,.T.);
#74064=ORIENTED_EDGE('',*,*,#44342,.T.);
#74065=ORIENTED_EDGE('',*,*,#44339,.T.);
#74066=ORIENTED_EDGE('',*,*,#44347,.T.);
#74067=ORIENTED_EDGE('',*,*,#44357,.T.);
#74068=ORIENTED_EDGE('',*,*,#44354,.T.);
#74069=ORIENTED_EDGE('',*,*,#44351,.T.);
#74070=ORIENTED_EDGE('',*,*,#44359,.T.);
#74071=ORIENTED_EDGE('',*,*,#44369,.T.);
#74072=ORIENTED_EDGE('',*,*,#44366,.T.);
#74073=ORIENTED_EDGE('',*,*,#44363,.T.);
#74074=ORIENTED_EDGE('',*,*,#44371,.T.);
#74075=ORIENTED_EDGE('',*,*,#44381,.T.);
#74076=ORIENTED_EDGE('',*,*,#44378,.T.);
#74077=ORIENTED_EDGE('',*,*,#44375,.T.);
#74078=ORIENTED_EDGE('',*,*,#44383,.T.);
#74079=ORIENTED_EDGE('',*,*,#44393,.T.);
#74080=ORIENTED_EDGE('',*,*,#44390,.T.);
#74081=ORIENTED_EDGE('',*,*,#44387,.T.);
#74082=ORIENTED_EDGE('',*,*,#44395,.T.);
#74083=ORIENTED_EDGE('',*,*,#44405,.T.);
#74084=ORIENTED_EDGE('',*,*,#44402,.T.);
#74085=ORIENTED_EDGE('',*,*,#44399,.T.);
#74086=ORIENTED_EDGE('',*,*,#44407,.T.);
#74087=ORIENTED_EDGE('',*,*,#44417,.T.);
#74088=ORIENTED_EDGE('',*,*,#44414,.T.);
#74089=ORIENTED_EDGE('',*,*,#44411,.T.);
#74090=ORIENTED_EDGE('',*,*,#44419,.T.);
#74091=ORIENTED_EDGE('',*,*,#44429,.T.);
#74092=ORIENTED_EDGE('',*,*,#44426,.T.);
#74093=ORIENTED_EDGE('',*,*,#44423,.T.);
#74094=ORIENTED_EDGE('',*,*,#44431,.T.);
#74095=ORIENTED_EDGE('',*,*,#44441,.T.);
#74096=ORIENTED_EDGE('',*,*,#44438,.T.);
#74097=ORIENTED_EDGE('',*,*,#44435,.T.);
#74098=ORIENTED_EDGE('',*,*,#44443,.T.);
#74099=ORIENTED_EDGE('',*,*,#44453,.T.);
#74100=ORIENTED_EDGE('',*,*,#44450,.T.);
#74101=ORIENTED_EDGE('',*,*,#44447,.T.);
#74102=ORIENTED_EDGE('',*,*,#44455,.T.);
#74103=ORIENTED_EDGE('',*,*,#44465,.T.);
#74104=ORIENTED_EDGE('',*,*,#44462,.T.);
#74105=ORIENTED_EDGE('',*,*,#44459,.T.);
#74106=ORIENTED_EDGE('',*,*,#44467,.T.);
#74107=ORIENTED_EDGE('',*,*,#44477,.T.);
#74108=ORIENTED_EDGE('',*,*,#44474,.T.);
#74109=ORIENTED_EDGE('',*,*,#44471,.T.);
#74110=ORIENTED_EDGE('',*,*,#44479,.T.);
#74111=ORIENTED_EDGE('',*,*,#44489,.T.);
#74112=ORIENTED_EDGE('',*,*,#44486,.T.);
#74113=ORIENTED_EDGE('',*,*,#44483,.T.);
#74114=ORIENTED_EDGE('',*,*,#44491,.T.);
#74115=ORIENTED_EDGE('',*,*,#44501,.T.);
#74116=ORIENTED_EDGE('',*,*,#44498,.T.);
#74117=ORIENTED_EDGE('',*,*,#44495,.T.);
#74118=ORIENTED_EDGE('',*,*,#44503,.T.);
#74119=ORIENTED_EDGE('',*,*,#44513,.T.);
#74120=ORIENTED_EDGE('',*,*,#44510,.T.);
#74121=ORIENTED_EDGE('',*,*,#44507,.T.);
#74122=ORIENTED_EDGE('',*,*,#44515,.T.);
#74123=ORIENTED_EDGE('',*,*,#44525,.T.);
#74124=ORIENTED_EDGE('',*,*,#44522,.T.);
#74125=ORIENTED_EDGE('',*,*,#44519,.T.);
#74126=ORIENTED_EDGE('',*,*,#44527,.T.);
#74127=ORIENTED_EDGE('',*,*,#44537,.T.);
#74128=ORIENTED_EDGE('',*,*,#44534,.T.);
#74129=ORIENTED_EDGE('',*,*,#44531,.T.);
#74130=ORIENTED_EDGE('',*,*,#44539,.T.);
#74131=ORIENTED_EDGE('',*,*,#44549,.T.);
#74132=ORIENTED_EDGE('',*,*,#44546,.T.);
#74133=ORIENTED_EDGE('',*,*,#44543,.T.);
#74134=ORIENTED_EDGE('',*,*,#44551,.T.);
#74135=ORIENTED_EDGE('',*,*,#44561,.T.);
#74136=ORIENTED_EDGE('',*,*,#44558,.T.);
#74137=ORIENTED_EDGE('',*,*,#44555,.T.);
#74138=ORIENTED_EDGE('',*,*,#44563,.T.);
#74139=ORIENTED_EDGE('',*,*,#44573,.T.);
#74140=ORIENTED_EDGE('',*,*,#44570,.T.);
#74141=ORIENTED_EDGE('',*,*,#44567,.T.);
#74142=ORIENTED_EDGE('',*,*,#44575,.T.);
#74143=ORIENTED_EDGE('',*,*,#44585,.T.);
#74144=ORIENTED_EDGE('',*,*,#44582,.T.);
#74145=ORIENTED_EDGE('',*,*,#44579,.T.);
#74146=ORIENTED_EDGE('',*,*,#44587,.T.);
#74147=ORIENTED_EDGE('',*,*,#44597,.T.);
#74148=ORIENTED_EDGE('',*,*,#44594,.T.);
#74149=ORIENTED_EDGE('',*,*,#44591,.T.);
#74150=ORIENTED_EDGE('',*,*,#44599,.T.);
#74151=ORIENTED_EDGE('',*,*,#44609,.T.);
#74152=ORIENTED_EDGE('',*,*,#44606,.T.);
#74153=ORIENTED_EDGE('',*,*,#44603,.T.);
#74154=ORIENTED_EDGE('',*,*,#44611,.T.);
#74155=ORIENTED_EDGE('',*,*,#44618,.T.);
#74156=ORIENTED_EDGE('',*,*,#44615,.T.);
#74157=ORIENTED_EDGE('',*,*,#44623,.T.);
#74158=ORIENTED_EDGE('',*,*,#44621,.T.);
#74159=ORIENTED_EDGE('',*,*,#44633,.T.);
#74160=ORIENTED_EDGE('',*,*,#44630,.T.);
#74161=ORIENTED_EDGE('',*,*,#44627,.T.);
#74162=ORIENTED_EDGE('',*,*,#44635,.T.);
#74163=ORIENTED_EDGE('',*,*,#44645,.T.);
#74164=ORIENTED_EDGE('',*,*,#44642,.T.);
#74165=ORIENTED_EDGE('',*,*,#44639,.T.);
#74166=ORIENTED_EDGE('',*,*,#44647,.T.);
#74167=ORIENTED_EDGE('',*,*,#44657,.T.);
#74168=ORIENTED_EDGE('',*,*,#44654,.T.);
#74169=ORIENTED_EDGE('',*,*,#44651,.T.);
#74170=ORIENTED_EDGE('',*,*,#44659,.T.);
#74171=ORIENTED_EDGE('',*,*,#44669,.T.);
#74172=ORIENTED_EDGE('',*,*,#44666,.T.);
#74173=ORIENTED_EDGE('',*,*,#44663,.T.);
#74174=ORIENTED_EDGE('',*,*,#44671,.T.);
#74175=ORIENTED_EDGE('',*,*,#44681,.T.);
#74176=ORIENTED_EDGE('',*,*,#44678,.T.);
#74177=ORIENTED_EDGE('',*,*,#44675,.T.);
#74178=ORIENTED_EDGE('',*,*,#44683,.T.);
#74179=ORIENTED_EDGE('',*,*,#44693,.T.);
#74180=ORIENTED_EDGE('',*,*,#44690,.T.);
#74181=ORIENTED_EDGE('',*,*,#44687,.T.);
#74182=ORIENTED_EDGE('',*,*,#44695,.T.);
#74183=ORIENTED_EDGE('',*,*,#44705,.T.);
#74184=ORIENTED_EDGE('',*,*,#44702,.T.);
#74185=ORIENTED_EDGE('',*,*,#44699,.T.);
#74186=ORIENTED_EDGE('',*,*,#44707,.T.);
#74187=ORIENTED_EDGE('',*,*,#44717,.T.);
#74188=ORIENTED_EDGE('',*,*,#44714,.T.);
#74189=ORIENTED_EDGE('',*,*,#44711,.T.);
#74190=ORIENTED_EDGE('',*,*,#44719,.T.);
#74191=ORIENTED_EDGE('',*,*,#44729,.T.);
#74192=ORIENTED_EDGE('',*,*,#44726,.T.);
#74193=ORIENTED_EDGE('',*,*,#44723,.T.);
#74194=ORIENTED_EDGE('',*,*,#44731,.T.);
#74195=ORIENTED_EDGE('',*,*,#44741,.T.);
#74196=ORIENTED_EDGE('',*,*,#44738,.T.);
#74197=ORIENTED_EDGE('',*,*,#44735,.T.);
#74198=ORIENTED_EDGE('',*,*,#44743,.T.);
#74199=ORIENTED_EDGE('',*,*,#44753,.T.);
#74200=ORIENTED_EDGE('',*,*,#44750,.T.);
#74201=ORIENTED_EDGE('',*,*,#44747,.T.);
#74202=ORIENTED_EDGE('',*,*,#44755,.T.);
#74203=ORIENTED_EDGE('',*,*,#44765,.T.);
#74204=ORIENTED_EDGE('',*,*,#44762,.T.);
#74205=ORIENTED_EDGE('',*,*,#44759,.T.);
#74206=ORIENTED_EDGE('',*,*,#44767,.T.);
#74207=ORIENTED_EDGE('',*,*,#44777,.T.);
#74208=ORIENTED_EDGE('',*,*,#44774,.T.);
#74209=ORIENTED_EDGE('',*,*,#44771,.T.);
#74210=ORIENTED_EDGE('',*,*,#44779,.T.);
#74211=ORIENTED_EDGE('',*,*,#44789,.T.);
#74212=ORIENTED_EDGE('',*,*,#44786,.T.);
#74213=ORIENTED_EDGE('',*,*,#44783,.T.);
#74214=ORIENTED_EDGE('',*,*,#44791,.T.);
#74215=ORIENTED_EDGE('',*,*,#44801,.T.);
#74216=ORIENTED_EDGE('',*,*,#44798,.T.);
#74217=ORIENTED_EDGE('',*,*,#44795,.T.);
#74218=ORIENTED_EDGE('',*,*,#44803,.T.);
#74219=ORIENTED_EDGE('',*,*,#44813,.T.);
#74220=ORIENTED_EDGE('',*,*,#44810,.T.);
#74221=ORIENTED_EDGE('',*,*,#44807,.T.);
#74222=ORIENTED_EDGE('',*,*,#44815,.T.);
#74223=ORIENTED_EDGE('',*,*,#44825,.T.);
#74224=ORIENTED_EDGE('',*,*,#44822,.T.);
#74225=ORIENTED_EDGE('',*,*,#44819,.T.);
#74226=ORIENTED_EDGE('',*,*,#44827,.T.);
#74227=ORIENTED_EDGE('',*,*,#44837,.T.);
#74228=ORIENTED_EDGE('',*,*,#44834,.T.);
#74229=ORIENTED_EDGE('',*,*,#44831,.T.);
#74230=ORIENTED_EDGE('',*,*,#44839,.T.);
#74231=ORIENTED_EDGE('',*,*,#44849,.T.);
#74232=ORIENTED_EDGE('',*,*,#44846,.T.);
#74233=ORIENTED_EDGE('',*,*,#44843,.T.);
#74234=ORIENTED_EDGE('',*,*,#44851,.T.);
#74235=ORIENTED_EDGE('',*,*,#44861,.T.);
#74236=ORIENTED_EDGE('',*,*,#44858,.T.);
#74237=ORIENTED_EDGE('',*,*,#44855,.T.);
#74238=ORIENTED_EDGE('',*,*,#44863,.T.);
#74239=ORIENTED_EDGE('',*,*,#44873,.T.);
#74240=ORIENTED_EDGE('',*,*,#44870,.T.);
#74241=ORIENTED_EDGE('',*,*,#44867,.T.);
#74242=ORIENTED_EDGE('',*,*,#44875,.T.);
#74243=ORIENTED_EDGE('',*,*,#44885,.T.);
#74244=ORIENTED_EDGE('',*,*,#44882,.T.);
#74245=ORIENTED_EDGE('',*,*,#44879,.T.);
#74246=ORIENTED_EDGE('',*,*,#44887,.T.);
#74247=ORIENTED_EDGE('',*,*,#44897,.T.);
#74248=ORIENTED_EDGE('',*,*,#44894,.T.);
#74249=ORIENTED_EDGE('',*,*,#44891,.T.);
#74250=ORIENTED_EDGE('',*,*,#44899,.T.);
#74251=ORIENTED_EDGE('',*,*,#44909,.T.);
#74252=ORIENTED_EDGE('',*,*,#44906,.T.);
#74253=ORIENTED_EDGE('',*,*,#44903,.T.);
#74254=ORIENTED_EDGE('',*,*,#44911,.T.);
#74255=ORIENTED_EDGE('',*,*,#44921,.T.);
#74256=ORIENTED_EDGE('',*,*,#44918,.T.);
#74257=ORIENTED_EDGE('',*,*,#44915,.T.);
#74258=ORIENTED_EDGE('',*,*,#44923,.T.);
#74259=ORIENTED_EDGE('',*,*,#44933,.T.);
#74260=ORIENTED_EDGE('',*,*,#44930,.T.);
#74261=ORIENTED_EDGE('',*,*,#44927,.T.);
#74262=ORIENTED_EDGE('',*,*,#44935,.T.);
#74263=ORIENTED_EDGE('',*,*,#44945,.T.);
#74264=ORIENTED_EDGE('',*,*,#44942,.T.);
#74265=ORIENTED_EDGE('',*,*,#44939,.T.);
#74266=ORIENTED_EDGE('',*,*,#44947,.T.);
#74267=ORIENTED_EDGE('',*,*,#44957,.T.);
#74268=ORIENTED_EDGE('',*,*,#44954,.T.);
#74269=ORIENTED_EDGE('',*,*,#44951,.T.);
#74270=ORIENTED_EDGE('',*,*,#44959,.T.);
#74271=ORIENTED_EDGE('',*,*,#44969,.T.);
#74272=ORIENTED_EDGE('',*,*,#44966,.T.);
#74273=ORIENTED_EDGE('',*,*,#44963,.T.);
#74274=ORIENTED_EDGE('',*,*,#44971,.T.);
#74275=ORIENTED_EDGE('',*,*,#44981,.T.);
#74276=ORIENTED_EDGE('',*,*,#44978,.T.);
#74277=ORIENTED_EDGE('',*,*,#44975,.T.);
#74278=ORIENTED_EDGE('',*,*,#44983,.T.);
#74279=ORIENTED_EDGE('',*,*,#44993,.T.);
#74280=ORIENTED_EDGE('',*,*,#44990,.T.);
#74281=ORIENTED_EDGE('',*,*,#44987,.T.);
#74282=ORIENTED_EDGE('',*,*,#44995,.T.);
#74283=ORIENTED_EDGE('',*,*,#45005,.T.);
#74284=ORIENTED_EDGE('',*,*,#45002,.T.);
#74285=ORIENTED_EDGE('',*,*,#44999,.T.);
#74286=ORIENTED_EDGE('',*,*,#45007,.T.);
#74287=ORIENTED_EDGE('',*,*,#45017,.T.);
#74288=ORIENTED_EDGE('',*,*,#45014,.T.);
#74289=ORIENTED_EDGE('',*,*,#45011,.T.);
#74290=ORIENTED_EDGE('',*,*,#45019,.T.);
#74291=ORIENTED_EDGE('',*,*,#45029,.T.);
#74292=ORIENTED_EDGE('',*,*,#45026,.T.);
#74293=ORIENTED_EDGE('',*,*,#45023,.T.);
#74294=ORIENTED_EDGE('',*,*,#45031,.T.);
#74295=ORIENTED_EDGE('',*,*,#45041,.T.);
#74296=ORIENTED_EDGE('',*,*,#45038,.T.);
#74297=ORIENTED_EDGE('',*,*,#45035,.T.);
#74298=ORIENTED_EDGE('',*,*,#45043,.T.);
#74299=ORIENTED_EDGE('',*,*,#45053,.T.);
#74300=ORIENTED_EDGE('',*,*,#45050,.T.);
#74301=ORIENTED_EDGE('',*,*,#45047,.T.);
#74302=ORIENTED_EDGE('',*,*,#45055,.T.);
#74303=ORIENTED_EDGE('',*,*,#45065,.T.);
#74304=ORIENTED_EDGE('',*,*,#45062,.T.);
#74305=ORIENTED_EDGE('',*,*,#45059,.T.);
#74306=ORIENTED_EDGE('',*,*,#45067,.T.);
#74307=ORIENTED_EDGE('',*,*,#45077,.T.);
#74308=ORIENTED_EDGE('',*,*,#45074,.T.);
#74309=ORIENTED_EDGE('',*,*,#45071,.T.);
#74310=ORIENTED_EDGE('',*,*,#45079,.T.);
#74311=ORIENTED_EDGE('',*,*,#45089,.T.);
#74312=ORIENTED_EDGE('',*,*,#45086,.T.);
#74313=ORIENTED_EDGE('',*,*,#45083,.T.);
#74314=ORIENTED_EDGE('',*,*,#45091,.T.);
#74315=ORIENTED_EDGE('',*,*,#45101,.T.);
#74316=ORIENTED_EDGE('',*,*,#45098,.T.);
#74317=ORIENTED_EDGE('',*,*,#45095,.T.);
#74318=ORIENTED_EDGE('',*,*,#45103,.T.);
#74319=ORIENTED_EDGE('',*,*,#45113,.T.);
#74320=ORIENTED_EDGE('',*,*,#45110,.T.);
#74321=ORIENTED_EDGE('',*,*,#45107,.T.);
#74322=ORIENTED_EDGE('',*,*,#45115,.T.);
#74323=ORIENTED_EDGE('',*,*,#45125,.T.);
#74324=ORIENTED_EDGE('',*,*,#45122,.T.);
#74325=ORIENTED_EDGE('',*,*,#45119,.T.);
#74326=ORIENTED_EDGE('',*,*,#45127,.T.);
#74327=ORIENTED_EDGE('',*,*,#45137,.T.);
#74328=ORIENTED_EDGE('',*,*,#45134,.T.);
#74329=ORIENTED_EDGE('',*,*,#45131,.T.);
#74330=ORIENTED_EDGE('',*,*,#45139,.T.);
#74331=ORIENTED_EDGE('',*,*,#51998,.T.);
#74332=ORIENTED_EDGE('',*,*,#51996,.T.);
#74333=ORIENTED_EDGE('',*,*,#51994,.T.);
#74334=ORIENTED_EDGE('',*,*,#51999,.T.);
#74335=ORIENTED_EDGE('',*,*,#43532,.T.);
#74336=ORIENTED_EDGE('',*,*,#52000,.F.);
#75297=SPHERICAL_SURFACE('',#85951,15.46041666667);
#75298=SPHERICAL_SURFACE('',#85964,15.76041666667);
#76284=ADVANCED_FACE('',(#20854),#2277,.T.);
#76285=ADVANCED_FACE('',(#20855),#2278,.T.);
#76286=ADVANCED_FACE('',(#20856),#2279,.T.);
#76287=ADVANCED_FACE('',(#20857),#2280,.T.);
#76288=ADVANCED_FACE('',(#20858),#1958,.F.);
#76289=ADVANCED_FACE('',(#20859),#1905,.F.);
#76290=ADVANCED_FACE('',(#20860),#1906,.T.);
#76291=ADVANCED_FACE('',(#20861),#2281,.F.);
#76292=ADVANCED_FACE('',(#20862),#2282,.F.);
#76293=ADVANCED_FACE('',(#20863,#319,#320,#321),#2283,.F.);
#76294=ADVANCED_FACE('',(#20864),#2284,.F.);
#76295=ADVANCED_FACE('',(#20865),#2285,.F.);
#76296=ADVANCED_FACE('',(#20866,#322,#323,#324),#2286,.T.);
#76297=ADVANCED_FACE('',(#20867),#1907,.T.);
#76298=ADVANCED_FACE('',(#20868),#2287,.F.);
#76299=ADVANCED_FACE('',(#20869),#2288,.T.);
#76300=ADVANCED_FACE('',(#20870),#1908,.F.);
#76301=ADVANCED_FACE('',(#20871),#1909,.T.);
#76302=ADVANCED_FACE('',(#20872),#1959,.T.);
#76303=ADVANCED_FACE('',(#20873),#2289,.F.);
#76304=ADVANCED_FACE('',(#20874),#2290,.F.);
#76305=ADVANCED_FACE('',(#20875),#2291,.T.);
#76306=ADVANCED_FACE('',(#20876),#2292,.T.);
#76307=ADVANCED_FACE('',(#20877),#1960,.T.);
#76308=ADVANCED_FACE('',(#20878),#2293,.F.);
#76309=ADVANCED_FACE('',(#20879),#201,.F.);
#76310=ADVANCED_FACE('',(#20880),#202,.F.);
#76311=ADVANCED_FACE('',(#20881),#203,.F.);
#76312=ADVANCED_FACE('',(#20882),#17023,.F.);
#76313=ADVANCED_FACE('',(#20883),#1961,.T.);
#76314=ADVANCED_FACE('',(#20884),#1962,.T.);
#76315=ADVANCED_FACE('',(#20885),#17024,.F.);
#76316=ADVANCED_FACE('',(#20886),#17025,.T.);
#76317=ADVANCED_FACE('',(#20887),#17026,.T.);
#76318=ADVANCED_FACE('',(#20888,#325),#17027,.F.);
#76319=ADVANCED_FACE('',(#20889,#326),#17028,.T.);
#76320=ADVANCED_FACE('',(#20890),#204,.F.);
#76321=ADVANCED_FACE('',(#20891),#2294,.T.);
#76322=ADVANCED_FACE('',(#20892),#205,.F.);
#76323=ADVANCED_FACE('',(#20893),#206,.F.);
#76324=ADVANCED_FACE('',(#20894,#327),#17029,.F.);
#76325=ADVANCED_FACE('',(#20895,#328),#17030,.F.);
#76326=ADVANCED_FACE('',(#20896,#329),#17031,.T.);
#76327=ADVANCED_FACE('',(#20897),#17032,.F.);
#76328=ADVANCED_FACE('',(#20898),#17033,.F.);
#76329=ADVANCED_FACE('',(#20899),#17034,.F.);
#76330=ADVANCED_FACE('',(#20900),#17035,.F.);
#76331=ADVANCED_FACE('',(#20901),#17036,.T.);
#76332=ADVANCED_FACE('',(#20902),#17037,.F.);
#76333=ADVANCED_FACE('',(#20903),#17038,.F.);
#76334=ADVANCED_FACE('',(#20904),#17039,.F.);
#76335=ADVANCED_FACE('',(#20905),#17040,.F.);
#76336=ADVANCED_FACE('',(#20906),#17041,.T.);
#76337=ADVANCED_FACE('',(#20907),#17042,.F.);
#76338=ADVANCED_FACE('',(#20908),#17043,.F.);
#76339=ADVANCED_FACE('',(#20909),#17044,.F.);
#76340=ADVANCED_FACE('',(#20910),#17045,.F.);
#76341=ADVANCED_FACE('',(#20911),#17046,.T.);
#76342=ADVANCED_FACE('',(#20912),#17047,.F.);
#76343=ADVANCED_FACE('',(#20913),#17048,.F.);
#76344=ADVANCED_FACE('',(#20914),#17049,.F.);
#76345=ADVANCED_FACE('',(#20915),#17050,.F.);
#76346=ADVANCED_FACE('',(#20916),#17051,.F.);
#76347=ADVANCED_FACE('',(#20917),#17052,.F.);
#76348=ADVANCED_FACE('',(#20918),#17053,.F.);
#76349=ADVANCED_FACE('',(#20919),#17054,.F.);
#76350=ADVANCED_FACE('',(#20920),#17055,.F.);
#76351=ADVANCED_FACE('',(#20921),#17056,.F.);
#76352=ADVANCED_FACE('',(#20922),#17057,.F.);
#76353=ADVANCED_FACE('',(#20923),#17058,.F.);
#76354=ADVANCED_FACE('',(#20924),#17059,.F.);
#76355=ADVANCED_FACE('',(#20925),#17060,.F.);
#76356=ADVANCED_FACE('',(#20926),#17061,.F.);
#76357=ADVANCED_FACE('',(#20927),#17062,.F.);
#76358=ADVANCED_FACE('',(#20928),#17063,.F.);
#76359=ADVANCED_FACE('',(#20929),#17064,.F.);
#76360=ADVANCED_FACE('',(#20930),#17065,.F.);
#76361=ADVANCED_FACE('',(#20931),#17066,.F.);
#76362=ADVANCED_FACE('',(#20932),#17067,.T.);
#76363=ADVANCED_FACE('',(#20933),#17068,.F.);
#76364=ADVANCED_FACE('',(#20934),#17069,.F.);
#76365=ADVANCED_FACE('',(#20935),#17070,.F.);
#76366=ADVANCED_FACE('',(#20936),#17071,.F.);
#76367=ADVANCED_FACE('',(#20937),#17072,.T.);
#76368=ADVANCED_FACE('',(#20938),#17073,.F.);
#76369=ADVANCED_FACE('',(#20939),#17074,.F.);
#76370=ADVANCED_FACE('',(#20940),#17075,.F.);
#76371=ADVANCED_FACE('',(#20941),#17076,.F.);
#76372=ADVANCED_FACE('',(#20942),#17077,.T.);
#76373=ADVANCED_FACE('',(#20943),#17078,.F.);
#76374=ADVANCED_FACE('',(#20944),#17079,.F.);
#76375=ADVANCED_FACE('',(#20945),#17080,.F.);
#76376=ADVANCED_FACE('',(#20946),#17081,.F.);
#76377=ADVANCED_FACE('',(#20947),#17082,.T.);
#76378=ADVANCED_FACE('',(#20948),#17083,.F.);
#76379=ADVANCED_FACE('',(#20949),#17084,.F.);
#76380=ADVANCED_FACE('',(#20950),#17085,.F.);
#76381=ADVANCED_FACE('',(#20951),#17086,.F.);
#76382=ADVANCED_FACE('',(#20952),#17087,.F.);
#76383=ADVANCED_FACE('',(#20953),#17088,.F.);
#76384=ADVANCED_FACE('',(#20954),#17089,.F.);
#76385=ADVANCED_FACE('',(#20955),#17090,.F.);
#76386=ADVANCED_FACE('',(#20956),#17091,.T.);
#76387=ADVANCED_FACE('',(#20957),#17092,.F.);
#76388=ADVANCED_FACE('',(#20958),#17093,.F.);
#76389=ADVANCED_FACE('',(#20959),#17094,.F.);
#76390=ADVANCED_FACE('',(#20960),#17095,.F.);
#76391=ADVANCED_FACE('',(#20961),#17096,.T.);
#76392=ADVANCED_FACE('',(#20962),#17097,.F.);
#76393=ADVANCED_FACE('',(#20963),#17098,.F.);
#76394=ADVANCED_FACE('',(#20964),#17099,.F.);
#76395=ADVANCED_FACE('',(#20965),#17100,.F.);
#76396=ADVANCED_FACE('',(#20966),#17101,.T.);
#76397=ADVANCED_FACE('',(#20967),#17102,.F.);
#76398=ADVANCED_FACE('',(#20968),#17103,.F.);
#76399=ADVANCED_FACE('',(#20969),#17104,.F.);
#76400=ADVANCED_FACE('',(#20970),#17105,.F.);
#76401=ADVANCED_FACE('',(#20971),#17106,.T.);
#76402=ADVANCED_FACE('',(#20972),#17107,.F.);
#76403=ADVANCED_FACE('',(#20973),#17108,.F.);
#76404=ADVANCED_FACE('',(#20974),#17109,.F.);
#76405=ADVANCED_FACE('',(#20975),#17110,.F.);
#76406=ADVANCED_FACE('',(#20976),#17111,.F.);
#76407=ADVANCED_FACE('',(#20977),#17112,.F.);
#76408=ADVANCED_FACE('',(#20978),#17113,.F.);
#76409=ADVANCED_FACE('',(#20979),#17114,.F.);
#76410=ADVANCED_FACE('',(#20980),#17115,.F.);
#76411=ADVANCED_FACE('',(#20981),#17116,.F.);
#76412=ADVANCED_FACE('',(#20982),#17117,.F.);
#76413=ADVANCED_FACE('',(#20983),#17118,.F.);
#76414=ADVANCED_FACE('',(#20984),#17119,.F.);
#76415=ADVANCED_FACE('',(#20985),#17120,.F.);
#76416=ADVANCED_FACE('',(#20986),#17121,.F.);
#76417=ADVANCED_FACE('',(#20987),#17122,.F.);
#76418=ADVANCED_FACE('',(#20988),#17123,.F.);
#76419=ADVANCED_FACE('',(#20989),#17124,.F.);
#76420=ADVANCED_FACE('',(#20990),#17125,.F.);
#76421=ADVANCED_FACE('',(#20991),#17126,.F.);
#76422=ADVANCED_FACE('',(#20992),#17127,.F.);
#76423=ADVANCED_FACE('',(#20993),#17128,.F.);
#76424=ADVANCED_FACE('',(#20994),#17129,.F.);
#76425=ADVANCED_FACE('',(#20995),#17130,.F.);
#76426=ADVANCED_FACE('',(#20996),#17131,.F.);
#76427=ADVANCED_FACE('',(#20997),#17132,.F.);
#76428=ADVANCED_FACE('',(#20998),#17133,.F.);
#76429=ADVANCED_FACE('',(#20999),#17134,.F.);
#76430=ADVANCED_FACE('',(#21000),#17135,.T.);
#76431=ADVANCED_FACE('',(#21001),#17136,.F.);
#76432=ADVANCED_FACE('',(#21002),#17137,.F.);
#76433=ADVANCED_FACE('',(#21003),#17138,.F.);
#76434=ADVANCED_FACE('',(#21004),#17139,.F.);
#76435=ADVANCED_FACE('',(#21005),#17140,.T.);
#76436=ADVANCED_FACE('',(#21006),#17141,.F.);
#76437=ADVANCED_FACE('',(#21007),#17142,.F.);
#76438=ADVANCED_FACE('',(#21008),#17143,.F.);
#76439=ADVANCED_FACE('',(#21009),#17144,.F.);
#76440=ADVANCED_FACE('',(#21010),#17145,.F.);
#76441=ADVANCED_FACE('',(#21011),#17146,.F.);
#76442=ADVANCED_FACE('',(#21012),#17147,.F.);
#76443=ADVANCED_FACE('',(#21013),#17148,.F.);
#76444=ADVANCED_FACE('',(#21014),#17149,.F.);
#76445=ADVANCED_FACE('',(#21015),#17150,.F.);
#76446=ADVANCED_FACE('',(#21016),#17151,.F.);
#76447=ADVANCED_FACE('',(#21017),#17152,.F.);
#76448=ADVANCED_FACE('',(#21018),#17153,.F.);
#76449=ADVANCED_FACE('',(#21019),#17154,.F.);
#76450=ADVANCED_FACE('',(#21020),#17155,.F.);
#76451=ADVANCED_FACE('',(#21021),#17156,.F.);
#76452=ADVANCED_FACE('',(#21022),#17157,.F.);
#76453=ADVANCED_FACE('',(#21023),#17158,.F.);
#76454=ADVANCED_FACE('',(#21024),#17159,.F.);
#76455=ADVANCED_FACE('',(#21025),#17160,.F.);
#76456=ADVANCED_FACE('',(#21026),#17161,.F.);
#76457=ADVANCED_FACE('',(#21027),#17162,.F.);
#76458=ADVANCED_FACE('',(#21028),#17163,.F.);
#76459=ADVANCED_FACE('',(#21029),#17164,.F.);
#76460=ADVANCED_FACE('',(#21030),#17165,.F.);
#76461=ADVANCED_FACE('',(#21031),#17166,.F.);
#76462=ADVANCED_FACE('',(#21032),#17167,.F.);
#76463=ADVANCED_FACE('',(#21033),#17168,.F.);
#76464=ADVANCED_FACE('',(#21034),#17169,.F.);
#76465=ADVANCED_FACE('',(#21035),#17170,.F.);
#76466=ADVANCED_FACE('',(#21036),#17171,.F.);
#76467=ADVANCED_FACE('',(#21037),#17172,.F.);
#76468=ADVANCED_FACE('',(#21038),#17173,.F.);
#76469=ADVANCED_FACE('',(#21039),#17174,.F.);
#76470=ADVANCED_FACE('',(#21040),#17175,.F.);
#76471=ADVANCED_FACE('',(#21041),#17176,.F.);
#76472=ADVANCED_FACE('',(#21042),#17177,.T.);
#76473=ADVANCED_FACE('',(#21043),#17178,.F.);
#76474=ADVANCED_FACE('',(#21044),#17179,.F.);
#76475=ADVANCED_FACE('',(#21045),#17180,.F.);
#76476=ADVANCED_FACE('',(#21046),#17181,.F.);
#76477=ADVANCED_FACE('',(#21047),#17182,.T.);
#76478=ADVANCED_FACE('',(#21048),#17183,.F.);
#76479=ADVANCED_FACE('',(#21049),#17184,.F.);
#76480=ADVANCED_FACE('',(#21050),#17185,.F.);
#76481=ADVANCED_FACE('',(#21051),#17186,.F.);
#76482=ADVANCED_FACE('',(#21052),#17187,.F.);
#76483=ADVANCED_FACE('',(#21053),#17188,.F.);
#76484=ADVANCED_FACE('',(#21054),#17189,.F.);
#76485=ADVANCED_FACE('',(#21055),#17190,.F.);
#76486=ADVANCED_FACE('',(#21056),#17191,.F.);
#76487=ADVANCED_FACE('',(#21057),#17192,.F.);
#76488=ADVANCED_FACE('',(#21058),#17193,.F.);
#76489=ADVANCED_FACE('',(#21059),#17194,.F.);
#76490=ADVANCED_FACE('',(#21060),#17195,.F.);
#76491=ADVANCED_FACE('',(#21061),#17196,.F.);
#76492=ADVANCED_FACE('',(#21062),#17197,.F.);
#76493=ADVANCED_FACE('',(#21063),#17198,.F.);
#76494=ADVANCED_FACE('',(#21064),#17199,.F.);
#76495=ADVANCED_FACE('',(#21065),#17200,.F.);
#76496=ADVANCED_FACE('',(#21066),#17201,.F.);
#76497=ADVANCED_FACE('',(#21067),#17202,.F.);
#76498=ADVANCED_FACE('',(#21068),#17203,.F.);
#76499=ADVANCED_FACE('',(#21069),#17204,.F.);
#76500=ADVANCED_FACE('',(#21070),#17205,.F.);
#76501=ADVANCED_FACE('',(#21071),#17206,.F.);
#76502=ADVANCED_FACE('',(#21072),#17207,.F.);
#76503=ADVANCED_FACE('',(#21073),#17208,.F.);
#76504=ADVANCED_FACE('',(#21074),#17209,.F.);
#76505=ADVANCED_FACE('',(#21075),#17210,.F.);
#76506=ADVANCED_FACE('',(#21076),#17211,.F.);
#76507=ADVANCED_FACE('',(#21077),#17212,.F.);
#76508=ADVANCED_FACE('',(#21078),#17213,.F.);
#76509=ADVANCED_FACE('',(#21079),#17214,.F.);
#76510=ADVANCED_FACE('',(#21080),#17215,.F.);
#76511=ADVANCED_FACE('',(#21081),#17216,.F.);
#76512=ADVANCED_FACE('',(#21082),#17217,.F.);
#76513=ADVANCED_FACE('',(#21083),#17218,.F.);
#76514=ADVANCED_FACE('',(#21084),#17219,.F.);
#76515=ADVANCED_FACE('',(#21085),#17220,.F.);
#76516=ADVANCED_FACE('',(#21086),#17221,.F.);
#76517=ADVANCED_FACE('',(#21087),#17222,.F.);
#76518=ADVANCED_FACE('',(#21088),#17223,.T.);
#76519=ADVANCED_FACE('',(#21089),#17224,.F.);
#76520=ADVANCED_FACE('',(#21090),#17225,.F.);
#76521=ADVANCED_FACE('',(#21091),#17226,.F.);
#76522=ADVANCED_FACE('',(#21092),#17227,.F.);
#76523=ADVANCED_FACE('',(#21093),#17228,.F.);
#76524=ADVANCED_FACE('',(#21094),#17229,.F.);
#76525=ADVANCED_FACE('',(#21095),#17230,.F.);
#76526=ADVANCED_FACE('',(#21096),#17231,.F.);
#76527=ADVANCED_FACE('',(#21097),#17232,.F.);
#76528=ADVANCED_FACE('',(#21098),#17233,.F.);
#76529=ADVANCED_FACE('',(#21099),#17234,.F.);
#76530=ADVANCED_FACE('',(#21100),#17235,.F.);
#76531=ADVANCED_FACE('',(#21101),#17236,.F.);
#76532=ADVANCED_FACE('',(#21102),#17237,.F.);
#76533=ADVANCED_FACE('',(#21103),#17238,.F.);
#76534=ADVANCED_FACE('',(#21104),#17239,.F.);
#76535=ADVANCED_FACE('',(#21105),#17240,.F.);
#76536=ADVANCED_FACE('',(#21106),#17241,.F.);
#76537=ADVANCED_FACE('',(#21107),#17242,.F.);
#76538=ADVANCED_FACE('',(#21108),#17243,.F.);
#76539=ADVANCED_FACE('',(#21109),#17244,.F.);
#76540=ADVANCED_FACE('',(#21110),#17245,.F.);
#76541=ADVANCED_FACE('',(#21111),#17246,.F.);
#76542=ADVANCED_FACE('',(#21112),#17247,.F.);
#76543=ADVANCED_FACE('',(#21113),#17248,.F.);
#76544=ADVANCED_FACE('',(#21114),#17249,.F.);
#76545=ADVANCED_FACE('',(#21115),#17250,.F.);
#76546=ADVANCED_FACE('',(#21116),#17251,.F.);
#76547=ADVANCED_FACE('',(#21117),#17252,.F.);
#76548=ADVANCED_FACE('',(#21118),#17253,.F.);
#76549=ADVANCED_FACE('',(#21119),#17254,.F.);
#76550=ADVANCED_FACE('',(#21120),#17255,.F.);
#76551=ADVANCED_FACE('',(#21121),#17256,.F.);
#76552=ADVANCED_FACE('',(#21122),#17257,.F.);
#76553=ADVANCED_FACE('',(#21123),#17258,.F.);
#76554=ADVANCED_FACE('',(#21124),#17259,.F.);
#76555=ADVANCED_FACE('',(#21125),#17260,.F.);
#76556=ADVANCED_FACE('',(#21126),#17261,.F.);
#76557=ADVANCED_FACE('',(#21127),#17262,.F.);
#76558=ADVANCED_FACE('',(#21128),#17263,.F.);
#76559=ADVANCED_FACE('',(#21129),#17264,.F.);
#76560=ADVANCED_FACE('',(#21130),#17265,.F.);
#76561=ADVANCED_FACE('',(#21131),#17266,.F.);
#76562=ADVANCED_FACE('',(#21132),#17267,.F.);
#76563=ADVANCED_FACE('',(#21133),#17268,.F.);
#76564=ADVANCED_FACE('',(#21134),#17269,.F.);
#76565=ADVANCED_FACE('',(#21135),#17270,.F.);
#76566=ADVANCED_FACE('',(#21136),#17271,.F.);
#76567=ADVANCED_FACE('',(#21137),#17272,.T.);
#76568=ADVANCED_FACE('',(#21138),#17273,.F.);
#76569=ADVANCED_FACE('',(#21139),#17274,.F.);
#76570=ADVANCED_FACE('',(#21140),#17275,.F.);
#76571=ADVANCED_FACE('',(#21141),#17276,.F.);
#76572=ADVANCED_FACE('',(#21142),#17277,.T.);
#76573=ADVANCED_FACE('',(#21143),#17278,.F.);
#76574=ADVANCED_FACE('',(#21144),#17279,.F.);
#76575=ADVANCED_FACE('',(#21145),#17280,.F.);
#76576=ADVANCED_FACE('',(#21146),#17281,.F.);
#76577=ADVANCED_FACE('',(#21147),#17282,.F.);
#76578=ADVANCED_FACE('',(#21148),#17283,.F.);
#76579=ADVANCED_FACE('',(#21149),#17284,.F.);
#76580=ADVANCED_FACE('',(#21150),#17285,.F.);
#76581=ADVANCED_FACE('',(#21151),#17286,.F.);
#76582=ADVANCED_FACE('',(#21152),#17287,.F.);
#76583=ADVANCED_FACE('',(#21153),#17288,.F.);
#76584=ADVANCED_FACE('',(#21154),#17289,.F.);
#76585=ADVANCED_FACE('',(#21155),#17290,.F.);
#76586=ADVANCED_FACE('',(#21156),#17291,.F.);
#76587=ADVANCED_FACE('',(#21157),#17292,.F.);
#76588=ADVANCED_FACE('',(#21158),#17293,.F.);
#76589=ADVANCED_FACE('',(#21159),#17294,.F.);
#76590=ADVANCED_FACE('',(#21160),#17295,.F.);
#76591=ADVANCED_FACE('',(#21161),#17296,.F.);
#76592=ADVANCED_FACE('',(#21162),#17297,.F.);
#76593=ADVANCED_FACE('',(#21163),#17298,.F.);
#76594=ADVANCED_FACE('',(#21164),#17299,.F.);
#76595=ADVANCED_FACE('',(#21165),#17300,.F.);
#76596=ADVANCED_FACE('',(#21166),#17301,.F.);
#76597=ADVANCED_FACE('',(#21167),#17302,.F.);
#76598=ADVANCED_FACE('',(#21168),#17303,.F.);
#76599=ADVANCED_FACE('',(#21169),#17304,.F.);
#76600=ADVANCED_FACE('',(#21170),#17305,.F.);
#76601=ADVANCED_FACE('',(#21171),#17306,.F.);
#76602=ADVANCED_FACE('',(#21172),#17307,.F.);
#76603=ADVANCED_FACE('',(#21173),#17308,.F.);
#76604=ADVANCED_FACE('',(#21174),#17309,.F.);
#76605=ADVANCED_FACE('',(#21175),#17310,.F.);
#76606=ADVANCED_FACE('',(#21176),#17311,.F.);
#76607=ADVANCED_FACE('',(#21177),#17312,.F.);
#76608=ADVANCED_FACE('',(#21178),#17313,.F.);
#76609=ADVANCED_FACE('',(#21179),#17314,.F.);
#76610=ADVANCED_FACE('',(#21180),#17315,.F.);
#76611=ADVANCED_FACE('',(#21181),#17316,.F.);
#76612=ADVANCED_FACE('',(#21182),#17317,.F.);
#76613=ADVANCED_FACE('',(#21183),#17318,.F.);
#76614=ADVANCED_FACE('',(#21184),#17319,.F.);
#76615=ADVANCED_FACE('',(#21185),#17320,.F.);
#76616=ADVANCED_FACE('',(#21186),#17321,.F.);
#76617=ADVANCED_FACE('',(#21187),#17322,.F.);
#76618=ADVANCED_FACE('',(#21188),#17323,.F.);
#76619=ADVANCED_FACE('',(#21189),#17324,.F.);
#76620=ADVANCED_FACE('',(#21190),#17325,.F.);
#76621=ADVANCED_FACE('',(#21191),#17326,.F.);
#76622=ADVANCED_FACE('',(#21192),#17327,.F.);
#76623=ADVANCED_FACE('',(#21193),#17328,.F.);
#76624=ADVANCED_FACE('',(#21194),#17329,.F.);
#76625=ADVANCED_FACE('',(#21195),#17330,.F.);
#76626=ADVANCED_FACE('',(#21196),#17331,.F.);
#76627=ADVANCED_FACE('',(#21197),#17332,.F.);
#76628=ADVANCED_FACE('',(#21198),#17333,.F.);
#76629=ADVANCED_FACE('',(#21199),#17334,.F.);
#76630=ADVANCED_FACE('',(#21200),#17335,.F.);
#76631=ADVANCED_FACE('',(#21201),#17336,.F.);
#76632=ADVANCED_FACE('',(#21202),#17337,.F.);
#76633=ADVANCED_FACE('',(#21203),#17338,.F.);
#76634=ADVANCED_FACE('',(#21204),#17339,.F.);
#76635=ADVANCED_FACE('',(#21205),#17340,.F.);
#76636=ADVANCED_FACE('',(#21206),#17341,.F.);
#76637=ADVANCED_FACE('',(#21207),#17342,.F.);
#76638=ADVANCED_FACE('',(#21208),#17343,.F.);
#76639=ADVANCED_FACE('',(#21209),#17344,.F.);
#76640=ADVANCED_FACE('',(#21210),#17345,.F.);
#76641=ADVANCED_FACE('',(#21211),#17346,.F.);
#76642=ADVANCED_FACE('',(#21212),#17347,.F.);
#76643=ADVANCED_FACE('',(#21213),#17348,.F.);
#76644=ADVANCED_FACE('',(#21214),#17349,.F.);
#76645=ADVANCED_FACE('',(#21215),#17350,.F.);
#76646=ADVANCED_FACE('',(#21216),#17351,.F.);
#76647=ADVANCED_FACE('',(#21217),#17352,.F.);
#76648=ADVANCED_FACE('',(#21218),#17353,.F.);
#76649=ADVANCED_FACE('',(#21219),#17354,.F.);
#76650=ADVANCED_FACE('',(#21220),#17355,.F.);
#76651=ADVANCED_FACE('',(#21221),#17356,.F.);
#76652=ADVANCED_FACE('',(#21222),#17357,.F.);
#76653=ADVANCED_FACE('',(#21223),#17358,.F.);
#76654=ADVANCED_FACE('',(#21224),#17359,.F.);
#76655=ADVANCED_FACE('',(#21225),#17360,.F.);
#76656=ADVANCED_FACE('',(#21226),#17361,.F.);
#76657=ADVANCED_FACE('',(#21227),#17362,.F.);
#76658=ADVANCED_FACE('',(#21228),#17363,.F.);
#76659=ADVANCED_FACE('',(#21229),#17364,.F.);
#76660=ADVANCED_FACE('',(#21230),#17365,.F.);
#76661=ADVANCED_FACE('',(#21231),#17366,.F.);
#76662=ADVANCED_FACE('',(#21232),#17367,.F.);
#76663=ADVANCED_FACE('',(#21233),#17368,.F.);
#76664=ADVANCED_FACE('',(#21234),#17369,.F.);
#76665=ADVANCED_FACE('',(#21235),#17370,.F.);
#76666=ADVANCED_FACE('',(#21236),#17371,.F.);
#76667=ADVANCED_FACE('',(#21237),#17372,.F.);
#76668=ADVANCED_FACE('',(#21238),#17373,.F.);
#76669=ADVANCED_FACE('',(#21239),#17374,.F.);
#76670=ADVANCED_FACE('',(#21240),#17375,.F.);
#76671=ADVANCED_FACE('',(#21241),#17376,.F.);
#76672=ADVANCED_FACE('',(#21242),#17377,.F.);
#76673=ADVANCED_FACE('',(#21243),#17378,.F.);
#76674=ADVANCED_FACE('',(#21244),#17379,.F.);
#76675=ADVANCED_FACE('',(#21245),#17380,.F.);
#76676=ADVANCED_FACE('',(#21246),#17381,.F.);
#76677=ADVANCED_FACE('',(#21247),#17382,.F.);
#76678=ADVANCED_FACE('',(#21248),#17383,.F.);
#76679=ADVANCED_FACE('',(#21249),#17384,.F.);
#76680=ADVANCED_FACE('',(#21250),#17385,.F.);
#76681=ADVANCED_FACE('',(#21251),#17386,.F.);
#76682=ADVANCED_FACE('',(#21252),#17387,.F.);
#76683=ADVANCED_FACE('',(#21253),#17388,.F.);
#76684=ADVANCED_FACE('',(#21254),#17389,.F.);
#76685=ADVANCED_FACE('',(#21255),#17390,.F.);
#76686=ADVANCED_FACE('',(#21256),#17391,.F.);
#76687=ADVANCED_FACE('',(#21257),#17392,.F.);
#76688=ADVANCED_FACE('',(#21258),#17393,.F.);
#76689=ADVANCED_FACE('',(#21259),#17394,.F.);
#76690=ADVANCED_FACE('',(#21260),#17395,.F.);
#76691=ADVANCED_FACE('',(#21261),#17396,.F.);
#76692=ADVANCED_FACE('',(#21262),#17397,.F.);
#76693=ADVANCED_FACE('',(#21263),#17398,.F.);
#76694=ADVANCED_FACE('',(#21264),#17399,.F.);
#76695=ADVANCED_FACE('',(#21265),#17400,.F.);
#76696=ADVANCED_FACE('',(#21266),#17401,.F.);
#76697=ADVANCED_FACE('',(#21267),#17402,.F.);
#76698=ADVANCED_FACE('',(#21268),#17403,.F.);
#76699=ADVANCED_FACE('',(#21269),#17404,.F.);
#76700=ADVANCED_FACE('',(#21270),#17405,.F.);
#76701=ADVANCED_FACE('',(#21271),#17406,.F.);
#76702=ADVANCED_FACE('',(#21272),#17407,.F.);
#76703=ADVANCED_FACE('',(#21273),#17408,.F.);
#76704=ADVANCED_FACE('',(#21274),#17409,.F.);
#76705=ADVANCED_FACE('',(#21275),#17410,.F.);
#76706=ADVANCED_FACE('',(#21276),#17411,.F.);
#76707=ADVANCED_FACE('',(#21277),#17412,.F.);
#76708=ADVANCED_FACE('',(#21278),#17413,.F.);
#76709=ADVANCED_FACE('',(#21279),#17414,.F.);
#76710=ADVANCED_FACE('',(#21280),#17415,.F.);
#76711=ADVANCED_FACE('',(#21281),#17416,.F.);
#76712=ADVANCED_FACE('',(#21282),#17417,.F.);
#76713=ADVANCED_FACE('',(#21283),#17418,.F.);
#76714=ADVANCED_FACE('',(#21284),#17419,.F.);
#76715=ADVANCED_FACE('',(#21285),#17420,.F.);
#76716=ADVANCED_FACE('',(#21286),#17421,.F.);
#76717=ADVANCED_FACE('',(#21287),#17422,.F.);
#76718=ADVANCED_FACE('',(#21288),#17423,.F.);
#76719=ADVANCED_FACE('',(#21289),#17424,.F.);
#76720=ADVANCED_FACE('',(#21290),#17425,.F.);
#76721=ADVANCED_FACE('',(#21291),#17426,.F.);
#76722=ADVANCED_FACE('',(#21292),#17427,.F.);
#76723=ADVANCED_FACE('',(#21293),#17428,.F.);
#76724=ADVANCED_FACE('',(#21294),#17429,.F.);
#76725=ADVANCED_FACE('',(#21295),#17430,.F.);
#76726=ADVANCED_FACE('',(#21296),#17431,.F.);
#76727=ADVANCED_FACE('',(#21297),#17432,.F.);
#76728=ADVANCED_FACE('',(#21298),#17433,.F.);
#76729=ADVANCED_FACE('',(#21299),#17434,.F.);
#76730=ADVANCED_FACE('',(#21300),#17435,.F.);
#76731=ADVANCED_FACE('',(#21301),#17436,.F.);
#76732=ADVANCED_FACE('',(#21302),#17437,.F.);
#76733=ADVANCED_FACE('',(#21303),#17438,.F.);
#76734=ADVANCED_FACE('',(#21304),#17439,.F.);
#76735=ADVANCED_FACE('',(#21305),#17440,.F.);
#76736=ADVANCED_FACE('',(#21306),#17441,.F.);
#76737=ADVANCED_FACE('',(#21307),#17442,.F.);
#76738=ADVANCED_FACE('',(#21308),#17443,.F.);
#76739=ADVANCED_FACE('',(#21309),#17444,.F.);
#76740=ADVANCED_FACE('',(#21310),#17445,.F.);
#76741=ADVANCED_FACE('',(#21311),#17446,.F.);
#76742=ADVANCED_FACE('',(#21312),#17447,.F.);
#76743=ADVANCED_FACE('',(#21313),#17448,.F.);
#76744=ADVANCED_FACE('',(#21314),#17449,.F.);
#76745=ADVANCED_FACE('',(#21315),#17450,.F.);
#76746=ADVANCED_FACE('',(#21316),#17451,.F.);
#76747=ADVANCED_FACE('',(#21317),#17452,.F.);
#76748=ADVANCED_FACE('',(#21318),#17453,.F.);
#76749=ADVANCED_FACE('',(#21319),#17454,.F.);
#76750=ADVANCED_FACE('',(#21320),#17455,.F.);
#76751=ADVANCED_FACE('',(#21321),#17456,.F.);
#76752=ADVANCED_FACE('',(#21322),#17457,.F.);
#76753=ADVANCED_FACE('',(#21323),#17458,.F.);
#76754=ADVANCED_FACE('',(#21324),#17459,.F.);
#76755=ADVANCED_FACE('',(#21325),#17460,.F.);
#76756=ADVANCED_FACE('',(#21326),#17461,.F.);
#76757=ADVANCED_FACE('',(#21327),#17462,.F.);
#76758=ADVANCED_FACE('',(#21328),#17463,.F.);
#76759=ADVANCED_FACE('',(#21329),#17464,.F.);
#76760=ADVANCED_FACE('',(#21330),#17465,.F.);
#76761=ADVANCED_FACE('',(#21331),#17466,.F.);
#76762=ADVANCED_FACE('',(#21332),#17467,.F.);
#76763=ADVANCED_FACE('',(#21333),#17468,.F.);
#76764=ADVANCED_FACE('',(#21334),#17469,.F.);
#76765=ADVANCED_FACE('',(#21335),#17470,.F.);
#76766=ADVANCED_FACE('',(#21336),#17471,.F.);
#76767=ADVANCED_FACE('',(#21337),#17472,.F.);
#76768=ADVANCED_FACE('',(#21338),#17473,.F.);
#76769=ADVANCED_FACE('',(#21339),#17474,.F.);
#76770=ADVANCED_FACE('',(#21340),#17475,.F.);
#76771=ADVANCED_FACE('',(#21341),#17476,.F.);
#76772=ADVANCED_FACE('',(#21342),#17477,.F.);
#76773=ADVANCED_FACE('',(#21343),#17478,.F.);
#76774=ADVANCED_FACE('',(#21344),#17479,.F.);
#76775=ADVANCED_FACE('',(#21345),#17480,.F.);
#76776=ADVANCED_FACE('',(#21346),#17481,.F.);
#76777=ADVANCED_FACE('',(#21347),#17482,.F.);
#76778=ADVANCED_FACE('',(#21348),#17483,.F.);
#76779=ADVANCED_FACE('',(#21349),#17484,.F.);
#76780=ADVANCED_FACE('',(#21350),#17485,.F.);
#76781=ADVANCED_FACE('',(#21351),#17486,.F.);
#76782=ADVANCED_FACE('',(#21352),#17487,.F.);
#76783=ADVANCED_FACE('',(#21353),#17488,.F.);
#76784=ADVANCED_FACE('',(#21354),#17489,.F.);
#76785=ADVANCED_FACE('',(#21355),#17490,.F.);
#76786=ADVANCED_FACE('',(#21356),#17491,.F.);
#76787=ADVANCED_FACE('',(#21357),#17492,.F.);
#76788=ADVANCED_FACE('',(#21358),#17493,.F.);
#76789=ADVANCED_FACE('',(#21359),#17494,.F.);
#76790=ADVANCED_FACE('',(#21360),#17495,.F.);
#76791=ADVANCED_FACE('',(#21361),#17496,.F.);
#76792=ADVANCED_FACE('',(#21362),#17497,.F.);
#76793=ADVANCED_FACE('',(#21363),#17498,.F.);
#76794=ADVANCED_FACE('',(#21364),#17499,.F.);
#76795=ADVANCED_FACE('',(#21365),#17500,.F.);
#76796=ADVANCED_FACE('',(#21366),#17501,.F.);
#76797=ADVANCED_FACE('',(#21367),#17502,.F.);
#76798=ADVANCED_FACE('',(#21368),#17503,.F.);
#76799=ADVANCED_FACE('',(#21369),#17504,.F.);
#76800=ADVANCED_FACE('',(#21370),#17505,.F.);
#76801=ADVANCED_FACE('',(#21371),#17506,.F.);
#76802=ADVANCED_FACE('',(#21372),#17507,.F.);
#76803=ADVANCED_FACE('',(#21373),#17508,.F.);
#76804=ADVANCED_FACE('',(#21374),#17509,.F.);
#76805=ADVANCED_FACE('',(#21375),#17510,.F.);
#76806=ADVANCED_FACE('',(#21376),#17511,.F.);
#76807=ADVANCED_FACE('',(#21377),#17512,.F.);
#76808=ADVANCED_FACE('',(#21378),#17513,.F.);
#76809=ADVANCED_FACE('',(#21379),#17514,.F.);
#76810=ADVANCED_FACE('',(#21380),#17515,.F.);
#76811=ADVANCED_FACE('',(#21381),#17516,.F.);
#76812=ADVANCED_FACE('',(#21382),#17517,.F.);
#76813=ADVANCED_FACE('',(#21383),#17518,.F.);
#76814=ADVANCED_FACE('',(#21384),#17519,.F.);
#76815=ADVANCED_FACE('',(#21385),#17520,.F.);
#76816=ADVANCED_FACE('',(#21386),#17521,.F.);
#76817=ADVANCED_FACE('',(#21387),#17522,.F.);
#76818=ADVANCED_FACE('',(#21388),#17523,.F.);
#76819=ADVANCED_FACE('',(#21389),#17524,.F.);
#76820=ADVANCED_FACE('',(#21390),#17525,.F.);
#76821=ADVANCED_FACE('',(#21391),#17526,.F.);
#76822=ADVANCED_FACE('',(#21392),#17527,.F.);
#76823=ADVANCED_FACE('',(#21393),#17528,.F.);
#76824=ADVANCED_FACE('',(#21394),#17529,.F.);
#76825=ADVANCED_FACE('',(#21395),#17530,.F.);
#76826=ADVANCED_FACE('',(#21396),#17531,.F.);
#76827=ADVANCED_FACE('',(#21397),#17532,.F.);
#76828=ADVANCED_FACE('',(#21398),#17533,.F.);
#76829=ADVANCED_FACE('',(#21399),#17534,.F.);
#76830=ADVANCED_FACE('',(#21400),#17535,.F.);
#76831=ADVANCED_FACE('',(#21401),#17536,.F.);
#76832=ADVANCED_FACE('',(#21402),#17537,.F.);
#76833=ADVANCED_FACE('',(#21403),#17538,.F.);
#76834=ADVANCED_FACE('',(#21404),#17539,.F.);
#76835=ADVANCED_FACE('',(#21405),#17540,.F.);
#76836=ADVANCED_FACE('',(#21406),#17541,.F.);
#76837=ADVANCED_FACE('',(#21407),#17542,.F.);
#76838=ADVANCED_FACE('',(#21408),#17543,.F.);
#76839=ADVANCED_FACE('',(#21409),#17544,.F.);
#76840=ADVANCED_FACE('',(#21410),#17545,.F.);
#76841=ADVANCED_FACE('',(#21411),#17546,.F.);
#76842=ADVANCED_FACE('',(#21412),#17547,.F.);
#76843=ADVANCED_FACE('',(#21413),#17548,.F.);
#76844=ADVANCED_FACE('',(#21414),#17549,.F.);
#76845=ADVANCED_FACE('',(#21415),#17550,.F.);
#76846=ADVANCED_FACE('',(#21416),#17551,.F.);
#76847=ADVANCED_FACE('',(#21417),#17552,.F.);
#76848=ADVANCED_FACE('',(#21418),#17553,.F.);
#76849=ADVANCED_FACE('',(#21419),#17554,.F.);
#76850=ADVANCED_FACE('',(#21420),#17555,.F.);
#76851=ADVANCED_FACE('',(#21421),#17556,.F.);
#76852=ADVANCED_FACE('',(#21422),#17557,.F.);
#76853=ADVANCED_FACE('',(#21423),#17558,.F.);
#76854=ADVANCED_FACE('',(#21424),#17559,.F.);
#76855=ADVANCED_FACE('',(#21425),#17560,.F.);
#76856=ADVANCED_FACE('',(#21426),#17561,.F.);
#76857=ADVANCED_FACE('',(#21427),#17562,.T.);
#76858=ADVANCED_FACE('',(#21428),#17563,.F.);
#76859=ADVANCED_FACE('',(#21429),#17564,.F.);
#76860=ADVANCED_FACE('',(#21430),#17565,.F.);
#76861=ADVANCED_FACE('',(#21431),#17566,.F.);
#76862=ADVANCED_FACE('',(#21432),#17567,.T.);
#76863=ADVANCED_FACE('',(#21433),#17568,.F.);
#76864=ADVANCED_FACE('',(#21434),#17569,.F.);
#76865=ADVANCED_FACE('',(#21435),#17570,.F.);
#76866=ADVANCED_FACE('',(#21436),#17571,.F.);
#76867=ADVANCED_FACE('',(#21437),#17572,.T.);
#76868=ADVANCED_FACE('',(#21438),#17573,.F.);
#76869=ADVANCED_FACE('',(#21439),#17574,.F.);
#76870=ADVANCED_FACE('',(#21440),#17575,.F.);
#76871=ADVANCED_FACE('',(#21441),#17576,.F.);
#76872=ADVANCED_FACE('',(#21442),#17577,.T.);
#76873=ADVANCED_FACE('',(#21443),#17578,.F.);
#76874=ADVANCED_FACE('',(#21444),#17579,.F.);
#76875=ADVANCED_FACE('',(#21445),#17580,.F.);
#76876=ADVANCED_FACE('',(#21446),#17581,.F.);
#76877=ADVANCED_FACE('',(#21447),#17582,.T.);
#76878=ADVANCED_FACE('',(#21448),#17583,.F.);
#76879=ADVANCED_FACE('',(#21449),#17584,.F.);
#76880=ADVANCED_FACE('',(#21450),#17585,.F.);
#76881=ADVANCED_FACE('',(#21451),#17586,.F.);
#76882=ADVANCED_FACE('',(#21452),#17587,.T.);
#76883=ADVANCED_FACE('',(#21453),#17588,.F.);
#76884=ADVANCED_FACE('',(#21454),#17589,.F.);
#76885=ADVANCED_FACE('',(#21455),#17590,.F.);
#76886=ADVANCED_FACE('',(#21456),#17591,.F.);
#76887=ADVANCED_FACE('',(#21457),#17592,.T.);
#76888=ADVANCED_FACE('',(#21458),#17593,.F.);
#76889=ADVANCED_FACE('',(#21459),#17594,.F.);
#76890=ADVANCED_FACE('',(#21460),#17595,.F.);
#76891=ADVANCED_FACE('',(#21461),#17596,.F.);
#76892=ADVANCED_FACE('',(#21462),#17597,.T.);
#76893=ADVANCED_FACE('',(#21463),#17598,.F.);
#76894=ADVANCED_FACE('',(#21464),#17599,.F.);
#76895=ADVANCED_FACE('',(#21465),#17600,.F.);
#76896=ADVANCED_FACE('',(#21466),#17601,.F.);
#76897=ADVANCED_FACE('',(#21467),#17602,.T.);
#76898=ADVANCED_FACE('',(#21468),#17603,.F.);
#76899=ADVANCED_FACE('',(#21469),#17604,.F.);
#76900=ADVANCED_FACE('',(#21470),#17605,.F.);
#76901=ADVANCED_FACE('',(#21471),#17606,.F.);
#76902=ADVANCED_FACE('',(#21472),#17607,.T.);
#76903=ADVANCED_FACE('',(#21473),#17608,.F.);
#76904=ADVANCED_FACE('',(#21474),#17609,.F.);
#76905=ADVANCED_FACE('',(#21475),#17610,.F.);
#76906=ADVANCED_FACE('',(#21476),#17611,.F.);
#76907=ADVANCED_FACE('',(#21477),#17612,.F.);
#76908=ADVANCED_FACE('',(#21478),#17613,.F.);
#76909=ADVANCED_FACE('',(#21479),#17614,.F.);
#76910=ADVANCED_FACE('',(#21480),#17615,.F.);
#76911=ADVANCED_FACE('',(#21481),#17616,.F.);
#76912=ADVANCED_FACE('',(#21482),#17617,.F.);
#76913=ADVANCED_FACE('',(#21483),#17618,.F.);
#76914=ADVANCED_FACE('',(#21484),#17619,.F.);
#76915=ADVANCED_FACE('',(#21485),#17620,.F.);
#76916=ADVANCED_FACE('',(#21486),#17621,.F.);
#76917=ADVANCED_FACE('',(#21487),#17622,.F.);
#76918=ADVANCED_FACE('',(#21488),#17623,.F.);
#76919=ADVANCED_FACE('',(#21489),#17624,.F.);
#76920=ADVANCED_FACE('',(#21490),#17625,.F.);
#76921=ADVANCED_FACE('',(#21491),#17626,.F.);
#76922=ADVANCED_FACE('',(#21492),#17627,.F.);
#76923=ADVANCED_FACE('',(#21493),#17628,.F.);
#76924=ADVANCED_FACE('',(#21494),#17629,.F.);
#76925=ADVANCED_FACE('',(#21495),#17630,.F.);
#76926=ADVANCED_FACE('',(#21496),#17631,.F.);
#76927=ADVANCED_FACE('',(#21497),#17632,.F.);
#76928=ADVANCED_FACE('',(#21498),#17633,.F.);
#76929=ADVANCED_FACE('',(#21499),#17634,.F.);
#76930=ADVANCED_FACE('',(#21500),#17635,.F.);
#76931=ADVANCED_FACE('',(#21501),#17636,.F.);
#76932=ADVANCED_FACE('',(#21502),#17637,.F.);
#76933=ADVANCED_FACE('',(#21503),#17638,.F.);
#76934=ADVANCED_FACE('',(#21504),#17639,.F.);
#76935=ADVANCED_FACE('',(#21505),#17640,.F.);
#76936=ADVANCED_FACE('',(#21506),#17641,.F.);
#76937=ADVANCED_FACE('',(#21507),#17642,.F.);
#76938=ADVANCED_FACE('',(#21508),#17643,.F.);
#76939=ADVANCED_FACE('',(#21509),#17644,.T.);
#76940=ADVANCED_FACE('',(#21510),#17645,.F.);
#76941=ADVANCED_FACE('',(#21511),#17646,.F.);
#76942=ADVANCED_FACE('',(#21512),#17647,.F.);
#76943=ADVANCED_FACE('',(#21513),#17648,.F.);
#76944=ADVANCED_FACE('',(#21514),#17649,.T.);
#76945=ADVANCED_FACE('',(#21515),#17650,.F.);
#76946=ADVANCED_FACE('',(#21516),#17651,.F.);
#76947=ADVANCED_FACE('',(#21517),#17652,.F.);
#76948=ADVANCED_FACE('',(#21518),#17653,.F.);
#76949=ADVANCED_FACE('',(#21519),#17654,.F.);
#76950=ADVANCED_FACE('',(#21520),#17655,.F.);
#76951=ADVANCED_FACE('',(#21521),#17656,.F.);
#76952=ADVANCED_FACE('',(#21522),#17657,.F.);
#76953=ADVANCED_FACE('',(#21523),#17658,.F.);
#76954=ADVANCED_FACE('',(#21524),#17659,.F.);
#76955=ADVANCED_FACE('',(#21525),#17660,.F.);
#76956=ADVANCED_FACE('',(#21526),#17661,.F.);
#76957=ADVANCED_FACE('',(#21527),#17662,.F.);
#76958=ADVANCED_FACE('',(#21528),#17663,.F.);
#76959=ADVANCED_FACE('',(#21529),#17664,.F.);
#76960=ADVANCED_FACE('',(#21530),#17665,.F.);
#76961=ADVANCED_FACE('',(#21531),#17666,.F.);
#76962=ADVANCED_FACE('',(#21532),#17667,.F.);
#76963=ADVANCED_FACE('',(#21533),#17668,.F.);
#76964=ADVANCED_FACE('',(#21534),#17669,.F.);
#76965=ADVANCED_FACE('',(#21535),#17670,.T.);
#76966=ADVANCED_FACE('',(#21536),#17671,.F.);
#76967=ADVANCED_FACE('',(#21537),#17672,.F.);
#76968=ADVANCED_FACE('',(#21538),#17673,.F.);
#76969=ADVANCED_FACE('',(#21539),#17674,.F.);
#76970=ADVANCED_FACE('',(#21540),#17675,.T.);
#76971=ADVANCED_FACE('',(#21541),#17676,.F.);
#76972=ADVANCED_FACE('',(#21542),#17677,.F.);
#76973=ADVANCED_FACE('',(#21543),#17678,.F.);
#76974=ADVANCED_FACE('',(#21544),#17679,.F.);
#76975=ADVANCED_FACE('',(#21545),#17680,.T.);
#76976=ADVANCED_FACE('',(#21546),#17681,.F.);
#76977=ADVANCED_FACE('',(#21547),#17682,.F.);
#76978=ADVANCED_FACE('',(#21548),#17683,.F.);
#76979=ADVANCED_FACE('',(#21549),#17684,.F.);
#76980=ADVANCED_FACE('',(#21550),#17685,.T.);
#76981=ADVANCED_FACE('',(#21551),#17686,.F.);
#76982=ADVANCED_FACE('',(#21552),#17687,.F.);
#76983=ADVANCED_FACE('',(#21553),#17688,.F.);
#76984=ADVANCED_FACE('',(#21554),#17689,.F.);
#76985=ADVANCED_FACE('',(#21555),#17690,.F.);
#76986=ADVANCED_FACE('',(#21556),#17691,.F.);
#76987=ADVANCED_FACE('',(#21557),#17692,.F.);
#76988=ADVANCED_FACE('',(#21558),#17693,.F.);
#76989=ADVANCED_FACE('',(#21559),#17694,.F.);
#76990=ADVANCED_FACE('',(#21560),#17695,.F.);
#76991=ADVANCED_FACE('',(#21561),#17696,.F.);
#76992=ADVANCED_FACE('',(#21562),#17697,.F.);
#76993=ADVANCED_FACE('',(#21563),#17698,.F.);
#76994=ADVANCED_FACE('',(#21564),#17699,.F.);
#76995=ADVANCED_FACE('',(#21565),#17700,.F.);
#76996=ADVANCED_FACE('',(#21566),#17701,.F.);
#76997=ADVANCED_FACE('',(#21567),#17702,.F.);
#76998=ADVANCED_FACE('',(#21568),#17703,.F.);
#76999=ADVANCED_FACE('',(#21569),#17704,.F.);
#77000=ADVANCED_FACE('',(#21570),#17705,.F.);
#77001=ADVANCED_FACE('',(#21571),#17706,.F.);
#77002=ADVANCED_FACE('',(#21572),#17707,.F.);
#77003=ADVANCED_FACE('',(#21573),#17708,.F.);
#77004=ADVANCED_FACE('',(#21574),#17709,.F.);
#77005=ADVANCED_FACE('',(#21575),#17710,.F.);
#77006=ADVANCED_FACE('',(#21576),#17711,.F.);
#77007=ADVANCED_FACE('',(#21577),#17712,.F.);
#77008=ADVANCED_FACE('',(#21578),#17713,.F.);
#77009=ADVANCED_FACE('',(#21579),#17714,.F.);
#77010=ADVANCED_FACE('',(#21580),#17715,.F.);
#77011=ADVANCED_FACE('',(#21581),#17716,.F.);
#77012=ADVANCED_FACE('',(#21582),#17717,.F.);
#77013=ADVANCED_FACE('',(#21583),#17718,.F.);
#77014=ADVANCED_FACE('',(#21584),#17719,.F.);
#77015=ADVANCED_FACE('',(#21585),#17720,.F.);
#77016=ADVANCED_FACE('',(#21586),#17721,.F.);
#77017=ADVANCED_FACE('',(#21587),#17722,.F.);
#77018=ADVANCED_FACE('',(#21588),#17723,.F.);
#77019=ADVANCED_FACE('',(#21589),#17724,.F.);
#77020=ADVANCED_FACE('',(#21590),#17725,.F.);
#77021=ADVANCED_FACE('',(#21591),#17726,.F.);
#77022=ADVANCED_FACE('',(#21592),#17727,.F.);
#77023=ADVANCED_FACE('',(#21593),#17728,.F.);
#77024=ADVANCED_FACE('',(#21594),#17729,.F.);
#77025=ADVANCED_FACE('',(#21595),#17730,.T.);
#77026=ADVANCED_FACE('',(#21596),#17731,.F.);
#77027=ADVANCED_FACE('',(#21597),#17732,.F.);
#77028=ADVANCED_FACE('',(#21598),#17733,.F.);
#77029=ADVANCED_FACE('',(#21599),#17734,.F.);
#77030=ADVANCED_FACE('',(#21600),#17735,.T.);
#77031=ADVANCED_FACE('',(#21601),#17736,.F.);
#77032=ADVANCED_FACE('',(#21602),#17737,.F.);
#77033=ADVANCED_FACE('',(#21603),#17738,.F.);
#77034=ADVANCED_FACE('',(#21604),#17739,.F.);
#77035=ADVANCED_FACE('',(#21605),#17740,.F.);
#77036=ADVANCED_FACE('',(#21606),#17741,.F.);
#77037=ADVANCED_FACE('',(#21607),#17742,.F.);
#77038=ADVANCED_FACE('',(#21608),#17743,.F.);
#77039=ADVANCED_FACE('',(#21609),#17744,.F.);
#77040=ADVANCED_FACE('',(#21610),#17745,.F.);
#77041=ADVANCED_FACE('',(#21611),#17746,.F.);
#77042=ADVANCED_FACE('',(#21612),#17747,.F.);
#77043=ADVANCED_FACE('',(#21613),#17748,.F.);
#77044=ADVANCED_FACE('',(#21614),#17749,.F.);
#77045=ADVANCED_FACE('',(#21615),#17750,.F.);
#77046=ADVANCED_FACE('',(#21616),#17751,.F.);
#77047=ADVANCED_FACE('',(#21617),#17752,.F.);
#77048=ADVANCED_FACE('',(#21618),#17753,.F.);
#77049=ADVANCED_FACE('',(#21619),#17754,.F.);
#77050=ADVANCED_FACE('',(#21620),#17755,.F.);
#77051=ADVANCED_FACE('',(#21621),#17756,.F.);
#77052=ADVANCED_FACE('',(#21622),#17757,.F.);
#77053=ADVANCED_FACE('',(#21623),#17758,.F.);
#77054=ADVANCED_FACE('',(#21624),#17759,.F.);
#77055=ADVANCED_FACE('',(#21625),#17760,.F.);
#77056=ADVANCED_FACE('',(#21626),#17761,.F.);
#77057=ADVANCED_FACE('',(#21627),#17762,.F.);
#77058=ADVANCED_FACE('',(#21628),#17763,.F.);
#77059=ADVANCED_FACE('',(#21629),#17764,.F.);
#77060=ADVANCED_FACE('',(#21630),#17765,.F.);
#77061=ADVANCED_FACE('',(#21631),#17766,.F.);
#77062=ADVANCED_FACE('',(#21632),#17767,.F.);
#77063=ADVANCED_FACE('',(#21633),#17768,.F.);
#77064=ADVANCED_FACE('',(#21634),#17769,.F.);
#77065=ADVANCED_FACE('',(#21635),#17770,.F.);
#77066=ADVANCED_FACE('',(#21636),#17771,.F.);
#77067=ADVANCED_FACE('',(#21637),#17772,.F.);
#77068=ADVANCED_FACE('',(#21638),#17773,.F.);
#77069=ADVANCED_FACE('',(#21639),#17774,.F.);
#77070=ADVANCED_FACE('',(#21640),#17775,.F.);
#77071=ADVANCED_FACE('',(#21641),#17776,.T.);
#77072=ADVANCED_FACE('',(#21642),#17777,.F.);
#77073=ADVANCED_FACE('',(#21643),#17778,.F.);
#77074=ADVANCED_FACE('',(#21644),#17779,.F.);
#77075=ADVANCED_FACE('',(#21645),#17780,.F.);
#77076=ADVANCED_FACE('',(#21646),#17781,.T.);
#77077=ADVANCED_FACE('',(#21647),#17782,.F.);
#77078=ADVANCED_FACE('',(#21648),#17783,.F.);
#77079=ADVANCED_FACE('',(#21649),#17784,.F.);
#77080=ADVANCED_FACE('',(#21650),#17785,.F.);
#77081=ADVANCED_FACE('',(#21651),#17786,.F.);
#77082=ADVANCED_FACE('',(#21652),#17787,.F.);
#77083=ADVANCED_FACE('',(#21653),#17788,.F.);
#77084=ADVANCED_FACE('',(#21654),#17789,.F.);
#77085=ADVANCED_FACE('',(#21655),#17790,.F.);
#77086=ADVANCED_FACE('',(#21656),#17791,.F.);
#77087=ADVANCED_FACE('',(#21657),#17792,.F.);
#77088=ADVANCED_FACE('',(#21658),#17793,.F.);
#77089=ADVANCED_FACE('',(#21659),#17794,.F.);
#77090=ADVANCED_FACE('',(#21660),#17795,.F.);
#77091=ADVANCED_FACE('',(#21661),#17796,.F.);
#77092=ADVANCED_FACE('',(#21662),#17797,.F.);
#77093=ADVANCED_FACE('',(#21663),#17798,.F.);
#77094=ADVANCED_FACE('',(#21664),#17799,.F.);
#77095=ADVANCED_FACE('',(#21665),#17800,.F.);
#77096=ADVANCED_FACE('',(#21666),#17801,.F.);
#77097=ADVANCED_FACE('',(#21667),#17802,.F.);
#77098=ADVANCED_FACE('',(#21668),#17803,.F.);
#77099=ADVANCED_FACE('',(#21669),#17804,.F.);
#77100=ADVANCED_FACE('',(#21670),#17805,.F.);
#77101=ADVANCED_FACE('',(#21671),#17806,.F.);
#77102=ADVANCED_FACE('',(#21672),#17807,.F.);
#77103=ADVANCED_FACE('',(#21673),#17808,.F.);
#77104=ADVANCED_FACE('',(#21674),#17809,.F.);
#77105=ADVANCED_FACE('',(#21675),#17810,.F.);
#77106=ADVANCED_FACE('',(#21676),#17811,.F.);
#77107=ADVANCED_FACE('',(#21677),#17812,.F.);
#77108=ADVANCED_FACE('',(#21678),#17813,.F.);
#77109=ADVANCED_FACE('',(#21679),#17814,.F.);
#77110=ADVANCED_FACE('',(#21680),#17815,.F.);
#77111=ADVANCED_FACE('',(#21681),#17816,.F.);
#77112=ADVANCED_FACE('',(#21682),#17817,.F.);
#77113=ADVANCED_FACE('',(#21683),#17818,.F.);
#77114=ADVANCED_FACE('',(#21684),#17819,.F.);
#77115=ADVANCED_FACE('',(#21685),#17820,.F.);
#77116=ADVANCED_FACE('',(#21686),#17821,.F.);
#77117=ADVANCED_FACE('',(#21687),#17822,.F.);
#77118=ADVANCED_FACE('',(#21688),#17823,.F.);
#77119=ADVANCED_FACE('',(#21689),#17824,.F.);
#77120=ADVANCED_FACE('',(#21690),#17825,.F.);
#77121=ADVANCED_FACE('',(#21691),#17826,.F.);
#77122=ADVANCED_FACE('',(#21692),#17827,.F.);
#77123=ADVANCED_FACE('',(#21693),#17828,.F.);
#77124=ADVANCED_FACE('',(#21694),#17829,.F.);
#77125=ADVANCED_FACE('',(#21695),#17830,.F.);
#77126=ADVANCED_FACE('',(#21696),#17831,.F.);
#77127=ADVANCED_FACE('',(#21697),#17832,.F.);
#77128=ADVANCED_FACE('',(#21698),#17833,.F.);
#77129=ADVANCED_FACE('',(#21699),#17834,.F.);
#77130=ADVANCED_FACE('',(#21700),#17835,.F.);
#77131=ADVANCED_FACE('',(#21701),#17836,.F.);
#77132=ADVANCED_FACE('',(#21702),#17837,.F.);
#77133=ADVANCED_FACE('',(#21703),#17838,.F.);
#77134=ADVANCED_FACE('',(#21704),#17839,.F.);
#77135=ADVANCED_FACE('',(#21705),#17840,.F.);
#77136=ADVANCED_FACE('',(#21706),#17841,.F.);
#77137=ADVANCED_FACE('',(#21707),#17842,.F.);
#77138=ADVANCED_FACE('',(#21708),#17843,.F.);
#77139=ADVANCED_FACE('',(#21709),#17844,.F.);
#77140=ADVANCED_FACE('',(#21710),#17845,.F.);
#77141=ADVANCED_FACE('',(#21711),#17846,.F.);
#77142=ADVANCED_FACE('',(#21712),#17847,.F.);
#77143=ADVANCED_FACE('',(#21713),#17848,.F.);
#77144=ADVANCED_FACE('',(#21714),#17849,.F.);
#77145=ADVANCED_FACE('',(#21715),#17850,.F.);
#77146=ADVANCED_FACE('',(#21716),#17851,.F.);
#77147=ADVANCED_FACE('',(#21717),#17852,.F.);
#77148=ADVANCED_FACE('',(#21718),#17853,.F.);
#77149=ADVANCED_FACE('',(#21719),#17854,.F.);
#77150=ADVANCED_FACE('',(#21720),#17855,.F.);
#77151=ADVANCED_FACE('',(#21721),#17856,.F.);
#77152=ADVANCED_FACE('',(#21722),#17857,.F.);
#77153=ADVANCED_FACE('',(#21723),#17858,.F.);
#77154=ADVANCED_FACE('',(#21724),#17859,.F.);
#77155=ADVANCED_FACE('',(#21725),#17860,.F.);
#77156=ADVANCED_FACE('',(#21726),#17861,.F.);
#77157=ADVANCED_FACE('',(#21727),#17862,.F.);
#77158=ADVANCED_FACE('',(#21728),#17863,.F.);
#77159=ADVANCED_FACE('',(#21729),#17864,.F.);
#77160=ADVANCED_FACE('',(#21730),#17865,.F.);
#77161=ADVANCED_FACE('',(#21731),#17866,.F.);
#77162=ADVANCED_FACE('',(#21732),#17867,.F.);
#77163=ADVANCED_FACE('',(#21733),#17868,.F.);
#77164=ADVANCED_FACE('',(#21734),#17869,.F.);
#77165=ADVANCED_FACE('',(#21735),#17870,.F.);
#77166=ADVANCED_FACE('',(#21736),#17871,.F.);
#77167=ADVANCED_FACE('',(#21737),#17872,.F.);
#77168=ADVANCED_FACE('',(#21738),#17873,.F.);
#77169=ADVANCED_FACE('',(#21739),#17874,.F.);
#77170=ADVANCED_FACE('',(#21740),#17875,.F.);
#77171=ADVANCED_FACE('',(#21741),#17876,.F.);
#77172=ADVANCED_FACE('',(#21742),#17877,.F.);
#77173=ADVANCED_FACE('',(#21743),#17878,.F.);
#77174=ADVANCED_FACE('',(#21744),#17879,.F.);
#77175=ADVANCED_FACE('',(#21745),#17880,.F.);
#77176=ADVANCED_FACE('',(#21746),#17881,.F.);
#77177=ADVANCED_FACE('',(#21747),#17882,.F.);
#77178=ADVANCED_FACE('',(#21748),#17883,.F.);
#77179=ADVANCED_FACE('',(#21749),#17884,.F.);
#77180=ADVANCED_FACE('',(#21750),#17885,.F.);
#77181=ADVANCED_FACE('',(#21751),#17886,.F.);
#77182=ADVANCED_FACE('',(#21752),#17887,.F.);
#77183=ADVANCED_FACE('',(#21753),#17888,.F.);
#77184=ADVANCED_FACE('',(#21754),#17889,.F.);
#77185=ADVANCED_FACE('',(#21755),#17890,.F.);
#77186=ADVANCED_FACE('',(#21756),#17891,.F.);
#77187=ADVANCED_FACE('',(#21757),#17892,.F.);
#77188=ADVANCED_FACE('',(#21758),#17893,.F.);
#77189=ADVANCED_FACE('',(#21759),#17894,.F.);
#77190=ADVANCED_FACE('',(#21760),#17895,.F.);
#77191=ADVANCED_FACE('',(#21761),#17896,.F.);
#77192=ADVANCED_FACE('',(#21762),#17897,.F.);
#77193=ADVANCED_FACE('',(#21763),#17898,.F.);
#77194=ADVANCED_FACE('',(#21764),#17899,.F.);
#77195=ADVANCED_FACE('',(#21765),#17900,.F.);
#77196=ADVANCED_FACE('',(#21766),#17901,.F.);
#77197=ADVANCED_FACE('',(#21767),#17902,.F.);
#77198=ADVANCED_FACE('',(#21768),#17903,.F.);
#77199=ADVANCED_FACE('',(#21769),#17904,.F.);
#77200=ADVANCED_FACE('',(#21770),#17905,.F.);
#77201=ADVANCED_FACE('',(#21771),#17906,.F.);
#77202=ADVANCED_FACE('',(#21772),#17907,.F.);
#77203=ADVANCED_FACE('',(#21773),#17908,.F.);
#77204=ADVANCED_FACE('',(#21774),#17909,.F.);
#77205=ADVANCED_FACE('',(#21775),#17910,.F.);
#77206=ADVANCED_FACE('',(#21776),#17911,.F.);
#77207=ADVANCED_FACE('',(#21777),#17912,.F.);
#77208=ADVANCED_FACE('',(#21778),#17913,.F.);
#77209=ADVANCED_FACE('',(#21779),#17914,.F.);
#77210=ADVANCED_FACE('',(#21780),#17915,.F.);
#77211=ADVANCED_FACE('',(#21781),#17916,.F.);
#77212=ADVANCED_FACE('',(#21782),#17917,.F.);
#77213=ADVANCED_FACE('',(#21783),#17918,.F.);
#77214=ADVANCED_FACE('',(#21784),#17919,.F.);
#77215=ADVANCED_FACE('',(#21785),#17920,.F.);
#77216=ADVANCED_FACE('',(#21786),#17921,.F.);
#77217=ADVANCED_FACE('',(#21787),#17922,.F.);
#77218=ADVANCED_FACE('',(#21788),#17923,.F.);
#77219=ADVANCED_FACE('',(#21789),#17924,.F.);
#77220=ADVANCED_FACE('',(#21790),#17925,.F.);
#77221=ADVANCED_FACE('',(#21791),#17926,.F.);
#77222=ADVANCED_FACE('',(#21792),#17927,.F.);
#77223=ADVANCED_FACE('',(#21793),#17928,.F.);
#77224=ADVANCED_FACE('',(#21794),#17929,.F.);
#77225=ADVANCED_FACE('',(#21795),#17930,.F.);
#77226=ADVANCED_FACE('',(#21796),#17931,.F.);
#77227=ADVANCED_FACE('',(#21797),#17932,.F.);
#77228=ADVANCED_FACE('',(#21798),#17933,.F.);
#77229=ADVANCED_FACE('',(#21799),#17934,.F.);
#77230=ADVANCED_FACE('',(#21800),#17935,.F.);
#77231=ADVANCED_FACE('',(#21801),#17936,.F.);
#77232=ADVANCED_FACE('',(#21802),#17937,.F.);
#77233=ADVANCED_FACE('',(#21803),#17938,.F.);
#77234=ADVANCED_FACE('',(#21804),#17939,.F.);
#77235=ADVANCED_FACE('',(#21805),#17940,.F.);
#77236=ADVANCED_FACE('',(#21806),#17941,.F.);
#77237=ADVANCED_FACE('',(#21807),#17942,.F.);
#77238=ADVANCED_FACE('',(#21808),#17943,.F.);
#77239=ADVANCED_FACE('',(#21809),#17944,.F.);
#77240=ADVANCED_FACE('',(#21810),#17945,.F.);
#77241=ADVANCED_FACE('',(#21811),#17946,.F.);
#77242=ADVANCED_FACE('',(#21812),#17947,.F.);
#77243=ADVANCED_FACE('',(#21813),#17948,.F.);
#77244=ADVANCED_FACE('',(#21814),#17949,.F.);
#77245=ADVANCED_FACE('',(#21815),#17950,.F.);
#77246=ADVANCED_FACE('',(#21816),#17951,.F.);
#77247=ADVANCED_FACE('',(#21817),#17952,.F.);
#77248=ADVANCED_FACE('',(#21818),#17953,.F.);
#77249=ADVANCED_FACE('',(#21819),#17954,.F.);
#77250=ADVANCED_FACE('',(#21820),#17955,.F.);
#77251=ADVANCED_FACE('',(#21821),#17956,.F.);
#77252=ADVANCED_FACE('',(#21822),#17957,.F.);
#77253=ADVANCED_FACE('',(#21823),#17958,.F.);
#77254=ADVANCED_FACE('',(#21824),#17959,.F.);
#77255=ADVANCED_FACE('',(#21825),#17960,.F.);
#77256=ADVANCED_FACE('',(#21826),#17961,.F.);
#77257=ADVANCED_FACE('',(#21827),#17962,.F.);
#77258=ADVANCED_FACE('',(#21828),#17963,.F.);
#77259=ADVANCED_FACE('',(#21829),#17964,.F.);
#77260=ADVANCED_FACE('',(#21830),#17965,.F.);
#77261=ADVANCED_FACE('',(#21831),#17966,.F.);
#77262=ADVANCED_FACE('',(#21832),#17967,.F.);
#77263=ADVANCED_FACE('',(#21833),#17968,.F.);
#77264=ADVANCED_FACE('',(#21834),#17969,.F.);
#77265=ADVANCED_FACE('',(#21835),#17970,.F.);
#77266=ADVANCED_FACE('',(#21836),#17971,.F.);
#77267=ADVANCED_FACE('',(#21837),#17972,.F.);
#77268=ADVANCED_FACE('',(#21838),#17973,.F.);
#77269=ADVANCED_FACE('',(#21839),#17974,.F.);
#77270=ADVANCED_FACE('',(#21840),#17975,.F.);
#77271=ADVANCED_FACE('',(#21841),#17976,.F.);
#77272=ADVANCED_FACE('',(#21842),#17977,.F.);
#77273=ADVANCED_FACE('',(#21843),#17978,.F.);
#77274=ADVANCED_FACE('',(#21844),#17979,.F.);
#77275=ADVANCED_FACE('',(#21845),#17980,.F.);
#77276=ADVANCED_FACE('',(#21846),#17981,.F.);
#77277=ADVANCED_FACE('',(#21847),#17982,.F.);
#77278=ADVANCED_FACE('',(#21848),#17983,.F.);
#77279=ADVANCED_FACE('',(#21849),#17984,.F.);
#77280=ADVANCED_FACE('',(#21850),#17985,.F.);
#77281=ADVANCED_FACE('',(#21851),#17986,.F.);
#77282=ADVANCED_FACE('',(#21852),#17987,.F.);
#77283=ADVANCED_FACE('',(#21853),#17988,.F.);
#77284=ADVANCED_FACE('',(#21854),#17989,.F.);
#77285=ADVANCED_FACE('',(#21855),#17990,.F.);
#77286=ADVANCED_FACE('',(#21856),#17991,.F.);
#77287=ADVANCED_FACE('',(#21857),#17992,.F.);
#77288=ADVANCED_FACE('',(#21858),#17993,.F.);
#77289=ADVANCED_FACE('',(#21859),#17994,.F.);
#77290=ADVANCED_FACE('',(#21860),#17995,.F.);
#77291=ADVANCED_FACE('',(#21861),#17996,.F.);
#77292=ADVANCED_FACE('',(#21862),#17997,.F.);
#77293=ADVANCED_FACE('',(#21863),#17998,.F.);
#77294=ADVANCED_FACE('',(#21864),#17999,.F.);
#77295=ADVANCED_FACE('',(#21865),#18000,.F.);
#77296=ADVANCED_FACE('',(#21866),#18001,.F.);
#77297=ADVANCED_FACE('',(#21867),#18002,.F.);
#77298=ADVANCED_FACE('',(#21868),#18003,.F.);
#77299=ADVANCED_FACE('',(#21869),#18004,.F.);
#77300=ADVANCED_FACE('',(#21870),#18005,.F.);
#77301=ADVANCED_FACE('',(#21871),#18006,.F.);
#77302=ADVANCED_FACE('',(#21872),#18007,.F.);
#77303=ADVANCED_FACE('',(#21873),#18008,.F.);
#77304=ADVANCED_FACE('',(#21874),#18009,.F.);
#77305=ADVANCED_FACE('',(#21875),#18010,.F.);
#77306=ADVANCED_FACE('',(#21876),#18011,.F.);
#77307=ADVANCED_FACE('',(#21877),#18012,.F.);
#77308=ADVANCED_FACE('',(#21878),#18013,.F.);
#77309=ADVANCED_FACE('',(#21879),#18014,.F.);
#77310=ADVANCED_FACE('',(#21880),#18015,.F.);
#77311=ADVANCED_FACE('',(#21881),#18016,.F.);
#77312=ADVANCED_FACE('',(#21882),#18017,.F.);
#77313=ADVANCED_FACE('',(#21883),#18018,.F.);
#77314=ADVANCED_FACE('',(#21884),#18019,.F.);
#77315=ADVANCED_FACE('',(#21885),#18020,.F.);
#77316=ADVANCED_FACE('',(#21886),#18021,.F.);
#77317=ADVANCED_FACE('',(#21887),#18022,.F.);
#77318=ADVANCED_FACE('',(#21888),#18023,.F.);
#77319=ADVANCED_FACE('',(#21889),#18024,.F.);
#77320=ADVANCED_FACE('',(#21890),#18025,.F.);
#77321=ADVANCED_FACE('',(#21891),#18026,.F.);
#77322=ADVANCED_FACE('',(#21892),#18027,.F.);
#77323=ADVANCED_FACE('',(#21893),#18028,.F.);
#77324=ADVANCED_FACE('',(#21894),#18029,.F.);
#77325=ADVANCED_FACE('',(#21895),#18030,.F.);
#77326=ADVANCED_FACE('',(#21896),#18031,.F.);
#77327=ADVANCED_FACE('',(#21897),#18032,.F.);
#77328=ADVANCED_FACE('',(#21898),#18033,.F.);
#77329=ADVANCED_FACE('',(#21899),#18034,.F.);
#77330=ADVANCED_FACE('',(#21900),#18035,.F.);
#77331=ADVANCED_FACE('',(#21901),#18036,.F.);
#77332=ADVANCED_FACE('',(#21902),#18037,.F.);
#77333=ADVANCED_FACE('',(#21903),#18038,.F.);
#77334=ADVANCED_FACE('',(#21904),#18039,.F.);
#77335=ADVANCED_FACE('',(#21905),#18040,.F.);
#77336=ADVANCED_FACE('',(#21906),#18041,.F.);
#77337=ADVANCED_FACE('',(#21907),#18042,.F.);
#77338=ADVANCED_FACE('',(#21908),#18043,.F.);
#77339=ADVANCED_FACE('',(#21909),#18044,.F.);
#77340=ADVANCED_FACE('',(#21910),#18045,.F.);
#77341=ADVANCED_FACE('',(#21911),#18046,.F.);
#77342=ADVANCED_FACE('',(#21912),#18047,.F.);
#77343=ADVANCED_FACE('',(#21913),#18048,.F.);
#77344=ADVANCED_FACE('',(#21914),#18049,.F.);
#77345=ADVANCED_FACE('',(#21915),#18050,.F.);
#77346=ADVANCED_FACE('',(#21916),#18051,.F.);
#77347=ADVANCED_FACE('',(#21917),#18052,.F.);
#77348=ADVANCED_FACE('',(#21918),#18053,.F.);
#77349=ADVANCED_FACE('',(#21919),#18054,.F.);
#77350=ADVANCED_FACE('',(#21920),#18055,.F.);
#77351=ADVANCED_FACE('',(#21921),#18056,.F.);
#77352=ADVANCED_FACE('',(#21922),#18057,.F.);
#77353=ADVANCED_FACE('',(#21923),#18058,.F.);
#77354=ADVANCED_FACE('',(#21924),#18059,.F.);
#77355=ADVANCED_FACE('',(#21925),#18060,.F.);
#77356=ADVANCED_FACE('',(#21926),#18061,.F.);
#77357=ADVANCED_FACE('',(#21927),#18062,.F.);
#77358=ADVANCED_FACE('',(#21928),#18063,.F.);
#77359=ADVANCED_FACE('',(#21929),#18064,.F.);
#77360=ADVANCED_FACE('',(#21930),#18065,.F.);
#77361=ADVANCED_FACE('',(#21931),#18066,.F.);
#77362=ADVANCED_FACE('',(#21932),#18067,.F.);
#77363=ADVANCED_FACE('',(#21933),#18068,.F.);
#77364=ADVANCED_FACE('',(#21934),#18069,.F.);
#77365=ADVANCED_FACE('',(#21935),#18070,.F.);
#77366=ADVANCED_FACE('',(#21936),#18071,.F.);
#77367=ADVANCED_FACE('',(#21937),#18072,.F.);
#77368=ADVANCED_FACE('',(#21938),#18073,.F.);
#77369=ADVANCED_FACE('',(#21939),#18074,.F.);
#77370=ADVANCED_FACE('',(#21940),#18075,.F.);
#77371=ADVANCED_FACE('',(#21941),#18076,.F.);
#77372=ADVANCED_FACE('',(#21942),#18077,.F.);
#77373=ADVANCED_FACE('',(#21943),#18078,.F.);
#77374=ADVANCED_FACE('',(#21944),#18079,.F.);
#77375=ADVANCED_FACE('',(#21945),#18080,.F.);
#77376=ADVANCED_FACE('',(#21946),#18081,.F.);
#77377=ADVANCED_FACE('',(#21947),#18082,.F.);
#77378=ADVANCED_FACE('',(#21948),#18083,.F.);
#77379=ADVANCED_FACE('',(#21949),#18084,.F.);
#77380=ADVANCED_FACE('',(#21950),#18085,.F.);
#77381=ADVANCED_FACE('',(#21951),#18086,.F.);
#77382=ADVANCED_FACE('',(#21952),#18087,.F.);
#77383=ADVANCED_FACE('',(#21953),#18088,.F.);
#77384=ADVANCED_FACE('',(#21954),#18089,.F.);
#77385=ADVANCED_FACE('',(#21955,#330),#18090,.T.);
#77386=ADVANCED_FACE('',(#21956),#18091,.F.);
#77387=ADVANCED_FACE('',(#21957),#18092,.F.);
#77388=ADVANCED_FACE('',(#21958),#18093,.F.);
#77389=ADVANCED_FACE('',(#21959),#18094,.F.);
#77390=ADVANCED_FACE('',(#21960),#18095,.F.);
#77391=ADVANCED_FACE('',(#21961),#18096,.F.);
#77392=ADVANCED_FACE('',(#21962),#18097,.F.);
#77393=ADVANCED_FACE('',(#21963),#18098,.F.);
#77394=ADVANCED_FACE('',(#21964),#18099,.F.);
#77395=ADVANCED_FACE('',(#21965),#18100,.F.);
#77396=ADVANCED_FACE('',(#21966),#18101,.F.);
#77397=ADVANCED_FACE('',(#21967),#18102,.F.);
#77398=ADVANCED_FACE('',(#21968),#18103,.F.);
#77399=ADVANCED_FACE('',(#21969),#18104,.F.);
#77400=ADVANCED_FACE('',(#21970),#18105,.F.);
#77401=ADVANCED_FACE('',(#21971),#18106,.F.);
#77402=ADVANCED_FACE('',(#21972),#18107,.F.);
#77403=ADVANCED_FACE('',(#21973),#18108,.F.);
#77404=ADVANCED_FACE('',(#21974),#18109,.F.);
#77405=ADVANCED_FACE('',(#21975),#18110,.F.);
#77406=ADVANCED_FACE('',(#21976),#18111,.F.);
#77407=ADVANCED_FACE('',(#21977),#18112,.F.);
#77408=ADVANCED_FACE('',(#21978),#18113,.F.);
#77409=ADVANCED_FACE('',(#21979),#18114,.F.);
#77410=ADVANCED_FACE('',(#21980),#18115,.F.);
#77411=ADVANCED_FACE('',(#21981),#18116,.F.);
#77412=ADVANCED_FACE('',(#21982),#18117,.F.);
#77413=ADVANCED_FACE('',(#21983),#18118,.F.);
#77414=ADVANCED_FACE('',(#21984),#18119,.F.);
#77415=ADVANCED_FACE('',(#21985),#18120,.F.);
#77416=ADVANCED_FACE('',(#21986),#18121,.F.);
#77417=ADVANCED_FACE('',(#21987),#18122,.F.);
#77418=ADVANCED_FACE('',(#21988),#18123,.F.);
#77419=ADVANCED_FACE('',(#21989),#18124,.F.);
#77420=ADVANCED_FACE('',(#21990),#18125,.F.);
#77421=ADVANCED_FACE('',(#21991),#18126,.F.);
#77422=ADVANCED_FACE('',(#21992),#18127,.F.);
#77423=ADVANCED_FACE('',(#21993),#18128,.F.);
#77424=ADVANCED_FACE('',(#21994),#18129,.F.);
#77425=ADVANCED_FACE('',(#21995),#18130,.F.);
#77426=ADVANCED_FACE('',(#21996),#18131,.F.);
#77427=ADVANCED_FACE('',(#21997),#18132,.F.);
#77428=ADVANCED_FACE('',(#21998),#18133,.F.);
#77429=ADVANCED_FACE('',(#21999),#18134,.F.);
#77430=ADVANCED_FACE('',(#22000),#18135,.F.);
#77431=ADVANCED_FACE('',(#22001),#18136,.F.);
#77432=ADVANCED_FACE('',(#22002),#18137,.F.);
#77433=ADVANCED_FACE('',(#22003),#18138,.F.);
#77434=ADVANCED_FACE('',(#22004),#18139,.F.);
#77435=ADVANCED_FACE('',(#22005),#18140,.F.);
#77436=ADVANCED_FACE('',(#22006),#18141,.F.);
#77437=ADVANCED_FACE('',(#22007),#18142,.F.);
#77438=ADVANCED_FACE('',(#22008),#18143,.F.);
#77439=ADVANCED_FACE('',(#22009),#18144,.F.);
#77440=ADVANCED_FACE('',(#22010),#18145,.F.);
#77441=ADVANCED_FACE('',(#22011),#18146,.F.);
#77442=ADVANCED_FACE('',(#22012),#18147,.F.);
#77443=ADVANCED_FACE('',(#22013),#18148,.F.);
#77444=ADVANCED_FACE('',(#22014),#18149,.F.);
#77445=ADVANCED_FACE('',(#22015),#18150,.F.);
#77446=ADVANCED_FACE('',(#22016),#18151,.F.);
#77447=ADVANCED_FACE('',(#22017),#18152,.F.);
#77448=ADVANCED_FACE('',(#22018),#18153,.F.);
#77449=ADVANCED_FACE('',(#22019),#18154,.F.);
#77450=ADVANCED_FACE('',(#22020),#18155,.F.);
#77451=ADVANCED_FACE('',(#22021),#18156,.F.);
#77452=ADVANCED_FACE('',(#22022),#18157,.F.);
#77453=ADVANCED_FACE('',(#22023),#18158,.F.);
#77454=ADVANCED_FACE('',(#22024),#18159,.F.);
#77455=ADVANCED_FACE('',(#22025),#18160,.F.);
#77456=ADVANCED_FACE('',(#22026),#18161,.F.);
#77457=ADVANCED_FACE('',(#22027),#18162,.F.);
#77458=ADVANCED_FACE('',(#22028),#18163,.F.);
#77459=ADVANCED_FACE('',(#22029),#18164,.F.);
#77460=ADVANCED_FACE('',(#22030),#18165,.F.);
#77461=ADVANCED_FACE('',(#22031),#18166,.F.);
#77462=ADVANCED_FACE('',(#22032),#18167,.F.);
#77463=ADVANCED_FACE('',(#22033),#18168,.F.);
#77464=ADVANCED_FACE('',(#22034),#18169,.F.);
#77465=ADVANCED_FACE('',(#22035),#18170,.F.);
#77466=ADVANCED_FACE('',(#22036),#18171,.F.);
#77467=ADVANCED_FACE('',(#22037),#18172,.F.);
#77468=ADVANCED_FACE('',(#22038),#18173,.F.);
#77469=ADVANCED_FACE('',(#22039),#18174,.F.);
#77470=ADVANCED_FACE('',(#22040),#18175,.F.);
#77471=ADVANCED_FACE('',(#22041),#18176,.F.);
#77472=ADVANCED_FACE('',(#22042),#18177,.F.);
#77473=ADVANCED_FACE('',(#22043),#18178,.F.);
#77474=ADVANCED_FACE('',(#22044),#18179,.F.);
#77475=ADVANCED_FACE('',(#22045),#18180,.F.);
#77476=ADVANCED_FACE('',(#22046),#18181,.F.);
#77477=ADVANCED_FACE('',(#22047),#18182,.F.);
#77478=ADVANCED_FACE('',(#22048),#18183,.F.);
#77479=ADVANCED_FACE('',(#22049),#18184,.F.);
#77480=ADVANCED_FACE('',(#22050),#18185,.F.);
#77481=ADVANCED_FACE('',(#22051),#18186,.F.);
#77482=ADVANCED_FACE('',(#22052),#18187,.F.);
#77483=ADVANCED_FACE('',(#22053),#18188,.F.);
#77484=ADVANCED_FACE('',(#22054),#18189,.F.);
#77485=ADVANCED_FACE('',(#22055),#18190,.F.);
#77486=ADVANCED_FACE('',(#22056),#18191,.F.);
#77487=ADVANCED_FACE('',(#22057),#18192,.F.);
#77488=ADVANCED_FACE('',(#22058),#18193,.F.);
#77489=ADVANCED_FACE('',(#22059),#18194,.F.);
#77490=ADVANCED_FACE('',(#22060),#18195,.F.);
#77491=ADVANCED_FACE('',(#22061),#18196,.F.);
#77492=ADVANCED_FACE('',(#22062),#18197,.F.);
#77493=ADVANCED_FACE('',(#22063),#18198,.F.);
#77494=ADVANCED_FACE('',(#22064),#18199,.F.);
#77495=ADVANCED_FACE('',(#22065),#18200,.F.);
#77496=ADVANCED_FACE('',(#22066),#18201,.F.);
#77497=ADVANCED_FACE('',(#22067),#18202,.F.);
#77498=ADVANCED_FACE('',(#22068),#18203,.F.);
#77499=ADVANCED_FACE('',(#22069),#18204,.F.);
#77500=ADVANCED_FACE('',(#22070),#18205,.F.);
#77501=ADVANCED_FACE('',(#22071),#18206,.F.);
#77502=ADVANCED_FACE('',(#22072),#18207,.F.);
#77503=ADVANCED_FACE('',(#22073),#18208,.F.);
#77504=ADVANCED_FACE('',(#22074),#18209,.F.);
#77505=ADVANCED_FACE('',(#22075),#18210,.F.);
#77506=ADVANCED_FACE('',(#22076),#18211,.F.);
#77507=ADVANCED_FACE('',(#22077),#18212,.F.);
#77508=ADVANCED_FACE('',(#22078),#18213,.F.);
#77509=ADVANCED_FACE('',(#22079),#18214,.F.);
#77510=ADVANCED_FACE('',(#22080),#18215,.F.);
#77511=ADVANCED_FACE('',(#22081),#18216,.F.);
#77512=ADVANCED_FACE('',(#22082),#18217,.F.);
#77513=ADVANCED_FACE('',(#22083),#18218,.F.);
#77514=ADVANCED_FACE('',(#22084),#18219,.F.);
#77515=ADVANCED_FACE('',(#22085),#18220,.F.);
#77516=ADVANCED_FACE('',(#22086),#18221,.F.);
#77517=ADVANCED_FACE('',(#22087),#18222,.F.);
#77518=ADVANCED_FACE('',(#22088),#18223,.F.);
#77519=ADVANCED_FACE('',(#22089),#18224,.F.);
#77520=ADVANCED_FACE('',(#22090),#18225,.F.);
#77521=ADVANCED_FACE('',(#22091),#18226,.F.);
#77522=ADVANCED_FACE('',(#22092),#18227,.F.);
#77523=ADVANCED_FACE('',(#22093),#18228,.F.);
#77524=ADVANCED_FACE('',(#22094),#18229,.F.);
#77525=ADVANCED_FACE('',(#22095),#18230,.F.);
#77526=ADVANCED_FACE('',(#22096),#18231,.F.);
#77527=ADVANCED_FACE('',(#22097),#18232,.F.);
#77528=ADVANCED_FACE('',(#22098),#18233,.F.);
#77529=ADVANCED_FACE('',(#22099),#18234,.F.);
#77530=ADVANCED_FACE('',(#22100),#18235,.F.);
#77531=ADVANCED_FACE('',(#22101),#18236,.F.);
#77532=ADVANCED_FACE('',(#22102),#18237,.F.);
#77533=ADVANCED_FACE('',(#22103),#18238,.F.);
#77534=ADVANCED_FACE('',(#22104),#18239,.F.);
#77535=ADVANCED_FACE('',(#22105),#18240,.F.);
#77536=ADVANCED_FACE('',(#22106),#18241,.F.);
#77537=ADVANCED_FACE('',(#22107),#18242,.F.);
#77538=ADVANCED_FACE('',(#22108),#18243,.F.);
#77539=ADVANCED_FACE('',(#22109),#18244,.F.);
#77540=ADVANCED_FACE('',(#22110),#18245,.F.);
#77541=ADVANCED_FACE('',(#22111),#18246,.F.);
#77542=ADVANCED_FACE('',(#22112),#18247,.F.);
#77543=ADVANCED_FACE('',(#22113),#18248,.F.);
#77544=ADVANCED_FACE('',(#22114),#18249,.F.);
#77545=ADVANCED_FACE('',(#22115),#18250,.F.);
#77546=ADVANCED_FACE('',(#22116),#18251,.F.);
#77547=ADVANCED_FACE('',(#22117),#18252,.F.);
#77548=ADVANCED_FACE('',(#22118),#18253,.F.);
#77549=ADVANCED_FACE('',(#22119),#18254,.F.);
#77550=ADVANCED_FACE('',(#22120),#18255,.F.);
#77551=ADVANCED_FACE('',(#22121),#18256,.F.);
#77552=ADVANCED_FACE('',(#22122),#18257,.F.);
#77553=ADVANCED_FACE('',(#22123),#18258,.F.);
#77554=ADVANCED_FACE('',(#22124),#18259,.F.);
#77555=ADVANCED_FACE('',(#22125),#18260,.F.);
#77556=ADVANCED_FACE('',(#22126),#18261,.F.);
#77557=ADVANCED_FACE('',(#22127),#18262,.F.);
#77558=ADVANCED_FACE('',(#22128),#18263,.F.);
#77559=ADVANCED_FACE('',(#22129),#18264,.F.);
#77560=ADVANCED_FACE('',(#22130),#18265,.F.);
#77561=ADVANCED_FACE('',(#22131),#18266,.F.);
#77562=ADVANCED_FACE('',(#22132),#18267,.F.);
#77563=ADVANCED_FACE('',(#22133),#18268,.F.);
#77564=ADVANCED_FACE('',(#22134),#18269,.F.);
#77565=ADVANCED_FACE('',(#22135),#18270,.F.);
#77566=ADVANCED_FACE('',(#22136),#18271,.F.);
#77567=ADVANCED_FACE('',(#22137),#18272,.F.);
#77568=ADVANCED_FACE('',(#22138),#18273,.F.);
#77569=ADVANCED_FACE('',(#22139),#18274,.F.);
#77570=ADVANCED_FACE('',(#22140),#18275,.F.);
#77571=ADVANCED_FACE('',(#22141),#18276,.F.);
#77572=ADVANCED_FACE('',(#22142),#18277,.F.);
#77573=ADVANCED_FACE('',(#22143),#18278,.F.);
#77574=ADVANCED_FACE('',(#22144),#18279,.F.);
#77575=ADVANCED_FACE('',(#22145),#18280,.F.);
#77576=ADVANCED_FACE('',(#22146),#18281,.F.);
#77577=ADVANCED_FACE('',(#22147),#18282,.F.);
#77578=ADVANCED_FACE('',(#22148),#18283,.F.);
#77579=ADVANCED_FACE('',(#22149),#18284,.F.);
#77580=ADVANCED_FACE('',(#22150),#18285,.F.);
#77581=ADVANCED_FACE('',(#22151),#18286,.F.);
#77582=ADVANCED_FACE('',(#22152),#18287,.F.);
#77583=ADVANCED_FACE('',(#22153),#18288,.F.);
#77584=ADVANCED_FACE('',(#22154),#18289,.F.);
#77585=ADVANCED_FACE('',(#22155),#18290,.F.);
#77586=ADVANCED_FACE('',(#22156),#18291,.F.);
#77587=ADVANCED_FACE('',(#22157),#18292,.F.);
#77588=ADVANCED_FACE('',(#22158),#18293,.F.);
#77589=ADVANCED_FACE('',(#22159),#18294,.F.);
#77590=ADVANCED_FACE('',(#22160),#18295,.F.);
#77591=ADVANCED_FACE('',(#22161),#18296,.F.);
#77592=ADVANCED_FACE('',(#22162),#18297,.F.);
#77593=ADVANCED_FACE('',(#22163),#18298,.F.);
#77594=ADVANCED_FACE('',(#22164),#18299,.F.);
#77595=ADVANCED_FACE('',(#22165),#18300,.F.);
#77596=ADVANCED_FACE('',(#22166),#18301,.F.);
#77597=ADVANCED_FACE('',(#22167),#18302,.F.);
#77598=ADVANCED_FACE('',(#22168),#18303,.F.);
#77599=ADVANCED_FACE('',(#22169),#18304,.F.);
#77600=ADVANCED_FACE('',(#22170),#18305,.F.);
#77601=ADVANCED_FACE('',(#22171),#18306,.F.);
#77602=ADVANCED_FACE('',(#22172),#18307,.F.);
#77603=ADVANCED_FACE('',(#22173),#18308,.F.);
#77604=ADVANCED_FACE('',(#22174),#18309,.F.);
#77605=ADVANCED_FACE('',(#22175),#18310,.F.);
#77606=ADVANCED_FACE('',(#22176),#18311,.F.);
#77607=ADVANCED_FACE('',(#22177),#18312,.F.);
#77608=ADVANCED_FACE('',(#22178),#18313,.F.);
#77609=ADVANCED_FACE('',(#22179),#18314,.F.);
#77610=ADVANCED_FACE('',(#22180),#18315,.F.);
#77611=ADVANCED_FACE('',(#22181),#18316,.F.);
#77612=ADVANCED_FACE('',(#22182),#18317,.F.);
#77613=ADVANCED_FACE('',(#22183),#18318,.F.);
#77614=ADVANCED_FACE('',(#22184),#18319,.F.);
#77615=ADVANCED_FACE('',(#22185),#18320,.F.);
#77616=ADVANCED_FACE('',(#22186),#18321,.F.);
#77617=ADVANCED_FACE('',(#22187),#18322,.F.);
#77618=ADVANCED_FACE('',(#22188),#18323,.F.);
#77619=ADVANCED_FACE('',(#22189),#18324,.F.);
#77620=ADVANCED_FACE('',(#22190),#18325,.F.);
#77621=ADVANCED_FACE('',(#22191),#18326,.F.);
#77622=ADVANCED_FACE('',(#22192),#18327,.F.);
#77623=ADVANCED_FACE('',(#22193),#18328,.F.);
#77624=ADVANCED_FACE('',(#22194),#18329,.F.);
#77625=ADVANCED_FACE('',(#22195),#18330,.F.);
#77626=ADVANCED_FACE('',(#22196),#18331,.F.);
#77627=ADVANCED_FACE('',(#22197),#18332,.F.);
#77628=ADVANCED_FACE('',(#22198),#18333,.F.);
#77629=ADVANCED_FACE('',(#22199),#18334,.F.);
#77630=ADVANCED_FACE('',(#22200),#18335,.F.);
#77631=ADVANCED_FACE('',(#22201),#18336,.F.);
#77632=ADVANCED_FACE('',(#22202),#18337,.F.);
#77633=ADVANCED_FACE('',(#22203),#18338,.F.);
#77634=ADVANCED_FACE('',(#22204),#18339,.F.);
#77635=ADVANCED_FACE('',(#22205),#18340,.F.);
#77636=ADVANCED_FACE('',(#22206),#18341,.F.);
#77637=ADVANCED_FACE('',(#22207),#18342,.F.);
#77638=ADVANCED_FACE('',(#22208),#18343,.F.);
#77639=ADVANCED_FACE('',(#22209),#18344,.F.);
#77640=ADVANCED_FACE('',(#22210),#18345,.F.);
#77641=ADVANCED_FACE('',(#22211),#18346,.F.);
#77642=ADVANCED_FACE('',(#22212),#18347,.F.);
#77643=ADVANCED_FACE('',(#22213),#18348,.F.);
#77644=ADVANCED_FACE('',(#22214),#18349,.F.);
#77645=ADVANCED_FACE('',(#22215),#18350,.F.);
#77646=ADVANCED_FACE('',(#22216),#18351,.F.);
#77647=ADVANCED_FACE('',(#22217),#18352,.F.);
#77648=ADVANCED_FACE('',(#22218),#18353,.F.);
#77649=ADVANCED_FACE('',(#22219),#18354,.F.);
#77650=ADVANCED_FACE('',(#22220),#18355,.F.);
#77651=ADVANCED_FACE('',(#22221),#18356,.F.);
#77652=ADVANCED_FACE('',(#22222),#18357,.F.);
#77653=ADVANCED_FACE('',(#22223),#18358,.F.);
#77654=ADVANCED_FACE('',(#22224),#18359,.F.);
#77655=ADVANCED_FACE('',(#22225),#18360,.F.);
#77656=ADVANCED_FACE('',(#22226),#18361,.F.);
#77657=ADVANCED_FACE('',(#22227),#18362,.F.);
#77658=ADVANCED_FACE('',(#22228),#18363,.F.);
#77659=ADVANCED_FACE('',(#22229),#18364,.F.);
#77660=ADVANCED_FACE('',(#22230),#18365,.F.);
#77661=ADVANCED_FACE('',(#22231),#18366,.F.);
#77662=ADVANCED_FACE('',(#22232),#18367,.F.);
#77663=ADVANCED_FACE('',(#22233),#18368,.F.);
#77664=ADVANCED_FACE('',(#22234),#18369,.F.);
#77665=ADVANCED_FACE('',(#22235),#18370,.F.);
#77666=ADVANCED_FACE('',(#22236),#18371,.F.);
#77667=ADVANCED_FACE('',(#22237),#18372,.F.);
#77668=ADVANCED_FACE('',(#22238),#18373,.F.);
#77669=ADVANCED_FACE('',(#22239),#18374,.F.);
#77670=ADVANCED_FACE('',(#22240),#18375,.F.);
#77671=ADVANCED_FACE('',(#22241),#18376,.F.);
#77672=ADVANCED_FACE('',(#22242),#18377,.F.);
#77673=ADVANCED_FACE('',(#22243),#18378,.F.);
#77674=ADVANCED_FACE('',(#22244),#18379,.F.);
#77675=ADVANCED_FACE('',(#22245),#18380,.F.);
#77676=ADVANCED_FACE('',(#22246),#18381,.F.);
#77677=ADVANCED_FACE('',(#22247),#18382,.F.);
#77678=ADVANCED_FACE('',(#22248),#18383,.F.);
#77679=ADVANCED_FACE('',(#22249),#18384,.F.);
#77680=ADVANCED_FACE('',(#22250),#18385,.F.);
#77681=ADVANCED_FACE('',(#22251),#18386,.F.);
#77682=ADVANCED_FACE('',(#22252),#18387,.F.);
#77683=ADVANCED_FACE('',(#22253),#18388,.F.);
#77684=ADVANCED_FACE('',(#22254),#18389,.F.);
#77685=ADVANCED_FACE('',(#22255),#18390,.F.);
#77686=ADVANCED_FACE('',(#22256),#18391,.F.);
#77687=ADVANCED_FACE('',(#22257),#18392,.F.);
#77688=ADVANCED_FACE('',(#22258),#18393,.F.);
#77689=ADVANCED_FACE('',(#22259),#18394,.F.);
#77690=ADVANCED_FACE('',(#22260),#18395,.F.);
#77691=ADVANCED_FACE('',(#22261),#18396,.F.);
#77692=ADVANCED_FACE('',(#22262),#18397,.F.);
#77693=ADVANCED_FACE('',(#22263),#18398,.F.);
#77694=ADVANCED_FACE('',(#22264),#18399,.F.);
#77695=ADVANCED_FACE('',(#22265),#18400,.F.);
#77696=ADVANCED_FACE('',(#22266),#18401,.F.);
#77697=ADVANCED_FACE('',(#22267),#18402,.F.);
#77698=ADVANCED_FACE('',(#22268),#18403,.F.);
#77699=ADVANCED_FACE('',(#22269),#18404,.F.);
#77700=ADVANCED_FACE('',(#22270),#18405,.F.);
#77701=ADVANCED_FACE('',(#22271),#18406,.F.);
#77702=ADVANCED_FACE('',(#22272),#18407,.F.);
#77703=ADVANCED_FACE('',(#22273),#18408,.F.);
#77704=ADVANCED_FACE('',(#22274),#18409,.F.);
#77705=ADVANCED_FACE('',(#22275),#18410,.F.);
#77706=ADVANCED_FACE('',(#22276),#18411,.F.);
#77707=ADVANCED_FACE('',(#22277),#18412,.F.);
#77708=ADVANCED_FACE('',(#22278),#18413,.F.);
#77709=ADVANCED_FACE('',(#22279),#18414,.F.);
#77710=ADVANCED_FACE('',(#22280),#18415,.F.);
#77711=ADVANCED_FACE('',(#22281),#18416,.F.);
#77712=ADVANCED_FACE('',(#22282),#18417,.F.);
#77713=ADVANCED_FACE('',(#22283),#18418,.F.);
#77714=ADVANCED_FACE('',(#22284),#18419,.F.);
#77715=ADVANCED_FACE('',(#22285),#18420,.F.);
#77716=ADVANCED_FACE('',(#22286),#18421,.F.);
#77717=ADVANCED_FACE('',(#22287),#18422,.F.);
#77718=ADVANCED_FACE('',(#22288),#18423,.F.);
#77719=ADVANCED_FACE('',(#22289),#18424,.F.);
#77720=ADVANCED_FACE('',(#22290),#18425,.F.);
#77721=ADVANCED_FACE('',(#22291),#18426,.F.);
#77722=ADVANCED_FACE('',(#22292),#18427,.F.);
#77723=ADVANCED_FACE('',(#22293),#18428,.F.);
#77724=ADVANCED_FACE('',(#22294),#18429,.F.);
#77725=ADVANCED_FACE('',(#22295),#18430,.F.);
#77726=ADVANCED_FACE('',(#22296),#18431,.F.);
#77727=ADVANCED_FACE('',(#22297),#18432,.F.);
#77728=ADVANCED_FACE('',(#22298),#18433,.F.);
#77729=ADVANCED_FACE('',(#22299),#18434,.F.);
#77730=ADVANCED_FACE('',(#22300),#18435,.F.);
#77731=ADVANCED_FACE('',(#22301),#18436,.F.);
#77732=ADVANCED_FACE('',(#22302),#18437,.F.);
#77733=ADVANCED_FACE('',(#22303),#18438,.F.);
#77734=ADVANCED_FACE('',(#22304),#18439,.F.);
#77735=ADVANCED_FACE('',(#22305),#18440,.F.);
#77736=ADVANCED_FACE('',(#22306),#18441,.F.);
#77737=ADVANCED_FACE('',(#22307),#18442,.F.);
#77738=ADVANCED_FACE('',(#22308),#18443,.F.);
#77739=ADVANCED_FACE('',(#22309),#18444,.F.);
#77740=ADVANCED_FACE('',(#22310),#18445,.F.);
#77741=ADVANCED_FACE('',(#22311),#18446,.F.);
#77742=ADVANCED_FACE('',(#22312),#18447,.F.);
#77743=ADVANCED_FACE('',(#22313),#18448,.F.);
#77744=ADVANCED_FACE('',(#22314),#18449,.F.);
#77745=ADVANCED_FACE('',(#22315),#18450,.F.);
#77746=ADVANCED_FACE('',(#22316),#18451,.F.);
#77747=ADVANCED_FACE('',(#22317),#18452,.F.);
#77748=ADVANCED_FACE('',(#22318),#18453,.F.);
#77749=ADVANCED_FACE('',(#22319),#18454,.F.);
#77750=ADVANCED_FACE('',(#22320),#18455,.F.);
#77751=ADVANCED_FACE('',(#22321),#18456,.F.);
#77752=ADVANCED_FACE('',(#22322),#18457,.F.);
#77753=ADVANCED_FACE('',(#22323),#18458,.F.);
#77754=ADVANCED_FACE('',(#22324),#18459,.F.);
#77755=ADVANCED_FACE('',(#22325),#18460,.F.);
#77756=ADVANCED_FACE('',(#22326),#18461,.F.);
#77757=ADVANCED_FACE('',(#22327),#18462,.F.);
#77758=ADVANCED_FACE('',(#22328),#18463,.F.);
#77759=ADVANCED_FACE('',(#22329),#18464,.F.);
#77760=ADVANCED_FACE('',(#22330),#18465,.F.);
#77761=ADVANCED_FACE('',(#22331),#18466,.F.);
#77762=ADVANCED_FACE('',(#22332),#18467,.F.);
#77763=ADVANCED_FACE('',(#22333),#18468,.F.);
#77764=ADVANCED_FACE('',(#22334),#18469,.F.);
#77765=ADVANCED_FACE('',(#22335),#18470,.F.);
#77766=ADVANCED_FACE('',(#22336),#18471,.F.);
#77767=ADVANCED_FACE('',(#22337),#18472,.F.);
#77768=ADVANCED_FACE('',(#22338),#18473,.F.);
#77769=ADVANCED_FACE('',(#22339),#18474,.F.);
#77770=ADVANCED_FACE('',(#22340),#18475,.F.);
#77771=ADVANCED_FACE('',(#22341),#18476,.F.);
#77772=ADVANCED_FACE('',(#22342),#18477,.F.);
#77773=ADVANCED_FACE('',(#22343),#18478,.F.);
#77774=ADVANCED_FACE('',(#22344),#18479,.F.);
#77775=ADVANCED_FACE('',(#22345),#18480,.F.);
#77776=ADVANCED_FACE('',(#22346),#18481,.F.);
#77777=ADVANCED_FACE('',(#22347),#18482,.F.);
#77778=ADVANCED_FACE('',(#22348),#18483,.F.);
#77779=ADVANCED_FACE('',(#22349),#18484,.F.);
#77780=ADVANCED_FACE('',(#22350),#18485,.F.);
#77781=ADVANCED_FACE('',(#22351),#18486,.F.);
#77782=ADVANCED_FACE('',(#22352),#18487,.F.);
#77783=ADVANCED_FACE('',(#22353),#18488,.F.);
#77784=ADVANCED_FACE('',(#22354),#18489,.F.);
#77785=ADVANCED_FACE('',(#22355),#18490,.F.);
#77786=ADVANCED_FACE('',(#22356),#18491,.F.);
#77787=ADVANCED_FACE('',(#22357),#18492,.F.);
#77788=ADVANCED_FACE('',(#22358),#18493,.F.);
#77789=ADVANCED_FACE('',(#22359),#18494,.F.);
#77790=ADVANCED_FACE('',(#22360),#18495,.F.);
#77791=ADVANCED_FACE('',(#22361),#18496,.F.);
#77792=ADVANCED_FACE('',(#22362),#18497,.F.);
#77793=ADVANCED_FACE('',(#22363),#18498,.F.);
#77794=ADVANCED_FACE('',(#22364),#18499,.F.);
#77795=ADVANCED_FACE('',(#22365),#18500,.F.);
#77796=ADVANCED_FACE('',(#22366),#18501,.F.);
#77797=ADVANCED_FACE('',(#22367),#18502,.F.);
#77798=ADVANCED_FACE('',(#22368),#18503,.F.);
#77799=ADVANCED_FACE('',(#22369),#18504,.F.);
#77800=ADVANCED_FACE('',(#22370),#18505,.F.);
#77801=ADVANCED_FACE('',(#22371),#18506,.F.);
#77802=ADVANCED_FACE('',(#22372),#18507,.F.);
#77803=ADVANCED_FACE('',(#22373),#18508,.F.);
#77804=ADVANCED_FACE('',(#22374),#18509,.F.);
#77805=ADVANCED_FACE('',(#22375),#18510,.F.);
#77806=ADVANCED_FACE('',(#22376),#18511,.F.);
#77807=ADVANCED_FACE('',(#22377),#18512,.F.);
#77808=ADVANCED_FACE('',(#22378),#18513,.F.);
#77809=ADVANCED_FACE('',(#22379),#18514,.F.);
#77810=ADVANCED_FACE('',(#22380),#18515,.F.);
#77811=ADVANCED_FACE('',(#22381),#18516,.F.);
#77812=ADVANCED_FACE('',(#22382),#18517,.F.);
#77813=ADVANCED_FACE('',(#22383),#18518,.F.);
#77814=ADVANCED_FACE('',(#22384),#18519,.F.);
#77815=ADVANCED_FACE('',(#22385),#18520,.F.);
#77816=ADVANCED_FACE('',(#22386),#18521,.F.);
#77817=ADVANCED_FACE('',(#22387),#18522,.F.);
#77818=ADVANCED_FACE('',(#22388),#18523,.F.);
#77819=ADVANCED_FACE('',(#22389),#18524,.F.);
#77820=ADVANCED_FACE('',(#22390),#18525,.F.);
#77821=ADVANCED_FACE('',(#22391),#18526,.F.);
#77822=ADVANCED_FACE('',(#22392),#18527,.F.);
#77823=ADVANCED_FACE('',(#22393),#18528,.F.);
#77824=ADVANCED_FACE('',(#22394),#18529,.F.);
#77825=ADVANCED_FACE('',(#22395),#18530,.F.);
#77826=ADVANCED_FACE('',(#22396),#18531,.F.);
#77827=ADVANCED_FACE('',(#22397),#18532,.F.);
#77828=ADVANCED_FACE('',(#22398),#18533,.F.);
#77829=ADVANCED_FACE('',(#22399),#18534,.F.);
#77830=ADVANCED_FACE('',(#22400),#18535,.F.);
#77831=ADVANCED_FACE('',(#22401),#18536,.F.);
#77832=ADVANCED_FACE('',(#22402),#18537,.F.);
#77833=ADVANCED_FACE('',(#22403),#18538,.F.);
#77834=ADVANCED_FACE('',(#22404),#18539,.F.);
#77835=ADVANCED_FACE('',(#22405),#18540,.F.);
#77836=ADVANCED_FACE('',(#22406),#18541,.F.);
#77837=ADVANCED_FACE('',(#22407),#18542,.F.);
#77838=ADVANCED_FACE('',(#22408),#18543,.F.);
#77839=ADVANCED_FACE('',(#22409),#18544,.F.);
#77840=ADVANCED_FACE('',(#22410),#18545,.F.);
#77841=ADVANCED_FACE('',(#22411),#18546,.F.);
#77842=ADVANCED_FACE('',(#22412),#18547,.F.);
#77843=ADVANCED_FACE('',(#22413),#18548,.F.);
#77844=ADVANCED_FACE('',(#22414),#18549,.F.);
#77845=ADVANCED_FACE('',(#22415),#18550,.F.);
#77846=ADVANCED_FACE('',(#22416),#18551,.F.);
#77847=ADVANCED_FACE('',(#22417),#18552,.F.);
#77848=ADVANCED_FACE('',(#22418),#18553,.F.);
#77849=ADVANCED_FACE('',(#22419),#18554,.F.);
#77850=ADVANCED_FACE('',(#22420),#18555,.F.);
#77851=ADVANCED_FACE('',(#22421),#18556,.F.);
#77852=ADVANCED_FACE('',(#22422),#18557,.F.);
#77853=ADVANCED_FACE('',(#22423),#18558,.F.);
#77854=ADVANCED_FACE('',(#22424),#18559,.F.);
#77855=ADVANCED_FACE('',(#22425),#18560,.F.);
#77856=ADVANCED_FACE('',(#22426),#18561,.F.);
#77857=ADVANCED_FACE('',(#22427),#18562,.F.);
#77858=ADVANCED_FACE('',(#22428),#18563,.F.);
#77859=ADVANCED_FACE('',(#22429),#18564,.F.);
#77860=ADVANCED_FACE('',(#22430),#18565,.F.);
#77861=ADVANCED_FACE('',(#22431),#18566,.F.);
#77862=ADVANCED_FACE('',(#22432),#18567,.F.);
#77863=ADVANCED_FACE('',(#22433),#18568,.F.);
#77864=ADVANCED_FACE('',(#22434),#18569,.F.);
#77865=ADVANCED_FACE('',(#22435),#18570,.F.);
#77866=ADVANCED_FACE('',(#22436),#18571,.F.);
#77867=ADVANCED_FACE('',(#22437),#18572,.F.);
#77868=ADVANCED_FACE('',(#22438),#18573,.F.);
#77869=ADVANCED_FACE('',(#22439),#18574,.F.);
#77870=ADVANCED_FACE('',(#22440),#18575,.F.);
#77871=ADVANCED_FACE('',(#22441),#18576,.F.);
#77872=ADVANCED_FACE('',(#22442),#18577,.F.);
#77873=ADVANCED_FACE('',(#22443),#18578,.F.);
#77874=ADVANCED_FACE('',(#22444),#18579,.F.);
#77875=ADVANCED_FACE('',(#22445),#18580,.F.);
#77876=ADVANCED_FACE('',(#22446),#18581,.F.);
#77877=ADVANCED_FACE('',(#22447),#18582,.F.);
#77878=ADVANCED_FACE('',(#22448),#18583,.F.);
#77879=ADVANCED_FACE('',(#22449),#18584,.F.);
#77880=ADVANCED_FACE('',(#22450),#18585,.F.);
#77881=ADVANCED_FACE('',(#22451),#18586,.F.);
#77882=ADVANCED_FACE('',(#22452),#18587,.F.);
#77883=ADVANCED_FACE('',(#22453),#18588,.F.);
#77884=ADVANCED_FACE('',(#22454),#18589,.F.);
#77885=ADVANCED_FACE('',(#22455),#18590,.F.);
#77886=ADVANCED_FACE('',(#22456),#18591,.F.);
#77887=ADVANCED_FACE('',(#22457),#18592,.F.);
#77888=ADVANCED_FACE('',(#22458),#18593,.F.);
#77889=ADVANCED_FACE('',(#22459),#18594,.F.);
#77890=ADVANCED_FACE('',(#22460),#18595,.F.);
#77891=ADVANCED_FACE('',(#22461),#18596,.F.);
#77892=ADVANCED_FACE('',(#22462),#18597,.F.);
#77893=ADVANCED_FACE('',(#22463),#18598,.F.);
#77894=ADVANCED_FACE('',(#22464),#18599,.F.);
#77895=ADVANCED_FACE('',(#22465),#18600,.F.);
#77896=ADVANCED_FACE('',(#22466),#18601,.F.);
#77897=ADVANCED_FACE('',(#22467),#18602,.F.);
#77898=ADVANCED_FACE('',(#22468),#18603,.F.);
#77899=ADVANCED_FACE('',(#22469),#18604,.F.);
#77900=ADVANCED_FACE('',(#22470),#18605,.F.);
#77901=ADVANCED_FACE('',(#22471),#18606,.F.);
#77902=ADVANCED_FACE('',(#22472),#18607,.F.);
#77903=ADVANCED_FACE('',(#22473),#18608,.F.);
#77904=ADVANCED_FACE('',(#22474),#18609,.F.);
#77905=ADVANCED_FACE('',(#22475),#18610,.F.);
#77906=ADVANCED_FACE('',(#22476),#18611,.F.);
#77907=ADVANCED_FACE('',(#22477),#18612,.F.);
#77908=ADVANCED_FACE('',(#22478),#18613,.F.);
#77909=ADVANCED_FACE('',(#22479),#18614,.F.);
#77910=ADVANCED_FACE('',(#22480),#18615,.F.);
#77911=ADVANCED_FACE('',(#22481),#18616,.F.);
#77912=ADVANCED_FACE('',(#22482),#18617,.F.);
#77913=ADVANCED_FACE('',(#22483),#18618,.F.);
#77914=ADVANCED_FACE('',(#22484),#18619,.F.);
#77915=ADVANCED_FACE('',(#22485),#18620,.F.);
#77916=ADVANCED_FACE('',(#22486),#18621,.F.);
#77917=ADVANCED_FACE('',(#22487),#18622,.F.);
#77918=ADVANCED_FACE('',(#22488),#18623,.F.);
#77919=ADVANCED_FACE('',(#22489),#18624,.F.);
#77920=ADVANCED_FACE('',(#22490),#18625,.F.);
#77921=ADVANCED_FACE('',(#22491),#18626,.F.);
#77922=ADVANCED_FACE('',(#22492),#18627,.F.);
#77923=ADVANCED_FACE('',(#22493),#18628,.F.);
#77924=ADVANCED_FACE('',(#22494),#18629,.F.);
#77925=ADVANCED_FACE('',(#22495),#18630,.F.);
#77926=ADVANCED_FACE('',(#22496),#18631,.F.);
#77927=ADVANCED_FACE('',(#22497),#18632,.F.);
#77928=ADVANCED_FACE('',(#22498),#18633,.F.);
#77929=ADVANCED_FACE('',(#22499),#18634,.F.);
#77930=ADVANCED_FACE('',(#22500),#18635,.F.);
#77931=ADVANCED_FACE('',(#22501),#18636,.F.);
#77932=ADVANCED_FACE('',(#22502),#18637,.F.);
#77933=ADVANCED_FACE('',(#22503),#18638,.F.);
#77934=ADVANCED_FACE('',(#22504),#18639,.F.);
#77935=ADVANCED_FACE('',(#22505),#18640,.F.);
#77936=ADVANCED_FACE('',(#22506),#18641,.F.);
#77937=ADVANCED_FACE('',(#22507),#18642,.F.);
#77938=ADVANCED_FACE('',(#22508),#18643,.F.);
#77939=ADVANCED_FACE('',(#22509),#18644,.F.);
#77940=ADVANCED_FACE('',(#22510),#18645,.F.);
#77941=ADVANCED_FACE('',(#22511),#18646,.F.);
#77942=ADVANCED_FACE('',(#22512),#18647,.F.);
#77943=ADVANCED_FACE('',(#22513),#18648,.F.);
#77944=ADVANCED_FACE('',(#22514),#18649,.F.);
#77945=ADVANCED_FACE('',(#22515),#18650,.F.);
#77946=ADVANCED_FACE('',(#22516),#18651,.F.);
#77947=ADVANCED_FACE('',(#22517),#18652,.F.);
#77948=ADVANCED_FACE('',(#22518),#18653,.F.);
#77949=ADVANCED_FACE('',(#22519),#18654,.F.);
#77950=ADVANCED_FACE('',(#22520),#18655,.F.);
#77951=ADVANCED_FACE('',(#22521),#18656,.F.);
#77952=ADVANCED_FACE('',(#22522),#18657,.F.);
#77953=ADVANCED_FACE('',(#22523),#18658,.F.);
#77954=ADVANCED_FACE('',(#22524),#18659,.F.);
#77955=ADVANCED_FACE('',(#22525),#18660,.F.);
#77956=ADVANCED_FACE('',(#22526),#18661,.F.);
#77957=ADVANCED_FACE('',(#22527),#18662,.F.);
#77958=ADVANCED_FACE('',(#22528),#18663,.F.);
#77959=ADVANCED_FACE('',(#22529),#18664,.F.);
#77960=ADVANCED_FACE('',(#22530),#18665,.F.);
#77961=ADVANCED_FACE('',(#22531),#18666,.F.);
#77962=ADVANCED_FACE('',(#22532),#18667,.F.);
#77963=ADVANCED_FACE('',(#22533),#18668,.F.);
#77964=ADVANCED_FACE('',(#22534),#18669,.F.);
#77965=ADVANCED_FACE('',(#22535),#18670,.F.);
#77966=ADVANCED_FACE('',(#22536),#18671,.F.);
#77967=ADVANCED_FACE('',(#22537),#18672,.F.);
#77968=ADVANCED_FACE('',(#22538),#18673,.F.);
#77969=ADVANCED_FACE('',(#22539),#18674,.F.);
#77970=ADVANCED_FACE('',(#22540),#18675,.F.);
#77971=ADVANCED_FACE('',(#22541),#18676,.F.);
#77972=ADVANCED_FACE('',(#22542),#18677,.F.);
#77973=ADVANCED_FACE('',(#22543),#18678,.F.);
#77974=ADVANCED_FACE('',(#22544),#18679,.F.);
#77975=ADVANCED_FACE('',(#22545),#18680,.F.);
#77976=ADVANCED_FACE('',(#22546),#18681,.F.);
#77977=ADVANCED_FACE('',(#22547),#18682,.F.);
#77978=ADVANCED_FACE('',(#22548),#18683,.F.);
#77979=ADVANCED_FACE('',(#22549),#18684,.F.);
#77980=ADVANCED_FACE('',(#22550),#18685,.F.);
#77981=ADVANCED_FACE('',(#22551),#18686,.F.);
#77982=ADVANCED_FACE('',(#22552),#18687,.F.);
#77983=ADVANCED_FACE('',(#22553),#18688,.F.);
#77984=ADVANCED_FACE('',(#22554),#18689,.F.);
#77985=ADVANCED_FACE('',(#22555),#18690,.F.);
#77986=ADVANCED_FACE('',(#22556),#18691,.F.);
#77987=ADVANCED_FACE('',(#22557),#18692,.F.);
#77988=ADVANCED_FACE('',(#22558),#18693,.F.);
#77989=ADVANCED_FACE('',(#22559),#18694,.F.);
#77990=ADVANCED_FACE('',(#22560),#18695,.F.);
#77991=ADVANCED_FACE('',(#22561),#18696,.F.);
#77992=ADVANCED_FACE('',(#22562),#18697,.F.);
#77993=ADVANCED_FACE('',(#22563),#18698,.F.);
#77994=ADVANCED_FACE('',(#22564),#18699,.F.);
#77995=ADVANCED_FACE('',(#22565),#18700,.F.);
#77996=ADVANCED_FACE('',(#22566),#18701,.F.);
#77997=ADVANCED_FACE('',(#22567),#18702,.F.);
#77998=ADVANCED_FACE('',(#22568),#18703,.F.);
#77999=ADVANCED_FACE('',(#22569),#18704,.F.);
#78000=ADVANCED_FACE('',(#22570),#18705,.F.);
#78001=ADVANCED_FACE('',(#22571),#18706,.F.);
#78002=ADVANCED_FACE('',(#22572),#18707,.F.);
#78003=ADVANCED_FACE('',(#22573),#18708,.F.);
#78004=ADVANCED_FACE('',(#22574),#18709,.F.);
#78005=ADVANCED_FACE('',(#22575),#18710,.F.);
#78006=ADVANCED_FACE('',(#22576),#18711,.F.);
#78007=ADVANCED_FACE('',(#22577),#18712,.F.);
#78008=ADVANCED_FACE('',(#22578),#18713,.F.);
#78009=ADVANCED_FACE('',(#22579),#18714,.F.);
#78010=ADVANCED_FACE('',(#22580),#18715,.F.);
#78011=ADVANCED_FACE('',(#22581),#18716,.F.);
#78012=ADVANCED_FACE('',(#22582),#18717,.F.);
#78013=ADVANCED_FACE('',(#22583),#18718,.F.);
#78014=ADVANCED_FACE('',(#22584),#18719,.F.);
#78015=ADVANCED_FACE('',(#22585),#18720,.F.);
#78016=ADVANCED_FACE('',(#22586),#18721,.F.);
#78017=ADVANCED_FACE('',(#22587),#18722,.F.);
#78018=ADVANCED_FACE('',(#22588),#18723,.F.);
#78019=ADVANCED_FACE('',(#22589),#18724,.F.);
#78020=ADVANCED_FACE('',(#22590),#18725,.F.);
#78021=ADVANCED_FACE('',(#22591),#18726,.F.);
#78022=ADVANCED_FACE('',(#22592),#18727,.F.);
#78023=ADVANCED_FACE('',(#22593),#18728,.F.);
#78024=ADVANCED_FACE('',(#22594),#18729,.F.);
#78025=ADVANCED_FACE('',(#22595),#18730,.F.);
#78026=ADVANCED_FACE('',(#22596),#18731,.F.);
#78027=ADVANCED_FACE('',(#22597),#18732,.F.);
#78028=ADVANCED_FACE('',(#22598),#18733,.F.);
#78029=ADVANCED_FACE('',(#22599),#18734,.F.);
#78030=ADVANCED_FACE('',(#22600),#18735,.F.);
#78031=ADVANCED_FACE('',(#22601),#18736,.F.);
#78032=ADVANCED_FACE('',(#22602),#18737,.F.);
#78033=ADVANCED_FACE('',(#22603),#18738,.F.);
#78034=ADVANCED_FACE('',(#22604),#18739,.F.);
#78035=ADVANCED_FACE('',(#22605),#18740,.F.);
#78036=ADVANCED_FACE('',(#22606),#18741,.F.);
#78037=ADVANCED_FACE('',(#22607),#18742,.F.);
#78038=ADVANCED_FACE('',(#22608),#18743,.F.);
#78039=ADVANCED_FACE('',(#22609),#18744,.F.);
#78040=ADVANCED_FACE('',(#22610),#18745,.F.);
#78041=ADVANCED_FACE('',(#22611),#18746,.F.);
#78042=ADVANCED_FACE('',(#22612),#18747,.F.);
#78043=ADVANCED_FACE('',(#22613),#18748,.F.);
#78044=ADVANCED_FACE('',(#22614),#18749,.F.);
#78045=ADVANCED_FACE('',(#22615),#18750,.F.);
#78046=ADVANCED_FACE('',(#22616),#18751,.F.);
#78047=ADVANCED_FACE('',(#22617),#18752,.F.);
#78048=ADVANCED_FACE('',(#22618),#18753,.F.);
#78049=ADVANCED_FACE('',(#22619),#18754,.F.);
#78050=ADVANCED_FACE('',(#22620),#18755,.F.);
#78051=ADVANCED_FACE('',(#22621),#18756,.F.);
#78052=ADVANCED_FACE('',(#22622),#18757,.F.);
#78053=ADVANCED_FACE('',(#22623),#18758,.F.);
#78054=ADVANCED_FACE('',(#22624),#18759,.F.);
#78055=ADVANCED_FACE('',(#22625),#18760,.F.);
#78056=ADVANCED_FACE('',(#22626),#18761,.F.);
#78057=ADVANCED_FACE('',(#22627),#18762,.F.);
#78058=ADVANCED_FACE('',(#22628),#18763,.F.);
#78059=ADVANCED_FACE('',(#22629),#18764,.F.);
#78060=ADVANCED_FACE('',(#22630),#18765,.F.);
#78061=ADVANCED_FACE('',(#22631),#18766,.F.);
#78062=ADVANCED_FACE('',(#22632),#18767,.F.);
#78063=ADVANCED_FACE('',(#22633),#18768,.F.);
#78064=ADVANCED_FACE('',(#22634),#18769,.F.);
#78065=ADVANCED_FACE('',(#22635),#18770,.F.);
#78066=ADVANCED_FACE('',(#22636),#18771,.F.);
#78067=ADVANCED_FACE('',(#22637),#18772,.F.);
#78068=ADVANCED_FACE('',(#22638),#18773,.F.);
#78069=ADVANCED_FACE('',(#22639),#18774,.F.);
#78070=ADVANCED_FACE('',(#22640),#18775,.F.);
#78071=ADVANCED_FACE('',(#22641),#18776,.F.);
#78072=ADVANCED_FACE('',(#22642),#18777,.F.);
#78073=ADVANCED_FACE('',(#22643),#18778,.F.);
#78074=ADVANCED_FACE('',(#22644),#18779,.F.);
#78075=ADVANCED_FACE('',(#22645),#18780,.F.);
#78076=ADVANCED_FACE('',(#22646),#18781,.F.);
#78077=ADVANCED_FACE('',(#22647),#18782,.F.);
#78078=ADVANCED_FACE('',(#22648),#18783,.F.);
#78079=ADVANCED_FACE('',(#22649),#18784,.F.);
#78080=ADVANCED_FACE('',(#22650),#18785,.F.);
#78081=ADVANCED_FACE('',(#22651),#18786,.F.);
#78082=ADVANCED_FACE('',(#22652),#18787,.F.);
#78083=ADVANCED_FACE('',(#22653),#18788,.F.);
#78084=ADVANCED_FACE('',(#22654),#18789,.F.);
#78085=ADVANCED_FACE('',(#22655),#18790,.F.);
#78086=ADVANCED_FACE('',(#22656),#18791,.F.);
#78087=ADVANCED_FACE('',(#22657),#18792,.F.);
#78088=ADVANCED_FACE('',(#22658),#18793,.F.);
#78089=ADVANCED_FACE('',(#22659),#18794,.F.);
#78090=ADVANCED_FACE('',(#22660),#18795,.F.);
#78091=ADVANCED_FACE('',(#22661),#18796,.F.);
#78092=ADVANCED_FACE('',(#22662),#18797,.F.);
#78093=ADVANCED_FACE('',(#22663),#18798,.F.);
#78094=ADVANCED_FACE('',(#22664),#18799,.F.);
#78095=ADVANCED_FACE('',(#22665),#18800,.F.);
#78096=ADVANCED_FACE('',(#22666),#18801,.F.);
#78097=ADVANCED_FACE('',(#22667),#18802,.F.);
#78098=ADVANCED_FACE('',(#22668),#18803,.F.);
#78099=ADVANCED_FACE('',(#22669),#18804,.F.);
#78100=ADVANCED_FACE('',(#22670),#18805,.F.);
#78101=ADVANCED_FACE('',(#22671),#18806,.F.);
#78102=ADVANCED_FACE('',(#22672),#18807,.F.);
#78103=ADVANCED_FACE('',(#22673),#18808,.F.);
#78104=ADVANCED_FACE('',(#22674),#18809,.F.);
#78105=ADVANCED_FACE('',(#22675),#18810,.F.);
#78106=ADVANCED_FACE('',(#22676),#18811,.F.);
#78107=ADVANCED_FACE('',(#22677),#18812,.F.);
#78108=ADVANCED_FACE('',(#22678),#18813,.F.);
#78109=ADVANCED_FACE('',(#22679),#18814,.F.);
#78110=ADVANCED_FACE('',(#22680),#18815,.F.);
#78111=ADVANCED_FACE('',(#22681),#18816,.F.);
#78112=ADVANCED_FACE('',(#22682),#18817,.F.);
#78113=ADVANCED_FACE('',(#22683),#18818,.F.);
#78114=ADVANCED_FACE('',(#22684),#18819,.F.);
#78115=ADVANCED_FACE('',(#22685),#18820,.F.);
#78116=ADVANCED_FACE('',(#22686),#18821,.F.);
#78117=ADVANCED_FACE('',(#22687),#18822,.F.);
#78118=ADVANCED_FACE('',(#22688),#18823,.F.);
#78119=ADVANCED_FACE('',(#22689),#18824,.F.);
#78120=ADVANCED_FACE('',(#22690),#18825,.F.);
#78121=ADVANCED_FACE('',(#22691),#18826,.F.);
#78122=ADVANCED_FACE('',(#22692),#18827,.F.);
#78123=ADVANCED_FACE('',(#22693),#18828,.F.);
#78124=ADVANCED_FACE('',(#22694),#18829,.F.);
#78125=ADVANCED_FACE('',(#22695),#18830,.F.);
#78126=ADVANCED_FACE('',(#22696),#18831,.F.);
#78127=ADVANCED_FACE('',(#22697),#18832,.F.);
#78128=ADVANCED_FACE('',(#22698),#18833,.F.);
#78129=ADVANCED_FACE('',(#22699),#18834,.F.);
#78130=ADVANCED_FACE('',(#22700),#18835,.F.);
#78131=ADVANCED_FACE('',(#22701),#18836,.F.);
#78132=ADVANCED_FACE('',(#22702),#18837,.F.);
#78133=ADVANCED_FACE('',(#22703),#18838,.F.);
#78134=ADVANCED_FACE('',(#22704),#18839,.F.);
#78135=ADVANCED_FACE('',(#22705),#18840,.F.);
#78136=ADVANCED_FACE('',(#22706),#18841,.F.);
#78137=ADVANCED_FACE('',(#22707),#18842,.F.);
#78138=ADVANCED_FACE('',(#22708),#18843,.F.);
#78139=ADVANCED_FACE('',(#22709),#18844,.F.);
#78140=ADVANCED_FACE('',(#22710),#18845,.F.);
#78141=ADVANCED_FACE('',(#22711),#18846,.F.);
#78142=ADVANCED_FACE('',(#22712),#18847,.F.);
#78143=ADVANCED_FACE('',(#22713),#18848,.F.);
#78144=ADVANCED_FACE('',(#22714),#18849,.F.);
#78145=ADVANCED_FACE('',(#22715),#18850,.F.);
#78146=ADVANCED_FACE('',(#22716),#18851,.F.);
#78147=ADVANCED_FACE('',(#22717),#18852,.F.);
#78148=ADVANCED_FACE('',(#22718),#18853,.F.);
#78149=ADVANCED_FACE('',(#22719),#18854,.F.);
#78150=ADVANCED_FACE('',(#22720),#18855,.F.);
#78151=ADVANCED_FACE('',(#22721),#18856,.F.);
#78152=ADVANCED_FACE('',(#22722),#18857,.F.);
#78153=ADVANCED_FACE('',(#22723),#18858,.F.);
#78154=ADVANCED_FACE('',(#22724),#18859,.F.);
#78155=ADVANCED_FACE('',(#22725),#18860,.F.);
#78156=ADVANCED_FACE('',(#22726),#18861,.F.);
#78157=ADVANCED_FACE('',(#22727),#18862,.F.);
#78158=ADVANCED_FACE('',(#22728),#18863,.F.);
#78159=ADVANCED_FACE('',(#22729),#18864,.F.);
#78160=ADVANCED_FACE('',(#22730),#18865,.F.);
#78161=ADVANCED_FACE('',(#22731),#18866,.F.);
#78162=ADVANCED_FACE('',(#22732),#18867,.F.);
#78163=ADVANCED_FACE('',(#22733),#18868,.F.);
#78164=ADVANCED_FACE('',(#22734),#18869,.F.);
#78165=ADVANCED_FACE('',(#22735),#18870,.F.);
#78166=ADVANCED_FACE('',(#22736),#18871,.F.);
#78167=ADVANCED_FACE('',(#22737),#18872,.F.);
#78168=ADVANCED_FACE('',(#22738),#18873,.F.);
#78169=ADVANCED_FACE('',(#22739),#18874,.F.);
#78170=ADVANCED_FACE('',(#22740),#18875,.F.);
#78171=ADVANCED_FACE('',(#22741),#18876,.F.);
#78172=ADVANCED_FACE('',(#22742),#18877,.F.);
#78173=ADVANCED_FACE('',(#22743),#18878,.F.);
#78174=ADVANCED_FACE('',(#22744),#18879,.F.);
#78175=ADVANCED_FACE('',(#22745),#18880,.F.);
#78176=ADVANCED_FACE('',(#22746),#18881,.F.);
#78177=ADVANCED_FACE('',(#22747),#18882,.F.);
#78178=ADVANCED_FACE('',(#22748),#18883,.F.);
#78179=ADVANCED_FACE('',(#22749),#18884,.F.);
#78180=ADVANCED_FACE('',(#22750),#18885,.F.);
#78181=ADVANCED_FACE('',(#22751),#18886,.F.);
#78182=ADVANCED_FACE('',(#22752),#18887,.F.);
#78183=ADVANCED_FACE('',(#22753),#18888,.F.);
#78184=ADVANCED_FACE('',(#22754),#18889,.F.);
#78185=ADVANCED_FACE('',(#22755),#18890,.F.);
#78186=ADVANCED_FACE('',(#22756),#18891,.F.);
#78187=ADVANCED_FACE('',(#22757),#18892,.F.);
#78188=ADVANCED_FACE('',(#22758),#18893,.F.);
#78189=ADVANCED_FACE('',(#22759),#18894,.F.);
#78190=ADVANCED_FACE('',(#22760),#18895,.F.);
#78191=ADVANCED_FACE('',(#22761),#18896,.F.);
#78192=ADVANCED_FACE('',(#22762),#18897,.F.);
#78193=ADVANCED_FACE('',(#22763),#18898,.F.);
#78194=ADVANCED_FACE('',(#22764),#18899,.F.);
#78195=ADVANCED_FACE('',(#22765),#18900,.F.);
#78196=ADVANCED_FACE('',(#22766),#18901,.F.);
#78197=ADVANCED_FACE('',(#22767),#18902,.F.);
#78198=ADVANCED_FACE('',(#22768),#18903,.F.);
#78199=ADVANCED_FACE('',(#22769),#18904,.F.);
#78200=ADVANCED_FACE('',(#22770),#18905,.F.);
#78201=ADVANCED_FACE('',(#22771),#18906,.F.);
#78202=ADVANCED_FACE('',(#22772),#18907,.F.);
#78203=ADVANCED_FACE('',(#22773),#18908,.F.);
#78204=ADVANCED_FACE('',(#22774),#18909,.F.);
#78205=ADVANCED_FACE('',(#22775),#18910,.F.);
#78206=ADVANCED_FACE('',(#22776),#18911,.F.);
#78207=ADVANCED_FACE('',(#22777),#18912,.F.);
#78208=ADVANCED_FACE('',(#22778),#18913,.F.);
#78209=ADVANCED_FACE('',(#22779),#18914,.F.);
#78210=ADVANCED_FACE('',(#22780),#18915,.F.);
#78211=ADVANCED_FACE('',(#22781),#18916,.F.);
#78212=ADVANCED_FACE('',(#22782),#18917,.F.);
#78213=ADVANCED_FACE('',(#22783),#18918,.F.);
#78214=ADVANCED_FACE('',(#22784),#18919,.F.);
#78215=ADVANCED_FACE('',(#22785),#18920,.F.);
#78216=ADVANCED_FACE('',(#22786),#18921,.F.);
#78217=ADVANCED_FACE('',(#22787),#18922,.F.);
#78218=ADVANCED_FACE('',(#22788),#18923,.F.);
#78219=ADVANCED_FACE('',(#22789),#18924,.F.);
#78220=ADVANCED_FACE('',(#22790),#18925,.F.);
#78221=ADVANCED_FACE('',(#22791),#18926,.F.);
#78222=ADVANCED_FACE('',(#22792),#18927,.F.);
#78223=ADVANCED_FACE('',(#22793),#18928,.F.);
#78224=ADVANCED_FACE('',(#22794),#18929,.F.);
#78225=ADVANCED_FACE('',(#22795),#18930,.F.);
#78226=ADVANCED_FACE('',(#22796),#18931,.F.);
#78227=ADVANCED_FACE('',(#22797),#18932,.F.);
#78228=ADVANCED_FACE('',(#22798),#18933,.F.);
#78229=ADVANCED_FACE('',(#22799),#18934,.F.);
#78230=ADVANCED_FACE('',(#22800),#18935,.F.);
#78231=ADVANCED_FACE('',(#22801),#18936,.F.);
#78232=ADVANCED_FACE('',(#22802),#18937,.F.);
#78233=ADVANCED_FACE('',(#22803),#18938,.F.);
#78234=ADVANCED_FACE('',(#22804),#18939,.F.);
#78235=ADVANCED_FACE('',(#22805),#18940,.F.);
#78236=ADVANCED_FACE('',(#22806),#18941,.F.);
#78237=ADVANCED_FACE('',(#22807),#18942,.F.);
#78238=ADVANCED_FACE('',(#22808),#18943,.F.);
#78239=ADVANCED_FACE('',(#22809),#18944,.F.);
#78240=ADVANCED_FACE('',(#22810),#18945,.F.);
#78241=ADVANCED_FACE('',(#22811),#18946,.F.);
#78242=ADVANCED_FACE('',(#22812),#18947,.F.);
#78243=ADVANCED_FACE('',(#22813),#18948,.F.);
#78244=ADVANCED_FACE('',(#22814),#18949,.F.);
#78245=ADVANCED_FACE('',(#22815),#18950,.F.);
#78246=ADVANCED_FACE('',(#22816),#18951,.F.);
#78247=ADVANCED_FACE('',(#22817),#18952,.F.);
#78248=ADVANCED_FACE('',(#22818),#18953,.F.);
#78249=ADVANCED_FACE('',(#22819),#18954,.F.);
#78250=ADVANCED_FACE('',(#22820),#18955,.F.);
#78251=ADVANCED_FACE('',(#22821),#18956,.F.);
#78252=ADVANCED_FACE('',(#22822),#18957,.F.);
#78253=ADVANCED_FACE('',(#22823),#18958,.F.);
#78254=ADVANCED_FACE('',(#22824),#18959,.F.);
#78255=ADVANCED_FACE('',(#22825),#18960,.F.);
#78256=ADVANCED_FACE('',(#22826),#18961,.F.);
#78257=ADVANCED_FACE('',(#22827),#18962,.F.);
#78258=ADVANCED_FACE('',(#22828),#18963,.F.);
#78259=ADVANCED_FACE('',(#22829),#18964,.F.);
#78260=ADVANCED_FACE('',(#22830),#18965,.F.);
#78261=ADVANCED_FACE('',(#22831),#18966,.F.);
#78262=ADVANCED_FACE('',(#22832),#18967,.F.);
#78263=ADVANCED_FACE('',(#22833),#18968,.F.);
#78264=ADVANCED_FACE('',(#22834),#18969,.F.);
#78265=ADVANCED_FACE('',(#22835),#18970,.F.);
#78266=ADVANCED_FACE('',(#22836),#18971,.F.);
#78267=ADVANCED_FACE('',(#22837),#18972,.F.);
#78268=ADVANCED_FACE('',(#22838),#18973,.F.);
#78269=ADVANCED_FACE('',(#22839),#18974,.F.);
#78270=ADVANCED_FACE('',(#22840),#18975,.F.);
#78271=ADVANCED_FACE('',(#22841),#18976,.F.);
#78272=ADVANCED_FACE('',(#22842),#18977,.F.);
#78273=ADVANCED_FACE('',(#22843),#18978,.F.);
#78274=ADVANCED_FACE('',(#22844),#18979,.F.);
#78275=ADVANCED_FACE('',(#22845),#18980,.F.);
#78276=ADVANCED_FACE('',(#22846),#18981,.F.);
#78277=ADVANCED_FACE('',(#22847),#18982,.F.);
#78278=ADVANCED_FACE('',(#22848),#18983,.F.);
#78279=ADVANCED_FACE('',(#22849),#18984,.F.);
#78280=ADVANCED_FACE('',(#22850),#18985,.F.);
#78281=ADVANCED_FACE('',(#22851),#18986,.F.);
#78282=ADVANCED_FACE('',(#22852),#18987,.F.);
#78283=ADVANCED_FACE('',(#22853),#18988,.F.);
#78284=ADVANCED_FACE('',(#22854),#18989,.F.);
#78285=ADVANCED_FACE('',(#22855),#18990,.F.);
#78286=ADVANCED_FACE('',(#22856),#18991,.F.);
#78287=ADVANCED_FACE('',(#22857),#18992,.F.);
#78288=ADVANCED_FACE('',(#22858),#18993,.F.);
#78289=ADVANCED_FACE('',(#22859),#18994,.F.);
#78290=ADVANCED_FACE('',(#22860),#18995,.F.);
#78291=ADVANCED_FACE('',(#22861),#18996,.F.);
#78292=ADVANCED_FACE('',(#22862),#18997,.F.);
#78293=ADVANCED_FACE('',(#22863),#18998,.F.);
#78294=ADVANCED_FACE('',(#22864),#18999,.F.);
#78295=ADVANCED_FACE('',(#22865),#19000,.F.);
#78296=ADVANCED_FACE('',(#22866),#19001,.F.);
#78297=ADVANCED_FACE('',(#22867),#19002,.F.);
#78298=ADVANCED_FACE('',(#22868),#19003,.F.);
#78299=ADVANCED_FACE('',(#22869),#19004,.F.);
#78300=ADVANCED_FACE('',(#22870),#19005,.F.);
#78301=ADVANCED_FACE('',(#22871),#19006,.F.);
#78302=ADVANCED_FACE('',(#22872),#19007,.F.);
#78303=ADVANCED_FACE('',(#22873),#19008,.F.);
#78304=ADVANCED_FACE('',(#22874),#19009,.F.);
#78305=ADVANCED_FACE('',(#22875),#19010,.F.);
#78306=ADVANCED_FACE('',(#22876),#19011,.F.);
#78307=ADVANCED_FACE('',(#22877),#19012,.F.);
#78308=ADVANCED_FACE('',(#22878),#19013,.F.);
#78309=ADVANCED_FACE('',(#22879),#19014,.F.);
#78310=ADVANCED_FACE('',(#22880),#19015,.F.);
#78311=ADVANCED_FACE('',(#22881),#19016,.F.);
#78312=ADVANCED_FACE('',(#22882),#19017,.F.);
#78313=ADVANCED_FACE('',(#22883),#19018,.F.);
#78314=ADVANCED_FACE('',(#22884),#19019,.F.);
#78315=ADVANCED_FACE('',(#22885),#19020,.F.);
#78316=ADVANCED_FACE('',(#22886),#19021,.F.);
#78317=ADVANCED_FACE('',(#22887),#19022,.F.);
#78318=ADVANCED_FACE('',(#22888),#19023,.F.);
#78319=ADVANCED_FACE('',(#22889),#19024,.F.);
#78320=ADVANCED_FACE('',(#22890),#19025,.F.);
#78321=ADVANCED_FACE('',(#22891),#19026,.F.);
#78322=ADVANCED_FACE('',(#22892),#19027,.F.);
#78323=ADVANCED_FACE('',(#22893),#19028,.F.);
#78324=ADVANCED_FACE('',(#22894),#19029,.F.);
#78325=ADVANCED_FACE('',(#22895),#19030,.F.);
#78326=ADVANCED_FACE('',(#22896),#19031,.F.);
#78327=ADVANCED_FACE('',(#22897),#19032,.F.);
#78328=ADVANCED_FACE('',(#22898),#19033,.F.);
#78329=ADVANCED_FACE('',(#22899),#19034,.F.);
#78330=ADVANCED_FACE('',(#22900),#19035,.F.);
#78331=ADVANCED_FACE('',(#22901),#19036,.F.);
#78332=ADVANCED_FACE('',(#22902),#19037,.F.);
#78333=ADVANCED_FACE('',(#22903),#19038,.F.);
#78334=ADVANCED_FACE('',(#22904),#19039,.F.);
#78335=ADVANCED_FACE('',(#22905),#19040,.F.);
#78336=ADVANCED_FACE('',(#22906),#19041,.F.);
#78337=ADVANCED_FACE('',(#22907),#19042,.F.);
#78338=ADVANCED_FACE('',(#22908),#19043,.F.);
#78339=ADVANCED_FACE('',(#22909),#19044,.F.);
#78340=ADVANCED_FACE('',(#22910),#19045,.F.);
#78341=ADVANCED_FACE('',(#22911),#19046,.F.);
#78342=ADVANCED_FACE('',(#22912),#19047,.F.);
#78343=ADVANCED_FACE('',(#22913),#19048,.F.);
#78344=ADVANCED_FACE('',(#22914),#19049,.F.);
#78345=ADVANCED_FACE('',(#22915),#19050,.F.);
#78346=ADVANCED_FACE('',(#22916),#19051,.F.);
#78347=ADVANCED_FACE('',(#22917),#19052,.F.);
#78348=ADVANCED_FACE('',(#22918),#19053,.F.);
#78349=ADVANCED_FACE('',(#22919),#19054,.F.);
#78350=ADVANCED_FACE('',(#22920),#19055,.F.);
#78351=ADVANCED_FACE('',(#22921),#19056,.F.);
#78352=ADVANCED_FACE('',(#22922),#19057,.F.);
#78353=ADVANCED_FACE('',(#22923),#19058,.F.);
#78354=ADVANCED_FACE('',(#22924),#19059,.F.);
#78355=ADVANCED_FACE('',(#22925),#19060,.F.);
#78356=ADVANCED_FACE('',(#22926),#19061,.F.);
#78357=ADVANCED_FACE('',(#22927),#19062,.F.);
#78358=ADVANCED_FACE('',(#22928),#19063,.F.);
#78359=ADVANCED_FACE('',(#22929),#19064,.F.);
#78360=ADVANCED_FACE('',(#22930),#19065,.F.);
#78361=ADVANCED_FACE('',(#22931),#19066,.F.);
#78362=ADVANCED_FACE('',(#22932),#19067,.F.);
#78363=ADVANCED_FACE('',(#22933),#19068,.F.);
#78364=ADVANCED_FACE('',(#22934),#19069,.F.);
#78365=ADVANCED_FACE('',(#22935),#19070,.F.);
#78366=ADVANCED_FACE('',(#22936),#19071,.F.);
#78367=ADVANCED_FACE('',(#22937),#19072,.F.);
#78368=ADVANCED_FACE('',(#22938),#19073,.F.);
#78369=ADVANCED_FACE('',(#22939),#19074,.F.);
#78370=ADVANCED_FACE('',(#22940),#19075,.F.);
#78371=ADVANCED_FACE('',(#22941),#19076,.F.);
#78372=ADVANCED_FACE('',(#22942),#19077,.F.);
#78373=ADVANCED_FACE('',(#22943),#19078,.F.);
#78374=ADVANCED_FACE('',(#22944),#19079,.F.);
#78375=ADVANCED_FACE('',(#22945),#19080,.F.);
#78376=ADVANCED_FACE('',(#22946),#19081,.F.);
#78377=ADVANCED_FACE('',(#22947),#19082,.F.);
#78378=ADVANCED_FACE('',(#22948),#19083,.F.);
#78379=ADVANCED_FACE('',(#22949),#19084,.F.);
#78380=ADVANCED_FACE('',(#22950),#19085,.F.);
#78381=ADVANCED_FACE('',(#22951),#19086,.F.);
#78382=ADVANCED_FACE('',(#22952),#19087,.F.);
#78383=ADVANCED_FACE('',(#22953),#19088,.F.);
#78384=ADVANCED_FACE('',(#22954),#19089,.F.);
#78385=ADVANCED_FACE('',(#22955),#19090,.F.);
#78386=ADVANCED_FACE('',(#22956),#19091,.F.);
#78387=ADVANCED_FACE('',(#22957),#19092,.F.);
#78388=ADVANCED_FACE('',(#22958),#19093,.F.);
#78389=ADVANCED_FACE('',(#22959),#19094,.F.);
#78390=ADVANCED_FACE('',(#22960),#19095,.F.);
#78391=ADVANCED_FACE('',(#22961),#19096,.F.);
#78392=ADVANCED_FACE('',(#22962),#19097,.F.);
#78393=ADVANCED_FACE('',(#22963),#19098,.F.);
#78394=ADVANCED_FACE('',(#22964),#19099,.F.);
#78395=ADVANCED_FACE('',(#22965),#19100,.F.);
#78396=ADVANCED_FACE('',(#22966),#19101,.F.);
#78397=ADVANCED_FACE('',(#22967),#19102,.F.);
#78398=ADVANCED_FACE('',(#22968),#19103,.F.);
#78399=ADVANCED_FACE('',(#22969),#19104,.F.);
#78400=ADVANCED_FACE('',(#22970),#19105,.F.);
#78401=ADVANCED_FACE('',(#22971),#19106,.F.);
#78402=ADVANCED_FACE('',(#22972),#19107,.F.);
#78403=ADVANCED_FACE('',(#22973),#19108,.F.);
#78404=ADVANCED_FACE('',(#22974),#19109,.F.);
#78405=ADVANCED_FACE('',(#22975),#19110,.F.);
#78406=ADVANCED_FACE('',(#22976),#19111,.F.);
#78407=ADVANCED_FACE('',(#22977),#19112,.F.);
#78408=ADVANCED_FACE('',(#22978),#19113,.F.);
#78409=ADVANCED_FACE('',(#22979),#19114,.F.);
#78410=ADVANCED_FACE('',(#22980),#19115,.F.);
#78411=ADVANCED_FACE('',(#22981),#19116,.F.);
#78412=ADVANCED_FACE('',(#22982),#19117,.F.);
#78413=ADVANCED_FACE('',(#22983),#19118,.F.);
#78414=ADVANCED_FACE('',(#22984),#19119,.F.);
#78415=ADVANCED_FACE('',(#22985),#19120,.F.);
#78416=ADVANCED_FACE('',(#22986),#19121,.F.);
#78417=ADVANCED_FACE('',(#22987),#19122,.F.);
#78418=ADVANCED_FACE('',(#22988),#19123,.F.);
#78419=ADVANCED_FACE('',(#22989),#19124,.F.);
#78420=ADVANCED_FACE('',(#22990),#19125,.F.);
#78421=ADVANCED_FACE('',(#22991),#19126,.F.);
#78422=ADVANCED_FACE('',(#22992),#19127,.F.);
#78423=ADVANCED_FACE('',(#22993),#19128,.F.);
#78424=ADVANCED_FACE('',(#22994),#19129,.F.);
#78425=ADVANCED_FACE('',(#22995),#19130,.F.);
#78426=ADVANCED_FACE('',(#22996),#19131,.F.);
#78427=ADVANCED_FACE('',(#22997),#19132,.F.);
#78428=ADVANCED_FACE('',(#22998),#19133,.F.);
#78429=ADVANCED_FACE('',(#22999),#19134,.F.);
#78430=ADVANCED_FACE('',(#23000),#19135,.F.);
#78431=ADVANCED_FACE('',(#23001),#19136,.F.);
#78432=ADVANCED_FACE('',(#23002),#19137,.F.);
#78433=ADVANCED_FACE('',(#23003),#19138,.F.);
#78434=ADVANCED_FACE('',(#23004),#19139,.F.);
#78435=ADVANCED_FACE('',(#23005),#19140,.F.);
#78436=ADVANCED_FACE('',(#23006),#19141,.F.);
#78437=ADVANCED_FACE('',(#23007),#19142,.F.);
#78438=ADVANCED_FACE('',(#23008),#19143,.F.);
#78439=ADVANCED_FACE('',(#23009),#19144,.F.);
#78440=ADVANCED_FACE('',(#23010),#19145,.F.);
#78441=ADVANCED_FACE('',(#23011),#19146,.F.);
#78442=ADVANCED_FACE('',(#23012),#19147,.F.);
#78443=ADVANCED_FACE('',(#23013),#19148,.F.);
#78444=ADVANCED_FACE('',(#23014),#19149,.F.);
#78445=ADVANCED_FACE('',(#23015),#19150,.F.);
#78446=ADVANCED_FACE('',(#23016),#19151,.F.);
#78447=ADVANCED_FACE('',(#23017),#19152,.F.);
#78448=ADVANCED_FACE('',(#23018),#19153,.F.);
#78449=ADVANCED_FACE('',(#23019),#19154,.F.);
#78450=ADVANCED_FACE('',(#23020),#19155,.F.);
#78451=ADVANCED_FACE('',(#23021),#19156,.F.);
#78452=ADVANCED_FACE('',(#23022),#19157,.F.);
#78453=ADVANCED_FACE('',(#23023),#19158,.F.);
#78454=ADVANCED_FACE('',(#23024),#19159,.F.);
#78455=ADVANCED_FACE('',(#23025),#19160,.F.);
#78456=ADVANCED_FACE('',(#23026),#19161,.F.);
#78457=ADVANCED_FACE('',(#23027),#19162,.F.);
#78458=ADVANCED_FACE('',(#23028),#19163,.F.);
#78459=ADVANCED_FACE('',(#23029),#19164,.F.);
#78460=ADVANCED_FACE('',(#23030),#19165,.F.);
#78461=ADVANCED_FACE('',(#23031),#19166,.F.);
#78462=ADVANCED_FACE('',(#23032),#19167,.F.);
#78463=ADVANCED_FACE('',(#23033),#19168,.F.);
#78464=ADVANCED_FACE('',(#23034),#19169,.F.);
#78465=ADVANCED_FACE('',(#23035),#19170,.F.);
#78466=ADVANCED_FACE('',(#23036),#19171,.F.);
#78467=ADVANCED_FACE('',(#23037),#19172,.F.);
#78468=ADVANCED_FACE('',(#23038),#19173,.F.);
#78469=ADVANCED_FACE('',(#23039),#19174,.F.);
#78470=ADVANCED_FACE('',(#23040),#19175,.F.);
#78471=ADVANCED_FACE('',(#23041),#19176,.F.);
#78472=ADVANCED_FACE('',(#23042),#19177,.F.);
#78473=ADVANCED_FACE('',(#23043),#19178,.F.);
#78474=ADVANCED_FACE('',(#23044),#19179,.F.);
#78475=ADVANCED_FACE('',(#23045),#19180,.F.);
#78476=ADVANCED_FACE('',(#23046),#19181,.F.);
#78477=ADVANCED_FACE('',(#23047),#19182,.F.);
#78478=ADVANCED_FACE('',(#23048),#19183,.F.);
#78479=ADVANCED_FACE('',(#23049),#19184,.F.);
#78480=ADVANCED_FACE('',(#23050),#19185,.F.);
#78481=ADVANCED_FACE('',(#23051),#19186,.F.);
#78482=ADVANCED_FACE('',(#23052),#19187,.F.);
#78483=ADVANCED_FACE('',(#23053),#19188,.F.);
#78484=ADVANCED_FACE('',(#23054),#19189,.F.);
#78485=ADVANCED_FACE('',(#23055),#19190,.F.);
#78486=ADVANCED_FACE('',(#23056),#19191,.F.);
#78487=ADVANCED_FACE('',(#23057),#19192,.F.);
#78488=ADVANCED_FACE('',(#23058),#19193,.F.);
#78489=ADVANCED_FACE('',(#23059),#19194,.F.);
#78490=ADVANCED_FACE('',(#23060),#19195,.F.);
#78491=ADVANCED_FACE('',(#23061),#19196,.F.);
#78492=ADVANCED_FACE('',(#23062),#19197,.F.);
#78493=ADVANCED_FACE('',(#23063),#19198,.F.);
#78494=ADVANCED_FACE('',(#23064),#19199,.F.);
#78495=ADVANCED_FACE('',(#23065),#19200,.F.);
#78496=ADVANCED_FACE('',(#23066),#19201,.F.);
#78497=ADVANCED_FACE('',(#23067),#19202,.F.);
#78498=ADVANCED_FACE('',(#23068),#19203,.F.);
#78499=ADVANCED_FACE('',(#23069),#19204,.F.);
#78500=ADVANCED_FACE('',(#23070),#19205,.F.);
#78501=ADVANCED_FACE('',(#23071),#19206,.F.);
#78502=ADVANCED_FACE('',(#23072),#19207,.F.);
#78503=ADVANCED_FACE('',(#23073),#19208,.F.);
#78504=ADVANCED_FACE('',(#23074),#19209,.F.);
#78505=ADVANCED_FACE('',(#23075),#19210,.F.);
#78506=ADVANCED_FACE('',(#23076),#19211,.F.);
#78507=ADVANCED_FACE('',(#23077),#19212,.F.);
#78508=ADVANCED_FACE('',(#23078),#19213,.F.);
#78509=ADVANCED_FACE('',(#23079),#19214,.F.);
#78510=ADVANCED_FACE('',(#23080),#19215,.F.);
#78511=ADVANCED_FACE('',(#23081),#19216,.F.);
#78512=ADVANCED_FACE('',(#23082),#19217,.F.);
#78513=ADVANCED_FACE('',(#23083),#19218,.F.);
#78514=ADVANCED_FACE('',(#23084),#19219,.F.);
#78515=ADVANCED_FACE('',(#23085),#19220,.F.);
#78516=ADVANCED_FACE('',(#23086),#19221,.F.);
#78517=ADVANCED_FACE('',(#23087),#19222,.F.);
#78518=ADVANCED_FACE('',(#23088),#19223,.F.);
#78519=ADVANCED_FACE('',(#23089),#19224,.F.);
#78520=ADVANCED_FACE('',(#23090),#19225,.F.);
#78521=ADVANCED_FACE('',(#23091),#19226,.F.);
#78522=ADVANCED_FACE('',(#23092),#19227,.F.);
#78523=ADVANCED_FACE('',(#23093),#19228,.F.);
#78524=ADVANCED_FACE('',(#23094),#19229,.F.);
#78525=ADVANCED_FACE('',(#23095),#19230,.F.);
#78526=ADVANCED_FACE('',(#23096),#19231,.F.);
#78527=ADVANCED_FACE('',(#23097),#19232,.F.);
#78528=ADVANCED_FACE('',(#23098),#19233,.F.);
#78529=ADVANCED_FACE('',(#23099),#19234,.F.);
#78530=ADVANCED_FACE('',(#23100),#19235,.F.);
#78531=ADVANCED_FACE('',(#23101),#19236,.F.);
#78532=ADVANCED_FACE('',(#23102),#19237,.F.);
#78533=ADVANCED_FACE('',(#23103),#19238,.F.);
#78534=ADVANCED_FACE('',(#23104),#19239,.F.);
#78535=ADVANCED_FACE('',(#23105),#19240,.F.);
#78536=ADVANCED_FACE('',(#23106),#19241,.F.);
#78537=ADVANCED_FACE('',(#23107),#19242,.F.);
#78538=ADVANCED_FACE('',(#23108),#19243,.F.);
#78539=ADVANCED_FACE('',(#23109),#19244,.F.);
#78540=ADVANCED_FACE('',(#23110),#19245,.F.);
#78541=ADVANCED_FACE('',(#23111),#19246,.F.);
#78542=ADVANCED_FACE('',(#23112),#19247,.F.);
#78543=ADVANCED_FACE('',(#23113),#19248,.F.);
#78544=ADVANCED_FACE('',(#23114),#19249,.F.);
#78545=ADVANCED_FACE('',(#23115),#19250,.F.);
#78546=ADVANCED_FACE('',(#23116),#19251,.F.);
#78547=ADVANCED_FACE('',(#23117),#19252,.F.);
#78548=ADVANCED_FACE('',(#23118),#19253,.F.);
#78549=ADVANCED_FACE('',(#23119),#19254,.F.);
#78550=ADVANCED_FACE('',(#23120),#19255,.F.);
#78551=ADVANCED_FACE('',(#23121),#19256,.F.);
#78552=ADVANCED_FACE('',(#23122),#19257,.F.);
#78553=ADVANCED_FACE('',(#23123),#19258,.F.);
#78554=ADVANCED_FACE('',(#23124),#19259,.F.);
#78555=ADVANCED_FACE('',(#23125),#19260,.F.);
#78556=ADVANCED_FACE('',(#23126),#19261,.F.);
#78557=ADVANCED_FACE('',(#23127),#19262,.F.);
#78558=ADVANCED_FACE('',(#23128),#19263,.F.);
#78559=ADVANCED_FACE('',(#23129),#19264,.F.);
#78560=ADVANCED_FACE('',(#23130),#19265,.F.);
#78561=ADVANCED_FACE('',(#23131),#19266,.F.);
#78562=ADVANCED_FACE('',(#23132),#19267,.F.);
#78563=ADVANCED_FACE('',(#23133),#19268,.F.);
#78564=ADVANCED_FACE('',(#23134),#19269,.F.);
#78565=ADVANCED_FACE('',(#23135),#19270,.F.);
#78566=ADVANCED_FACE('',(#23136),#19271,.F.);
#78567=ADVANCED_FACE('',(#23137),#19272,.F.);
#78568=ADVANCED_FACE('',(#23138),#19273,.F.);
#78569=ADVANCED_FACE('',(#23139),#19274,.F.);
#78570=ADVANCED_FACE('',(#23140),#19275,.F.);
#78571=ADVANCED_FACE('',(#23141),#19276,.F.);
#78572=ADVANCED_FACE('',(#23142),#19277,.F.);
#78573=ADVANCED_FACE('',(#23143),#19278,.F.);
#78574=ADVANCED_FACE('',(#23144),#19279,.F.);
#78575=ADVANCED_FACE('',(#23145),#19280,.F.);
#78576=ADVANCED_FACE('',(#23146),#19281,.F.);
#78577=ADVANCED_FACE('',(#23147),#19282,.F.);
#78578=ADVANCED_FACE('',(#23148),#19283,.F.);
#78579=ADVANCED_FACE('',(#23149),#19284,.F.);
#78580=ADVANCED_FACE('',(#23150),#19285,.F.);
#78581=ADVANCED_FACE('',(#23151),#19286,.F.);
#78582=ADVANCED_FACE('',(#23152),#19287,.F.);
#78583=ADVANCED_FACE('',(#23153),#19288,.F.);
#78584=ADVANCED_FACE('',(#23154),#19289,.F.);
#78585=ADVANCED_FACE('',(#23155),#19290,.F.);
#78586=ADVANCED_FACE('',(#23156),#19291,.F.);
#78587=ADVANCED_FACE('',(#23157),#19292,.F.);
#78588=ADVANCED_FACE('',(#23158),#19293,.F.);
#78589=ADVANCED_FACE('',(#23159),#19294,.F.);
#78590=ADVANCED_FACE('',(#23160),#19295,.F.);
#78591=ADVANCED_FACE('',(#23161),#19296,.F.);
#78592=ADVANCED_FACE('',(#23162),#19297,.F.);
#78593=ADVANCED_FACE('',(#23163),#19298,.F.);
#78594=ADVANCED_FACE('',(#23164),#19299,.F.);
#78595=ADVANCED_FACE('',(#23165),#19300,.F.);
#78596=ADVANCED_FACE('',(#23166),#19301,.F.);
#78597=ADVANCED_FACE('',(#23167),#19302,.F.);
#78598=ADVANCED_FACE('',(#23168),#19303,.F.);
#78599=ADVANCED_FACE('',(#23169),#19304,.F.);
#78600=ADVANCED_FACE('',(#23170),#19305,.F.);
#78601=ADVANCED_FACE('',(#23171),#19306,.F.);
#78602=ADVANCED_FACE('',(#23172),#19307,.F.);
#78603=ADVANCED_FACE('',(#23173),#19308,.F.);
#78604=ADVANCED_FACE('',(#23174),#19309,.F.);
#78605=ADVANCED_FACE('',(#23175),#19310,.F.);
#78606=ADVANCED_FACE('',(#23176),#19311,.F.);
#78607=ADVANCED_FACE('',(#23177),#19312,.F.);
#78608=ADVANCED_FACE('',(#23178),#19313,.F.);
#78609=ADVANCED_FACE('',(#23179),#19314,.F.);
#78610=ADVANCED_FACE('',(#23180),#19315,.F.);
#78611=ADVANCED_FACE('',(#23181),#19316,.F.);
#78612=ADVANCED_FACE('',(#23182),#19317,.F.);
#78613=ADVANCED_FACE('',(#23183),#19318,.F.);
#78614=ADVANCED_FACE('',(#23184),#19319,.F.);
#78615=ADVANCED_FACE('',(#23185),#19320,.F.);
#78616=ADVANCED_FACE('',(#23186),#19321,.F.);
#78617=ADVANCED_FACE('',(#23187),#19322,.F.);
#78618=ADVANCED_FACE('',(#23188),#19323,.F.);
#78619=ADVANCED_FACE('',(#23189),#19324,.F.);
#78620=ADVANCED_FACE('',(#23190),#19325,.F.);
#78621=ADVANCED_FACE('',(#23191),#19326,.F.);
#78622=ADVANCED_FACE('',(#23192),#19327,.F.);
#78623=ADVANCED_FACE('',(#23193),#19328,.F.);
#78624=ADVANCED_FACE('',(#23194),#19329,.F.);
#78625=ADVANCED_FACE('',(#23195),#19330,.F.);
#78626=ADVANCED_FACE('',(#23196),#19331,.F.);
#78627=ADVANCED_FACE('',(#23197),#19332,.F.);
#78628=ADVANCED_FACE('',(#23198),#19333,.F.);
#78629=ADVANCED_FACE('',(#23199),#19334,.F.);
#78630=ADVANCED_FACE('',(#23200),#19335,.F.);
#78631=ADVANCED_FACE('',(#23201),#19336,.F.);
#78632=ADVANCED_FACE('',(#23202),#19337,.F.);
#78633=ADVANCED_FACE('',(#23203),#19338,.F.);
#78634=ADVANCED_FACE('',(#23204),#19339,.F.);
#78635=ADVANCED_FACE('',(#23205),#19340,.F.);
#78636=ADVANCED_FACE('',(#23206),#19341,.F.);
#78637=ADVANCED_FACE('',(#23207),#19342,.F.);
#78638=ADVANCED_FACE('',(#23208),#19343,.F.);
#78639=ADVANCED_FACE('',(#23209),#19344,.F.);
#78640=ADVANCED_FACE('',(#23210),#19345,.F.);
#78641=ADVANCED_FACE('',(#23211),#19346,.F.);
#78642=ADVANCED_FACE('',(#23212),#19347,.F.);
#78643=ADVANCED_FACE('',(#23213),#19348,.F.);
#78644=ADVANCED_FACE('',(#23214),#19349,.F.);
#78645=ADVANCED_FACE('',(#23215),#19350,.F.);
#78646=ADVANCED_FACE('',(#23216),#19351,.F.);
#78647=ADVANCED_FACE('',(#23217),#19352,.F.);
#78648=ADVANCED_FACE('',(#23218),#19353,.F.);
#78649=ADVANCED_FACE('',(#23219),#19354,.F.);
#78650=ADVANCED_FACE('',(#23220),#19355,.F.);
#78651=ADVANCED_FACE('',(#23221),#19356,.F.);
#78652=ADVANCED_FACE('',(#23222),#19357,.F.);
#78653=ADVANCED_FACE('',(#23223),#19358,.F.);
#78654=ADVANCED_FACE('',(#23224),#19359,.F.);
#78655=ADVANCED_FACE('',(#23225),#19360,.F.);
#78656=ADVANCED_FACE('',(#23226),#19361,.F.);
#78657=ADVANCED_FACE('',(#23227),#19362,.F.);
#78658=ADVANCED_FACE('',(#23228),#19363,.F.);
#78659=ADVANCED_FACE('',(#23229),#19364,.F.);
#78660=ADVANCED_FACE('',(#23230),#19365,.F.);
#78661=ADVANCED_FACE('',(#23231),#19366,.F.);
#78662=ADVANCED_FACE('',(#23232),#19367,.F.);
#78663=ADVANCED_FACE('',(#23233),#19368,.F.);
#78664=ADVANCED_FACE('',(#23234),#19369,.F.);
#78665=ADVANCED_FACE('',(#23235),#19370,.F.);
#78666=ADVANCED_FACE('',(#23236),#19371,.F.);
#78667=ADVANCED_FACE('',(#23237),#19372,.F.);
#78668=ADVANCED_FACE('',(#23238),#19373,.F.);
#78669=ADVANCED_FACE('',(#23239),#19374,.F.);
#78670=ADVANCED_FACE('',(#23240),#19375,.F.);
#78671=ADVANCED_FACE('',(#23241),#19376,.F.);
#78672=ADVANCED_FACE('',(#23242),#19377,.F.);
#78673=ADVANCED_FACE('',(#23243),#19378,.F.);
#78674=ADVANCED_FACE('',(#23244),#19379,.F.);
#78675=ADVANCED_FACE('',(#23245),#19380,.F.);
#78676=ADVANCED_FACE('',(#23246),#19381,.F.);
#78677=ADVANCED_FACE('',(#23247),#19382,.F.);
#78678=ADVANCED_FACE('',(#23248),#19383,.F.);
#78679=ADVANCED_FACE('',(#23249),#19384,.F.);
#78680=ADVANCED_FACE('',(#23250),#19385,.F.);
#78681=ADVANCED_FACE('',(#23251),#19386,.F.);
#78682=ADVANCED_FACE('',(#23252),#19387,.F.);
#78683=ADVANCED_FACE('',(#23253),#19388,.F.);
#78684=ADVANCED_FACE('',(#23254),#19389,.F.);
#78685=ADVANCED_FACE('',(#23255),#19390,.F.);
#78686=ADVANCED_FACE('',(#23256),#19391,.F.);
#78687=ADVANCED_FACE('',(#23257),#19392,.F.);
#78688=ADVANCED_FACE('',(#23258),#19393,.F.);
#78689=ADVANCED_FACE('',(#23259),#19394,.F.);
#78690=ADVANCED_FACE('',(#23260),#19395,.F.);
#78691=ADVANCED_FACE('',(#23261),#19396,.F.);
#78692=ADVANCED_FACE('',(#23262),#19397,.F.);
#78693=ADVANCED_FACE('',(#23263),#19398,.F.);
#78694=ADVANCED_FACE('',(#23264),#19399,.F.);
#78695=ADVANCED_FACE('',(#23265),#19400,.F.);
#78696=ADVANCED_FACE('',(#23266),#19401,.F.);
#78697=ADVANCED_FACE('',(#23267),#19402,.F.);
#78698=ADVANCED_FACE('',(#23268),#19403,.F.);
#78699=ADVANCED_FACE('',(#23269),#19404,.F.);
#78700=ADVANCED_FACE('',(#23270),#19405,.F.);
#78701=ADVANCED_FACE('',(#23271),#19406,.F.);
#78702=ADVANCED_FACE('',(#23272),#19407,.F.);
#78703=ADVANCED_FACE('',(#23273),#19408,.F.);
#78704=ADVANCED_FACE('',(#23274),#19409,.F.);
#78705=ADVANCED_FACE('',(#23275),#19410,.F.);
#78706=ADVANCED_FACE('',(#23276),#19411,.F.);
#78707=ADVANCED_FACE('',(#23277),#19412,.F.);
#78708=ADVANCED_FACE('',(#23278),#19413,.F.);
#78709=ADVANCED_FACE('',(#23279),#19414,.F.);
#78710=ADVANCED_FACE('',(#23280),#19415,.F.);
#78711=ADVANCED_FACE('',(#23281),#19416,.F.);
#78712=ADVANCED_FACE('',(#23282),#19417,.F.);
#78713=ADVANCED_FACE('',(#23283),#19418,.F.);
#78714=ADVANCED_FACE('',(#23284),#19419,.F.);
#78715=ADVANCED_FACE('',(#23285),#19420,.F.);
#78716=ADVANCED_FACE('',(#23286),#19421,.F.);
#78717=ADVANCED_FACE('',(#23287),#19422,.F.);
#78718=ADVANCED_FACE('',(#23288),#19423,.F.);
#78719=ADVANCED_FACE('',(#23289),#19424,.F.);
#78720=ADVANCED_FACE('',(#23290),#19425,.F.);
#78721=ADVANCED_FACE('',(#23291),#19426,.F.);
#78722=ADVANCED_FACE('',(#23292),#19427,.F.);
#78723=ADVANCED_FACE('',(#23293),#19428,.F.);
#78724=ADVANCED_FACE('',(#23294),#19429,.F.);
#78725=ADVANCED_FACE('',(#23295),#19430,.F.);
#78726=ADVANCED_FACE('',(#23296),#19431,.F.);
#78727=ADVANCED_FACE('',(#23297),#19432,.F.);
#78728=ADVANCED_FACE('',(#23298),#19433,.F.);
#78729=ADVANCED_FACE('',(#23299),#19434,.F.);
#78730=ADVANCED_FACE('',(#23300),#19435,.F.);
#78731=ADVANCED_FACE('',(#23301),#19436,.F.);
#78732=ADVANCED_FACE('',(#23302),#19437,.F.);
#78733=ADVANCED_FACE('',(#23303),#19438,.F.);
#78734=ADVANCED_FACE('',(#23304),#19439,.F.);
#78735=ADVANCED_FACE('',(#23305),#19440,.F.);
#78736=ADVANCED_FACE('',(#23306),#19441,.F.);
#78737=ADVANCED_FACE('',(#23307),#19442,.F.);
#78738=ADVANCED_FACE('',(#23308),#19443,.F.);
#78739=ADVANCED_FACE('',(#23309),#19444,.F.);
#78740=ADVANCED_FACE('',(#23310),#19445,.F.);
#78741=ADVANCED_FACE('',(#23311),#19446,.F.);
#78742=ADVANCED_FACE('',(#23312),#19447,.F.);
#78743=ADVANCED_FACE('',(#23313),#19448,.F.);
#78744=ADVANCED_FACE('',(#23314),#19449,.F.);
#78745=ADVANCED_FACE('',(#23315),#19450,.F.);
#78746=ADVANCED_FACE('',(#23316),#19451,.F.);
#78747=ADVANCED_FACE('',(#23317),#19452,.F.);
#78748=ADVANCED_FACE('',(#23318),#19453,.F.);
#78749=ADVANCED_FACE('',(#23319),#19454,.F.);
#78750=ADVANCED_FACE('',(#23320),#19455,.F.);
#78751=ADVANCED_FACE('',(#23321),#19456,.F.);
#78752=ADVANCED_FACE('',(#23322),#19457,.F.);
#78753=ADVANCED_FACE('',(#23323),#19458,.F.);
#78754=ADVANCED_FACE('',(#23324),#19459,.F.);
#78755=ADVANCED_FACE('',(#23325),#19460,.F.);
#78756=ADVANCED_FACE('',(#23326),#19461,.F.);
#78757=ADVANCED_FACE('',(#23327),#19462,.F.);
#78758=ADVANCED_FACE('',(#23328),#19463,.F.);
#78759=ADVANCED_FACE('',(#23329),#19464,.F.);
#78760=ADVANCED_FACE('',(#23330),#19465,.F.);
#78761=ADVANCED_FACE('',(#23331),#19466,.F.);
#78762=ADVANCED_FACE('',(#23332),#19467,.F.);
#78763=ADVANCED_FACE('',(#23333),#19468,.F.);
#78764=ADVANCED_FACE('',(#23334),#19469,.F.);
#78765=ADVANCED_FACE('',(#23335),#19470,.F.);
#78766=ADVANCED_FACE('',(#23336),#19471,.F.);
#78767=ADVANCED_FACE('',(#23337),#19472,.F.);
#78768=ADVANCED_FACE('',(#23338),#19473,.F.);
#78769=ADVANCED_FACE('',(#23339),#19474,.F.);
#78770=ADVANCED_FACE('',(#23340),#19475,.F.);
#78771=ADVANCED_FACE('',(#23341),#19476,.F.);
#78772=ADVANCED_FACE('',(#23342),#19477,.F.);
#78773=ADVANCED_FACE('',(#23343),#19478,.F.);
#78774=ADVANCED_FACE('',(#23344),#19479,.F.);
#78775=ADVANCED_FACE('',(#23345),#19480,.F.);
#78776=ADVANCED_FACE('',(#23346),#19481,.F.);
#78777=ADVANCED_FACE('',(#23347),#19482,.F.);
#78778=ADVANCED_FACE('',(#23348),#19483,.F.);
#78779=ADVANCED_FACE('',(#23349),#19484,.F.);
#78780=ADVANCED_FACE('',(#23350),#19485,.F.);
#78781=ADVANCED_FACE('',(#23351),#19486,.F.);
#78782=ADVANCED_FACE('',(#23352),#19487,.F.);
#78783=ADVANCED_FACE('',(#23353),#19488,.F.);
#78784=ADVANCED_FACE('',(#23354),#19489,.F.);
#78785=ADVANCED_FACE('',(#23355),#19490,.F.);
#78786=ADVANCED_FACE('',(#23356),#19491,.F.);
#78787=ADVANCED_FACE('',(#23357),#19492,.F.);
#78788=ADVANCED_FACE('',(#23358),#19493,.F.);
#78789=ADVANCED_FACE('',(#23359),#19494,.F.);
#78790=ADVANCED_FACE('',(#23360),#19495,.F.);
#78791=ADVANCED_FACE('',(#23361),#19496,.F.);
#78792=ADVANCED_FACE('',(#23362),#19497,.F.);
#78793=ADVANCED_FACE('',(#23363),#19498,.F.);
#78794=ADVANCED_FACE('',(#23364),#19499,.F.);
#78795=ADVANCED_FACE('',(#23365),#19500,.F.);
#78796=ADVANCED_FACE('',(#23366),#19501,.F.);
#78797=ADVANCED_FACE('',(#23367),#19502,.F.);
#78798=ADVANCED_FACE('',(#23368),#19503,.F.);
#78799=ADVANCED_FACE('',(#23369),#19504,.F.);
#78800=ADVANCED_FACE('',(#23370),#19505,.F.);
#78801=ADVANCED_FACE('',(#23371),#19506,.F.);
#78802=ADVANCED_FACE('',(#23372),#19507,.F.);
#78803=ADVANCED_FACE('',(#23373),#19508,.F.);
#78804=ADVANCED_FACE('',(#23374),#19509,.F.);
#78805=ADVANCED_FACE('',(#23375),#19510,.F.);
#78806=ADVANCED_FACE('',(#23376),#19511,.F.);
#78807=ADVANCED_FACE('',(#23377),#19512,.F.);
#78808=ADVANCED_FACE('',(#23378),#19513,.F.);
#78809=ADVANCED_FACE('',(#23379),#19514,.F.);
#78810=ADVANCED_FACE('',(#23380),#19515,.F.);
#78811=ADVANCED_FACE('',(#23381),#19516,.F.);
#78812=ADVANCED_FACE('',(#23382),#19517,.F.);
#78813=ADVANCED_FACE('',(#23383),#19518,.F.);
#78814=ADVANCED_FACE('',(#23384),#19519,.F.);
#78815=ADVANCED_FACE('',(#23385),#19520,.F.);
#78816=ADVANCED_FACE('',(#23386),#19521,.F.);
#78817=ADVANCED_FACE('',(#23387),#19522,.F.);
#78818=ADVANCED_FACE('',(#23388),#19523,.F.);
#78819=ADVANCED_FACE('',(#23389),#19524,.F.);
#78820=ADVANCED_FACE('',(#23390),#19525,.F.);
#78821=ADVANCED_FACE('',(#23391),#19526,.F.);
#78822=ADVANCED_FACE('',(#23392),#19527,.F.);
#78823=ADVANCED_FACE('',(#23393),#19528,.F.);
#78824=ADVANCED_FACE('',(#23394),#19529,.F.);
#78825=ADVANCED_FACE('',(#23395),#19530,.F.);
#78826=ADVANCED_FACE('',(#23396),#19531,.F.);
#78827=ADVANCED_FACE('',(#23397),#19532,.F.);
#78828=ADVANCED_FACE('',(#23398),#19533,.F.);
#78829=ADVANCED_FACE('',(#23399),#19534,.F.);
#78830=ADVANCED_FACE('',(#23400),#19535,.F.);
#78831=ADVANCED_FACE('',(#23401),#19536,.F.);
#78832=ADVANCED_FACE('',(#23402),#19537,.F.);
#78833=ADVANCED_FACE('',(#23403),#19538,.F.);
#78834=ADVANCED_FACE('',(#23404),#19539,.F.);
#78835=ADVANCED_FACE('',(#23405),#19540,.F.);
#78836=ADVANCED_FACE('',(#23406),#19541,.F.);
#78837=ADVANCED_FACE('',(#23407),#19542,.F.);
#78838=ADVANCED_FACE('',(#23408),#19543,.F.);
#78839=ADVANCED_FACE('',(#23409),#19544,.F.);
#78840=ADVANCED_FACE('',(#23410),#19545,.F.);
#78841=ADVANCED_FACE('',(#23411),#19546,.F.);
#78842=ADVANCED_FACE('',(#23412),#19547,.F.);
#78843=ADVANCED_FACE('',(#23413),#19548,.F.);
#78844=ADVANCED_FACE('',(#23414),#19549,.F.);
#78845=ADVANCED_FACE('',(#23415),#19550,.F.);
#78846=ADVANCED_FACE('',(#23416),#19551,.F.);
#78847=ADVANCED_FACE('',(#23417),#19552,.F.);
#78848=ADVANCED_FACE('',(#23418),#19553,.F.);
#78849=ADVANCED_FACE('',(#23419),#19554,.F.);
#78850=ADVANCED_FACE('',(#23420),#19555,.F.);
#78851=ADVANCED_FACE('',(#23421),#19556,.F.);
#78852=ADVANCED_FACE('',(#23422),#19557,.F.);
#78853=ADVANCED_FACE('',(#23423),#19558,.F.);
#78854=ADVANCED_FACE('',(#23424),#19559,.F.);
#78855=ADVANCED_FACE('',(#23425),#19560,.F.);
#78856=ADVANCED_FACE('',(#23426),#19561,.F.);
#78857=ADVANCED_FACE('',(#23427),#19562,.F.);
#78858=ADVANCED_FACE('',(#23428),#19563,.F.);
#78859=ADVANCED_FACE('',(#23429),#19564,.F.);
#78860=ADVANCED_FACE('',(#23430),#19565,.F.);
#78861=ADVANCED_FACE('',(#23431),#19566,.F.);
#78862=ADVANCED_FACE('',(#23432),#19567,.F.);
#78863=ADVANCED_FACE('',(#23433),#19568,.F.);
#78864=ADVANCED_FACE('',(#23434),#19569,.F.);
#78865=ADVANCED_FACE('',(#23435),#19570,.F.);
#78866=ADVANCED_FACE('',(#23436),#19571,.F.);
#78867=ADVANCED_FACE('',(#23437),#19572,.F.);
#78868=ADVANCED_FACE('',(#23438),#19573,.F.);
#78869=ADVANCED_FACE('',(#23439),#19574,.F.);
#78870=ADVANCED_FACE('',(#23440),#19575,.F.);
#78871=ADVANCED_FACE('',(#23441),#19576,.F.);
#78872=ADVANCED_FACE('',(#23442),#19577,.F.);
#78873=ADVANCED_FACE('',(#23443),#19578,.F.);
#78874=ADVANCED_FACE('',(#23444),#19579,.F.);
#78875=ADVANCED_FACE('',(#23445),#19580,.F.);
#78876=ADVANCED_FACE('',(#23446),#19581,.F.);
#78877=ADVANCED_FACE('',(#23447),#19582,.F.);
#78878=ADVANCED_FACE('',(#23448),#19583,.F.);
#78879=ADVANCED_FACE('',(#23449),#19584,.F.);
#78880=ADVANCED_FACE('',(#23450),#19585,.F.);
#78881=ADVANCED_FACE('',(#23451),#19586,.F.);
#78882=ADVANCED_FACE('',(#23452),#19587,.F.);
#78883=ADVANCED_FACE('',(#23453),#19588,.F.);
#78884=ADVANCED_FACE('',(#23454),#19589,.F.);
#78885=ADVANCED_FACE('',(#23455),#19590,.F.);
#78886=ADVANCED_FACE('',(#23456),#19591,.F.);
#78887=ADVANCED_FACE('',(#23457),#19592,.F.);
#78888=ADVANCED_FACE('',(#23458),#19593,.F.);
#78889=ADVANCED_FACE('',(#23459),#19594,.F.);
#78890=ADVANCED_FACE('',(#23460),#19595,.F.);
#78891=ADVANCED_FACE('',(#23461),#19596,.F.);
#78892=ADVANCED_FACE('',(#23462),#19597,.F.);
#78893=ADVANCED_FACE('',(#23463),#19598,.F.);
#78894=ADVANCED_FACE('',(#23464),#19599,.F.);
#78895=ADVANCED_FACE('',(#23465),#19600,.F.);
#78896=ADVANCED_FACE('',(#23466),#19601,.F.);
#78897=ADVANCED_FACE('',(#23467),#19602,.F.);
#78898=ADVANCED_FACE('',(#23468),#19603,.F.);
#78899=ADVANCED_FACE('',(#23469),#19604,.F.);
#78900=ADVANCED_FACE('',(#23470),#19605,.F.);
#78901=ADVANCED_FACE('',(#23471),#19606,.F.);
#78902=ADVANCED_FACE('',(#23472),#19607,.F.);
#78903=ADVANCED_FACE('',(#23473),#19608,.F.);
#78904=ADVANCED_FACE('',(#23474),#19609,.F.);
#78905=ADVANCED_FACE('',(#23475),#19610,.F.);
#78906=ADVANCED_FACE('',(#23476),#19611,.F.);
#78907=ADVANCED_FACE('',(#23477),#19612,.F.);
#78908=ADVANCED_FACE('',(#23478),#19613,.F.);
#78909=ADVANCED_FACE('',(#23479),#19614,.F.);
#78910=ADVANCED_FACE('',(#23480),#19615,.F.);
#78911=ADVANCED_FACE('',(#23481),#19616,.F.);
#78912=ADVANCED_FACE('',(#23482),#19617,.F.);
#78913=ADVANCED_FACE('',(#23483),#19618,.F.);
#78914=ADVANCED_FACE('',(#23484),#19619,.F.);
#78915=ADVANCED_FACE('',(#23485),#19620,.F.);
#78916=ADVANCED_FACE('',(#23486),#19621,.F.);
#78917=ADVANCED_FACE('',(#23487),#19622,.F.);
#78918=ADVANCED_FACE('',(#23488),#19623,.F.);
#78919=ADVANCED_FACE('',(#23489),#19624,.F.);
#78920=ADVANCED_FACE('',(#23490),#19625,.F.);
#78921=ADVANCED_FACE('',(#23491),#19626,.F.);
#78922=ADVANCED_FACE('',(#23492),#19627,.F.);
#78923=ADVANCED_FACE('',(#23493),#19628,.F.);
#78924=ADVANCED_FACE('',(#23494),#19629,.F.);
#78925=ADVANCED_FACE('',(#23495),#19630,.F.);
#78926=ADVANCED_FACE('',(#23496),#19631,.F.);
#78927=ADVANCED_FACE('',(#23497),#19632,.F.);
#78928=ADVANCED_FACE('',(#23498),#19633,.F.);
#78929=ADVANCED_FACE('',(#23499),#19634,.F.);
#78930=ADVANCED_FACE('',(#23500),#19635,.F.);
#78931=ADVANCED_FACE('',(#23501),#19636,.F.);
#78932=ADVANCED_FACE('',(#23502),#19637,.F.);
#78933=ADVANCED_FACE('',(#23503),#19638,.F.);
#78934=ADVANCED_FACE('',(#23504),#19639,.F.);
#78935=ADVANCED_FACE('',(#23505),#19640,.F.);
#78936=ADVANCED_FACE('',(#23506),#19641,.F.);
#78937=ADVANCED_FACE('',(#23507),#19642,.F.);
#78938=ADVANCED_FACE('',(#23508),#19643,.F.);
#78939=ADVANCED_FACE('',(#23509),#19644,.F.);
#78940=ADVANCED_FACE('',(#23510),#19645,.F.);
#78941=ADVANCED_FACE('',(#23511),#19646,.F.);
#78942=ADVANCED_FACE('',(#23512),#19647,.F.);
#78943=ADVANCED_FACE('',(#23513),#19648,.F.);
#78944=ADVANCED_FACE('',(#23514),#19649,.F.);
#78945=ADVANCED_FACE('',(#23515),#19650,.F.);
#78946=ADVANCED_FACE('',(#23516),#19651,.F.);
#78947=ADVANCED_FACE('',(#23517),#19652,.F.);
#78948=ADVANCED_FACE('',(#23518),#19653,.F.);
#78949=ADVANCED_FACE('',(#23519),#19654,.F.);
#78950=ADVANCED_FACE('',(#23520),#19655,.F.);
#78951=ADVANCED_FACE('',(#23521),#19656,.F.);
#78952=ADVANCED_FACE('',(#23522),#19657,.F.);
#78953=ADVANCED_FACE('',(#23523),#19658,.F.);
#78954=ADVANCED_FACE('',(#23524),#19659,.F.);
#78955=ADVANCED_FACE('',(#23525),#19660,.F.);
#78956=ADVANCED_FACE('',(#23526),#19661,.F.);
#78957=ADVANCED_FACE('',(#23527),#19662,.F.);
#78958=ADVANCED_FACE('',(#23528),#19663,.F.);
#78959=ADVANCED_FACE('',(#23529),#19664,.F.);
#78960=ADVANCED_FACE('',(#23530),#19665,.F.);
#78961=ADVANCED_FACE('',(#23531),#19666,.F.);
#78962=ADVANCED_FACE('',(#23532),#19667,.F.);
#78963=ADVANCED_FACE('',(#23533),#19668,.F.);
#78964=ADVANCED_FACE('',(#23534),#19669,.F.);
#78965=ADVANCED_FACE('',(#23535),#19670,.F.);
#78966=ADVANCED_FACE('',(#23536),#19671,.F.);
#78967=ADVANCED_FACE('',(#23537),#19672,.F.);
#78968=ADVANCED_FACE('',(#23538),#19673,.F.);
#78969=ADVANCED_FACE('',(#23539),#19674,.F.);
#78970=ADVANCED_FACE('',(#23540),#19675,.F.);
#78971=ADVANCED_FACE('',(#23541),#19676,.F.);
#78972=ADVANCED_FACE('',(#23542),#19677,.F.);
#78973=ADVANCED_FACE('',(#23543),#19678,.F.);
#78974=ADVANCED_FACE('',(#23544),#19679,.F.);
#78975=ADVANCED_FACE('',(#23545),#19680,.F.);
#78976=ADVANCED_FACE('',(#23546),#19681,.F.);
#78977=ADVANCED_FACE('',(#23547),#19682,.F.);
#78978=ADVANCED_FACE('',(#23548),#19683,.F.);
#78979=ADVANCED_FACE('',(#23549),#19684,.F.);
#78980=ADVANCED_FACE('',(#23550),#19685,.F.);
#78981=ADVANCED_FACE('',(#23551),#19686,.F.);
#78982=ADVANCED_FACE('',(#23552),#19687,.F.);
#78983=ADVANCED_FACE('',(#23553),#19688,.F.);
#78984=ADVANCED_FACE('',(#23554),#19689,.F.);
#78985=ADVANCED_FACE('',(#23555),#19690,.F.);
#78986=ADVANCED_FACE('',(#23556),#19691,.F.);
#78987=ADVANCED_FACE('',(#23557),#19692,.F.);
#78988=ADVANCED_FACE('',(#23558),#19693,.F.);
#78989=ADVANCED_FACE('',(#23559),#19694,.F.);
#78990=ADVANCED_FACE('',(#23560),#19695,.F.);
#78991=ADVANCED_FACE('',(#23561),#19696,.F.);
#78992=ADVANCED_FACE('',(#23562),#19697,.F.);
#78993=ADVANCED_FACE('',(#23563),#19698,.F.);
#78994=ADVANCED_FACE('',(#23564),#19699,.F.);
#78995=ADVANCED_FACE('',(#23565),#19700,.F.);
#78996=ADVANCED_FACE('',(#23566),#19701,.F.);
#78997=ADVANCED_FACE('',(#23567),#19702,.F.);
#78998=ADVANCED_FACE('',(#23568),#19703,.F.);
#78999=ADVANCED_FACE('',(#23569),#19704,.F.);
#79000=ADVANCED_FACE('',(#23570),#19705,.F.);
#79001=ADVANCED_FACE('',(#23571),#19706,.F.);
#79002=ADVANCED_FACE('',(#23572),#19707,.F.);
#79003=ADVANCED_FACE('',(#23573),#19708,.F.);
#79004=ADVANCED_FACE('',(#23574),#19709,.F.);
#79005=ADVANCED_FACE('',(#23575),#19710,.F.);
#79006=ADVANCED_FACE('',(#23576),#19711,.F.);
#79007=ADVANCED_FACE('',(#23577),#19712,.F.);
#79008=ADVANCED_FACE('',(#23578),#19713,.F.);
#79009=ADVANCED_FACE('',(#23579),#19714,.F.);
#79010=ADVANCED_FACE('',(#23580),#19715,.F.);
#79011=ADVANCED_FACE('',(#23581),#19716,.F.);
#79012=ADVANCED_FACE('',(#23582),#19717,.F.);
#79013=ADVANCED_FACE('',(#23583),#19718,.F.);
#79014=ADVANCED_FACE('',(#23584),#19719,.F.);
#79015=ADVANCED_FACE('',(#23585),#19720,.F.);
#79016=ADVANCED_FACE('',(#23586),#19721,.F.);
#79017=ADVANCED_FACE('',(#23587),#19722,.F.);
#79018=ADVANCED_FACE('',(#23588),#19723,.F.);
#79019=ADVANCED_FACE('',(#23589),#19724,.F.);
#79020=ADVANCED_FACE('',(#23590),#19725,.F.);
#79021=ADVANCED_FACE('',(#23591),#19726,.F.);
#79022=ADVANCED_FACE('',(#23592),#19727,.F.);
#79023=ADVANCED_FACE('',(#23593),#19728,.F.);
#79024=ADVANCED_FACE('',(#23594),#19729,.F.);
#79025=ADVANCED_FACE('',(#23595),#19730,.F.);
#79026=ADVANCED_FACE('',(#23596),#19731,.F.);
#79027=ADVANCED_FACE('',(#23597),#19732,.F.);
#79028=ADVANCED_FACE('',(#23598),#19733,.F.);
#79029=ADVANCED_FACE('',(#23599),#19734,.F.);
#79030=ADVANCED_FACE('',(#23600),#19735,.F.);
#79031=ADVANCED_FACE('',(#23601),#19736,.F.);
#79032=ADVANCED_FACE('',(#23602),#19737,.F.);
#79033=ADVANCED_FACE('',(#23603),#19738,.F.);
#79034=ADVANCED_FACE('',(#23604),#19739,.F.);
#79035=ADVANCED_FACE('',(#23605),#19740,.F.);
#79036=ADVANCED_FACE('',(#23606),#19741,.F.);
#79037=ADVANCED_FACE('',(#23607),#19742,.F.);
#79038=ADVANCED_FACE('',(#23608),#19743,.F.);
#79039=ADVANCED_FACE('',(#23609),#19744,.F.);
#79040=ADVANCED_FACE('',(#23610),#19745,.F.);
#79041=ADVANCED_FACE('',(#23611),#19746,.F.);
#79042=ADVANCED_FACE('',(#23612),#19747,.F.);
#79043=ADVANCED_FACE('',(#23613),#19748,.F.);
#79044=ADVANCED_FACE('',(#23614),#19749,.F.);
#79045=ADVANCED_FACE('',(#23615),#19750,.F.);
#79046=ADVANCED_FACE('',(#23616),#19751,.F.);
#79047=ADVANCED_FACE('',(#23617),#19752,.F.);
#79048=ADVANCED_FACE('',(#23618),#19753,.F.);
#79049=ADVANCED_FACE('',(#23619),#19754,.F.);
#79050=ADVANCED_FACE('',(#23620),#19755,.F.);
#79051=ADVANCED_FACE('',(#23621),#19756,.F.);
#79052=ADVANCED_FACE('',(#23622),#19757,.F.);
#79053=ADVANCED_FACE('',(#23623),#19758,.F.);
#79054=ADVANCED_FACE('',(#23624),#19759,.F.);
#79055=ADVANCED_FACE('',(#23625),#19760,.F.);
#79056=ADVANCED_FACE('',(#23626),#19761,.F.);
#79057=ADVANCED_FACE('',(#23627),#19762,.F.);
#79058=ADVANCED_FACE('',(#23628),#19763,.F.);
#79059=ADVANCED_FACE('',(#23629),#19764,.F.);
#79060=ADVANCED_FACE('',(#23630),#19765,.F.);
#79061=ADVANCED_FACE('',(#23631),#19766,.F.);
#79062=ADVANCED_FACE('',(#23632),#19767,.F.);
#79063=ADVANCED_FACE('',(#23633),#19768,.F.);
#79064=ADVANCED_FACE('',(#23634),#19769,.F.);
#79065=ADVANCED_FACE('',(#23635),#19770,.F.);
#79066=ADVANCED_FACE('',(#23636),#19771,.F.);
#79067=ADVANCED_FACE('',(#23637),#19772,.F.);
#79068=ADVANCED_FACE('',(#23638),#19773,.F.);
#79069=ADVANCED_FACE('',(#23639),#19774,.F.);
#79070=ADVANCED_FACE('',(#23640),#19775,.F.);
#79071=ADVANCED_FACE('',(#23641),#19776,.F.);
#79072=ADVANCED_FACE('',(#23642),#19777,.F.);
#79073=ADVANCED_FACE('',(#23643),#19778,.F.);
#79074=ADVANCED_FACE('',(#23644),#19779,.F.);
#79075=ADVANCED_FACE('',(#23645),#19780,.F.);
#79076=ADVANCED_FACE('',(#23646),#19781,.F.);
#79077=ADVANCED_FACE('',(#23647),#19782,.F.);
#79078=ADVANCED_FACE('',(#23648),#19783,.F.);
#79079=ADVANCED_FACE('',(#23649),#19784,.F.);
#79080=ADVANCED_FACE('',(#23650),#19785,.F.);
#79081=ADVANCED_FACE('',(#23651),#19786,.F.);
#79082=ADVANCED_FACE('',(#23652),#19787,.F.);
#79083=ADVANCED_FACE('',(#23653),#19788,.F.);
#79084=ADVANCED_FACE('',(#23654),#19789,.F.);
#79085=ADVANCED_FACE('',(#23655),#19790,.F.);
#79086=ADVANCED_FACE('',(#23656),#19791,.F.);
#79087=ADVANCED_FACE('',(#23657),#19792,.F.);
#79088=ADVANCED_FACE('',(#23658),#19793,.F.);
#79089=ADVANCED_FACE('',(#23659),#19794,.F.);
#79090=ADVANCED_FACE('',(#23660),#19795,.F.);
#79091=ADVANCED_FACE('',(#23661),#19796,.F.);
#79092=ADVANCED_FACE('',(#23662),#19797,.F.);
#79093=ADVANCED_FACE('',(#23663),#19798,.F.);
#79094=ADVANCED_FACE('',(#23664),#19799,.F.);
#79095=ADVANCED_FACE('',(#23665),#19800,.F.);
#79096=ADVANCED_FACE('',(#23666),#19801,.F.);
#79097=ADVANCED_FACE('',(#23667),#19802,.F.);
#79098=ADVANCED_FACE('',(#23668),#19803,.F.);
#79099=ADVANCED_FACE('',(#23669),#19804,.F.);
#79100=ADVANCED_FACE('',(#23670),#19805,.F.);
#79101=ADVANCED_FACE('',(#23671),#19806,.F.);
#79102=ADVANCED_FACE('',(#23672),#19807,.F.);
#79103=ADVANCED_FACE('',(#23673),#19808,.F.);
#79104=ADVANCED_FACE('',(#23674),#19809,.F.);
#79105=ADVANCED_FACE('',(#23675),#19810,.F.);
#79106=ADVANCED_FACE('',(#23676),#19811,.F.);
#79107=ADVANCED_FACE('',(#23677),#19812,.F.);
#79108=ADVANCED_FACE('',(#23678),#19813,.F.);
#79109=ADVANCED_FACE('',(#23679),#19814,.F.);
#79110=ADVANCED_FACE('',(#23680),#19815,.F.);
#79111=ADVANCED_FACE('',(#23681),#19816,.F.);
#79112=ADVANCED_FACE('',(#23682),#19817,.F.);
#79113=ADVANCED_FACE('',(#23683),#19818,.F.);
#79114=ADVANCED_FACE('',(#23684),#19819,.F.);
#79115=ADVANCED_FACE('',(#23685),#19820,.F.);
#79116=ADVANCED_FACE('',(#23686),#19821,.F.);
#79117=ADVANCED_FACE('',(#23687),#19822,.F.);
#79118=ADVANCED_FACE('',(#23688),#19823,.F.);
#79119=ADVANCED_FACE('',(#23689),#19824,.F.);
#79120=ADVANCED_FACE('',(#23690),#19825,.F.);
#79121=ADVANCED_FACE('',(#23691),#19826,.F.);
#79122=ADVANCED_FACE('',(#23692),#19827,.F.);
#79123=ADVANCED_FACE('',(#23693),#19828,.F.);
#79124=ADVANCED_FACE('',(#23694),#19829,.F.);
#79125=ADVANCED_FACE('',(#23695),#19830,.F.);
#79126=ADVANCED_FACE('',(#23696),#19831,.F.);
#79127=ADVANCED_FACE('',(#23697),#19832,.F.);
#79128=ADVANCED_FACE('',(#23698),#19833,.F.);
#79129=ADVANCED_FACE('',(#23699),#19834,.F.);
#79130=ADVANCED_FACE('',(#23700,#331),#19835,.F.);
#79131=ADVANCED_FACE('',(#23701,#332,#333,#334,#335,#336,#337,#338,#339,
#340,#341,#342,#343,#344,#345,#346,#347,#348,#349,#350,#351,#352,#353,#354,
#355,#356,#357,#358,#359,#360,#361,#362,#363,#364,#365,#366,#367,#368,#369,
#370,#371,#372,#373,#374,#375,#376,#377,#378,#379,#380,#381,#382,#383,#384,
#385,#386,#387,#388,#389,#390,#391,#392,#393,#394,#395,#396,#397,#398,#399,
#400,#401,#402,#403,#404,#405,#406,#407,#408,#409,#410,#411,#412,#413,#414,
#415,#416,#417,#418,#419,#420,#421,#422,#423,#424,#425,#426,#427,#428,#429,
#430,#431,#432,#433,#434,#435,#436,#437,#438,#439,#440,#441,#442,#443,#444,
#445,#446,#447,#448,#449,#450,#451,#452,#453,#454,#455,#456,#457,#458,#459,
#460,#461,#462,#463,#464,#465,#466,#467,#468,#469,#470,#471,#472,#473,#474,
#475,#476,#477,#478,#479,#480,#481,#482,#483,#484,#485,#486,#487,#488,#489,
#490,#491,#492,#493,#494,#495,#496,#497,#498,#499,#500,#501,#502,#503,#504,
#505,#506,#507,#508,#509,#510,#511,#512,#513,#514,#515,#516,#517,#518,#519,
#520,#521,#522,#523,#524,#525,#526,#527,#528,#529,#530,#531,#532,#533,#534,
#535,#536,#537,#538,#539,#540,#541,#542,#543,#544,#545,#546,#547,#548,#549,
#550,#551,#552,#553,#554,#555,#556,#557,#558,#559,#560,#561,#562,#563,#564,
#565,#566,#567,#568,#569,#570,#571,#572,#573,#574,#575,#576,#577,#578,#579,
#580,#581,#582,#583,#584,#585,#586,#587,#588,#589,#590,#591,#592,#593,#594,
#595,#596,#597,#598,#599,#600,#601,#602,#603,#604,#605,#606,#607,#608,#609,
#610,#611,#612,#613,#614,#615,#616,#617,#618,#619,#620,#621,#622,#623,#624,
#625,#626,#627,#628,#629,#630,#631,#632,#633,#634,#635,#636,#637,#638,#639,
#640,#641,#642,#643,#644,#645,#646,#647,#648,#649,#650,#651,#652,#653,#654,
#655,#656,#657,#658,#659,#660,#661,#662,#663,#664,#665,#666,#667,#668,#669,
#670,#671,#672,#673,#674,#675,#676,#677,#678,#679,#680,#681,#682,#683,#684,
#685,#686,#687,#688,#689,#690,#691,#692,#693,#694,#695,#696,#697,#698,#699,
#700,#701,#702,#703,#704,#705,#706,#707,#708,#709,#710,#711,#712,#713,#714,
#715,#716,#717,#718,#719,#720,#721,#722,#723,#724,#725,#726,#727,#728,#729,
#730,#731,#732,#733,#734,#735,#736,#737,#738,#739,#740,#741,#742,#743,#744,
#745,#746,#747,#748,#749,#750,#751,#752,#753,#754,#755,#756,#757,#758,#759,
#760,#761,#762,#763,#764,#765,#766,#767,#768),#19836,.F.);
#79132=ADVANCED_FACE('',(#23702),#19837,.F.);
#79133=ADVANCED_FACE('',(#23703),#19838,.F.);
#79134=ADVANCED_FACE('',(#23704),#19839,.F.);
#79135=ADVANCED_FACE('',(#23705),#19840,.F.);
#79136=ADVANCED_FACE('',(#23706,#769,#770,#771,#772,#773,#774,#775,#776,
#777,#778,#779,#780,#781,#782,#783,#784,#785,#786,#787,#788,#789,#790,#791,
#792,#793,#794,#795,#796,#797,#798,#799,#800,#801,#802,#803,#804,#805,#806,
#807,#808,#809,#810,#811,#812,#813,#814,#815,#816,#817,#818,#819,#820,#821,
#822,#823,#824,#825,#826,#827,#828,#829,#830,#831,#832,#833,#834,#835,#836,
#837,#838,#839,#840,#841,#842,#843,#844,#845,#846,#847,#848,#849,#850,#851,
#852,#853,#854,#855,#856,#857,#858,#859,#860,#861,#862,#863,#864,#865,#866,
#867,#868,#869,#870,#871,#872,#873,#874,#875,#876,#877,#878,#879,#880,#881,
#882,#883,#884,#885,#886,#887,#888,#889,#890,#891,#892,#893,#894,#895,#896,
#897,#898,#899,#900,#901,#902,#903,#904,#905,#906,#907,#908,#909,#910,#911,
#912,#913,#914,#915,#916,#917,#918,#919,#920,#921,#922,#923,#924,#925,#926,
#927,#928,#929,#930,#931,#932,#933,#934,#935,#936,#937,#938,#939,#940,#941,
#942,#943,#944,#945,#946,#947,#948,#949,#950,#951,#952,#953,#954,#955,#956,
#957,#958,#959,#960,#961,#962,#963,#964,#965,#966,#967,#968,#969,#970,#971,
#972,#973,#974,#975,#976,#977,#978,#979,#980,#981,#982,#983,#984,#985,#986,
#987,#988,#989,#990,#991,#992,#993,#994,#995,#996,#997,#998,#999,#1000,
#1001,#1002,#1003,#1004,#1005,#1006,#1007,#1008,#1009,#1010,#1011,#1012,
#1013,#1014,#1015,#1016,#1017,#1018,#1019,#1020,#1021,#1022,#1023,#1024,
#1025,#1026,#1027,#1028,#1029,#1030,#1031,#1032,#1033,#1034,#1035,#1036,
#1037,#1038,#1039,#1040,#1041,#1042,#1043,#1044,#1045,#1046,#1047,#1048,
#1049,#1050,#1051,#1052,#1053,#1054,#1055,#1056,#1057,#1058,#1059,#1060,
#1061,#1062,#1063,#1064,#1065,#1066,#1067,#1068,#1069,#1070,#1071,#1072,
#1073,#1074,#1075,#1076,#1077,#1078,#1079,#1080,#1081,#1082,#1083,#1084,
#1085,#1086,#1087,#1088,#1089,#1090,#1091,#1092,#1093,#1094,#1095,#1096,
#1097,#1098,#1099,#1100,#1101,#1102,#1103,#1104,#1105,#1106,#1107,#1108,
#1109,#1110,#1111,#1112,#1113,#1114,#1115,#1116,#1117,#1118,#1119,#1120,
#1121,#1122,#1123,#1124,#1125,#1126,#1127,#1128,#1129,#1130,#1131,#1132,
#1133,#1134,#1135,#1136,#1137,#1138,#1139,#1140,#1141,#1142,#1143,#1144,
#1145,#1146,#1147,#1148,#1149,#1150,#1151,#1152,#1153,#1154,#1155,#1156,
#1157,#1158,#1159,#1160,#1161,#1162,#1163,#1164,#1165,#1166,#1167,#1168,
#1169,#1170,#1171,#1172,#1173,#1174,#1175,#1176,#1177,#1178,#1179,#1180,
#1181,#1182,#1183,#1184,#1185,#1186,#1187,#1188,#1189,#1190,#1191,#1192,
#1193,#1194,#1195,#1196,#1197,#1198,#1199,#1200,#1201,#1202,#1203,#1204,
#1205),#19841,.T.);
#79137=ADVANCED_FACE('',(#23707,#1206),#19842,.T.);
#79138=ADVANCED_FACE('',(#23708),#19843,.F.);
#79139=ADVANCED_FACE('',(#23709),#19844,.F.);
#79140=ADVANCED_FACE('',(#23710),#19845,.F.);
#79141=ADVANCED_FACE('',(#23711),#19846,.F.);
#79142=ADVANCED_FACE('',(#23712),#2295,.F.);
#79143=ADVANCED_FACE('',(#23713),#2296,.F.);
#79144=ADVANCED_FACE('',(#23714),#19847,.F.);
#79145=ADVANCED_FACE('',(#23715),#19848,.F.);
#79146=ADVANCED_FACE('',(#23716),#19849,.F.);
#79147=ADVANCED_FACE('',(#23717),#19850,.F.);
#79148=ADVANCED_FACE('',(#23718),#2297,.F.);
#79149=ADVANCED_FACE('',(#23719),#2298,.F.);
#79150=ADVANCED_FACE('',(#23720,#1207),#19851,.T.);
#79151=ADVANCED_FACE('',(#23721,#1208,#1209,#1210,#1211,#1212,#1213,#1214,
#1215,#1216,#1217,#1218,#1219,#1220,#1221,#1222,#1223,#1224,#1225,#1226,
#1227,#1228,#1229,#1230,#1231,#1232,#1233,#1234,#1235,#1236,#1237,#1238,
#1239,#1240,#1241,#1242,#1243,#1244,#1245,#1246,#1247,#1248,#1249,#1250,
#1251,#1252,#1253,#1254,#1255,#1256,#1257,#1258,#1259,#1260,#1261,#1262,
#1263,#1264,#1265,#1266,#1267,#1268,#1269,#1270,#1271,#1272,#1273,#1274,
#1275,#1276,#1277,#1278,#1279,#1280,#1281,#1282,#1283,#1284,#1285,#1286,
#1287,#1288,#1289,#1290,#1291,#1292,#1293,#1294,#1295,#1296,#1297,#1298,
#1299,#1300,#1301,#1302,#1303,#1304,#1305,#1306,#1307,#1308,#1309,#1310,
#1311,#1312,#1313,#1314,#1315,#1316,#1317,#1318,#1319,#1320,#1321,#1322,
#1323,#1324,#1325,#1326,#1327,#1328,#1329,#1330,#1331,#1332,#1333,#1334,
#1335,#1336,#1337,#1338,#1339,#1340,#1341,#1342,#1343,#1344,#1345,#1346,
#1347,#1348,#1349,#1350,#1351,#1352,#1353,#1354,#1355,#1356,#1357,#1358,
#1359,#1360,#1361,#1362,#1363,#1364,#1365,#1366,#1367,#1368,#1369,#1370,
#1371,#1372,#1373,#1374,#1375,#1376,#1377,#1378,#1379,#1380,#1381,#1382,
#1383,#1384,#1385,#1386,#1387,#1388,#1389,#1390,#1391,#1392,#1393,#1394,
#1395,#1396,#1397,#1398,#1399,#1400,#1401,#1402,#1403,#1404,#1405,#1406,
#1407,#1408,#1409,#1410,#1411,#1412,#1413,#1414,#1415,#1416,#1417,#1418,
#1419,#1420,#1421,#1422,#1423,#1424,#1425,#1426,#1427,#1428,#1429,#1430,
#1431,#1432,#1433,#1434,#1435,#1436,#1437,#1438,#1439,#1440,#1441,#1442,
#1443,#1444,#1445,#1446,#1447,#1448,#1449,#1450,#1451,#1452,#1453,#1454,
#1455,#1456,#1457,#1458,#1459,#1460,#1461,#1462,#1463),#75297,.F.);
#79152=ADVANCED_FACE('',(#23722),#19852,.F.);
#79153=ADVANCED_FACE('',(#23723),#19853,.F.);
#79154=ADVANCED_FACE('',(#23724),#19854,.F.);
#79155=ADVANCED_FACE('',(#23725),#19855,.F.);
#79156=ADVANCED_FACE('',(#23726,#1464,#1465,#1466,#1467,#1468,#1469,#1470,
#1471,#1472,#1473,#1474,#1475,#1476,#1477,#1478,#1479,#1480,#1481,#1482,
#1483,#1484,#1485,#1486,#1487,#1488,#1489,#1490,#1491,#1492,#1493,#1494,
#1495,#1496,#1497,#1498,#1499,#1500,#1501,#1502,#1503,#1504,#1505,#1506,
#1507,#1508,#1509,#1510,#1511,#1512,#1513,#1514,#1515,#1516,#1517,#1518,
#1519,#1520,#1521,#1522,#1523,#1524,#1525,#1526,#1527,#1528,#1529,#1530,
#1531,#1532,#1533,#1534,#1535,#1536,#1537,#1538,#1539,#1540,#1541,#1542,
#1543,#1544,#1545,#1546,#1547,#1548,#1549,#1550,#1551,#1552,#1553,#1554,
#1555,#1556,#1557,#1558,#1559,#1560,#1561,#1562,#1563,#1564,#1565,#1566,
#1567,#1568,#1569,#1570,#1571,#1572,#1573,#1574,#1575,#1576,#1577,#1578,
#1579,#1580,#1581,#1582,#1583,#1584,#1585,#1586,#1587,#1588,#1589,#1590,
#1591,#1592,#1593,#1594,#1595,#1596,#1597,#1598,#1599,#1600,#1601,#1602,
#1603,#1604,#1605,#1606,#1607,#1608,#1609,#1610,#1611,#1612,#1613,#1614,
#1615,#1616,#1617,#1618,#1619,#1620,#1621,#1622,#1623,#1624,#1625,#1626,
#1627,#1628,#1629,#1630,#1631,#1632,#1633,#1634,#1635,#1636,#1637,#1638,
#1639,#1640,#1641,#1642,#1643,#1644,#1645,#1646,#1647,#1648,#1649,#1650,
#1651,#1652,#1653,#1654,#1655,#1656,#1657,#1658,#1659,#1660,#1661,#1662,
#1663,#1664,#1665,#1666,#1667,#1668,#1669,#1670,#1671,#1672,#1673,#1674,
#1675,#1676,#1677,#1678,#1679,#1680,#1681,#1682,#1683,#1684,#1685,#1686,
#1687,#1688,#1689,#1690,#1691,#1692,#1693,#1694,#1695,#1696,#1697,#1698,
#1699,#1700,#1701,#1702,#1703,#1704,#1705,#1706,#1707,#1708,#1709,#1710,
#1711,#1712,#1713,#1714,#1715,#1716,#1717,#1718,#1719),#75298,.T.);
#79157=ADVANCED_FACE('',(#23727,#1720),#19856,.F.);
#79333=CLOSED_SHELL('',(#76284,#76285,#76286,#76287,#76288,#76289,#76290,
#76291,#76292,#76293,#76294,#76295,#76296,#76297,#76298,#76299,#76300,#76301,
#76302,#76303,#76304,#76305,#76306,#76307,#76308,#76309,#76310,#76311,#76312,
#76313,#76314,#76315,#76316,#76317,#76318,#76319,#76320,#76321,#76322,#76323,
#76324,#76325,#76326,#76327,#76328,#76329,#76330,#76331,#76332,#76333,#76334,
#76335,#76336,#76337,#76338,#76339,#76340,#76341,#76342,#76343,#76344,#76345,
#76346,#76347,#76348,#76349,#76350,#76351,#76352,#76353,#76354,#76355,#76356,
#76357,#76358,#76359,#76360,#76361,#76362,#76363,#76364,#76365,#76366,#76367,
#76368,#76369,#76370,#76371,#76372,#76373,#76374,#76375,#76376,#76377,#76378,
#76379,#76380,#76381,#76382,#76383,#76384,#76385,#76386,#76387,#76388,#76389,
#76390,#76391,#76392,#76393,#76394,#76395,#76396,#76397,#76398,#76399,#76400,
#76401,#76402,#76403,#76404,#76405,#76406,#76407,#76408,#76409,#76410,#76411,
#76412,#76413,#76414,#76415,#76416,#76417,#76418,#76419,#76420,#76421,#76422,
#76423,#76424,#76425,#76426,#76427,#76428,#76429,#76430,#76431,#76432,#76433,
#76434,#76435,#76436,#76437,#76438,#76439,#76440,#76441,#76442,#76443,#76444,
#76445,#76446,#76447,#76448,#76449,#76450,#76451,#76452,#76453,#76454,#76455,
#76456,#76457,#76458,#76459,#76460,#76461,#76462,#76463,#76464,#76465,#76466,
#76467,#76468,#76469,#76470,#76471,#76472,#76473,#76474,#76475,#76476,#76477,
#76478,#76479,#76480,#76481,#76482,#76483,#76484,#76485,#76486,#76487,#76488,
#76489,#76490,#76491,#76492,#76493,#76494,#76495,#76496,#76497,#76498,#76499,
#76500,#76501,#76502,#76503,#76504,#76505,#76506,#76507,#76508,#76509,#76510,
#76511,#76512,#76513,#76514,#76515,#76516,#76517,#76518,#76519,#76520,#76521,
#76522,#76523,#76524,#76525,#76526,#76527,#76528,#76529,#76530,#76531,#76532,
#76533,#76534,#76535,#76536,#76537,#76538,#76539,#76540,#76541,#76542,#76543,
#76544,#76545,#76546,#76547,#76548,#76549,#76550,#76551,#76552,#76553,#76554,
#76555,#76556,#76557,#76558,#76559,#76560,#76561,#76562,#76563,#76564,#76565,
#76566,#76567,#76568,#76569,#76570,#76571,#76572,#76573,#76574,#76575,#76576,
#76577,#76578,#76579,#76580,#76581,#76582,#76583,#76584,#76585,#76586,#76587,
#76588,#76589,#76590,#76591,#76592,#76593,#76594,#76595,#76596,#76597,#76598,
#76599,#76600,#76601,#76602,#76603,#76604,#76605,#76606,#76607,#76608,#76609,
#76610,#76611,#76612,#76613,#76614,#76615,#76616,#76617,#76618,#76619,#76620,
#76621,#76622,#76623,#76624,#76625,#76626,#76627,#76628,#76629,#76630,#76631,
#76632,#76633,#76634,#76635,#76636,#76637,#76638,#76639,#76640,#76641,#76642,
#76643,#76644,#76645,#76646,#76647,#76648,#76649,#76650,#76651,#76652,#76653,
#76654,#76655,#76656,#76657,#76658,#76659,#76660,#76661,#76662,#76663,#76664,
#76665,#76666,#76667,#76668,#76669,#76670,#76671,#76672,#76673,#76674,#76675,
#76676,#76677,#76678,#76679,#76680,#76681,#76682,#76683,#76684,#76685,#76686,
#76687,#76688,#76689,#76690,#76691,#76692,#76693,#76694,#76695,#76696,#76697,
#76698,#76699,#76700,#76701,#76702,#76703,#76704,#76705,#76706,#76707,#76708,
#76709,#76710,#76711,#76712,#76713,#76714,#76715,#76716,#76717,#76718,#76719,
#76720,#76721,#76722,#76723,#76724,#76725,#76726,#76727,#76728,#76729,#76730,
#76731,#76732,#76733,#76734,#76735,#76736,#76737,#76738,#76739,#76740,#76741,
#76742,#76743,#76744,#76745,#76746,#76747,#76748,#76749,#76750,#76751,#76752,
#76753,#76754,#76755,#76756,#76757,#76758,#76759,#76760,#76761,#76762,#76763,
#76764,#76765,#76766,#76767,#76768,#76769,#76770,#76771,#76772,#76773,#76774,
#76775,#76776,#76777,#76778,#76779,#76780,#76781,#76782,#76783,#76784,#76785,
#76786,#76787,#76788,#76789,#76790,#76791,#76792,#76793,#76794,#76795,#76796,
#76797,#76798,#76799,#76800,#76801,#76802,#76803,#76804,#76805,#76806,#76807,
#76808,#76809,#76810,#76811,#76812,#76813,#76814,#76815,#76816,#76817,#76818,
#76819,#76820,#76821,#76822,#76823,#76824,#76825,#76826,#76827,#76828,#76829,
#76830,#76831,#76832,#76833,#76834,#76835,#76836,#76837,#76838,#76839,#76840,
#76841,#76842,#76843,#76844,#76845,#76846,#76847,#76848,#76849,#76850,#76851,
#76852,#76853,#76854,#76855,#76856,#76857,#76858,#76859,#76860,#76861,#76862,
#76863,#76864,#76865,#76866,#76867,#76868,#76869,#76870,#76871,#76872,#76873,
#76874,#76875,#76876,#76877,#76878,#76879,#76880,#76881,#76882,#76883,#76884,
#76885,#76886,#76887,#76888,#76889,#76890,#76891,#76892,#76893,#76894,#76895,
#76896,#76897,#76898,#76899,#76900,#76901,#76902,#76903,#76904,#76905,#76906,
#76907,#76908,#76909,#76910,#76911,#76912,#76913,#76914,#76915,#76916,#76917,
#76918,#76919,#76920,#76921,#76922,#76923,#76924,#76925,#76926,#76927,#76928,
#76929,#76930,#76931,#76932,#76933,#76934,#76935,#76936,#76937,#76938,#76939,
#76940,#76941,#76942,#76943,#76944,#76945,#76946,#76947,#76948,#76949,#76950,
#76951,#76952,#76953,#76954,#76955,#76956,#76957,#76958,#76959,#76960,#76961,
#76962,#76963,#76964,#76965,#76966,#76967,#76968,#76969,#76970,#76971,#76972,
#76973,#76974,#76975,#76976,#76977,#76978,#76979,#76980,#76981,#76982,#76983,
#76984,#76985,#76986,#76987,#76988,#76989,#76990,#76991,#76992,#76993,#76994,
#76995,#76996,#76997,#76998,#76999,#77000,#77001,#77002,#77003,#77004,#77005,
#77006,#77007,#77008,#77009,#77010,#77011,#77012,#77013,#77014,#77015,#77016,
#77017,#77018,#77019,#77020,#77021,#77022,#77023,#77024,#77025,#77026,#77027,
#77028,#77029,#77030,#77031,#77032,#77033,#77034,#77035,#77036,#77037,#77038,
#77039,#77040,#77041,#77042,#77043,#77044,#77045,#77046,#77047,#77048,#77049,
#77050,#77051,#77052,#77053,#77054,#77055,#77056,#77057,#77058,#77059,#77060,
#77061,#77062,#77063,#77064,#77065,#77066,#77067,#77068,#77069,#77070,#77071,
#77072,#77073,#77074,#77075,#77076,#77077,#77078,#77079,#77080,#77081,#77082,
#77083,#77084,#77085,#77086,#77087,#77088,#77089,#77090,#77091,#77092,#77093,
#77094,#77095,#77096,#77097,#77098,#77099,#77100,#77101,#77102,#77103,#77104,
#77105,#77106,#77107,#77108,#77109,#77110,#77111,#77112,#77113,#77114,#77115,
#77116,#77117,#77118,#77119,#77120,#77121,#77122,#77123,#77124,#77125,#77126,
#77127,#77128,#77129,#77130,#77131,#77132,#77133,#77134,#77135,#77136,#77137,
#77138,#77139,#77140,#77141,#77142,#77143,#77144,#77145,#77146,#77147,#77148,
#77149,#77150,#77151,#77152,#77153,#77154,#77155,#77156,#77157,#77158,#77159,
#77160,#77161,#77162,#77163,#77164,#77165,#77166,#77167,#77168,#77169,#77170,
#77171,#77172,#77173,#77174,#77175,#77176,#77177,#77178,#77179,#77180,#77181,
#77182,#77183,#77184,#77185,#77186,#77187,#77188,#77189,#77190,#77191,#77192,
#77193,#77194,#77195,#77196,#77197,#77198,#77199,#77200,#77201,#77202,#77203,
#77204,#77205,#77206,#77207,#77208,#77209,#77210,#77211,#77212,#77213,#77214,
#77215,#77216,#77217,#77218,#77219,#77220,#77221,#77222,#77223,#77224,#77225,
#77226,#77227,#77228,#77229,#77230,#77231,#77232,#77233,#77234,#77235,#77236,
#77237,#77238,#77239,#77240,#77241,#77242,#77243,#77244,#77245,#77246,#77247,
#77248,#77249,#77250,#77251,#77252,#77253,#77254,#77255,#77256,#77257,#77258,
#77259,#77260,#77261,#77262,#77263,#77264,#77265,#77266,#77267,#77268,#77269,
#77270,#77271,#77272,#77273,#77274,#77275,#77276,#77277,#77278,#77279,#77280,
#77281,#77282,#77283,#77284,#77285,#77286,#77287,#77288,#77289,#77290,#77291,
#77292,#77293,#77294,#77295,#77296,#77297,#77298,#77299,#77300,#77301,#77302,
#77303,#77304,#77305,#77306,#77307,#77308,#77309,#77310,#77311,#77312,#77313,
#77314,#77315,#77316,#77317,#77318,#77319,#77320,#77321,#77322,#77323,#77324,
#77325,#77326,#77327,#77328,#77329,#77330,#77331,#77332,#77333,#77334,#77335,
#77336,#77337,#77338,#77339,#77340,#77341,#77342,#77343,#77344,#77345,#77346,
#77347,#77348,#77349,#77350,#77351,#77352,#77353,#77354,#77355,#77356,#77357,
#77358,#77359,#77360,#77361,#77362,#77363,#77364,#77365,#77366,#77367,#77368,
#77369,#77370,#77371,#77372,#77373,#77374,#77375,#77376,#77377,#77378,#77379,
#77380,#77381,#77382,#77383,#77384,#77385,#77386,#77387,#77388,#77389,#77390,
#77391,#77392,#77393,#77394,#77395,#77396,#77397,#77398,#77399,#77400,#77401,
#77402,#77403,#77404,#77405,#77406,#77407,#77408,#77409,#77410,#77411,#77412,
#77413,#77414,#77415,#77416,#77417,#77418,#77419,#77420,#77421,#77422,#77423,
#77424,#77425,#77426,#77427,#77428,#77429,#77430,#77431,#77432,#77433,#77434,
#77435,#77436,#77437,#77438,#77439,#77440,#77441,#77442,#77443,#77444,#77445,
#77446,#77447,#77448,#77449,#77450,#77451,#77452,#77453,#77454,#77455,#77456,
#77457,#77458,#77459,#77460,#77461,#77462,#77463,#77464,#77465,#77466,#77467,
#77468,#77469,#77470,#77471,#77472,#77473,#77474,#77475,#77476,#77477,#77478,
#77479,#77480,#77481,#77482,#77483,#77484,#77485,#77486,#77487,#77488,#77489,
#77490,#77491,#77492,#77493,#77494,#77495,#77496,#77497,#77498,#77499,#77500,
#77501,#77502,#77503,#77504,#77505,#77506,#77507,#77508,#77509,#77510,#77511,
#77512,#77513,#77514,#77515,#77516,#77517,#77518,#77519,#77520,#77521,#77522,
#77523,#77524,#77525,#77526,#77527,#77528,#77529,#77530,#77531,#77532,#77533,
#77534,#77535,#77536,#77537,#77538,#77539,#77540,#77541,#77542,#77543,#77544,
#77545,#77546,#77547,#77548,#77549,#77550,#77551,#77552,#77553,#77554,#77555,
#77556,#77557,#77558,#77559,#77560,#77561,#77562,#77563,#77564,#77565,#77566,
#77567,#77568,#77569,#77570,#77571,#77572,#77573,#77574,#77575,#77576,#77577,
#77578,#77579,#77580,#77581,#77582,#77583,#77584,#77585,#77586,#77587,#77588,
#77589,#77590,#77591,#77592,#77593,#77594,#77595,#77596,#77597,#77598,#77599,
#77600,#77601,#77602,#77603,#77604,#77605,#77606,#77607,#77608,#77609,#77610,
#77611,#77612,#77613,#77614,#77615,#77616,#77617,#77618,#77619,#77620,#77621,
#77622,#77623,#77624,#77625,#77626,#77627,#77628,#77629,#77630,#77631,#77632,
#77633,#77634,#77635,#77636,#77637,#77638,#77639,#77640,#77641,#77642,#77643,
#77644,#77645,#77646,#77647,#77648,#77649,#77650,#77651,#77652,#77653,#77654,
#77655,#77656,#77657,#77658,#77659,#77660,#77661,#77662,#77663,#77664,#77665,
#77666,#77667,#77668,#77669,#77670,#77671,#77672,#77673,#77674,#77675,#77676,
#77677,#77678,#77679,#77680,#77681,#77682,#77683,#77684,#77685,#77686,#77687,
#77688,#77689,#77690,#77691,#77692,#77693,#77694,#77695,#77696,#77697,#77698,
#77699,#77700,#77701,#77702,#77703,#77704,#77705,#77706,#77707,#77708,#77709,
#77710,#77711,#77712,#77713,#77714,#77715,#77716,#77717,#77718,#77719,#77720,
#77721,#77722,#77723,#77724,#77725,#77726,#77727,#77728,#77729,#77730,#77731,
#77732,#77733,#77734,#77735,#77736,#77737,#77738,#77739,#77740,#77741,#77742,
#77743,#77744,#77745,#77746,#77747,#77748,#77749,#77750,#77751,#77752,#77753,
#77754,#77755,#77756,#77757,#77758,#77759,#77760,#77761,#77762,#77763,#77764,
#77765,#77766,#77767,#77768,#77769,#77770,#77771,#77772,#77773,#77774,#77775,
#77776,#77777,#77778,#77779,#77780,#77781,#77782,#77783,#77784,#77785,#77786,
#77787,#77788,#77789,#77790,#77791,#77792,#77793,#77794,#77795,#77796,#77797,
#77798,#77799,#77800,#77801,#77802,#77803,#77804,#77805,#77806,#77807,#77808,
#77809,#77810,#77811,#77812,#77813,#77814,#77815,#77816,#77817,#77818,#77819,
#77820,#77821,#77822,#77823,#77824,#77825,#77826,#77827,#77828,#77829,#77830,
#77831,#77832,#77833,#77834,#77835,#77836,#77837,#77838,#77839,#77840,#77841,
#77842,#77843,#77844,#77845,#77846,#77847,#77848,#77849,#77850,#77851,#77852,
#77853,#77854,#77855,#77856,#77857,#77858,#77859,#77860,#77861,#77862,#77863,
#77864,#77865,#77866,#77867,#77868,#77869,#77870,#77871,#77872,#77873,#77874,
#77875,#77876,#77877,#77878,#77879,#77880,#77881,#77882,#77883,#77884,#77885,
#77886,#77887,#77888,#77889,#77890,#77891,#77892,#77893,#77894,#77895,#77896,
#77897,#77898,#77899,#77900,#77901,#77902,#77903,#77904,#77905,#77906,#77907,
#77908,#77909,#77910,#77911,#77912,#77913,#77914,#77915,#77916,#77917,#77918,
#77919,#77920,#77921,#77922,#77923,#77924,#77925,#77926,#77927,#77928,#77929,
#77930,#77931,#77932,#77933,#77934,#77935,#77936,#77937,#77938,#77939,#77940,
#77941,#77942,#77943,#77944,#77945,#77946,#77947,#77948,#77949,#77950,#77951,
#77952,#77953,#77954,#77955,#77956,#77957,#77958,#77959,#77960,#77961,#77962,
#77963,#77964,#77965,#77966,#77967,#77968,#77969,#77970,#77971,#77972,#77973,
#77974,#77975,#77976,#77977,#77978,#77979,#77980,#77981,#77982,#77983,#77984,
#77985,#77986,#77987,#77988,#77989,#77990,#77991,#77992,#77993,#77994,#77995,
#77996,#77997,#77998,#77999,#78000,#78001,#78002,#78003,#78004,#78005,#78006,
#78007,#78008,#78009,#78010,#78011,#78012,#78013,#78014,#78015,#78016,#78017,
#78018,#78019,#78020,#78021,#78022,#78023,#78024,#78025,#78026,#78027,#78028,
#78029,#78030,#78031,#78032,#78033,#78034,#78035,#78036,#78037,#78038,#78039,
#78040,#78041,#78042,#78043,#78044,#78045,#78046,#78047,#78048,#78049,#78050,
#78051,#78052,#78053,#78054,#78055,#78056,#78057,#78058,#78059,#78060,#78061,
#78062,#78063,#78064,#78065,#78066,#78067,#78068,#78069,#78070,#78071,#78072,
#78073,#78074,#78075,#78076,#78077,#78078,#78079,#78080,#78081,#78082,#78083,
#78084,#78085,#78086,#78087,#78088,#78089,#78090,#78091,#78092,#78093,#78094,
#78095,#78096,#78097,#78098,#78099,#78100,#78101,#78102,#78103,#78104,#78105,
#78106,#78107,#78108,#78109,#78110,#78111,#78112,#78113,#78114,#78115,#78116,
#78117,#78118,#78119,#78120,#78121,#78122,#78123,#78124,#78125,#78126,#78127,
#78128,#78129,#78130,#78131,#78132,#78133,#78134,#78135,#78136,#78137,#78138,
#78139,#78140,#78141,#78142,#78143,#78144,#78145,#78146,#78147,#78148,#78149,
#78150,#78151,#78152,#78153,#78154,#78155,#78156,#78157,#78158,#78159,#78160,
#78161,#78162,#78163,#78164,#78165,#78166,#78167,#78168,#78169,#78170,#78171,
#78172,#78173,#78174,#78175,#78176,#78177,#78178,#78179,#78180,#78181,#78182,
#78183,#78184,#78185,#78186,#78187,#78188,#78189,#78190,#78191,#78192,#78193,
#78194,#78195,#78196,#78197,#78198,#78199,#78200,#78201,#78202,#78203,#78204,
#78205,#78206,#78207,#78208,#78209,#78210,#78211,#78212,#78213,#78214,#78215,
#78216,#78217,#78218,#78219,#78220,#78221,#78222,#78223,#78224,#78225,#78226,
#78227,#78228,#78229,#78230,#78231,#78232,#78233,#78234,#78235,#78236,#78237,
#78238,#78239,#78240,#78241,#78242,#78243,#78244,#78245,#78246,#78247,#78248,
#78249,#78250,#78251,#78252,#78253,#78254,#78255,#78256,#78257,#78258,#78259,
#78260,#78261,#78262,#78263,#78264,#78265,#78266,#78267,#78268,#78269,#78270,
#78271,#78272,#78273,#78274,#78275,#78276,#78277,#78278,#78279,#78280,#78281,
#78282,#78283,#78284,#78285,#78286,#78287,#78288,#78289,#78290,#78291,#78292,
#78293,#78294,#78295,#78296,#78297,#78298,#78299,#78300,#78301,#78302,#78303,
#78304,#78305,#78306,#78307,#78308,#78309,#78310,#78311,#78312,#78313,#78314,
#78315,#78316,#78317,#78318,#78319,#78320,#78321,#78322,#78323,#78324,#78325,
#78326,#78327,#78328,#78329,#78330,#78331,#78332,#78333,#78334,#78335,#78336,
#78337,#78338,#78339,#78340,#78341,#78342,#78343,#78344,#78345,#78346,#78347,
#78348,#78349,#78350,#78351,#78352,#78353,#78354,#78355,#78356,#78357,#78358,
#78359,#78360,#78361,#78362,#78363,#78364,#78365,#78366,#78367,#78368,#78369,
#78370,#78371,#78372,#78373,#78374,#78375,#78376,#78377,#78378,#78379,#78380,
#78381,#78382,#78383,#78384,#78385,#78386,#78387,#78388,#78389,#78390,#78391,
#78392,#78393,#78394,#78395,#78396,#78397,#78398,#78399,#78400,#78401,#78402,
#78403,#78404,#78405,#78406,#78407,#78408,#78409,#78410,#78411,#78412,#78413,
#78414,#78415,#78416,#78417,#78418,#78419,#78420,#78421,#78422,#78423,#78424,
#78425,#78426,#78427,#78428,#78429,#78430,#78431,#78432,#78433,#78434,#78435,
#78436,#78437,#78438,#78439,#78440,#78441,#78442,#78443,#78444,#78445,#78446,
#78447,#78448,#78449,#78450,#78451,#78452,#78453,#78454,#78455,#78456,#78457,
#78458,#78459,#78460,#78461,#78462,#78463,#78464,#78465,#78466,#78467,#78468,
#78469,#78470,#78471,#78472,#78473,#78474,#78475,#78476,#78477,#78478,#78479,
#78480,#78481,#78482,#78483,#78484,#78485,#78486,#78487,#78488,#78489,#78490,
#78491,#78492,#78493,#78494,#78495,#78496,#78497,#78498,#78499,#78500,#78501,
#78502,#78503,#78504,#78505,#78506,#78507,#78508,#78509,#78510,#78511,#78512,
#78513,#78514,#78515,#78516,#78517,#78518,#78519,#78520,#78521,#78522,#78523,
#78524,#78525,#78526,#78527,#78528,#78529,#78530,#78531,#78532,#78533,#78534,
#78535,#78536,#78537,#78538,#78539,#78540,#78541,#78542,#78543,#78544,#78545,
#78546,#78547,#78548,#78549,#78550,#78551,#78552,#78553,#78554,#78555,#78556,
#78557,#78558,#78559,#78560,#78561,#78562,#78563,#78564,#78565,#78566,#78567,
#78568,#78569,#78570,#78571,#78572,#78573,#78574,#78575,#78576,#78577,#78578,
#78579,#78580,#78581,#78582,#78583,#78584,#78585,#78586,#78587,#78588,#78589,
#78590,#78591,#78592,#78593,#78594,#78595,#78596,#78597,#78598,#78599,#78600,
#78601,#78602,#78603,#78604,#78605,#78606,#78607,#78608,#78609,#78610,#78611,
#78612,#78613,#78614,#78615,#78616,#78617,#78618,#78619,#78620,#78621,#78622,
#78623,#78624,#78625,#78626,#78627,#78628,#78629,#78630,#78631,#78632,#78633,
#78634,#78635,#78636,#78637,#78638,#78639,#78640,#78641,#78642,#78643,#78644,
#78645,#78646,#78647,#78648,#78649,#78650,#78651,#78652,#78653,#78654,#78655,
#78656,#78657,#78658,#78659,#78660,#78661,#78662,#78663,#78664,#78665,#78666,
#78667,#78668,#78669,#78670,#78671,#78672,#78673,#78674,#78675,#78676,#78677,
#78678,#78679,#78680,#78681,#78682,#78683,#78684,#78685,#78686,#78687,#78688,
#78689,#78690,#78691,#78692,#78693,#78694,#78695,#78696,#78697,#78698,#78699,
#78700,#78701,#78702,#78703,#78704,#78705,#78706,#78707,#78708,#78709,#78710,
#78711,#78712,#78713,#78714,#78715,#78716,#78717,#78718,#78719,#78720,#78721,
#78722,#78723,#78724,#78725,#78726,#78727,#78728,#78729,#78730,#78731,#78732,
#78733,#78734,#78735,#78736,#78737,#78738,#78739,#78740,#78741,#78742,#78743,
#78744,#78745,#78746,#78747,#78748,#78749,#78750,#78751,#78752,#78753,#78754,
#78755,#78756,#78757,#78758,#78759,#78760,#78761,#78762,#78763,#78764,#78765,
#78766,#78767,#78768,#78769,#78770,#78771,#78772,#78773,#78774,#78775,#78776,
#78777,#78778,#78779,#78780,#78781,#78782,#78783,#78784,#78785,#78786,#78787,
#78788,#78789,#78790,#78791,#78792,#78793,#78794,#78795,#78796,#78797,#78798,
#78799,#78800,#78801,#78802,#78803,#78804,#78805,#78806,#78807,#78808,#78809,
#78810,#78811,#78812,#78813,#78814,#78815,#78816,#78817,#78818,#78819,#78820,
#78821,#78822,#78823,#78824,#78825,#78826,#78827,#78828,#78829,#78830,#78831,
#78832,#78833,#78834,#78835,#78836,#78837,#78838,#78839,#78840,#78841,#78842,
#78843,#78844,#78845,#78846,#78847,#78848,#78849,#78850,#78851,#78852,#78853,
#78854,#78855,#78856,#78857,#78858,#78859,#78860,#78861,#78862,#78863,#78864,
#78865,#78866,#78867,#78868,#78869,#78870,#78871,#78872,#78873,#78874,#78875,
#78876,#78877,#78878,#78879,#78880,#78881,#78882,#78883,#78884,#78885,#78886,
#78887,#78888,#78889,#78890,#78891,#78892,#78893,#78894,#78895,#78896,#78897,
#78898,#78899,#78900,#78901,#78902,#78903,#78904,#78905,#78906,#78907,#78908,
#78909,#78910,#78911,#78912,#78913,#78914,#78915,#78916,#78917,#78918,#78919,
#78920,#78921,#78922,#78923,#78924,#78925,#78926,#78927,#78928,#78929,#78930,
#78931,#78932,#78933,#78934,#78935,#78936,#78937,#78938,#78939,#78940,#78941,
#78942,#78943,#78944,#78945,#78946,#78947,#78948,#78949,#78950,#78951,#78952,
#78953,#78954,#78955,#78956,#78957,#78958,#78959,#78960,#78961,#78962,#78963,
#78964,#78965,#78966,#78967,#78968,#78969,#78970,#78971,#78972,#78973,#78974,
#78975,#78976,#78977,#78978,#78979,#78980,#78981,#78982,#78983,#78984,#78985,
#78986,#78987,#78988,#78989,#78990,#78991,#78992,#78993,#78994,#78995,#78996,
#78997,#78998,#78999,#79000,#79001,#79002,#79003,#79004,#79005,#79006,#79007,
#79008,#79009,#79010,#79011,#79012,#79013,#79014,#79015,#79016,#79017,#79018,
#79019,#79020,#79021,#79022,#79023,#79024,#79025,#79026,#79027,#79028,#79029,
#79030,#79031,#79032,#79033,#79034,#79035,#79036,#79037,#79038,#79039,#79040,
#79041,#79042,#79043,#79044,#79045,#79046,#79047,#79048,#79049,#79050,#79051,
#79052,#79053,#79054,#79055,#79056,#79057,#79058,#79059,#79060,#79061,#79062,
#79063,#79064,#79065,#79066,#79067,#79068,#79069,#79070,#79071,#79072,#79073,
#79074,#79075,#79076,#79077,#79078,#79079,#79080,#79081,#79082,#79083,#79084,
#79085,#79086,#79087,#79088,#79089,#79090,#79091,#79092,#79093,#79094,#79095,
#79096,#79097,#79098,#79099,#79100,#79101,#79102,#79103,#79104,#79105,#79106,
#79107,#79108,#79109,#79110,#79111,#79112,#79113,#79114,#79115,#79116,#79117,
#79118,#79119,#79120,#79121,#79122,#79123,#79124,#79125,#79126,#79127,#79128,
#79129,#79130,#79131,#79132,#79133,#79134,#79135,#79136,#79137,#79138,#79139,
#79140,#79141,#79142,#79143,#79144,#79145,#79146,#79147,#79148,#79149,#79150,
#79151,#79152,#79153,#79154,#79155,#79156,#79157));
#80981=AXIS2_PLACEMENT_3D('',#183807,#89687,#89688);
#80982=AXIS2_PLACEMENT_3D('',#183808,#89689,#89690);
#80983=AXIS2_PLACEMENT_3D('',#183821,#89692,#89693);
#80984=AXIS2_PLACEMENT_3D('',#183822,#89694,#89695);
#80985=AXIS2_PLACEMENT_3D('',#183909,#89697,#89698);
#80986=AXIS2_PLACEMENT_3D('',#183964,#89699,#89700);
#80987=AXIS2_PLACEMENT_3D('',#184162,#89702,#89703);
#80988=AXIS2_PLACEMENT_3D('',#184167,#89705,#89706);
#80989=AXIS2_PLACEMENT_3D('',#184348,#89707,#89708);
#80990=AXIS2_PLACEMENT_3D('',#184351,#89709,#89710);
#80991=AXIS2_PLACEMENT_3D('',#184354,#89712,#89713);
#80992=AXIS2_PLACEMENT_3D('',#184355,#89714,#89715);
#80993=AXIS2_PLACEMENT_3D('',#184356,#89716,#89717);
#80994=AXIS2_PLACEMENT_3D('',#184358,#89718,#89719);
#80995=AXIS2_PLACEMENT_3D('',#184359,#89720,#89721);
#80996=AXIS2_PLACEMENT_3D('',#184360,#89722,#89723);
#80997=AXIS2_PLACEMENT_3D('',#184362,#89724,#89725);
#80998=AXIS2_PLACEMENT_3D('',#184363,#89726,#89727);
#80999=AXIS2_PLACEMENT_3D('',#184364,#89728,#89729);
#81000=AXIS2_PLACEMENT_3D('',#184407,#89732,#89733);
#81001=AXIS2_PLACEMENT_3D('',#184450,#89736,#89737);
#81002=AXIS2_PLACEMENT_3D('',#184454,#89739,#89740);
#81003=AXIS2_PLACEMENT_3D('',#184476,#89741,#89742);
#81004=AXIS2_PLACEMENT_3D('',#184479,#89744,#89745);
#81005=AXIS2_PLACEMENT_3D('',#184480,#89746,#89747);
#81006=AXIS2_PLACEMENT_3D('',#184481,#89748,#89749);
#81007=AXIS2_PLACEMENT_3D('',#184484,#89750,#89751);
#81008=AXIS2_PLACEMENT_3D('',#184505,#89752,#89753);
#81009=AXIS2_PLACEMENT_3D('',#184527,#89754,#89755);
#81010=AXIS2_PLACEMENT_3D('',#184548,#89756,#89757);
#81011=AXIS2_PLACEMENT_3D('',#184569,#89758,#89759);
#81012=AXIS2_PLACEMENT_3D('',#184590,#89760,#89761);
#81013=AXIS2_PLACEMENT_3D('',#184591,#89762,#89763);
#81014=AXIS2_PLACEMENT_3D('',#184614,#89766,#89767);
#81015=AXIS2_PLACEMENT_3D('',#184637,#89770,#89771);
#81016=AXIS2_PLACEMENT_3D('',#184639,#89772,#89773);
#81017=AXIS2_PLACEMENT_3D('',#184643,#89775,#89776);
#81018=AXIS2_PLACEMENT_3D('',#184665,#89777,#89778);
#81019=AXIS2_PLACEMENT_3D('',#184668,#89780,#89781);
#81020=AXIS2_PLACEMENT_3D('',#184669,#89782,#89783);
#81021=AXIS2_PLACEMENT_3D('',#184670,#89784,#89785);
#81022=AXIS2_PLACEMENT_3D('',#184672,#89786,#89787);
#81023=AXIS2_PLACEMENT_3D('',#184674,#89788,#89789);
#81024=AXIS2_PLACEMENT_3D('',#184695,#89790,#89791);
#81025=AXIS2_PLACEMENT_3D('',#184697,#89792,#89793);
#81026=AXIS2_PLACEMENT_3D('',#184718,#89794,#89795);
#81027=AXIS2_PLACEMENT_3D('',#184720,#89796,#89797);
#81028=AXIS2_PLACEMENT_3D('',#184740,#89798,#89799);
#81029=AXIS2_PLACEMENT_3D('',#184742,#89800,#89801);
#81030=AXIS2_PLACEMENT_3D('',#184743,#89802,#89803);
#81031=AXIS2_PLACEMENT_3D('',#184744,#89804,#89805);
#81032=AXIS2_PLACEMENT_3D('',#184746,#89806,#89807);
#81033=AXIS2_PLACEMENT_3D('',#184749,#89809,#89810);
#81034=AXIS2_PLACEMENT_3D('',#184750,#89811,#89812);
#81035=AXIS2_PLACEMENT_3D('',#184752,#89813,#89814);
#81036=AXIS2_PLACEMENT_3D('',#184755,#89816,#89817);
#81037=AXIS2_PLACEMENT_3D('',#184756,#89818,#89819);
#81038=AXIS2_PLACEMENT_3D('',#184758,#89820,#89821);
#81039=AXIS2_PLACEMENT_3D('',#184759,#89822,#89823);
#81040=AXIS2_PLACEMENT_3D('',#184760,#89824,#89825);
#81041=AXIS2_PLACEMENT_3D('',#184762,#89826,#89827);
#81042=AXIS2_PLACEMENT_3D('',#184764,#89828,#89829);
#81043=AXIS2_PLACEMENT_3D('',#184765,#89830,#89831);
#81044=AXIS2_PLACEMENT_3D('',#184766,#89832,#89833);
#81045=AXIS2_PLACEMENT_3D('',#184768,#89834,#89835);
#81046=AXIS2_PLACEMENT_3D('',#184770,#89837,#89838);
#81047=AXIS2_PLACEMENT_3D('',#184772,#89839,#89840);
#81048=AXIS2_PLACEMENT_3D('',#184775,#89842,#89843);
#81049=AXIS2_PLACEMENT_3D('',#184776,#89844,#89845);
#81050=AXIS2_PLACEMENT_3D('',#184778,#89846,#89847);
#81051=AXIS2_PLACEMENT_3D('',#184781,#89849,#89850);
#81052=AXIS2_PLACEMENT_3D('',#184782,#89851,#89852);
#81053=AXIS2_PLACEMENT_3D('',#184784,#89853,#89854);
#81054=AXIS2_PLACEMENT_3D('',#184787,#89856,#89857);
#81055=AXIS2_PLACEMENT_3D('',#184788,#89858,#89859);
#81056=AXIS2_PLACEMENT_3D('',#184791,#89860,#89861);
#81057=AXIS2_PLACEMENT_3D('',#184795,#89863,#89864);
#81058=AXIS2_PLACEMENT_3D('',#184799,#89866,#89867);
#81059=AXIS2_PLACEMENT_3D('',#184803,#89869,#89870);
#81060=AXIS2_PLACEMENT_3D('',#184806,#89872,#89873);
#81061=AXIS2_PLACEMENT_3D('',#184808,#89874,#89875);
#81062=AXIS2_PLACEMENT_3D('',#184810,#89877,#89878);
#81063=AXIS2_PLACEMENT_3D('',#184869,#89879,#89880);
#81064=AXIS2_PLACEMENT_3D('',#184908,#89881,#89882);
#81065=AXIS2_PLACEMENT_3D('',#184910,#89883,#89884);
#81066=AXIS2_PLACEMENT_3D('',#184913,#89886,#89887);
#81067=AXIS2_PLACEMENT_3D('',#186585,#89890,#89891);
#81068=AXIS2_PLACEMENT_3D('',#186596,#89894,#89895);
#81069=AXIS2_PLACEMENT_3D('',#186601,#89896,#89897);
#81070=AXIS2_PLACEMENT_3D('',#186602,#89898,#89899);
#81071=AXIS2_PLACEMENT_3D('',#186607,#89900,#89901);
#81072=AXIS2_PLACEMENT_3D('',#186608,#89902,#89903);
#81073=AXIS2_PLACEMENT_3D('',#186611,#89906,#89907);
#81074=AXIS2_PLACEMENT_3D('',#186612,#89908,#89909);
#81075=AXIS2_PLACEMENT_3D('',#186613,#89910,#89911);
#81076=AXIS2_PLACEMENT_3D('',#186614,#89912,#89913);
#81077=AXIS2_PLACEMENT_3D('',#186634,#89914,#89915);
#81078=AXIS2_PLACEMENT_3D('',#186904,#89917,#89918);
#81079=AXIS2_PLACEMENT_3D('',#187074,#89919,#89920);
#81080=AXIS2_PLACEMENT_3D('',#187075,#89921,#89922);
#81081=AXIS2_PLACEMENT_3D('',#187076,#89923,#89924);
#81082=AXIS2_PLACEMENT_3D('',#187077,#89925,#89926);
#81083=AXIS2_PLACEMENT_3D('',#187080,#89927,#89928);
#81084=AXIS2_PLACEMENT_3D('',#187086,#89932,#89933);
#81085=AXIS2_PLACEMENT_3D('',#187090,#89935,#89936);
#81086=AXIS2_PLACEMENT_3D('',#187093,#89938,#89939);
#81087=AXIS2_PLACEMENT_3D('',#187094,#89940,#89941);
#81088=AXIS2_PLACEMENT_3D('',#187096,#89942,#89943);
#81089=AXIS2_PLACEMENT_3D('',#187098,#89944,#89945);
#81090=AXIS2_PLACEMENT_3D('',#187100,#89947,#89948);
#81091=AXIS2_PLACEMENT_3D('',#187101,#89949,#89950);
#81092=AXIS2_PLACEMENT_3D('',#187103,#89951,#89952);
#81093=AXIS2_PLACEMENT_3D('',#187105,#89954,#89955);
#81094=AXIS2_PLACEMENT_3D('',#187106,#89956,#89957);
#81095=AXIS2_PLACEMENT_3D('',#187107,#89958,#89959);
#81096=AXIS2_PLACEMENT_3D('',#187110,#89960,#89961);
#81097=AXIS2_PLACEMENT_3D('',#187116,#89965,#89966);
#81098=AXIS2_PLACEMENT_3D('',#187119,#89967,#89968);
#81099=AXIS2_PLACEMENT_3D('',#187122,#89970,#89971);
#81100=AXIS2_PLACEMENT_3D('',#187124,#89973,#89974);
#81101=AXIS2_PLACEMENT_3D('',#187126,#89975,#89976);
#81102=AXIS2_PLACEMENT_3D('',#187128,#89977,#89978);
#81103=AXIS2_PLACEMENT_3D('',#187130,#89980,#89981);
#81104=AXIS2_PLACEMENT_3D('',#187131,#89982,#89983);
#81105=AXIS2_PLACEMENT_3D('',#187133,#89984,#89985);
#81106=AXIS2_PLACEMENT_3D('',#187135,#89987,#89988);
#81107=AXIS2_PLACEMENT_3D('',#187136,#89989,#89990);
#81108=AXIS2_PLACEMENT_3D('',#187137,#89991,#89992);
#81109=AXIS2_PLACEMENT_3D('',#187142,#89994,#89995);
#81110=AXIS2_PLACEMENT_3D('',#187145,#89997,#89998);
#81111=AXIS2_PLACEMENT_3D('',#187146,#89999,#90000);
#81112=AXIS2_PLACEMENT_3D('',#187151,#90003,#90004);
#81113=AXIS2_PLACEMENT_3D('',#187152,#90005,#90006);
#81114=AXIS2_PLACEMENT_3D('',#187157,#90009,#90010);
#81115=AXIS2_PLACEMENT_3D('',#187158,#90011,#90012);
#81116=AXIS2_PLACEMENT_3D('',#187160,#90013,#90014);
#81117=AXIS2_PLACEMENT_3D('',#187162,#90016,#90017);
#81118=AXIS2_PLACEMENT_3D('',#187163,#90018,#90019);
#81119=AXIS2_PLACEMENT_3D('',#187164,#90020,#90021);
#81120=AXIS2_PLACEMENT_3D('',#187165,#90022,#90023);
#81121=AXIS2_PLACEMENT_3D('',#187170,#90025,#90026);
#81122=AXIS2_PLACEMENT_3D('',#187173,#90028,#90029);
#81123=AXIS2_PLACEMENT_3D('',#187174,#90030,#90031);
#81124=AXIS2_PLACEMENT_3D('',#187178,#90033,#90034);
#81125=AXIS2_PLACEMENT_3D('',#187179,#90035,#90036);
#81126=AXIS2_PLACEMENT_3D('',#187180,#90037,#90038);
#81127=AXIS2_PLACEMENT_3D('',#187184,#90040,#90041);
#81128=AXIS2_PLACEMENT_3D('',#187185,#90042,#90043);
#81129=AXIS2_PLACEMENT_3D('',#187186,#90044,#90045);
#81130=AXIS2_PLACEMENT_3D('',#187187,#90046,#90047);
#81131=AXIS2_PLACEMENT_3D('',#187188,#90048,#90049);
#81132=AXIS2_PLACEMENT_3D('',#187189,#90050,#90051);
#81133=AXIS2_PLACEMENT_3D('',#187194,#90053,#90054);
#81134=AXIS2_PLACEMENT_3D('',#187197,#90056,#90057);
#81135=AXIS2_PLACEMENT_3D('',#187198,#90058,#90059);
#81136=AXIS2_PLACEMENT_3D('',#187202,#90061,#90062);
#81137=AXIS2_PLACEMENT_3D('',#187203,#90063,#90064);
#81138=AXIS2_PLACEMENT_3D('',#187204,#90065,#90066);
#81139=AXIS2_PLACEMENT_3D('',#187208,#90068,#90069);
#81140=AXIS2_PLACEMENT_3D('',#187209,#90070,#90071);
#81141=AXIS2_PLACEMENT_3D('',#187210,#90072,#90073);
#81142=AXIS2_PLACEMENT_3D('',#187211,#90074,#90075);
#81143=AXIS2_PLACEMENT_3D('',#187212,#90076,#90077);
#81144=AXIS2_PLACEMENT_3D('',#187213,#90078,#90079);
#81145=AXIS2_PLACEMENT_3D('',#187218,#90081,#90082);
#81146=AXIS2_PLACEMENT_3D('',#187221,#90084,#90085);
#81147=AXIS2_PLACEMENT_3D('',#187222,#90086,#90087);
#81148=AXIS2_PLACEMENT_3D('',#187226,#90089,#90090);
#81149=AXIS2_PLACEMENT_3D('',#187227,#90091,#90092);
#81150=AXIS2_PLACEMENT_3D('',#187228,#90093,#90094);
#81151=AXIS2_PLACEMENT_3D('',#187232,#90096,#90097);
#81152=AXIS2_PLACEMENT_3D('',#187233,#90098,#90099);
#81153=AXIS2_PLACEMENT_3D('',#187234,#90100,#90101);
#81154=AXIS2_PLACEMENT_3D('',#187235,#90102,#90103);
#81155=AXIS2_PLACEMENT_3D('',#187236,#90104,#90105);
#81156=AXIS2_PLACEMENT_3D('',#187237,#90106,#90107);
#81157=AXIS2_PLACEMENT_3D('',#187242,#90109,#90110);
#81158=AXIS2_PLACEMENT_3D('',#187245,#90112,#90113);
#81159=AXIS2_PLACEMENT_3D('',#187246,#90114,#90115);
#81160=AXIS2_PLACEMENT_3D('',#187250,#90117,#90118);
#81161=AXIS2_PLACEMENT_3D('',#187251,#90119,#90120);
#81162=AXIS2_PLACEMENT_3D('',#187252,#90121,#90122);
#81163=AXIS2_PLACEMENT_3D('',#187256,#90124,#90125);
#81164=AXIS2_PLACEMENT_3D('',#187257,#90126,#90127);
#81165=AXIS2_PLACEMENT_3D('',#187258,#90128,#90129);
#81166=AXIS2_PLACEMENT_3D('',#187259,#90130,#90131);
#81167=AXIS2_PLACEMENT_3D('',#187260,#90132,#90133);
#81168=AXIS2_PLACEMENT_3D('',#187261,#90134,#90135);
#81169=AXIS2_PLACEMENT_3D('',#187264,#90136,#90137);
#81170=AXIS2_PLACEMENT_3D('',#187270,#90141,#90142);
#81171=AXIS2_PLACEMENT_3D('',#187273,#90143,#90144);
#81172=AXIS2_PLACEMENT_3D('',#187276,#90146,#90147);
#81173=AXIS2_PLACEMENT_3D('',#187278,#90149,#90150);
#81174=AXIS2_PLACEMENT_3D('',#187280,#90151,#90152);
#81175=AXIS2_PLACEMENT_3D('',#187282,#90153,#90154);
#81176=AXIS2_PLACEMENT_3D('',#187284,#90156,#90157);
#81177=AXIS2_PLACEMENT_3D('',#187285,#90158,#90159);
#81178=AXIS2_PLACEMENT_3D('',#187287,#90160,#90161);
#81179=AXIS2_PLACEMENT_3D('',#187289,#90163,#90164);
#81180=AXIS2_PLACEMENT_3D('',#187290,#90165,#90166);
#81181=AXIS2_PLACEMENT_3D('',#187291,#90167,#90168);
#81182=AXIS2_PLACEMENT_3D('',#187296,#90170,#90171);
#81183=AXIS2_PLACEMENT_3D('',#187299,#90173,#90174);
#81184=AXIS2_PLACEMENT_3D('',#187300,#90175,#90176);
#81185=AXIS2_PLACEMENT_3D('',#187306,#90179,#90180);
#81186=AXIS2_PLACEMENT_3D('',#187307,#90181,#90182);
#81187=AXIS2_PLACEMENT_3D('',#187308,#90183,#90184);
#81188=AXIS2_PLACEMENT_3D('',#187313,#90187,#90188);
#81189=AXIS2_PLACEMENT_3D('',#187314,#90189,#90190);
#81190=AXIS2_PLACEMENT_3D('',#187316,#90191,#90192);
#81191=AXIS2_PLACEMENT_3D('',#187318,#90194,#90195);
#81192=AXIS2_PLACEMENT_3D('',#187319,#90196,#90197);
#81193=AXIS2_PLACEMENT_3D('',#187320,#90198,#90199);
#81194=AXIS2_PLACEMENT_3D('',#187321,#90200,#90201);
#81195=AXIS2_PLACEMENT_3D('',#187326,#90203,#90204);
#81196=AXIS2_PLACEMENT_3D('',#187329,#90206,#90207);
#81197=AXIS2_PLACEMENT_3D('',#187330,#90208,#90209);
#81198=AXIS2_PLACEMENT_3D('',#187336,#90212,#90213);
#81199=AXIS2_PLACEMENT_3D('',#187337,#90214,#90215);
#81200=AXIS2_PLACEMENT_3D('',#187338,#90216,#90217);
#81201=AXIS2_PLACEMENT_3D('',#187343,#90220,#90221);
#81202=AXIS2_PLACEMENT_3D('',#187344,#90222,#90223);
#81203=AXIS2_PLACEMENT_3D('',#187346,#90224,#90225);
#81204=AXIS2_PLACEMENT_3D('',#187348,#90227,#90228);
#81205=AXIS2_PLACEMENT_3D('',#187349,#90229,#90230);
#81206=AXIS2_PLACEMENT_3D('',#187350,#90231,#90232);
#81207=AXIS2_PLACEMENT_3D('',#187351,#90233,#90234);
#81208=AXIS2_PLACEMENT_3D('',#187356,#90236,#90237);
#81209=AXIS2_PLACEMENT_3D('',#187359,#90239,#90240);
#81210=AXIS2_PLACEMENT_3D('',#187360,#90241,#90242);
#81211=AXIS2_PLACEMENT_3D('',#187364,#90244,#90245);
#81212=AXIS2_PLACEMENT_3D('',#187365,#90246,#90247);
#81213=AXIS2_PLACEMENT_3D('',#187366,#90248,#90249);
#81214=AXIS2_PLACEMENT_3D('',#187372,#90252,#90253);
#81215=AXIS2_PLACEMENT_3D('',#187373,#90254,#90255);
#81216=AXIS2_PLACEMENT_3D('',#187374,#90256,#90257);
#81217=AXIS2_PLACEMENT_3D('',#187376,#90258,#90259);
#81218=AXIS2_PLACEMENT_3D('',#187378,#90261,#90262);
#81219=AXIS2_PLACEMENT_3D('',#187379,#90263,#90264);
#81220=AXIS2_PLACEMENT_3D('',#187380,#90265,#90266);
#81221=AXIS2_PLACEMENT_3D('',#187381,#90267,#90268);
#81222=AXIS2_PLACEMENT_3D('',#187386,#90270,#90271);
#81223=AXIS2_PLACEMENT_3D('',#187389,#90273,#90274);
#81224=AXIS2_PLACEMENT_3D('',#187390,#90275,#90276);
#81225=AXIS2_PLACEMENT_3D('',#187394,#90278,#90279);
#81226=AXIS2_PLACEMENT_3D('',#187395,#90280,#90281);
#81227=AXIS2_PLACEMENT_3D('',#187396,#90282,#90283);
#81228=AXIS2_PLACEMENT_3D('',#187400,#90285,#90286);
#81229=AXIS2_PLACEMENT_3D('',#187401,#90287,#90288);
#81230=AXIS2_PLACEMENT_3D('',#187402,#90289,#90290);
#81231=AXIS2_PLACEMENT_3D('',#187403,#90291,#90292);
#81232=AXIS2_PLACEMENT_3D('',#187404,#90293,#90294);
#81233=AXIS2_PLACEMENT_3D('',#187405,#90295,#90296);
#81234=AXIS2_PLACEMENT_3D('',#187410,#90298,#90299);
#81235=AXIS2_PLACEMENT_3D('',#187413,#90301,#90302);
#81236=AXIS2_PLACEMENT_3D('',#187414,#90303,#90304);
#81237=AXIS2_PLACEMENT_3D('',#187420,#90307,#90308);
#81238=AXIS2_PLACEMENT_3D('',#187421,#90309,#90310);
#81239=AXIS2_PLACEMENT_3D('',#187422,#90311,#90312);
#81240=AXIS2_PLACEMENT_3D('',#187427,#90315,#90316);
#81241=AXIS2_PLACEMENT_3D('',#187428,#90317,#90318);
#81242=AXIS2_PLACEMENT_3D('',#187430,#90319,#90320);
#81243=AXIS2_PLACEMENT_3D('',#187432,#90322,#90323);
#81244=AXIS2_PLACEMENT_3D('',#187433,#90324,#90325);
#81245=AXIS2_PLACEMENT_3D('',#187434,#90326,#90327);
#81246=AXIS2_PLACEMENT_3D('',#187435,#90328,#90329);
#81247=AXIS2_PLACEMENT_3D('',#187440,#90331,#90332);
#81248=AXIS2_PLACEMENT_3D('',#187443,#90334,#90335);
#81249=AXIS2_PLACEMENT_3D('',#187444,#90336,#90337);
#81250=AXIS2_PLACEMENT_3D('',#187450,#90340,#90341);
#81251=AXIS2_PLACEMENT_3D('',#187451,#90342,#90343);
#81252=AXIS2_PLACEMENT_3D('',#187452,#90344,#90345);
#81253=AXIS2_PLACEMENT_3D('',#187457,#90348,#90349);
#81254=AXIS2_PLACEMENT_3D('',#187458,#90350,#90351);
#81255=AXIS2_PLACEMENT_3D('',#187460,#90352,#90353);
#81256=AXIS2_PLACEMENT_3D('',#187462,#90355,#90356);
#81257=AXIS2_PLACEMENT_3D('',#187463,#90357,#90358);
#81258=AXIS2_PLACEMENT_3D('',#187464,#90359,#90360);
#81259=AXIS2_PLACEMENT_3D('',#187465,#90361,#90362);
#81260=AXIS2_PLACEMENT_3D('',#187470,#90364,#90365);
#81261=AXIS2_PLACEMENT_3D('',#187473,#90367,#90368);
#81262=AXIS2_PLACEMENT_3D('',#187474,#90369,#90370);
#81263=AXIS2_PLACEMENT_3D('',#187480,#90373,#90374);
#81264=AXIS2_PLACEMENT_3D('',#187481,#90375,#90376);
#81265=AXIS2_PLACEMENT_3D('',#187482,#90377,#90378);
#81266=AXIS2_PLACEMENT_3D('',#187487,#90381,#90382);
#81267=AXIS2_PLACEMENT_3D('',#187488,#90383,#90384);
#81268=AXIS2_PLACEMENT_3D('',#187490,#90385,#90386);
#81269=AXIS2_PLACEMENT_3D('',#187492,#90388,#90389);
#81270=AXIS2_PLACEMENT_3D('',#187493,#90390,#90391);
#81271=AXIS2_PLACEMENT_3D('',#187494,#90392,#90393);
#81272=AXIS2_PLACEMENT_3D('',#187495,#90394,#90395);
#81273=AXIS2_PLACEMENT_3D('',#187500,#90397,#90398);
#81274=AXIS2_PLACEMENT_3D('',#187503,#90400,#90401);
#81275=AXIS2_PLACEMENT_3D('',#187504,#90402,#90403);
#81276=AXIS2_PLACEMENT_3D('',#187510,#90406,#90407);
#81277=AXIS2_PLACEMENT_3D('',#187511,#90408,#90409);
#81278=AXIS2_PLACEMENT_3D('',#187512,#90410,#90411);
#81279=AXIS2_PLACEMENT_3D('',#187517,#90414,#90415);
#81280=AXIS2_PLACEMENT_3D('',#187518,#90416,#90417);
#81281=AXIS2_PLACEMENT_3D('',#187520,#90418,#90419);
#81282=AXIS2_PLACEMENT_3D('',#187522,#90421,#90422);
#81283=AXIS2_PLACEMENT_3D('',#187523,#90423,#90424);
#81284=AXIS2_PLACEMENT_3D('',#187524,#90425,#90426);
#81285=AXIS2_PLACEMENT_3D('',#187525,#90427,#90428);
#81286=AXIS2_PLACEMENT_3D('',#187530,#90430,#90431);
#81287=AXIS2_PLACEMENT_3D('',#187533,#90433,#90434);
#81288=AXIS2_PLACEMENT_3D('',#187534,#90435,#90436);
#81289=AXIS2_PLACEMENT_3D('',#187538,#90438,#90439);
#81290=AXIS2_PLACEMENT_3D('',#187539,#90440,#90441);
#81291=AXIS2_PLACEMENT_3D('',#187540,#90442,#90443);
#81292=AXIS2_PLACEMENT_3D('',#187544,#90445,#90446);
#81293=AXIS2_PLACEMENT_3D('',#187545,#90447,#90448);
#81294=AXIS2_PLACEMENT_3D('',#187546,#90449,#90450);
#81295=AXIS2_PLACEMENT_3D('',#187547,#90451,#90452);
#81296=AXIS2_PLACEMENT_3D('',#187548,#90453,#90454);
#81297=AXIS2_PLACEMENT_3D('',#187549,#90455,#90456);
#81298=AXIS2_PLACEMENT_3D('',#187554,#90458,#90459);
#81299=AXIS2_PLACEMENT_3D('',#187557,#90461,#90462);
#81300=AXIS2_PLACEMENT_3D('',#187558,#90463,#90464);
#81301=AXIS2_PLACEMENT_3D('',#187562,#90466,#90467);
#81302=AXIS2_PLACEMENT_3D('',#187563,#90468,#90469);
#81303=AXIS2_PLACEMENT_3D('',#187564,#90470,#90471);
#81304=AXIS2_PLACEMENT_3D('',#187568,#90473,#90474);
#81305=AXIS2_PLACEMENT_3D('',#187569,#90475,#90476);
#81306=AXIS2_PLACEMENT_3D('',#187570,#90477,#90478);
#81307=AXIS2_PLACEMENT_3D('',#187571,#90479,#90480);
#81308=AXIS2_PLACEMENT_3D('',#187572,#90481,#90482);
#81309=AXIS2_PLACEMENT_3D('',#187573,#90483,#90484);
#81310=AXIS2_PLACEMENT_3D('',#187578,#90486,#90487);
#81311=AXIS2_PLACEMENT_3D('',#187581,#90489,#90490);
#81312=AXIS2_PLACEMENT_3D('',#187582,#90491,#90492);
#81313=AXIS2_PLACEMENT_3D('',#187586,#90494,#90495);
#81314=AXIS2_PLACEMENT_3D('',#187587,#90496,#90497);
#81315=AXIS2_PLACEMENT_3D('',#187588,#90498,#90499);
#81316=AXIS2_PLACEMENT_3D('',#187592,#90501,#90502);
#81317=AXIS2_PLACEMENT_3D('',#187593,#90503,#90504);
#81318=AXIS2_PLACEMENT_3D('',#187594,#90505,#90506);
#81319=AXIS2_PLACEMENT_3D('',#187595,#90507,#90508);
#81320=AXIS2_PLACEMENT_3D('',#187596,#90509,#90510);
#81321=AXIS2_PLACEMENT_3D('',#187597,#90511,#90512);
#81322=AXIS2_PLACEMENT_3D('',#187602,#90514,#90515);
#81323=AXIS2_PLACEMENT_3D('',#187605,#90517,#90518);
#81324=AXIS2_PLACEMENT_3D('',#187606,#90519,#90520);
#81325=AXIS2_PLACEMENT_3D('',#187610,#90522,#90523);
#81326=AXIS2_PLACEMENT_3D('',#187611,#90524,#90525);
#81327=AXIS2_PLACEMENT_3D('',#187612,#90526,#90527);
#81328=AXIS2_PLACEMENT_3D('',#187616,#90529,#90530);
#81329=AXIS2_PLACEMENT_3D('',#187617,#90531,#90532);
#81330=AXIS2_PLACEMENT_3D('',#187618,#90533,#90534);
#81331=AXIS2_PLACEMENT_3D('',#187619,#90535,#90536);
#81332=AXIS2_PLACEMENT_3D('',#187620,#90537,#90538);
#81333=AXIS2_PLACEMENT_3D('',#187621,#90539,#90540);
#81334=AXIS2_PLACEMENT_3D('',#187626,#90542,#90543);
#81335=AXIS2_PLACEMENT_3D('',#187629,#90545,#90546);
#81336=AXIS2_PLACEMENT_3D('',#187630,#90547,#90548);
#81337=AXIS2_PLACEMENT_3D('',#187634,#90550,#90551);
#81338=AXIS2_PLACEMENT_3D('',#187635,#90552,#90553);
#81339=AXIS2_PLACEMENT_3D('',#187636,#90554,#90555);
#81340=AXIS2_PLACEMENT_3D('',#187640,#90557,#90558);
#81341=AXIS2_PLACEMENT_3D('',#187641,#90559,#90560);
#81342=AXIS2_PLACEMENT_3D('',#187642,#90561,#90562);
#81343=AXIS2_PLACEMENT_3D('',#187643,#90563,#90564);
#81344=AXIS2_PLACEMENT_3D('',#187644,#90565,#90566);
#81345=AXIS2_PLACEMENT_3D('',#187645,#90567,#90568);
#81346=AXIS2_PLACEMENT_3D('',#187650,#90570,#90571);
#81347=AXIS2_PLACEMENT_3D('',#187653,#90573,#90574);
#81348=AXIS2_PLACEMENT_3D('',#187654,#90575,#90576);
#81349=AXIS2_PLACEMENT_3D('',#187658,#90578,#90579);
#81350=AXIS2_PLACEMENT_3D('',#187659,#90580,#90581);
#81351=AXIS2_PLACEMENT_3D('',#187660,#90582,#90583);
#81352=AXIS2_PLACEMENT_3D('',#187664,#90585,#90586);
#81353=AXIS2_PLACEMENT_3D('',#187665,#90587,#90588);
#81354=AXIS2_PLACEMENT_3D('',#187666,#90589,#90590);
#81355=AXIS2_PLACEMENT_3D('',#187667,#90591,#90592);
#81356=AXIS2_PLACEMENT_3D('',#187668,#90593,#90594);
#81357=AXIS2_PLACEMENT_3D('',#187669,#90595,#90596);
#81358=AXIS2_PLACEMENT_3D('',#187672,#90597,#90598);
#81359=AXIS2_PLACEMENT_3D('',#187676,#90600,#90601);
#81360=AXIS2_PLACEMENT_3D('',#187678,#90603,#90604);
#81361=AXIS2_PLACEMENT_3D('',#187680,#90605,#90606);
#81362=AXIS2_PLACEMENT_3D('',#187683,#90608,#90609);
#81363=AXIS2_PLACEMENT_3D('',#187684,#90610,#90611);
#81364=AXIS2_PLACEMENT_3D('',#187688,#90613,#90614);
#81365=AXIS2_PLACEMENT_3D('',#187690,#90615,#90616);
#81366=AXIS2_PLACEMENT_3D('',#187692,#90618,#90619);
#81367=AXIS2_PLACEMENT_3D('',#187693,#90620,#90621);
#81368=AXIS2_PLACEMENT_3D('',#187695,#90622,#90623);
#81369=AXIS2_PLACEMENT_3D('',#187697,#90625,#90626);
#81370=AXIS2_PLACEMENT_3D('',#187698,#90627,#90628);
#81371=AXIS2_PLACEMENT_3D('',#187699,#90629,#90630);
#81372=AXIS2_PLACEMENT_3D('',#187704,#90632,#90633);
#81373=AXIS2_PLACEMENT_3D('',#187707,#90635,#90636);
#81374=AXIS2_PLACEMENT_3D('',#187708,#90637,#90638);
#81375=AXIS2_PLACEMENT_3D('',#187714,#90641,#90642);
#81376=AXIS2_PLACEMENT_3D('',#187715,#90643,#90644);
#81377=AXIS2_PLACEMENT_3D('',#187716,#90645,#90646);
#81378=AXIS2_PLACEMENT_3D('',#187721,#90649,#90650);
#81379=AXIS2_PLACEMENT_3D('',#187722,#90651,#90652);
#81380=AXIS2_PLACEMENT_3D('',#187724,#90653,#90654);
#81381=AXIS2_PLACEMENT_3D('',#187726,#90656,#90657);
#81382=AXIS2_PLACEMENT_3D('',#187727,#90658,#90659);
#81383=AXIS2_PLACEMENT_3D('',#187728,#90660,#90661);
#81384=AXIS2_PLACEMENT_3D('',#187729,#90662,#90663);
#81385=AXIS2_PLACEMENT_3D('',#187734,#90665,#90666);
#81386=AXIS2_PLACEMENT_3D('',#187737,#90668,#90669);
#81387=AXIS2_PLACEMENT_3D('',#187738,#90670,#90671);
#81388=AXIS2_PLACEMENT_3D('',#187742,#90673,#90674);
#81389=AXIS2_PLACEMENT_3D('',#187743,#90675,#90676);
#81390=AXIS2_PLACEMENT_3D('',#187744,#90677,#90678);
#81391=AXIS2_PLACEMENT_3D('',#187748,#90680,#90681);
#81392=AXIS2_PLACEMENT_3D('',#187749,#90682,#90683);
#81393=AXIS2_PLACEMENT_3D('',#187750,#90684,#90685);
#81394=AXIS2_PLACEMENT_3D('',#187751,#90686,#90687);
#81395=AXIS2_PLACEMENT_3D('',#187752,#90688,#90689);
#81396=AXIS2_PLACEMENT_3D('',#187753,#90690,#90691);
#81397=AXIS2_PLACEMENT_3D('',#187758,#90693,#90694);
#81398=AXIS2_PLACEMENT_3D('',#187761,#90696,#90697);
#81399=AXIS2_PLACEMENT_3D('',#187762,#90698,#90699);
#81400=AXIS2_PLACEMENT_3D('',#187766,#90701,#90702);
#81401=AXIS2_PLACEMENT_3D('',#187767,#90703,#90704);
#81402=AXIS2_PLACEMENT_3D('',#187768,#90705,#90706);
#81403=AXIS2_PLACEMENT_3D('',#187772,#90708,#90709);
#81404=AXIS2_PLACEMENT_3D('',#187773,#90710,#90711);
#81405=AXIS2_PLACEMENT_3D('',#187774,#90712,#90713);
#81406=AXIS2_PLACEMENT_3D('',#187775,#90714,#90715);
#81407=AXIS2_PLACEMENT_3D('',#187776,#90716,#90717);
#81408=AXIS2_PLACEMENT_3D('',#187777,#90718,#90719);
#81409=AXIS2_PLACEMENT_3D('',#187782,#90721,#90722);
#81410=AXIS2_PLACEMENT_3D('',#187785,#90724,#90725);
#81411=AXIS2_PLACEMENT_3D('',#187786,#90726,#90727);
#81412=AXIS2_PLACEMENT_3D('',#187790,#90729,#90730);
#81413=AXIS2_PLACEMENT_3D('',#187791,#90731,#90732);
#81414=AXIS2_PLACEMENT_3D('',#187792,#90733,#90734);
#81415=AXIS2_PLACEMENT_3D('',#187796,#90736,#90737);
#81416=AXIS2_PLACEMENT_3D('',#187797,#90738,#90739);
#81417=AXIS2_PLACEMENT_3D('',#187798,#90740,#90741);
#81418=AXIS2_PLACEMENT_3D('',#187799,#90742,#90743);
#81419=AXIS2_PLACEMENT_3D('',#187800,#90744,#90745);
#81420=AXIS2_PLACEMENT_3D('',#187801,#90746,#90747);
#81421=AXIS2_PLACEMENT_3D('',#187806,#90749,#90750);
#81422=AXIS2_PLACEMENT_3D('',#187809,#90752,#90753);
#81423=AXIS2_PLACEMENT_3D('',#187810,#90754,#90755);
#81424=AXIS2_PLACEMENT_3D('',#187814,#90757,#90758);
#81425=AXIS2_PLACEMENT_3D('',#187815,#90759,#90760);
#81426=AXIS2_PLACEMENT_3D('',#187816,#90761,#90762);
#81427=AXIS2_PLACEMENT_3D('',#187820,#90764,#90765);
#81428=AXIS2_PLACEMENT_3D('',#187821,#90766,#90767);
#81429=AXIS2_PLACEMENT_3D('',#187822,#90768,#90769);
#81430=AXIS2_PLACEMENT_3D('',#187823,#90770,#90771);
#81431=AXIS2_PLACEMENT_3D('',#187824,#90772,#90773);
#81432=AXIS2_PLACEMENT_3D('',#187825,#90774,#90775);
#81433=AXIS2_PLACEMENT_3D('',#187830,#90777,#90778);
#81434=AXIS2_PLACEMENT_3D('',#187833,#90780,#90781);
#81435=AXIS2_PLACEMENT_3D('',#187834,#90782,#90783);
#81436=AXIS2_PLACEMENT_3D('',#187838,#90785,#90786);
#81437=AXIS2_PLACEMENT_3D('',#187839,#90787,#90788);
#81438=AXIS2_PLACEMENT_3D('',#187840,#90789,#90790);
#81439=AXIS2_PLACEMENT_3D('',#187844,#90792,#90793);
#81440=AXIS2_PLACEMENT_3D('',#187845,#90794,#90795);
#81441=AXIS2_PLACEMENT_3D('',#187846,#90796,#90797);
#81442=AXIS2_PLACEMENT_3D('',#187847,#90798,#90799);
#81443=AXIS2_PLACEMENT_3D('',#187848,#90800,#90801);
#81444=AXIS2_PLACEMENT_3D('',#187849,#90802,#90803);
#81445=AXIS2_PLACEMENT_3D('',#187854,#90805,#90806);
#81446=AXIS2_PLACEMENT_3D('',#187857,#90808,#90809);
#81447=AXIS2_PLACEMENT_3D('',#187858,#90810,#90811);
#81448=AXIS2_PLACEMENT_3D('',#187862,#90813,#90814);
#81449=AXIS2_PLACEMENT_3D('',#187863,#90815,#90816);
#81450=AXIS2_PLACEMENT_3D('',#187864,#90817,#90818);
#81451=AXIS2_PLACEMENT_3D('',#187868,#90820,#90821);
#81452=AXIS2_PLACEMENT_3D('',#187869,#90822,#90823);
#81453=AXIS2_PLACEMENT_3D('',#187870,#90824,#90825);
#81454=AXIS2_PLACEMENT_3D('',#187871,#90826,#90827);
#81455=AXIS2_PLACEMENT_3D('',#187872,#90828,#90829);
#81456=AXIS2_PLACEMENT_3D('',#187873,#90830,#90831);
#81457=AXIS2_PLACEMENT_3D('',#187878,#90833,#90834);
#81458=AXIS2_PLACEMENT_3D('',#187881,#90836,#90837);
#81459=AXIS2_PLACEMENT_3D('',#187882,#90838,#90839);
#81460=AXIS2_PLACEMENT_3D('',#187886,#90841,#90842);
#81461=AXIS2_PLACEMENT_3D('',#187887,#90843,#90844);
#81462=AXIS2_PLACEMENT_3D('',#187888,#90845,#90846);
#81463=AXIS2_PLACEMENT_3D('',#187892,#90848,#90849);
#81464=AXIS2_PLACEMENT_3D('',#187893,#90850,#90851);
#81465=AXIS2_PLACEMENT_3D('',#187894,#90852,#90853);
#81466=AXIS2_PLACEMENT_3D('',#187895,#90854,#90855);
#81467=AXIS2_PLACEMENT_3D('',#187896,#90856,#90857);
#81468=AXIS2_PLACEMENT_3D('',#187897,#90858,#90859);
#81469=AXIS2_PLACEMENT_3D('',#187902,#90861,#90862);
#81470=AXIS2_PLACEMENT_3D('',#187905,#90864,#90865);
#81471=AXIS2_PLACEMENT_3D('',#187906,#90866,#90867);
#81472=AXIS2_PLACEMENT_3D('',#187910,#90869,#90870);
#81473=AXIS2_PLACEMENT_3D('',#187911,#90871,#90872);
#81474=AXIS2_PLACEMENT_3D('',#187912,#90873,#90874);
#81475=AXIS2_PLACEMENT_3D('',#187916,#90876,#90877);
#81476=AXIS2_PLACEMENT_3D('',#187917,#90878,#90879);
#81477=AXIS2_PLACEMENT_3D('',#187918,#90880,#90881);
#81478=AXIS2_PLACEMENT_3D('',#187919,#90882,#90883);
#81479=AXIS2_PLACEMENT_3D('',#187920,#90884,#90885);
#81480=AXIS2_PLACEMENT_3D('',#187921,#90886,#90887);
#81481=AXIS2_PLACEMENT_3D('',#187926,#90889,#90890);
#81482=AXIS2_PLACEMENT_3D('',#187929,#90892,#90893);
#81483=AXIS2_PLACEMENT_3D('',#187930,#90894,#90895);
#81484=AXIS2_PLACEMENT_3D('',#187936,#90898,#90899);
#81485=AXIS2_PLACEMENT_3D('',#187937,#90900,#90901);
#81486=AXIS2_PLACEMENT_3D('',#187938,#90902,#90903);
#81487=AXIS2_PLACEMENT_3D('',#187943,#90906,#90907);
#81488=AXIS2_PLACEMENT_3D('',#187944,#90908,#90909);
#81489=AXIS2_PLACEMENT_3D('',#187946,#90910,#90911);
#81490=AXIS2_PLACEMENT_3D('',#187948,#90913,#90914);
#81491=AXIS2_PLACEMENT_3D('',#187949,#90915,#90916);
#81492=AXIS2_PLACEMENT_3D('',#187950,#90917,#90918);
#81493=AXIS2_PLACEMENT_3D('',#187951,#90919,#90920);
#81494=AXIS2_PLACEMENT_3D('',#187956,#90922,#90923);
#81495=AXIS2_PLACEMENT_3D('',#187959,#90925,#90926);
#81496=AXIS2_PLACEMENT_3D('',#187960,#90927,#90928);
#81497=AXIS2_PLACEMENT_3D('',#187966,#90931,#90932);
#81498=AXIS2_PLACEMENT_3D('',#187967,#90933,#90934);
#81499=AXIS2_PLACEMENT_3D('',#187968,#90935,#90936);
#81500=AXIS2_PLACEMENT_3D('',#187973,#90939,#90940);
#81501=AXIS2_PLACEMENT_3D('',#187974,#90941,#90942);
#81502=AXIS2_PLACEMENT_3D('',#187976,#90943,#90944);
#81503=AXIS2_PLACEMENT_3D('',#187978,#90946,#90947);
#81504=AXIS2_PLACEMENT_3D('',#187979,#90948,#90949);
#81505=AXIS2_PLACEMENT_3D('',#187980,#90950,#90951);
#81506=AXIS2_PLACEMENT_3D('',#187981,#90952,#90953);
#81507=AXIS2_PLACEMENT_3D('',#187986,#90955,#90956);
#81508=AXIS2_PLACEMENT_3D('',#187989,#90958,#90959);
#81509=AXIS2_PLACEMENT_3D('',#187990,#90960,#90961);
#81510=AXIS2_PLACEMENT_3D('',#187994,#90963,#90964);
#81511=AXIS2_PLACEMENT_3D('',#187995,#90965,#90966);
#81512=AXIS2_PLACEMENT_3D('',#187996,#90967,#90968);
#81513=AXIS2_PLACEMENT_3D('',#188000,#90970,#90971);
#81514=AXIS2_PLACEMENT_3D('',#188001,#90972,#90973);
#81515=AXIS2_PLACEMENT_3D('',#188002,#90974,#90975);
#81516=AXIS2_PLACEMENT_3D('',#188003,#90976,#90977);
#81517=AXIS2_PLACEMENT_3D('',#188004,#90978,#90979);
#81518=AXIS2_PLACEMENT_3D('',#188005,#90980,#90981);
#81519=AXIS2_PLACEMENT_3D('',#188010,#90983,#90984);
#81520=AXIS2_PLACEMENT_3D('',#188013,#90986,#90987);
#81521=AXIS2_PLACEMENT_3D('',#188014,#90988,#90989);
#81522=AXIS2_PLACEMENT_3D('',#188018,#90991,#90992);
#81523=AXIS2_PLACEMENT_3D('',#188019,#90993,#90994);
#81524=AXIS2_PLACEMENT_3D('',#188020,#90995,#90996);
#81525=AXIS2_PLACEMENT_3D('',#188024,#90998,#90999);
#81526=AXIS2_PLACEMENT_3D('',#188025,#91000,#91001);
#81527=AXIS2_PLACEMENT_3D('',#188026,#91002,#91003);
#81528=AXIS2_PLACEMENT_3D('',#188027,#91004,#91005);
#81529=AXIS2_PLACEMENT_3D('',#188028,#91006,#91007);
#81530=AXIS2_PLACEMENT_3D('',#188029,#91008,#91009);
#81531=AXIS2_PLACEMENT_3D('',#188034,#91011,#91012);
#81532=AXIS2_PLACEMENT_3D('',#188037,#91014,#91015);
#81533=AXIS2_PLACEMENT_3D('',#188038,#91016,#91017);
#81534=AXIS2_PLACEMENT_3D('',#188042,#91019,#91020);
#81535=AXIS2_PLACEMENT_3D('',#188043,#91021,#91022);
#81536=AXIS2_PLACEMENT_3D('',#188044,#91023,#91024);
#81537=AXIS2_PLACEMENT_3D('',#188048,#91026,#91027);
#81538=AXIS2_PLACEMENT_3D('',#188049,#91028,#91029);
#81539=AXIS2_PLACEMENT_3D('',#188050,#91030,#91031);
#81540=AXIS2_PLACEMENT_3D('',#188051,#91032,#91033);
#81541=AXIS2_PLACEMENT_3D('',#188052,#91034,#91035);
#81542=AXIS2_PLACEMENT_3D('',#188053,#91036,#91037);
#81543=AXIS2_PLACEMENT_3D('',#188058,#91039,#91040);
#81544=AXIS2_PLACEMENT_3D('',#188061,#91042,#91043);
#81545=AXIS2_PLACEMENT_3D('',#188062,#91044,#91045);
#81546=AXIS2_PLACEMENT_3D('',#188066,#91047,#91048);
#81547=AXIS2_PLACEMENT_3D('',#188067,#91049,#91050);
#81548=AXIS2_PLACEMENT_3D('',#188068,#91051,#91052);
#81549=AXIS2_PLACEMENT_3D('',#188072,#91054,#91055);
#81550=AXIS2_PLACEMENT_3D('',#188073,#91056,#91057);
#81551=AXIS2_PLACEMENT_3D('',#188074,#91058,#91059);
#81552=AXIS2_PLACEMENT_3D('',#188075,#91060,#91061);
#81553=AXIS2_PLACEMENT_3D('',#188076,#91062,#91063);
#81554=AXIS2_PLACEMENT_3D('',#188077,#91064,#91065);
#81555=AXIS2_PLACEMENT_3D('',#188082,#91067,#91068);
#81556=AXIS2_PLACEMENT_3D('',#188085,#91070,#91071);
#81557=AXIS2_PLACEMENT_3D('',#188086,#91072,#91073);
#81558=AXIS2_PLACEMENT_3D('',#188090,#91075,#91076);
#81559=AXIS2_PLACEMENT_3D('',#188091,#91077,#91078);
#81560=AXIS2_PLACEMENT_3D('',#188092,#91079,#91080);
#81561=AXIS2_PLACEMENT_3D('',#188096,#91082,#91083);
#81562=AXIS2_PLACEMENT_3D('',#188097,#91084,#91085);
#81563=AXIS2_PLACEMENT_3D('',#188098,#91086,#91087);
#81564=AXIS2_PLACEMENT_3D('',#188099,#91088,#91089);
#81565=AXIS2_PLACEMENT_3D('',#188100,#91090,#91091);
#81566=AXIS2_PLACEMENT_3D('',#188101,#91092,#91093);
#81567=AXIS2_PLACEMENT_3D('',#188106,#91095,#91096);
#81568=AXIS2_PLACEMENT_3D('',#188109,#91098,#91099);
#81569=AXIS2_PLACEMENT_3D('',#188110,#91100,#91101);
#81570=AXIS2_PLACEMENT_3D('',#188114,#91103,#91104);
#81571=AXIS2_PLACEMENT_3D('',#188115,#91105,#91106);
#81572=AXIS2_PLACEMENT_3D('',#188116,#91107,#91108);
#81573=AXIS2_PLACEMENT_3D('',#188120,#91110,#91111);
#81574=AXIS2_PLACEMENT_3D('',#188121,#91112,#91113);
#81575=AXIS2_PLACEMENT_3D('',#188122,#91114,#91115);
#81576=AXIS2_PLACEMENT_3D('',#188123,#91116,#91117);
#81577=AXIS2_PLACEMENT_3D('',#188124,#91118,#91119);
#81578=AXIS2_PLACEMENT_3D('',#188125,#91120,#91121);
#81579=AXIS2_PLACEMENT_3D('',#188130,#91123,#91124);
#81580=AXIS2_PLACEMENT_3D('',#188133,#91126,#91127);
#81581=AXIS2_PLACEMENT_3D('',#188134,#91128,#91129);
#81582=AXIS2_PLACEMENT_3D('',#188138,#91131,#91132);
#81583=AXIS2_PLACEMENT_3D('',#188139,#91133,#91134);
#81584=AXIS2_PLACEMENT_3D('',#188140,#91135,#91136);
#81585=AXIS2_PLACEMENT_3D('',#188144,#91138,#91139);
#81586=AXIS2_PLACEMENT_3D('',#188145,#91140,#91141);
#81587=AXIS2_PLACEMENT_3D('',#188146,#91142,#91143);
#81588=AXIS2_PLACEMENT_3D('',#188147,#91144,#91145);
#81589=AXIS2_PLACEMENT_3D('',#188148,#91146,#91147);
#81590=AXIS2_PLACEMENT_3D('',#188149,#91148,#91149);
#81591=AXIS2_PLACEMENT_3D('',#188154,#91151,#91152);
#81592=AXIS2_PLACEMENT_3D('',#188157,#91154,#91155);
#81593=AXIS2_PLACEMENT_3D('',#188158,#91156,#91157);
#81594=AXIS2_PLACEMENT_3D('',#188162,#91159,#91160);
#81595=AXIS2_PLACEMENT_3D('',#188163,#91161,#91162);
#81596=AXIS2_PLACEMENT_3D('',#188164,#91163,#91164);
#81597=AXIS2_PLACEMENT_3D('',#188168,#91166,#91167);
#81598=AXIS2_PLACEMENT_3D('',#188169,#91168,#91169);
#81599=AXIS2_PLACEMENT_3D('',#188170,#91170,#91171);
#81600=AXIS2_PLACEMENT_3D('',#188171,#91172,#91173);
#81601=AXIS2_PLACEMENT_3D('',#188172,#91174,#91175);
#81602=AXIS2_PLACEMENT_3D('',#188173,#91176,#91177);
#81603=AXIS2_PLACEMENT_3D('',#188178,#91179,#91180);
#81604=AXIS2_PLACEMENT_3D('',#188181,#91182,#91183);
#81605=AXIS2_PLACEMENT_3D('',#188182,#91184,#91185);
#81606=AXIS2_PLACEMENT_3D('',#188186,#91187,#91188);
#81607=AXIS2_PLACEMENT_3D('',#188187,#91189,#91190);
#81608=AXIS2_PLACEMENT_3D('',#188188,#91191,#91192);
#81609=AXIS2_PLACEMENT_3D('',#188192,#91194,#91195);
#81610=AXIS2_PLACEMENT_3D('',#188193,#91196,#91197);
#81611=AXIS2_PLACEMENT_3D('',#188194,#91198,#91199);
#81612=AXIS2_PLACEMENT_3D('',#188195,#91200,#91201);
#81613=AXIS2_PLACEMENT_3D('',#188196,#91202,#91203);
#81614=AXIS2_PLACEMENT_3D('',#188197,#91204,#91205);
#81615=AXIS2_PLACEMENT_3D('',#188202,#91207,#91208);
#81616=AXIS2_PLACEMENT_3D('',#188205,#91210,#91211);
#81617=AXIS2_PLACEMENT_3D('',#188206,#91212,#91213);
#81618=AXIS2_PLACEMENT_3D('',#188210,#91215,#91216);
#81619=AXIS2_PLACEMENT_3D('',#188211,#91217,#91218);
#81620=AXIS2_PLACEMENT_3D('',#188212,#91219,#91220);
#81621=AXIS2_PLACEMENT_3D('',#188216,#91222,#91223);
#81622=AXIS2_PLACEMENT_3D('',#188217,#91224,#91225);
#81623=AXIS2_PLACEMENT_3D('',#188218,#91226,#91227);
#81624=AXIS2_PLACEMENT_3D('',#188219,#91228,#91229);
#81625=AXIS2_PLACEMENT_3D('',#188220,#91230,#91231);
#81626=AXIS2_PLACEMENT_3D('',#188221,#91232,#91233);
#81627=AXIS2_PLACEMENT_3D('',#188227,#91236,#91237);
#81628=AXIS2_PLACEMENT_3D('',#188228,#91238,#91239);
#81629=AXIS2_PLACEMENT_3D('',#188233,#91241,#91242);
#81630=AXIS2_PLACEMENT_3D('',#188236,#91244,#91245);
#81631=AXIS2_PLACEMENT_3D('',#188237,#91246,#91247);
#81632=AXIS2_PLACEMENT_3D('',#188241,#91249,#91250);
#81633=AXIS2_PLACEMENT_3D('',#188242,#91251,#91252);
#81634=AXIS2_PLACEMENT_3D('',#188243,#91253,#91254);
#81635=AXIS2_PLACEMENT_3D('',#188246,#91256,#91257);
#81636=AXIS2_PLACEMENT_3D('',#188247,#91258,#91259);
#81637=AXIS2_PLACEMENT_3D('',#188248,#91260,#91261);
#81638=AXIS2_PLACEMENT_3D('',#188249,#91262,#91263);
#81639=AXIS2_PLACEMENT_3D('',#188250,#91264,#91265);
#81640=AXIS2_PLACEMENT_3D('',#188251,#91266,#91267);
#81641=AXIS2_PLACEMENT_3D('',#188256,#91269,#91270);
#81642=AXIS2_PLACEMENT_3D('',#188259,#91272,#91273);
#81643=AXIS2_PLACEMENT_3D('',#188260,#91274,#91275);
#81644=AXIS2_PLACEMENT_3D('',#188264,#91277,#91278);
#81645=AXIS2_PLACEMENT_3D('',#188265,#91279,#91280);
#81646=AXIS2_PLACEMENT_3D('',#188266,#91281,#91282);
#81647=AXIS2_PLACEMENT_3D('',#188270,#91284,#91285);
#81648=AXIS2_PLACEMENT_3D('',#188271,#91286,#91287);
#81649=AXIS2_PLACEMENT_3D('',#188272,#91288,#91289);
#81650=AXIS2_PLACEMENT_3D('',#188273,#91290,#91291);
#81651=AXIS2_PLACEMENT_3D('',#188274,#91292,#91293);
#81652=AXIS2_PLACEMENT_3D('',#188275,#91294,#91295);
#81653=AXIS2_PLACEMENT_3D('',#188280,#91297,#91298);
#81654=AXIS2_PLACEMENT_3D('',#188283,#91300,#91301);
#81655=AXIS2_PLACEMENT_3D('',#188284,#91302,#91303);
#81656=AXIS2_PLACEMENT_3D('',#188288,#91305,#91306);
#81657=AXIS2_PLACEMENT_3D('',#188289,#91307,#91308);
#81658=AXIS2_PLACEMENT_3D('',#188290,#91309,#91310);
#81659=AXIS2_PLACEMENT_3D('',#188294,#91312,#91313);
#81660=AXIS2_PLACEMENT_3D('',#188295,#91314,#91315);
#81661=AXIS2_PLACEMENT_3D('',#188296,#91316,#91317);
#81662=AXIS2_PLACEMENT_3D('',#188297,#91318,#91319);
#81663=AXIS2_PLACEMENT_3D('',#188298,#91320,#91321);
#81664=AXIS2_PLACEMENT_3D('',#188299,#91322,#91323);
#81665=AXIS2_PLACEMENT_3D('',#188304,#91325,#91326);
#81666=AXIS2_PLACEMENT_3D('',#188307,#91328,#91329);
#81667=AXIS2_PLACEMENT_3D('',#188308,#91330,#91331);
#81668=AXIS2_PLACEMENT_3D('',#188312,#91333,#91334);
#81669=AXIS2_PLACEMENT_3D('',#188313,#91335,#91336);
#81670=AXIS2_PLACEMENT_3D('',#188314,#91337,#91338);
#81671=AXIS2_PLACEMENT_3D('',#188318,#91340,#91341);
#81672=AXIS2_PLACEMENT_3D('',#188319,#91342,#91343);
#81673=AXIS2_PLACEMENT_3D('',#188320,#91344,#91345);
#81674=AXIS2_PLACEMENT_3D('',#188321,#91346,#91347);
#81675=AXIS2_PLACEMENT_3D('',#188322,#91348,#91349);
#81676=AXIS2_PLACEMENT_3D('',#188323,#91350,#91351);
#81677=AXIS2_PLACEMENT_3D('',#188328,#91353,#91354);
#81678=AXIS2_PLACEMENT_3D('',#188331,#91356,#91357);
#81679=AXIS2_PLACEMENT_3D('',#188332,#91358,#91359);
#81680=AXIS2_PLACEMENT_3D('',#188336,#91361,#91362);
#81681=AXIS2_PLACEMENT_3D('',#188337,#91363,#91364);
#81682=AXIS2_PLACEMENT_3D('',#188338,#91365,#91366);
#81683=AXIS2_PLACEMENT_3D('',#188342,#91368,#91369);
#81684=AXIS2_PLACEMENT_3D('',#188343,#91370,#91371);
#81685=AXIS2_PLACEMENT_3D('',#188344,#91372,#91373);
#81686=AXIS2_PLACEMENT_3D('',#188345,#91374,#91375);
#81687=AXIS2_PLACEMENT_3D('',#188346,#91376,#91377);
#81688=AXIS2_PLACEMENT_3D('',#188347,#91378,#91379);
#81689=AXIS2_PLACEMENT_3D('',#188352,#91381,#91382);
#81690=AXIS2_PLACEMENT_3D('',#188355,#91384,#91385);
#81691=AXIS2_PLACEMENT_3D('',#188356,#91386,#91387);
#81692=AXIS2_PLACEMENT_3D('',#188360,#91389,#91390);
#81693=AXIS2_PLACEMENT_3D('',#188361,#91391,#91392);
#81694=AXIS2_PLACEMENT_3D('',#188362,#91393,#91394);
#81695=AXIS2_PLACEMENT_3D('',#188366,#91396,#91397);
#81696=AXIS2_PLACEMENT_3D('',#188367,#91398,#91399);
#81697=AXIS2_PLACEMENT_3D('',#188368,#91400,#91401);
#81698=AXIS2_PLACEMENT_3D('',#188369,#91402,#91403);
#81699=AXIS2_PLACEMENT_3D('',#188370,#91404,#91405);
#81700=AXIS2_PLACEMENT_3D('',#188371,#91406,#91407);
#81701=AXIS2_PLACEMENT_3D('',#188376,#91409,#91410);
#81702=AXIS2_PLACEMENT_3D('',#188379,#91412,#91413);
#81703=AXIS2_PLACEMENT_3D('',#188380,#91414,#91415);
#81704=AXIS2_PLACEMENT_3D('',#188384,#91417,#91418);
#81705=AXIS2_PLACEMENT_3D('',#188385,#91419,#91420);
#81706=AXIS2_PLACEMENT_3D('',#188386,#91421,#91422);
#81707=AXIS2_PLACEMENT_3D('',#188390,#91424,#91425);
#81708=AXIS2_PLACEMENT_3D('',#188391,#91426,#91427);
#81709=AXIS2_PLACEMENT_3D('',#188392,#91428,#91429);
#81710=AXIS2_PLACEMENT_3D('',#188393,#91430,#91431);
#81711=AXIS2_PLACEMENT_3D('',#188394,#91432,#91433);
#81712=AXIS2_PLACEMENT_3D('',#188395,#91434,#91435);
#81713=AXIS2_PLACEMENT_3D('',#188400,#91437,#91438);
#81714=AXIS2_PLACEMENT_3D('',#188403,#91440,#91441);
#81715=AXIS2_PLACEMENT_3D('',#188404,#91442,#91443);
#81716=AXIS2_PLACEMENT_3D('',#188408,#91445,#91446);
#81717=AXIS2_PLACEMENT_3D('',#188409,#91447,#91448);
#81718=AXIS2_PLACEMENT_3D('',#188410,#91449,#91450);
#81719=AXIS2_PLACEMENT_3D('',#188414,#91452,#91453);
#81720=AXIS2_PLACEMENT_3D('',#188415,#91454,#91455);
#81721=AXIS2_PLACEMENT_3D('',#188416,#91456,#91457);
#81722=AXIS2_PLACEMENT_3D('',#188417,#91458,#91459);
#81723=AXIS2_PLACEMENT_3D('',#188418,#91460,#91461);
#81724=AXIS2_PLACEMENT_3D('',#188419,#91462,#91463);
#81725=AXIS2_PLACEMENT_3D('',#188424,#91465,#91466);
#81726=AXIS2_PLACEMENT_3D('',#188427,#91468,#91469);
#81727=AXIS2_PLACEMENT_3D('',#188428,#91470,#91471);
#81728=AXIS2_PLACEMENT_3D('',#188432,#91473,#91474);
#81729=AXIS2_PLACEMENT_3D('',#188433,#91475,#91476);
#81730=AXIS2_PLACEMENT_3D('',#188434,#91477,#91478);
#81731=AXIS2_PLACEMENT_3D('',#188438,#91480,#91481);
#81732=AXIS2_PLACEMENT_3D('',#188439,#91482,#91483);
#81733=AXIS2_PLACEMENT_3D('',#188440,#91484,#91485);
#81734=AXIS2_PLACEMENT_3D('',#188441,#91486,#91487);
#81735=AXIS2_PLACEMENT_3D('',#188442,#91488,#91489);
#81736=AXIS2_PLACEMENT_3D('',#188443,#91490,#91491);
#81737=AXIS2_PLACEMENT_3D('',#188448,#91493,#91494);
#81738=AXIS2_PLACEMENT_3D('',#188451,#91496,#91497);
#81739=AXIS2_PLACEMENT_3D('',#188452,#91498,#91499);
#81740=AXIS2_PLACEMENT_3D('',#188456,#91501,#91502);
#81741=AXIS2_PLACEMENT_3D('',#188457,#91503,#91504);
#81742=AXIS2_PLACEMENT_3D('',#188458,#91505,#91506);
#81743=AXIS2_PLACEMENT_3D('',#188462,#91508,#91509);
#81744=AXIS2_PLACEMENT_3D('',#188463,#91510,#91511);
#81745=AXIS2_PLACEMENT_3D('',#188464,#91512,#91513);
#81746=AXIS2_PLACEMENT_3D('',#188465,#91514,#91515);
#81747=AXIS2_PLACEMENT_3D('',#188466,#91516,#91517);
#81748=AXIS2_PLACEMENT_3D('',#188467,#91518,#91519);
#81749=AXIS2_PLACEMENT_3D('',#188472,#91521,#91522);
#81750=AXIS2_PLACEMENT_3D('',#188475,#91524,#91525);
#81751=AXIS2_PLACEMENT_3D('',#188476,#91526,#91527);
#81752=AXIS2_PLACEMENT_3D('',#188480,#91529,#91530);
#81753=AXIS2_PLACEMENT_3D('',#188481,#91531,#91532);
#81754=AXIS2_PLACEMENT_3D('',#188482,#91533,#91534);
#81755=AXIS2_PLACEMENT_3D('',#188486,#91536,#91537);
#81756=AXIS2_PLACEMENT_3D('',#188487,#91538,#91539);
#81757=AXIS2_PLACEMENT_3D('',#188488,#91540,#91541);
#81758=AXIS2_PLACEMENT_3D('',#188489,#91542,#91543);
#81759=AXIS2_PLACEMENT_3D('',#188490,#91544,#91545);
#81760=AXIS2_PLACEMENT_3D('',#188491,#91546,#91547);
#81761=AXIS2_PLACEMENT_3D('',#188496,#91549,#91550);
#81762=AXIS2_PLACEMENT_3D('',#188499,#91552,#91553);
#81763=AXIS2_PLACEMENT_3D('',#188500,#91554,#91555);
#81764=AXIS2_PLACEMENT_3D('',#188504,#91557,#91558);
#81765=AXIS2_PLACEMENT_3D('',#188505,#91559,#91560);
#81766=AXIS2_PLACEMENT_3D('',#188506,#91561,#91562);
#81767=AXIS2_PLACEMENT_3D('',#188512,#91565,#91566);
#81768=AXIS2_PLACEMENT_3D('',#188513,#91567,#91568);
#81769=AXIS2_PLACEMENT_3D('',#188514,#91569,#91570);
#81770=AXIS2_PLACEMENT_3D('',#188516,#91571,#91572);
#81771=AXIS2_PLACEMENT_3D('',#188518,#91574,#91575);
#81772=AXIS2_PLACEMENT_3D('',#188519,#91576,#91577);
#81773=AXIS2_PLACEMENT_3D('',#188520,#91578,#91579);
#81774=AXIS2_PLACEMENT_3D('',#188521,#91580,#91581);
#81775=AXIS2_PLACEMENT_3D('',#188526,#91583,#91584);
#81776=AXIS2_PLACEMENT_3D('',#188529,#91586,#91587);
#81777=AXIS2_PLACEMENT_3D('',#188530,#91588,#91589);
#81778=AXIS2_PLACEMENT_3D('',#188534,#91591,#91592);
#81779=AXIS2_PLACEMENT_3D('',#188535,#91593,#91594);
#81780=AXIS2_PLACEMENT_3D('',#188536,#91595,#91596);
#81781=AXIS2_PLACEMENT_3D('',#188542,#91599,#91600);
#81782=AXIS2_PLACEMENT_3D('',#188543,#91601,#91602);
#81783=AXIS2_PLACEMENT_3D('',#188544,#91603,#91604);
#81784=AXIS2_PLACEMENT_3D('',#188546,#91605,#91606);
#81785=AXIS2_PLACEMENT_3D('',#188548,#91608,#91609);
#81786=AXIS2_PLACEMENT_3D('',#188549,#91610,#91611);
#81787=AXIS2_PLACEMENT_3D('',#188550,#91612,#91613);
#81788=AXIS2_PLACEMENT_3D('',#188551,#91614,#91615);
#81789=AXIS2_PLACEMENT_3D('',#188556,#91617,#91618);
#81790=AXIS2_PLACEMENT_3D('',#188559,#91620,#91621);
#81791=AXIS2_PLACEMENT_3D('',#188560,#91622,#91623);
#81792=AXIS2_PLACEMENT_3D('',#188564,#91625,#91626);
#81793=AXIS2_PLACEMENT_3D('',#188565,#91627,#91628);
#81794=AXIS2_PLACEMENT_3D('',#188566,#91629,#91630);
#81795=AXIS2_PLACEMENT_3D('',#188570,#91632,#91633);
#81796=AXIS2_PLACEMENT_3D('',#188571,#91634,#91635);
#81797=AXIS2_PLACEMENT_3D('',#188572,#91636,#91637);
#81798=AXIS2_PLACEMENT_3D('',#188573,#91638,#91639);
#81799=AXIS2_PLACEMENT_3D('',#188574,#91640,#91641);
#81800=AXIS2_PLACEMENT_3D('',#188575,#91642,#91643);
#81801=AXIS2_PLACEMENT_3D('',#188580,#91645,#91646);
#81802=AXIS2_PLACEMENT_3D('',#188583,#91648,#91649);
#81803=AXIS2_PLACEMENT_3D('',#188584,#91650,#91651);
#81804=AXIS2_PLACEMENT_3D('',#188588,#91653,#91654);
#81805=AXIS2_PLACEMENT_3D('',#188589,#91655,#91656);
#81806=AXIS2_PLACEMENT_3D('',#188590,#91657,#91658);
#81807=AXIS2_PLACEMENT_3D('',#188594,#91660,#91661);
#81808=AXIS2_PLACEMENT_3D('',#188595,#91662,#91663);
#81809=AXIS2_PLACEMENT_3D('',#188596,#91664,#91665);
#81810=AXIS2_PLACEMENT_3D('',#188597,#91666,#91667);
#81811=AXIS2_PLACEMENT_3D('',#188598,#91668,#91669);
#81812=AXIS2_PLACEMENT_3D('',#188599,#91670,#91671);
#81813=AXIS2_PLACEMENT_3D('',#188604,#91673,#91674);
#81814=AXIS2_PLACEMENT_3D('',#188607,#91676,#91677);
#81815=AXIS2_PLACEMENT_3D('',#188608,#91678,#91679);
#81816=AXIS2_PLACEMENT_3D('',#188612,#91681,#91682);
#81817=AXIS2_PLACEMENT_3D('',#188613,#91683,#91684);
#81818=AXIS2_PLACEMENT_3D('',#188614,#91685,#91686);
#81819=AXIS2_PLACEMENT_3D('',#188618,#91688,#91689);
#81820=AXIS2_PLACEMENT_3D('',#188619,#91690,#91691);
#81821=AXIS2_PLACEMENT_3D('',#188620,#91692,#91693);
#81822=AXIS2_PLACEMENT_3D('',#188621,#91694,#91695);
#81823=AXIS2_PLACEMENT_3D('',#188622,#91696,#91697);
#81824=AXIS2_PLACEMENT_3D('',#188623,#91698,#91699);
#81825=AXIS2_PLACEMENT_3D('',#188628,#91701,#91702);
#81826=AXIS2_PLACEMENT_3D('',#188631,#91704,#91705);
#81827=AXIS2_PLACEMENT_3D('',#188632,#91706,#91707);
#81828=AXIS2_PLACEMENT_3D('',#188636,#91709,#91710);
#81829=AXIS2_PLACEMENT_3D('',#188637,#91711,#91712);
#81830=AXIS2_PLACEMENT_3D('',#188638,#91713,#91714);
#81831=AXIS2_PLACEMENT_3D('',#188642,#91716,#91717);
#81832=AXIS2_PLACEMENT_3D('',#188643,#91718,#91719);
#81833=AXIS2_PLACEMENT_3D('',#188644,#91720,#91721);
#81834=AXIS2_PLACEMENT_3D('',#188645,#91722,#91723);
#81835=AXIS2_PLACEMENT_3D('',#188646,#91724,#91725);
#81836=AXIS2_PLACEMENT_3D('',#188647,#91726,#91727);
#81837=AXIS2_PLACEMENT_3D('',#188652,#91729,#91730);
#81838=AXIS2_PLACEMENT_3D('',#188655,#91732,#91733);
#81839=AXIS2_PLACEMENT_3D('',#188656,#91734,#91735);
#81840=AXIS2_PLACEMENT_3D('',#188660,#91737,#91738);
#81841=AXIS2_PLACEMENT_3D('',#188661,#91739,#91740);
#81842=AXIS2_PLACEMENT_3D('',#188662,#91741,#91742);
#81843=AXIS2_PLACEMENT_3D('',#188666,#91744,#91745);
#81844=AXIS2_PLACEMENT_3D('',#188667,#91746,#91747);
#81845=AXIS2_PLACEMENT_3D('',#188668,#91748,#91749);
#81846=AXIS2_PLACEMENT_3D('',#188669,#91750,#91751);
#81847=AXIS2_PLACEMENT_3D('',#188670,#91752,#91753);
#81848=AXIS2_PLACEMENT_3D('',#188671,#91754,#91755);
#81849=AXIS2_PLACEMENT_3D('',#188676,#91757,#91758);
#81850=AXIS2_PLACEMENT_3D('',#188679,#91760,#91761);
#81851=AXIS2_PLACEMENT_3D('',#188680,#91762,#91763);
#81852=AXIS2_PLACEMENT_3D('',#188684,#91765,#91766);
#81853=AXIS2_PLACEMENT_3D('',#188685,#91767,#91768);
#81854=AXIS2_PLACEMENT_3D('',#188686,#91769,#91770);
#81855=AXIS2_PLACEMENT_3D('',#188690,#91772,#91773);
#81856=AXIS2_PLACEMENT_3D('',#188691,#91774,#91775);
#81857=AXIS2_PLACEMENT_3D('',#188692,#91776,#91777);
#81858=AXIS2_PLACEMENT_3D('',#188693,#91778,#91779);
#81859=AXIS2_PLACEMENT_3D('',#188694,#91780,#91781);
#81860=AXIS2_PLACEMENT_3D('',#188695,#91782,#91783);
#81861=AXIS2_PLACEMENT_3D('',#188700,#91785,#91786);
#81862=AXIS2_PLACEMENT_3D('',#188703,#91788,#91789);
#81863=AXIS2_PLACEMENT_3D('',#188704,#91790,#91791);
#81864=AXIS2_PLACEMENT_3D('',#188708,#91793,#91794);
#81865=AXIS2_PLACEMENT_3D('',#188709,#91795,#91796);
#81866=AXIS2_PLACEMENT_3D('',#188710,#91797,#91798);
#81867=AXIS2_PLACEMENT_3D('',#188714,#91800,#91801);
#81868=AXIS2_PLACEMENT_3D('',#188715,#91802,#91803);
#81869=AXIS2_PLACEMENT_3D('',#188716,#91804,#91805);
#81870=AXIS2_PLACEMENT_3D('',#188717,#91806,#91807);
#81871=AXIS2_PLACEMENT_3D('',#188718,#91808,#91809);
#81872=AXIS2_PLACEMENT_3D('',#188719,#91810,#91811);
#81873=AXIS2_PLACEMENT_3D('',#188724,#91813,#91814);
#81874=AXIS2_PLACEMENT_3D('',#188727,#91816,#91817);
#81875=AXIS2_PLACEMENT_3D('',#188728,#91818,#91819);
#81876=AXIS2_PLACEMENT_3D('',#188732,#91821,#91822);
#81877=AXIS2_PLACEMENT_3D('',#188733,#91823,#91824);
#81878=AXIS2_PLACEMENT_3D('',#188734,#91825,#91826);
#81879=AXIS2_PLACEMENT_3D('',#188738,#91828,#91829);
#81880=AXIS2_PLACEMENT_3D('',#188739,#91830,#91831);
#81881=AXIS2_PLACEMENT_3D('',#188740,#91832,#91833);
#81882=AXIS2_PLACEMENT_3D('',#188741,#91834,#91835);
#81883=AXIS2_PLACEMENT_3D('',#188742,#91836,#91837);
#81884=AXIS2_PLACEMENT_3D('',#188743,#91838,#91839);
#81885=AXIS2_PLACEMENT_3D('',#188748,#91841,#91842);
#81886=AXIS2_PLACEMENT_3D('',#188751,#91844,#91845);
#81887=AXIS2_PLACEMENT_3D('',#188752,#91846,#91847);
#81888=AXIS2_PLACEMENT_3D('',#188756,#91849,#91850);
#81889=AXIS2_PLACEMENT_3D('',#188757,#91851,#91852);
#81890=AXIS2_PLACEMENT_3D('',#188758,#91853,#91854);
#81891=AXIS2_PLACEMENT_3D('',#188762,#91856,#91857);
#81892=AXIS2_PLACEMENT_3D('',#188763,#91858,#91859);
#81893=AXIS2_PLACEMENT_3D('',#188764,#91860,#91861);
#81894=AXIS2_PLACEMENT_3D('',#188765,#91862,#91863);
#81895=AXIS2_PLACEMENT_3D('',#188766,#91864,#91865);
#81896=AXIS2_PLACEMENT_3D('',#188767,#91866,#91867);
#81897=AXIS2_PLACEMENT_3D('',#188772,#91869,#91870);
#81898=AXIS2_PLACEMENT_3D('',#188775,#91872,#91873);
#81899=AXIS2_PLACEMENT_3D('',#188776,#91874,#91875);
#81900=AXIS2_PLACEMENT_3D('',#188780,#91877,#91878);
#81901=AXIS2_PLACEMENT_3D('',#188781,#91879,#91880);
#81902=AXIS2_PLACEMENT_3D('',#188782,#91881,#91882);
#81903=AXIS2_PLACEMENT_3D('',#188786,#91884,#91885);
#81904=AXIS2_PLACEMENT_3D('',#188787,#91886,#91887);
#81905=AXIS2_PLACEMENT_3D('',#188788,#91888,#91889);
#81906=AXIS2_PLACEMENT_3D('',#188789,#91890,#91891);
#81907=AXIS2_PLACEMENT_3D('',#188790,#91892,#91893);
#81908=AXIS2_PLACEMENT_3D('',#188791,#91894,#91895);
#81909=AXIS2_PLACEMENT_3D('',#188796,#91897,#91898);
#81910=AXIS2_PLACEMENT_3D('',#188799,#91900,#91901);
#81911=AXIS2_PLACEMENT_3D('',#188800,#91902,#91903);
#81912=AXIS2_PLACEMENT_3D('',#188804,#91905,#91906);
#81913=AXIS2_PLACEMENT_3D('',#188805,#91907,#91908);
#81914=AXIS2_PLACEMENT_3D('',#188806,#91909,#91910);
#81915=AXIS2_PLACEMENT_3D('',#188810,#91912,#91913);
#81916=AXIS2_PLACEMENT_3D('',#188811,#91914,#91915);
#81917=AXIS2_PLACEMENT_3D('',#188812,#91916,#91917);
#81918=AXIS2_PLACEMENT_3D('',#188813,#91918,#91919);
#81919=AXIS2_PLACEMENT_3D('',#188814,#91920,#91921);
#81920=AXIS2_PLACEMENT_3D('',#188815,#91922,#91923);
#81921=AXIS2_PLACEMENT_3D('',#188820,#91925,#91926);
#81922=AXIS2_PLACEMENT_3D('',#188823,#91928,#91929);
#81923=AXIS2_PLACEMENT_3D('',#188824,#91930,#91931);
#81924=AXIS2_PLACEMENT_3D('',#188828,#91933,#91934);
#81925=AXIS2_PLACEMENT_3D('',#188829,#91935,#91936);
#81926=AXIS2_PLACEMENT_3D('',#188830,#91937,#91938);
#81927=AXIS2_PLACEMENT_3D('',#188834,#91940,#91941);
#81928=AXIS2_PLACEMENT_3D('',#188835,#91942,#91943);
#81929=AXIS2_PLACEMENT_3D('',#188836,#91944,#91945);
#81930=AXIS2_PLACEMENT_3D('',#188837,#91946,#91947);
#81931=AXIS2_PLACEMENT_3D('',#188838,#91948,#91949);
#81932=AXIS2_PLACEMENT_3D('',#188839,#91950,#91951);
#81933=AXIS2_PLACEMENT_3D('',#188844,#91953,#91954);
#81934=AXIS2_PLACEMENT_3D('',#188847,#91956,#91957);
#81935=AXIS2_PLACEMENT_3D('',#188848,#91958,#91959);
#81936=AXIS2_PLACEMENT_3D('',#188852,#91961,#91962);
#81937=AXIS2_PLACEMENT_3D('',#188853,#91963,#91964);
#81938=AXIS2_PLACEMENT_3D('',#188854,#91965,#91966);
#81939=AXIS2_PLACEMENT_3D('',#188858,#91968,#91969);
#81940=AXIS2_PLACEMENT_3D('',#188859,#91970,#91971);
#81941=AXIS2_PLACEMENT_3D('',#188860,#91972,#91973);
#81942=AXIS2_PLACEMENT_3D('',#188861,#91974,#91975);
#81943=AXIS2_PLACEMENT_3D('',#188862,#91976,#91977);
#81944=AXIS2_PLACEMENT_3D('',#188863,#91978,#91979);
#81945=AXIS2_PLACEMENT_3D('',#188868,#91981,#91982);
#81946=AXIS2_PLACEMENT_3D('',#188871,#91984,#91985);
#81947=AXIS2_PLACEMENT_3D('',#188872,#91986,#91987);
#81948=AXIS2_PLACEMENT_3D('',#188876,#91989,#91990);
#81949=AXIS2_PLACEMENT_3D('',#188877,#91991,#91992);
#81950=AXIS2_PLACEMENT_3D('',#188878,#91993,#91994);
#81951=AXIS2_PLACEMENT_3D('',#188882,#91996,#91997);
#81952=AXIS2_PLACEMENT_3D('',#188883,#91998,#91999);
#81953=AXIS2_PLACEMENT_3D('',#188884,#92000,#92001);
#81954=AXIS2_PLACEMENT_3D('',#188885,#92002,#92003);
#81955=AXIS2_PLACEMENT_3D('',#188886,#92004,#92005);
#81956=AXIS2_PLACEMENT_3D('',#188887,#92006,#92007);
#81957=AXIS2_PLACEMENT_3D('',#188892,#92009,#92010);
#81958=AXIS2_PLACEMENT_3D('',#188895,#92012,#92013);
#81959=AXIS2_PLACEMENT_3D('',#188896,#92014,#92015);
#81960=AXIS2_PLACEMENT_3D('',#188900,#92017,#92018);
#81961=AXIS2_PLACEMENT_3D('',#188901,#92019,#92020);
#81962=AXIS2_PLACEMENT_3D('',#188902,#92021,#92022);
#81963=AXIS2_PLACEMENT_3D('',#188906,#92024,#92025);
#81964=AXIS2_PLACEMENT_3D('',#188907,#92026,#92027);
#81965=AXIS2_PLACEMENT_3D('',#188908,#92028,#92029);
#81966=AXIS2_PLACEMENT_3D('',#188909,#92030,#92031);
#81967=AXIS2_PLACEMENT_3D('',#188910,#92032,#92033);
#81968=AXIS2_PLACEMENT_3D('',#188911,#92034,#92035);
#81969=AXIS2_PLACEMENT_3D('',#188916,#92037,#92038);
#81970=AXIS2_PLACEMENT_3D('',#188919,#92040,#92041);
#81971=AXIS2_PLACEMENT_3D('',#188920,#92042,#92043);
#81972=AXIS2_PLACEMENT_3D('',#188924,#92045,#92046);
#81973=AXIS2_PLACEMENT_3D('',#188925,#92047,#92048);
#81974=AXIS2_PLACEMENT_3D('',#188926,#92049,#92050);
#81975=AXIS2_PLACEMENT_3D('',#188930,#92052,#92053);
#81976=AXIS2_PLACEMENT_3D('',#188931,#92054,#92055);
#81977=AXIS2_PLACEMENT_3D('',#188932,#92056,#92057);
#81978=AXIS2_PLACEMENT_3D('',#188933,#92058,#92059);
#81979=AXIS2_PLACEMENT_3D('',#188934,#92060,#92061);
#81980=AXIS2_PLACEMENT_3D('',#188935,#92062,#92063);
#81981=AXIS2_PLACEMENT_3D('',#188940,#92065,#92066);
#81982=AXIS2_PLACEMENT_3D('',#188943,#92068,#92069);
#81983=AXIS2_PLACEMENT_3D('',#188944,#92070,#92071);
#81984=AXIS2_PLACEMENT_3D('',#188948,#92073,#92074);
#81985=AXIS2_PLACEMENT_3D('',#188949,#92075,#92076);
#81986=AXIS2_PLACEMENT_3D('',#188950,#92077,#92078);
#81987=AXIS2_PLACEMENT_3D('',#188954,#92080,#92081);
#81988=AXIS2_PLACEMENT_3D('',#188955,#92082,#92083);
#81989=AXIS2_PLACEMENT_3D('',#188956,#92084,#92085);
#81990=AXIS2_PLACEMENT_3D('',#188957,#92086,#92087);
#81991=AXIS2_PLACEMENT_3D('',#188958,#92088,#92089);
#81992=AXIS2_PLACEMENT_3D('',#188959,#92090,#92091);
#81993=AXIS2_PLACEMENT_3D('',#188964,#92093,#92094);
#81994=AXIS2_PLACEMENT_3D('',#188967,#92096,#92097);
#81995=AXIS2_PLACEMENT_3D('',#188968,#92098,#92099);
#81996=AXIS2_PLACEMENT_3D('',#188972,#92101,#92102);
#81997=AXIS2_PLACEMENT_3D('',#188973,#92103,#92104);
#81998=AXIS2_PLACEMENT_3D('',#188974,#92105,#92106);
#81999=AXIS2_PLACEMENT_3D('',#188978,#92108,#92109);
#82000=AXIS2_PLACEMENT_3D('',#188979,#92110,#92111);
#82001=AXIS2_PLACEMENT_3D('',#188980,#92112,#92113);
#82002=AXIS2_PLACEMENT_3D('',#188981,#92114,#92115);
#82003=AXIS2_PLACEMENT_3D('',#188982,#92116,#92117);
#82004=AXIS2_PLACEMENT_3D('',#188983,#92118,#92119);
#82005=AXIS2_PLACEMENT_3D('',#188988,#92121,#92122);
#82006=AXIS2_PLACEMENT_3D('',#188991,#92124,#92125);
#82007=AXIS2_PLACEMENT_3D('',#188992,#92126,#92127);
#82008=AXIS2_PLACEMENT_3D('',#188996,#92129,#92130);
#82009=AXIS2_PLACEMENT_3D('',#188997,#92131,#92132);
#82010=AXIS2_PLACEMENT_3D('',#188998,#92133,#92134);
#82011=AXIS2_PLACEMENT_3D('',#189002,#92136,#92137);
#82012=AXIS2_PLACEMENT_3D('',#189003,#92138,#92139);
#82013=AXIS2_PLACEMENT_3D('',#189004,#92140,#92141);
#82014=AXIS2_PLACEMENT_3D('',#189005,#92142,#92143);
#82015=AXIS2_PLACEMENT_3D('',#189006,#92144,#92145);
#82016=AXIS2_PLACEMENT_3D('',#189007,#92146,#92147);
#82017=AXIS2_PLACEMENT_3D('',#189012,#92149,#92150);
#82018=AXIS2_PLACEMENT_3D('',#189015,#92152,#92153);
#82019=AXIS2_PLACEMENT_3D('',#189016,#92154,#92155);
#82020=AXIS2_PLACEMENT_3D('',#189020,#92157,#92158);
#82021=AXIS2_PLACEMENT_3D('',#189021,#92159,#92160);
#82022=AXIS2_PLACEMENT_3D('',#189022,#92161,#92162);
#82023=AXIS2_PLACEMENT_3D('',#189026,#92164,#92165);
#82024=AXIS2_PLACEMENT_3D('',#189027,#92166,#92167);
#82025=AXIS2_PLACEMENT_3D('',#189028,#92168,#92169);
#82026=AXIS2_PLACEMENT_3D('',#189029,#92170,#92171);
#82027=AXIS2_PLACEMENT_3D('',#189030,#92172,#92173);
#82028=AXIS2_PLACEMENT_3D('',#189031,#92174,#92175);
#82029=AXIS2_PLACEMENT_3D('',#189036,#92177,#92178);
#82030=AXIS2_PLACEMENT_3D('',#189039,#92180,#92181);
#82031=AXIS2_PLACEMENT_3D('',#189040,#92182,#92183);
#82032=AXIS2_PLACEMENT_3D('',#189044,#92185,#92186);
#82033=AXIS2_PLACEMENT_3D('',#189045,#92187,#92188);
#82034=AXIS2_PLACEMENT_3D('',#189046,#92189,#92190);
#82035=AXIS2_PLACEMENT_3D('',#189050,#92192,#92193);
#82036=AXIS2_PLACEMENT_3D('',#189051,#92194,#92195);
#82037=AXIS2_PLACEMENT_3D('',#189052,#92196,#92197);
#82038=AXIS2_PLACEMENT_3D('',#189053,#92198,#92199);
#82039=AXIS2_PLACEMENT_3D('',#189054,#92200,#92201);
#82040=AXIS2_PLACEMENT_3D('',#189055,#92202,#92203);
#82041=AXIS2_PLACEMENT_3D('',#189060,#92205,#92206);
#82042=AXIS2_PLACEMENT_3D('',#189063,#92208,#92209);
#82043=AXIS2_PLACEMENT_3D('',#189064,#92210,#92211);
#82044=AXIS2_PLACEMENT_3D('',#189068,#92213,#92214);
#82045=AXIS2_PLACEMENT_3D('',#189069,#92215,#92216);
#82046=AXIS2_PLACEMENT_3D('',#189070,#92217,#92218);
#82047=AXIS2_PLACEMENT_3D('',#189074,#92220,#92221);
#82048=AXIS2_PLACEMENT_3D('',#189075,#92222,#92223);
#82049=AXIS2_PLACEMENT_3D('',#189076,#92224,#92225);
#82050=AXIS2_PLACEMENT_3D('',#189077,#92226,#92227);
#82051=AXIS2_PLACEMENT_3D('',#189078,#92228,#92229);
#82052=AXIS2_PLACEMENT_3D('',#189079,#92230,#92231);
#82053=AXIS2_PLACEMENT_3D('',#189084,#92233,#92234);
#82054=AXIS2_PLACEMENT_3D('',#189087,#92236,#92237);
#82055=AXIS2_PLACEMENT_3D('',#189088,#92238,#92239);
#82056=AXIS2_PLACEMENT_3D('',#189092,#92241,#92242);
#82057=AXIS2_PLACEMENT_3D('',#189093,#92243,#92244);
#82058=AXIS2_PLACEMENT_3D('',#189094,#92245,#92246);
#82059=AXIS2_PLACEMENT_3D('',#189098,#92248,#92249);
#82060=AXIS2_PLACEMENT_3D('',#189099,#92250,#92251);
#82061=AXIS2_PLACEMENT_3D('',#189100,#92252,#92253);
#82062=AXIS2_PLACEMENT_3D('',#189101,#92254,#92255);
#82063=AXIS2_PLACEMENT_3D('',#189102,#92256,#92257);
#82064=AXIS2_PLACEMENT_3D('',#189103,#92258,#92259);
#82065=AXIS2_PLACEMENT_3D('',#189108,#92261,#92262);
#82066=AXIS2_PLACEMENT_3D('',#189111,#92264,#92265);
#82067=AXIS2_PLACEMENT_3D('',#189112,#92266,#92267);
#82068=AXIS2_PLACEMENT_3D('',#189116,#92269,#92270);
#82069=AXIS2_PLACEMENT_3D('',#189117,#92271,#92272);
#82070=AXIS2_PLACEMENT_3D('',#189118,#92273,#92274);
#82071=AXIS2_PLACEMENT_3D('',#189122,#92276,#92277);
#82072=AXIS2_PLACEMENT_3D('',#189123,#92278,#92279);
#82073=AXIS2_PLACEMENT_3D('',#189124,#92280,#92281);
#82074=AXIS2_PLACEMENT_3D('',#189125,#92282,#92283);
#82075=AXIS2_PLACEMENT_3D('',#189126,#92284,#92285);
#82076=AXIS2_PLACEMENT_3D('',#189127,#92286,#92287);
#82077=AXIS2_PLACEMENT_3D('',#189132,#92289,#92290);
#82078=AXIS2_PLACEMENT_3D('',#189135,#92292,#92293);
#82079=AXIS2_PLACEMENT_3D('',#189136,#92294,#92295);
#82080=AXIS2_PLACEMENT_3D('',#189140,#92297,#92298);
#82081=AXIS2_PLACEMENT_3D('',#189141,#92299,#92300);
#82082=AXIS2_PLACEMENT_3D('',#189142,#92301,#92302);
#82083=AXIS2_PLACEMENT_3D('',#189146,#92304,#92305);
#82084=AXIS2_PLACEMENT_3D('',#189147,#92306,#92307);
#82085=AXIS2_PLACEMENT_3D('',#189148,#92308,#92309);
#82086=AXIS2_PLACEMENT_3D('',#189149,#92310,#92311);
#82087=AXIS2_PLACEMENT_3D('',#189150,#92312,#92313);
#82088=AXIS2_PLACEMENT_3D('',#189151,#92314,#92315);
#82089=AXIS2_PLACEMENT_3D('',#189156,#92317,#92318);
#82090=AXIS2_PLACEMENT_3D('',#189159,#92320,#92321);
#82091=AXIS2_PLACEMENT_3D('',#189160,#92322,#92323);
#82092=AXIS2_PLACEMENT_3D('',#189164,#92325,#92326);
#82093=AXIS2_PLACEMENT_3D('',#189165,#92327,#92328);
#82094=AXIS2_PLACEMENT_3D('',#189166,#92329,#92330);
#82095=AXIS2_PLACEMENT_3D('',#189170,#92332,#92333);
#82096=AXIS2_PLACEMENT_3D('',#189171,#92334,#92335);
#82097=AXIS2_PLACEMENT_3D('',#189172,#92336,#92337);
#82098=AXIS2_PLACEMENT_3D('',#189173,#92338,#92339);
#82099=AXIS2_PLACEMENT_3D('',#189174,#92340,#92341);
#82100=AXIS2_PLACEMENT_3D('',#189175,#92342,#92343);
#82101=AXIS2_PLACEMENT_3D('',#189180,#92345,#92346);
#82102=AXIS2_PLACEMENT_3D('',#189183,#92348,#92349);
#82103=AXIS2_PLACEMENT_3D('',#189184,#92350,#92351);
#82104=AXIS2_PLACEMENT_3D('',#189188,#92353,#92354);
#82105=AXIS2_PLACEMENT_3D('',#189189,#92355,#92356);
#82106=AXIS2_PLACEMENT_3D('',#189190,#92357,#92358);
#82107=AXIS2_PLACEMENT_3D('',#189194,#92360,#92361);
#82108=AXIS2_PLACEMENT_3D('',#189195,#92362,#92363);
#82109=AXIS2_PLACEMENT_3D('',#189196,#92364,#92365);
#82110=AXIS2_PLACEMENT_3D('',#189197,#92366,#92367);
#82111=AXIS2_PLACEMENT_3D('',#189198,#92368,#92369);
#82112=AXIS2_PLACEMENT_3D('',#189199,#92370,#92371);
#82113=AXIS2_PLACEMENT_3D('',#189204,#92373,#92374);
#82114=AXIS2_PLACEMENT_3D('',#189207,#92376,#92377);
#82115=AXIS2_PLACEMENT_3D('',#189208,#92378,#92379);
#82116=AXIS2_PLACEMENT_3D('',#189212,#92381,#92382);
#82117=AXIS2_PLACEMENT_3D('',#189213,#92383,#92384);
#82118=AXIS2_PLACEMENT_3D('',#189214,#92385,#92386);
#82119=AXIS2_PLACEMENT_3D('',#189218,#92388,#92389);
#82120=AXIS2_PLACEMENT_3D('',#189219,#92390,#92391);
#82121=AXIS2_PLACEMENT_3D('',#189220,#92392,#92393);
#82122=AXIS2_PLACEMENT_3D('',#189221,#92394,#92395);
#82123=AXIS2_PLACEMENT_3D('',#189222,#92396,#92397);
#82124=AXIS2_PLACEMENT_3D('',#189223,#92398,#92399);
#82125=AXIS2_PLACEMENT_3D('',#189228,#92401,#92402);
#82126=AXIS2_PLACEMENT_3D('',#189231,#92404,#92405);
#82127=AXIS2_PLACEMENT_3D('',#189232,#92406,#92407);
#82128=AXIS2_PLACEMENT_3D('',#189236,#92409,#92410);
#82129=AXIS2_PLACEMENT_3D('',#189237,#92411,#92412);
#82130=AXIS2_PLACEMENT_3D('',#189238,#92413,#92414);
#82131=AXIS2_PLACEMENT_3D('',#189242,#92416,#92417);
#82132=AXIS2_PLACEMENT_3D('',#189243,#92418,#92419);
#82133=AXIS2_PLACEMENT_3D('',#189244,#92420,#92421);
#82134=AXIS2_PLACEMENT_3D('',#189245,#92422,#92423);
#82135=AXIS2_PLACEMENT_3D('',#189246,#92424,#92425);
#82136=AXIS2_PLACEMENT_3D('',#189247,#92426,#92427);
#82137=AXIS2_PLACEMENT_3D('',#189252,#92429,#92430);
#82138=AXIS2_PLACEMENT_3D('',#189255,#92432,#92433);
#82139=AXIS2_PLACEMENT_3D('',#189256,#92434,#92435);
#82140=AXIS2_PLACEMENT_3D('',#189260,#92437,#92438);
#82141=AXIS2_PLACEMENT_3D('',#189261,#92439,#92440);
#82142=AXIS2_PLACEMENT_3D('',#189262,#92441,#92442);
#82143=AXIS2_PLACEMENT_3D('',#189266,#92444,#92445);
#82144=AXIS2_PLACEMENT_3D('',#189267,#92446,#92447);
#82145=AXIS2_PLACEMENT_3D('',#189268,#92448,#92449);
#82146=AXIS2_PLACEMENT_3D('',#189269,#92450,#92451);
#82147=AXIS2_PLACEMENT_3D('',#189270,#92452,#92453);
#82148=AXIS2_PLACEMENT_3D('',#189271,#92454,#92455);
#82149=AXIS2_PLACEMENT_3D('',#189276,#92457,#92458);
#82150=AXIS2_PLACEMENT_3D('',#189279,#92460,#92461);
#82151=AXIS2_PLACEMENT_3D('',#189280,#92462,#92463);
#82152=AXIS2_PLACEMENT_3D('',#189284,#92465,#92466);
#82153=AXIS2_PLACEMENT_3D('',#189285,#92467,#92468);
#82154=AXIS2_PLACEMENT_3D('',#189286,#92469,#92470);
#82155=AXIS2_PLACEMENT_3D('',#189290,#92472,#92473);
#82156=AXIS2_PLACEMENT_3D('',#189291,#92474,#92475);
#82157=AXIS2_PLACEMENT_3D('',#189292,#92476,#92477);
#82158=AXIS2_PLACEMENT_3D('',#189293,#92478,#92479);
#82159=AXIS2_PLACEMENT_3D('',#189294,#92480,#92481);
#82160=AXIS2_PLACEMENT_3D('',#189295,#92482,#92483);
#82161=AXIS2_PLACEMENT_3D('',#189300,#92485,#92486);
#82162=AXIS2_PLACEMENT_3D('',#189303,#92488,#92489);
#82163=AXIS2_PLACEMENT_3D('',#189304,#92490,#92491);
#82164=AXIS2_PLACEMENT_3D('',#189308,#92493,#92494);
#82165=AXIS2_PLACEMENT_3D('',#189309,#92495,#92496);
#82166=AXIS2_PLACEMENT_3D('',#189310,#92497,#92498);
#82167=AXIS2_PLACEMENT_3D('',#189314,#92500,#92501);
#82168=AXIS2_PLACEMENT_3D('',#189315,#92502,#92503);
#82169=AXIS2_PLACEMENT_3D('',#189316,#92504,#92505);
#82170=AXIS2_PLACEMENT_3D('',#189317,#92506,#92507);
#82171=AXIS2_PLACEMENT_3D('',#189318,#92508,#92509);
#82172=AXIS2_PLACEMENT_3D('',#189319,#92510,#92511);
#82173=AXIS2_PLACEMENT_3D('',#189324,#92513,#92514);
#82174=AXIS2_PLACEMENT_3D('',#189327,#92516,#92517);
#82175=AXIS2_PLACEMENT_3D('',#189328,#92518,#92519);
#82176=AXIS2_PLACEMENT_3D('',#189332,#92521,#92522);
#82177=AXIS2_PLACEMENT_3D('',#189333,#92523,#92524);
#82178=AXIS2_PLACEMENT_3D('',#189334,#92525,#92526);
#82179=AXIS2_PLACEMENT_3D('',#189338,#92528,#92529);
#82180=AXIS2_PLACEMENT_3D('',#189339,#92530,#92531);
#82181=AXIS2_PLACEMENT_3D('',#189340,#92532,#92533);
#82182=AXIS2_PLACEMENT_3D('',#189341,#92534,#92535);
#82183=AXIS2_PLACEMENT_3D('',#189342,#92536,#92537);
#82184=AXIS2_PLACEMENT_3D('',#189343,#92538,#92539);
#82185=AXIS2_PLACEMENT_3D('',#189348,#92541,#92542);
#82186=AXIS2_PLACEMENT_3D('',#189351,#92544,#92545);
#82187=AXIS2_PLACEMENT_3D('',#189352,#92546,#92547);
#82188=AXIS2_PLACEMENT_3D('',#189356,#92549,#92550);
#82189=AXIS2_PLACEMENT_3D('',#189357,#92551,#92552);
#82190=AXIS2_PLACEMENT_3D('',#189358,#92553,#92554);
#82191=AXIS2_PLACEMENT_3D('',#189362,#92556,#92557);
#82192=AXIS2_PLACEMENT_3D('',#189363,#92558,#92559);
#82193=AXIS2_PLACEMENT_3D('',#189364,#92560,#92561);
#82194=AXIS2_PLACEMENT_3D('',#189365,#92562,#92563);
#82195=AXIS2_PLACEMENT_3D('',#189366,#92564,#92565);
#82196=AXIS2_PLACEMENT_3D('',#189367,#92566,#92567);
#82197=AXIS2_PLACEMENT_3D('',#189372,#92569,#92570);
#82198=AXIS2_PLACEMENT_3D('',#189375,#92572,#92573);
#82199=AXIS2_PLACEMENT_3D('',#189376,#92574,#92575);
#82200=AXIS2_PLACEMENT_3D('',#189380,#92577,#92578);
#82201=AXIS2_PLACEMENT_3D('',#189381,#92579,#92580);
#82202=AXIS2_PLACEMENT_3D('',#189382,#92581,#92582);
#82203=AXIS2_PLACEMENT_3D('',#189386,#92584,#92585);
#82204=AXIS2_PLACEMENT_3D('',#189387,#92586,#92587);
#82205=AXIS2_PLACEMENT_3D('',#189388,#92588,#92589);
#82206=AXIS2_PLACEMENT_3D('',#189389,#92590,#92591);
#82207=AXIS2_PLACEMENT_3D('',#189390,#92592,#92593);
#82208=AXIS2_PLACEMENT_3D('',#189391,#92594,#92595);
#82209=AXIS2_PLACEMENT_3D('',#189396,#92597,#92598);
#82210=AXIS2_PLACEMENT_3D('',#189399,#92600,#92601);
#82211=AXIS2_PLACEMENT_3D('',#189400,#92602,#92603);
#82212=AXIS2_PLACEMENT_3D('',#189404,#92605,#92606);
#82213=AXIS2_PLACEMENT_3D('',#189405,#92607,#92608);
#82214=AXIS2_PLACEMENT_3D('',#189406,#92609,#92610);
#82215=AXIS2_PLACEMENT_3D('',#189410,#92612,#92613);
#82216=AXIS2_PLACEMENT_3D('',#189411,#92614,#92615);
#82217=AXIS2_PLACEMENT_3D('',#189412,#92616,#92617);
#82218=AXIS2_PLACEMENT_3D('',#189413,#92618,#92619);
#82219=AXIS2_PLACEMENT_3D('',#189414,#92620,#92621);
#82220=AXIS2_PLACEMENT_3D('',#189415,#92622,#92623);
#82221=AXIS2_PLACEMENT_3D('',#189420,#92625,#92626);
#82222=AXIS2_PLACEMENT_3D('',#189423,#92628,#92629);
#82223=AXIS2_PLACEMENT_3D('',#189424,#92630,#92631);
#82224=AXIS2_PLACEMENT_3D('',#189428,#92633,#92634);
#82225=AXIS2_PLACEMENT_3D('',#189429,#92635,#92636);
#82226=AXIS2_PLACEMENT_3D('',#189430,#92637,#92638);
#82227=AXIS2_PLACEMENT_3D('',#189434,#92640,#92641);
#82228=AXIS2_PLACEMENT_3D('',#189435,#92642,#92643);
#82229=AXIS2_PLACEMENT_3D('',#189436,#92644,#92645);
#82230=AXIS2_PLACEMENT_3D('',#189437,#92646,#92647);
#82231=AXIS2_PLACEMENT_3D('',#189438,#92648,#92649);
#82232=AXIS2_PLACEMENT_3D('',#189439,#92650,#92651);
#82233=AXIS2_PLACEMENT_3D('',#189444,#92653,#92654);
#82234=AXIS2_PLACEMENT_3D('',#189447,#92656,#92657);
#82235=AXIS2_PLACEMENT_3D('',#189448,#92658,#92659);
#82236=AXIS2_PLACEMENT_3D('',#189452,#92661,#92662);
#82237=AXIS2_PLACEMENT_3D('',#189453,#92663,#92664);
#82238=AXIS2_PLACEMENT_3D('',#189454,#92665,#92666);
#82239=AXIS2_PLACEMENT_3D('',#189458,#92668,#92669);
#82240=AXIS2_PLACEMENT_3D('',#189459,#92670,#92671);
#82241=AXIS2_PLACEMENT_3D('',#189460,#92672,#92673);
#82242=AXIS2_PLACEMENT_3D('',#189461,#92674,#92675);
#82243=AXIS2_PLACEMENT_3D('',#189462,#92676,#92677);
#82244=AXIS2_PLACEMENT_3D('',#189463,#92678,#92679);
#82245=AXIS2_PLACEMENT_3D('',#189468,#92681,#92682);
#82246=AXIS2_PLACEMENT_3D('',#189471,#92684,#92685);
#82247=AXIS2_PLACEMENT_3D('',#189472,#92686,#92687);
#82248=AXIS2_PLACEMENT_3D('',#189476,#92689,#92690);
#82249=AXIS2_PLACEMENT_3D('',#189477,#92691,#92692);
#82250=AXIS2_PLACEMENT_3D('',#189478,#92693,#92694);
#82251=AXIS2_PLACEMENT_3D('',#189482,#92696,#92697);
#82252=AXIS2_PLACEMENT_3D('',#189483,#92698,#92699);
#82253=AXIS2_PLACEMENT_3D('',#189484,#92700,#92701);
#82254=AXIS2_PLACEMENT_3D('',#189485,#92702,#92703);
#82255=AXIS2_PLACEMENT_3D('',#189486,#92704,#92705);
#82256=AXIS2_PLACEMENT_3D('',#189487,#92706,#92707);
#82257=AXIS2_PLACEMENT_3D('',#189492,#92709,#92710);
#82258=AXIS2_PLACEMENT_3D('',#189495,#92712,#92713);
#82259=AXIS2_PLACEMENT_3D('',#189496,#92714,#92715);
#82260=AXIS2_PLACEMENT_3D('',#189500,#92717,#92718);
#82261=AXIS2_PLACEMENT_3D('',#189501,#92719,#92720);
#82262=AXIS2_PLACEMENT_3D('',#189502,#92721,#92722);
#82263=AXIS2_PLACEMENT_3D('',#189506,#92724,#92725);
#82264=AXIS2_PLACEMENT_3D('',#189507,#92726,#92727);
#82265=AXIS2_PLACEMENT_3D('',#189508,#92728,#92729);
#82266=AXIS2_PLACEMENT_3D('',#189509,#92730,#92731);
#82267=AXIS2_PLACEMENT_3D('',#189510,#92732,#92733);
#82268=AXIS2_PLACEMENT_3D('',#189511,#92734,#92735);
#82269=AXIS2_PLACEMENT_3D('',#189516,#92737,#92738);
#82270=AXIS2_PLACEMENT_3D('',#189519,#92740,#92741);
#82271=AXIS2_PLACEMENT_3D('',#189520,#92742,#92743);
#82272=AXIS2_PLACEMENT_3D('',#189524,#92745,#92746);
#82273=AXIS2_PLACEMENT_3D('',#189525,#92747,#92748);
#82274=AXIS2_PLACEMENT_3D('',#189526,#92749,#92750);
#82275=AXIS2_PLACEMENT_3D('',#189530,#92752,#92753);
#82276=AXIS2_PLACEMENT_3D('',#189531,#92754,#92755);
#82277=AXIS2_PLACEMENT_3D('',#189532,#92756,#92757);
#82278=AXIS2_PLACEMENT_3D('',#189533,#92758,#92759);
#82279=AXIS2_PLACEMENT_3D('',#189534,#92760,#92761);
#82280=AXIS2_PLACEMENT_3D('',#189535,#92762,#92763);
#82281=AXIS2_PLACEMENT_3D('',#189540,#92765,#92766);
#82282=AXIS2_PLACEMENT_3D('',#189543,#92768,#92769);
#82283=AXIS2_PLACEMENT_3D('',#189544,#92770,#92771);
#82284=AXIS2_PLACEMENT_3D('',#189548,#92773,#92774);
#82285=AXIS2_PLACEMENT_3D('',#189549,#92775,#92776);
#82286=AXIS2_PLACEMENT_3D('',#189550,#92777,#92778);
#82287=AXIS2_PLACEMENT_3D('',#189554,#92780,#92781);
#82288=AXIS2_PLACEMENT_3D('',#189555,#92782,#92783);
#82289=AXIS2_PLACEMENT_3D('',#189556,#92784,#92785);
#82290=AXIS2_PLACEMENT_3D('',#189557,#92786,#92787);
#82291=AXIS2_PLACEMENT_3D('',#189558,#92788,#92789);
#82292=AXIS2_PLACEMENT_3D('',#189559,#92790,#92791);
#82293=AXIS2_PLACEMENT_3D('',#189564,#92793,#92794);
#82294=AXIS2_PLACEMENT_3D('',#189567,#92796,#92797);
#82295=AXIS2_PLACEMENT_3D('',#189568,#92798,#92799);
#82296=AXIS2_PLACEMENT_3D('',#189572,#92801,#92802);
#82297=AXIS2_PLACEMENT_3D('',#189573,#92803,#92804);
#82298=AXIS2_PLACEMENT_3D('',#189574,#92805,#92806);
#82299=AXIS2_PLACEMENT_3D('',#189578,#92808,#92809);
#82300=AXIS2_PLACEMENT_3D('',#189579,#92810,#92811);
#82301=AXIS2_PLACEMENT_3D('',#189580,#92812,#92813);
#82302=AXIS2_PLACEMENT_3D('',#189581,#92814,#92815);
#82303=AXIS2_PLACEMENT_3D('',#189582,#92816,#92817);
#82304=AXIS2_PLACEMENT_3D('',#189583,#92818,#92819);
#82305=AXIS2_PLACEMENT_3D('',#189588,#92821,#92822);
#82306=AXIS2_PLACEMENT_3D('',#189591,#92824,#92825);
#82307=AXIS2_PLACEMENT_3D('',#189592,#92826,#92827);
#82308=AXIS2_PLACEMENT_3D('',#189596,#92829,#92830);
#82309=AXIS2_PLACEMENT_3D('',#189597,#92831,#92832);
#82310=AXIS2_PLACEMENT_3D('',#189598,#92833,#92834);
#82311=AXIS2_PLACEMENT_3D('',#189602,#92836,#92837);
#82312=AXIS2_PLACEMENT_3D('',#189603,#92838,#92839);
#82313=AXIS2_PLACEMENT_3D('',#189604,#92840,#92841);
#82314=AXIS2_PLACEMENT_3D('',#189605,#92842,#92843);
#82315=AXIS2_PLACEMENT_3D('',#189606,#92844,#92845);
#82316=AXIS2_PLACEMENT_3D('',#189607,#92846,#92847);
#82317=AXIS2_PLACEMENT_3D('',#189612,#92849,#92850);
#82318=AXIS2_PLACEMENT_3D('',#189615,#92852,#92853);
#82319=AXIS2_PLACEMENT_3D('',#189616,#92854,#92855);
#82320=AXIS2_PLACEMENT_3D('',#189620,#92857,#92858);
#82321=AXIS2_PLACEMENT_3D('',#189621,#92859,#92860);
#82322=AXIS2_PLACEMENT_3D('',#189622,#92861,#92862);
#82323=AXIS2_PLACEMENT_3D('',#189626,#92864,#92865);
#82324=AXIS2_PLACEMENT_3D('',#189627,#92866,#92867);
#82325=AXIS2_PLACEMENT_3D('',#189628,#92868,#92869);
#82326=AXIS2_PLACEMENT_3D('',#189629,#92870,#92871);
#82327=AXIS2_PLACEMENT_3D('',#189630,#92872,#92873);
#82328=AXIS2_PLACEMENT_3D('',#189631,#92874,#92875);
#82329=AXIS2_PLACEMENT_3D('',#189636,#92877,#92878);
#82330=AXIS2_PLACEMENT_3D('',#189639,#92880,#92881);
#82331=AXIS2_PLACEMENT_3D('',#189640,#92882,#92883);
#82332=AXIS2_PLACEMENT_3D('',#189644,#92885,#92886);
#82333=AXIS2_PLACEMENT_3D('',#189645,#92887,#92888);
#82334=AXIS2_PLACEMENT_3D('',#189646,#92889,#92890);
#82335=AXIS2_PLACEMENT_3D('',#189650,#92892,#92893);
#82336=AXIS2_PLACEMENT_3D('',#189651,#92894,#92895);
#82337=AXIS2_PLACEMENT_3D('',#189652,#92896,#92897);
#82338=AXIS2_PLACEMENT_3D('',#189653,#92898,#92899);
#82339=AXIS2_PLACEMENT_3D('',#189654,#92900,#92901);
#82340=AXIS2_PLACEMENT_3D('',#189655,#92902,#92903);
#82341=AXIS2_PLACEMENT_3D('',#189660,#92905,#92906);
#82342=AXIS2_PLACEMENT_3D('',#189663,#92908,#92909);
#82343=AXIS2_PLACEMENT_3D('',#189664,#92910,#92911);
#82344=AXIS2_PLACEMENT_3D('',#189668,#92913,#92914);
#82345=AXIS2_PLACEMENT_3D('',#189669,#92915,#92916);
#82346=AXIS2_PLACEMENT_3D('',#189670,#92917,#92918);
#82347=AXIS2_PLACEMENT_3D('',#189674,#92920,#92921);
#82348=AXIS2_PLACEMENT_3D('',#189675,#92922,#92923);
#82349=AXIS2_PLACEMENT_3D('',#189676,#92924,#92925);
#82350=AXIS2_PLACEMENT_3D('',#189677,#92926,#92927);
#82351=AXIS2_PLACEMENT_3D('',#189678,#92928,#92929);
#82352=AXIS2_PLACEMENT_3D('',#189679,#92930,#92931);
#82353=AXIS2_PLACEMENT_3D('',#189684,#92933,#92934);
#82354=AXIS2_PLACEMENT_3D('',#189687,#92936,#92937);
#82355=AXIS2_PLACEMENT_3D('',#189688,#92938,#92939);
#82356=AXIS2_PLACEMENT_3D('',#189692,#92941,#92942);
#82357=AXIS2_PLACEMENT_3D('',#189693,#92943,#92944);
#82358=AXIS2_PLACEMENT_3D('',#189694,#92945,#92946);
#82359=AXIS2_PLACEMENT_3D('',#189698,#92948,#92949);
#82360=AXIS2_PLACEMENT_3D('',#189699,#92950,#92951);
#82361=AXIS2_PLACEMENT_3D('',#189700,#92952,#92953);
#82362=AXIS2_PLACEMENT_3D('',#189701,#92954,#92955);
#82363=AXIS2_PLACEMENT_3D('',#189702,#92956,#92957);
#82364=AXIS2_PLACEMENT_3D('',#189703,#92958,#92959);
#82365=AXIS2_PLACEMENT_3D('',#189708,#92961,#92962);
#82366=AXIS2_PLACEMENT_3D('',#189711,#92964,#92965);
#82367=AXIS2_PLACEMENT_3D('',#189712,#92966,#92967);
#82368=AXIS2_PLACEMENT_3D('',#189716,#92969,#92970);
#82369=AXIS2_PLACEMENT_3D('',#189717,#92971,#92972);
#82370=AXIS2_PLACEMENT_3D('',#189718,#92973,#92974);
#82371=AXIS2_PLACEMENT_3D('',#189722,#92976,#92977);
#82372=AXIS2_PLACEMENT_3D('',#189723,#92978,#92979);
#82373=AXIS2_PLACEMENT_3D('',#189724,#92980,#92981);
#82374=AXIS2_PLACEMENT_3D('',#189725,#92982,#92983);
#82375=AXIS2_PLACEMENT_3D('',#189726,#92984,#92985);
#82376=AXIS2_PLACEMENT_3D('',#189727,#92986,#92987);
#82377=AXIS2_PLACEMENT_3D('',#189732,#92989,#92990);
#82378=AXIS2_PLACEMENT_3D('',#189735,#92992,#92993);
#82379=AXIS2_PLACEMENT_3D('',#189736,#92994,#92995);
#82380=AXIS2_PLACEMENT_3D('',#189740,#92997,#92998);
#82381=AXIS2_PLACEMENT_3D('',#189741,#92999,#93000);
#82382=AXIS2_PLACEMENT_3D('',#189742,#93001,#93002);
#82383=AXIS2_PLACEMENT_3D('',#189746,#93004,#93005);
#82384=AXIS2_PLACEMENT_3D('',#189747,#93006,#93007);
#82385=AXIS2_PLACEMENT_3D('',#189748,#93008,#93009);
#82386=AXIS2_PLACEMENT_3D('',#189749,#93010,#93011);
#82387=AXIS2_PLACEMENT_3D('',#189750,#93012,#93013);
#82388=AXIS2_PLACEMENT_3D('',#189751,#93014,#93015);
#82389=AXIS2_PLACEMENT_3D('',#189756,#93017,#93018);
#82390=AXIS2_PLACEMENT_3D('',#189759,#93020,#93021);
#82391=AXIS2_PLACEMENT_3D('',#189760,#93022,#93023);
#82392=AXIS2_PLACEMENT_3D('',#189764,#93025,#93026);
#82393=AXIS2_PLACEMENT_3D('',#189765,#93027,#93028);
#82394=AXIS2_PLACEMENT_3D('',#189766,#93029,#93030);
#82395=AXIS2_PLACEMENT_3D('',#189770,#93032,#93033);
#82396=AXIS2_PLACEMENT_3D('',#189771,#93034,#93035);
#82397=AXIS2_PLACEMENT_3D('',#189772,#93036,#93037);
#82398=AXIS2_PLACEMENT_3D('',#189773,#93038,#93039);
#82399=AXIS2_PLACEMENT_3D('',#189774,#93040,#93041);
#82400=AXIS2_PLACEMENT_3D('',#189775,#93042,#93043);
#82401=AXIS2_PLACEMENT_3D('',#189780,#93045,#93046);
#82402=AXIS2_PLACEMENT_3D('',#189783,#93048,#93049);
#82403=AXIS2_PLACEMENT_3D('',#189784,#93050,#93051);
#82404=AXIS2_PLACEMENT_3D('',#189788,#93053,#93054);
#82405=AXIS2_PLACEMENT_3D('',#189789,#93055,#93056);
#82406=AXIS2_PLACEMENT_3D('',#189790,#93057,#93058);
#82407=AXIS2_PLACEMENT_3D('',#189794,#93060,#93061);
#82408=AXIS2_PLACEMENT_3D('',#189795,#93062,#93063);
#82409=AXIS2_PLACEMENT_3D('',#189796,#93064,#93065);
#82410=AXIS2_PLACEMENT_3D('',#189797,#93066,#93067);
#82411=AXIS2_PLACEMENT_3D('',#189798,#93068,#93069);
#82412=AXIS2_PLACEMENT_3D('',#189799,#93070,#93071);
#82413=AXIS2_PLACEMENT_3D('',#189804,#93073,#93074);
#82414=AXIS2_PLACEMENT_3D('',#189807,#93076,#93077);
#82415=AXIS2_PLACEMENT_3D('',#189808,#93078,#93079);
#82416=AXIS2_PLACEMENT_3D('',#189812,#93081,#93082);
#82417=AXIS2_PLACEMENT_3D('',#189813,#93083,#93084);
#82418=AXIS2_PLACEMENT_3D('',#189814,#93085,#93086);
#82419=AXIS2_PLACEMENT_3D('',#189818,#93088,#93089);
#82420=AXIS2_PLACEMENT_3D('',#189819,#93090,#93091);
#82421=AXIS2_PLACEMENT_3D('',#189820,#93092,#93093);
#82422=AXIS2_PLACEMENT_3D('',#189821,#93094,#93095);
#82423=AXIS2_PLACEMENT_3D('',#189822,#93096,#93097);
#82424=AXIS2_PLACEMENT_3D('',#189823,#93098,#93099);
#82425=AXIS2_PLACEMENT_3D('',#189828,#93101,#93102);
#82426=AXIS2_PLACEMENT_3D('',#189831,#93104,#93105);
#82427=AXIS2_PLACEMENT_3D('',#189832,#93106,#93107);
#82428=AXIS2_PLACEMENT_3D('',#189836,#93109,#93110);
#82429=AXIS2_PLACEMENT_3D('',#189837,#93111,#93112);
#82430=AXIS2_PLACEMENT_3D('',#189838,#93113,#93114);
#82431=AXIS2_PLACEMENT_3D('',#189842,#93116,#93117);
#82432=AXIS2_PLACEMENT_3D('',#189843,#93118,#93119);
#82433=AXIS2_PLACEMENT_3D('',#189844,#93120,#93121);
#82434=AXIS2_PLACEMENT_3D('',#189845,#93122,#93123);
#82435=AXIS2_PLACEMENT_3D('',#189846,#93124,#93125);
#82436=AXIS2_PLACEMENT_3D('',#189847,#93126,#93127);
#82437=AXIS2_PLACEMENT_3D('',#189852,#93129,#93130);
#82438=AXIS2_PLACEMENT_3D('',#189855,#93132,#93133);
#82439=AXIS2_PLACEMENT_3D('',#189856,#93134,#93135);
#82440=AXIS2_PLACEMENT_3D('',#189860,#93137,#93138);
#82441=AXIS2_PLACEMENT_3D('',#189861,#93139,#93140);
#82442=AXIS2_PLACEMENT_3D('',#189862,#93141,#93142);
#82443=AXIS2_PLACEMENT_3D('',#189866,#93144,#93145);
#82444=AXIS2_PLACEMENT_3D('',#189867,#93146,#93147);
#82445=AXIS2_PLACEMENT_3D('',#189868,#93148,#93149);
#82446=AXIS2_PLACEMENT_3D('',#189869,#93150,#93151);
#82447=AXIS2_PLACEMENT_3D('',#189870,#93152,#93153);
#82448=AXIS2_PLACEMENT_3D('',#189871,#93154,#93155);
#82449=AXIS2_PLACEMENT_3D('',#189876,#93157,#93158);
#82450=AXIS2_PLACEMENT_3D('',#189879,#93160,#93161);
#82451=AXIS2_PLACEMENT_3D('',#189880,#93162,#93163);
#82452=AXIS2_PLACEMENT_3D('',#189884,#93165,#93166);
#82453=AXIS2_PLACEMENT_3D('',#189885,#93167,#93168);
#82454=AXIS2_PLACEMENT_3D('',#189886,#93169,#93170);
#82455=AXIS2_PLACEMENT_3D('',#189890,#93172,#93173);
#82456=AXIS2_PLACEMENT_3D('',#189891,#93174,#93175);
#82457=AXIS2_PLACEMENT_3D('',#189892,#93176,#93177);
#82458=AXIS2_PLACEMENT_3D('',#189893,#93178,#93179);
#82459=AXIS2_PLACEMENT_3D('',#189894,#93180,#93181);
#82460=AXIS2_PLACEMENT_3D('',#189895,#93182,#93183);
#82461=AXIS2_PLACEMENT_3D('',#189900,#93185,#93186);
#82462=AXIS2_PLACEMENT_3D('',#189903,#93188,#93189);
#82463=AXIS2_PLACEMENT_3D('',#189904,#93190,#93191);
#82464=AXIS2_PLACEMENT_3D('',#189908,#93193,#93194);
#82465=AXIS2_PLACEMENT_3D('',#189909,#93195,#93196);
#82466=AXIS2_PLACEMENT_3D('',#189910,#93197,#93198);
#82467=AXIS2_PLACEMENT_3D('',#189914,#93200,#93201);
#82468=AXIS2_PLACEMENT_3D('',#189915,#93202,#93203);
#82469=AXIS2_PLACEMENT_3D('',#189916,#93204,#93205);
#82470=AXIS2_PLACEMENT_3D('',#189917,#93206,#93207);
#82471=AXIS2_PLACEMENT_3D('',#189918,#93208,#93209);
#82472=AXIS2_PLACEMENT_3D('',#189919,#93210,#93211);
#82473=AXIS2_PLACEMENT_3D('',#189924,#93213,#93214);
#82474=AXIS2_PLACEMENT_3D('',#189927,#93216,#93217);
#82475=AXIS2_PLACEMENT_3D('',#189928,#93218,#93219);
#82476=AXIS2_PLACEMENT_3D('',#189932,#93221,#93222);
#82477=AXIS2_PLACEMENT_3D('',#189933,#93223,#93224);
#82478=AXIS2_PLACEMENT_3D('',#189934,#93225,#93226);
#82479=AXIS2_PLACEMENT_3D('',#189938,#93228,#93229);
#82480=AXIS2_PLACEMENT_3D('',#189939,#93230,#93231);
#82481=AXIS2_PLACEMENT_3D('',#189940,#93232,#93233);
#82482=AXIS2_PLACEMENT_3D('',#189941,#93234,#93235);
#82483=AXIS2_PLACEMENT_3D('',#189942,#93236,#93237);
#82484=AXIS2_PLACEMENT_3D('',#189943,#93238,#93239);
#82485=AXIS2_PLACEMENT_3D('',#189948,#93241,#93242);
#82486=AXIS2_PLACEMENT_3D('',#189951,#93244,#93245);
#82487=AXIS2_PLACEMENT_3D('',#189952,#93246,#93247);
#82488=AXIS2_PLACEMENT_3D('',#189956,#93249,#93250);
#82489=AXIS2_PLACEMENT_3D('',#189957,#93251,#93252);
#82490=AXIS2_PLACEMENT_3D('',#189958,#93253,#93254);
#82491=AXIS2_PLACEMENT_3D('',#189962,#93256,#93257);
#82492=AXIS2_PLACEMENT_3D('',#189963,#93258,#93259);
#82493=AXIS2_PLACEMENT_3D('',#189964,#93260,#93261);
#82494=AXIS2_PLACEMENT_3D('',#189965,#93262,#93263);
#82495=AXIS2_PLACEMENT_3D('',#189966,#93264,#93265);
#82496=AXIS2_PLACEMENT_3D('',#189967,#93266,#93267);
#82497=AXIS2_PLACEMENT_3D('',#189972,#93269,#93270);
#82498=AXIS2_PLACEMENT_3D('',#189975,#93272,#93273);
#82499=AXIS2_PLACEMENT_3D('',#189976,#93274,#93275);
#82500=AXIS2_PLACEMENT_3D('',#189980,#93277,#93278);
#82501=AXIS2_PLACEMENT_3D('',#189981,#93279,#93280);
#82502=AXIS2_PLACEMENT_3D('',#189982,#93281,#93282);
#82503=AXIS2_PLACEMENT_3D('',#189986,#93284,#93285);
#82504=AXIS2_PLACEMENT_3D('',#189987,#93286,#93287);
#82505=AXIS2_PLACEMENT_3D('',#189988,#93288,#93289);
#82506=AXIS2_PLACEMENT_3D('',#189989,#93290,#93291);
#82507=AXIS2_PLACEMENT_3D('',#189990,#93292,#93293);
#82508=AXIS2_PLACEMENT_3D('',#189991,#93294,#93295);
#82509=AXIS2_PLACEMENT_3D('',#189996,#93297,#93298);
#82510=AXIS2_PLACEMENT_3D('',#189999,#93300,#93301);
#82511=AXIS2_PLACEMENT_3D('',#190000,#93302,#93303);
#82512=AXIS2_PLACEMENT_3D('',#190004,#93305,#93306);
#82513=AXIS2_PLACEMENT_3D('',#190005,#93307,#93308);
#82514=AXIS2_PLACEMENT_3D('',#190006,#93309,#93310);
#82515=AXIS2_PLACEMENT_3D('',#190010,#93312,#93313);
#82516=AXIS2_PLACEMENT_3D('',#190011,#93314,#93315);
#82517=AXIS2_PLACEMENT_3D('',#190012,#93316,#93317);
#82518=AXIS2_PLACEMENT_3D('',#190013,#93318,#93319);
#82519=AXIS2_PLACEMENT_3D('',#190014,#93320,#93321);
#82520=AXIS2_PLACEMENT_3D('',#190015,#93322,#93323);
#82521=AXIS2_PLACEMENT_3D('',#190020,#93325,#93326);
#82522=AXIS2_PLACEMENT_3D('',#190023,#93328,#93329);
#82523=AXIS2_PLACEMENT_3D('',#190024,#93330,#93331);
#82524=AXIS2_PLACEMENT_3D('',#190028,#93333,#93334);
#82525=AXIS2_PLACEMENT_3D('',#190029,#93335,#93336);
#82526=AXIS2_PLACEMENT_3D('',#190030,#93337,#93338);
#82527=AXIS2_PLACEMENT_3D('',#190034,#93340,#93341);
#82528=AXIS2_PLACEMENT_3D('',#190035,#93342,#93343);
#82529=AXIS2_PLACEMENT_3D('',#190036,#93344,#93345);
#82530=AXIS2_PLACEMENT_3D('',#190037,#93346,#93347);
#82531=AXIS2_PLACEMENT_3D('',#190038,#93348,#93349);
#82532=AXIS2_PLACEMENT_3D('',#190039,#93350,#93351);
#82533=AXIS2_PLACEMENT_3D('',#190044,#93353,#93354);
#82534=AXIS2_PLACEMENT_3D('',#190047,#93356,#93357);
#82535=AXIS2_PLACEMENT_3D('',#190048,#93358,#93359);
#82536=AXIS2_PLACEMENT_3D('',#190052,#93361,#93362);
#82537=AXIS2_PLACEMENT_3D('',#190053,#93363,#93364);
#82538=AXIS2_PLACEMENT_3D('',#190054,#93365,#93366);
#82539=AXIS2_PLACEMENT_3D('',#190058,#93368,#93369);
#82540=AXIS2_PLACEMENT_3D('',#190059,#93370,#93371);
#82541=AXIS2_PLACEMENT_3D('',#190060,#93372,#93373);
#82542=AXIS2_PLACEMENT_3D('',#190061,#93374,#93375);
#82543=AXIS2_PLACEMENT_3D('',#190062,#93376,#93377);
#82544=AXIS2_PLACEMENT_3D('',#190063,#93378,#93379);
#82545=AXIS2_PLACEMENT_3D('',#190068,#93381,#93382);
#82546=AXIS2_PLACEMENT_3D('',#190071,#93384,#93385);
#82547=AXIS2_PLACEMENT_3D('',#190072,#93386,#93387);
#82548=AXIS2_PLACEMENT_3D('',#190076,#93389,#93390);
#82549=AXIS2_PLACEMENT_3D('',#190077,#93391,#93392);
#82550=AXIS2_PLACEMENT_3D('',#190078,#93393,#93394);
#82551=AXIS2_PLACEMENT_3D('',#190082,#93396,#93397);
#82552=AXIS2_PLACEMENT_3D('',#190083,#93398,#93399);
#82553=AXIS2_PLACEMENT_3D('',#190084,#93400,#93401);
#82554=AXIS2_PLACEMENT_3D('',#190085,#93402,#93403);
#82555=AXIS2_PLACEMENT_3D('',#190086,#93404,#93405);
#82556=AXIS2_PLACEMENT_3D('',#190087,#93406,#93407);
#82557=AXIS2_PLACEMENT_3D('',#190092,#93409,#93410);
#82558=AXIS2_PLACEMENT_3D('',#190095,#93412,#93413);
#82559=AXIS2_PLACEMENT_3D('',#190096,#93414,#93415);
#82560=AXIS2_PLACEMENT_3D('',#190100,#93417,#93418);
#82561=AXIS2_PLACEMENT_3D('',#190101,#93419,#93420);
#82562=AXIS2_PLACEMENT_3D('',#190102,#93421,#93422);
#82563=AXIS2_PLACEMENT_3D('',#190106,#93424,#93425);
#82564=AXIS2_PLACEMENT_3D('',#190107,#93426,#93427);
#82565=AXIS2_PLACEMENT_3D('',#190108,#93428,#93429);
#82566=AXIS2_PLACEMENT_3D('',#190109,#93430,#93431);
#82567=AXIS2_PLACEMENT_3D('',#190110,#93432,#93433);
#82568=AXIS2_PLACEMENT_3D('',#190111,#93434,#93435);
#82569=AXIS2_PLACEMENT_3D('',#190116,#93437,#93438);
#82570=AXIS2_PLACEMENT_3D('',#190119,#93440,#93441);
#82571=AXIS2_PLACEMENT_3D('',#190120,#93442,#93443);
#82572=AXIS2_PLACEMENT_3D('',#190124,#93445,#93446);
#82573=AXIS2_PLACEMENT_3D('',#190125,#93447,#93448);
#82574=AXIS2_PLACEMENT_3D('',#190126,#93449,#93450);
#82575=AXIS2_PLACEMENT_3D('',#190130,#93452,#93453);
#82576=AXIS2_PLACEMENT_3D('',#190131,#93454,#93455);
#82577=AXIS2_PLACEMENT_3D('',#190132,#93456,#93457);
#82578=AXIS2_PLACEMENT_3D('',#190133,#93458,#93459);
#82579=AXIS2_PLACEMENT_3D('',#190134,#93460,#93461);
#82580=AXIS2_PLACEMENT_3D('',#190135,#93462,#93463);
#82581=AXIS2_PLACEMENT_3D('',#190140,#93465,#93466);
#82582=AXIS2_PLACEMENT_3D('',#190143,#93468,#93469);
#82583=AXIS2_PLACEMENT_3D('',#190144,#93470,#93471);
#82584=AXIS2_PLACEMENT_3D('',#190148,#93473,#93474);
#82585=AXIS2_PLACEMENT_3D('',#190149,#93475,#93476);
#82586=AXIS2_PLACEMENT_3D('',#190150,#93477,#93478);
#82587=AXIS2_PLACEMENT_3D('',#190154,#93480,#93481);
#82588=AXIS2_PLACEMENT_3D('',#190155,#93482,#93483);
#82589=AXIS2_PLACEMENT_3D('',#190156,#93484,#93485);
#82590=AXIS2_PLACEMENT_3D('',#190157,#93486,#93487);
#82591=AXIS2_PLACEMENT_3D('',#190158,#93488,#93489);
#82592=AXIS2_PLACEMENT_3D('',#190159,#93490,#93491);
#82593=AXIS2_PLACEMENT_3D('',#190164,#93493,#93494);
#82594=AXIS2_PLACEMENT_3D('',#190167,#93496,#93497);
#82595=AXIS2_PLACEMENT_3D('',#190168,#93498,#93499);
#82596=AXIS2_PLACEMENT_3D('',#190172,#93501,#93502);
#82597=AXIS2_PLACEMENT_3D('',#190173,#93503,#93504);
#82598=AXIS2_PLACEMENT_3D('',#190174,#93505,#93506);
#82599=AXIS2_PLACEMENT_3D('',#190178,#93508,#93509);
#82600=AXIS2_PLACEMENT_3D('',#190179,#93510,#93511);
#82601=AXIS2_PLACEMENT_3D('',#190180,#93512,#93513);
#82602=AXIS2_PLACEMENT_3D('',#190181,#93514,#93515);
#82603=AXIS2_PLACEMENT_3D('',#190182,#93516,#93517);
#82604=AXIS2_PLACEMENT_3D('',#190183,#93518,#93519);
#82605=AXIS2_PLACEMENT_3D('',#190188,#93521,#93522);
#82606=AXIS2_PLACEMENT_3D('',#190191,#93524,#93525);
#82607=AXIS2_PLACEMENT_3D('',#190192,#93526,#93527);
#82608=AXIS2_PLACEMENT_3D('',#190196,#93529,#93530);
#82609=AXIS2_PLACEMENT_3D('',#190197,#93531,#93532);
#82610=AXIS2_PLACEMENT_3D('',#190198,#93533,#93534);
#82611=AXIS2_PLACEMENT_3D('',#190202,#93536,#93537);
#82612=AXIS2_PLACEMENT_3D('',#190203,#93538,#93539);
#82613=AXIS2_PLACEMENT_3D('',#190204,#93540,#93541);
#82614=AXIS2_PLACEMENT_3D('',#190205,#93542,#93543);
#82615=AXIS2_PLACEMENT_3D('',#190206,#93544,#93545);
#82616=AXIS2_PLACEMENT_3D('',#190207,#93546,#93547);
#82617=AXIS2_PLACEMENT_3D('',#190212,#93549,#93550);
#82618=AXIS2_PLACEMENT_3D('',#190215,#93552,#93553);
#82619=AXIS2_PLACEMENT_3D('',#190216,#93554,#93555);
#82620=AXIS2_PLACEMENT_3D('',#190220,#93557,#93558);
#82621=AXIS2_PLACEMENT_3D('',#190221,#93559,#93560);
#82622=AXIS2_PLACEMENT_3D('',#190222,#93561,#93562);
#82623=AXIS2_PLACEMENT_3D('',#190226,#93564,#93565);
#82624=AXIS2_PLACEMENT_3D('',#190227,#93566,#93567);
#82625=AXIS2_PLACEMENT_3D('',#190228,#93568,#93569);
#82626=AXIS2_PLACEMENT_3D('',#190229,#93570,#93571);
#82627=AXIS2_PLACEMENT_3D('',#190230,#93572,#93573);
#82628=AXIS2_PLACEMENT_3D('',#190231,#93574,#93575);
#82629=AXIS2_PLACEMENT_3D('',#190236,#93577,#93578);
#82630=AXIS2_PLACEMENT_3D('',#190239,#93580,#93581);
#82631=AXIS2_PLACEMENT_3D('',#190240,#93582,#93583);
#82632=AXIS2_PLACEMENT_3D('',#190246,#93586,#93587);
#82633=AXIS2_PLACEMENT_3D('',#190247,#93588,#93589);
#82634=AXIS2_PLACEMENT_3D('',#190248,#93590,#93591);
#82635=AXIS2_PLACEMENT_3D('',#190253,#93594,#93595);
#82636=AXIS2_PLACEMENT_3D('',#190254,#93596,#93597);
#82637=AXIS2_PLACEMENT_3D('',#190256,#93599,#93600);
#82638=AXIS2_PLACEMENT_3D('',#190257,#93601,#93602);
#82639=AXIS2_PLACEMENT_3D('',#190258,#93603,#93604);
#82640=AXIS2_PLACEMENT_3D('',#190259,#93605,#93606);
#82641=AXIS2_PLACEMENT_3D('',#190264,#93608,#93609);
#82642=AXIS2_PLACEMENT_3D('',#190267,#93611,#93612);
#82643=AXIS2_PLACEMENT_3D('',#190268,#93613,#93614);
#82644=AXIS2_PLACEMENT_3D('',#190274,#93617,#93618);
#82645=AXIS2_PLACEMENT_3D('',#190275,#93619,#93620);
#82646=AXIS2_PLACEMENT_3D('',#190276,#93621,#93622);
#82647=AXIS2_PLACEMENT_3D('',#190281,#93625,#93626);
#82648=AXIS2_PLACEMENT_3D('',#190282,#93627,#93628);
#82649=AXIS2_PLACEMENT_3D('',#190284,#93629,#93630);
#82650=AXIS2_PLACEMENT_3D('',#190286,#93632,#93633);
#82651=AXIS2_PLACEMENT_3D('',#190287,#93634,#93635);
#82652=AXIS2_PLACEMENT_3D('',#190288,#93636,#93637);
#82653=AXIS2_PLACEMENT_3D('',#190289,#93638,#93639);
#82654=AXIS2_PLACEMENT_3D('',#190294,#93641,#93642);
#82655=AXIS2_PLACEMENT_3D('',#190297,#93644,#93645);
#82656=AXIS2_PLACEMENT_3D('',#190298,#93646,#93647);
#82657=AXIS2_PLACEMENT_3D('',#190304,#93650,#93651);
#82658=AXIS2_PLACEMENT_3D('',#190305,#93652,#93653);
#82659=AXIS2_PLACEMENT_3D('',#190306,#93654,#93655);
#82660=AXIS2_PLACEMENT_3D('',#190311,#93658,#93659);
#82661=AXIS2_PLACEMENT_3D('',#190312,#93660,#93661);
#82662=AXIS2_PLACEMENT_3D('',#190314,#93662,#93663);
#82663=AXIS2_PLACEMENT_3D('',#190316,#93665,#93666);
#82664=AXIS2_PLACEMENT_3D('',#190317,#93667,#93668);
#82665=AXIS2_PLACEMENT_3D('',#190318,#93669,#93670);
#82666=AXIS2_PLACEMENT_3D('',#190319,#93671,#93672);
#82667=AXIS2_PLACEMENT_3D('',#190324,#93674,#93675);
#82668=AXIS2_PLACEMENT_3D('',#190327,#93677,#93678);
#82669=AXIS2_PLACEMENT_3D('',#190328,#93679,#93680);
#82670=AXIS2_PLACEMENT_3D('',#190334,#93683,#93684);
#82671=AXIS2_PLACEMENT_3D('',#190335,#93685,#93686);
#82672=AXIS2_PLACEMENT_3D('',#190336,#93687,#93688);
#82673=AXIS2_PLACEMENT_3D('',#190341,#93691,#93692);
#82674=AXIS2_PLACEMENT_3D('',#190342,#93693,#93694);
#82675=AXIS2_PLACEMENT_3D('',#190344,#93695,#93696);
#82676=AXIS2_PLACEMENT_3D('',#190346,#93698,#93699);
#82677=AXIS2_PLACEMENT_3D('',#190347,#93700,#93701);
#82678=AXIS2_PLACEMENT_3D('',#190348,#93702,#93703);
#82679=AXIS2_PLACEMENT_3D('',#190349,#93704,#93705);
#82680=AXIS2_PLACEMENT_3D('',#190354,#93707,#93708);
#82681=AXIS2_PLACEMENT_3D('',#190357,#93710,#93711);
#82682=AXIS2_PLACEMENT_3D('',#190358,#93712,#93713);
#82683=AXIS2_PLACEMENT_3D('',#190364,#93716,#93717);
#82684=AXIS2_PLACEMENT_3D('',#190365,#93718,#93719);
#82685=AXIS2_PLACEMENT_3D('',#190366,#93720,#93721);
#82686=AXIS2_PLACEMENT_3D('',#190371,#93724,#93725);
#82687=AXIS2_PLACEMENT_3D('',#190372,#93726,#93727);
#82688=AXIS2_PLACEMENT_3D('',#190374,#93728,#93729);
#82689=AXIS2_PLACEMENT_3D('',#190376,#93731,#93732);
#82690=AXIS2_PLACEMENT_3D('',#190377,#93733,#93734);
#82691=AXIS2_PLACEMENT_3D('',#190378,#93735,#93736);
#82692=AXIS2_PLACEMENT_3D('',#190379,#93737,#93738);
#82693=AXIS2_PLACEMENT_3D('',#190386,#93741,#93742);
#82694=AXIS2_PLACEMENT_3D('',#190389,#93744,#93745);
#82695=AXIS2_PLACEMENT_3D('',#190390,#93746,#93747);
#82696=AXIS2_PLACEMENT_3D('',#190395,#93750,#93751);
#82697=AXIS2_PLACEMENT_3D('',#190396,#93752,#93753);
#82698=AXIS2_PLACEMENT_3D('',#190401,#93756,#93757);
#82699=AXIS2_PLACEMENT_3D('',#190402,#93758,#93759);
#82700=AXIS2_PLACEMENT_3D('',#190404,#93760,#93761);
#82701=AXIS2_PLACEMENT_3D('',#190406,#93763,#93764);
#82702=AXIS2_PLACEMENT_3D('',#190407,#93765,#93766);
#82703=AXIS2_PLACEMENT_3D('',#190408,#93767,#93768);
#82704=AXIS2_PLACEMENT_3D('',#190409,#93769,#93770);
#82705=AXIS2_PLACEMENT_3D('',#190416,#93773,#93774);
#82706=AXIS2_PLACEMENT_3D('',#190419,#93776,#93777);
#82707=AXIS2_PLACEMENT_3D('',#190420,#93778,#93779);
#82708=AXIS2_PLACEMENT_3D('',#190425,#93782,#93783);
#82709=AXIS2_PLACEMENT_3D('',#190426,#93784,#93785);
#82710=AXIS2_PLACEMENT_3D('',#190431,#93788,#93789);
#82711=AXIS2_PLACEMENT_3D('',#190432,#93790,#93791);
#82712=AXIS2_PLACEMENT_3D('',#190434,#93792,#93793);
#82713=AXIS2_PLACEMENT_3D('',#190436,#93795,#93796);
#82714=AXIS2_PLACEMENT_3D('',#190437,#93797,#93798);
#82715=AXIS2_PLACEMENT_3D('',#190438,#93799,#93800);
#82716=AXIS2_PLACEMENT_3D('',#190439,#93801,#93802);
#82717=AXIS2_PLACEMENT_3D('',#190444,#93804,#93805);
#82718=AXIS2_PLACEMENT_3D('',#190447,#93807,#93808);
#82719=AXIS2_PLACEMENT_3D('',#190448,#93809,#93810);
#82720=AXIS2_PLACEMENT_3D('',#190454,#93813,#93814);
#82721=AXIS2_PLACEMENT_3D('',#190455,#93815,#93816);
#82722=AXIS2_PLACEMENT_3D('',#190456,#93817,#93818);
#82723=AXIS2_PLACEMENT_3D('',#190461,#93821,#93822);
#82724=AXIS2_PLACEMENT_3D('',#190462,#93823,#93824);
#82725=AXIS2_PLACEMENT_3D('',#190464,#93825,#93826);
#82726=AXIS2_PLACEMENT_3D('',#190466,#93828,#93829);
#82727=AXIS2_PLACEMENT_3D('',#190467,#93830,#93831);
#82728=AXIS2_PLACEMENT_3D('',#190468,#93832,#93833);
#82729=AXIS2_PLACEMENT_3D('',#190469,#93834,#93835);
#82730=AXIS2_PLACEMENT_3D('',#190474,#93837,#93838);
#82731=AXIS2_PLACEMENT_3D('',#190477,#93840,#93841);
#82732=AXIS2_PLACEMENT_3D('',#190478,#93842,#93843);
#82733=AXIS2_PLACEMENT_3D('',#190484,#93846,#93847);
#82734=AXIS2_PLACEMENT_3D('',#190485,#93848,#93849);
#82735=AXIS2_PLACEMENT_3D('',#190486,#93850,#93851);
#82736=AXIS2_PLACEMENT_3D('',#190491,#93854,#93855);
#82737=AXIS2_PLACEMENT_3D('',#190492,#93856,#93857);
#82738=AXIS2_PLACEMENT_3D('',#190494,#93858,#93859);
#82739=AXIS2_PLACEMENT_3D('',#190496,#93861,#93862);
#82740=AXIS2_PLACEMENT_3D('',#190497,#93863,#93864);
#82741=AXIS2_PLACEMENT_3D('',#190498,#93865,#93866);
#82742=AXIS2_PLACEMENT_3D('',#190499,#93867,#93868);
#82743=AXIS2_PLACEMENT_3D('',#190504,#93870,#93871);
#82744=AXIS2_PLACEMENT_3D('',#190507,#93873,#93874);
#82745=AXIS2_PLACEMENT_3D('',#190508,#93875,#93876);
#82746=AXIS2_PLACEMENT_3D('',#190514,#93879,#93880);
#82747=AXIS2_PLACEMENT_3D('',#190515,#93881,#93882);
#82748=AXIS2_PLACEMENT_3D('',#190516,#93883,#93884);
#82749=AXIS2_PLACEMENT_3D('',#190521,#93887,#93888);
#82750=AXIS2_PLACEMENT_3D('',#190522,#93889,#93890);
#82751=AXIS2_PLACEMENT_3D('',#190524,#93891,#93892);
#82752=AXIS2_PLACEMENT_3D('',#190526,#93894,#93895);
#82753=AXIS2_PLACEMENT_3D('',#190527,#93896,#93897);
#82754=AXIS2_PLACEMENT_3D('',#190528,#93898,#93899);
#82755=AXIS2_PLACEMENT_3D('',#190529,#93900,#93901);
#82756=AXIS2_PLACEMENT_3D('',#190534,#93903,#93904);
#82757=AXIS2_PLACEMENT_3D('',#190537,#93906,#93907);
#82758=AXIS2_PLACEMENT_3D('',#190538,#93908,#93909);
#82759=AXIS2_PLACEMENT_3D('',#190542,#93911,#93912);
#82760=AXIS2_PLACEMENT_3D('',#190543,#93913,#93914);
#82761=AXIS2_PLACEMENT_3D('',#190544,#93915,#93916);
#82762=AXIS2_PLACEMENT_3D('',#190548,#93918,#93919);
#82763=AXIS2_PLACEMENT_3D('',#190549,#93920,#93921);
#82764=AXIS2_PLACEMENT_3D('',#190550,#93922,#93923);
#82765=AXIS2_PLACEMENT_3D('',#190551,#93924,#93925);
#82766=AXIS2_PLACEMENT_3D('',#190552,#93926,#93927);
#82767=AXIS2_PLACEMENT_3D('',#190553,#93928,#93929);
#82768=AXIS2_PLACEMENT_3D('',#190558,#93931,#93932);
#82769=AXIS2_PLACEMENT_3D('',#190561,#93934,#93935);
#82770=AXIS2_PLACEMENT_3D('',#190562,#93936,#93937);
#82771=AXIS2_PLACEMENT_3D('',#190566,#93939,#93940);
#82772=AXIS2_PLACEMENT_3D('',#190567,#93941,#93942);
#82773=AXIS2_PLACEMENT_3D('',#190568,#93943,#93944);
#82774=AXIS2_PLACEMENT_3D('',#190572,#93946,#93947);
#82775=AXIS2_PLACEMENT_3D('',#190573,#93948,#93949);
#82776=AXIS2_PLACEMENT_3D('',#190574,#93950,#93951);
#82777=AXIS2_PLACEMENT_3D('',#190575,#93952,#93953);
#82778=AXIS2_PLACEMENT_3D('',#190576,#93954,#93955);
#82779=AXIS2_PLACEMENT_3D('',#190577,#93956,#93957);
#82780=AXIS2_PLACEMENT_3D('',#190582,#93959,#93960);
#82781=AXIS2_PLACEMENT_3D('',#190585,#93962,#93963);
#82782=AXIS2_PLACEMENT_3D('',#190586,#93964,#93965);
#82783=AXIS2_PLACEMENT_3D('',#190590,#93967,#93968);
#82784=AXIS2_PLACEMENT_3D('',#190591,#93969,#93970);
#82785=AXIS2_PLACEMENT_3D('',#190592,#93971,#93972);
#82786=AXIS2_PLACEMENT_3D('',#190596,#93974,#93975);
#82787=AXIS2_PLACEMENT_3D('',#190597,#93976,#93977);
#82788=AXIS2_PLACEMENT_3D('',#190598,#93978,#93979);
#82789=AXIS2_PLACEMENT_3D('',#190599,#93980,#93981);
#82790=AXIS2_PLACEMENT_3D('',#190600,#93982,#93983);
#82791=AXIS2_PLACEMENT_3D('',#190601,#93984,#93985);
#82792=AXIS2_PLACEMENT_3D('',#190606,#93987,#93988);
#82793=AXIS2_PLACEMENT_3D('',#190609,#93990,#93991);
#82794=AXIS2_PLACEMENT_3D('',#190610,#93992,#93993);
#82795=AXIS2_PLACEMENT_3D('',#190614,#93995,#93996);
#82796=AXIS2_PLACEMENT_3D('',#190615,#93997,#93998);
#82797=AXIS2_PLACEMENT_3D('',#190616,#93999,#94000);
#82798=AXIS2_PLACEMENT_3D('',#190620,#94002,#94003);
#82799=AXIS2_PLACEMENT_3D('',#190621,#94004,#94005);
#82800=AXIS2_PLACEMENT_3D('',#190622,#94006,#94007);
#82801=AXIS2_PLACEMENT_3D('',#190623,#94008,#94009);
#82802=AXIS2_PLACEMENT_3D('',#190624,#94010,#94011);
#82803=AXIS2_PLACEMENT_3D('',#190625,#94012,#94013);
#82804=AXIS2_PLACEMENT_3D('',#190630,#94015,#94016);
#82805=AXIS2_PLACEMENT_3D('',#190633,#94018,#94019);
#82806=AXIS2_PLACEMENT_3D('',#190634,#94020,#94021);
#82807=AXIS2_PLACEMENT_3D('',#190638,#94023,#94024);
#82808=AXIS2_PLACEMENT_3D('',#190639,#94025,#94026);
#82809=AXIS2_PLACEMENT_3D('',#190640,#94027,#94028);
#82810=AXIS2_PLACEMENT_3D('',#190644,#94030,#94031);
#82811=AXIS2_PLACEMENT_3D('',#190645,#94032,#94033);
#82812=AXIS2_PLACEMENT_3D('',#190646,#94034,#94035);
#82813=AXIS2_PLACEMENT_3D('',#190647,#94036,#94037);
#82814=AXIS2_PLACEMENT_3D('',#190648,#94038,#94039);
#82815=AXIS2_PLACEMENT_3D('',#190649,#94040,#94041);
#82816=AXIS2_PLACEMENT_3D('',#190654,#94043,#94044);
#82817=AXIS2_PLACEMENT_3D('',#190657,#94046,#94047);
#82818=AXIS2_PLACEMENT_3D('',#190658,#94048,#94049);
#82819=AXIS2_PLACEMENT_3D('',#190662,#94051,#94052);
#82820=AXIS2_PLACEMENT_3D('',#190663,#94053,#94054);
#82821=AXIS2_PLACEMENT_3D('',#190664,#94055,#94056);
#82822=AXIS2_PLACEMENT_3D('',#190668,#94058,#94059);
#82823=AXIS2_PLACEMENT_3D('',#190669,#94060,#94061);
#82824=AXIS2_PLACEMENT_3D('',#190670,#94062,#94063);
#82825=AXIS2_PLACEMENT_3D('',#190671,#94064,#94065);
#82826=AXIS2_PLACEMENT_3D('',#190672,#94066,#94067);
#82827=AXIS2_PLACEMENT_3D('',#190673,#94068,#94069);
#82828=AXIS2_PLACEMENT_3D('',#190678,#94071,#94072);
#82829=AXIS2_PLACEMENT_3D('',#190681,#94074,#94075);
#82830=AXIS2_PLACEMENT_3D('',#190682,#94076,#94077);
#82831=AXIS2_PLACEMENT_3D('',#190686,#94079,#94080);
#82832=AXIS2_PLACEMENT_3D('',#190687,#94081,#94082);
#82833=AXIS2_PLACEMENT_3D('',#190688,#94083,#94084);
#82834=AXIS2_PLACEMENT_3D('',#190692,#94086,#94087);
#82835=AXIS2_PLACEMENT_3D('',#190693,#94088,#94089);
#82836=AXIS2_PLACEMENT_3D('',#190694,#94090,#94091);
#82837=AXIS2_PLACEMENT_3D('',#190695,#94092,#94093);
#82838=AXIS2_PLACEMENT_3D('',#190696,#94094,#94095);
#82839=AXIS2_PLACEMENT_3D('',#190697,#94096,#94097);
#82840=AXIS2_PLACEMENT_3D('',#190702,#94099,#94100);
#82841=AXIS2_PLACEMENT_3D('',#190705,#94102,#94103);
#82842=AXIS2_PLACEMENT_3D('',#190706,#94104,#94105);
#82843=AXIS2_PLACEMENT_3D('',#190710,#94107,#94108);
#82844=AXIS2_PLACEMENT_3D('',#190711,#94109,#94110);
#82845=AXIS2_PLACEMENT_3D('',#190712,#94111,#94112);
#82846=AXIS2_PLACEMENT_3D('',#190716,#94114,#94115);
#82847=AXIS2_PLACEMENT_3D('',#190717,#94116,#94117);
#82848=AXIS2_PLACEMENT_3D('',#190718,#94118,#94119);
#82849=AXIS2_PLACEMENT_3D('',#190719,#94120,#94121);
#82850=AXIS2_PLACEMENT_3D('',#190720,#94122,#94123);
#82851=AXIS2_PLACEMENT_3D('',#190721,#94124,#94125);
#82852=AXIS2_PLACEMENT_3D('',#190728,#94128,#94129);
#82853=AXIS2_PLACEMENT_3D('',#190731,#94131,#94132);
#82854=AXIS2_PLACEMENT_3D('',#190732,#94133,#94134);
#82855=AXIS2_PLACEMENT_3D('',#190737,#94137,#94138);
#82856=AXIS2_PLACEMENT_3D('',#190738,#94139,#94140);
#82857=AXIS2_PLACEMENT_3D('',#190743,#94143,#94144);
#82858=AXIS2_PLACEMENT_3D('',#190744,#94145,#94146);
#82859=AXIS2_PLACEMENT_3D('',#190746,#94147,#94148);
#82860=AXIS2_PLACEMENT_3D('',#190748,#94150,#94151);
#82861=AXIS2_PLACEMENT_3D('',#190749,#94152,#94153);
#82862=AXIS2_PLACEMENT_3D('',#190750,#94154,#94155);
#82863=AXIS2_PLACEMENT_3D('',#190751,#94156,#94157);
#82864=AXIS2_PLACEMENT_3D('',#190758,#94160,#94161);
#82865=AXIS2_PLACEMENT_3D('',#190761,#94163,#94164);
#82866=AXIS2_PLACEMENT_3D('',#190762,#94165,#94166);
#82867=AXIS2_PLACEMENT_3D('',#190767,#94169,#94170);
#82868=AXIS2_PLACEMENT_3D('',#190768,#94171,#94172);
#82869=AXIS2_PLACEMENT_3D('',#190773,#94175,#94176);
#82870=AXIS2_PLACEMENT_3D('',#190774,#94177,#94178);
#82871=AXIS2_PLACEMENT_3D('',#190776,#94179,#94180);
#82872=AXIS2_PLACEMENT_3D('',#190778,#94182,#94183);
#82873=AXIS2_PLACEMENT_3D('',#190779,#94184,#94185);
#82874=AXIS2_PLACEMENT_3D('',#190780,#94186,#94187);
#82875=AXIS2_PLACEMENT_3D('',#190781,#94188,#94189);
#82876=AXIS2_PLACEMENT_3D('',#190786,#94191,#94192);
#82877=AXIS2_PLACEMENT_3D('',#190789,#94194,#94195);
#82878=AXIS2_PLACEMENT_3D('',#190790,#94196,#94197);
#82879=AXIS2_PLACEMENT_3D('',#190794,#94199,#94200);
#82880=AXIS2_PLACEMENT_3D('',#190795,#94201,#94202);
#82881=AXIS2_PLACEMENT_3D('',#190796,#94203,#94204);
#82882=AXIS2_PLACEMENT_3D('',#190800,#94206,#94207);
#82883=AXIS2_PLACEMENT_3D('',#190801,#94208,#94209);
#82884=AXIS2_PLACEMENT_3D('',#190802,#94210,#94211);
#82885=AXIS2_PLACEMENT_3D('',#190803,#94212,#94213);
#82886=AXIS2_PLACEMENT_3D('',#190804,#94214,#94215);
#82887=AXIS2_PLACEMENT_3D('',#190805,#94216,#94217);
#82888=AXIS2_PLACEMENT_3D('',#190810,#94219,#94220);
#82889=AXIS2_PLACEMENT_3D('',#190813,#94222,#94223);
#82890=AXIS2_PLACEMENT_3D('',#190814,#94224,#94225);
#82891=AXIS2_PLACEMENT_3D('',#190818,#94227,#94228);
#82892=AXIS2_PLACEMENT_3D('',#190819,#94229,#94230);
#82893=AXIS2_PLACEMENT_3D('',#190820,#94231,#94232);
#82894=AXIS2_PLACEMENT_3D('',#190824,#94234,#94235);
#82895=AXIS2_PLACEMENT_3D('',#190825,#94236,#94237);
#82896=AXIS2_PLACEMENT_3D('',#190826,#94238,#94239);
#82897=AXIS2_PLACEMENT_3D('',#190827,#94240,#94241);
#82898=AXIS2_PLACEMENT_3D('',#190828,#94242,#94243);
#82899=AXIS2_PLACEMENT_3D('',#190829,#94244,#94245);
#82900=AXIS2_PLACEMENT_3D('',#190834,#94247,#94248);
#82901=AXIS2_PLACEMENT_3D('',#190837,#94250,#94251);
#82902=AXIS2_PLACEMENT_3D('',#190838,#94252,#94253);
#82903=AXIS2_PLACEMENT_3D('',#190842,#94255,#94256);
#82904=AXIS2_PLACEMENT_3D('',#190843,#94257,#94258);
#82905=AXIS2_PLACEMENT_3D('',#190844,#94259,#94260);
#82906=AXIS2_PLACEMENT_3D('',#190848,#94262,#94263);
#82907=AXIS2_PLACEMENT_3D('',#190849,#94264,#94265);
#82908=AXIS2_PLACEMENT_3D('',#190850,#94266,#94267);
#82909=AXIS2_PLACEMENT_3D('',#190851,#94268,#94269);
#82910=AXIS2_PLACEMENT_3D('',#190852,#94270,#94271);
#82911=AXIS2_PLACEMENT_3D('',#190853,#94272,#94273);
#82912=AXIS2_PLACEMENT_3D('',#190858,#94275,#94276);
#82913=AXIS2_PLACEMENT_3D('',#190861,#94278,#94279);
#82914=AXIS2_PLACEMENT_3D('',#190862,#94280,#94281);
#82915=AXIS2_PLACEMENT_3D('',#190866,#94283,#94284);
#82916=AXIS2_PLACEMENT_3D('',#190867,#94285,#94286);
#82917=AXIS2_PLACEMENT_3D('',#190868,#94287,#94288);
#82918=AXIS2_PLACEMENT_3D('',#190872,#94290,#94291);
#82919=AXIS2_PLACEMENT_3D('',#190873,#94292,#94293);
#82920=AXIS2_PLACEMENT_3D('',#190874,#94294,#94295);
#82921=AXIS2_PLACEMENT_3D('',#190875,#94296,#94297);
#82922=AXIS2_PLACEMENT_3D('',#190876,#94298,#94299);
#82923=AXIS2_PLACEMENT_3D('',#190877,#94300,#94301);
#82924=AXIS2_PLACEMENT_3D('',#190882,#94303,#94304);
#82925=AXIS2_PLACEMENT_3D('',#190885,#94306,#94307);
#82926=AXIS2_PLACEMENT_3D('',#190886,#94308,#94309);
#82927=AXIS2_PLACEMENT_3D('',#190890,#94311,#94312);
#82928=AXIS2_PLACEMENT_3D('',#190891,#94313,#94314);
#82929=AXIS2_PLACEMENT_3D('',#190892,#94315,#94316);
#82930=AXIS2_PLACEMENT_3D('',#190898,#94319,#94320);
#82931=AXIS2_PLACEMENT_3D('',#190899,#94321,#94322);
#82932=AXIS2_PLACEMENT_3D('',#190900,#94323,#94324);
#82933=AXIS2_PLACEMENT_3D('',#190902,#94325,#94326);
#82934=AXIS2_PLACEMENT_3D('',#190904,#94328,#94329);
#82935=AXIS2_PLACEMENT_3D('',#190905,#94330,#94331);
#82936=AXIS2_PLACEMENT_3D('',#190906,#94332,#94333);
#82937=AXIS2_PLACEMENT_3D('',#190907,#94334,#94335);
#82938=AXIS2_PLACEMENT_3D('',#190912,#94337,#94338);
#82939=AXIS2_PLACEMENT_3D('',#190915,#94340,#94341);
#82940=AXIS2_PLACEMENT_3D('',#190916,#94342,#94343);
#82941=AXIS2_PLACEMENT_3D('',#190922,#94346,#94347);
#82942=AXIS2_PLACEMENT_3D('',#190923,#94348,#94349);
#82943=AXIS2_PLACEMENT_3D('',#190924,#94350,#94351);
#82944=AXIS2_PLACEMENT_3D('',#190929,#94354,#94355);
#82945=AXIS2_PLACEMENT_3D('',#190930,#94356,#94357);
#82946=AXIS2_PLACEMENT_3D('',#190932,#94358,#94359);
#82947=AXIS2_PLACEMENT_3D('',#190934,#94361,#94362);
#82948=AXIS2_PLACEMENT_3D('',#190935,#94363,#94364);
#82949=AXIS2_PLACEMENT_3D('',#190936,#94365,#94366);
#82950=AXIS2_PLACEMENT_3D('',#190937,#94367,#94368);
#82951=AXIS2_PLACEMENT_3D('',#190942,#94370,#94371);
#82952=AXIS2_PLACEMENT_3D('',#190945,#94373,#94374);
#82953=AXIS2_PLACEMENT_3D('',#190946,#94375,#94376);
#82954=AXIS2_PLACEMENT_3D('',#190952,#94379,#94380);
#82955=AXIS2_PLACEMENT_3D('',#190953,#94381,#94382);
#82956=AXIS2_PLACEMENT_3D('',#190954,#94383,#94384);
#82957=AXIS2_PLACEMENT_3D('',#190959,#94387,#94388);
#82958=AXIS2_PLACEMENT_3D('',#190960,#94389,#94390);
#82959=AXIS2_PLACEMENT_3D('',#190962,#94391,#94392);
#82960=AXIS2_PLACEMENT_3D('',#190964,#94394,#94395);
#82961=AXIS2_PLACEMENT_3D('',#190965,#94396,#94397);
#82962=AXIS2_PLACEMENT_3D('',#190966,#94398,#94399);
#82963=AXIS2_PLACEMENT_3D('',#190967,#94400,#94401);
#82964=AXIS2_PLACEMENT_3D('',#190972,#94403,#94404);
#82965=AXIS2_PLACEMENT_3D('',#190975,#94406,#94407);
#82966=AXIS2_PLACEMENT_3D('',#190976,#94408,#94409);
#82967=AXIS2_PLACEMENT_3D('',#190980,#94411,#94412);
#82968=AXIS2_PLACEMENT_3D('',#190981,#94413,#94414);
#82969=AXIS2_PLACEMENT_3D('',#190982,#94415,#94416);
#82970=AXIS2_PLACEMENT_3D('',#190988,#94419,#94420);
#82971=AXIS2_PLACEMENT_3D('',#190989,#94421,#94422);
#82972=AXIS2_PLACEMENT_3D('',#190990,#94423,#94424);
#82973=AXIS2_PLACEMENT_3D('',#190992,#94425,#94426);
#82974=AXIS2_PLACEMENT_3D('',#190994,#94428,#94429);
#82975=AXIS2_PLACEMENT_3D('',#190995,#94430,#94431);
#82976=AXIS2_PLACEMENT_3D('',#190996,#94432,#94433);
#82977=AXIS2_PLACEMENT_3D('',#190997,#94434,#94435);
#82978=AXIS2_PLACEMENT_3D('',#191002,#94437,#94438);
#82979=AXIS2_PLACEMENT_3D('',#191005,#94440,#94441);
#82980=AXIS2_PLACEMENT_3D('',#191006,#94442,#94443);
#82981=AXIS2_PLACEMENT_3D('',#191010,#94445,#94446);
#82982=AXIS2_PLACEMENT_3D('',#191011,#94447,#94448);
#82983=AXIS2_PLACEMENT_3D('',#191012,#94449,#94450);
#82984=AXIS2_PLACEMENT_3D('',#191016,#94452,#94453);
#82985=AXIS2_PLACEMENT_3D('',#191017,#94454,#94455);
#82986=AXIS2_PLACEMENT_3D('',#191018,#94456,#94457);
#82987=AXIS2_PLACEMENT_3D('',#191019,#94458,#94459);
#82988=AXIS2_PLACEMENT_3D('',#191020,#94460,#94461);
#82989=AXIS2_PLACEMENT_3D('',#191021,#94462,#94463);
#82990=AXIS2_PLACEMENT_3D('',#191026,#94465,#94466);
#82991=AXIS2_PLACEMENT_3D('',#191029,#94468,#94469);
#82992=AXIS2_PLACEMENT_3D('',#191030,#94470,#94471);
#82993=AXIS2_PLACEMENT_3D('',#191034,#94473,#94474);
#82994=AXIS2_PLACEMENT_3D('',#191035,#94475,#94476);
#82995=AXIS2_PLACEMENT_3D('',#191036,#94477,#94478);
#82996=AXIS2_PLACEMENT_3D('',#191040,#94480,#94481);
#82997=AXIS2_PLACEMENT_3D('',#191041,#94482,#94483);
#82998=AXIS2_PLACEMENT_3D('',#191042,#94484,#94485);
#82999=AXIS2_PLACEMENT_3D('',#191043,#94486,#94487);
#83000=AXIS2_PLACEMENT_3D('',#191044,#94488,#94489);
#83001=AXIS2_PLACEMENT_3D('',#191045,#94490,#94491);
#83002=AXIS2_PLACEMENT_3D('',#191050,#94493,#94494);
#83003=AXIS2_PLACEMENT_3D('',#191053,#94496,#94497);
#83004=AXIS2_PLACEMENT_3D('',#191054,#94498,#94499);
#83005=AXIS2_PLACEMENT_3D('',#191058,#94501,#94502);
#83006=AXIS2_PLACEMENT_3D('',#191059,#94503,#94504);
#83007=AXIS2_PLACEMENT_3D('',#191060,#94505,#94506);
#83008=AXIS2_PLACEMENT_3D('',#191064,#94508,#94509);
#83009=AXIS2_PLACEMENT_3D('',#191065,#94510,#94511);
#83010=AXIS2_PLACEMENT_3D('',#191066,#94512,#94513);
#83011=AXIS2_PLACEMENT_3D('',#191067,#94514,#94515);
#83012=AXIS2_PLACEMENT_3D('',#191068,#94516,#94517);
#83013=AXIS2_PLACEMENT_3D('',#191069,#94518,#94519);
#83014=AXIS2_PLACEMENT_3D('',#191074,#94521,#94522);
#83015=AXIS2_PLACEMENT_3D('',#191077,#94524,#94525);
#83016=AXIS2_PLACEMENT_3D('',#191078,#94526,#94527);
#83017=AXIS2_PLACEMENT_3D('',#191082,#94529,#94530);
#83018=AXIS2_PLACEMENT_3D('',#191083,#94531,#94532);
#83019=AXIS2_PLACEMENT_3D('',#191084,#94533,#94534);
#83020=AXIS2_PLACEMENT_3D('',#191088,#94536,#94537);
#83021=AXIS2_PLACEMENT_3D('',#191089,#94538,#94539);
#83022=AXIS2_PLACEMENT_3D('',#191090,#94540,#94541);
#83023=AXIS2_PLACEMENT_3D('',#191091,#94542,#94543);
#83024=AXIS2_PLACEMENT_3D('',#191092,#94544,#94545);
#83025=AXIS2_PLACEMENT_3D('',#191093,#94546,#94547);
#83026=AXIS2_PLACEMENT_3D('',#191098,#94549,#94550);
#83027=AXIS2_PLACEMENT_3D('',#191101,#94552,#94553);
#83028=AXIS2_PLACEMENT_3D('',#191102,#94554,#94555);
#83029=AXIS2_PLACEMENT_3D('',#191106,#94557,#94558);
#83030=AXIS2_PLACEMENT_3D('',#191107,#94559,#94560);
#83031=AXIS2_PLACEMENT_3D('',#191108,#94561,#94562);
#83032=AXIS2_PLACEMENT_3D('',#191112,#94564,#94565);
#83033=AXIS2_PLACEMENT_3D('',#191113,#94566,#94567);
#83034=AXIS2_PLACEMENT_3D('',#191114,#94568,#94569);
#83035=AXIS2_PLACEMENT_3D('',#191115,#94570,#94571);
#83036=AXIS2_PLACEMENT_3D('',#191116,#94572,#94573);
#83037=AXIS2_PLACEMENT_3D('',#191117,#94574,#94575);
#83038=AXIS2_PLACEMENT_3D('',#191122,#94577,#94578);
#83039=AXIS2_PLACEMENT_3D('',#191125,#94580,#94581);
#83040=AXIS2_PLACEMENT_3D('',#191126,#94582,#94583);
#83041=AXIS2_PLACEMENT_3D('',#191130,#94585,#94586);
#83042=AXIS2_PLACEMENT_3D('',#191131,#94587,#94588);
#83043=AXIS2_PLACEMENT_3D('',#191132,#94589,#94590);
#83044=AXIS2_PLACEMENT_3D('',#191136,#94592,#94593);
#83045=AXIS2_PLACEMENT_3D('',#191137,#94594,#94595);
#83046=AXIS2_PLACEMENT_3D('',#191138,#94596,#94597);
#83047=AXIS2_PLACEMENT_3D('',#191139,#94598,#94599);
#83048=AXIS2_PLACEMENT_3D('',#191140,#94600,#94601);
#83049=AXIS2_PLACEMENT_3D('',#191141,#94602,#94603);
#83050=AXIS2_PLACEMENT_3D('',#191146,#94605,#94606);
#83051=AXIS2_PLACEMENT_3D('',#191149,#94608,#94609);
#83052=AXIS2_PLACEMENT_3D('',#191150,#94610,#94611);
#83053=AXIS2_PLACEMENT_3D('',#191154,#94613,#94614);
#83054=AXIS2_PLACEMENT_3D('',#191155,#94615,#94616);
#83055=AXIS2_PLACEMENT_3D('',#191156,#94617,#94618);
#83056=AXIS2_PLACEMENT_3D('',#191160,#94620,#94621);
#83057=AXIS2_PLACEMENT_3D('',#191161,#94622,#94623);
#83058=AXIS2_PLACEMENT_3D('',#191162,#94624,#94625);
#83059=AXIS2_PLACEMENT_3D('',#191163,#94626,#94627);
#83060=AXIS2_PLACEMENT_3D('',#191164,#94628,#94629);
#83061=AXIS2_PLACEMENT_3D('',#191165,#94630,#94631);
#83062=AXIS2_PLACEMENT_3D('',#191170,#94633,#94634);
#83063=AXIS2_PLACEMENT_3D('',#191173,#94636,#94637);
#83064=AXIS2_PLACEMENT_3D('',#191174,#94638,#94639);
#83065=AXIS2_PLACEMENT_3D('',#191178,#94641,#94642);
#83066=AXIS2_PLACEMENT_3D('',#191179,#94643,#94644);
#83067=AXIS2_PLACEMENT_3D('',#191180,#94645,#94646);
#83068=AXIS2_PLACEMENT_3D('',#191184,#94648,#94649);
#83069=AXIS2_PLACEMENT_3D('',#191185,#94650,#94651);
#83070=AXIS2_PLACEMENT_3D('',#191186,#94652,#94653);
#83071=AXIS2_PLACEMENT_3D('',#191187,#94654,#94655);
#83072=AXIS2_PLACEMENT_3D('',#191188,#94656,#94657);
#83073=AXIS2_PLACEMENT_3D('',#191189,#94658,#94659);
#83074=AXIS2_PLACEMENT_3D('',#191194,#94661,#94662);
#83075=AXIS2_PLACEMENT_3D('',#191197,#94664,#94665);
#83076=AXIS2_PLACEMENT_3D('',#191198,#94666,#94667);
#83077=AXIS2_PLACEMENT_3D('',#191202,#94669,#94670);
#83078=AXIS2_PLACEMENT_3D('',#191203,#94671,#94672);
#83079=AXIS2_PLACEMENT_3D('',#191204,#94673,#94674);
#83080=AXIS2_PLACEMENT_3D('',#191208,#94676,#94677);
#83081=AXIS2_PLACEMENT_3D('',#191209,#94678,#94679);
#83082=AXIS2_PLACEMENT_3D('',#191210,#94680,#94681);
#83083=AXIS2_PLACEMENT_3D('',#191211,#94682,#94683);
#83084=AXIS2_PLACEMENT_3D('',#191212,#94684,#94685);
#83085=AXIS2_PLACEMENT_3D('',#191213,#94686,#94687);
#83086=AXIS2_PLACEMENT_3D('',#191218,#94689,#94690);
#83087=AXIS2_PLACEMENT_3D('',#191221,#94692,#94693);
#83088=AXIS2_PLACEMENT_3D('',#191222,#94694,#94695);
#83089=AXIS2_PLACEMENT_3D('',#191226,#94697,#94698);
#83090=AXIS2_PLACEMENT_3D('',#191227,#94699,#94700);
#83091=AXIS2_PLACEMENT_3D('',#191228,#94701,#94702);
#83092=AXIS2_PLACEMENT_3D('',#191232,#94704,#94705);
#83093=AXIS2_PLACEMENT_3D('',#191233,#94706,#94707);
#83094=AXIS2_PLACEMENT_3D('',#191234,#94708,#94709);
#83095=AXIS2_PLACEMENT_3D('',#191235,#94710,#94711);
#83096=AXIS2_PLACEMENT_3D('',#191236,#94712,#94713);
#83097=AXIS2_PLACEMENT_3D('',#191237,#94714,#94715);
#83098=AXIS2_PLACEMENT_3D('',#191242,#94717,#94718);
#83099=AXIS2_PLACEMENT_3D('',#191245,#94720,#94721);
#83100=AXIS2_PLACEMENT_3D('',#191246,#94722,#94723);
#83101=AXIS2_PLACEMENT_3D('',#191250,#94725,#94726);
#83102=AXIS2_PLACEMENT_3D('',#191251,#94727,#94728);
#83103=AXIS2_PLACEMENT_3D('',#191252,#94729,#94730);
#83104=AXIS2_PLACEMENT_3D('',#191258,#94733,#94734);
#83105=AXIS2_PLACEMENT_3D('',#191259,#94735,#94736);
#83106=AXIS2_PLACEMENT_3D('',#191260,#94737,#94738);
#83107=AXIS2_PLACEMENT_3D('',#191262,#94739,#94740);
#83108=AXIS2_PLACEMENT_3D('',#191264,#94742,#94743);
#83109=AXIS2_PLACEMENT_3D('',#191265,#94744,#94745);
#83110=AXIS2_PLACEMENT_3D('',#191266,#94746,#94747);
#83111=AXIS2_PLACEMENT_3D('',#191267,#94748,#94749);
#83112=AXIS2_PLACEMENT_3D('',#191272,#94751,#94752);
#83113=AXIS2_PLACEMENT_3D('',#191275,#94754,#94755);
#83114=AXIS2_PLACEMENT_3D('',#191276,#94756,#94757);
#83115=AXIS2_PLACEMENT_3D('',#191280,#94759,#94760);
#83116=AXIS2_PLACEMENT_3D('',#191281,#94761,#94762);
#83117=AXIS2_PLACEMENT_3D('',#191282,#94763,#94764);
#83118=AXIS2_PLACEMENT_3D('',#191288,#94767,#94768);
#83119=AXIS2_PLACEMENT_3D('',#191289,#94769,#94770);
#83120=AXIS2_PLACEMENT_3D('',#191290,#94771,#94772);
#83121=AXIS2_PLACEMENT_3D('',#191292,#94773,#94774);
#83122=AXIS2_PLACEMENT_3D('',#191294,#94776,#94777);
#83123=AXIS2_PLACEMENT_3D('',#191295,#94778,#94779);
#83124=AXIS2_PLACEMENT_3D('',#191296,#94780,#94781);
#83125=AXIS2_PLACEMENT_3D('',#191297,#94782,#94783);
#83126=AXIS2_PLACEMENT_3D('',#191302,#94785,#94786);
#83127=AXIS2_PLACEMENT_3D('',#191305,#94788,#94789);
#83128=AXIS2_PLACEMENT_3D('',#191306,#94790,#94791);
#83129=AXIS2_PLACEMENT_3D('',#191310,#94793,#94794);
#83130=AXIS2_PLACEMENT_3D('',#191311,#94795,#94796);
#83131=AXIS2_PLACEMENT_3D('',#191312,#94797,#94798);
#83132=AXIS2_PLACEMENT_3D('',#191316,#94800,#94801);
#83133=AXIS2_PLACEMENT_3D('',#191317,#94802,#94803);
#83134=AXIS2_PLACEMENT_3D('',#191318,#94804,#94805);
#83135=AXIS2_PLACEMENT_3D('',#191319,#94806,#94807);
#83136=AXIS2_PLACEMENT_3D('',#191320,#94808,#94809);
#83137=AXIS2_PLACEMENT_3D('',#191321,#94810,#94811);
#83138=AXIS2_PLACEMENT_3D('',#191326,#94813,#94814);
#83139=AXIS2_PLACEMENT_3D('',#191329,#94816,#94817);
#83140=AXIS2_PLACEMENT_3D('',#191330,#94818,#94819);
#83141=AXIS2_PLACEMENT_3D('',#191334,#94821,#94822);
#83142=AXIS2_PLACEMENT_3D('',#191335,#94823,#94824);
#83143=AXIS2_PLACEMENT_3D('',#191336,#94825,#94826);
#83144=AXIS2_PLACEMENT_3D('',#191340,#94828,#94829);
#83145=AXIS2_PLACEMENT_3D('',#191341,#94830,#94831);
#83146=AXIS2_PLACEMENT_3D('',#191342,#94832,#94833);
#83147=AXIS2_PLACEMENT_3D('',#191343,#94834,#94835);
#83148=AXIS2_PLACEMENT_3D('',#191344,#94836,#94837);
#83149=AXIS2_PLACEMENT_3D('',#191345,#94838,#94839);
#83150=AXIS2_PLACEMENT_3D('',#191350,#94841,#94842);
#83151=AXIS2_PLACEMENT_3D('',#191353,#94844,#94845);
#83152=AXIS2_PLACEMENT_3D('',#191354,#94846,#94847);
#83153=AXIS2_PLACEMENT_3D('',#191358,#94849,#94850);
#83154=AXIS2_PLACEMENT_3D('',#191359,#94851,#94852);
#83155=AXIS2_PLACEMENT_3D('',#191360,#94853,#94854);
#83156=AXIS2_PLACEMENT_3D('',#191364,#94856,#94857);
#83157=AXIS2_PLACEMENT_3D('',#191365,#94858,#94859);
#83158=AXIS2_PLACEMENT_3D('',#191366,#94860,#94861);
#83159=AXIS2_PLACEMENT_3D('',#191367,#94862,#94863);
#83160=AXIS2_PLACEMENT_3D('',#191368,#94864,#94865);
#83161=AXIS2_PLACEMENT_3D('',#191369,#94866,#94867);
#83162=AXIS2_PLACEMENT_3D('',#191374,#94869,#94870);
#83163=AXIS2_PLACEMENT_3D('',#191377,#94872,#94873);
#83164=AXIS2_PLACEMENT_3D('',#191378,#94874,#94875);
#83165=AXIS2_PLACEMENT_3D('',#191382,#94877,#94878);
#83166=AXIS2_PLACEMENT_3D('',#191383,#94879,#94880);
#83167=AXIS2_PLACEMENT_3D('',#191384,#94881,#94882);
#83168=AXIS2_PLACEMENT_3D('',#191388,#94884,#94885);
#83169=AXIS2_PLACEMENT_3D('',#191389,#94886,#94887);
#83170=AXIS2_PLACEMENT_3D('',#191390,#94888,#94889);
#83171=AXIS2_PLACEMENT_3D('',#191391,#94890,#94891);
#83172=AXIS2_PLACEMENT_3D('',#191392,#94892,#94893);
#83173=AXIS2_PLACEMENT_3D('',#191393,#94894,#94895);
#83174=AXIS2_PLACEMENT_3D('',#191398,#94897,#94898);
#83175=AXIS2_PLACEMENT_3D('',#191401,#94900,#94901);
#83176=AXIS2_PLACEMENT_3D('',#191402,#94902,#94903);
#83177=AXIS2_PLACEMENT_3D('',#191406,#94905,#94906);
#83178=AXIS2_PLACEMENT_3D('',#191407,#94907,#94908);
#83179=AXIS2_PLACEMENT_3D('',#191408,#94909,#94910);
#83180=AXIS2_PLACEMENT_3D('',#191412,#94912,#94913);
#83181=AXIS2_PLACEMENT_3D('',#191413,#94914,#94915);
#83182=AXIS2_PLACEMENT_3D('',#191414,#94916,#94917);
#83183=AXIS2_PLACEMENT_3D('',#191415,#94918,#94919);
#83184=AXIS2_PLACEMENT_3D('',#191416,#94920,#94921);
#83185=AXIS2_PLACEMENT_3D('',#191417,#94922,#94923);
#83186=AXIS2_PLACEMENT_3D('',#191422,#94925,#94926);
#83187=AXIS2_PLACEMENT_3D('',#191425,#94928,#94929);
#83188=AXIS2_PLACEMENT_3D('',#191426,#94930,#94931);
#83189=AXIS2_PLACEMENT_3D('',#191430,#94933,#94934);
#83190=AXIS2_PLACEMENT_3D('',#191431,#94935,#94936);
#83191=AXIS2_PLACEMENT_3D('',#191432,#94937,#94938);
#83192=AXIS2_PLACEMENT_3D('',#191436,#94940,#94941);
#83193=AXIS2_PLACEMENT_3D('',#191437,#94942,#94943);
#83194=AXIS2_PLACEMENT_3D('',#191438,#94944,#94945);
#83195=AXIS2_PLACEMENT_3D('',#191439,#94946,#94947);
#83196=AXIS2_PLACEMENT_3D('',#191440,#94948,#94949);
#83197=AXIS2_PLACEMENT_3D('',#191441,#94950,#94951);
#83198=AXIS2_PLACEMENT_3D('',#191446,#94953,#94954);
#83199=AXIS2_PLACEMENT_3D('',#191449,#94956,#94957);
#83200=AXIS2_PLACEMENT_3D('',#191450,#94958,#94959);
#83201=AXIS2_PLACEMENT_3D('',#191454,#94961,#94962);
#83202=AXIS2_PLACEMENT_3D('',#191455,#94963,#94964);
#83203=AXIS2_PLACEMENT_3D('',#191456,#94965,#94966);
#83204=AXIS2_PLACEMENT_3D('',#191460,#94968,#94969);
#83205=AXIS2_PLACEMENT_3D('',#191461,#94970,#94971);
#83206=AXIS2_PLACEMENT_3D('',#191462,#94972,#94973);
#83207=AXIS2_PLACEMENT_3D('',#191463,#94974,#94975);
#83208=AXIS2_PLACEMENT_3D('',#191464,#94976,#94977);
#83209=AXIS2_PLACEMENT_3D('',#191465,#94978,#94979);
#83210=AXIS2_PLACEMENT_3D('',#191470,#94981,#94982);
#83211=AXIS2_PLACEMENT_3D('',#191473,#94984,#94985);
#83212=AXIS2_PLACEMENT_3D('',#191474,#94986,#94987);
#83213=AXIS2_PLACEMENT_3D('',#191478,#94989,#94990);
#83214=AXIS2_PLACEMENT_3D('',#191479,#94991,#94992);
#83215=AXIS2_PLACEMENT_3D('',#191480,#94993,#94994);
#83216=AXIS2_PLACEMENT_3D('',#191484,#94996,#94997);
#83217=AXIS2_PLACEMENT_3D('',#191485,#94998,#94999);
#83218=AXIS2_PLACEMENT_3D('',#191486,#95000,#95001);
#83219=AXIS2_PLACEMENT_3D('',#191487,#95002,#95003);
#83220=AXIS2_PLACEMENT_3D('',#191488,#95004,#95005);
#83221=AXIS2_PLACEMENT_3D('',#191489,#95006,#95007);
#83222=AXIS2_PLACEMENT_3D('',#191494,#95009,#95010);
#83223=AXIS2_PLACEMENT_3D('',#191497,#95012,#95013);
#83224=AXIS2_PLACEMENT_3D('',#191498,#95014,#95015);
#83225=AXIS2_PLACEMENT_3D('',#191502,#95017,#95018);
#83226=AXIS2_PLACEMENT_3D('',#191503,#95019,#95020);
#83227=AXIS2_PLACEMENT_3D('',#191504,#95021,#95022);
#83228=AXIS2_PLACEMENT_3D('',#191508,#95024,#95025);
#83229=AXIS2_PLACEMENT_3D('',#191509,#95026,#95027);
#83230=AXIS2_PLACEMENT_3D('',#191510,#95028,#95029);
#83231=AXIS2_PLACEMENT_3D('',#191511,#95030,#95031);
#83232=AXIS2_PLACEMENT_3D('',#191512,#95032,#95033);
#83233=AXIS2_PLACEMENT_3D('',#191513,#95034,#95035);
#83234=AXIS2_PLACEMENT_3D('',#191518,#95037,#95038);
#83235=AXIS2_PLACEMENT_3D('',#191521,#95040,#95041);
#83236=AXIS2_PLACEMENT_3D('',#191522,#95042,#95043);
#83237=AXIS2_PLACEMENT_3D('',#191528,#95046,#95047);
#83238=AXIS2_PLACEMENT_3D('',#191529,#95048,#95049);
#83239=AXIS2_PLACEMENT_3D('',#191530,#95050,#95051);
#83240=AXIS2_PLACEMENT_3D('',#191535,#95054,#95055);
#83241=AXIS2_PLACEMENT_3D('',#191536,#95056,#95057);
#83242=AXIS2_PLACEMENT_3D('',#191538,#95058,#95059);
#83243=AXIS2_PLACEMENT_3D('',#191540,#95061,#95062);
#83244=AXIS2_PLACEMENT_3D('',#191541,#95063,#95064);
#83245=AXIS2_PLACEMENT_3D('',#191542,#95065,#95066);
#83246=AXIS2_PLACEMENT_3D('',#191543,#95067,#95068);
#83247=AXIS2_PLACEMENT_3D('',#191548,#95070,#95071);
#83248=AXIS2_PLACEMENT_3D('',#191551,#95073,#95074);
#83249=AXIS2_PLACEMENT_3D('',#191552,#95075,#95076);
#83250=AXIS2_PLACEMENT_3D('',#191556,#95078,#95079);
#83251=AXIS2_PLACEMENT_3D('',#191557,#95080,#95081);
#83252=AXIS2_PLACEMENT_3D('',#191558,#95082,#95083);
#83253=AXIS2_PLACEMENT_3D('',#191564,#95086,#95087);
#83254=AXIS2_PLACEMENT_3D('',#191565,#95088,#95089);
#83255=AXIS2_PLACEMENT_3D('',#191566,#95090,#95091);
#83256=AXIS2_PLACEMENT_3D('',#191568,#95092,#95093);
#83257=AXIS2_PLACEMENT_3D('',#191570,#95095,#95096);
#83258=AXIS2_PLACEMENT_3D('',#191571,#95097,#95098);
#83259=AXIS2_PLACEMENT_3D('',#191572,#95099,#95100);
#83260=AXIS2_PLACEMENT_3D('',#191573,#95101,#95102);
#83261=AXIS2_PLACEMENT_3D('',#191578,#95104,#95105);
#83262=AXIS2_PLACEMENT_3D('',#191581,#95107,#95108);
#83263=AXIS2_PLACEMENT_3D('',#191582,#95109,#95110);
#83264=AXIS2_PLACEMENT_3D('',#191586,#95112,#95113);
#83265=AXIS2_PLACEMENT_3D('',#191587,#95114,#95115);
#83266=AXIS2_PLACEMENT_3D('',#191588,#95116,#95117);
#83267=AXIS2_PLACEMENT_3D('',#191592,#95119,#95120);
#83268=AXIS2_PLACEMENT_3D('',#191593,#95121,#95122);
#83269=AXIS2_PLACEMENT_3D('',#191594,#95123,#95124);
#83270=AXIS2_PLACEMENT_3D('',#191595,#95125,#95126);
#83271=AXIS2_PLACEMENT_3D('',#191596,#95127,#95128);
#83272=AXIS2_PLACEMENT_3D('',#191597,#95129,#95130);
#83273=AXIS2_PLACEMENT_3D('',#191602,#95132,#95133);
#83274=AXIS2_PLACEMENT_3D('',#191605,#95135,#95136);
#83275=AXIS2_PLACEMENT_3D('',#191606,#95137,#95138);
#83276=AXIS2_PLACEMENT_3D('',#191610,#95140,#95141);
#83277=AXIS2_PLACEMENT_3D('',#191611,#95142,#95143);
#83278=AXIS2_PLACEMENT_3D('',#191612,#95144,#95145);
#83279=AXIS2_PLACEMENT_3D('',#191616,#95147,#95148);
#83280=AXIS2_PLACEMENT_3D('',#191617,#95149,#95150);
#83281=AXIS2_PLACEMENT_3D('',#191618,#95151,#95152);
#83282=AXIS2_PLACEMENT_3D('',#191619,#95153,#95154);
#83283=AXIS2_PLACEMENT_3D('',#191620,#95155,#95156);
#83284=AXIS2_PLACEMENT_3D('',#191621,#95157,#95158);
#83285=AXIS2_PLACEMENT_3D('',#191626,#95160,#95161);
#83286=AXIS2_PLACEMENT_3D('',#191629,#95163,#95164);
#83287=AXIS2_PLACEMENT_3D('',#191630,#95165,#95166);
#83288=AXIS2_PLACEMENT_3D('',#191634,#95168,#95169);
#83289=AXIS2_PLACEMENT_3D('',#191635,#95170,#95171);
#83290=AXIS2_PLACEMENT_3D('',#191636,#95172,#95173);
#83291=AXIS2_PLACEMENT_3D('',#191640,#95175,#95176);
#83292=AXIS2_PLACEMENT_3D('',#191641,#95177,#95178);
#83293=AXIS2_PLACEMENT_3D('',#191642,#95179,#95180);
#83294=AXIS2_PLACEMENT_3D('',#191643,#95181,#95182);
#83295=AXIS2_PLACEMENT_3D('',#191644,#95183,#95184);
#83296=AXIS2_PLACEMENT_3D('',#191645,#95185,#95186);
#83297=AXIS2_PLACEMENT_3D('',#191650,#95188,#95189);
#83298=AXIS2_PLACEMENT_3D('',#191653,#95191,#95192);
#83299=AXIS2_PLACEMENT_3D('',#191654,#95193,#95194);
#83300=AXIS2_PLACEMENT_3D('',#191658,#95196,#95197);
#83301=AXIS2_PLACEMENT_3D('',#191659,#95198,#95199);
#83302=AXIS2_PLACEMENT_3D('',#191660,#95200,#95201);
#83303=AXIS2_PLACEMENT_3D('',#191664,#95203,#95204);
#83304=AXIS2_PLACEMENT_3D('',#191665,#95205,#95206);
#83305=AXIS2_PLACEMENT_3D('',#191666,#95207,#95208);
#83306=AXIS2_PLACEMENT_3D('',#191667,#95209,#95210);
#83307=AXIS2_PLACEMENT_3D('',#191668,#95211,#95212);
#83308=AXIS2_PLACEMENT_3D('',#191669,#95213,#95214);
#83309=AXIS2_PLACEMENT_3D('',#191674,#95216,#95217);
#83310=AXIS2_PLACEMENT_3D('',#191677,#95219,#95220);
#83311=AXIS2_PLACEMENT_3D('',#191678,#95221,#95222);
#83312=AXIS2_PLACEMENT_3D('',#191682,#95224,#95225);
#83313=AXIS2_PLACEMENT_3D('',#191683,#95226,#95227);
#83314=AXIS2_PLACEMENT_3D('',#191684,#95228,#95229);
#83315=AXIS2_PLACEMENT_3D('',#191688,#95231,#95232);
#83316=AXIS2_PLACEMENT_3D('',#191689,#95233,#95234);
#83317=AXIS2_PLACEMENT_3D('',#191690,#95235,#95236);
#83318=AXIS2_PLACEMENT_3D('',#191691,#95237,#95238);
#83319=AXIS2_PLACEMENT_3D('',#191692,#95239,#95240);
#83320=AXIS2_PLACEMENT_3D('',#191693,#95241,#95242);
#83321=AXIS2_PLACEMENT_3D('',#191698,#95244,#95245);
#83322=AXIS2_PLACEMENT_3D('',#191701,#95247,#95248);
#83323=AXIS2_PLACEMENT_3D('',#191702,#95249,#95250);
#83324=AXIS2_PLACEMENT_3D('',#191706,#95252,#95253);
#83325=AXIS2_PLACEMENT_3D('',#191707,#95254,#95255);
#83326=AXIS2_PLACEMENT_3D('',#191708,#95256,#95257);
#83327=AXIS2_PLACEMENT_3D('',#191712,#95259,#95260);
#83328=AXIS2_PLACEMENT_3D('',#191713,#95261,#95262);
#83329=AXIS2_PLACEMENT_3D('',#191714,#95263,#95264);
#83330=AXIS2_PLACEMENT_3D('',#191715,#95265,#95266);
#83331=AXIS2_PLACEMENT_3D('',#191716,#95267,#95268);
#83332=AXIS2_PLACEMENT_3D('',#191717,#95269,#95270);
#83333=AXIS2_PLACEMENT_3D('',#191722,#95272,#95273);
#83334=AXIS2_PLACEMENT_3D('',#191725,#95275,#95276);
#83335=AXIS2_PLACEMENT_3D('',#191726,#95277,#95278);
#83336=AXIS2_PLACEMENT_3D('',#191730,#95280,#95281);
#83337=AXIS2_PLACEMENT_3D('',#191731,#95282,#95283);
#83338=AXIS2_PLACEMENT_3D('',#191732,#95284,#95285);
#83339=AXIS2_PLACEMENT_3D('',#191736,#95287,#95288);
#83340=AXIS2_PLACEMENT_3D('',#191737,#95289,#95290);
#83341=AXIS2_PLACEMENT_3D('',#191738,#95291,#95292);
#83342=AXIS2_PLACEMENT_3D('',#191739,#95293,#95294);
#83343=AXIS2_PLACEMENT_3D('',#191740,#95295,#95296);
#83344=AXIS2_PLACEMENT_3D('',#191741,#95297,#95298);
#83345=AXIS2_PLACEMENT_3D('',#191746,#95300,#95301);
#83346=AXIS2_PLACEMENT_3D('',#191749,#95303,#95304);
#83347=AXIS2_PLACEMENT_3D('',#191750,#95305,#95306);
#83348=AXIS2_PLACEMENT_3D('',#191754,#95308,#95309);
#83349=AXIS2_PLACEMENT_3D('',#191755,#95310,#95311);
#83350=AXIS2_PLACEMENT_3D('',#191756,#95312,#95313);
#83351=AXIS2_PLACEMENT_3D('',#191760,#95315,#95316);
#83352=AXIS2_PLACEMENT_3D('',#191761,#95317,#95318);
#83353=AXIS2_PLACEMENT_3D('',#191762,#95319,#95320);
#83354=AXIS2_PLACEMENT_3D('',#191763,#95321,#95322);
#83355=AXIS2_PLACEMENT_3D('',#191764,#95323,#95324);
#83356=AXIS2_PLACEMENT_3D('',#191765,#95325,#95326);
#83357=AXIS2_PLACEMENT_3D('',#191770,#95328,#95329);
#83358=AXIS2_PLACEMENT_3D('',#191773,#95331,#95332);
#83359=AXIS2_PLACEMENT_3D('',#191774,#95333,#95334);
#83360=AXIS2_PLACEMENT_3D('',#191778,#95336,#95337);
#83361=AXIS2_PLACEMENT_3D('',#191779,#95338,#95339);
#83362=AXIS2_PLACEMENT_3D('',#191780,#95340,#95341);
#83363=AXIS2_PLACEMENT_3D('',#191784,#95343,#95344);
#83364=AXIS2_PLACEMENT_3D('',#191785,#95345,#95346);
#83365=AXIS2_PLACEMENT_3D('',#191786,#95347,#95348);
#83366=AXIS2_PLACEMENT_3D('',#191787,#95349,#95350);
#83367=AXIS2_PLACEMENT_3D('',#191788,#95351,#95352);
#83368=AXIS2_PLACEMENT_3D('',#191789,#95353,#95354);
#83369=AXIS2_PLACEMENT_3D('',#191794,#95356,#95357);
#83370=AXIS2_PLACEMENT_3D('',#191797,#95359,#95360);
#83371=AXIS2_PLACEMENT_3D('',#191798,#95361,#95362);
#83372=AXIS2_PLACEMENT_3D('',#191802,#95364,#95365);
#83373=AXIS2_PLACEMENT_3D('',#191803,#95366,#95367);
#83374=AXIS2_PLACEMENT_3D('',#191804,#95368,#95369);
#83375=AXIS2_PLACEMENT_3D('',#191808,#95371,#95372);
#83376=AXIS2_PLACEMENT_3D('',#191809,#95373,#95374);
#83377=AXIS2_PLACEMENT_3D('',#191810,#95375,#95376);
#83378=AXIS2_PLACEMENT_3D('',#191811,#95377,#95378);
#83379=AXIS2_PLACEMENT_3D('',#191812,#95379,#95380);
#83380=AXIS2_PLACEMENT_3D('',#191813,#95381,#95382);
#83381=AXIS2_PLACEMENT_3D('',#191818,#95384,#95385);
#83382=AXIS2_PLACEMENT_3D('',#191821,#95387,#95388);
#83383=AXIS2_PLACEMENT_3D('',#191822,#95389,#95390);
#83384=AXIS2_PLACEMENT_3D('',#191826,#95392,#95393);
#83385=AXIS2_PLACEMENT_3D('',#191827,#95394,#95395);
#83386=AXIS2_PLACEMENT_3D('',#191828,#95396,#95397);
#83387=AXIS2_PLACEMENT_3D('',#191832,#95399,#95400);
#83388=AXIS2_PLACEMENT_3D('',#191833,#95401,#95402);
#83389=AXIS2_PLACEMENT_3D('',#191834,#95403,#95404);
#83390=AXIS2_PLACEMENT_3D('',#191835,#95405,#95406);
#83391=AXIS2_PLACEMENT_3D('',#191836,#95407,#95408);
#83392=AXIS2_PLACEMENT_3D('',#191837,#95409,#95410);
#83393=AXIS2_PLACEMENT_3D('',#191842,#95412,#95413);
#83394=AXIS2_PLACEMENT_3D('',#191845,#95415,#95416);
#83395=AXIS2_PLACEMENT_3D('',#191846,#95417,#95418);
#83396=AXIS2_PLACEMENT_3D('',#191850,#95420,#95421);
#83397=AXIS2_PLACEMENT_3D('',#191851,#95422,#95423);
#83398=AXIS2_PLACEMENT_3D('',#191852,#95424,#95425);
#83399=AXIS2_PLACEMENT_3D('',#191856,#95427,#95428);
#83400=AXIS2_PLACEMENT_3D('',#191857,#95429,#95430);
#83401=AXIS2_PLACEMENT_3D('',#191858,#95431,#95432);
#83402=AXIS2_PLACEMENT_3D('',#191859,#95433,#95434);
#83403=AXIS2_PLACEMENT_3D('',#191860,#95435,#95436);
#83404=AXIS2_PLACEMENT_3D('',#191861,#95437,#95438);
#83405=AXIS2_PLACEMENT_3D('',#191866,#95440,#95441);
#83406=AXIS2_PLACEMENT_3D('',#191869,#95443,#95444);
#83407=AXIS2_PLACEMENT_3D('',#191870,#95445,#95446);
#83408=AXIS2_PLACEMENT_3D('',#191874,#95448,#95449);
#83409=AXIS2_PLACEMENT_3D('',#191875,#95450,#95451);
#83410=AXIS2_PLACEMENT_3D('',#191876,#95452,#95453);
#83411=AXIS2_PLACEMENT_3D('',#191880,#95455,#95456);
#83412=AXIS2_PLACEMENT_3D('',#191881,#95457,#95458);
#83413=AXIS2_PLACEMENT_3D('',#191882,#95459,#95460);
#83414=AXIS2_PLACEMENT_3D('',#191883,#95461,#95462);
#83415=AXIS2_PLACEMENT_3D('',#191884,#95463,#95464);
#83416=AXIS2_PLACEMENT_3D('',#191885,#95465,#95466);
#83417=AXIS2_PLACEMENT_3D('',#191890,#95468,#95469);
#83418=AXIS2_PLACEMENT_3D('',#191893,#95471,#95472);
#83419=AXIS2_PLACEMENT_3D('',#191894,#95473,#95474);
#83420=AXIS2_PLACEMENT_3D('',#191898,#95476,#95477);
#83421=AXIS2_PLACEMENT_3D('',#191899,#95478,#95479);
#83422=AXIS2_PLACEMENT_3D('',#191900,#95480,#95481);
#83423=AXIS2_PLACEMENT_3D('',#191904,#95483,#95484);
#83424=AXIS2_PLACEMENT_3D('',#191905,#95485,#95486);
#83425=AXIS2_PLACEMENT_3D('',#191906,#95487,#95488);
#83426=AXIS2_PLACEMENT_3D('',#191907,#95489,#95490);
#83427=AXIS2_PLACEMENT_3D('',#191908,#95491,#95492);
#83428=AXIS2_PLACEMENT_3D('',#191909,#95493,#95494);
#83429=AXIS2_PLACEMENT_3D('',#191914,#95496,#95497);
#83430=AXIS2_PLACEMENT_3D('',#191917,#95499,#95500);
#83431=AXIS2_PLACEMENT_3D('',#191918,#95501,#95502);
#83432=AXIS2_PLACEMENT_3D('',#191922,#95504,#95505);
#83433=AXIS2_PLACEMENT_3D('',#191923,#95506,#95507);
#83434=AXIS2_PLACEMENT_3D('',#191924,#95508,#95509);
#83435=AXIS2_PLACEMENT_3D('',#191928,#95511,#95512);
#83436=AXIS2_PLACEMENT_3D('',#191929,#95513,#95514);
#83437=AXIS2_PLACEMENT_3D('',#191930,#95515,#95516);
#83438=AXIS2_PLACEMENT_3D('',#191931,#95517,#95518);
#83439=AXIS2_PLACEMENT_3D('',#191932,#95519,#95520);
#83440=AXIS2_PLACEMENT_3D('',#191933,#95521,#95522);
#83441=AXIS2_PLACEMENT_3D('',#191938,#95524,#95525);
#83442=AXIS2_PLACEMENT_3D('',#191941,#95527,#95528);
#83443=AXIS2_PLACEMENT_3D('',#191942,#95529,#95530);
#83444=AXIS2_PLACEMENT_3D('',#191946,#95532,#95533);
#83445=AXIS2_PLACEMENT_3D('',#191947,#95534,#95535);
#83446=AXIS2_PLACEMENT_3D('',#191948,#95536,#95537);
#83447=AXIS2_PLACEMENT_3D('',#191952,#95539,#95540);
#83448=AXIS2_PLACEMENT_3D('',#191953,#95541,#95542);
#83449=AXIS2_PLACEMENT_3D('',#191954,#95543,#95544);
#83450=AXIS2_PLACEMENT_3D('',#191955,#95545,#95546);
#83451=AXIS2_PLACEMENT_3D('',#191956,#95547,#95548);
#83452=AXIS2_PLACEMENT_3D('',#191957,#95549,#95550);
#83453=AXIS2_PLACEMENT_3D('',#191962,#95552,#95553);
#83454=AXIS2_PLACEMENT_3D('',#191965,#95555,#95556);
#83455=AXIS2_PLACEMENT_3D('',#191966,#95557,#95558);
#83456=AXIS2_PLACEMENT_3D('',#191970,#95560,#95561);
#83457=AXIS2_PLACEMENT_3D('',#191971,#95562,#95563);
#83458=AXIS2_PLACEMENT_3D('',#191972,#95564,#95565);
#83459=AXIS2_PLACEMENT_3D('',#191976,#95567,#95568);
#83460=AXIS2_PLACEMENT_3D('',#191977,#95569,#95570);
#83461=AXIS2_PLACEMENT_3D('',#191978,#95571,#95572);
#83462=AXIS2_PLACEMENT_3D('',#191979,#95573,#95574);
#83463=AXIS2_PLACEMENT_3D('',#191980,#95575,#95576);
#83464=AXIS2_PLACEMENT_3D('',#191981,#95577,#95578);
#83465=AXIS2_PLACEMENT_3D('',#191986,#95580,#95581);
#83466=AXIS2_PLACEMENT_3D('',#191989,#95583,#95584);
#83467=AXIS2_PLACEMENT_3D('',#191990,#95585,#95586);
#83468=AXIS2_PLACEMENT_3D('',#191994,#95588,#95589);
#83469=AXIS2_PLACEMENT_3D('',#191995,#95590,#95591);
#83470=AXIS2_PLACEMENT_3D('',#191996,#95592,#95593);
#83471=AXIS2_PLACEMENT_3D('',#192000,#95595,#95596);
#83472=AXIS2_PLACEMENT_3D('',#192001,#95597,#95598);
#83473=AXIS2_PLACEMENT_3D('',#192002,#95599,#95600);
#83474=AXIS2_PLACEMENT_3D('',#192003,#95601,#95602);
#83475=AXIS2_PLACEMENT_3D('',#192004,#95603,#95604);
#83476=AXIS2_PLACEMENT_3D('',#192005,#95605,#95606);
#83477=AXIS2_PLACEMENT_3D('',#192010,#95608,#95609);
#83478=AXIS2_PLACEMENT_3D('',#192013,#95611,#95612);
#83479=AXIS2_PLACEMENT_3D('',#192014,#95613,#95614);
#83480=AXIS2_PLACEMENT_3D('',#192018,#95616,#95617);
#83481=AXIS2_PLACEMENT_3D('',#192019,#95618,#95619);
#83482=AXIS2_PLACEMENT_3D('',#192020,#95620,#95621);
#83483=AXIS2_PLACEMENT_3D('',#192024,#95623,#95624);
#83484=AXIS2_PLACEMENT_3D('',#192025,#95625,#95626);
#83485=AXIS2_PLACEMENT_3D('',#192026,#95627,#95628);
#83486=AXIS2_PLACEMENT_3D('',#192027,#95629,#95630);
#83487=AXIS2_PLACEMENT_3D('',#192028,#95631,#95632);
#83488=AXIS2_PLACEMENT_3D('',#192029,#95633,#95634);
#83489=AXIS2_PLACEMENT_3D('',#192034,#95636,#95637);
#83490=AXIS2_PLACEMENT_3D('',#192037,#95639,#95640);
#83491=AXIS2_PLACEMENT_3D('',#192038,#95641,#95642);
#83492=AXIS2_PLACEMENT_3D('',#192042,#95644,#95645);
#83493=AXIS2_PLACEMENT_3D('',#192043,#95646,#95647);
#83494=AXIS2_PLACEMENT_3D('',#192044,#95648,#95649);
#83495=AXIS2_PLACEMENT_3D('',#192048,#95651,#95652);
#83496=AXIS2_PLACEMENT_3D('',#192049,#95653,#95654);
#83497=AXIS2_PLACEMENT_3D('',#192050,#95655,#95656);
#83498=AXIS2_PLACEMENT_3D('',#192051,#95657,#95658);
#83499=AXIS2_PLACEMENT_3D('',#192052,#95659,#95660);
#83500=AXIS2_PLACEMENT_3D('',#192053,#95661,#95662);
#83501=AXIS2_PLACEMENT_3D('',#192058,#95664,#95665);
#83502=AXIS2_PLACEMENT_3D('',#192061,#95667,#95668);
#83503=AXIS2_PLACEMENT_3D('',#192062,#95669,#95670);
#83504=AXIS2_PLACEMENT_3D('',#192066,#95672,#95673);
#83505=AXIS2_PLACEMENT_3D('',#192067,#95674,#95675);
#83506=AXIS2_PLACEMENT_3D('',#192068,#95676,#95677);
#83507=AXIS2_PLACEMENT_3D('',#192072,#95679,#95680);
#83508=AXIS2_PLACEMENT_3D('',#192073,#95681,#95682);
#83509=AXIS2_PLACEMENT_3D('',#192074,#95683,#95684);
#83510=AXIS2_PLACEMENT_3D('',#192075,#95685,#95686);
#83511=AXIS2_PLACEMENT_3D('',#192076,#95687,#95688);
#83512=AXIS2_PLACEMENT_3D('',#192077,#95689,#95690);
#83513=AXIS2_PLACEMENT_3D('',#192082,#95692,#95693);
#83514=AXIS2_PLACEMENT_3D('',#192085,#95695,#95696);
#83515=AXIS2_PLACEMENT_3D('',#192086,#95697,#95698);
#83516=AXIS2_PLACEMENT_3D('',#192090,#95700,#95701);
#83517=AXIS2_PLACEMENT_3D('',#192091,#95702,#95703);
#83518=AXIS2_PLACEMENT_3D('',#192092,#95704,#95705);
#83519=AXIS2_PLACEMENT_3D('',#192096,#95707,#95708);
#83520=AXIS2_PLACEMENT_3D('',#192097,#95709,#95710);
#83521=AXIS2_PLACEMENT_3D('',#192098,#95711,#95712);
#83522=AXIS2_PLACEMENT_3D('',#192099,#95713,#95714);
#83523=AXIS2_PLACEMENT_3D('',#192100,#95715,#95716);
#83524=AXIS2_PLACEMENT_3D('',#192101,#95717,#95718);
#83525=AXIS2_PLACEMENT_3D('',#192106,#95720,#95721);
#83526=AXIS2_PLACEMENT_3D('',#192109,#95723,#95724);
#83527=AXIS2_PLACEMENT_3D('',#192110,#95725,#95726);
#83528=AXIS2_PLACEMENT_3D('',#192114,#95728,#95729);
#83529=AXIS2_PLACEMENT_3D('',#192115,#95730,#95731);
#83530=AXIS2_PLACEMENT_3D('',#192116,#95732,#95733);
#83531=AXIS2_PLACEMENT_3D('',#192120,#95735,#95736);
#83532=AXIS2_PLACEMENT_3D('',#192121,#95737,#95738);
#83533=AXIS2_PLACEMENT_3D('',#192122,#95739,#95740);
#83534=AXIS2_PLACEMENT_3D('',#192123,#95741,#95742);
#83535=AXIS2_PLACEMENT_3D('',#192124,#95743,#95744);
#83536=AXIS2_PLACEMENT_3D('',#192125,#95745,#95746);
#83537=AXIS2_PLACEMENT_3D('',#192130,#95748,#95749);
#83538=AXIS2_PLACEMENT_3D('',#192133,#95751,#95752);
#83539=AXIS2_PLACEMENT_3D('',#192134,#95753,#95754);
#83540=AXIS2_PLACEMENT_3D('',#192138,#95756,#95757);
#83541=AXIS2_PLACEMENT_3D('',#192139,#95758,#95759);
#83542=AXIS2_PLACEMENT_3D('',#192140,#95760,#95761);
#83543=AXIS2_PLACEMENT_3D('',#192144,#95763,#95764);
#83544=AXIS2_PLACEMENT_3D('',#192145,#95765,#95766);
#83545=AXIS2_PLACEMENT_3D('',#192146,#95767,#95768);
#83546=AXIS2_PLACEMENT_3D('',#192147,#95769,#95770);
#83547=AXIS2_PLACEMENT_3D('',#192148,#95771,#95772);
#83548=AXIS2_PLACEMENT_3D('',#192149,#95773,#95774);
#83549=AXIS2_PLACEMENT_3D('',#192154,#95776,#95777);
#83550=AXIS2_PLACEMENT_3D('',#192157,#95779,#95780);
#83551=AXIS2_PLACEMENT_3D('',#192158,#95781,#95782);
#83552=AXIS2_PLACEMENT_3D('',#192162,#95784,#95785);
#83553=AXIS2_PLACEMENT_3D('',#192163,#95786,#95787);
#83554=AXIS2_PLACEMENT_3D('',#192164,#95788,#95789);
#83555=AXIS2_PLACEMENT_3D('',#192168,#95791,#95792);
#83556=AXIS2_PLACEMENT_3D('',#192169,#95793,#95794);
#83557=AXIS2_PLACEMENT_3D('',#192170,#95795,#95796);
#83558=AXIS2_PLACEMENT_3D('',#192171,#95797,#95798);
#83559=AXIS2_PLACEMENT_3D('',#192172,#95799,#95800);
#83560=AXIS2_PLACEMENT_3D('',#192173,#95801,#95802);
#83561=AXIS2_PLACEMENT_3D('',#192178,#95804,#95805);
#83562=AXIS2_PLACEMENT_3D('',#192181,#95807,#95808);
#83563=AXIS2_PLACEMENT_3D('',#192182,#95809,#95810);
#83564=AXIS2_PLACEMENT_3D('',#192186,#95812,#95813);
#83565=AXIS2_PLACEMENT_3D('',#192187,#95814,#95815);
#83566=AXIS2_PLACEMENT_3D('',#192188,#95816,#95817);
#83567=AXIS2_PLACEMENT_3D('',#192192,#95819,#95820);
#83568=AXIS2_PLACEMENT_3D('',#192193,#95821,#95822);
#83569=AXIS2_PLACEMENT_3D('',#192194,#95823,#95824);
#83570=AXIS2_PLACEMENT_3D('',#192195,#95825,#95826);
#83571=AXIS2_PLACEMENT_3D('',#192196,#95827,#95828);
#83572=AXIS2_PLACEMENT_3D('',#192197,#95829,#95830);
#83573=AXIS2_PLACEMENT_3D('',#192202,#95832,#95833);
#83574=AXIS2_PLACEMENT_3D('',#192205,#95835,#95836);
#83575=AXIS2_PLACEMENT_3D('',#192206,#95837,#95838);
#83576=AXIS2_PLACEMENT_3D('',#192210,#95840,#95841);
#83577=AXIS2_PLACEMENT_3D('',#192211,#95842,#95843);
#83578=AXIS2_PLACEMENT_3D('',#192212,#95844,#95845);
#83579=AXIS2_PLACEMENT_3D('',#192216,#95847,#95848);
#83580=AXIS2_PLACEMENT_3D('',#192217,#95849,#95850);
#83581=AXIS2_PLACEMENT_3D('',#192218,#95851,#95852);
#83582=AXIS2_PLACEMENT_3D('',#192219,#95853,#95854);
#83583=AXIS2_PLACEMENT_3D('',#192220,#95855,#95856);
#83584=AXIS2_PLACEMENT_3D('',#192221,#95857,#95858);
#83585=AXIS2_PLACEMENT_3D('',#192226,#95860,#95861);
#83586=AXIS2_PLACEMENT_3D('',#192229,#95863,#95864);
#83587=AXIS2_PLACEMENT_3D('',#192230,#95865,#95866);
#83588=AXIS2_PLACEMENT_3D('',#192234,#95868,#95869);
#83589=AXIS2_PLACEMENT_3D('',#192235,#95870,#95871);
#83590=AXIS2_PLACEMENT_3D('',#192236,#95872,#95873);
#83591=AXIS2_PLACEMENT_3D('',#192240,#95875,#95876);
#83592=AXIS2_PLACEMENT_3D('',#192241,#95877,#95878);
#83593=AXIS2_PLACEMENT_3D('',#192242,#95879,#95880);
#83594=AXIS2_PLACEMENT_3D('',#192243,#95881,#95882);
#83595=AXIS2_PLACEMENT_3D('',#192244,#95883,#95884);
#83596=AXIS2_PLACEMENT_3D('',#192245,#95885,#95886);
#83597=AXIS2_PLACEMENT_3D('',#192250,#95888,#95889);
#83598=AXIS2_PLACEMENT_3D('',#192253,#95891,#95892);
#83599=AXIS2_PLACEMENT_3D('',#192254,#95893,#95894);
#83600=AXIS2_PLACEMENT_3D('',#192258,#95896,#95897);
#83601=AXIS2_PLACEMENT_3D('',#192259,#95898,#95899);
#83602=AXIS2_PLACEMENT_3D('',#192260,#95900,#95901);
#83603=AXIS2_PLACEMENT_3D('',#192264,#95903,#95904);
#83604=AXIS2_PLACEMENT_3D('',#192265,#95905,#95906);
#83605=AXIS2_PLACEMENT_3D('',#192266,#95907,#95908);
#83606=AXIS2_PLACEMENT_3D('',#192267,#95909,#95910);
#83607=AXIS2_PLACEMENT_3D('',#192268,#95911,#95912);
#83608=AXIS2_PLACEMENT_3D('',#192269,#95913,#95914);
#83609=AXIS2_PLACEMENT_3D('',#192274,#95916,#95917);
#83610=AXIS2_PLACEMENT_3D('',#192277,#95919,#95920);
#83611=AXIS2_PLACEMENT_3D('',#192278,#95921,#95922);
#83612=AXIS2_PLACEMENT_3D('',#192282,#95924,#95925);
#83613=AXIS2_PLACEMENT_3D('',#192283,#95926,#95927);
#83614=AXIS2_PLACEMENT_3D('',#192284,#95928,#95929);
#83615=AXIS2_PLACEMENT_3D('',#192288,#95931,#95932);
#83616=AXIS2_PLACEMENT_3D('',#192289,#95933,#95934);
#83617=AXIS2_PLACEMENT_3D('',#192290,#95935,#95936);
#83618=AXIS2_PLACEMENT_3D('',#192291,#95937,#95938);
#83619=AXIS2_PLACEMENT_3D('',#192292,#95939,#95940);
#83620=AXIS2_PLACEMENT_3D('',#192293,#95941,#95942);
#83621=AXIS2_PLACEMENT_3D('',#192298,#95944,#95945);
#83622=AXIS2_PLACEMENT_3D('',#192301,#95947,#95948);
#83623=AXIS2_PLACEMENT_3D('',#192302,#95949,#95950);
#83624=AXIS2_PLACEMENT_3D('',#192306,#95952,#95953);
#83625=AXIS2_PLACEMENT_3D('',#192307,#95954,#95955);
#83626=AXIS2_PLACEMENT_3D('',#192308,#95956,#95957);
#83627=AXIS2_PLACEMENT_3D('',#192312,#95959,#95960);
#83628=AXIS2_PLACEMENT_3D('',#192313,#95961,#95962);
#83629=AXIS2_PLACEMENT_3D('',#192314,#95963,#95964);
#83630=AXIS2_PLACEMENT_3D('',#192315,#95965,#95966);
#83631=AXIS2_PLACEMENT_3D('',#192316,#95967,#95968);
#83632=AXIS2_PLACEMENT_3D('',#192317,#95969,#95970);
#83633=AXIS2_PLACEMENT_3D('',#192322,#95972,#95973);
#83634=AXIS2_PLACEMENT_3D('',#192325,#95975,#95976);
#83635=AXIS2_PLACEMENT_3D('',#192326,#95977,#95978);
#83636=AXIS2_PLACEMENT_3D('',#192330,#95980,#95981);
#83637=AXIS2_PLACEMENT_3D('',#192331,#95982,#95983);
#83638=AXIS2_PLACEMENT_3D('',#192332,#95984,#95985);
#83639=AXIS2_PLACEMENT_3D('',#192336,#95987,#95988);
#83640=AXIS2_PLACEMENT_3D('',#192337,#95989,#95990);
#83641=AXIS2_PLACEMENT_3D('',#192338,#95991,#95992);
#83642=AXIS2_PLACEMENT_3D('',#192339,#95993,#95994);
#83643=AXIS2_PLACEMENT_3D('',#192340,#95995,#95996);
#83644=AXIS2_PLACEMENT_3D('',#192341,#95997,#95998);
#83645=AXIS2_PLACEMENT_3D('',#192346,#96000,#96001);
#83646=AXIS2_PLACEMENT_3D('',#192349,#96003,#96004);
#83647=AXIS2_PLACEMENT_3D('',#192350,#96005,#96006);
#83648=AXIS2_PLACEMENT_3D('',#192354,#96008,#96009);
#83649=AXIS2_PLACEMENT_3D('',#192355,#96010,#96011);
#83650=AXIS2_PLACEMENT_3D('',#192356,#96012,#96013);
#83651=AXIS2_PLACEMENT_3D('',#192360,#96015,#96016);
#83652=AXIS2_PLACEMENT_3D('',#192361,#96017,#96018);
#83653=AXIS2_PLACEMENT_3D('',#192362,#96019,#96020);
#83654=AXIS2_PLACEMENT_3D('',#192363,#96021,#96022);
#83655=AXIS2_PLACEMENT_3D('',#192364,#96023,#96024);
#83656=AXIS2_PLACEMENT_3D('',#192365,#96025,#96026);
#83657=AXIS2_PLACEMENT_3D('',#192370,#96028,#96029);
#83658=AXIS2_PLACEMENT_3D('',#192373,#96031,#96032);
#83659=AXIS2_PLACEMENT_3D('',#192374,#96033,#96034);
#83660=AXIS2_PLACEMENT_3D('',#192378,#96036,#96037);
#83661=AXIS2_PLACEMENT_3D('',#192379,#96038,#96039);
#83662=AXIS2_PLACEMENT_3D('',#192380,#96040,#96041);
#83663=AXIS2_PLACEMENT_3D('',#192384,#96043,#96044);
#83664=AXIS2_PLACEMENT_3D('',#192385,#96045,#96046);
#83665=AXIS2_PLACEMENT_3D('',#192386,#96047,#96048);
#83666=AXIS2_PLACEMENT_3D('',#192387,#96049,#96050);
#83667=AXIS2_PLACEMENT_3D('',#192388,#96051,#96052);
#83668=AXIS2_PLACEMENT_3D('',#192389,#96053,#96054);
#83669=AXIS2_PLACEMENT_3D('',#192394,#96056,#96057);
#83670=AXIS2_PLACEMENT_3D('',#192397,#96059,#96060);
#83671=AXIS2_PLACEMENT_3D('',#192398,#96061,#96062);
#83672=AXIS2_PLACEMENT_3D('',#192402,#96064,#96065);
#83673=AXIS2_PLACEMENT_3D('',#192403,#96066,#96067);
#83674=AXIS2_PLACEMENT_3D('',#192404,#96068,#96069);
#83675=AXIS2_PLACEMENT_3D('',#192408,#96071,#96072);
#83676=AXIS2_PLACEMENT_3D('',#192409,#96073,#96074);
#83677=AXIS2_PLACEMENT_3D('',#192410,#96075,#96076);
#83678=AXIS2_PLACEMENT_3D('',#192411,#96077,#96078);
#83679=AXIS2_PLACEMENT_3D('',#192412,#96079,#96080);
#83680=AXIS2_PLACEMENT_3D('',#192413,#96081,#96082);
#83681=AXIS2_PLACEMENT_3D('',#192418,#96084,#96085);
#83682=AXIS2_PLACEMENT_3D('',#192421,#96087,#96088);
#83683=AXIS2_PLACEMENT_3D('',#192422,#96089,#96090);
#83684=AXIS2_PLACEMENT_3D('',#192426,#96092,#96093);
#83685=AXIS2_PLACEMENT_3D('',#192427,#96094,#96095);
#83686=AXIS2_PLACEMENT_3D('',#192428,#96096,#96097);
#83687=AXIS2_PLACEMENT_3D('',#192432,#96099,#96100);
#83688=AXIS2_PLACEMENT_3D('',#192433,#96101,#96102);
#83689=AXIS2_PLACEMENT_3D('',#192434,#96103,#96104);
#83690=AXIS2_PLACEMENT_3D('',#192435,#96105,#96106);
#83691=AXIS2_PLACEMENT_3D('',#192436,#96107,#96108);
#83692=AXIS2_PLACEMENT_3D('',#192437,#96109,#96110);
#83693=AXIS2_PLACEMENT_3D('',#192442,#96112,#96113);
#83694=AXIS2_PLACEMENT_3D('',#192445,#96115,#96116);
#83695=AXIS2_PLACEMENT_3D('',#192446,#96117,#96118);
#83696=AXIS2_PLACEMENT_3D('',#192450,#96120,#96121);
#83697=AXIS2_PLACEMENT_3D('',#192451,#96122,#96123);
#83698=AXIS2_PLACEMENT_3D('',#192452,#96124,#96125);
#83699=AXIS2_PLACEMENT_3D('',#192456,#96127,#96128);
#83700=AXIS2_PLACEMENT_3D('',#192457,#96129,#96130);
#83701=AXIS2_PLACEMENT_3D('',#192458,#96131,#96132);
#83702=AXIS2_PLACEMENT_3D('',#192459,#96133,#96134);
#83703=AXIS2_PLACEMENT_3D('',#192460,#96135,#96136);
#83704=AXIS2_PLACEMENT_3D('',#192461,#96137,#96138);
#83705=AXIS2_PLACEMENT_3D('',#192466,#96140,#96141);
#83706=AXIS2_PLACEMENT_3D('',#192469,#96143,#96144);
#83707=AXIS2_PLACEMENT_3D('',#192470,#96145,#96146);
#83708=AXIS2_PLACEMENT_3D('',#192474,#96148,#96149);
#83709=AXIS2_PLACEMENT_3D('',#192475,#96150,#96151);
#83710=AXIS2_PLACEMENT_3D('',#192476,#96152,#96153);
#83711=AXIS2_PLACEMENT_3D('',#192480,#96155,#96156);
#83712=AXIS2_PLACEMENT_3D('',#192481,#96157,#96158);
#83713=AXIS2_PLACEMENT_3D('',#192482,#96159,#96160);
#83714=AXIS2_PLACEMENT_3D('',#192483,#96161,#96162);
#83715=AXIS2_PLACEMENT_3D('',#192484,#96163,#96164);
#83716=AXIS2_PLACEMENT_3D('',#192485,#96165,#96166);
#83717=AXIS2_PLACEMENT_3D('',#192490,#96168,#96169);
#83718=AXIS2_PLACEMENT_3D('',#192493,#96171,#96172);
#83719=AXIS2_PLACEMENT_3D('',#192494,#96173,#96174);
#83720=AXIS2_PLACEMENT_3D('',#192498,#96176,#96177);
#83721=AXIS2_PLACEMENT_3D('',#192499,#96178,#96179);
#83722=AXIS2_PLACEMENT_3D('',#192500,#96180,#96181);
#83723=AXIS2_PLACEMENT_3D('',#192504,#96183,#96184);
#83724=AXIS2_PLACEMENT_3D('',#192505,#96185,#96186);
#83725=AXIS2_PLACEMENT_3D('',#192506,#96187,#96188);
#83726=AXIS2_PLACEMENT_3D('',#192507,#96189,#96190);
#83727=AXIS2_PLACEMENT_3D('',#192508,#96191,#96192);
#83728=AXIS2_PLACEMENT_3D('',#192509,#96193,#96194);
#83729=AXIS2_PLACEMENT_3D('',#192514,#96196,#96197);
#83730=AXIS2_PLACEMENT_3D('',#192517,#96199,#96200);
#83731=AXIS2_PLACEMENT_3D('',#192518,#96201,#96202);
#83732=AXIS2_PLACEMENT_3D('',#192522,#96204,#96205);
#83733=AXIS2_PLACEMENT_3D('',#192523,#96206,#96207);
#83734=AXIS2_PLACEMENT_3D('',#192524,#96208,#96209);
#83735=AXIS2_PLACEMENT_3D('',#192528,#96211,#96212);
#83736=AXIS2_PLACEMENT_3D('',#192529,#96213,#96214);
#83737=AXIS2_PLACEMENT_3D('',#192530,#96215,#96216);
#83738=AXIS2_PLACEMENT_3D('',#192531,#96217,#96218);
#83739=AXIS2_PLACEMENT_3D('',#192532,#96219,#96220);
#83740=AXIS2_PLACEMENT_3D('',#192533,#96221,#96222);
#83741=AXIS2_PLACEMENT_3D('',#192538,#96224,#96225);
#83742=AXIS2_PLACEMENT_3D('',#192541,#96227,#96228);
#83743=AXIS2_PLACEMENT_3D('',#192542,#96229,#96230);
#83744=AXIS2_PLACEMENT_3D('',#192546,#96232,#96233);
#83745=AXIS2_PLACEMENT_3D('',#192547,#96234,#96235);
#83746=AXIS2_PLACEMENT_3D('',#192548,#96236,#96237);
#83747=AXIS2_PLACEMENT_3D('',#192552,#96239,#96240);
#83748=AXIS2_PLACEMENT_3D('',#192553,#96241,#96242);
#83749=AXIS2_PLACEMENT_3D('',#192554,#96243,#96244);
#83750=AXIS2_PLACEMENT_3D('',#192555,#96245,#96246);
#83751=AXIS2_PLACEMENT_3D('',#192556,#96247,#96248);
#83752=AXIS2_PLACEMENT_3D('',#192557,#96249,#96250);
#83753=AXIS2_PLACEMENT_3D('',#192562,#96252,#96253);
#83754=AXIS2_PLACEMENT_3D('',#192565,#96255,#96256);
#83755=AXIS2_PLACEMENT_3D('',#192566,#96257,#96258);
#83756=AXIS2_PLACEMENT_3D('',#192570,#96260,#96261);
#83757=AXIS2_PLACEMENT_3D('',#192571,#96262,#96263);
#83758=AXIS2_PLACEMENT_3D('',#192572,#96264,#96265);
#83759=AXIS2_PLACEMENT_3D('',#192576,#96267,#96268);
#83760=AXIS2_PLACEMENT_3D('',#192577,#96269,#96270);
#83761=AXIS2_PLACEMENT_3D('',#192578,#96271,#96272);
#83762=AXIS2_PLACEMENT_3D('',#192579,#96273,#96274);
#83763=AXIS2_PLACEMENT_3D('',#192580,#96275,#96276);
#83764=AXIS2_PLACEMENT_3D('',#192581,#96277,#96278);
#83765=AXIS2_PLACEMENT_3D('',#192586,#96280,#96281);
#83766=AXIS2_PLACEMENT_3D('',#192589,#96283,#96284);
#83767=AXIS2_PLACEMENT_3D('',#192590,#96285,#96286);
#83768=AXIS2_PLACEMENT_3D('',#192594,#96288,#96289);
#83769=AXIS2_PLACEMENT_3D('',#192595,#96290,#96291);
#83770=AXIS2_PLACEMENT_3D('',#192596,#96292,#96293);
#83771=AXIS2_PLACEMENT_3D('',#192600,#96295,#96296);
#83772=AXIS2_PLACEMENT_3D('',#192601,#96297,#96298);
#83773=AXIS2_PLACEMENT_3D('',#192602,#96299,#96300);
#83774=AXIS2_PLACEMENT_3D('',#192603,#96301,#96302);
#83775=AXIS2_PLACEMENT_3D('',#192604,#96303,#96304);
#83776=AXIS2_PLACEMENT_3D('',#192605,#96305,#96306);
#83777=AXIS2_PLACEMENT_3D('',#192610,#96308,#96309);
#83778=AXIS2_PLACEMENT_3D('',#192613,#96311,#96312);
#83779=AXIS2_PLACEMENT_3D('',#192614,#96313,#96314);
#83780=AXIS2_PLACEMENT_3D('',#192618,#96316,#96317);
#83781=AXIS2_PLACEMENT_3D('',#192619,#96318,#96319);
#83782=AXIS2_PLACEMENT_3D('',#192620,#96320,#96321);
#83783=AXIS2_PLACEMENT_3D('',#192624,#96323,#96324);
#83784=AXIS2_PLACEMENT_3D('',#192625,#96325,#96326);
#83785=AXIS2_PLACEMENT_3D('',#192626,#96327,#96328);
#83786=AXIS2_PLACEMENT_3D('',#192627,#96329,#96330);
#83787=AXIS2_PLACEMENT_3D('',#192628,#96331,#96332);
#83788=AXIS2_PLACEMENT_3D('',#192629,#96333,#96334);
#83789=AXIS2_PLACEMENT_3D('',#192634,#96336,#96337);
#83790=AXIS2_PLACEMENT_3D('',#192637,#96339,#96340);
#83791=AXIS2_PLACEMENT_3D('',#192638,#96341,#96342);
#83792=AXIS2_PLACEMENT_3D('',#192642,#96344,#96345);
#83793=AXIS2_PLACEMENT_3D('',#192643,#96346,#96347);
#83794=AXIS2_PLACEMENT_3D('',#192644,#96348,#96349);
#83795=AXIS2_PLACEMENT_3D('',#192648,#96351,#96352);
#83796=AXIS2_PLACEMENT_3D('',#192649,#96353,#96354);
#83797=AXIS2_PLACEMENT_3D('',#192650,#96355,#96356);
#83798=AXIS2_PLACEMENT_3D('',#192651,#96357,#96358);
#83799=AXIS2_PLACEMENT_3D('',#192652,#96359,#96360);
#83800=AXIS2_PLACEMENT_3D('',#192653,#96361,#96362);
#83801=AXIS2_PLACEMENT_3D('',#192658,#96364,#96365);
#83802=AXIS2_PLACEMENT_3D('',#192661,#96367,#96368);
#83803=AXIS2_PLACEMENT_3D('',#192662,#96369,#96370);
#83804=AXIS2_PLACEMENT_3D('',#192666,#96372,#96373);
#83805=AXIS2_PLACEMENT_3D('',#192667,#96374,#96375);
#83806=AXIS2_PLACEMENT_3D('',#192668,#96376,#96377);
#83807=AXIS2_PLACEMENT_3D('',#192672,#96379,#96380);
#83808=AXIS2_PLACEMENT_3D('',#192673,#96381,#96382);
#83809=AXIS2_PLACEMENT_3D('',#192674,#96383,#96384);
#83810=AXIS2_PLACEMENT_3D('',#192675,#96385,#96386);
#83811=AXIS2_PLACEMENT_3D('',#192676,#96387,#96388);
#83812=AXIS2_PLACEMENT_3D('',#192677,#96389,#96390);
#83813=AXIS2_PLACEMENT_3D('',#192682,#96392,#96393);
#83814=AXIS2_PLACEMENT_3D('',#192685,#96395,#96396);
#83815=AXIS2_PLACEMENT_3D('',#192686,#96397,#96398);
#83816=AXIS2_PLACEMENT_3D('',#192690,#96400,#96401);
#83817=AXIS2_PLACEMENT_3D('',#192691,#96402,#96403);
#83818=AXIS2_PLACEMENT_3D('',#192692,#96404,#96405);
#83819=AXIS2_PLACEMENT_3D('',#192696,#96407,#96408);
#83820=AXIS2_PLACEMENT_3D('',#192697,#96409,#96410);
#83821=AXIS2_PLACEMENT_3D('',#192698,#96411,#96412);
#83822=AXIS2_PLACEMENT_3D('',#192699,#96413,#96414);
#83823=AXIS2_PLACEMENT_3D('',#192700,#96415,#96416);
#83824=AXIS2_PLACEMENT_3D('',#192701,#96417,#96418);
#83825=AXIS2_PLACEMENT_3D('',#192706,#96420,#96421);
#83826=AXIS2_PLACEMENT_3D('',#192709,#96423,#96424);
#83827=AXIS2_PLACEMENT_3D('',#192710,#96425,#96426);
#83828=AXIS2_PLACEMENT_3D('',#192714,#96428,#96429);
#83829=AXIS2_PLACEMENT_3D('',#192715,#96430,#96431);
#83830=AXIS2_PLACEMENT_3D('',#192716,#96432,#96433);
#83831=AXIS2_PLACEMENT_3D('',#192720,#96435,#96436);
#83832=AXIS2_PLACEMENT_3D('',#192721,#96437,#96438);
#83833=AXIS2_PLACEMENT_3D('',#192722,#96439,#96440);
#83834=AXIS2_PLACEMENT_3D('',#192723,#96441,#96442);
#83835=AXIS2_PLACEMENT_3D('',#192724,#96443,#96444);
#83836=AXIS2_PLACEMENT_3D('',#192725,#96445,#96446);
#83837=AXIS2_PLACEMENT_3D('',#192730,#96448,#96449);
#83838=AXIS2_PLACEMENT_3D('',#192733,#96451,#96452);
#83839=AXIS2_PLACEMENT_3D('',#192734,#96453,#96454);
#83840=AXIS2_PLACEMENT_3D('',#192738,#96456,#96457);
#83841=AXIS2_PLACEMENT_3D('',#192739,#96458,#96459);
#83842=AXIS2_PLACEMENT_3D('',#192740,#96460,#96461);
#83843=AXIS2_PLACEMENT_3D('',#192744,#96463,#96464);
#83844=AXIS2_PLACEMENT_3D('',#192745,#96465,#96466);
#83845=AXIS2_PLACEMENT_3D('',#192746,#96467,#96468);
#83846=AXIS2_PLACEMENT_3D('',#192747,#96469,#96470);
#83847=AXIS2_PLACEMENT_3D('',#192748,#96471,#96472);
#83848=AXIS2_PLACEMENT_3D('',#192749,#96473,#96474);
#83849=AXIS2_PLACEMENT_3D('',#192754,#96476,#96477);
#83850=AXIS2_PLACEMENT_3D('',#192757,#96479,#96480);
#83851=AXIS2_PLACEMENT_3D('',#192758,#96481,#96482);
#83852=AXIS2_PLACEMENT_3D('',#192762,#96484,#96485);
#83853=AXIS2_PLACEMENT_3D('',#192763,#96486,#96487);
#83854=AXIS2_PLACEMENT_3D('',#192764,#96488,#96489);
#83855=AXIS2_PLACEMENT_3D('',#192768,#96491,#96492);
#83856=AXIS2_PLACEMENT_3D('',#192769,#96493,#96494);
#83857=AXIS2_PLACEMENT_3D('',#192770,#96495,#96496);
#83858=AXIS2_PLACEMENT_3D('',#192771,#96497,#96498);
#83859=AXIS2_PLACEMENT_3D('',#192772,#96499,#96500);
#83860=AXIS2_PLACEMENT_3D('',#192773,#96501,#96502);
#83861=AXIS2_PLACEMENT_3D('',#192778,#96504,#96505);
#83862=AXIS2_PLACEMENT_3D('',#192781,#96507,#96508);
#83863=AXIS2_PLACEMENT_3D('',#192782,#96509,#96510);
#83864=AXIS2_PLACEMENT_3D('',#192786,#96512,#96513);
#83865=AXIS2_PLACEMENT_3D('',#192787,#96514,#96515);
#83866=AXIS2_PLACEMENT_3D('',#192788,#96516,#96517);
#83867=AXIS2_PLACEMENT_3D('',#192792,#96519,#96520);
#83868=AXIS2_PLACEMENT_3D('',#192793,#96521,#96522);
#83869=AXIS2_PLACEMENT_3D('',#192794,#96523,#96524);
#83870=AXIS2_PLACEMENT_3D('',#192795,#96525,#96526);
#83871=AXIS2_PLACEMENT_3D('',#192796,#96527,#96528);
#83872=AXIS2_PLACEMENT_3D('',#192797,#96529,#96530);
#83873=AXIS2_PLACEMENT_3D('',#192802,#96532,#96533);
#83874=AXIS2_PLACEMENT_3D('',#192805,#96535,#96536);
#83875=AXIS2_PLACEMENT_3D('',#192806,#96537,#96538);
#83876=AXIS2_PLACEMENT_3D('',#192810,#96540,#96541);
#83877=AXIS2_PLACEMENT_3D('',#192811,#96542,#96543);
#83878=AXIS2_PLACEMENT_3D('',#192812,#96544,#96545);
#83879=AXIS2_PLACEMENT_3D('',#192816,#96547,#96548);
#83880=AXIS2_PLACEMENT_3D('',#192817,#96549,#96550);
#83881=AXIS2_PLACEMENT_3D('',#192818,#96551,#96552);
#83882=AXIS2_PLACEMENT_3D('',#192819,#96553,#96554);
#83883=AXIS2_PLACEMENT_3D('',#192820,#96555,#96556);
#83884=AXIS2_PLACEMENT_3D('',#192821,#96557,#96558);
#83885=AXIS2_PLACEMENT_3D('',#192826,#96560,#96561);
#83886=AXIS2_PLACEMENT_3D('',#192829,#96563,#96564);
#83887=AXIS2_PLACEMENT_3D('',#192830,#96565,#96566);
#83888=AXIS2_PLACEMENT_3D('',#192834,#96568,#96569);
#83889=AXIS2_PLACEMENT_3D('',#192835,#96570,#96571);
#83890=AXIS2_PLACEMENT_3D('',#192836,#96572,#96573);
#83891=AXIS2_PLACEMENT_3D('',#192840,#96575,#96576);
#83892=AXIS2_PLACEMENT_3D('',#192841,#96577,#96578);
#83893=AXIS2_PLACEMENT_3D('',#192842,#96579,#96580);
#83894=AXIS2_PLACEMENT_3D('',#192843,#96581,#96582);
#83895=AXIS2_PLACEMENT_3D('',#192844,#96583,#96584);
#83896=AXIS2_PLACEMENT_3D('',#192845,#96585,#96586);
#83897=AXIS2_PLACEMENT_3D('',#192850,#96588,#96589);
#83898=AXIS2_PLACEMENT_3D('',#192853,#96591,#96592);
#83899=AXIS2_PLACEMENT_3D('',#192854,#96593,#96594);
#83900=AXIS2_PLACEMENT_3D('',#192858,#96596,#96597);
#83901=AXIS2_PLACEMENT_3D('',#192859,#96598,#96599);
#83902=AXIS2_PLACEMENT_3D('',#192860,#96600,#96601);
#83903=AXIS2_PLACEMENT_3D('',#192864,#96603,#96604);
#83904=AXIS2_PLACEMENT_3D('',#192865,#96605,#96606);
#83905=AXIS2_PLACEMENT_3D('',#192866,#96607,#96608);
#83906=AXIS2_PLACEMENT_3D('',#192867,#96609,#96610);
#83907=AXIS2_PLACEMENT_3D('',#192868,#96611,#96612);
#83908=AXIS2_PLACEMENT_3D('',#192869,#96613,#96614);
#83909=AXIS2_PLACEMENT_3D('',#192874,#96616,#96617);
#83910=AXIS2_PLACEMENT_3D('',#192877,#96619,#96620);
#83911=AXIS2_PLACEMENT_3D('',#192878,#96621,#96622);
#83912=AXIS2_PLACEMENT_3D('',#192882,#96624,#96625);
#83913=AXIS2_PLACEMENT_3D('',#192883,#96626,#96627);
#83914=AXIS2_PLACEMENT_3D('',#192884,#96628,#96629);
#83915=AXIS2_PLACEMENT_3D('',#192888,#96631,#96632);
#83916=AXIS2_PLACEMENT_3D('',#192889,#96633,#96634);
#83917=AXIS2_PLACEMENT_3D('',#192890,#96635,#96636);
#83918=AXIS2_PLACEMENT_3D('',#192891,#96637,#96638);
#83919=AXIS2_PLACEMENT_3D('',#192892,#96639,#96640);
#83920=AXIS2_PLACEMENT_3D('',#192893,#96641,#96642);
#83921=AXIS2_PLACEMENT_3D('',#192898,#96644,#96645);
#83922=AXIS2_PLACEMENT_3D('',#192901,#96647,#96648);
#83923=AXIS2_PLACEMENT_3D('',#192902,#96649,#96650);
#83924=AXIS2_PLACEMENT_3D('',#192906,#96652,#96653);
#83925=AXIS2_PLACEMENT_3D('',#192907,#96654,#96655);
#83926=AXIS2_PLACEMENT_3D('',#192908,#96656,#96657);
#83927=AXIS2_PLACEMENT_3D('',#192912,#96659,#96660);
#83928=AXIS2_PLACEMENT_3D('',#192913,#96661,#96662);
#83929=AXIS2_PLACEMENT_3D('',#192914,#96663,#96664);
#83930=AXIS2_PLACEMENT_3D('',#192915,#96665,#96666);
#83931=AXIS2_PLACEMENT_3D('',#192916,#96667,#96668);
#83932=AXIS2_PLACEMENT_3D('',#192917,#96669,#96670);
#83933=AXIS2_PLACEMENT_3D('',#192922,#96672,#96673);
#83934=AXIS2_PLACEMENT_3D('',#192925,#96675,#96676);
#83935=AXIS2_PLACEMENT_3D('',#192926,#96677,#96678);
#83936=AXIS2_PLACEMENT_3D('',#192930,#96680,#96681);
#83937=AXIS2_PLACEMENT_3D('',#192931,#96682,#96683);
#83938=AXIS2_PLACEMENT_3D('',#192932,#96684,#96685);
#83939=AXIS2_PLACEMENT_3D('',#192936,#96687,#96688);
#83940=AXIS2_PLACEMENT_3D('',#192937,#96689,#96690);
#83941=AXIS2_PLACEMENT_3D('',#192938,#96691,#96692);
#83942=AXIS2_PLACEMENT_3D('',#192939,#96693,#96694);
#83943=AXIS2_PLACEMENT_3D('',#192940,#96695,#96696);
#83944=AXIS2_PLACEMENT_3D('',#192941,#96697,#96698);
#83945=AXIS2_PLACEMENT_3D('',#192946,#96700,#96701);
#83946=AXIS2_PLACEMENT_3D('',#192949,#96703,#96704);
#83947=AXIS2_PLACEMENT_3D('',#192950,#96705,#96706);
#83948=AXIS2_PLACEMENT_3D('',#192954,#96708,#96709);
#83949=AXIS2_PLACEMENT_3D('',#192955,#96710,#96711);
#83950=AXIS2_PLACEMENT_3D('',#192956,#96712,#96713);
#83951=AXIS2_PLACEMENT_3D('',#192960,#96715,#96716);
#83952=AXIS2_PLACEMENT_3D('',#192961,#96717,#96718);
#83953=AXIS2_PLACEMENT_3D('',#192962,#96719,#96720);
#83954=AXIS2_PLACEMENT_3D('',#192963,#96721,#96722);
#83955=AXIS2_PLACEMENT_3D('',#192964,#96723,#96724);
#83956=AXIS2_PLACEMENT_3D('',#192965,#96725,#96726);
#83957=AXIS2_PLACEMENT_3D('',#192970,#96728,#96729);
#83958=AXIS2_PLACEMENT_3D('',#192973,#96731,#96732);
#83959=AXIS2_PLACEMENT_3D('',#192974,#96733,#96734);
#83960=AXIS2_PLACEMENT_3D('',#192978,#96736,#96737);
#83961=AXIS2_PLACEMENT_3D('',#192979,#96738,#96739);
#83962=AXIS2_PLACEMENT_3D('',#192980,#96740,#96741);
#83963=AXIS2_PLACEMENT_3D('',#192984,#96743,#96744);
#83964=AXIS2_PLACEMENT_3D('',#192985,#96745,#96746);
#83965=AXIS2_PLACEMENT_3D('',#192986,#96747,#96748);
#83966=AXIS2_PLACEMENT_3D('',#192987,#96749,#96750);
#83967=AXIS2_PLACEMENT_3D('',#192988,#96751,#96752);
#83968=AXIS2_PLACEMENT_3D('',#192989,#96753,#96754);
#83969=AXIS2_PLACEMENT_3D('',#192994,#96756,#96757);
#83970=AXIS2_PLACEMENT_3D('',#192997,#96759,#96760);
#83971=AXIS2_PLACEMENT_3D('',#192998,#96761,#96762);
#83972=AXIS2_PLACEMENT_3D('',#193002,#96764,#96765);
#83973=AXIS2_PLACEMENT_3D('',#193003,#96766,#96767);
#83974=AXIS2_PLACEMENT_3D('',#193004,#96768,#96769);
#83975=AXIS2_PLACEMENT_3D('',#193008,#96771,#96772);
#83976=AXIS2_PLACEMENT_3D('',#193009,#96773,#96774);
#83977=AXIS2_PLACEMENT_3D('',#193010,#96775,#96776);
#83978=AXIS2_PLACEMENT_3D('',#193011,#96777,#96778);
#83979=AXIS2_PLACEMENT_3D('',#193012,#96779,#96780);
#83980=AXIS2_PLACEMENT_3D('',#193013,#96781,#96782);
#83981=AXIS2_PLACEMENT_3D('',#193018,#96784,#96785);
#83982=AXIS2_PLACEMENT_3D('',#193021,#96787,#96788);
#83983=AXIS2_PLACEMENT_3D('',#193022,#96789,#96790);
#83984=AXIS2_PLACEMENT_3D('',#193026,#96792,#96793);
#83985=AXIS2_PLACEMENT_3D('',#193027,#96794,#96795);
#83986=AXIS2_PLACEMENT_3D('',#193028,#96796,#96797);
#83987=AXIS2_PLACEMENT_3D('',#193032,#96799,#96800);
#83988=AXIS2_PLACEMENT_3D('',#193033,#96801,#96802);
#83989=AXIS2_PLACEMENT_3D('',#193034,#96803,#96804);
#83990=AXIS2_PLACEMENT_3D('',#193035,#96805,#96806);
#83991=AXIS2_PLACEMENT_3D('',#193036,#96807,#96808);
#83992=AXIS2_PLACEMENT_3D('',#193037,#96809,#96810);
#83993=AXIS2_PLACEMENT_3D('',#193042,#96812,#96813);
#83994=AXIS2_PLACEMENT_3D('',#193045,#96815,#96816);
#83995=AXIS2_PLACEMENT_3D('',#193046,#96817,#96818);
#83996=AXIS2_PLACEMENT_3D('',#193050,#96820,#96821);
#83997=AXIS2_PLACEMENT_3D('',#193051,#96822,#96823);
#83998=AXIS2_PLACEMENT_3D('',#193052,#96824,#96825);
#83999=AXIS2_PLACEMENT_3D('',#193056,#96827,#96828);
#84000=AXIS2_PLACEMENT_3D('',#193057,#96829,#96830);
#84001=AXIS2_PLACEMENT_3D('',#193058,#96831,#96832);
#84002=AXIS2_PLACEMENT_3D('',#193059,#96833,#96834);
#84003=AXIS2_PLACEMENT_3D('',#193060,#96835,#96836);
#84004=AXIS2_PLACEMENT_3D('',#193061,#96837,#96838);
#84005=AXIS2_PLACEMENT_3D('',#193066,#96840,#96841);
#84006=AXIS2_PLACEMENT_3D('',#193069,#96843,#96844);
#84007=AXIS2_PLACEMENT_3D('',#193070,#96845,#96846);
#84008=AXIS2_PLACEMENT_3D('',#193074,#96848,#96849);
#84009=AXIS2_PLACEMENT_3D('',#193075,#96850,#96851);
#84010=AXIS2_PLACEMENT_3D('',#193076,#96852,#96853);
#84011=AXIS2_PLACEMENT_3D('',#193080,#96855,#96856);
#84012=AXIS2_PLACEMENT_3D('',#193081,#96857,#96858);
#84013=AXIS2_PLACEMENT_3D('',#193082,#96859,#96860);
#84014=AXIS2_PLACEMENT_3D('',#193083,#96861,#96862);
#84015=AXIS2_PLACEMENT_3D('',#193084,#96863,#96864);
#84016=AXIS2_PLACEMENT_3D('',#193085,#96865,#96866);
#84017=AXIS2_PLACEMENT_3D('',#193090,#96868,#96869);
#84018=AXIS2_PLACEMENT_3D('',#193093,#96871,#96872);
#84019=AXIS2_PLACEMENT_3D('',#193094,#96873,#96874);
#84020=AXIS2_PLACEMENT_3D('',#193098,#96876,#96877);
#84021=AXIS2_PLACEMENT_3D('',#193099,#96878,#96879);
#84022=AXIS2_PLACEMENT_3D('',#193100,#96880,#96881);
#84023=AXIS2_PLACEMENT_3D('',#193104,#96883,#96884);
#84024=AXIS2_PLACEMENT_3D('',#193105,#96885,#96886);
#84025=AXIS2_PLACEMENT_3D('',#193106,#96887,#96888);
#84026=AXIS2_PLACEMENT_3D('',#193107,#96889,#96890);
#84027=AXIS2_PLACEMENT_3D('',#193108,#96891,#96892);
#84028=AXIS2_PLACEMENT_3D('',#193109,#96893,#96894);
#84029=AXIS2_PLACEMENT_3D('',#193114,#96896,#96897);
#84030=AXIS2_PLACEMENT_3D('',#193117,#96899,#96900);
#84031=AXIS2_PLACEMENT_3D('',#193118,#96901,#96902);
#84032=AXIS2_PLACEMENT_3D('',#193122,#96904,#96905);
#84033=AXIS2_PLACEMENT_3D('',#193123,#96906,#96907);
#84034=AXIS2_PLACEMENT_3D('',#193124,#96908,#96909);
#84035=AXIS2_PLACEMENT_3D('',#193128,#96911,#96912);
#84036=AXIS2_PLACEMENT_3D('',#193129,#96913,#96914);
#84037=AXIS2_PLACEMENT_3D('',#193130,#96915,#96916);
#84038=AXIS2_PLACEMENT_3D('',#193131,#96917,#96918);
#84039=AXIS2_PLACEMENT_3D('',#193132,#96919,#96920);
#84040=AXIS2_PLACEMENT_3D('',#193133,#96921,#96922);
#84041=AXIS2_PLACEMENT_3D('',#193138,#96924,#96925);
#84042=AXIS2_PLACEMENT_3D('',#193141,#96927,#96928);
#84043=AXIS2_PLACEMENT_3D('',#193142,#96929,#96930);
#84044=AXIS2_PLACEMENT_3D('',#193146,#96932,#96933);
#84045=AXIS2_PLACEMENT_3D('',#193147,#96934,#96935);
#84046=AXIS2_PLACEMENT_3D('',#193148,#96936,#96937);
#84047=AXIS2_PLACEMENT_3D('',#193152,#96939,#96940);
#84048=AXIS2_PLACEMENT_3D('',#193153,#96941,#96942);
#84049=AXIS2_PLACEMENT_3D('',#193154,#96943,#96944);
#84050=AXIS2_PLACEMENT_3D('',#193155,#96945,#96946);
#84051=AXIS2_PLACEMENT_3D('',#193156,#96947,#96948);
#84052=AXIS2_PLACEMENT_3D('',#193157,#96949,#96950);
#84053=AXIS2_PLACEMENT_3D('',#193162,#96952,#96953);
#84054=AXIS2_PLACEMENT_3D('',#193165,#96955,#96956);
#84055=AXIS2_PLACEMENT_3D('',#193166,#96957,#96958);
#84056=AXIS2_PLACEMENT_3D('',#193170,#96960,#96961);
#84057=AXIS2_PLACEMENT_3D('',#193171,#96962,#96963);
#84058=AXIS2_PLACEMENT_3D('',#193172,#96964,#96965);
#84059=AXIS2_PLACEMENT_3D('',#193176,#96967,#96968);
#84060=AXIS2_PLACEMENT_3D('',#193177,#96969,#96970);
#84061=AXIS2_PLACEMENT_3D('',#193178,#96971,#96972);
#84062=AXIS2_PLACEMENT_3D('',#193179,#96973,#96974);
#84063=AXIS2_PLACEMENT_3D('',#193180,#96975,#96976);
#84064=AXIS2_PLACEMENT_3D('',#193181,#96977,#96978);
#84065=AXIS2_PLACEMENT_3D('',#193186,#96980,#96981);
#84066=AXIS2_PLACEMENT_3D('',#193189,#96983,#96984);
#84067=AXIS2_PLACEMENT_3D('',#193190,#96985,#96986);
#84068=AXIS2_PLACEMENT_3D('',#193194,#96988,#96989);
#84069=AXIS2_PLACEMENT_3D('',#193195,#96990,#96991);
#84070=AXIS2_PLACEMENT_3D('',#193196,#96992,#96993);
#84071=AXIS2_PLACEMENT_3D('',#193200,#96995,#96996);
#84072=AXIS2_PLACEMENT_3D('',#193201,#96997,#96998);
#84073=AXIS2_PLACEMENT_3D('',#193202,#96999,#97000);
#84074=AXIS2_PLACEMENT_3D('',#193203,#97001,#97002);
#84075=AXIS2_PLACEMENT_3D('',#193204,#97003,#97004);
#84076=AXIS2_PLACEMENT_3D('',#193205,#97005,#97006);
#84077=AXIS2_PLACEMENT_3D('',#193210,#97008,#97009);
#84078=AXIS2_PLACEMENT_3D('',#193213,#97011,#97012);
#84079=AXIS2_PLACEMENT_3D('',#193214,#97013,#97014);
#84080=AXIS2_PLACEMENT_3D('',#193218,#97016,#97017);
#84081=AXIS2_PLACEMENT_3D('',#193219,#97018,#97019);
#84082=AXIS2_PLACEMENT_3D('',#193220,#97020,#97021);
#84083=AXIS2_PLACEMENT_3D('',#193224,#97023,#97024);
#84084=AXIS2_PLACEMENT_3D('',#193225,#97025,#97026);
#84085=AXIS2_PLACEMENT_3D('',#193226,#97027,#97028);
#84086=AXIS2_PLACEMENT_3D('',#193227,#97029,#97030);
#84087=AXIS2_PLACEMENT_3D('',#193228,#97031,#97032);
#84088=AXIS2_PLACEMENT_3D('',#193229,#97033,#97034);
#84089=AXIS2_PLACEMENT_3D('',#193234,#97036,#97037);
#84090=AXIS2_PLACEMENT_3D('',#193237,#97039,#97040);
#84091=AXIS2_PLACEMENT_3D('',#193238,#97041,#97042);
#84092=AXIS2_PLACEMENT_3D('',#193242,#97044,#97045);
#84093=AXIS2_PLACEMENT_3D('',#193243,#97046,#97047);
#84094=AXIS2_PLACEMENT_3D('',#193244,#97048,#97049);
#84095=AXIS2_PLACEMENT_3D('',#193248,#97051,#97052);
#84096=AXIS2_PLACEMENT_3D('',#193249,#97053,#97054);
#84097=AXIS2_PLACEMENT_3D('',#193250,#97055,#97056);
#84098=AXIS2_PLACEMENT_3D('',#193251,#97057,#97058);
#84099=AXIS2_PLACEMENT_3D('',#193252,#97059,#97060);
#84100=AXIS2_PLACEMENT_3D('',#193253,#97061,#97062);
#84101=AXIS2_PLACEMENT_3D('',#193258,#97064,#97065);
#84102=AXIS2_PLACEMENT_3D('',#193261,#97067,#97068);
#84103=AXIS2_PLACEMENT_3D('',#193262,#97069,#97070);
#84104=AXIS2_PLACEMENT_3D('',#193266,#97072,#97073);
#84105=AXIS2_PLACEMENT_3D('',#193267,#97074,#97075);
#84106=AXIS2_PLACEMENT_3D('',#193268,#97076,#97077);
#84107=AXIS2_PLACEMENT_3D('',#193272,#97079,#97080);
#84108=AXIS2_PLACEMENT_3D('',#193273,#97081,#97082);
#84109=AXIS2_PLACEMENT_3D('',#193274,#97083,#97084);
#84110=AXIS2_PLACEMENT_3D('',#193275,#97085,#97086);
#84111=AXIS2_PLACEMENT_3D('',#193276,#97087,#97088);
#84112=AXIS2_PLACEMENT_3D('',#193277,#97089,#97090);
#84113=AXIS2_PLACEMENT_3D('',#193282,#97092,#97093);
#84114=AXIS2_PLACEMENT_3D('',#193285,#97095,#97096);
#84115=AXIS2_PLACEMENT_3D('',#193286,#97097,#97098);
#84116=AXIS2_PLACEMENT_3D('',#193290,#97100,#97101);
#84117=AXIS2_PLACEMENT_3D('',#193291,#97102,#97103);
#84118=AXIS2_PLACEMENT_3D('',#193292,#97104,#97105);
#84119=AXIS2_PLACEMENT_3D('',#193296,#97107,#97108);
#84120=AXIS2_PLACEMENT_3D('',#193297,#97109,#97110);
#84121=AXIS2_PLACEMENT_3D('',#193298,#97111,#97112);
#84122=AXIS2_PLACEMENT_3D('',#193299,#97113,#97114);
#84123=AXIS2_PLACEMENT_3D('',#193300,#97115,#97116);
#84124=AXIS2_PLACEMENT_3D('',#193301,#97117,#97118);
#84125=AXIS2_PLACEMENT_3D('',#193306,#97120,#97121);
#84126=AXIS2_PLACEMENT_3D('',#193309,#97123,#97124);
#84127=AXIS2_PLACEMENT_3D('',#193310,#97125,#97126);
#84128=AXIS2_PLACEMENT_3D('',#193314,#97128,#97129);
#84129=AXIS2_PLACEMENT_3D('',#193315,#97130,#97131);
#84130=AXIS2_PLACEMENT_3D('',#193316,#97132,#97133);
#84131=AXIS2_PLACEMENT_3D('',#193320,#97135,#97136);
#84132=AXIS2_PLACEMENT_3D('',#193321,#97137,#97138);
#84133=AXIS2_PLACEMENT_3D('',#193322,#97139,#97140);
#84134=AXIS2_PLACEMENT_3D('',#193323,#97141,#97142);
#84135=AXIS2_PLACEMENT_3D('',#193324,#97143,#97144);
#84136=AXIS2_PLACEMENT_3D('',#193325,#97145,#97146);
#84137=AXIS2_PLACEMENT_3D('',#193330,#97148,#97149);
#84138=AXIS2_PLACEMENT_3D('',#193333,#97151,#97152);
#84139=AXIS2_PLACEMENT_3D('',#193334,#97153,#97154);
#84140=AXIS2_PLACEMENT_3D('',#193338,#97156,#97157);
#84141=AXIS2_PLACEMENT_3D('',#193339,#97158,#97159);
#84142=AXIS2_PLACEMENT_3D('',#193340,#97160,#97161);
#84143=AXIS2_PLACEMENT_3D('',#193344,#97163,#97164);
#84144=AXIS2_PLACEMENT_3D('',#193345,#97165,#97166);
#84145=AXIS2_PLACEMENT_3D('',#193346,#97167,#97168);
#84146=AXIS2_PLACEMENT_3D('',#193347,#97169,#97170);
#84147=AXIS2_PLACEMENT_3D('',#193348,#97171,#97172);
#84148=AXIS2_PLACEMENT_3D('',#193349,#97173,#97174);
#84149=AXIS2_PLACEMENT_3D('',#193354,#97176,#97177);
#84150=AXIS2_PLACEMENT_3D('',#193357,#97179,#97180);
#84151=AXIS2_PLACEMENT_3D('',#193358,#97181,#97182);
#84152=AXIS2_PLACEMENT_3D('',#193362,#97184,#97185);
#84153=AXIS2_PLACEMENT_3D('',#193363,#97186,#97187);
#84154=AXIS2_PLACEMENT_3D('',#193364,#97188,#97189);
#84155=AXIS2_PLACEMENT_3D('',#193368,#97191,#97192);
#84156=AXIS2_PLACEMENT_3D('',#193369,#97193,#97194);
#84157=AXIS2_PLACEMENT_3D('',#193370,#97195,#97196);
#84158=AXIS2_PLACEMENT_3D('',#193371,#97197,#97198);
#84159=AXIS2_PLACEMENT_3D('',#193372,#97199,#97200);
#84160=AXIS2_PLACEMENT_3D('',#193373,#97201,#97202);
#84161=AXIS2_PLACEMENT_3D('',#193378,#97204,#97205);
#84162=AXIS2_PLACEMENT_3D('',#193381,#97207,#97208);
#84163=AXIS2_PLACEMENT_3D('',#193382,#97209,#97210);
#84164=AXIS2_PLACEMENT_3D('',#193386,#97212,#97213);
#84165=AXIS2_PLACEMENT_3D('',#193387,#97214,#97215);
#84166=AXIS2_PLACEMENT_3D('',#193388,#97216,#97217);
#84167=AXIS2_PLACEMENT_3D('',#193392,#97219,#97220);
#84168=AXIS2_PLACEMENT_3D('',#193393,#97221,#97222);
#84169=AXIS2_PLACEMENT_3D('',#193394,#97223,#97224);
#84170=AXIS2_PLACEMENT_3D('',#193395,#97225,#97226);
#84171=AXIS2_PLACEMENT_3D('',#193396,#97227,#97228);
#84172=AXIS2_PLACEMENT_3D('',#193397,#97229,#97230);
#84173=AXIS2_PLACEMENT_3D('',#193402,#97232,#97233);
#84174=AXIS2_PLACEMENT_3D('',#193405,#97235,#97236);
#84175=AXIS2_PLACEMENT_3D('',#193406,#97237,#97238);
#84176=AXIS2_PLACEMENT_3D('',#193410,#97240,#97241);
#84177=AXIS2_PLACEMENT_3D('',#193411,#97242,#97243);
#84178=AXIS2_PLACEMENT_3D('',#193412,#97244,#97245);
#84179=AXIS2_PLACEMENT_3D('',#193416,#97247,#97248);
#84180=AXIS2_PLACEMENT_3D('',#193417,#97249,#97250);
#84181=AXIS2_PLACEMENT_3D('',#193418,#97251,#97252);
#84182=AXIS2_PLACEMENT_3D('',#193419,#97253,#97254);
#84183=AXIS2_PLACEMENT_3D('',#193420,#97255,#97256);
#84184=AXIS2_PLACEMENT_3D('',#193421,#97257,#97258);
#84185=AXIS2_PLACEMENT_3D('',#193422,#97259,#97260);
#84186=AXIS2_PLACEMENT_3D('',#193431,#97265,#97266);
#84187=AXIS2_PLACEMENT_3D('',#193437,#97270,#97271);
#84188=AXIS2_PLACEMENT_3D('',#193443,#97275,#97276);
#84189=AXIS2_PLACEMENT_3D('',#193446,#97279,#97280);
#84190=AXIS2_PLACEMENT_3D('',#193455,#97285,#97286);
#84191=AXIS2_PLACEMENT_3D('',#193461,#97290,#97291);
#84192=AXIS2_PLACEMENT_3D('',#193467,#97295,#97296);
#84193=AXIS2_PLACEMENT_3D('',#193470,#97299,#97300);
#84194=AXIS2_PLACEMENT_3D('',#193479,#97305,#97306);
#84195=AXIS2_PLACEMENT_3D('',#193485,#97310,#97311);
#84196=AXIS2_PLACEMENT_3D('',#193491,#97315,#97316);
#84197=AXIS2_PLACEMENT_3D('',#193494,#97319,#97320);
#84198=AXIS2_PLACEMENT_3D('',#193503,#97325,#97326);
#84199=AXIS2_PLACEMENT_3D('',#193509,#97330,#97331);
#84200=AXIS2_PLACEMENT_3D('',#193515,#97335,#97336);
#84201=AXIS2_PLACEMENT_3D('',#193518,#97339,#97340);
#84202=AXIS2_PLACEMENT_3D('',#193527,#97345,#97346);
#84203=AXIS2_PLACEMENT_3D('',#193533,#97350,#97351);
#84204=AXIS2_PLACEMENT_3D('',#193539,#97355,#97356);
#84205=AXIS2_PLACEMENT_3D('',#193542,#97359,#97360);
#84206=AXIS2_PLACEMENT_3D('',#193551,#97365,#97366);
#84207=AXIS2_PLACEMENT_3D('',#193557,#97370,#97371);
#84208=AXIS2_PLACEMENT_3D('',#193563,#97375,#97376);
#84209=AXIS2_PLACEMENT_3D('',#193566,#97379,#97380);
#84210=AXIS2_PLACEMENT_3D('',#193575,#97385,#97386);
#84211=AXIS2_PLACEMENT_3D('',#193581,#97390,#97391);
#84212=AXIS2_PLACEMENT_3D('',#193587,#97395,#97396);
#84213=AXIS2_PLACEMENT_3D('',#193590,#97399,#97400);
#84214=AXIS2_PLACEMENT_3D('',#193599,#97405,#97406);
#84215=AXIS2_PLACEMENT_3D('',#193605,#97410,#97411);
#84216=AXIS2_PLACEMENT_3D('',#193611,#97415,#97416);
#84217=AXIS2_PLACEMENT_3D('',#193614,#97419,#97420);
#84218=AXIS2_PLACEMENT_3D('',#193623,#97425,#97426);
#84219=AXIS2_PLACEMENT_3D('',#193629,#97430,#97431);
#84220=AXIS2_PLACEMENT_3D('',#193635,#97435,#97436);
#84221=AXIS2_PLACEMENT_3D('',#193638,#97439,#97440);
#84222=AXIS2_PLACEMENT_3D('',#193647,#97445,#97446);
#84223=AXIS2_PLACEMENT_3D('',#193653,#97450,#97451);
#84224=AXIS2_PLACEMENT_3D('',#193659,#97455,#97456);
#84225=AXIS2_PLACEMENT_3D('',#193662,#97459,#97460);
#84226=AXIS2_PLACEMENT_3D('',#193671,#97465,#97466);
#84227=AXIS2_PLACEMENT_3D('',#193677,#97470,#97471);
#84228=AXIS2_PLACEMENT_3D('',#193683,#97475,#97476);
#84229=AXIS2_PLACEMENT_3D('',#193686,#97479,#97480);
#84230=AXIS2_PLACEMENT_3D('',#193695,#97485,#97486);
#84231=AXIS2_PLACEMENT_3D('',#193701,#97490,#97491);
#84232=AXIS2_PLACEMENT_3D('',#193707,#97495,#97496);
#84233=AXIS2_PLACEMENT_3D('',#193710,#97499,#97500);
#84234=AXIS2_PLACEMENT_3D('',#193719,#97505,#97506);
#84235=AXIS2_PLACEMENT_3D('',#193725,#97510,#97511);
#84236=AXIS2_PLACEMENT_3D('',#193731,#97515,#97516);
#84237=AXIS2_PLACEMENT_3D('',#193734,#97519,#97520);
#84238=AXIS2_PLACEMENT_3D('',#193743,#97525,#97526);
#84239=AXIS2_PLACEMENT_3D('',#193749,#97530,#97531);
#84240=AXIS2_PLACEMENT_3D('',#193755,#97535,#97536);
#84241=AXIS2_PLACEMENT_3D('',#193758,#97539,#97540);
#84242=AXIS2_PLACEMENT_3D('',#193767,#97545,#97546);
#84243=AXIS2_PLACEMENT_3D('',#193773,#97550,#97551);
#84244=AXIS2_PLACEMENT_3D('',#193779,#97555,#97556);
#84245=AXIS2_PLACEMENT_3D('',#193782,#97559,#97560);
#84246=AXIS2_PLACEMENT_3D('',#193791,#97565,#97566);
#84247=AXIS2_PLACEMENT_3D('',#193797,#97570,#97571);
#84248=AXIS2_PLACEMENT_3D('',#193803,#97575,#97576);
#84249=AXIS2_PLACEMENT_3D('',#193806,#97579,#97580);
#84250=AXIS2_PLACEMENT_3D('',#193815,#97585,#97586);
#84251=AXIS2_PLACEMENT_3D('',#193821,#97590,#97591);
#84252=AXIS2_PLACEMENT_3D('',#193827,#97595,#97596);
#84253=AXIS2_PLACEMENT_3D('',#193830,#97599,#97600);
#84254=AXIS2_PLACEMENT_3D('',#193839,#97605,#97606);
#84255=AXIS2_PLACEMENT_3D('',#193845,#97610,#97611);
#84256=AXIS2_PLACEMENT_3D('',#193851,#97615,#97616);
#84257=AXIS2_PLACEMENT_3D('',#193854,#97619,#97620);
#84258=AXIS2_PLACEMENT_3D('',#193863,#97625,#97626);
#84259=AXIS2_PLACEMENT_3D('',#193869,#97630,#97631);
#84260=AXIS2_PLACEMENT_3D('',#193875,#97635,#97636);
#84261=AXIS2_PLACEMENT_3D('',#193878,#97639,#97640);
#84262=AXIS2_PLACEMENT_3D('',#193887,#97645,#97646);
#84263=AXIS2_PLACEMENT_3D('',#193893,#97650,#97651);
#84264=AXIS2_PLACEMENT_3D('',#193899,#97655,#97656);
#84265=AXIS2_PLACEMENT_3D('',#193902,#97659,#97660);
#84266=AXIS2_PLACEMENT_3D('',#193911,#97665,#97666);
#84267=AXIS2_PLACEMENT_3D('',#193917,#97670,#97671);
#84268=AXIS2_PLACEMENT_3D('',#193923,#97675,#97676);
#84269=AXIS2_PLACEMENT_3D('',#193926,#97679,#97680);
#84270=AXIS2_PLACEMENT_3D('',#193935,#97685,#97686);
#84271=AXIS2_PLACEMENT_3D('',#193941,#97690,#97691);
#84272=AXIS2_PLACEMENT_3D('',#193947,#97695,#97696);
#84273=AXIS2_PLACEMENT_3D('',#193950,#97699,#97700);
#84274=AXIS2_PLACEMENT_3D('',#193959,#97705,#97706);
#84275=AXIS2_PLACEMENT_3D('',#193965,#97710,#97711);
#84276=AXIS2_PLACEMENT_3D('',#193971,#97715,#97716);
#84277=AXIS2_PLACEMENT_3D('',#193974,#97719,#97720);
#84278=AXIS2_PLACEMENT_3D('',#193983,#97725,#97726);
#84279=AXIS2_PLACEMENT_3D('',#193989,#97730,#97731);
#84280=AXIS2_PLACEMENT_3D('',#193995,#97735,#97736);
#84281=AXIS2_PLACEMENT_3D('',#193998,#97739,#97740);
#84282=AXIS2_PLACEMENT_3D('',#194007,#97745,#97746);
#84283=AXIS2_PLACEMENT_3D('',#194013,#97750,#97751);
#84284=AXIS2_PLACEMENT_3D('',#194019,#97755,#97756);
#84285=AXIS2_PLACEMENT_3D('',#194022,#97759,#97760);
#84286=AXIS2_PLACEMENT_3D('',#194031,#97765,#97766);
#84287=AXIS2_PLACEMENT_3D('',#194037,#97770,#97771);
#84288=AXIS2_PLACEMENT_3D('',#194043,#97775,#97776);
#84289=AXIS2_PLACEMENT_3D('',#194046,#97779,#97780);
#84290=AXIS2_PLACEMENT_3D('',#194055,#97785,#97786);
#84291=AXIS2_PLACEMENT_3D('',#194061,#97790,#97791);
#84292=AXIS2_PLACEMENT_3D('',#194067,#97795,#97796);
#84293=AXIS2_PLACEMENT_3D('',#194070,#97799,#97800);
#84294=AXIS2_PLACEMENT_3D('',#194079,#97805,#97806);
#84295=AXIS2_PLACEMENT_3D('',#194085,#97810,#97811);
#84296=AXIS2_PLACEMENT_3D('',#194091,#97815,#97816);
#84297=AXIS2_PLACEMENT_3D('',#194094,#97819,#97820);
#84298=AXIS2_PLACEMENT_3D('',#194103,#97825,#97826);
#84299=AXIS2_PLACEMENT_3D('',#194109,#97830,#97831);
#84300=AXIS2_PLACEMENT_3D('',#194115,#97835,#97836);
#84301=AXIS2_PLACEMENT_3D('',#194118,#97839,#97840);
#84302=AXIS2_PLACEMENT_3D('',#194127,#97845,#97846);
#84303=AXIS2_PLACEMENT_3D('',#194133,#97850,#97851);
#84304=AXIS2_PLACEMENT_3D('',#194139,#97855,#97856);
#84305=AXIS2_PLACEMENT_3D('',#194142,#97859,#97860);
#84306=AXIS2_PLACEMENT_3D('',#194151,#97865,#97866);
#84307=AXIS2_PLACEMENT_3D('',#194157,#97870,#97871);
#84308=AXIS2_PLACEMENT_3D('',#194163,#97875,#97876);
#84309=AXIS2_PLACEMENT_3D('',#194166,#97879,#97880);
#84310=AXIS2_PLACEMENT_3D('',#194175,#97885,#97886);
#84311=AXIS2_PLACEMENT_3D('',#194181,#97890,#97891);
#84312=AXIS2_PLACEMENT_3D('',#194187,#97895,#97896);
#84313=AXIS2_PLACEMENT_3D('',#194190,#97899,#97900);
#84314=AXIS2_PLACEMENT_3D('',#194199,#97905,#97906);
#84315=AXIS2_PLACEMENT_3D('',#194205,#97910,#97911);
#84316=AXIS2_PLACEMENT_3D('',#194211,#97915,#97916);
#84317=AXIS2_PLACEMENT_3D('',#194214,#97919,#97920);
#84318=AXIS2_PLACEMENT_3D('',#194223,#97925,#97926);
#84319=AXIS2_PLACEMENT_3D('',#194229,#97930,#97931);
#84320=AXIS2_PLACEMENT_3D('',#194235,#97935,#97936);
#84321=AXIS2_PLACEMENT_3D('',#194238,#97939,#97940);
#84322=AXIS2_PLACEMENT_3D('',#194247,#97945,#97946);
#84323=AXIS2_PLACEMENT_3D('',#194253,#97950,#97951);
#84324=AXIS2_PLACEMENT_3D('',#194259,#97955,#97956);
#84325=AXIS2_PLACEMENT_3D('',#194262,#97959,#97960);
#84326=AXIS2_PLACEMENT_3D('',#194271,#97965,#97966);
#84327=AXIS2_PLACEMENT_3D('',#194277,#97970,#97971);
#84328=AXIS2_PLACEMENT_3D('',#194283,#97975,#97976);
#84329=AXIS2_PLACEMENT_3D('',#194286,#97979,#97980);
#84330=AXIS2_PLACEMENT_3D('',#194295,#97985,#97986);
#84331=AXIS2_PLACEMENT_3D('',#194301,#97990,#97991);
#84332=AXIS2_PLACEMENT_3D('',#194307,#97995,#97996);
#84333=AXIS2_PLACEMENT_3D('',#194310,#97999,#98000);
#84334=AXIS2_PLACEMENT_3D('',#194319,#98005,#98006);
#84335=AXIS2_PLACEMENT_3D('',#194325,#98010,#98011);
#84336=AXIS2_PLACEMENT_3D('',#194331,#98015,#98016);
#84337=AXIS2_PLACEMENT_3D('',#194334,#98019,#98020);
#84338=AXIS2_PLACEMENT_3D('',#194343,#98025,#98026);
#84339=AXIS2_PLACEMENT_3D('',#194349,#98030,#98031);
#84340=AXIS2_PLACEMENT_3D('',#194355,#98035,#98036);
#84341=AXIS2_PLACEMENT_3D('',#194358,#98039,#98040);
#84342=AXIS2_PLACEMENT_3D('',#194367,#98045,#98046);
#84343=AXIS2_PLACEMENT_3D('',#194373,#98050,#98051);
#84344=AXIS2_PLACEMENT_3D('',#194379,#98055,#98056);
#84345=AXIS2_PLACEMENT_3D('',#194382,#98059,#98060);
#84346=AXIS2_PLACEMENT_3D('',#194391,#98065,#98066);
#84347=AXIS2_PLACEMENT_3D('',#194397,#98070,#98071);
#84348=AXIS2_PLACEMENT_3D('',#194403,#98075,#98076);
#84349=AXIS2_PLACEMENT_3D('',#194406,#98079,#98080);
#84350=AXIS2_PLACEMENT_3D('',#194415,#98085,#98086);
#84351=AXIS2_PLACEMENT_3D('',#194421,#98090,#98091);
#84352=AXIS2_PLACEMENT_3D('',#194427,#98095,#98096);
#84353=AXIS2_PLACEMENT_3D('',#194430,#98099,#98100);
#84354=AXIS2_PLACEMENT_3D('',#194439,#98105,#98106);
#84355=AXIS2_PLACEMENT_3D('',#194445,#98110,#98111);
#84356=AXIS2_PLACEMENT_3D('',#194451,#98115,#98116);
#84357=AXIS2_PLACEMENT_3D('',#194454,#98119,#98120);
#84358=AXIS2_PLACEMENT_3D('',#194463,#98125,#98126);
#84359=AXIS2_PLACEMENT_3D('',#194469,#98130,#98131);
#84360=AXIS2_PLACEMENT_3D('',#194475,#98135,#98136);
#84361=AXIS2_PLACEMENT_3D('',#194478,#98139,#98140);
#84362=AXIS2_PLACEMENT_3D('',#194487,#98145,#98146);
#84363=AXIS2_PLACEMENT_3D('',#194493,#98150,#98151);
#84364=AXIS2_PLACEMENT_3D('',#194499,#98155,#98156);
#84365=AXIS2_PLACEMENT_3D('',#194502,#98159,#98160);
#84366=AXIS2_PLACEMENT_3D('',#194511,#98165,#98166);
#84367=AXIS2_PLACEMENT_3D('',#194517,#98170,#98171);
#84368=AXIS2_PLACEMENT_3D('',#194523,#98175,#98176);
#84369=AXIS2_PLACEMENT_3D('',#194526,#98179,#98180);
#84370=AXIS2_PLACEMENT_3D('',#194535,#98185,#98186);
#84371=AXIS2_PLACEMENT_3D('',#194541,#98190,#98191);
#84372=AXIS2_PLACEMENT_3D('',#194547,#98195,#98196);
#84373=AXIS2_PLACEMENT_3D('',#194550,#98199,#98200);
#84374=AXIS2_PLACEMENT_3D('',#194559,#98205,#98206);
#84375=AXIS2_PLACEMENT_3D('',#194565,#98210,#98211);
#84376=AXIS2_PLACEMENT_3D('',#194571,#98215,#98216);
#84377=AXIS2_PLACEMENT_3D('',#194574,#98219,#98220);
#84378=AXIS2_PLACEMENT_3D('',#194583,#98225,#98226);
#84379=AXIS2_PLACEMENT_3D('',#194589,#98230,#98231);
#84380=AXIS2_PLACEMENT_3D('',#194595,#98235,#98236);
#84381=AXIS2_PLACEMENT_3D('',#194598,#98239,#98240);
#84382=AXIS2_PLACEMENT_3D('',#194607,#98245,#98246);
#84383=AXIS2_PLACEMENT_3D('',#194613,#98250,#98251);
#84384=AXIS2_PLACEMENT_3D('',#194619,#98255,#98256);
#84385=AXIS2_PLACEMENT_3D('',#194622,#98259,#98260);
#84386=AXIS2_PLACEMENT_3D('',#194631,#98265,#98266);
#84387=AXIS2_PLACEMENT_3D('',#194637,#98270,#98271);
#84388=AXIS2_PLACEMENT_3D('',#194643,#98275,#98276);
#84389=AXIS2_PLACEMENT_3D('',#194646,#98279,#98280);
#84390=AXIS2_PLACEMENT_3D('',#194655,#98285,#98286);
#84391=AXIS2_PLACEMENT_3D('',#194661,#98290,#98291);
#84392=AXIS2_PLACEMENT_3D('',#194667,#98295,#98296);
#84393=AXIS2_PLACEMENT_3D('',#194670,#98299,#98300);
#84394=AXIS2_PLACEMENT_3D('',#194679,#98305,#98306);
#84395=AXIS2_PLACEMENT_3D('',#194685,#98310,#98311);
#84396=AXIS2_PLACEMENT_3D('',#194691,#98315,#98316);
#84397=AXIS2_PLACEMENT_3D('',#194694,#98319,#98320);
#84398=AXIS2_PLACEMENT_3D('',#194703,#98325,#98326);
#84399=AXIS2_PLACEMENT_3D('',#194709,#98330,#98331);
#84400=AXIS2_PLACEMENT_3D('',#194715,#98335,#98336);
#84401=AXIS2_PLACEMENT_3D('',#194718,#98339,#98340);
#84402=AXIS2_PLACEMENT_3D('',#194727,#98345,#98346);
#84403=AXIS2_PLACEMENT_3D('',#194733,#98350,#98351);
#84404=AXIS2_PLACEMENT_3D('',#194739,#98355,#98356);
#84405=AXIS2_PLACEMENT_3D('',#194742,#98359,#98360);
#84406=AXIS2_PLACEMENT_3D('',#194751,#98365,#98366);
#84407=AXIS2_PLACEMENT_3D('',#194757,#98370,#98371);
#84408=AXIS2_PLACEMENT_3D('',#194763,#98375,#98376);
#84409=AXIS2_PLACEMENT_3D('',#194766,#98379,#98380);
#84410=AXIS2_PLACEMENT_3D('',#194775,#98385,#98386);
#84411=AXIS2_PLACEMENT_3D('',#194781,#98390,#98391);
#84412=AXIS2_PLACEMENT_3D('',#194787,#98395,#98396);
#84413=AXIS2_PLACEMENT_3D('',#194790,#98399,#98400);
#84414=AXIS2_PLACEMENT_3D('',#194799,#98405,#98406);
#84415=AXIS2_PLACEMENT_3D('',#194805,#98410,#98411);
#84416=AXIS2_PLACEMENT_3D('',#194811,#98415,#98416);
#84417=AXIS2_PLACEMENT_3D('',#194814,#98419,#98420);
#84418=AXIS2_PLACEMENT_3D('',#194823,#98425,#98426);
#84419=AXIS2_PLACEMENT_3D('',#194829,#98430,#98431);
#84420=AXIS2_PLACEMENT_3D('',#194835,#98435,#98436);
#84421=AXIS2_PLACEMENT_3D('',#194838,#98439,#98440);
#84422=AXIS2_PLACEMENT_3D('',#194847,#98445,#98446);
#84423=AXIS2_PLACEMENT_3D('',#194853,#98450,#98451);
#84424=AXIS2_PLACEMENT_3D('',#194859,#98455,#98456);
#84425=AXIS2_PLACEMENT_3D('',#194862,#98459,#98460);
#84426=AXIS2_PLACEMENT_3D('',#194871,#98465,#98466);
#84427=AXIS2_PLACEMENT_3D('',#194877,#98470,#98471);
#84428=AXIS2_PLACEMENT_3D('',#194883,#98475,#98476);
#84429=AXIS2_PLACEMENT_3D('',#194886,#98479,#98480);
#84430=AXIS2_PLACEMENT_3D('',#194895,#98485,#98486);
#84431=AXIS2_PLACEMENT_3D('',#194901,#98490,#98491);
#84432=AXIS2_PLACEMENT_3D('',#194907,#98495,#98496);
#84433=AXIS2_PLACEMENT_3D('',#194910,#98499,#98500);
#84434=AXIS2_PLACEMENT_3D('',#194919,#98505,#98506);
#84435=AXIS2_PLACEMENT_3D('',#194925,#98510,#98511);
#84436=AXIS2_PLACEMENT_3D('',#194931,#98515,#98516);
#84437=AXIS2_PLACEMENT_3D('',#194934,#98519,#98520);
#84438=AXIS2_PLACEMENT_3D('',#194943,#98525,#98526);
#84439=AXIS2_PLACEMENT_3D('',#194949,#98530,#98531);
#84440=AXIS2_PLACEMENT_3D('',#194955,#98535,#98536);
#84441=AXIS2_PLACEMENT_3D('',#194958,#98539,#98540);
#84442=AXIS2_PLACEMENT_3D('',#194967,#98545,#98546);
#84443=AXIS2_PLACEMENT_3D('',#194973,#98550,#98551);
#84444=AXIS2_PLACEMENT_3D('',#194979,#98555,#98556);
#84445=AXIS2_PLACEMENT_3D('',#194982,#98559,#98560);
#84446=AXIS2_PLACEMENT_3D('',#194991,#98565,#98566);
#84447=AXIS2_PLACEMENT_3D('',#194997,#98570,#98571);
#84448=AXIS2_PLACEMENT_3D('',#195003,#98575,#98576);
#84449=AXIS2_PLACEMENT_3D('',#195006,#98579,#98580);
#84450=AXIS2_PLACEMENT_3D('',#195015,#98585,#98586);
#84451=AXIS2_PLACEMENT_3D('',#195021,#98590,#98591);
#84452=AXIS2_PLACEMENT_3D('',#195027,#98595,#98596);
#84453=AXIS2_PLACEMENT_3D('',#195030,#98599,#98600);
#84454=AXIS2_PLACEMENT_3D('',#195039,#98605,#98606);
#84455=AXIS2_PLACEMENT_3D('',#195045,#98610,#98611);
#84456=AXIS2_PLACEMENT_3D('',#195051,#98615,#98616);
#84457=AXIS2_PLACEMENT_3D('',#195054,#98619,#98620);
#84458=AXIS2_PLACEMENT_3D('',#195063,#98625,#98626);
#84459=AXIS2_PLACEMENT_3D('',#195069,#98630,#98631);
#84460=AXIS2_PLACEMENT_3D('',#195075,#98635,#98636);
#84461=AXIS2_PLACEMENT_3D('',#195078,#98639,#98640);
#84462=AXIS2_PLACEMENT_3D('',#195087,#98645,#98646);
#84463=AXIS2_PLACEMENT_3D('',#195093,#98650,#98651);
#84464=AXIS2_PLACEMENT_3D('',#195099,#98655,#98656);
#84465=AXIS2_PLACEMENT_3D('',#195102,#98659,#98660);
#84466=AXIS2_PLACEMENT_3D('',#195111,#98665,#98666);
#84467=AXIS2_PLACEMENT_3D('',#195117,#98670,#98671);
#84468=AXIS2_PLACEMENT_3D('',#195123,#98675,#98676);
#84469=AXIS2_PLACEMENT_3D('',#195126,#98679,#98680);
#84470=AXIS2_PLACEMENT_3D('',#195135,#98685,#98686);
#84471=AXIS2_PLACEMENT_3D('',#195141,#98690,#98691);
#84472=AXIS2_PLACEMENT_3D('',#195147,#98695,#98696);
#84473=AXIS2_PLACEMENT_3D('',#195150,#98699,#98700);
#84474=AXIS2_PLACEMENT_3D('',#195159,#98705,#98706);
#84475=AXIS2_PLACEMENT_3D('',#195165,#98710,#98711);
#84476=AXIS2_PLACEMENT_3D('',#195171,#98715,#98716);
#84477=AXIS2_PLACEMENT_3D('',#195174,#98719,#98720);
#84478=AXIS2_PLACEMENT_3D('',#195183,#98725,#98726);
#84479=AXIS2_PLACEMENT_3D('',#195189,#98730,#98731);
#84480=AXIS2_PLACEMENT_3D('',#195195,#98735,#98736);
#84481=AXIS2_PLACEMENT_3D('',#195198,#98739,#98740);
#84482=AXIS2_PLACEMENT_3D('',#195207,#98745,#98746);
#84483=AXIS2_PLACEMENT_3D('',#195213,#98750,#98751);
#84484=AXIS2_PLACEMENT_3D('',#195219,#98755,#98756);
#84485=AXIS2_PLACEMENT_3D('',#195222,#98759,#98760);
#84486=AXIS2_PLACEMENT_3D('',#195231,#98765,#98766);
#84487=AXIS2_PLACEMENT_3D('',#195237,#98770,#98771);
#84488=AXIS2_PLACEMENT_3D('',#195243,#98775,#98776);
#84489=AXIS2_PLACEMENT_3D('',#195246,#98779,#98780);
#84490=AXIS2_PLACEMENT_3D('',#195255,#98785,#98786);
#84491=AXIS2_PLACEMENT_3D('',#195261,#98790,#98791);
#84492=AXIS2_PLACEMENT_3D('',#195267,#98795,#98796);
#84493=AXIS2_PLACEMENT_3D('',#195270,#98799,#98800);
#84494=AXIS2_PLACEMENT_3D('',#195279,#98805,#98806);
#84495=AXIS2_PLACEMENT_3D('',#195285,#98810,#98811);
#84496=AXIS2_PLACEMENT_3D('',#195291,#98815,#98816);
#84497=AXIS2_PLACEMENT_3D('',#195294,#98819,#98820);
#84498=AXIS2_PLACEMENT_3D('',#195303,#98825,#98826);
#84499=AXIS2_PLACEMENT_3D('',#195309,#98830,#98831);
#84500=AXIS2_PLACEMENT_3D('',#195315,#98835,#98836);
#84501=AXIS2_PLACEMENT_3D('',#195318,#98839,#98840);
#84502=AXIS2_PLACEMENT_3D('',#195327,#98845,#98846);
#84503=AXIS2_PLACEMENT_3D('',#195333,#98850,#98851);
#84504=AXIS2_PLACEMENT_3D('',#195339,#98855,#98856);
#84505=AXIS2_PLACEMENT_3D('',#195342,#98859,#98860);
#84506=AXIS2_PLACEMENT_3D('',#195351,#98865,#98866);
#84507=AXIS2_PLACEMENT_3D('',#195357,#98870,#98871);
#84508=AXIS2_PLACEMENT_3D('',#195363,#98875,#98876);
#84509=AXIS2_PLACEMENT_3D('',#195366,#98879,#98880);
#84510=AXIS2_PLACEMENT_3D('',#195375,#98885,#98886);
#84511=AXIS2_PLACEMENT_3D('',#195381,#98890,#98891);
#84512=AXIS2_PLACEMENT_3D('',#195387,#98895,#98896);
#84513=AXIS2_PLACEMENT_3D('',#195390,#98899,#98900);
#84514=AXIS2_PLACEMENT_3D('',#195399,#98905,#98906);
#84515=AXIS2_PLACEMENT_3D('',#195405,#98910,#98911);
#84516=AXIS2_PLACEMENT_3D('',#195411,#98915,#98916);
#84517=AXIS2_PLACEMENT_3D('',#195414,#98919,#98920);
#84518=AXIS2_PLACEMENT_3D('',#195423,#98925,#98926);
#84519=AXIS2_PLACEMENT_3D('',#195429,#98930,#98931);
#84520=AXIS2_PLACEMENT_3D('',#195435,#98935,#98936);
#84521=AXIS2_PLACEMENT_3D('',#195438,#98939,#98940);
#84522=AXIS2_PLACEMENT_3D('',#195447,#98945,#98946);
#84523=AXIS2_PLACEMENT_3D('',#195453,#98950,#98951);
#84524=AXIS2_PLACEMENT_3D('',#195459,#98955,#98956);
#84525=AXIS2_PLACEMENT_3D('',#195462,#98959,#98960);
#84526=AXIS2_PLACEMENT_3D('',#195471,#98965,#98966);
#84527=AXIS2_PLACEMENT_3D('',#195477,#98970,#98971);
#84528=AXIS2_PLACEMENT_3D('',#195483,#98975,#98976);
#84529=AXIS2_PLACEMENT_3D('',#195486,#98979,#98980);
#84530=AXIS2_PLACEMENT_3D('',#195495,#98985,#98986);
#84531=AXIS2_PLACEMENT_3D('',#195501,#98990,#98991);
#84532=AXIS2_PLACEMENT_3D('',#195507,#98995,#98996);
#84533=AXIS2_PLACEMENT_3D('',#195510,#98999,#99000);
#84534=AXIS2_PLACEMENT_3D('',#195519,#99005,#99006);
#84535=AXIS2_PLACEMENT_3D('',#195525,#99010,#99011);
#84536=AXIS2_PLACEMENT_3D('',#195531,#99015,#99016);
#84537=AXIS2_PLACEMENT_3D('',#195534,#99019,#99020);
#84538=AXIS2_PLACEMENT_3D('',#195543,#99025,#99026);
#84539=AXIS2_PLACEMENT_3D('',#195549,#99030,#99031);
#84540=AXIS2_PLACEMENT_3D('',#195555,#99035,#99036);
#84541=AXIS2_PLACEMENT_3D('',#195558,#99039,#99040);
#84542=AXIS2_PLACEMENT_3D('',#195567,#99045,#99046);
#84543=AXIS2_PLACEMENT_3D('',#195573,#99050,#99051);
#84544=AXIS2_PLACEMENT_3D('',#195579,#99055,#99056);
#84545=AXIS2_PLACEMENT_3D('',#195582,#99059,#99060);
#84546=AXIS2_PLACEMENT_3D('',#195591,#99065,#99066);
#84547=AXIS2_PLACEMENT_3D('',#195597,#99070,#99071);
#84548=AXIS2_PLACEMENT_3D('',#195603,#99075,#99076);
#84549=AXIS2_PLACEMENT_3D('',#195606,#99079,#99080);
#84550=AXIS2_PLACEMENT_3D('',#195615,#99085,#99086);
#84551=AXIS2_PLACEMENT_3D('',#195621,#99090,#99091);
#84552=AXIS2_PLACEMENT_3D('',#195627,#99095,#99096);
#84553=AXIS2_PLACEMENT_3D('',#195630,#99099,#99100);
#84554=AXIS2_PLACEMENT_3D('',#195639,#99105,#99106);
#84555=AXIS2_PLACEMENT_3D('',#195645,#99110,#99111);
#84556=AXIS2_PLACEMENT_3D('',#195651,#99115,#99116);
#84557=AXIS2_PLACEMENT_3D('',#195654,#99119,#99120);
#84558=AXIS2_PLACEMENT_3D('',#195663,#99125,#99126);
#84559=AXIS2_PLACEMENT_3D('',#195669,#99130,#99131);
#84560=AXIS2_PLACEMENT_3D('',#195675,#99135,#99136);
#84561=AXIS2_PLACEMENT_3D('',#195678,#99139,#99140);
#84562=AXIS2_PLACEMENT_3D('',#195687,#99145,#99146);
#84563=AXIS2_PLACEMENT_3D('',#195693,#99150,#99151);
#84564=AXIS2_PLACEMENT_3D('',#195699,#99155,#99156);
#84565=AXIS2_PLACEMENT_3D('',#195702,#99159,#99160);
#84566=AXIS2_PLACEMENT_3D('',#195711,#99165,#99166);
#84567=AXIS2_PLACEMENT_3D('',#195717,#99170,#99171);
#84568=AXIS2_PLACEMENT_3D('',#195723,#99175,#99176);
#84569=AXIS2_PLACEMENT_3D('',#195726,#99179,#99180);
#84570=AXIS2_PLACEMENT_3D('',#195735,#99185,#99186);
#84571=AXIS2_PLACEMENT_3D('',#195741,#99190,#99191);
#84572=AXIS2_PLACEMENT_3D('',#195747,#99195,#99196);
#84573=AXIS2_PLACEMENT_3D('',#195750,#99199,#99200);
#84574=AXIS2_PLACEMENT_3D('',#195759,#99205,#99206);
#84575=AXIS2_PLACEMENT_3D('',#195765,#99210,#99211);
#84576=AXIS2_PLACEMENT_3D('',#195771,#99215,#99216);
#84577=AXIS2_PLACEMENT_3D('',#195774,#99219,#99220);
#84578=AXIS2_PLACEMENT_3D('',#195783,#99225,#99226);
#84579=AXIS2_PLACEMENT_3D('',#195789,#99230,#99231);
#84580=AXIS2_PLACEMENT_3D('',#195795,#99235,#99236);
#84581=AXIS2_PLACEMENT_3D('',#195798,#99239,#99240);
#84582=AXIS2_PLACEMENT_3D('',#195807,#99245,#99246);
#84583=AXIS2_PLACEMENT_3D('',#195813,#99250,#99251);
#84584=AXIS2_PLACEMENT_3D('',#195819,#99255,#99256);
#84585=AXIS2_PLACEMENT_3D('',#195822,#99259,#99260);
#84586=AXIS2_PLACEMENT_3D('',#195831,#99265,#99266);
#84587=AXIS2_PLACEMENT_3D('',#195837,#99270,#99271);
#84588=AXIS2_PLACEMENT_3D('',#195843,#99275,#99276);
#84589=AXIS2_PLACEMENT_3D('',#195846,#99279,#99280);
#84590=AXIS2_PLACEMENT_3D('',#195855,#99285,#99286);
#84591=AXIS2_PLACEMENT_3D('',#195861,#99290,#99291);
#84592=AXIS2_PLACEMENT_3D('',#195867,#99295,#99296);
#84593=AXIS2_PLACEMENT_3D('',#195870,#99299,#99300);
#84594=AXIS2_PLACEMENT_3D('',#195879,#99305,#99306);
#84595=AXIS2_PLACEMENT_3D('',#195885,#99310,#99311);
#84596=AXIS2_PLACEMENT_3D('',#195891,#99315,#99316);
#84597=AXIS2_PLACEMENT_3D('',#195894,#99319,#99320);
#84598=AXIS2_PLACEMENT_3D('',#195903,#99325,#99326);
#84599=AXIS2_PLACEMENT_3D('',#195909,#99330,#99331);
#84600=AXIS2_PLACEMENT_3D('',#195915,#99335,#99336);
#84601=AXIS2_PLACEMENT_3D('',#195918,#99339,#99340);
#84602=AXIS2_PLACEMENT_3D('',#195927,#99345,#99346);
#84603=AXIS2_PLACEMENT_3D('',#195933,#99350,#99351);
#84604=AXIS2_PLACEMENT_3D('',#195939,#99355,#99356);
#84605=AXIS2_PLACEMENT_3D('',#195942,#99359,#99360);
#84606=AXIS2_PLACEMENT_3D('',#195951,#99365,#99366);
#84607=AXIS2_PLACEMENT_3D('',#195957,#99370,#99371);
#84608=AXIS2_PLACEMENT_3D('',#195963,#99375,#99376);
#84609=AXIS2_PLACEMENT_3D('',#195966,#99379,#99380);
#84610=AXIS2_PLACEMENT_3D('',#195975,#99385,#99386);
#84611=AXIS2_PLACEMENT_3D('',#195981,#99390,#99391);
#84612=AXIS2_PLACEMENT_3D('',#195987,#99395,#99396);
#84613=AXIS2_PLACEMENT_3D('',#195990,#99399,#99400);
#84614=AXIS2_PLACEMENT_3D('',#195999,#99405,#99406);
#84615=AXIS2_PLACEMENT_3D('',#196005,#99410,#99411);
#84616=AXIS2_PLACEMENT_3D('',#196011,#99415,#99416);
#84617=AXIS2_PLACEMENT_3D('',#196014,#99419,#99420);
#84618=AXIS2_PLACEMENT_3D('',#196023,#99425,#99426);
#84619=AXIS2_PLACEMENT_3D('',#196029,#99430,#99431);
#84620=AXIS2_PLACEMENT_3D('',#196035,#99435,#99436);
#84621=AXIS2_PLACEMENT_3D('',#196038,#99439,#99440);
#84622=AXIS2_PLACEMENT_3D('',#196047,#99445,#99446);
#84623=AXIS2_PLACEMENT_3D('',#196053,#99450,#99451);
#84624=AXIS2_PLACEMENT_3D('',#196059,#99455,#99456);
#84625=AXIS2_PLACEMENT_3D('',#196062,#99459,#99460);
#84626=AXIS2_PLACEMENT_3D('',#196071,#99465,#99466);
#84627=AXIS2_PLACEMENT_3D('',#196077,#99470,#99471);
#84628=AXIS2_PLACEMENT_3D('',#196083,#99475,#99476);
#84629=AXIS2_PLACEMENT_3D('',#196086,#99479,#99480);
#84630=AXIS2_PLACEMENT_3D('',#196095,#99485,#99486);
#84631=AXIS2_PLACEMENT_3D('',#196101,#99490,#99491);
#84632=AXIS2_PLACEMENT_3D('',#196107,#99495,#99496);
#84633=AXIS2_PLACEMENT_3D('',#196110,#99499,#99500);
#84634=AXIS2_PLACEMENT_3D('',#196119,#99505,#99506);
#84635=AXIS2_PLACEMENT_3D('',#196125,#99510,#99511);
#84636=AXIS2_PLACEMENT_3D('',#196131,#99515,#99516);
#84637=AXIS2_PLACEMENT_3D('',#196134,#99519,#99520);
#84638=AXIS2_PLACEMENT_3D('',#196143,#99525,#99526);
#84639=AXIS2_PLACEMENT_3D('',#196149,#99530,#99531);
#84640=AXIS2_PLACEMENT_3D('',#196155,#99535,#99536);
#84641=AXIS2_PLACEMENT_3D('',#196158,#99539,#99540);
#84642=AXIS2_PLACEMENT_3D('',#196167,#99545,#99546);
#84643=AXIS2_PLACEMENT_3D('',#196173,#99550,#99551);
#84644=AXIS2_PLACEMENT_3D('',#196179,#99555,#99556);
#84645=AXIS2_PLACEMENT_3D('',#196182,#99559,#99560);
#84646=AXIS2_PLACEMENT_3D('',#196191,#99565,#99566);
#84647=AXIS2_PLACEMENT_3D('',#196197,#99570,#99571);
#84648=AXIS2_PLACEMENT_3D('',#196203,#99575,#99576);
#84649=AXIS2_PLACEMENT_3D('',#196206,#99579,#99580);
#84650=AXIS2_PLACEMENT_3D('',#196215,#99585,#99586);
#84651=AXIS2_PLACEMENT_3D('',#196221,#99590,#99591);
#84652=AXIS2_PLACEMENT_3D('',#196227,#99595,#99596);
#84653=AXIS2_PLACEMENT_3D('',#196230,#99599,#99600);
#84654=AXIS2_PLACEMENT_3D('',#196239,#99605,#99606);
#84655=AXIS2_PLACEMENT_3D('',#196245,#99610,#99611);
#84656=AXIS2_PLACEMENT_3D('',#196251,#99615,#99616);
#84657=AXIS2_PLACEMENT_3D('',#196254,#99619,#99620);
#84658=AXIS2_PLACEMENT_3D('',#196263,#99625,#99626);
#84659=AXIS2_PLACEMENT_3D('',#196269,#99630,#99631);
#84660=AXIS2_PLACEMENT_3D('',#196275,#99635,#99636);
#84661=AXIS2_PLACEMENT_3D('',#196278,#99639,#99640);
#84662=AXIS2_PLACEMENT_3D('',#196287,#99645,#99646);
#84663=AXIS2_PLACEMENT_3D('',#196293,#99650,#99651);
#84664=AXIS2_PLACEMENT_3D('',#196299,#99655,#99656);
#84665=AXIS2_PLACEMENT_3D('',#196302,#99659,#99660);
#84666=AXIS2_PLACEMENT_3D('',#196311,#99665,#99666);
#84667=AXIS2_PLACEMENT_3D('',#196317,#99670,#99671);
#84668=AXIS2_PLACEMENT_3D('',#196323,#99675,#99676);
#84669=AXIS2_PLACEMENT_3D('',#196326,#99679,#99680);
#84670=AXIS2_PLACEMENT_3D('',#196335,#99685,#99686);
#84671=AXIS2_PLACEMENT_3D('',#196341,#99690,#99691);
#84672=AXIS2_PLACEMENT_3D('',#196347,#99695,#99696);
#84673=AXIS2_PLACEMENT_3D('',#196350,#99699,#99700);
#84674=AXIS2_PLACEMENT_3D('',#196359,#99705,#99706);
#84675=AXIS2_PLACEMENT_3D('',#196365,#99710,#99711);
#84676=AXIS2_PLACEMENT_3D('',#196371,#99715,#99716);
#84677=AXIS2_PLACEMENT_3D('',#196374,#99719,#99720);
#84678=AXIS2_PLACEMENT_3D('',#196383,#99725,#99726);
#84679=AXIS2_PLACEMENT_3D('',#196389,#99730,#99731);
#84680=AXIS2_PLACEMENT_3D('',#196395,#99735,#99736);
#84681=AXIS2_PLACEMENT_3D('',#196398,#99739,#99740);
#84682=AXIS2_PLACEMENT_3D('',#196407,#99745,#99746);
#84683=AXIS2_PLACEMENT_3D('',#196413,#99750,#99751);
#84684=AXIS2_PLACEMENT_3D('',#196419,#99755,#99756);
#84685=AXIS2_PLACEMENT_3D('',#196422,#99759,#99760);
#84686=AXIS2_PLACEMENT_3D('',#196431,#99765,#99766);
#84687=AXIS2_PLACEMENT_3D('',#196437,#99770,#99771);
#84688=AXIS2_PLACEMENT_3D('',#196443,#99775,#99776);
#84689=AXIS2_PLACEMENT_3D('',#196446,#99779,#99780);
#84690=AXIS2_PLACEMENT_3D('',#196455,#99785,#99786);
#84691=AXIS2_PLACEMENT_3D('',#196461,#99790,#99791);
#84692=AXIS2_PLACEMENT_3D('',#196467,#99795,#99796);
#84693=AXIS2_PLACEMENT_3D('',#196470,#99799,#99800);
#84694=AXIS2_PLACEMENT_3D('',#196479,#99805,#99806);
#84695=AXIS2_PLACEMENT_3D('',#196485,#99810,#99811);
#84696=AXIS2_PLACEMENT_3D('',#196491,#99815,#99816);
#84697=AXIS2_PLACEMENT_3D('',#196494,#99819,#99820);
#84698=AXIS2_PLACEMENT_3D('',#196503,#99825,#99826);
#84699=AXIS2_PLACEMENT_3D('',#196509,#99830,#99831);
#84700=AXIS2_PLACEMENT_3D('',#196515,#99835,#99836);
#84701=AXIS2_PLACEMENT_3D('',#196518,#99839,#99840);
#84702=AXIS2_PLACEMENT_3D('',#196527,#99845,#99846);
#84703=AXIS2_PLACEMENT_3D('',#196533,#99850,#99851);
#84704=AXIS2_PLACEMENT_3D('',#196539,#99855,#99856);
#84705=AXIS2_PLACEMENT_3D('',#196542,#99859,#99860);
#84706=AXIS2_PLACEMENT_3D('',#196551,#99865,#99866);
#84707=AXIS2_PLACEMENT_3D('',#196557,#99870,#99871);
#84708=AXIS2_PLACEMENT_3D('',#196563,#99875,#99876);
#84709=AXIS2_PLACEMENT_3D('',#196566,#99879,#99880);
#84710=AXIS2_PLACEMENT_3D('',#196575,#99885,#99886);
#84711=AXIS2_PLACEMENT_3D('',#196581,#99890,#99891);
#84712=AXIS2_PLACEMENT_3D('',#196587,#99895,#99896);
#84713=AXIS2_PLACEMENT_3D('',#196590,#99899,#99900);
#84714=AXIS2_PLACEMENT_3D('',#196599,#99905,#99906);
#84715=AXIS2_PLACEMENT_3D('',#196605,#99910,#99911);
#84716=AXIS2_PLACEMENT_3D('',#196611,#99915,#99916);
#84717=AXIS2_PLACEMENT_3D('',#196614,#99919,#99920);
#84718=AXIS2_PLACEMENT_3D('',#196623,#99925,#99926);
#84719=AXIS2_PLACEMENT_3D('',#196629,#99930,#99931);
#84720=AXIS2_PLACEMENT_3D('',#196635,#99935,#99936);
#84721=AXIS2_PLACEMENT_3D('',#196638,#99939,#99940);
#84722=AXIS2_PLACEMENT_3D('',#196647,#99945,#99946);
#84723=AXIS2_PLACEMENT_3D('',#196653,#99950,#99951);
#84724=AXIS2_PLACEMENT_3D('',#196659,#99955,#99956);
#84725=AXIS2_PLACEMENT_3D('',#196662,#99959,#99960);
#84726=AXIS2_PLACEMENT_3D('',#196671,#99965,#99966);
#84727=AXIS2_PLACEMENT_3D('',#196677,#99970,#99971);
#84728=AXIS2_PLACEMENT_3D('',#196683,#99975,#99976);
#84729=AXIS2_PLACEMENT_3D('',#196686,#99979,#99980);
#84730=AXIS2_PLACEMENT_3D('',#196695,#99985,#99986);
#84731=AXIS2_PLACEMENT_3D('',#196701,#99990,#99991);
#84732=AXIS2_PLACEMENT_3D('',#196707,#99995,#99996);
#84733=AXIS2_PLACEMENT_3D('',#196710,#99999,#100000);
#84734=AXIS2_PLACEMENT_3D('',#196719,#100005,#100006);
#84735=AXIS2_PLACEMENT_3D('',#196725,#100010,#100011);
#84736=AXIS2_PLACEMENT_3D('',#196731,#100015,#100016);
#84737=AXIS2_PLACEMENT_3D('',#196734,#100019,#100020);
#84738=AXIS2_PLACEMENT_3D('',#196743,#100025,#100026);
#84739=AXIS2_PLACEMENT_3D('',#196749,#100030,#100031);
#84740=AXIS2_PLACEMENT_3D('',#196755,#100035,#100036);
#84741=AXIS2_PLACEMENT_3D('',#196758,#100039,#100040);
#84742=AXIS2_PLACEMENT_3D('',#196767,#100045,#100046);
#84743=AXIS2_PLACEMENT_3D('',#196773,#100050,#100051);
#84744=AXIS2_PLACEMENT_3D('',#196779,#100055,#100056);
#84745=AXIS2_PLACEMENT_3D('',#196782,#100059,#100060);
#84746=AXIS2_PLACEMENT_3D('',#196791,#100065,#100066);
#84747=AXIS2_PLACEMENT_3D('',#196797,#100070,#100071);
#84748=AXIS2_PLACEMENT_3D('',#196803,#100075,#100076);
#84749=AXIS2_PLACEMENT_3D('',#196806,#100079,#100080);
#84750=AXIS2_PLACEMENT_3D('',#196815,#100085,#100086);
#84751=AXIS2_PLACEMENT_3D('',#196821,#100090,#100091);
#84752=AXIS2_PLACEMENT_3D('',#196827,#100095,#100096);
#84753=AXIS2_PLACEMENT_3D('',#196830,#100099,#100100);
#84754=AXIS2_PLACEMENT_3D('',#196839,#100105,#100106);
#84755=AXIS2_PLACEMENT_3D('',#196845,#100110,#100111);
#84756=AXIS2_PLACEMENT_3D('',#196851,#100115,#100116);
#84757=AXIS2_PLACEMENT_3D('',#196854,#100119,#100120);
#84758=AXIS2_PLACEMENT_3D('',#196863,#100125,#100126);
#84759=AXIS2_PLACEMENT_3D('',#196869,#100130,#100131);
#84760=AXIS2_PLACEMENT_3D('',#196875,#100135,#100136);
#84761=AXIS2_PLACEMENT_3D('',#196878,#100139,#100140);
#84762=AXIS2_PLACEMENT_3D('',#196887,#100145,#100146);
#84763=AXIS2_PLACEMENT_3D('',#196893,#100150,#100151);
#84764=AXIS2_PLACEMENT_3D('',#196899,#100155,#100156);
#84765=AXIS2_PLACEMENT_3D('',#196902,#100159,#100160);
#84766=AXIS2_PLACEMENT_3D('',#196911,#100165,#100166);
#84767=AXIS2_PLACEMENT_3D('',#196917,#100170,#100171);
#84768=AXIS2_PLACEMENT_3D('',#196923,#100175,#100176);
#84769=AXIS2_PLACEMENT_3D('',#196926,#100179,#100180);
#84770=AXIS2_PLACEMENT_3D('',#196935,#100185,#100186);
#84771=AXIS2_PLACEMENT_3D('',#196941,#100190,#100191);
#84772=AXIS2_PLACEMENT_3D('',#196947,#100195,#100196);
#84773=AXIS2_PLACEMENT_3D('',#196950,#100199,#100200);
#84774=AXIS2_PLACEMENT_3D('',#196959,#100205,#100206);
#84775=AXIS2_PLACEMENT_3D('',#196965,#100210,#100211);
#84776=AXIS2_PLACEMENT_3D('',#196971,#100215,#100216);
#84777=AXIS2_PLACEMENT_3D('',#196974,#100219,#100220);
#84778=AXIS2_PLACEMENT_3D('',#196983,#100225,#100226);
#84779=AXIS2_PLACEMENT_3D('',#196989,#100230,#100231);
#84780=AXIS2_PLACEMENT_3D('',#196995,#100235,#100236);
#84781=AXIS2_PLACEMENT_3D('',#196998,#100239,#100240);
#84782=AXIS2_PLACEMENT_3D('',#197007,#100245,#100246);
#84783=AXIS2_PLACEMENT_3D('',#197013,#100250,#100251);
#84784=AXIS2_PLACEMENT_3D('',#197019,#100255,#100256);
#84785=AXIS2_PLACEMENT_3D('',#197022,#100259,#100260);
#84786=AXIS2_PLACEMENT_3D('',#197031,#100265,#100266);
#84787=AXIS2_PLACEMENT_3D('',#197037,#100270,#100271);
#84788=AXIS2_PLACEMENT_3D('',#197043,#100275,#100276);
#84789=AXIS2_PLACEMENT_3D('',#197046,#100279,#100280);
#84790=AXIS2_PLACEMENT_3D('',#197055,#100285,#100286);
#84791=AXIS2_PLACEMENT_3D('',#197061,#100290,#100291);
#84792=AXIS2_PLACEMENT_3D('',#197067,#100295,#100296);
#84793=AXIS2_PLACEMENT_3D('',#197070,#100299,#100300);
#84794=AXIS2_PLACEMENT_3D('',#197079,#100305,#100306);
#84795=AXIS2_PLACEMENT_3D('',#197085,#100310,#100311);
#84796=AXIS2_PLACEMENT_3D('',#197091,#100315,#100316);
#84797=AXIS2_PLACEMENT_3D('',#197094,#100319,#100320);
#84798=AXIS2_PLACEMENT_3D('',#197103,#100325,#100326);
#84799=AXIS2_PLACEMENT_3D('',#197109,#100330,#100331);
#84800=AXIS2_PLACEMENT_3D('',#197115,#100335,#100336);
#84801=AXIS2_PLACEMENT_3D('',#197118,#100339,#100340);
#84802=AXIS2_PLACEMENT_3D('',#197127,#100345,#100346);
#84803=AXIS2_PLACEMENT_3D('',#197133,#100350,#100351);
#84804=AXIS2_PLACEMENT_3D('',#197139,#100355,#100356);
#84805=AXIS2_PLACEMENT_3D('',#197142,#100359,#100360);
#84806=AXIS2_PLACEMENT_3D('',#197151,#100365,#100366);
#84807=AXIS2_PLACEMENT_3D('',#197157,#100370,#100371);
#84808=AXIS2_PLACEMENT_3D('',#197163,#100375,#100376);
#84809=AXIS2_PLACEMENT_3D('',#197166,#100379,#100380);
#84810=AXIS2_PLACEMENT_3D('',#197175,#100385,#100386);
#84811=AXIS2_PLACEMENT_3D('',#197181,#100390,#100391);
#84812=AXIS2_PLACEMENT_3D('',#197187,#100395,#100396);
#84813=AXIS2_PLACEMENT_3D('',#197190,#100399,#100400);
#84814=AXIS2_PLACEMENT_3D('',#197199,#100405,#100406);
#84815=AXIS2_PLACEMENT_3D('',#197205,#100410,#100411);
#84816=AXIS2_PLACEMENT_3D('',#197211,#100415,#100416);
#84817=AXIS2_PLACEMENT_3D('',#197214,#100419,#100420);
#84818=AXIS2_PLACEMENT_3D('',#197223,#100425,#100426);
#84819=AXIS2_PLACEMENT_3D('',#197229,#100430,#100431);
#84820=AXIS2_PLACEMENT_3D('',#197235,#100435,#100436);
#84821=AXIS2_PLACEMENT_3D('',#197238,#100439,#100440);
#84822=AXIS2_PLACEMENT_3D('',#197247,#100445,#100446);
#84823=AXIS2_PLACEMENT_3D('',#197253,#100450,#100451);
#84824=AXIS2_PLACEMENT_3D('',#197259,#100455,#100456);
#84825=AXIS2_PLACEMENT_3D('',#197262,#100459,#100460);
#84826=AXIS2_PLACEMENT_3D('',#197271,#100465,#100466);
#84827=AXIS2_PLACEMENT_3D('',#197277,#100470,#100471);
#84828=AXIS2_PLACEMENT_3D('',#197283,#100475,#100476);
#84829=AXIS2_PLACEMENT_3D('',#197286,#100479,#100480);
#84830=AXIS2_PLACEMENT_3D('',#197295,#100485,#100486);
#84831=AXIS2_PLACEMENT_3D('',#197301,#100490,#100491);
#84832=AXIS2_PLACEMENT_3D('',#197307,#100495,#100496);
#84833=AXIS2_PLACEMENT_3D('',#197310,#100499,#100500);
#84834=AXIS2_PLACEMENT_3D('',#197319,#100505,#100506);
#84835=AXIS2_PLACEMENT_3D('',#197325,#100510,#100511);
#84836=AXIS2_PLACEMENT_3D('',#197331,#100515,#100516);
#84837=AXIS2_PLACEMENT_3D('',#197334,#100519,#100520);
#84838=AXIS2_PLACEMENT_3D('',#197343,#100525,#100526);
#84839=AXIS2_PLACEMENT_3D('',#197349,#100530,#100531);
#84840=AXIS2_PLACEMENT_3D('',#197355,#100535,#100536);
#84841=AXIS2_PLACEMENT_3D('',#197358,#100539,#100540);
#84842=AXIS2_PLACEMENT_3D('',#197367,#100545,#100546);
#84843=AXIS2_PLACEMENT_3D('',#197373,#100550,#100551);
#84844=AXIS2_PLACEMENT_3D('',#197379,#100555,#100556);
#84845=AXIS2_PLACEMENT_3D('',#197382,#100559,#100560);
#84846=AXIS2_PLACEMENT_3D('',#197391,#100565,#100566);
#84847=AXIS2_PLACEMENT_3D('',#197397,#100570,#100571);
#84848=AXIS2_PLACEMENT_3D('',#197403,#100575,#100576);
#84849=AXIS2_PLACEMENT_3D('',#197406,#100579,#100580);
#84850=AXIS2_PLACEMENT_3D('',#197415,#100585,#100586);
#84851=AXIS2_PLACEMENT_3D('',#197421,#100590,#100591);
#84852=AXIS2_PLACEMENT_3D('',#197427,#100595,#100596);
#84853=AXIS2_PLACEMENT_3D('',#197430,#100599,#100600);
#84854=AXIS2_PLACEMENT_3D('',#197439,#100605,#100606);
#84855=AXIS2_PLACEMENT_3D('',#197445,#100610,#100611);
#84856=AXIS2_PLACEMENT_3D('',#197451,#100615,#100616);
#84857=AXIS2_PLACEMENT_3D('',#197454,#100619,#100620);
#84858=AXIS2_PLACEMENT_3D('',#197463,#100625,#100626);
#84859=AXIS2_PLACEMENT_3D('',#197469,#100630,#100631);
#84860=AXIS2_PLACEMENT_3D('',#197475,#100635,#100636);
#84861=AXIS2_PLACEMENT_3D('',#197478,#100639,#100640);
#84862=AXIS2_PLACEMENT_3D('',#197487,#100645,#100646);
#84863=AXIS2_PLACEMENT_3D('',#197493,#100650,#100651);
#84864=AXIS2_PLACEMENT_3D('',#197499,#100655,#100656);
#84865=AXIS2_PLACEMENT_3D('',#197502,#100659,#100660);
#84866=AXIS2_PLACEMENT_3D('',#197511,#100665,#100666);
#84867=AXIS2_PLACEMENT_3D('',#197517,#100670,#100671);
#84868=AXIS2_PLACEMENT_3D('',#197523,#100675,#100676);
#84869=AXIS2_PLACEMENT_3D('',#197526,#100679,#100680);
#84870=AXIS2_PLACEMENT_3D('',#197535,#100685,#100686);
#84871=AXIS2_PLACEMENT_3D('',#197541,#100690,#100691);
#84872=AXIS2_PLACEMENT_3D('',#197547,#100695,#100696);
#84873=AXIS2_PLACEMENT_3D('',#197550,#100699,#100700);
#84874=AXIS2_PLACEMENT_3D('',#197559,#100705,#100706);
#84875=AXIS2_PLACEMENT_3D('',#197565,#100710,#100711);
#84876=AXIS2_PLACEMENT_3D('',#197571,#100715,#100716);
#84877=AXIS2_PLACEMENT_3D('',#197574,#100719,#100720);
#84878=AXIS2_PLACEMENT_3D('',#197583,#100725,#100726);
#84879=AXIS2_PLACEMENT_3D('',#197589,#100730,#100731);
#84880=AXIS2_PLACEMENT_3D('',#197595,#100735,#100736);
#84881=AXIS2_PLACEMENT_3D('',#197598,#100739,#100740);
#84882=AXIS2_PLACEMENT_3D('',#197607,#100745,#100746);
#84883=AXIS2_PLACEMENT_3D('',#197613,#100750,#100751);
#84884=AXIS2_PLACEMENT_3D('',#197619,#100755,#100756);
#84885=AXIS2_PLACEMENT_3D('',#197622,#100759,#100760);
#84886=AXIS2_PLACEMENT_3D('',#197631,#100765,#100766);
#84887=AXIS2_PLACEMENT_3D('',#197637,#100770,#100771);
#84888=AXIS2_PLACEMENT_3D('',#197643,#100775,#100776);
#84889=AXIS2_PLACEMENT_3D('',#197646,#100779,#100780);
#84890=AXIS2_PLACEMENT_3D('',#197655,#100785,#100786);
#84891=AXIS2_PLACEMENT_3D('',#197661,#100790,#100791);
#84892=AXIS2_PLACEMENT_3D('',#197667,#100795,#100796);
#84893=AXIS2_PLACEMENT_3D('',#197670,#100799,#100800);
#84894=AXIS2_PLACEMENT_3D('',#197679,#100805,#100806);
#84895=AXIS2_PLACEMENT_3D('',#197685,#100810,#100811);
#84896=AXIS2_PLACEMENT_3D('',#197691,#100815,#100816);
#84897=AXIS2_PLACEMENT_3D('',#197694,#100819,#100820);
#84898=AXIS2_PLACEMENT_3D('',#197703,#100825,#100826);
#84899=AXIS2_PLACEMENT_3D('',#197709,#100830,#100831);
#84900=AXIS2_PLACEMENT_3D('',#197715,#100835,#100836);
#84901=AXIS2_PLACEMENT_3D('',#197718,#100839,#100840);
#84902=AXIS2_PLACEMENT_3D('',#197727,#100845,#100846);
#84903=AXIS2_PLACEMENT_3D('',#197733,#100850,#100851);
#84904=AXIS2_PLACEMENT_3D('',#197739,#100855,#100856);
#84905=AXIS2_PLACEMENT_3D('',#197742,#100859,#100860);
#84906=AXIS2_PLACEMENT_3D('',#197751,#100865,#100866);
#84907=AXIS2_PLACEMENT_3D('',#197757,#100870,#100871);
#84908=AXIS2_PLACEMENT_3D('',#197763,#100875,#100876);
#84909=AXIS2_PLACEMENT_3D('',#197766,#100879,#100880);
#84910=AXIS2_PLACEMENT_3D('',#197775,#100885,#100886);
#84911=AXIS2_PLACEMENT_3D('',#197781,#100890,#100891);
#84912=AXIS2_PLACEMENT_3D('',#197787,#100895,#100896);
#84913=AXIS2_PLACEMENT_3D('',#197790,#100899,#100900);
#84914=AXIS2_PLACEMENT_3D('',#197799,#100905,#100906);
#84915=AXIS2_PLACEMENT_3D('',#197805,#100910,#100911);
#84916=AXIS2_PLACEMENT_3D('',#197811,#100915,#100916);
#84917=AXIS2_PLACEMENT_3D('',#197814,#100919,#100920);
#84918=AXIS2_PLACEMENT_3D('',#197823,#100925,#100926);
#84919=AXIS2_PLACEMENT_3D('',#197829,#100930,#100931);
#84920=AXIS2_PLACEMENT_3D('',#197835,#100935,#100936);
#84921=AXIS2_PLACEMENT_3D('',#197838,#100939,#100940);
#84922=AXIS2_PLACEMENT_3D('',#197847,#100945,#100946);
#84923=AXIS2_PLACEMENT_3D('',#197853,#100950,#100951);
#84924=AXIS2_PLACEMENT_3D('',#197859,#100955,#100956);
#84925=AXIS2_PLACEMENT_3D('',#197862,#100959,#100960);
#84926=AXIS2_PLACEMENT_3D('',#197871,#100965,#100966);
#84927=AXIS2_PLACEMENT_3D('',#197877,#100970,#100971);
#84928=AXIS2_PLACEMENT_3D('',#197883,#100975,#100976);
#84929=AXIS2_PLACEMENT_3D('',#197886,#100979,#100980);
#84930=AXIS2_PLACEMENT_3D('',#197895,#100985,#100986);
#84931=AXIS2_PLACEMENT_3D('',#197901,#100990,#100991);
#84932=AXIS2_PLACEMENT_3D('',#197907,#100995,#100996);
#84933=AXIS2_PLACEMENT_3D('',#197910,#100999,#101000);
#84934=AXIS2_PLACEMENT_3D('',#197919,#101005,#101006);
#84935=AXIS2_PLACEMENT_3D('',#197925,#101010,#101011);
#84936=AXIS2_PLACEMENT_3D('',#197931,#101015,#101016);
#84937=AXIS2_PLACEMENT_3D('',#197934,#101019,#101020);
#84938=AXIS2_PLACEMENT_3D('',#197943,#101025,#101026);
#84939=AXIS2_PLACEMENT_3D('',#197949,#101030,#101031);
#84940=AXIS2_PLACEMENT_3D('',#197955,#101035,#101036);
#84941=AXIS2_PLACEMENT_3D('',#197958,#101039,#101040);
#84942=AXIS2_PLACEMENT_3D('',#197967,#101045,#101046);
#84943=AXIS2_PLACEMENT_3D('',#197973,#101050,#101051);
#84944=AXIS2_PLACEMENT_3D('',#197979,#101055,#101056);
#84945=AXIS2_PLACEMENT_3D('',#197982,#101059,#101060);
#84946=AXIS2_PLACEMENT_3D('',#197991,#101065,#101066);
#84947=AXIS2_PLACEMENT_3D('',#197997,#101070,#101071);
#84948=AXIS2_PLACEMENT_3D('',#198003,#101075,#101076);
#84949=AXIS2_PLACEMENT_3D('',#198006,#101079,#101080);
#84950=AXIS2_PLACEMENT_3D('',#198015,#101085,#101086);
#84951=AXIS2_PLACEMENT_3D('',#198021,#101090,#101091);
#84952=AXIS2_PLACEMENT_3D('',#198027,#101095,#101096);
#84953=AXIS2_PLACEMENT_3D('',#198030,#101099,#101100);
#84954=AXIS2_PLACEMENT_3D('',#198039,#101105,#101106);
#84955=AXIS2_PLACEMENT_3D('',#198045,#101110,#101111);
#84956=AXIS2_PLACEMENT_3D('',#198051,#101115,#101116);
#84957=AXIS2_PLACEMENT_3D('',#198054,#101119,#101120);
#84958=AXIS2_PLACEMENT_3D('',#198063,#101125,#101126);
#84959=AXIS2_PLACEMENT_3D('',#198069,#101130,#101131);
#84960=AXIS2_PLACEMENT_3D('',#198075,#101135,#101136);
#84961=AXIS2_PLACEMENT_3D('',#198078,#101139,#101140);
#84962=AXIS2_PLACEMENT_3D('',#198087,#101145,#101146);
#84963=AXIS2_PLACEMENT_3D('',#198093,#101150,#101151);
#84964=AXIS2_PLACEMENT_3D('',#198099,#101155,#101156);
#84965=AXIS2_PLACEMENT_3D('',#198102,#101159,#101160);
#84966=AXIS2_PLACEMENT_3D('',#198111,#101165,#101166);
#84967=AXIS2_PLACEMENT_3D('',#198117,#101170,#101171);
#84968=AXIS2_PLACEMENT_3D('',#198123,#101175,#101176);
#84969=AXIS2_PLACEMENT_3D('',#198126,#101179,#101180);
#84970=AXIS2_PLACEMENT_3D('',#198135,#101185,#101186);
#84971=AXIS2_PLACEMENT_3D('',#198141,#101190,#101191);
#84972=AXIS2_PLACEMENT_3D('',#198147,#101195,#101196);
#84973=AXIS2_PLACEMENT_3D('',#198150,#101199,#101200);
#84974=AXIS2_PLACEMENT_3D('',#198159,#101205,#101206);
#84975=AXIS2_PLACEMENT_3D('',#198165,#101210,#101211);
#84976=AXIS2_PLACEMENT_3D('',#198171,#101215,#101216);
#84977=AXIS2_PLACEMENT_3D('',#198174,#101219,#101220);
#84978=AXIS2_PLACEMENT_3D('',#198183,#101225,#101226);
#84979=AXIS2_PLACEMENT_3D('',#198189,#101230,#101231);
#84980=AXIS2_PLACEMENT_3D('',#198195,#101235,#101236);
#84981=AXIS2_PLACEMENT_3D('',#198198,#101239,#101240);
#84982=AXIS2_PLACEMENT_3D('',#198207,#101245,#101246);
#84983=AXIS2_PLACEMENT_3D('',#198213,#101250,#101251);
#84984=AXIS2_PLACEMENT_3D('',#198219,#101255,#101256);
#84985=AXIS2_PLACEMENT_3D('',#198222,#101259,#101260);
#84986=AXIS2_PLACEMENT_3D('',#198231,#101265,#101266);
#84987=AXIS2_PLACEMENT_3D('',#198237,#101270,#101271);
#84988=AXIS2_PLACEMENT_3D('',#198243,#101275,#101276);
#84989=AXIS2_PLACEMENT_3D('',#198246,#101279,#101280);
#84990=AXIS2_PLACEMENT_3D('',#198255,#101285,#101286);
#84991=AXIS2_PLACEMENT_3D('',#198261,#101290,#101291);
#84992=AXIS2_PLACEMENT_3D('',#198267,#101295,#101296);
#84993=AXIS2_PLACEMENT_3D('',#198270,#101299,#101300);
#84994=AXIS2_PLACEMENT_3D('',#198279,#101305,#101306);
#84995=AXIS2_PLACEMENT_3D('',#198285,#101310,#101311);
#84996=AXIS2_PLACEMENT_3D('',#198291,#101315,#101316);
#84997=AXIS2_PLACEMENT_3D('',#198294,#101319,#101320);
#84998=AXIS2_PLACEMENT_3D('',#198303,#101325,#101326);
#84999=AXIS2_PLACEMENT_3D('',#198309,#101330,#101331);
#85000=AXIS2_PLACEMENT_3D('',#198315,#101335,#101336);
#85001=AXIS2_PLACEMENT_3D('',#198318,#101339,#101340);
#85002=AXIS2_PLACEMENT_3D('',#198327,#101345,#101346);
#85003=AXIS2_PLACEMENT_3D('',#198333,#101350,#101351);
#85004=AXIS2_PLACEMENT_3D('',#198339,#101355,#101356);
#85005=AXIS2_PLACEMENT_3D('',#198342,#101359,#101360);
#85006=AXIS2_PLACEMENT_3D('',#198351,#101365,#101366);
#85007=AXIS2_PLACEMENT_3D('',#198357,#101370,#101371);
#85008=AXIS2_PLACEMENT_3D('',#198363,#101375,#101376);
#85009=AXIS2_PLACEMENT_3D('',#198366,#101379,#101380);
#85010=AXIS2_PLACEMENT_3D('',#198375,#101385,#101386);
#85011=AXIS2_PLACEMENT_3D('',#198381,#101390,#101391);
#85012=AXIS2_PLACEMENT_3D('',#198387,#101395,#101396);
#85013=AXIS2_PLACEMENT_3D('',#198390,#101399,#101400);
#85014=AXIS2_PLACEMENT_3D('',#198399,#101405,#101406);
#85015=AXIS2_PLACEMENT_3D('',#198405,#101410,#101411);
#85016=AXIS2_PLACEMENT_3D('',#198411,#101415,#101416);
#85017=AXIS2_PLACEMENT_3D('',#198414,#101419,#101420);
#85018=AXIS2_PLACEMENT_3D('',#198423,#101425,#101426);
#85019=AXIS2_PLACEMENT_3D('',#198429,#101430,#101431);
#85020=AXIS2_PLACEMENT_3D('',#198435,#101435,#101436);
#85021=AXIS2_PLACEMENT_3D('',#198438,#101439,#101440);
#85022=AXIS2_PLACEMENT_3D('',#198447,#101445,#101446);
#85023=AXIS2_PLACEMENT_3D('',#198453,#101450,#101451);
#85024=AXIS2_PLACEMENT_3D('',#198459,#101455,#101456);
#85025=AXIS2_PLACEMENT_3D('',#198462,#101459,#101460);
#85026=AXIS2_PLACEMENT_3D('',#198471,#101465,#101466);
#85027=AXIS2_PLACEMENT_3D('',#198477,#101470,#101471);
#85028=AXIS2_PLACEMENT_3D('',#198483,#101475,#101476);
#85029=AXIS2_PLACEMENT_3D('',#198486,#101479,#101480);
#85030=AXIS2_PLACEMENT_3D('',#198495,#101485,#101486);
#85031=AXIS2_PLACEMENT_3D('',#198501,#101490,#101491);
#85032=AXIS2_PLACEMENT_3D('',#198507,#101495,#101496);
#85033=AXIS2_PLACEMENT_3D('',#198510,#101499,#101500);
#85034=AXIS2_PLACEMENT_3D('',#198519,#101505,#101506);
#85035=AXIS2_PLACEMENT_3D('',#198525,#101510,#101511);
#85036=AXIS2_PLACEMENT_3D('',#198531,#101515,#101516);
#85037=AXIS2_PLACEMENT_3D('',#198534,#101519,#101520);
#85038=AXIS2_PLACEMENT_3D('',#198543,#101525,#101526);
#85039=AXIS2_PLACEMENT_3D('',#198549,#101530,#101531);
#85040=AXIS2_PLACEMENT_3D('',#198555,#101535,#101536);
#85041=AXIS2_PLACEMENT_3D('',#198558,#101539,#101540);
#85042=AXIS2_PLACEMENT_3D('',#198567,#101545,#101546);
#85043=AXIS2_PLACEMENT_3D('',#198573,#101550,#101551);
#85044=AXIS2_PLACEMENT_3D('',#198579,#101555,#101556);
#85045=AXIS2_PLACEMENT_3D('',#198582,#101559,#101560);
#85046=AXIS2_PLACEMENT_3D('',#198591,#101565,#101566);
#85047=AXIS2_PLACEMENT_3D('',#198597,#101570,#101571);
#85048=AXIS2_PLACEMENT_3D('',#198603,#101575,#101576);
#85049=AXIS2_PLACEMENT_3D('',#198606,#101579,#101580);
#85050=AXIS2_PLACEMENT_3D('',#198615,#101585,#101586);
#85051=AXIS2_PLACEMENT_3D('',#198621,#101590,#101591);
#85052=AXIS2_PLACEMENT_3D('',#198627,#101595,#101596);
#85053=AXIS2_PLACEMENT_3D('',#198630,#101599,#101600);
#85054=AXIS2_PLACEMENT_3D('',#198639,#101605,#101606);
#85055=AXIS2_PLACEMENT_3D('',#198645,#101610,#101611);
#85056=AXIS2_PLACEMENT_3D('',#198651,#101615,#101616);
#85057=AXIS2_PLACEMENT_3D('',#198654,#101619,#101620);
#85058=AXIS2_PLACEMENT_3D('',#198663,#101625,#101626);
#85059=AXIS2_PLACEMENT_3D('',#198669,#101630,#101631);
#85060=AXIS2_PLACEMENT_3D('',#198675,#101635,#101636);
#85061=AXIS2_PLACEMENT_3D('',#198678,#101639,#101640);
#85062=AXIS2_PLACEMENT_3D('',#198687,#101645,#101646);
#85063=AXIS2_PLACEMENT_3D('',#198693,#101650,#101651);
#85064=AXIS2_PLACEMENT_3D('',#198699,#101655,#101656);
#85065=AXIS2_PLACEMENT_3D('',#198702,#101659,#101660);
#85066=AXIS2_PLACEMENT_3D('',#198711,#101665,#101666);
#85067=AXIS2_PLACEMENT_3D('',#198717,#101670,#101671);
#85068=AXIS2_PLACEMENT_3D('',#198723,#101675,#101676);
#85069=AXIS2_PLACEMENT_3D('',#198726,#101679,#101680);
#85070=AXIS2_PLACEMENT_3D('',#198735,#101685,#101686);
#85071=AXIS2_PLACEMENT_3D('',#198741,#101690,#101691);
#85072=AXIS2_PLACEMENT_3D('',#198747,#101695,#101696);
#85073=AXIS2_PLACEMENT_3D('',#198750,#101699,#101700);
#85074=AXIS2_PLACEMENT_3D('',#198759,#101705,#101706);
#85075=AXIS2_PLACEMENT_3D('',#198765,#101710,#101711);
#85076=AXIS2_PLACEMENT_3D('',#198771,#101715,#101716);
#85077=AXIS2_PLACEMENT_3D('',#198774,#101719,#101720);
#85078=AXIS2_PLACEMENT_3D('',#198783,#101725,#101726);
#85079=AXIS2_PLACEMENT_3D('',#198789,#101730,#101731);
#85080=AXIS2_PLACEMENT_3D('',#198795,#101735,#101736);
#85081=AXIS2_PLACEMENT_3D('',#198798,#101739,#101740);
#85082=AXIS2_PLACEMENT_3D('',#198807,#101745,#101746);
#85083=AXIS2_PLACEMENT_3D('',#198813,#101750,#101751);
#85084=AXIS2_PLACEMENT_3D('',#198819,#101755,#101756);
#85085=AXIS2_PLACEMENT_3D('',#198822,#101759,#101760);
#85086=AXIS2_PLACEMENT_3D('',#198831,#101765,#101766);
#85087=AXIS2_PLACEMENT_3D('',#198837,#101770,#101771);
#85088=AXIS2_PLACEMENT_3D('',#198843,#101775,#101776);
#85089=AXIS2_PLACEMENT_3D('',#198846,#101779,#101780);
#85090=AXIS2_PLACEMENT_3D('',#198855,#101785,#101786);
#85091=AXIS2_PLACEMENT_3D('',#198861,#101790,#101791);
#85092=AXIS2_PLACEMENT_3D('',#198867,#101795,#101796);
#85093=AXIS2_PLACEMENT_3D('',#198870,#101799,#101800);
#85094=AXIS2_PLACEMENT_3D('',#198879,#101805,#101806);
#85095=AXIS2_PLACEMENT_3D('',#198885,#101810,#101811);
#85096=AXIS2_PLACEMENT_3D('',#198891,#101815,#101816);
#85097=AXIS2_PLACEMENT_3D('',#198894,#101819,#101820);
#85098=AXIS2_PLACEMENT_3D('',#198903,#101825,#101826);
#85099=AXIS2_PLACEMENT_3D('',#198909,#101830,#101831);
#85100=AXIS2_PLACEMENT_3D('',#198915,#101835,#101836);
#85101=AXIS2_PLACEMENT_3D('',#198918,#101839,#101840);
#85102=AXIS2_PLACEMENT_3D('',#198927,#101845,#101846);
#85103=AXIS2_PLACEMENT_3D('',#198933,#101850,#101851);
#85104=AXIS2_PLACEMENT_3D('',#198939,#101855,#101856);
#85105=AXIS2_PLACEMENT_3D('',#198942,#101859,#101860);
#85106=AXIS2_PLACEMENT_3D('',#198951,#101865,#101866);
#85107=AXIS2_PLACEMENT_3D('',#198957,#101870,#101871);
#85108=AXIS2_PLACEMENT_3D('',#198963,#101875,#101876);
#85109=AXIS2_PLACEMENT_3D('',#198966,#101879,#101880);
#85110=AXIS2_PLACEMENT_3D('',#198975,#101885,#101886);
#85111=AXIS2_PLACEMENT_3D('',#198981,#101890,#101891);
#85112=AXIS2_PLACEMENT_3D('',#198987,#101895,#101896);
#85113=AXIS2_PLACEMENT_3D('',#198990,#101899,#101900);
#85114=AXIS2_PLACEMENT_3D('',#198999,#101905,#101906);
#85115=AXIS2_PLACEMENT_3D('',#199005,#101910,#101911);
#85116=AXIS2_PLACEMENT_3D('',#199011,#101915,#101916);
#85117=AXIS2_PLACEMENT_3D('',#199014,#101919,#101920);
#85118=AXIS2_PLACEMENT_3D('',#199023,#101925,#101926);
#85119=AXIS2_PLACEMENT_3D('',#199029,#101930,#101931);
#85120=AXIS2_PLACEMENT_3D('',#199035,#101935,#101936);
#85121=AXIS2_PLACEMENT_3D('',#199038,#101939,#101940);
#85122=AXIS2_PLACEMENT_3D('',#199047,#101945,#101946);
#85123=AXIS2_PLACEMENT_3D('',#199053,#101950,#101951);
#85124=AXIS2_PLACEMENT_3D('',#199059,#101955,#101956);
#85125=AXIS2_PLACEMENT_3D('',#199062,#101959,#101960);
#85126=AXIS2_PLACEMENT_3D('',#199071,#101965,#101966);
#85127=AXIS2_PLACEMENT_3D('',#199077,#101970,#101971);
#85128=AXIS2_PLACEMENT_3D('',#199083,#101975,#101976);
#85129=AXIS2_PLACEMENT_3D('',#199086,#101979,#101980);
#85130=AXIS2_PLACEMENT_3D('',#199095,#101985,#101986);
#85131=AXIS2_PLACEMENT_3D('',#199101,#101990,#101991);
#85132=AXIS2_PLACEMENT_3D('',#199107,#101995,#101996);
#85133=AXIS2_PLACEMENT_3D('',#199110,#101999,#102000);
#85134=AXIS2_PLACEMENT_3D('',#199119,#102005,#102006);
#85135=AXIS2_PLACEMENT_3D('',#199125,#102010,#102011);
#85136=AXIS2_PLACEMENT_3D('',#199131,#102015,#102016);
#85137=AXIS2_PLACEMENT_3D('',#199134,#102019,#102020);
#85138=AXIS2_PLACEMENT_3D('',#199143,#102025,#102026);
#85139=AXIS2_PLACEMENT_3D('',#199149,#102030,#102031);
#85140=AXIS2_PLACEMENT_3D('',#199155,#102035,#102036);
#85141=AXIS2_PLACEMENT_3D('',#199158,#102039,#102040);
#85142=AXIS2_PLACEMENT_3D('',#199167,#102045,#102046);
#85143=AXIS2_PLACEMENT_3D('',#199173,#102050,#102051);
#85144=AXIS2_PLACEMENT_3D('',#199179,#102055,#102056);
#85145=AXIS2_PLACEMENT_3D('',#199182,#102059,#102060);
#85146=AXIS2_PLACEMENT_3D('',#199191,#102065,#102066);
#85147=AXIS2_PLACEMENT_3D('',#199197,#102070,#102071);
#85148=AXIS2_PLACEMENT_3D('',#199203,#102075,#102076);
#85149=AXIS2_PLACEMENT_3D('',#199206,#102079,#102080);
#85150=AXIS2_PLACEMENT_3D('',#199215,#102085,#102086);
#85151=AXIS2_PLACEMENT_3D('',#199221,#102090,#102091);
#85152=AXIS2_PLACEMENT_3D('',#199227,#102095,#102096);
#85153=AXIS2_PLACEMENT_3D('',#199230,#102099,#102100);
#85154=AXIS2_PLACEMENT_3D('',#199239,#102105,#102106);
#85155=AXIS2_PLACEMENT_3D('',#199245,#102110,#102111);
#85156=AXIS2_PLACEMENT_3D('',#199251,#102115,#102116);
#85157=AXIS2_PLACEMENT_3D('',#199254,#102119,#102120);
#85158=AXIS2_PLACEMENT_3D('',#199263,#102125,#102126);
#85159=AXIS2_PLACEMENT_3D('',#199269,#102130,#102131);
#85160=AXIS2_PLACEMENT_3D('',#199275,#102135,#102136);
#85161=AXIS2_PLACEMENT_3D('',#199278,#102139,#102140);
#85162=AXIS2_PLACEMENT_3D('',#199287,#102145,#102146);
#85163=AXIS2_PLACEMENT_3D('',#199293,#102150,#102151);
#85164=AXIS2_PLACEMENT_3D('',#199299,#102155,#102156);
#85165=AXIS2_PLACEMENT_3D('',#199302,#102159,#102160);
#85166=AXIS2_PLACEMENT_3D('',#199311,#102165,#102166);
#85167=AXIS2_PLACEMENT_3D('',#199317,#102170,#102171);
#85168=AXIS2_PLACEMENT_3D('',#199323,#102175,#102176);
#85169=AXIS2_PLACEMENT_3D('',#199326,#102179,#102180);
#85170=AXIS2_PLACEMENT_3D('',#199335,#102185,#102186);
#85171=AXIS2_PLACEMENT_3D('',#199341,#102190,#102191);
#85172=AXIS2_PLACEMENT_3D('',#199347,#102195,#102196);
#85173=AXIS2_PLACEMENT_3D('',#199350,#102199,#102200);
#85174=AXIS2_PLACEMENT_3D('',#199359,#102205,#102206);
#85175=AXIS2_PLACEMENT_3D('',#199365,#102210,#102211);
#85176=AXIS2_PLACEMENT_3D('',#199371,#102215,#102216);
#85177=AXIS2_PLACEMENT_3D('',#199374,#102219,#102220);
#85178=AXIS2_PLACEMENT_3D('',#199383,#102225,#102226);
#85179=AXIS2_PLACEMENT_3D('',#199389,#102230,#102231);
#85180=AXIS2_PLACEMENT_3D('',#199395,#102235,#102236);
#85181=AXIS2_PLACEMENT_3D('',#199398,#102239,#102240);
#85182=AXIS2_PLACEMENT_3D('',#199407,#102245,#102246);
#85183=AXIS2_PLACEMENT_3D('',#199413,#102250,#102251);
#85184=AXIS2_PLACEMENT_3D('',#199419,#102255,#102256);
#85185=AXIS2_PLACEMENT_3D('',#199422,#102259,#102260);
#85186=AXIS2_PLACEMENT_3D('',#199431,#102265,#102266);
#85187=AXIS2_PLACEMENT_3D('',#199437,#102270,#102271);
#85188=AXIS2_PLACEMENT_3D('',#199443,#102275,#102276);
#85189=AXIS2_PLACEMENT_3D('',#199446,#102279,#102280);
#85190=AXIS2_PLACEMENT_3D('',#199455,#102285,#102286);
#85191=AXIS2_PLACEMENT_3D('',#199461,#102290,#102291);
#85192=AXIS2_PLACEMENT_3D('',#199467,#102295,#102296);
#85193=AXIS2_PLACEMENT_3D('',#199470,#102299,#102300);
#85194=AXIS2_PLACEMENT_3D('',#199479,#102305,#102306);
#85195=AXIS2_PLACEMENT_3D('',#199485,#102310,#102311);
#85196=AXIS2_PLACEMENT_3D('',#199491,#102315,#102316);
#85197=AXIS2_PLACEMENT_3D('',#199494,#102319,#102320);
#85198=AXIS2_PLACEMENT_3D('',#199503,#102325,#102326);
#85199=AXIS2_PLACEMENT_3D('',#199509,#102330,#102331);
#85200=AXIS2_PLACEMENT_3D('',#199515,#102335,#102336);
#85201=AXIS2_PLACEMENT_3D('',#199518,#102339,#102340);
#85202=AXIS2_PLACEMENT_3D('',#199527,#102345,#102346);
#85203=AXIS2_PLACEMENT_3D('',#199533,#102350,#102351);
#85204=AXIS2_PLACEMENT_3D('',#199539,#102355,#102356);
#85205=AXIS2_PLACEMENT_3D('',#199542,#102359,#102360);
#85206=AXIS2_PLACEMENT_3D('',#199551,#102365,#102366);
#85207=AXIS2_PLACEMENT_3D('',#199557,#102370,#102371);
#85208=AXIS2_PLACEMENT_3D('',#199563,#102375,#102376);
#85209=AXIS2_PLACEMENT_3D('',#199566,#102379,#102380);
#85210=AXIS2_PLACEMENT_3D('',#199575,#102385,#102386);
#85211=AXIS2_PLACEMENT_3D('',#199581,#102390,#102391);
#85212=AXIS2_PLACEMENT_3D('',#199587,#102395,#102396);
#85213=AXIS2_PLACEMENT_3D('',#199590,#102399,#102400);
#85214=AXIS2_PLACEMENT_3D('',#199599,#102405,#102406);
#85215=AXIS2_PLACEMENT_3D('',#199605,#102410,#102411);
#85216=AXIS2_PLACEMENT_3D('',#199611,#102415,#102416);
#85217=AXIS2_PLACEMENT_3D('',#199614,#102419,#102420);
#85218=AXIS2_PLACEMENT_3D('',#199623,#102425,#102426);
#85219=AXIS2_PLACEMENT_3D('',#199629,#102430,#102431);
#85220=AXIS2_PLACEMENT_3D('',#199635,#102435,#102436);
#85221=AXIS2_PLACEMENT_3D('',#199638,#102439,#102440);
#85222=AXIS2_PLACEMENT_3D('',#199647,#102445,#102446);
#85223=AXIS2_PLACEMENT_3D('',#199653,#102450,#102451);
#85224=AXIS2_PLACEMENT_3D('',#199659,#102455,#102456);
#85225=AXIS2_PLACEMENT_3D('',#199662,#102459,#102460);
#85226=AXIS2_PLACEMENT_3D('',#199671,#102465,#102466);
#85227=AXIS2_PLACEMENT_3D('',#199677,#102470,#102471);
#85228=AXIS2_PLACEMENT_3D('',#199683,#102475,#102476);
#85229=AXIS2_PLACEMENT_3D('',#199686,#102479,#102480);
#85230=AXIS2_PLACEMENT_3D('',#199695,#102485,#102486);
#85231=AXIS2_PLACEMENT_3D('',#199701,#102490,#102491);
#85232=AXIS2_PLACEMENT_3D('',#199707,#102495,#102496);
#85233=AXIS2_PLACEMENT_3D('',#199710,#102499,#102500);
#85234=AXIS2_PLACEMENT_3D('',#199719,#102505,#102506);
#85235=AXIS2_PLACEMENT_3D('',#199725,#102510,#102511);
#85236=AXIS2_PLACEMENT_3D('',#199731,#102515,#102516);
#85237=AXIS2_PLACEMENT_3D('',#199734,#102519,#102520);
#85238=AXIS2_PLACEMENT_3D('',#199743,#102525,#102526);
#85239=AXIS2_PLACEMENT_3D('',#199749,#102530,#102531);
#85240=AXIS2_PLACEMENT_3D('',#199755,#102535,#102536);
#85241=AXIS2_PLACEMENT_3D('',#199758,#102539,#102540);
#85242=AXIS2_PLACEMENT_3D('',#199767,#102545,#102546);
#85243=AXIS2_PLACEMENT_3D('',#199773,#102550,#102551);
#85244=AXIS2_PLACEMENT_3D('',#199779,#102555,#102556);
#85245=AXIS2_PLACEMENT_3D('',#199782,#102559,#102560);
#85246=AXIS2_PLACEMENT_3D('',#199791,#102565,#102566);
#85247=AXIS2_PLACEMENT_3D('',#199797,#102570,#102571);
#85248=AXIS2_PLACEMENT_3D('',#199803,#102575,#102576);
#85249=AXIS2_PLACEMENT_3D('',#199806,#102579,#102580);
#85250=AXIS2_PLACEMENT_3D('',#199815,#102585,#102586);
#85251=AXIS2_PLACEMENT_3D('',#199821,#102590,#102591);
#85252=AXIS2_PLACEMENT_3D('',#199827,#102595,#102596);
#85253=AXIS2_PLACEMENT_3D('',#199830,#102599,#102600);
#85254=AXIS2_PLACEMENT_3D('',#199839,#102605,#102606);
#85255=AXIS2_PLACEMENT_3D('',#199845,#102610,#102611);
#85256=AXIS2_PLACEMENT_3D('',#199851,#102615,#102616);
#85257=AXIS2_PLACEMENT_3D('',#199854,#102619,#102620);
#85258=AXIS2_PLACEMENT_3D('',#199863,#102625,#102626);
#85259=AXIS2_PLACEMENT_3D('',#199869,#102630,#102631);
#85260=AXIS2_PLACEMENT_3D('',#199875,#102635,#102636);
#85261=AXIS2_PLACEMENT_3D('',#199878,#102639,#102640);
#85262=AXIS2_PLACEMENT_3D('',#199887,#102645,#102646);
#85263=AXIS2_PLACEMENT_3D('',#199893,#102650,#102651);
#85264=AXIS2_PLACEMENT_3D('',#199899,#102655,#102656);
#85265=AXIS2_PLACEMENT_3D('',#199902,#102659,#102660);
#85266=AXIS2_PLACEMENT_3D('',#199911,#102665,#102666);
#85267=AXIS2_PLACEMENT_3D('',#199917,#102670,#102671);
#85268=AXIS2_PLACEMENT_3D('',#199923,#102675,#102676);
#85269=AXIS2_PLACEMENT_3D('',#199926,#102679,#102680);
#85270=AXIS2_PLACEMENT_3D('',#199935,#102685,#102686);
#85271=AXIS2_PLACEMENT_3D('',#199941,#102690,#102691);
#85272=AXIS2_PLACEMENT_3D('',#199947,#102695,#102696);
#85273=AXIS2_PLACEMENT_3D('',#199950,#102699,#102700);
#85274=AXIS2_PLACEMENT_3D('',#199959,#102705,#102706);
#85275=AXIS2_PLACEMENT_3D('',#199965,#102710,#102711);
#85276=AXIS2_PLACEMENT_3D('',#199971,#102715,#102716);
#85277=AXIS2_PLACEMENT_3D('',#199974,#102719,#102720);
#85278=AXIS2_PLACEMENT_3D('',#199983,#102725,#102726);
#85279=AXIS2_PLACEMENT_3D('',#199989,#102730,#102731);
#85280=AXIS2_PLACEMENT_3D('',#199995,#102735,#102736);
#85281=AXIS2_PLACEMENT_3D('',#199998,#102739,#102740);
#85282=AXIS2_PLACEMENT_3D('',#200007,#102745,#102746);
#85283=AXIS2_PLACEMENT_3D('',#200013,#102750,#102751);
#85284=AXIS2_PLACEMENT_3D('',#200019,#102755,#102756);
#85285=AXIS2_PLACEMENT_3D('',#200022,#102759,#102760);
#85286=AXIS2_PLACEMENT_3D('',#200031,#102765,#102766);
#85287=AXIS2_PLACEMENT_3D('',#200037,#102770,#102771);
#85288=AXIS2_PLACEMENT_3D('',#200043,#102775,#102776);
#85289=AXIS2_PLACEMENT_3D('',#200046,#102779,#102780);
#85290=AXIS2_PLACEMENT_3D('',#200055,#102785,#102786);
#85291=AXIS2_PLACEMENT_3D('',#200061,#102790,#102791);
#85292=AXIS2_PLACEMENT_3D('',#200067,#102795,#102796);
#85293=AXIS2_PLACEMENT_3D('',#200070,#102799,#102800);
#85294=AXIS2_PLACEMENT_3D('',#200079,#102805,#102806);
#85295=AXIS2_PLACEMENT_3D('',#200085,#102810,#102811);
#85296=AXIS2_PLACEMENT_3D('',#200091,#102815,#102816);
#85297=AXIS2_PLACEMENT_3D('',#200094,#102819,#102820);
#85298=AXIS2_PLACEMENT_3D('',#200103,#102825,#102826);
#85299=AXIS2_PLACEMENT_3D('',#200109,#102830,#102831);
#85300=AXIS2_PLACEMENT_3D('',#200115,#102835,#102836);
#85301=AXIS2_PLACEMENT_3D('',#200118,#102839,#102840);
#85302=AXIS2_PLACEMENT_3D('',#200127,#102845,#102846);
#85303=AXIS2_PLACEMENT_3D('',#200133,#102850,#102851);
#85304=AXIS2_PLACEMENT_3D('',#200139,#102855,#102856);
#85305=AXIS2_PLACEMENT_3D('',#200142,#102859,#102860);
#85306=AXIS2_PLACEMENT_3D('',#200151,#102865,#102866);
#85307=AXIS2_PLACEMENT_3D('',#200157,#102870,#102871);
#85308=AXIS2_PLACEMENT_3D('',#200163,#102875,#102876);
#85309=AXIS2_PLACEMENT_3D('',#200166,#102879,#102880);
#85310=AXIS2_PLACEMENT_3D('',#200175,#102885,#102886);
#85311=AXIS2_PLACEMENT_3D('',#200181,#102890,#102891);
#85312=AXIS2_PLACEMENT_3D('',#200187,#102895,#102896);
#85313=AXIS2_PLACEMENT_3D('',#200190,#102899,#102900);
#85314=AXIS2_PLACEMENT_3D('',#200199,#102905,#102906);
#85315=AXIS2_PLACEMENT_3D('',#200205,#102910,#102911);
#85316=AXIS2_PLACEMENT_3D('',#200211,#102915,#102916);
#85317=AXIS2_PLACEMENT_3D('',#200214,#102919,#102920);
#85318=AXIS2_PLACEMENT_3D('',#200223,#102925,#102926);
#85319=AXIS2_PLACEMENT_3D('',#200229,#102930,#102931);
#85320=AXIS2_PLACEMENT_3D('',#200235,#102935,#102936);
#85321=AXIS2_PLACEMENT_3D('',#200238,#102939,#102940);
#85322=AXIS2_PLACEMENT_3D('',#200247,#102945,#102946);
#85323=AXIS2_PLACEMENT_3D('',#200253,#102950,#102951);
#85324=AXIS2_PLACEMENT_3D('',#200259,#102955,#102956);
#85325=AXIS2_PLACEMENT_3D('',#200262,#102959,#102960);
#85326=AXIS2_PLACEMENT_3D('',#200271,#102965,#102966);
#85327=AXIS2_PLACEMENT_3D('',#200277,#102970,#102971);
#85328=AXIS2_PLACEMENT_3D('',#200283,#102975,#102976);
#85329=AXIS2_PLACEMENT_3D('',#200286,#102979,#102980);
#85330=AXIS2_PLACEMENT_3D('',#200295,#102985,#102986);
#85331=AXIS2_PLACEMENT_3D('',#200301,#102990,#102991);
#85332=AXIS2_PLACEMENT_3D('',#200307,#102995,#102996);
#85333=AXIS2_PLACEMENT_3D('',#200310,#102999,#103000);
#85334=AXIS2_PLACEMENT_3D('',#200319,#103005,#103006);
#85335=AXIS2_PLACEMENT_3D('',#200325,#103010,#103011);
#85336=AXIS2_PLACEMENT_3D('',#200331,#103015,#103016);
#85337=AXIS2_PLACEMENT_3D('',#200334,#103019,#103020);
#85338=AXIS2_PLACEMENT_3D('',#200343,#103025,#103026);
#85339=AXIS2_PLACEMENT_3D('',#200349,#103030,#103031);
#85340=AXIS2_PLACEMENT_3D('',#200355,#103035,#103036);
#85341=AXIS2_PLACEMENT_3D('',#200358,#103039,#103040);
#85342=AXIS2_PLACEMENT_3D('',#200367,#103045,#103046);
#85343=AXIS2_PLACEMENT_3D('',#200373,#103050,#103051);
#85344=AXIS2_PLACEMENT_3D('',#200379,#103055,#103056);
#85345=AXIS2_PLACEMENT_3D('',#200382,#103059,#103060);
#85346=AXIS2_PLACEMENT_3D('',#200391,#103065,#103066);
#85347=AXIS2_PLACEMENT_3D('',#200397,#103070,#103071);
#85348=AXIS2_PLACEMENT_3D('',#200403,#103075,#103076);
#85349=AXIS2_PLACEMENT_3D('',#200406,#103079,#103080);
#85350=AXIS2_PLACEMENT_3D('',#200415,#103085,#103086);
#85351=AXIS2_PLACEMENT_3D('',#200421,#103090,#103091);
#85352=AXIS2_PLACEMENT_3D('',#200427,#103095,#103096);
#85353=AXIS2_PLACEMENT_3D('',#200430,#103099,#103100);
#85354=AXIS2_PLACEMENT_3D('',#200439,#103105,#103106);
#85355=AXIS2_PLACEMENT_3D('',#200445,#103110,#103111);
#85356=AXIS2_PLACEMENT_3D('',#200451,#103115,#103116);
#85357=AXIS2_PLACEMENT_3D('',#200454,#103119,#103120);
#85358=AXIS2_PLACEMENT_3D('',#200463,#103125,#103126);
#85359=AXIS2_PLACEMENT_3D('',#200469,#103130,#103131);
#85360=AXIS2_PLACEMENT_3D('',#200475,#103135,#103136);
#85361=AXIS2_PLACEMENT_3D('',#200478,#103139,#103140);
#85362=AXIS2_PLACEMENT_3D('',#200487,#103145,#103146);
#85363=AXIS2_PLACEMENT_3D('',#200493,#103150,#103151);
#85364=AXIS2_PLACEMENT_3D('',#200499,#103155,#103156);
#85365=AXIS2_PLACEMENT_3D('',#200502,#103159,#103160);
#85366=AXIS2_PLACEMENT_3D('',#200511,#103165,#103166);
#85367=AXIS2_PLACEMENT_3D('',#200517,#103170,#103171);
#85368=AXIS2_PLACEMENT_3D('',#200523,#103175,#103176);
#85369=AXIS2_PLACEMENT_3D('',#200526,#103179,#103180);
#85370=AXIS2_PLACEMENT_3D('',#200535,#103185,#103186);
#85371=AXIS2_PLACEMENT_3D('',#200541,#103190,#103191);
#85372=AXIS2_PLACEMENT_3D('',#200547,#103195,#103196);
#85373=AXIS2_PLACEMENT_3D('',#200550,#103199,#103200);
#85374=AXIS2_PLACEMENT_3D('',#200559,#103205,#103206);
#85375=AXIS2_PLACEMENT_3D('',#200565,#103210,#103211);
#85376=AXIS2_PLACEMENT_3D('',#200571,#103215,#103216);
#85377=AXIS2_PLACEMENT_3D('',#200574,#103219,#103220);
#85378=AXIS2_PLACEMENT_3D('',#200583,#103225,#103226);
#85379=AXIS2_PLACEMENT_3D('',#200589,#103230,#103231);
#85380=AXIS2_PLACEMENT_3D('',#200595,#103235,#103236);
#85381=AXIS2_PLACEMENT_3D('',#200598,#103239,#103240);
#85382=AXIS2_PLACEMENT_3D('',#200607,#103245,#103246);
#85383=AXIS2_PLACEMENT_3D('',#200613,#103250,#103251);
#85384=AXIS2_PLACEMENT_3D('',#200619,#103255,#103256);
#85385=AXIS2_PLACEMENT_3D('',#200622,#103259,#103260);
#85386=AXIS2_PLACEMENT_3D('',#200631,#103265,#103266);
#85387=AXIS2_PLACEMENT_3D('',#200637,#103270,#103271);
#85388=AXIS2_PLACEMENT_3D('',#200643,#103275,#103276);
#85389=AXIS2_PLACEMENT_3D('',#200646,#103279,#103280);
#85390=AXIS2_PLACEMENT_3D('',#200655,#103285,#103286);
#85391=AXIS2_PLACEMENT_3D('',#200661,#103290,#103291);
#85392=AXIS2_PLACEMENT_3D('',#200667,#103295,#103296);
#85393=AXIS2_PLACEMENT_3D('',#200670,#103299,#103300);
#85394=AXIS2_PLACEMENT_3D('',#200679,#103305,#103306);
#85395=AXIS2_PLACEMENT_3D('',#200685,#103310,#103311);
#85396=AXIS2_PLACEMENT_3D('',#200691,#103315,#103316);
#85397=AXIS2_PLACEMENT_3D('',#200694,#103319,#103320);
#85398=AXIS2_PLACEMENT_3D('',#200703,#103325,#103326);
#85399=AXIS2_PLACEMENT_3D('',#200709,#103330,#103331);
#85400=AXIS2_PLACEMENT_3D('',#200715,#103335,#103336);
#85401=AXIS2_PLACEMENT_3D('',#200718,#103339,#103340);
#85402=AXIS2_PLACEMENT_3D('',#200727,#103345,#103346);
#85403=AXIS2_PLACEMENT_3D('',#200733,#103350,#103351);
#85404=AXIS2_PLACEMENT_3D('',#200739,#103355,#103356);
#85405=AXIS2_PLACEMENT_3D('',#200742,#103359,#103360);
#85406=AXIS2_PLACEMENT_3D('',#200751,#103365,#103366);
#85407=AXIS2_PLACEMENT_3D('',#200757,#103370,#103371);
#85408=AXIS2_PLACEMENT_3D('',#200763,#103375,#103376);
#85409=AXIS2_PLACEMENT_3D('',#200766,#103379,#103380);
#85410=AXIS2_PLACEMENT_3D('',#200775,#103385,#103386);
#85411=AXIS2_PLACEMENT_3D('',#200781,#103390,#103391);
#85412=AXIS2_PLACEMENT_3D('',#200787,#103395,#103396);
#85413=AXIS2_PLACEMENT_3D('',#200790,#103399,#103400);
#85414=AXIS2_PLACEMENT_3D('',#200799,#103405,#103406);
#85415=AXIS2_PLACEMENT_3D('',#200805,#103410,#103411);
#85416=AXIS2_PLACEMENT_3D('',#200811,#103415,#103416);
#85417=AXIS2_PLACEMENT_3D('',#200814,#103419,#103420);
#85418=AXIS2_PLACEMENT_3D('',#200823,#103425,#103426);
#85419=AXIS2_PLACEMENT_3D('',#200829,#103430,#103431);
#85420=AXIS2_PLACEMENT_3D('',#200835,#103435,#103436);
#85421=AXIS2_PLACEMENT_3D('',#200838,#103439,#103440);
#85422=AXIS2_PLACEMENT_3D('',#200847,#103445,#103446);
#85423=AXIS2_PLACEMENT_3D('',#200853,#103450,#103451);
#85424=AXIS2_PLACEMENT_3D('',#200859,#103455,#103456);
#85425=AXIS2_PLACEMENT_3D('',#200862,#103459,#103460);
#85426=AXIS2_PLACEMENT_3D('',#200871,#103465,#103466);
#85427=AXIS2_PLACEMENT_3D('',#200877,#103470,#103471);
#85428=AXIS2_PLACEMENT_3D('',#200883,#103475,#103476);
#85429=AXIS2_PLACEMENT_3D('',#200886,#103479,#103480);
#85430=AXIS2_PLACEMENT_3D('',#200895,#103485,#103486);
#85431=AXIS2_PLACEMENT_3D('',#200901,#103490,#103491);
#85432=AXIS2_PLACEMENT_3D('',#200907,#103495,#103496);
#85433=AXIS2_PLACEMENT_3D('',#200910,#103499,#103500);
#85434=AXIS2_PLACEMENT_3D('',#200919,#103505,#103506);
#85435=AXIS2_PLACEMENT_3D('',#200925,#103510,#103511);
#85436=AXIS2_PLACEMENT_3D('',#200931,#103515,#103516);
#85437=AXIS2_PLACEMENT_3D('',#200934,#103519,#103520);
#85438=AXIS2_PLACEMENT_3D('',#200943,#103525,#103526);
#85439=AXIS2_PLACEMENT_3D('',#200949,#103530,#103531);
#85440=AXIS2_PLACEMENT_3D('',#200955,#103535,#103536);
#85441=AXIS2_PLACEMENT_3D('',#200958,#103539,#103540);
#85442=AXIS2_PLACEMENT_3D('',#200967,#103545,#103546);
#85443=AXIS2_PLACEMENT_3D('',#200973,#103550,#103551);
#85444=AXIS2_PLACEMENT_3D('',#200979,#103555,#103556);
#85445=AXIS2_PLACEMENT_3D('',#200982,#103559,#103560);
#85446=AXIS2_PLACEMENT_3D('',#200991,#103565,#103566);
#85447=AXIS2_PLACEMENT_3D('',#200997,#103570,#103571);
#85448=AXIS2_PLACEMENT_3D('',#201003,#103575,#103576);
#85449=AXIS2_PLACEMENT_3D('',#201006,#103579,#103580);
#85450=AXIS2_PLACEMENT_3D('',#201015,#103585,#103586);
#85451=AXIS2_PLACEMENT_3D('',#201021,#103590,#103591);
#85452=AXIS2_PLACEMENT_3D('',#201027,#103595,#103596);
#85453=AXIS2_PLACEMENT_3D('',#201030,#103599,#103600);
#85454=AXIS2_PLACEMENT_3D('',#201039,#103605,#103606);
#85455=AXIS2_PLACEMENT_3D('',#201045,#103610,#103611);
#85456=AXIS2_PLACEMENT_3D('',#201051,#103615,#103616);
#85457=AXIS2_PLACEMENT_3D('',#201054,#103619,#103620);
#85458=AXIS2_PLACEMENT_3D('',#201063,#103625,#103626);
#85459=AXIS2_PLACEMENT_3D('',#201069,#103630,#103631);
#85460=AXIS2_PLACEMENT_3D('',#201075,#103635,#103636);
#85461=AXIS2_PLACEMENT_3D('',#201078,#103639,#103640);
#85462=AXIS2_PLACEMENT_3D('',#201087,#103645,#103646);
#85463=AXIS2_PLACEMENT_3D('',#201093,#103650,#103651);
#85464=AXIS2_PLACEMENT_3D('',#201099,#103655,#103656);
#85465=AXIS2_PLACEMENT_3D('',#201102,#103659,#103660);
#85466=AXIS2_PLACEMENT_3D('',#201111,#103665,#103666);
#85467=AXIS2_PLACEMENT_3D('',#201117,#103670,#103671);
#85468=AXIS2_PLACEMENT_3D('',#201123,#103675,#103676);
#85469=AXIS2_PLACEMENT_3D('',#201126,#103679,#103680);
#85470=AXIS2_PLACEMENT_3D('',#201135,#103685,#103686);
#85471=AXIS2_PLACEMENT_3D('',#201141,#103690,#103691);
#85472=AXIS2_PLACEMENT_3D('',#201147,#103695,#103696);
#85473=AXIS2_PLACEMENT_3D('',#201150,#103699,#103700);
#85474=AXIS2_PLACEMENT_3D('',#201159,#103705,#103706);
#85475=AXIS2_PLACEMENT_3D('',#201165,#103710,#103711);
#85476=AXIS2_PLACEMENT_3D('',#201171,#103715,#103716);
#85477=AXIS2_PLACEMENT_3D('',#201174,#103719,#103720);
#85478=AXIS2_PLACEMENT_3D('',#201183,#103725,#103726);
#85479=AXIS2_PLACEMENT_3D('',#201189,#103730,#103731);
#85480=AXIS2_PLACEMENT_3D('',#201195,#103735,#103736);
#85481=AXIS2_PLACEMENT_3D('',#201198,#103739,#103740);
#85482=AXIS2_PLACEMENT_3D('',#201207,#103745,#103746);
#85483=AXIS2_PLACEMENT_3D('',#201213,#103750,#103751);
#85484=AXIS2_PLACEMENT_3D('',#201219,#103755,#103756);
#85485=AXIS2_PLACEMENT_3D('',#201222,#103759,#103760);
#85486=AXIS2_PLACEMENT_3D('',#201231,#103765,#103766);
#85487=AXIS2_PLACEMENT_3D('',#201237,#103770,#103771);
#85488=AXIS2_PLACEMENT_3D('',#201243,#103775,#103776);
#85489=AXIS2_PLACEMENT_3D('',#201246,#103779,#103780);
#85490=AXIS2_PLACEMENT_3D('',#201255,#103785,#103786);
#85491=AXIS2_PLACEMENT_3D('',#201261,#103790,#103791);
#85492=AXIS2_PLACEMENT_3D('',#201267,#103795,#103796);
#85493=AXIS2_PLACEMENT_3D('',#201270,#103799,#103800);
#85494=AXIS2_PLACEMENT_3D('',#201279,#103805,#103806);
#85495=AXIS2_PLACEMENT_3D('',#201285,#103810,#103811);
#85496=AXIS2_PLACEMENT_3D('',#201291,#103815,#103816);
#85497=AXIS2_PLACEMENT_3D('',#201294,#103819,#103820);
#85498=AXIS2_PLACEMENT_3D('',#201303,#103825,#103826);
#85499=AXIS2_PLACEMENT_3D('',#201309,#103830,#103831);
#85500=AXIS2_PLACEMENT_3D('',#201315,#103835,#103836);
#85501=AXIS2_PLACEMENT_3D('',#201318,#103839,#103840);
#85502=AXIS2_PLACEMENT_3D('',#201327,#103845,#103846);
#85503=AXIS2_PLACEMENT_3D('',#201333,#103850,#103851);
#85504=AXIS2_PLACEMENT_3D('',#201339,#103855,#103856);
#85505=AXIS2_PLACEMENT_3D('',#201342,#103859,#103860);
#85506=AXIS2_PLACEMENT_3D('',#201351,#103865,#103866);
#85507=AXIS2_PLACEMENT_3D('',#201357,#103870,#103871);
#85508=AXIS2_PLACEMENT_3D('',#201363,#103875,#103876);
#85509=AXIS2_PLACEMENT_3D('',#201366,#103879,#103880);
#85510=AXIS2_PLACEMENT_3D('',#201375,#103885,#103886);
#85511=AXIS2_PLACEMENT_3D('',#201381,#103890,#103891);
#85512=AXIS2_PLACEMENT_3D('',#201387,#103895,#103896);
#85513=AXIS2_PLACEMENT_3D('',#201390,#103899,#103900);
#85514=AXIS2_PLACEMENT_3D('',#201399,#103905,#103906);
#85515=AXIS2_PLACEMENT_3D('',#201405,#103910,#103911);
#85516=AXIS2_PLACEMENT_3D('',#201411,#103915,#103916);
#85517=AXIS2_PLACEMENT_3D('',#201414,#103919,#103920);
#85518=AXIS2_PLACEMENT_3D('',#201423,#103925,#103926);
#85519=AXIS2_PLACEMENT_3D('',#201429,#103930,#103931);
#85520=AXIS2_PLACEMENT_3D('',#201435,#103935,#103936);
#85521=AXIS2_PLACEMENT_3D('',#201438,#103939,#103940);
#85522=AXIS2_PLACEMENT_3D('',#201447,#103945,#103946);
#85523=AXIS2_PLACEMENT_3D('',#201453,#103950,#103951);
#85524=AXIS2_PLACEMENT_3D('',#201459,#103955,#103956);
#85525=AXIS2_PLACEMENT_3D('',#201462,#103959,#103960);
#85526=AXIS2_PLACEMENT_3D('',#201471,#103965,#103966);
#85527=AXIS2_PLACEMENT_3D('',#201477,#103970,#103971);
#85528=AXIS2_PLACEMENT_3D('',#201483,#103975,#103976);
#85529=AXIS2_PLACEMENT_3D('',#201486,#103979,#103980);
#85530=AXIS2_PLACEMENT_3D('',#201495,#103985,#103986);
#85531=AXIS2_PLACEMENT_3D('',#201501,#103990,#103991);
#85532=AXIS2_PLACEMENT_3D('',#201507,#103995,#103996);
#85533=AXIS2_PLACEMENT_3D('',#201510,#103999,#104000);
#85534=AXIS2_PLACEMENT_3D('',#201519,#104005,#104006);
#85535=AXIS2_PLACEMENT_3D('',#201525,#104010,#104011);
#85536=AXIS2_PLACEMENT_3D('',#201531,#104015,#104016);
#85537=AXIS2_PLACEMENT_3D('',#201534,#104019,#104020);
#85538=AXIS2_PLACEMENT_3D('',#201543,#104025,#104026);
#85539=AXIS2_PLACEMENT_3D('',#201549,#104030,#104031);
#85540=AXIS2_PLACEMENT_3D('',#201555,#104035,#104036);
#85541=AXIS2_PLACEMENT_3D('',#201558,#104039,#104040);
#85542=AXIS2_PLACEMENT_3D('',#201567,#104045,#104046);
#85543=AXIS2_PLACEMENT_3D('',#201573,#104050,#104051);
#85544=AXIS2_PLACEMENT_3D('',#201579,#104055,#104056);
#85545=AXIS2_PLACEMENT_3D('',#201582,#104059,#104060);
#85546=AXIS2_PLACEMENT_3D('',#201591,#104065,#104066);
#85547=AXIS2_PLACEMENT_3D('',#201597,#104070,#104071);
#85548=AXIS2_PLACEMENT_3D('',#201603,#104075,#104076);
#85549=AXIS2_PLACEMENT_3D('',#201606,#104079,#104080);
#85550=AXIS2_PLACEMENT_3D('',#201615,#104085,#104086);
#85551=AXIS2_PLACEMENT_3D('',#201621,#104090,#104091);
#85552=AXIS2_PLACEMENT_3D('',#201627,#104095,#104096);
#85553=AXIS2_PLACEMENT_3D('',#201630,#104099,#104100);
#85554=AXIS2_PLACEMENT_3D('',#201639,#104105,#104106);
#85555=AXIS2_PLACEMENT_3D('',#201645,#104110,#104111);
#85556=AXIS2_PLACEMENT_3D('',#201651,#104115,#104116);
#85557=AXIS2_PLACEMENT_3D('',#201654,#104119,#104120);
#85558=AXIS2_PLACEMENT_3D('',#201663,#104125,#104126);
#85559=AXIS2_PLACEMENT_3D('',#201669,#104130,#104131);
#85560=AXIS2_PLACEMENT_3D('',#201675,#104135,#104136);
#85561=AXIS2_PLACEMENT_3D('',#201678,#104139,#104140);
#85562=AXIS2_PLACEMENT_3D('',#201687,#104145,#104146);
#85563=AXIS2_PLACEMENT_3D('',#201693,#104150,#104151);
#85564=AXIS2_PLACEMENT_3D('',#201699,#104155,#104156);
#85565=AXIS2_PLACEMENT_3D('',#201702,#104159,#104160);
#85566=AXIS2_PLACEMENT_3D('',#201711,#104165,#104166);
#85567=AXIS2_PLACEMENT_3D('',#201717,#104170,#104171);
#85568=AXIS2_PLACEMENT_3D('',#201723,#104175,#104176);
#85569=AXIS2_PLACEMENT_3D('',#201726,#104179,#104180);
#85570=AXIS2_PLACEMENT_3D('',#201735,#104185,#104186);
#85571=AXIS2_PLACEMENT_3D('',#201741,#104190,#104191);
#85572=AXIS2_PLACEMENT_3D('',#201747,#104195,#104196);
#85573=AXIS2_PLACEMENT_3D('',#201750,#104199,#104200);
#85574=AXIS2_PLACEMENT_3D('',#201759,#104205,#104206);
#85575=AXIS2_PLACEMENT_3D('',#201765,#104210,#104211);
#85576=AXIS2_PLACEMENT_3D('',#201771,#104215,#104216);
#85577=AXIS2_PLACEMENT_3D('',#201774,#104219,#104220);
#85578=AXIS2_PLACEMENT_3D('',#201783,#104225,#104226);
#85579=AXIS2_PLACEMENT_3D('',#201789,#104230,#104231);
#85580=AXIS2_PLACEMENT_3D('',#201795,#104235,#104236);
#85581=AXIS2_PLACEMENT_3D('',#201798,#104239,#104240);
#85582=AXIS2_PLACEMENT_3D('',#201807,#104245,#104246);
#85583=AXIS2_PLACEMENT_3D('',#201813,#104250,#104251);
#85584=AXIS2_PLACEMENT_3D('',#201819,#104255,#104256);
#85585=AXIS2_PLACEMENT_3D('',#201822,#104259,#104260);
#85586=AXIS2_PLACEMENT_3D('',#201831,#104265,#104266);
#85587=AXIS2_PLACEMENT_3D('',#201837,#104270,#104271);
#85588=AXIS2_PLACEMENT_3D('',#201843,#104275,#104276);
#85589=AXIS2_PLACEMENT_3D('',#201846,#104279,#104280);
#85590=AXIS2_PLACEMENT_3D('',#201855,#104285,#104286);
#85591=AXIS2_PLACEMENT_3D('',#201861,#104290,#104291);
#85592=AXIS2_PLACEMENT_3D('',#201867,#104295,#104296);
#85593=AXIS2_PLACEMENT_3D('',#201870,#104299,#104300);
#85594=AXIS2_PLACEMENT_3D('',#201879,#104305,#104306);
#85595=AXIS2_PLACEMENT_3D('',#201885,#104310,#104311);
#85596=AXIS2_PLACEMENT_3D('',#201891,#104315,#104316);
#85597=AXIS2_PLACEMENT_3D('',#201894,#104319,#104320);
#85598=AXIS2_PLACEMENT_3D('',#201903,#104325,#104326);
#85599=AXIS2_PLACEMENT_3D('',#201909,#104330,#104331);
#85600=AXIS2_PLACEMENT_3D('',#201915,#104335,#104336);
#85601=AXIS2_PLACEMENT_3D('',#201918,#104339,#104340);
#85602=AXIS2_PLACEMENT_3D('',#201927,#104345,#104346);
#85603=AXIS2_PLACEMENT_3D('',#201933,#104350,#104351);
#85604=AXIS2_PLACEMENT_3D('',#201939,#104355,#104356);
#85605=AXIS2_PLACEMENT_3D('',#201942,#104359,#104360);
#85606=AXIS2_PLACEMENT_3D('',#201951,#104365,#104366);
#85607=AXIS2_PLACEMENT_3D('',#201957,#104370,#104371);
#85608=AXIS2_PLACEMENT_3D('',#201963,#104375,#104376);
#85609=AXIS2_PLACEMENT_3D('',#201966,#104379,#104380);
#85610=AXIS2_PLACEMENT_3D('',#201975,#104385,#104386);
#85611=AXIS2_PLACEMENT_3D('',#201981,#104390,#104391);
#85612=AXIS2_PLACEMENT_3D('',#201987,#104395,#104396);
#85613=AXIS2_PLACEMENT_3D('',#201990,#104399,#104400);
#85614=AXIS2_PLACEMENT_3D('',#201999,#104405,#104406);
#85615=AXIS2_PLACEMENT_3D('',#202005,#104410,#104411);
#85616=AXIS2_PLACEMENT_3D('',#202011,#104415,#104416);
#85617=AXIS2_PLACEMENT_3D('',#202014,#104419,#104420);
#85618=AXIS2_PLACEMENT_3D('',#202023,#104425,#104426);
#85619=AXIS2_PLACEMENT_3D('',#202029,#104430,#104431);
#85620=AXIS2_PLACEMENT_3D('',#202035,#104435,#104436);
#85621=AXIS2_PLACEMENT_3D('',#202038,#104439,#104440);
#85622=AXIS2_PLACEMENT_3D('',#202047,#104445,#104446);
#85623=AXIS2_PLACEMENT_3D('',#202053,#104450,#104451);
#85624=AXIS2_PLACEMENT_3D('',#202059,#104455,#104456);
#85625=AXIS2_PLACEMENT_3D('',#202062,#104459,#104460);
#85626=AXIS2_PLACEMENT_3D('',#202071,#104465,#104466);
#85627=AXIS2_PLACEMENT_3D('',#202077,#104470,#104471);
#85628=AXIS2_PLACEMENT_3D('',#202083,#104475,#104476);
#85629=AXIS2_PLACEMENT_3D('',#202086,#104479,#104480);
#85630=AXIS2_PLACEMENT_3D('',#202095,#104485,#104486);
#85631=AXIS2_PLACEMENT_3D('',#202101,#104490,#104491);
#85632=AXIS2_PLACEMENT_3D('',#202107,#104495,#104496);
#85633=AXIS2_PLACEMENT_3D('',#202110,#104499,#104500);
#85634=AXIS2_PLACEMENT_3D('',#202119,#104505,#104506);
#85635=AXIS2_PLACEMENT_3D('',#202125,#104510,#104511);
#85636=AXIS2_PLACEMENT_3D('',#202131,#104515,#104516);
#85637=AXIS2_PLACEMENT_3D('',#202134,#104519,#104520);
#85638=AXIS2_PLACEMENT_3D('',#202143,#104525,#104526);
#85639=AXIS2_PLACEMENT_3D('',#202149,#104530,#104531);
#85640=AXIS2_PLACEMENT_3D('',#202155,#104535,#104536);
#85641=AXIS2_PLACEMENT_3D('',#202158,#104539,#104540);
#85642=AXIS2_PLACEMENT_3D('',#202167,#104545,#104546);
#85643=AXIS2_PLACEMENT_3D('',#202173,#104550,#104551);
#85644=AXIS2_PLACEMENT_3D('',#202179,#104555,#104556);
#85645=AXIS2_PLACEMENT_3D('',#202182,#104559,#104560);
#85646=AXIS2_PLACEMENT_3D('',#202191,#104565,#104566);
#85647=AXIS2_PLACEMENT_3D('',#202197,#104570,#104571);
#85648=AXIS2_PLACEMENT_3D('',#202203,#104575,#104576);
#85649=AXIS2_PLACEMENT_3D('',#202206,#104579,#104580);
#85650=AXIS2_PLACEMENT_3D('',#202215,#104585,#104586);
#85651=AXIS2_PLACEMENT_3D('',#202221,#104590,#104591);
#85652=AXIS2_PLACEMENT_3D('',#202227,#104595,#104596);
#85653=AXIS2_PLACEMENT_3D('',#202230,#104599,#104600);
#85654=AXIS2_PLACEMENT_3D('',#202239,#104605,#104606);
#85655=AXIS2_PLACEMENT_3D('',#202245,#104610,#104611);
#85656=AXIS2_PLACEMENT_3D('',#202251,#104615,#104616);
#85657=AXIS2_PLACEMENT_3D('',#202254,#104619,#104620);
#85658=AXIS2_PLACEMENT_3D('',#202263,#104625,#104626);
#85659=AXIS2_PLACEMENT_3D('',#202269,#104630,#104631);
#85660=AXIS2_PLACEMENT_3D('',#202275,#104635,#104636);
#85661=AXIS2_PLACEMENT_3D('',#202278,#104639,#104640);
#85662=AXIS2_PLACEMENT_3D('',#202287,#104645,#104646);
#85663=AXIS2_PLACEMENT_3D('',#202293,#104650,#104651);
#85664=AXIS2_PLACEMENT_3D('',#202299,#104655,#104656);
#85665=AXIS2_PLACEMENT_3D('',#202302,#104659,#104660);
#85666=AXIS2_PLACEMENT_3D('',#202311,#104665,#104666);
#85667=AXIS2_PLACEMENT_3D('',#202317,#104670,#104671);
#85668=AXIS2_PLACEMENT_3D('',#202323,#104675,#104676);
#85669=AXIS2_PLACEMENT_3D('',#202326,#104679,#104680);
#85670=AXIS2_PLACEMENT_3D('',#202335,#104685,#104686);
#85671=AXIS2_PLACEMENT_3D('',#202341,#104690,#104691);
#85672=AXIS2_PLACEMENT_3D('',#202347,#104695,#104696);
#85673=AXIS2_PLACEMENT_3D('',#202350,#104699,#104700);
#85674=AXIS2_PLACEMENT_3D('',#202359,#104705,#104706);
#85675=AXIS2_PLACEMENT_3D('',#202365,#104710,#104711);
#85676=AXIS2_PLACEMENT_3D('',#202371,#104715,#104716);
#85677=AXIS2_PLACEMENT_3D('',#202374,#104719,#104720);
#85678=AXIS2_PLACEMENT_3D('',#202383,#104725,#104726);
#85679=AXIS2_PLACEMENT_3D('',#202389,#104730,#104731);
#85680=AXIS2_PLACEMENT_3D('',#202395,#104735,#104736);
#85681=AXIS2_PLACEMENT_3D('',#202398,#104739,#104740);
#85682=AXIS2_PLACEMENT_3D('',#202407,#104745,#104746);
#85683=AXIS2_PLACEMENT_3D('',#202413,#104750,#104751);
#85684=AXIS2_PLACEMENT_3D('',#202419,#104755,#104756);
#85685=AXIS2_PLACEMENT_3D('',#202422,#104759,#104760);
#85686=AXIS2_PLACEMENT_3D('',#202431,#104765,#104766);
#85687=AXIS2_PLACEMENT_3D('',#202437,#104770,#104771);
#85688=AXIS2_PLACEMENT_3D('',#202443,#104775,#104776);
#85689=AXIS2_PLACEMENT_3D('',#202446,#104779,#104780);
#85690=AXIS2_PLACEMENT_3D('',#202455,#104785,#104786);
#85691=AXIS2_PLACEMENT_3D('',#202461,#104790,#104791);
#85692=AXIS2_PLACEMENT_3D('',#202467,#104795,#104796);
#85693=AXIS2_PLACEMENT_3D('',#202470,#104799,#104800);
#85694=AXIS2_PLACEMENT_3D('',#202479,#104805,#104806);
#85695=AXIS2_PLACEMENT_3D('',#202485,#104810,#104811);
#85696=AXIS2_PLACEMENT_3D('',#202491,#104815,#104816);
#85697=AXIS2_PLACEMENT_3D('',#202494,#104819,#104820);
#85698=AXIS2_PLACEMENT_3D('',#202503,#104825,#104826);
#85699=AXIS2_PLACEMENT_3D('',#202509,#104830,#104831);
#85700=AXIS2_PLACEMENT_3D('',#202515,#104835,#104836);
#85701=AXIS2_PLACEMENT_3D('',#202518,#104839,#104840);
#85702=AXIS2_PLACEMENT_3D('',#202527,#104845,#104846);
#85703=AXIS2_PLACEMENT_3D('',#202533,#104850,#104851);
#85704=AXIS2_PLACEMENT_3D('',#202539,#104855,#104856);
#85705=AXIS2_PLACEMENT_3D('',#202542,#104859,#104860);
#85706=AXIS2_PLACEMENT_3D('',#202551,#104865,#104866);
#85707=AXIS2_PLACEMENT_3D('',#202557,#104870,#104871);
#85708=AXIS2_PLACEMENT_3D('',#202563,#104875,#104876);
#85709=AXIS2_PLACEMENT_3D('',#202566,#104879,#104880);
#85710=AXIS2_PLACEMENT_3D('',#202575,#104885,#104886);
#85711=AXIS2_PLACEMENT_3D('',#202581,#104890,#104891);
#85712=AXIS2_PLACEMENT_3D('',#202587,#104895,#104896);
#85713=AXIS2_PLACEMENT_3D('',#202590,#104899,#104900);
#85714=AXIS2_PLACEMENT_3D('',#202599,#104905,#104906);
#85715=AXIS2_PLACEMENT_3D('',#202605,#104910,#104911);
#85716=AXIS2_PLACEMENT_3D('',#202611,#104915,#104916);
#85717=AXIS2_PLACEMENT_3D('',#202614,#104919,#104920);
#85718=AXIS2_PLACEMENT_3D('',#202623,#104925,#104926);
#85719=AXIS2_PLACEMENT_3D('',#202629,#104930,#104931);
#85720=AXIS2_PLACEMENT_3D('',#202635,#104935,#104936);
#85721=AXIS2_PLACEMENT_3D('',#202638,#104939,#104940);
#85722=AXIS2_PLACEMENT_3D('',#202647,#104945,#104946);
#85723=AXIS2_PLACEMENT_3D('',#202653,#104950,#104951);
#85724=AXIS2_PLACEMENT_3D('',#202659,#104955,#104956);
#85725=AXIS2_PLACEMENT_3D('',#202662,#104959,#104960);
#85726=AXIS2_PLACEMENT_3D('',#202671,#104965,#104966);
#85727=AXIS2_PLACEMENT_3D('',#202677,#104970,#104971);
#85728=AXIS2_PLACEMENT_3D('',#202683,#104975,#104976);
#85729=AXIS2_PLACEMENT_3D('',#202686,#104979,#104980);
#85730=AXIS2_PLACEMENT_3D('',#202695,#104985,#104986);
#85731=AXIS2_PLACEMENT_3D('',#202701,#104990,#104991);
#85732=AXIS2_PLACEMENT_3D('',#202707,#104995,#104996);
#85733=AXIS2_PLACEMENT_3D('',#202710,#104999,#105000);
#85734=AXIS2_PLACEMENT_3D('',#202719,#105005,#105006);
#85735=AXIS2_PLACEMENT_3D('',#202725,#105010,#105011);
#85736=AXIS2_PLACEMENT_3D('',#202731,#105015,#105016);
#85737=AXIS2_PLACEMENT_3D('',#202734,#105019,#105020);
#85738=AXIS2_PLACEMENT_3D('',#202743,#105025,#105026);
#85739=AXIS2_PLACEMENT_3D('',#202749,#105030,#105031);
#85740=AXIS2_PLACEMENT_3D('',#202755,#105035,#105036);
#85741=AXIS2_PLACEMENT_3D('',#202758,#105039,#105040);
#85742=AXIS2_PLACEMENT_3D('',#202767,#105045,#105046);
#85743=AXIS2_PLACEMENT_3D('',#202773,#105050,#105051);
#85744=AXIS2_PLACEMENT_3D('',#202779,#105055,#105056);
#85745=AXIS2_PLACEMENT_3D('',#202782,#105059,#105060);
#85746=AXIS2_PLACEMENT_3D('',#202791,#105065,#105066);
#85747=AXIS2_PLACEMENT_3D('',#202797,#105070,#105071);
#85748=AXIS2_PLACEMENT_3D('',#202803,#105075,#105076);
#85749=AXIS2_PLACEMENT_3D('',#202806,#105079,#105080);
#85750=AXIS2_PLACEMENT_3D('',#202815,#105085,#105086);
#85751=AXIS2_PLACEMENT_3D('',#202821,#105090,#105091);
#85752=AXIS2_PLACEMENT_3D('',#202827,#105095,#105096);
#85753=AXIS2_PLACEMENT_3D('',#202830,#105099,#105100);
#85754=AXIS2_PLACEMENT_3D('',#202839,#105105,#105106);
#85755=AXIS2_PLACEMENT_3D('',#202845,#105110,#105111);
#85756=AXIS2_PLACEMENT_3D('',#202851,#105115,#105116);
#85757=AXIS2_PLACEMENT_3D('',#202854,#105119,#105120);
#85758=AXIS2_PLACEMENT_3D('',#202863,#105125,#105126);
#85759=AXIS2_PLACEMENT_3D('',#202869,#105130,#105131);
#85760=AXIS2_PLACEMENT_3D('',#202875,#105135,#105136);
#85761=AXIS2_PLACEMENT_3D('',#202878,#105139,#105140);
#85762=AXIS2_PLACEMENT_3D('',#202887,#105145,#105146);
#85763=AXIS2_PLACEMENT_3D('',#202893,#105150,#105151);
#85764=AXIS2_PLACEMENT_3D('',#202899,#105155,#105156);
#85765=AXIS2_PLACEMENT_3D('',#202902,#105159,#105160);
#85766=AXIS2_PLACEMENT_3D('',#202911,#105165,#105166);
#85767=AXIS2_PLACEMENT_3D('',#202917,#105170,#105171);
#85768=AXIS2_PLACEMENT_3D('',#202923,#105175,#105176);
#85769=AXIS2_PLACEMENT_3D('',#202926,#105179,#105180);
#85770=AXIS2_PLACEMENT_3D('',#202935,#105185,#105186);
#85771=AXIS2_PLACEMENT_3D('',#202941,#105190,#105191);
#85772=AXIS2_PLACEMENT_3D('',#202947,#105195,#105196);
#85773=AXIS2_PLACEMENT_3D('',#202950,#105199,#105200);
#85774=AXIS2_PLACEMENT_3D('',#202959,#105205,#105206);
#85775=AXIS2_PLACEMENT_3D('',#202965,#105210,#105211);
#85776=AXIS2_PLACEMENT_3D('',#202971,#105215,#105216);
#85777=AXIS2_PLACEMENT_3D('',#202974,#105219,#105220);
#85778=AXIS2_PLACEMENT_3D('',#202983,#105225,#105226);
#85779=AXIS2_PLACEMENT_3D('',#202989,#105230,#105231);
#85780=AXIS2_PLACEMENT_3D('',#202995,#105235,#105236);
#85781=AXIS2_PLACEMENT_3D('',#202998,#105239,#105240);
#85782=AXIS2_PLACEMENT_3D('',#203007,#105245,#105246);
#85783=AXIS2_PLACEMENT_3D('',#203013,#105250,#105251);
#85784=AXIS2_PLACEMENT_3D('',#203019,#105255,#105256);
#85785=AXIS2_PLACEMENT_3D('',#203022,#105259,#105260);
#85786=AXIS2_PLACEMENT_3D('',#203031,#105265,#105266);
#85787=AXIS2_PLACEMENT_3D('',#203037,#105270,#105271);
#85788=AXIS2_PLACEMENT_3D('',#203043,#105275,#105276);
#85789=AXIS2_PLACEMENT_3D('',#203046,#105279,#105280);
#85790=AXIS2_PLACEMENT_3D('',#203055,#105285,#105286);
#85791=AXIS2_PLACEMENT_3D('',#203061,#105290,#105291);
#85792=AXIS2_PLACEMENT_3D('',#203067,#105295,#105296);
#85793=AXIS2_PLACEMENT_3D('',#203070,#105299,#105300);
#85794=AXIS2_PLACEMENT_3D('',#203079,#105305,#105306);
#85795=AXIS2_PLACEMENT_3D('',#203085,#105310,#105311);
#85796=AXIS2_PLACEMENT_3D('',#203091,#105315,#105316);
#85797=AXIS2_PLACEMENT_3D('',#203094,#105319,#105320);
#85798=AXIS2_PLACEMENT_3D('',#203103,#105325,#105326);
#85799=AXIS2_PLACEMENT_3D('',#203109,#105330,#105331);
#85800=AXIS2_PLACEMENT_3D('',#203115,#105335,#105336);
#85801=AXIS2_PLACEMENT_3D('',#203118,#105339,#105340);
#85802=AXIS2_PLACEMENT_3D('',#203127,#105345,#105346);
#85803=AXIS2_PLACEMENT_3D('',#203133,#105350,#105351);
#85804=AXIS2_PLACEMENT_3D('',#203139,#105355,#105356);
#85805=AXIS2_PLACEMENT_3D('',#203142,#105359,#105360);
#85806=AXIS2_PLACEMENT_3D('',#203151,#105365,#105366);
#85807=AXIS2_PLACEMENT_3D('',#203157,#105370,#105371);
#85808=AXIS2_PLACEMENT_3D('',#203163,#105375,#105376);
#85809=AXIS2_PLACEMENT_3D('',#203166,#105379,#105380);
#85810=AXIS2_PLACEMENT_3D('',#203175,#105385,#105386);
#85811=AXIS2_PLACEMENT_3D('',#203181,#105390,#105391);
#85812=AXIS2_PLACEMENT_3D('',#203187,#105395,#105396);
#85813=AXIS2_PLACEMENT_3D('',#203190,#105399,#105400);
#85814=AXIS2_PLACEMENT_3D('',#203199,#105405,#105406);
#85815=AXIS2_PLACEMENT_3D('',#203205,#105410,#105411);
#85816=AXIS2_PLACEMENT_3D('',#203211,#105415,#105416);
#85817=AXIS2_PLACEMENT_3D('',#203214,#105419,#105420);
#85818=AXIS2_PLACEMENT_3D('',#203223,#105425,#105426);
#85819=AXIS2_PLACEMENT_3D('',#203229,#105430,#105431);
#85820=AXIS2_PLACEMENT_3D('',#203235,#105435,#105436);
#85821=AXIS2_PLACEMENT_3D('',#203238,#105439,#105440);
#85822=AXIS2_PLACEMENT_3D('',#203247,#105445,#105446);
#85823=AXIS2_PLACEMENT_3D('',#203253,#105450,#105451);
#85824=AXIS2_PLACEMENT_3D('',#203259,#105455,#105456);
#85825=AXIS2_PLACEMENT_3D('',#203262,#105459,#105460);
#85826=AXIS2_PLACEMENT_3D('',#203271,#105465,#105466);
#85827=AXIS2_PLACEMENT_3D('',#203277,#105470,#105471);
#85828=AXIS2_PLACEMENT_3D('',#203283,#105475,#105476);
#85829=AXIS2_PLACEMENT_3D('',#203286,#105479,#105480);
#85830=AXIS2_PLACEMENT_3D('',#203295,#105485,#105486);
#85831=AXIS2_PLACEMENT_3D('',#203301,#105490,#105491);
#85832=AXIS2_PLACEMENT_3D('',#203307,#105495,#105496);
#85833=AXIS2_PLACEMENT_3D('',#203310,#105499,#105500);
#85834=AXIS2_PLACEMENT_3D('',#203319,#105505,#105506);
#85835=AXIS2_PLACEMENT_3D('',#203325,#105510,#105511);
#85836=AXIS2_PLACEMENT_3D('',#203331,#105515,#105516);
#85837=AXIS2_PLACEMENT_3D('',#203334,#105519,#105520);
#85838=AXIS2_PLACEMENT_3D('',#203343,#105525,#105526);
#85839=AXIS2_PLACEMENT_3D('',#203349,#105530,#105531);
#85840=AXIS2_PLACEMENT_3D('',#203355,#105535,#105536);
#85841=AXIS2_PLACEMENT_3D('',#203358,#105539,#105540);
#85842=AXIS2_PLACEMENT_3D('',#203367,#105545,#105546);
#85843=AXIS2_PLACEMENT_3D('',#203373,#105550,#105551);
#85844=AXIS2_PLACEMENT_3D('',#203379,#105555,#105556);
#85845=AXIS2_PLACEMENT_3D('',#203382,#105559,#105560);
#85846=AXIS2_PLACEMENT_3D('',#203391,#105565,#105566);
#85847=AXIS2_PLACEMENT_3D('',#203397,#105570,#105571);
#85848=AXIS2_PLACEMENT_3D('',#203403,#105575,#105576);
#85849=AXIS2_PLACEMENT_3D('',#203406,#105579,#105580);
#85850=AXIS2_PLACEMENT_3D('',#203415,#105585,#105586);
#85851=AXIS2_PLACEMENT_3D('',#203421,#105590,#105591);
#85852=AXIS2_PLACEMENT_3D('',#203427,#105595,#105596);
#85853=AXIS2_PLACEMENT_3D('',#203430,#105599,#105600);
#85854=AXIS2_PLACEMENT_3D('',#203439,#105605,#105606);
#85855=AXIS2_PLACEMENT_3D('',#203445,#105610,#105611);
#85856=AXIS2_PLACEMENT_3D('',#203451,#105615,#105616);
#85857=AXIS2_PLACEMENT_3D('',#203454,#105619,#105620);
#85858=AXIS2_PLACEMENT_3D('',#203463,#105625,#105626);
#85859=AXIS2_PLACEMENT_3D('',#203469,#105630,#105631);
#85860=AXIS2_PLACEMENT_3D('',#203475,#105635,#105636);
#85861=AXIS2_PLACEMENT_3D('',#203478,#105639,#105640);
#85862=AXIS2_PLACEMENT_3D('',#203487,#105645,#105646);
#85863=AXIS2_PLACEMENT_3D('',#203493,#105650,#105651);
#85864=AXIS2_PLACEMENT_3D('',#203499,#105655,#105656);
#85865=AXIS2_PLACEMENT_3D('',#203502,#105659,#105660);
#85866=AXIS2_PLACEMENT_3D('',#203511,#105665,#105666);
#85867=AXIS2_PLACEMENT_3D('',#203517,#105670,#105671);
#85868=AXIS2_PLACEMENT_3D('',#203523,#105675,#105676);
#85869=AXIS2_PLACEMENT_3D('',#203526,#105679,#105680);
#85870=AXIS2_PLACEMENT_3D('',#203535,#105685,#105686);
#85871=AXIS2_PLACEMENT_3D('',#203541,#105690,#105691);
#85872=AXIS2_PLACEMENT_3D('',#203547,#105695,#105696);
#85873=AXIS2_PLACEMENT_3D('',#203550,#105699,#105700);
#85874=AXIS2_PLACEMENT_3D('',#203559,#105705,#105706);
#85875=AXIS2_PLACEMENT_3D('',#203565,#105710,#105711);
#85876=AXIS2_PLACEMENT_3D('',#203571,#105715,#105716);
#85877=AXIS2_PLACEMENT_3D('',#203574,#105719,#105720);
#85878=AXIS2_PLACEMENT_3D('',#203583,#105725,#105726);
#85879=AXIS2_PLACEMENT_3D('',#203589,#105730,#105731);
#85880=AXIS2_PLACEMENT_3D('',#203595,#105735,#105736);
#85881=AXIS2_PLACEMENT_3D('',#203598,#105739,#105740);
#85882=AXIS2_PLACEMENT_3D('',#203607,#105745,#105746);
#85883=AXIS2_PLACEMENT_3D('',#203613,#105750,#105751);
#85884=AXIS2_PLACEMENT_3D('',#203619,#105755,#105756);
#85885=AXIS2_PLACEMENT_3D('',#203622,#105759,#105760);
#85886=AXIS2_PLACEMENT_3D('',#203631,#105765,#105766);
#85887=AXIS2_PLACEMENT_3D('',#203637,#105770,#105771);
#85888=AXIS2_PLACEMENT_3D('',#203643,#105775,#105776);
#85889=AXIS2_PLACEMENT_3D('',#203646,#105779,#105780);
#85890=AXIS2_PLACEMENT_3D('',#203655,#105785,#105786);
#85891=AXIS2_PLACEMENT_3D('',#203661,#105790,#105791);
#85892=AXIS2_PLACEMENT_3D('',#203667,#105795,#105796);
#85893=AXIS2_PLACEMENT_3D('',#203670,#105799,#105800);
#85894=AXIS2_PLACEMENT_3D('',#203679,#105805,#105806);
#85895=AXIS2_PLACEMENT_3D('',#203685,#105810,#105811);
#85896=AXIS2_PLACEMENT_3D('',#203691,#105815,#105816);
#85897=AXIS2_PLACEMENT_3D('',#203694,#105819,#105820);
#85898=AXIS2_PLACEMENT_3D('',#203703,#105825,#105826);
#85899=AXIS2_PLACEMENT_3D('',#203709,#105830,#105831);
#85900=AXIS2_PLACEMENT_3D('',#203715,#105835,#105836);
#85901=AXIS2_PLACEMENT_3D('',#203718,#105839,#105840);
#85902=AXIS2_PLACEMENT_3D('',#203727,#105845,#105846);
#85903=AXIS2_PLACEMENT_3D('',#203733,#105850,#105851);
#85904=AXIS2_PLACEMENT_3D('',#203739,#105855,#105856);
#85905=AXIS2_PLACEMENT_3D('',#203742,#105859,#105860);
#85906=AXIS2_PLACEMENT_3D('',#203751,#105865,#105866);
#85907=AXIS2_PLACEMENT_3D('',#203757,#105870,#105871);
#85908=AXIS2_PLACEMENT_3D('',#203763,#105875,#105876);
#85909=AXIS2_PLACEMENT_3D('',#203766,#105879,#105880);
#85910=AXIS2_PLACEMENT_3D('',#203775,#105885,#105886);
#85911=AXIS2_PLACEMENT_3D('',#203781,#105890,#105891);
#85912=AXIS2_PLACEMENT_3D('',#203787,#105895,#105896);
#85913=AXIS2_PLACEMENT_3D('',#203790,#105899,#105900);
#85914=AXIS2_PLACEMENT_3D('',#203799,#105905,#105906);
#85915=AXIS2_PLACEMENT_3D('',#203805,#105910,#105911);
#85916=AXIS2_PLACEMENT_3D('',#203811,#105915,#105916);
#85917=AXIS2_PLACEMENT_3D('',#203814,#105919,#105920);
#85918=AXIS2_PLACEMENT_3D('',#203823,#105925,#105926);
#85919=AXIS2_PLACEMENT_3D('',#203829,#105930,#105931);
#85920=AXIS2_PLACEMENT_3D('',#203835,#105935,#105936);
#85921=AXIS2_PLACEMENT_3D('',#203838,#105939,#105940);
#85922=AXIS2_PLACEMENT_3D('',#203847,#105945,#105946);
#85923=AXIS2_PLACEMENT_3D('',#203853,#105950,#105951);
#85924=AXIS2_PLACEMENT_3D('',#203859,#105955,#105956);
#85925=AXIS2_PLACEMENT_3D('',#203862,#105959,#105960);
#85926=AXIS2_PLACEMENT_3D('',#203871,#105965,#105966);
#85927=AXIS2_PLACEMENT_3D('',#203877,#105970,#105971);
#85928=AXIS2_PLACEMENT_3D('',#203883,#105975,#105976);
#85929=AXIS2_PLACEMENT_3D('',#203886,#105979,#105980);
#85930=AXIS2_PLACEMENT_3D('',#203887,#105981,#105982);
#85931=AXIS2_PLACEMENT_3D('',#203896,#105987,#105988);
#85932=AXIS2_PLACEMENT_3D('',#203902,#105992,#105993);
#85933=AXIS2_PLACEMENT_3D('',#203906,#105996,#105997);
#85934=AXIS2_PLACEMENT_3D('',#203910,#106000,#106001);
#85935=AXIS2_PLACEMENT_3D('',#203912,#106003,#106004);
#85936=AXIS2_PLACEMENT_3D('',#203913,#106005,#106006);
#85937=AXIS2_PLACEMENT_3D('',#203914,#106007,#106008);
#85938=AXIS2_PLACEMENT_3D('',#203916,#106010,#106011);
#85939=AXIS2_PLACEMENT_3D('',#203918,#106013,#106014);
#85940=AXIS2_PLACEMENT_3D('',#203920,#106016,#106017);
#85941=AXIS2_PLACEMENT_3D('',#203922,#106019,#106020);
#85942=AXIS2_PLACEMENT_3D('',#203923,#106021,#106022);
#85943=AXIS2_PLACEMENT_3D('',#203924,#106023,#106024);
#85944=AXIS2_PLACEMENT_3D('',#203926,#106026,#106027);
#85945=AXIS2_PLACEMENT_3D('',#203928,#106029,#106030);
#85946=AXIS2_PLACEMENT_3D('',#203930,#106032,#106033);
#85947=AXIS2_PLACEMENT_3D('',#203932,#106035,#106036);
#85948=AXIS2_PLACEMENT_3D('',#203933,#106037,#106038);
#85949=AXIS2_PLACEMENT_3D('',#203934,#106039,#106040);
#85950=AXIS2_PLACEMENT_3D('',#203936,#106041,#106042);
#85951=AXIS2_PLACEMENT_3D('',#203937,#106043,#106044);
#85952=AXIS2_PLACEMENT_3D('',#203940,#106045,#106046);
#85953=AXIS2_PLACEMENT_3D('',#203942,#106047,#106048);
#85954=AXIS2_PLACEMENT_3D('',#203944,#106049,#106050);
#85955=AXIS2_PLACEMENT_3D('',#203945,#106051,#106052);
#85956=AXIS2_PLACEMENT_3D('',#203946,#106053,#106054);
#85957=AXIS2_PLACEMENT_3D('',#203951,#106057,#106058);
#85958=AXIS2_PLACEMENT_3D('',#203952,#106059,#106060);
#85959=AXIS2_PLACEMENT_3D('',#203955,#106062,#106063);
#85960=AXIS2_PLACEMENT_3D('',#203956,#106064,#106065);
#85961=AXIS2_PLACEMENT_3D('',#203959,#106067,#106068);
#85962=AXIS2_PLACEMENT_3D('',#203960,#106069,#106070);
#85963=AXIS2_PLACEMENT_3D('',#203961,#106071,#106072);
#85964=AXIS2_PLACEMENT_3D('',#203962,#106073,#106074);
#85965=AXIS2_PLACEMENT_3D('',#203964,#106075,#106076);
#85966=AXIS2_PLACEMENT_3D('',#203965,#106077,#106078);
#89687=DIRECTION('axis',(0.,0.,1.));
#89688=DIRECTION('refdir',(1.,0.,0.));
#89689=DIRECTION('center_axis',(0.190809912898503,0.,-0.981627005099017));
#89690=DIRECTION('ref_axis',(0.,1.,0.));
#89691=DIRECTION('',(-0.190809912898503,0.,0.981627005099017));
#89692=DIRECTION('center_axis',(0.190809912898504,-3.49368872714712E-16,
-0.981627005099017));
#89693=DIRECTION('ref_axis',(0.574140136795491,-0.811115328353722,0.11160209420118));
#89694=DIRECTION('center_axis',(0.190809912898503,0.,-0.981627005099017));
#89695=DIRECTION('ref_axis',(0.,1.,0.));
#89696=DIRECTION('',(-0.190809912898503,0.,0.981627005099017));
#89697=DIRECTION('center_axis',(0.190809912898504,-3.49368872714712E-16,
-0.981627005099017));
#89698=DIRECTION('ref_axis',(0.574140136795491,-0.811115328353722,0.11160209420118));
#89699=DIRECTION('center_axis',(0.190809912898503,0.,-0.981627005099017));
#89700=DIRECTION('ref_axis',(0.,1.,0.));
#89701=DIRECTION('',(-0.190809912898503,0.,0.981627005099017));
#89702=DIRECTION('center_axis',(0.190809912898503,0.,-0.981627005099017));
#89703=DIRECTION('ref_axis',(0.,1.,0.));
#89704=DIRECTION('',(-0.190809912898503,0.,0.981627005099017));
#89705=DIRECTION('center_axis',(0.190809912898504,-6.43574239211312E-16,
-0.981627005099017));
#89706=DIRECTION('ref_axis',(0.574140136791955,-0.811115328356319,0.111602094200493));
#89707=DIRECTION('center_axis',(-0.190809912898503,1.46277694072906E-15,
0.981627005099017));
#89708=DIRECTION('ref_axis',(5.57389751783728E-17,-1.,1.50099017455135E-15));
#89709=DIRECTION('center_axis',(0.190809912898503,0.,-0.981627005099017));
#89710=DIRECTION('ref_axis',(0.981627005099017,0.,0.190809912898503));
#89711=DIRECTION('',(-0.190693676655342,0.0348994966626399,0.981029024451551));
#89712=DIRECTION('center_axis',(-0.190809912898503,0.,0.981627005099017));
#89713=DIRECTION('ref_axis',(-0.981627005099017,0.,-0.190809912898503));
#89714=DIRECTION('center_axis',(0.190809912898503,0.,-0.981627005099017));
#89715=DIRECTION('ref_axis',(0.981627005099017,0.,0.190809912898503));
#89716=DIRECTION('center_axis',(0.190809912898503,0.,-0.981627005099017));
#89717=DIRECTION('ref_axis',(0.,1.,0.));
#89718=DIRECTION('center_axis',(0.981627005099017,0.,0.190809912898503));
#89719=DIRECTION('ref_axis',(0.,-1.,0.));
#89720=DIRECTION('center_axis',(-0.190809912898504,0.,0.981627005099017));
#89721=DIRECTION('ref_axis',(0.981627005099017,0.,0.190809912898504));
#89722=DIRECTION('center_axis',(0.190809912898503,0.,-0.981627005099017));
#89723=DIRECTION('ref_axis',(0.,1.,0.));
#89724=DIRECTION('center_axis',(-0.981627005099017,0.,-0.190809912898503));
#89725=DIRECTION('ref_axis',(0.,-1.,0.));
#89726=DIRECTION('center_axis',(-0.190809912898504,0.,0.981627005099017));
#89727=DIRECTION('ref_axis',(0.981627005099017,0.,0.190809912898504));
#89728=DIRECTION('center_axis',(0.,-1.,0.));
#89729=DIRECTION('ref_axis',(0.981627005099017,0.,0.190809912898502));
#89730=DIRECTION('',(0.,-1.,0.));
#89731=DIRECTION('',(0.,-1.,0.));
#89732=DIRECTION('center_axis',(0.,-1.,0.));
#89733=DIRECTION('ref_axis',(0.981627005099017,0.,0.190809912898502));
#89734=DIRECTION('',(0.,-1.,0.));
#89735=DIRECTION('',(0.,-1.,0.));
#89736=DIRECTION('center_axis',(0.190809912898503,0.,-0.981627005099017));
#89737=DIRECTION('ref_axis',(0.,1.,0.));
#89738=DIRECTION('',(0.190809912898503,0.,-0.981627005099017));
#89739=DIRECTION('center_axis',(0.190809912898503,-2.47317346244379E-16,
-0.981627005099017));
#89740=DIRECTION('ref_axis',(0.421966359657993,-0.902893528415321,0.0820223607482341));
#89741=DIRECTION('center_axis',(0.190809912898503,-2.47317346244379E-16,
-0.981627005099017));
#89742=DIRECTION('ref_axis',(0.421966359657993,-0.902893528415321,0.0820223607482341));
#89743=DIRECTION('',(0.190809912898503,0.,-0.981627005099017));
#89744=DIRECTION('center_axis',(-0.190809912898504,0.,0.981627005099017));
#89745=DIRECTION('ref_axis',(0.981627005099017,0.,0.190809912898504));
#89746=DIRECTION('center_axis',(0.190809912898503,-2.47317346244379E-16,
-0.981627005099017));
#89747=DIRECTION('ref_axis',(0.421966359657993,-0.902893528415321,0.0820223607482341));
#89748=DIRECTION('center_axis',(0.190809912898503,-2.47317346244379E-16,
-0.981627005099017));
#89749=DIRECTION('ref_axis',(0.421966359657993,-0.902893528415321,0.0820223607482341));
#89750=DIRECTION('center_axis',(0.190809912898504,2.18221187862687E-16,
-0.981627005099017));
#89751=DIRECTION('ref_axis',(-0.886304670221616,-0.42986425339371,-0.17228103551355));
#89752=DIRECTION('center_axis',(0.190809912898504,0.,-0.981627005099017));
#89753=DIRECTION('ref_axis',(-0.981627005099017,0.,-0.190809912898504));
#89754=DIRECTION('center_axis',(0.190809912898504,1.30932712717612E-16,
-0.981627005099017));
#89755=DIRECTION('ref_axis',(0.886304670221616,0.429864253393709,0.17228103551355));
#89756=DIRECTION('center_axis',(0.190809912898504,1.30932712717612E-16,
-0.981627005099017));
#89757=DIRECTION('ref_axis',(0.886304670221616,0.429864253393709,0.17228103551355));
#89758=DIRECTION('center_axis',(0.190809912898503,-2.47317346244379E-16,
-0.981627005099017));
#89759=DIRECTION('ref_axis',(-0.421966359657993,0.902893528415321,-0.0820223607482341));
#89760=DIRECTION('center_axis',(0.190809912898503,-2.47317346244379E-16,
-0.981627005099017));
#89761=DIRECTION('ref_axis',(-0.421966359657993,0.902893528415321,-0.0820223607482341));
#89762=DIRECTION('center_axis',(-0.981627005099017,0.,-0.190809912898503));
#89763=DIRECTION('ref_axis',(0.,-1.,0.));
#89764=DIRECTION('',(-0.981627005099017,0.,-0.190809912898503));
#89765=DIRECTION('',(-0.981627005099017,-1.072434343069E-14,-0.190809912898503));
#89766=DIRECTION('center_axis',(-0.981627005099017,0.,-0.190809912898503));
#89767=DIRECTION('ref_axis',(0.,-1.,0.));
#89768=DIRECTION('',(-0.981627005099017,0.,-0.190809912898503));
#89769=DIRECTION('',(-0.981627005099017,0.,-0.190809912898503));
#89770=DIRECTION('center_axis',(0.190809912898503,0.,-0.981627005099017));
#89771=DIRECTION('ref_axis',(0.,1.,0.));
#89772=DIRECTION('center_axis',(-0.190809912898503,0.,0.981627005099017));
#89773=DIRECTION('ref_axis',(0.981627005099017,0.,0.190809912898503));
#89774=DIRECTION('',(-0.190809912898503,0.,0.981627005099017));
#89775=DIRECTION('center_axis',(0.190809912898503,5.5156726174395E-17,-0.981627005099017));
#89776=DIRECTION('ref_axis',(0.410813063807969,-0.908215781839759,0.0798543688341771));
#89777=DIRECTION('center_axis',(0.190809912898503,5.5156726174395E-17,-0.981627005099017));
#89778=DIRECTION('ref_axis',(0.410813063807969,-0.908215781839759,0.0798543688341771));
#89779=DIRECTION('',(-0.190809912898503,0.,0.981627005099017));
#89780=DIRECTION('center_axis',(-0.190809912898503,0.,0.981627005099017));
#89781=DIRECTION('ref_axis',(0.981627005099017,0.,0.190809912898503));
#89782=DIRECTION('center_axis',(0.190809912898503,5.5156726174395E-17,-0.981627005099017));
#89783=DIRECTION('ref_axis',(0.410813063807969,-0.908215781839759,0.0798543688341771));
#89784=DIRECTION('center_axis',(0.190809912898503,5.5156726174395E-17,-0.981627005099017));
#89785=DIRECTION('ref_axis',(0.410813063807969,-0.908215781839759,0.0798543688341771));
#89786=DIRECTION('center_axis',(0.190809912898503,-9.65242708051913E-17,
-0.981627005099017));
#89787=DIRECTION('ref_axis',(0.891529137911025,0.418502202643181,0.17329657422589));
#89788=DIRECTION('center_axis',(0.190809912898503,-9.65242708051913E-17,
-0.981627005099017));
#89789=DIRECTION('ref_axis',(0.891529137911025,0.418502202643181,0.17329657422589));
#89790=DIRECTION('center_axis',(0.190809912898503,0.,-0.981627005099017));
#89791=DIRECTION('ref_axis',(-0.981627005099017,0.,-0.190809912898503));
#89792=DIRECTION('center_axis',(0.190809912898503,0.,-0.981627005099017));
#89793=DIRECTION('ref_axis',(-0.981627005099017,0.,-0.190809912898503));
#89794=DIRECTION('center_axis',(0.190809912898503,5.5156726174395E-17,-0.981627005099017));
#89795=DIRECTION('ref_axis',(-0.410813063807969,0.908215781839759,-0.0798543688341771));
#89796=DIRECTION('center_axis',(0.190809912898503,5.5156726174395E-17,-0.981627005099017));
#89797=DIRECTION('ref_axis',(-0.410813063807969,0.908215781839759,-0.0798543688341771));
#89798=DIRECTION('center_axis',(0.190809912898503,0.,-0.981627005099017));
#89799=DIRECTION('ref_axis',(0.,1.,0.));
#89800=DIRECTION('center_axis',(-0.190809912898503,0.,0.981627005099017));
#89801=DIRECTION('ref_axis',(0.981627005099017,0.,0.190809912898503));
#89802=DIRECTION('center_axis',(-0.981627005099017,0.,-0.190809912898503));
#89803=DIRECTION('ref_axis',(0.,-1.,0.));
#89804=DIRECTION('center_axis',(0.190809912898503,0.,-0.981627005099017));
#89805=DIRECTION('ref_axis',(0.,1.,0.));
#89806=DIRECTION('center_axis',(-0.190809912898503,0.,0.981627005099017));
#89807=DIRECTION('ref_axis',(0.981627005099017,0.,0.190809912898503));
#89808=DIRECTION('',(0.190809912898503,0.,-0.981627005099017));
#89809=DIRECTION('center_axis',(-0.190809912898503,0.,0.981627005099017));
#89810=DIRECTION('ref_axis',(0.981627005099017,0.,0.190809912898503));
#89811=DIRECTION('center_axis',(0.190809912898503,0.,-0.981627005099017));
#89812=DIRECTION('ref_axis',(0.,1.,0.));
#89813=DIRECTION('center_axis',(-0.190809912898504,0.,0.981627005099017));
#89814=DIRECTION('ref_axis',(0.981627005099017,0.,0.190809912898504));
#89815=DIRECTION('',(-0.190809912898503,0.,0.981627005099017));
#89816=DIRECTION('center_axis',(-0.190809912898504,0.,0.981627005099017));
#89817=DIRECTION('ref_axis',(0.981627005099017,0.,0.190809912898504));
#89818=DIRECTION('center_axis',(0.190809912898503,0.,-0.981627005099017));
#89819=DIRECTION('ref_axis',(0.,1.,0.));
#89820=DIRECTION('center_axis',(0.981627005099017,0.,0.190809912898503));
#89821=DIRECTION('ref_axis',(0.,-1.,0.));
#89822=DIRECTION('center_axis',(-0.190809912898503,0.,0.981627005099017));
#89823=DIRECTION('ref_axis',(0.981627005099017,0.,0.190809912898503));
#89824=DIRECTION('center_axis',(0.190809912898503,0.,-0.981627005099017));
#89825=DIRECTION('ref_axis',(0.,1.,0.));
#89826=DIRECTION('center_axis',(-0.981627005099017,0.,-0.190809912898503));
#89827=DIRECTION('ref_axis',(0.,-1.,0.));
#89828=DIRECTION('center_axis',(-0.190809912898503,0.,0.981627005099017));
#89829=DIRECTION('ref_axis',(0.981627005099017,0.,0.190809912898503));
#89830=DIRECTION('center_axis',(-0.190809912898503,0.,0.981627005099017));
#89831=DIRECTION('ref_axis',(0.981627005099017,0.,0.190809912898503));
#89832=DIRECTION('center_axis',(-0.190809912898503,1.16273051859071E-15,
0.981627005099017));
#89833=DIRECTION('ref_axis',(-4.2332613184886E-18,-1.,1.18367033947895E-15));
#89834=DIRECTION('center_axis',(0.190809912898503,0.,-0.981627005099017));
#89835=DIRECTION('ref_axis',(0.981627005099017,0.,0.190809912898503));
#89836=DIRECTION('',(0.190693676655342,-0.0348994966626396,-0.981029024451551));
#89837=DIRECTION('center_axis',(0.190809912898503,0.,-0.981627005099017));
#89838=DIRECTION('ref_axis',(0.,1.,0.));
#89839=DIRECTION('center_axis',(-0.190809912898503,0.,0.981627005099017));
#89840=DIRECTION('ref_axis',(0.,1.,0.));
#89841=DIRECTION('',(0.190809912898503,0.,-0.981627005099017));
#89842=DIRECTION('center_axis',(-0.190809912898503,0.,0.981627005099017));
#89843=DIRECTION('ref_axis',(0.981627005099017,0.,0.190809912898503));
#89844=DIRECTION('center_axis',(0.190809912898503,0.,-0.981627005099017));
#89845=DIRECTION('ref_axis',(0.,1.,0.));
#89846=DIRECTION('center_axis',(-0.190809912898503,0.,0.981627005099017));
#89847=DIRECTION('ref_axis',(0.981627005099017,0.,0.190809912898503));
#89848=DIRECTION('',(0.190809912898503,0.,-0.981627005099017));
#89849=DIRECTION('center_axis',(-0.190809912898503,0.,0.981627005099017));
#89850=DIRECTION('ref_axis',(0.,1.,0.));
#89851=DIRECTION('center_axis',(0.190809912898503,0.,-0.981627005099017));
#89852=DIRECTION('ref_axis',(0.,1.,0.));
#89853=DIRECTION('center_axis',(-0.190809912898503,0.,0.981627005099017));
#89854=DIRECTION('ref_axis',(0.981627005099017,0.,0.190809912898503));
#89855=DIRECTION('',(-0.190809912898503,0.,0.981627005099017));
#89856=DIRECTION('center_axis',(-0.190809912898503,0.,0.981627005099017));
#89857=DIRECTION('ref_axis',(0.981627005099017,0.,0.190809912898503));
#89858=DIRECTION('center_axis',(0.190809912898503,0.,-0.981627005099017));
#89859=DIRECTION('ref_axis',(0.,1.,0.));
#89860=DIRECTION('center_axis',(-0.190809912898503,0.,0.981627005099017));
#89861=DIRECTION('ref_axis',(0.981627005099017,0.,0.190809912898503));
#89862=DIRECTION('',(0.190809912898503,0.,-0.981627005099017));
#89863=DIRECTION('center_axis',(0.190809912898503,-2.65000753919799E-16,
-0.981627005099017));
#89864=DIRECTION('ref_axis',(-0.309763741346266,0.948905109489044,-0.0602122722769161));
#89865=DIRECTION('',(0.190809912898503,0.,-0.981627005099017));
#89866=DIRECTION('center_axis',(-0.190809912898503,2.65000753919799E-16,
0.981627005099017));
#89867=DIRECTION('ref_axis',(-0.309763741346266,0.948905109489044,-0.0602122722769161));
#89868=DIRECTION('',(-0.190809912898503,0.,0.981627005099017));
#89869=DIRECTION('center_axis',(0.190809912898503,-2.65000753919799E-16,
-0.981627005099017));
#89870=DIRECTION('ref_axis',(0.309763741346266,-0.948905109489044,0.0602122722769161));
#89871=DIRECTION('',(-0.190809912898503,0.,0.981627005099017));
#89872=DIRECTION('center_axis',(-0.190809912898503,0.,0.981627005099017));
#89873=DIRECTION('ref_axis',(0.981627005099017,0.,0.190809912898503));
#89874=DIRECTION('center_axis',(0.190809912898503,-2.65000753919799E-16,
-0.981627005099017));
#89875=DIRECTION('ref_axis',(0.309763741346266,-0.948905109489044,0.0602122722769161));
#89876=DIRECTION('',(-0.190809912898503,0.,0.981627005099017));
#89877=DIRECTION('center_axis',(0.190809912898503,2.42663671716433E-17,
-0.981627005099017));
#89878=DIRECTION('ref_axis',(0.549709825015208,0.828493500750504,0.106853298947315));
#89879=DIRECTION('center_axis',(-0.190809912898503,-1.38499642189817E-16,
0.981627005099017));
#89880=DIRECTION('ref_axis',(0.733440712215292,-0.664634735150065,0.142567143820477));
#89881=DIRECTION('center_axis',(0.190809912898503,0.,-0.981627005099017));
#89882=DIRECTION('ref_axis',(0.,1.,0.));
#89883=DIRECTION('center_axis',(-0.190809912898503,0.,0.981627005099017));
#89884=DIRECTION('ref_axis',(0.981627005099017,0.,0.190809912898503));
#89885=DIRECTION('',(0.190809912898503,0.,-0.981627005099017));
#89886=DIRECTION('center_axis',(-0.190809912898503,0.,0.981627005099017));
#89887=DIRECTION('ref_axis',(0.981627005099017,0.,0.190809912898503));
#89888=DIRECTION('',(0.0954145326459342,-0.865996387817356,-0.490862835471632));
#89889=DIRECTION('',(0.190809912899824,0.,-0.98162700509876));
#89890=DIRECTION('center_axis',(0.,-1.,0.));
#89891=DIRECTION('ref_axis',(0.,0.,-1.));
#89892=DIRECTION('',(-0.981627005099017,0.,-0.190809912898503));
#89893=DIRECTION('',(-0.981627005099017,0.,-0.190809912898503));
#89894=DIRECTION('center_axis',(-0.190809912898503,-2.68840323315103E-17,
0.981627005099017));
#89895=DIRECTION('ref_axis',(5.12973986753602E-18,-1.,-2.63900921425656E-17));
#89896=DIRECTION('center_axis',(0.190809912898503,2.80359349652818E-16,
-0.981627005099017));
#89897=DIRECTION('ref_axis',(-0.170230827332271,-0.984848484848479,-0.0330896859674664));
#89898=DIRECTION('center_axis',(-0.190809912898503,-2.68840323315103E-17,
0.981627005099017));
#89899=DIRECTION('ref_axis',(5.12973986753602E-18,-1.,-2.63900921425656E-17));
#89900=DIRECTION('center_axis',(0.190809912898503,2.80359349652818E-16,
-0.981627005099017));
#89901=DIRECTION('ref_axis',(0.170230827332271,0.984848484848479,0.0330896859674664));
#89902=DIRECTION('center_axis',(0.,1.,0.));
#89903=DIRECTION('ref_axis',(1.,0.,0.));
#89904=DIRECTION('',(0.981627005099017,0.,0.190809912898503));
#89905=DIRECTION('',(0.981627005099017,0.,0.190809912898503));
#89906=DIRECTION('center_axis',(0.190809912898503,0.,-0.981627005099017));
#89907=DIRECTION('ref_axis',(0.,-1.,0.));
#89908=DIRECTION('center_axis',(0.190809912898503,0.,-0.981627005099017));
#89909=DIRECTION('ref_axis',(0.,-1.,0.));
#89910=DIRECTION('center_axis',(0.190809912898503,0.,-0.981627005099017));
#89911=DIRECTION('ref_axis',(0.,-1.,0.));
#89912=DIRECTION('center_axis',(0.190809912898503,0.,-0.981627005099017));
#89913=DIRECTION('ref_axis',(0.,-1.,0.));
#89914=DIRECTION('center_axis',(0.190809912898504,-6.43574239211312E-16,
-0.981627005099017));
#89915=DIRECTION('ref_axis',(0.574140136791955,-0.811115328356319,0.111602094200493));
#89916=DIRECTION('',(0.0954057063114802,0.866023134057401,-0.49081736163323));
#89917=DIRECTION('center_axis',(0.190809912898503,0.,-0.981627005099017));
#89918=DIRECTION('ref_axis',(0.,1.,0.));
#89919=DIRECTION('center_axis',(0.190809912898503,0.,-0.981627005099017));
#89920=DIRECTION('ref_axis',(0.,-1.,0.));
#89921=DIRECTION('center_axis',(0.190809912898503,0.,-0.981627005099017));
#89922=DIRECTION('ref_axis',(0.,-1.,0.));
#89923=DIRECTION('center_axis',(0.190809912898503,0.,-0.981627005099017));
#89924=DIRECTION('ref_axis',(0.,-1.,0.));
#89925=DIRECTION('center_axis',(-0.981627005099017,0.,-0.190809912898503));
#89926=DIRECTION('ref_axis',(-0.190809912898503,0.,0.981627005099017));
#89927=DIRECTION('center_axis',(-0.981627005099017,4.22136220887777E-18,
-0.190809912898503));
#89928=DIRECTION('ref_axis',(-0.190787588212088,0.0152965859522907,0.981512155117001));
#89929=DIRECTION('',(-0.190809912898503,0.,0.981627005099017));
#89930=DIRECTION('',(0.,-1.,0.));
#89931=DIRECTION('',(-0.190809912898503,0.,0.981627005099017));
#89932=DIRECTION('center_axis',(0.,1.,0.));
#89933=DIRECTION('ref_axis',(1.,0.,0.));
#89934=DIRECTION('',(-0.981627005099017,0.,-0.190809912898503));
#89935=DIRECTION('center_axis',(0.,1.,0.));
#89936=DIRECTION('ref_axis',(-0.710663462661499,0.,0.703532119265331));
#89937=DIRECTION('',(-0.190809912898503,0.,0.981627005099017));
#89938=DIRECTION('center_axis',(0.,1.,0.));
#89939=DIRECTION('ref_axis',(-0.706868204155822,0.,0.707345277748797));
#89940=DIRECTION('center_axis',(0.981627005099017,0.,0.190809912898503));
#89941=DIRECTION('ref_axis',(0.,-1.,0.));
#89942=DIRECTION('center_axis',(0.981627005099017,1.36071346699076E-17,
0.190809912898504));
#89943=DIRECTION('ref_axis',(-0.190549299057218,0.0522474292087793,0.980286269805854));
#89944=DIRECTION('center_axis',(0.981627005099017,3.13226948961353E-17,
0.190809912898504));
#89945=DIRECTION('ref_axis',(-0.190534941381885,0.0536663262517514,0.980212406338158));
#89946=DIRECTION('',(-0.190809912898503,0.,0.981627005099017));
#89947=DIRECTION('center_axis',(0.,-1.,0.));
#89948=DIRECTION('ref_axis',(0.,0.,-1.));
#89949=DIRECTION('center_axis',(0.,-1.,0.));
#89950=DIRECTION('ref_axis',(-0.679202351867065,0.,0.733951064593715));
#89951=DIRECTION('center_axis',(0.,-1.,0.));
#89952=DIRECTION('ref_axis',(-0.688011363844931,0.,0.725699912650014));
#89953=DIRECTION('',(0.981627005099012,0.,0.190809912898527));
#89954=DIRECTION('center_axis',(-0.190809912898503,0.,0.981627005099017));
#89955=DIRECTION('ref_axis',(0.,1.,0.));
#89956=DIRECTION('center_axis',(0.190809912898503,7.28528651098404E-18,
-0.981627005099017));
#89957=DIRECTION('ref_axis',(-0.98136931371192,0.0229120103408305,-0.190759822517053));
#89958=DIRECTION('center_axis',(-0.981627005099017,0.,-0.190809912898503));
#89959=DIRECTION('ref_axis',(-0.190809912898503,0.,0.981627005099017));
#89960=DIRECTION('center_axis',(-0.981627005099017,3.63686590303316E-17,
-0.190809912898503));
#89961=DIRECTION('ref_axis',(-0.190004571672825,0.0917795157137274,0.977483904337447));
#89962=DIRECTION('',(-0.190809912898503,0.,0.981627005099017));
#89963=DIRECTION('',(0.,-1.,0.));
#89964=DIRECTION('',(-0.190809912898503,0.,0.981627005099017));
#89965=DIRECTION('center_axis',(0.,1.,0.));
#89966=DIRECTION('ref_axis',(1.,0.,0.));
#89967=DIRECTION('center_axis',(0.,1.,0.));
#89968=DIRECTION('ref_axis',(-0.705384737821605,0.,0.708824640971479));
#89969=DIRECTION('',(-0.190809912898503,0.,0.981627005099017));
#89970=DIRECTION('center_axis',(0.,1.,0.));
#89971=DIRECTION('ref_axis',(-0.709191690509886,0.,0.705015706287264));
#89972=DIRECTION('',(-0.981627005099017,0.,-0.190809912898503));
#89973=DIRECTION('center_axis',(0.981627005099017,0.,0.190809912898503));
#89974=DIRECTION('ref_axis',(0.,-1.,0.));
#89975=DIRECTION('center_axis',(0.981627005099017,-3.95843917670041E-17,
0.190809912898503));
#89976=DIRECTION('ref_axis',(-0.189267639880765,0.126886613792695,0.973692737846077));
#89977=DIRECTION('center_axis',(0.981627005099017,7.30862880909824E-17,
0.190809912898504));
#89978=DIRECTION('ref_axis',(-0.189182369469026,0.130332506611401,0.973254061796032));
#89979=DIRECTION('',(-0.190809912898503,0.,0.981627005099017));
#89980=DIRECTION('center_axis',(0.,-1.,0.));
#89981=DIRECTION('ref_axis',(0.,0.,-1.));
#89982=DIRECTION('center_axis',(0.,-1.,0.));
#89983=DIRECTION('ref_axis',(-0.680489170594158,0.,0.732758137930979));
#89984=DIRECTION('center_axis',(0.,-1.,0.));
#89985=DIRECTION('ref_axis',(-0.689369692174638,0.,0.724409709702351));
#89986=DIRECTION('',(0.981627005099017,0.,0.190809912898503));
#89987=DIRECTION('center_axis',(-0.190809912898503,0.,0.981627005099017));
#89988=DIRECTION('ref_axis',(0.,1.,0.));
#89989=DIRECTION('center_axis',(0.190809912898504,-6.41105212966596E-17,
-0.981627005099017));
#89990=DIRECTION('ref_axis',(-0.972307089527912,0.137472062045006,-0.18899829578823));
#89991=DIRECTION('center_axis',(0.981627005099017,0.,0.190809912898503));
#89992=DIRECTION('ref_axis',(0.,-1.,0.));
#89993=DIRECTION('',(-0.190809912898503,0.,0.981627005099017));
#89994=DIRECTION('center_axis',(0.981627005099017,6.26453897922707E-17,
0.190809912898504));
#89995=DIRECTION('ref_axis',(-0.186677203055246,0.206998686971002,0.960366162175527));
#89996=DIRECTION('',(-0.190809912898503,0.,0.981627005099017));
#89997=DIRECTION('center_axis',(0.981627005099017,-1.03909028388386E-16,
0.190809912898503));
#89998=DIRECTION('ref_axis',(-0.186895105393115,0.201525798376691,0.961487166928781));
#89999=DIRECTION('center_axis',(0.,1.,0.));
#90000=DIRECTION('ref_axis',(1.,0.,0.));
#90001=DIRECTION('',(-0.190809912898503,0.,0.981627005099017));
#90002=DIRECTION('',(-0.981627005099017,0.,-0.190809912898503));
#90003=DIRECTION('center_axis',(0.,1.,0.));
#90004=DIRECTION('ref_axis',(-0.713534436527226,0.,0.700620159494268));
#90005=DIRECTION('center_axis',(-0.981627005099017,0.,-0.190809912898503));
#90006=DIRECTION('ref_axis',(-0.190809912898503,0.,0.981627005099017));
#90007=DIRECTION('',(-0.190809912898503,0.,0.981627005099017));
#90008=DIRECTION('',(0.,-1.,0.));
#90009=DIRECTION('center_axis',(-0.981627005099017,-4.15641817489504E-17,
-0.190809912898504));
#90010=DIRECTION('ref_axis',(-0.188089389572928,0.168262445475198,0.967631195741843));
#90011=DIRECTION('center_axis',(0.,-1.,0.));
#90012=DIRECTION('ref_axis',(0.,0.,-1.));
#90013=DIRECTION('center_axis',(0.,-1.,0.));
#90014=DIRECTION('ref_axis',(-0.692715647339658,0.,0.721210809632522));
#90015=DIRECTION('',(0.981627005099017,0.,0.190809912898503));
#90016=DIRECTION('center_axis',(0.,-1.,0.));
#90017=DIRECTION('ref_axis',(-0.683657405158267,0.,0.729803091506377));
#90018=DIRECTION('center_axis',(-0.190809912898503,0.,0.981627005099017));
#90019=DIRECTION('ref_axis',(0.,1.,0.));
#90020=DIRECTION('center_axis',(0.190809912898503,5.24540628790851E-17,
-0.981627005099017));
#90021=DIRECTION('ref_axis',(-0.94993897729484,0.252032113749207,-0.184650353520213));
#90022=DIRECTION('center_axis',(0.,-1.,0.));
#90023=DIRECTION('ref_axis',(0.,0.,-1.));
#90024=DIRECTION('',(-0.190809912898503,0.,0.981627005099017));
#90025=DIRECTION('center_axis',(0.,-1.,0.));
#90026=DIRECTION('ref_axis',(-0.631733075007243,0.,0.775185991838019));
#90027=DIRECTION('',(-0.190809912898503,0.,0.981627005099017));
#90028=DIRECTION('center_axis',(0.,-1.,0.));
#90029=DIRECTION('ref_axis',(-0.623815939113541,0.,0.781571285365507));
#90030=DIRECTION('center_axis',(0.981627005099017,0.,0.190809912898503));
#90031=DIRECTION('ref_axis',(0.,-1.,0.));
#90032=DIRECTION('',(-0.190809912898503,0.,0.981627005099017));
#90033=DIRECTION('center_axis',(0.981627005099017,8.36846343838454E-18,
0.190809912898503));
#90034=DIRECTION('ref_axis',(-0.190558051740874,0.0513631640146422,0.980331298235003));
#90035=DIRECTION('center_axis',(0.981627005099017,-1.02429212253849E-17,
0.190809912898503));
#90036=DIRECTION('ref_axis',(-0.190570150509215,0.0501150985729195,0.980393540691656));
#90037=DIRECTION('center_axis',(0.,1.,0.));
#90038=DIRECTION('ref_axis',(1.,0.,0.));
#90039=DIRECTION('',(-0.190809912898503,0.,0.981627005099017));
#90040=DIRECTION('center_axis',(0.,1.,0.));
#90041=DIRECTION('ref_axis',(-0.660441325182145,0.,0.750877657139732));
#90042=DIRECTION('center_axis',(0.,1.,0.));
#90043=DIRECTION('ref_axis',(-0.652047602561264,0.,0.758178029221441));
#90044=DIRECTION('center_axis',(-0.981627005099017,0.,-0.190809912898503));
#90045=DIRECTION('ref_axis',(-0.190809912898503,0.,0.981627005099017));
#90046=DIRECTION('center_axis',(-0.981627005099017,-1.43307256972171E-17,
-0.190809912898504));
#90047=DIRECTION('ref_axis',(-0.19078849457757,0.0149828714853907,0.981516817939905));
#90048=DIRECTION('center_axis',(-0.981627005099017,3.55175265017129E-18,
-0.190809912898503));
#90049=DIRECTION('ref_axis',(-0.190789564261716,0.0146039592402605,0.98152232096032));
#90050=DIRECTION('center_axis',(0.,-1.,0.));
#90051=DIRECTION('ref_axis',(0.,0.,-1.));
#90052=DIRECTION('',(-0.190809912898503,0.,0.981627005099017));
#90053=DIRECTION('center_axis',(0.,-1.,0.));
#90054=DIRECTION('ref_axis',(-0.632954523642759,0.,0.774188976284323));
#90055=DIRECTION('',(-0.190809912898503,0.,0.981627005099017));
#90056=DIRECTION('center_axis',(0.,-1.,0.));
#90057=DIRECTION('ref_axis',(-0.624972028608451,0.,0.780647144013887));
#90058=DIRECTION('center_axis',(0.981627005099017,0.,0.190809912898503));
#90059=DIRECTION('ref_axis',(0.,-1.,0.));
#90060=DIRECTION('',(-0.190809912898503,0.,0.981627005099017));
#90061=DIRECTION('center_axis',(0.981627005099017,7.65116657223729E-17,
0.190809912898504));
#90062=DIRECTION('ref_axis',(-0.189319606485261,0.124739112606999,0.97396008151581));
#90063=DIRECTION('center_axis',(0.981627005099017,5.00765037685485E-17,
0.190809912898504));
#90064=DIRECTION('ref_axis',(-0.189391419979737,0.121708096534195,0.974329528073578));
#90065=DIRECTION('center_axis',(0.,1.,0.));
#90066=DIRECTION('ref_axis',(1.,0.,0.));
#90067=DIRECTION('',(-0.190809912898503,0.,0.981627005099017));
#90068=DIRECTION('center_axis',(0.,1.,0.));
#90069=DIRECTION('ref_axis',(-0.662667500259754,0.,0.7489137360868));
#90070=DIRECTION('center_axis',(0.,1.,0.));
#90071=DIRECTION('ref_axis',(-0.654155114939017,0.,0.756360420434016));
#90072=DIRECTION('center_axis',(-0.981627005099017,0.,-0.190809912898503));
#90073=DIRECTION('ref_axis',(-0.190809912898503,0.,0.981627005099017));
#90074=DIRECTION('center_axis',(-0.981627005099017,-1.74461008487861E-17,
-0.190809912898503));
#90075=DIRECTION('ref_axis',(-0.190037332549694,0.0898972289123082,0.977652443597051));
#90076=DIRECTION('center_axis',(-0.981627005099017,-7.57707232036542E-17,
-0.190809912898504));
#90077=DIRECTION('ref_axis',(-0.190075989568967,0.0876237554415419,0.977851315728367));
#90078=DIRECTION('center_axis',(0.,-1.,0.));
#90079=DIRECTION('ref_axis',(0.,0.,-1.));
#90080=DIRECTION('',(-0.190809912898503,0.,0.981627005099017));
#90081=DIRECTION('center_axis',(0.,-1.,0.));
#90082=DIRECTION('ref_axis',(-0.635964061167762,0.,0.771718674714437));
#90083=DIRECTION('',(-0.190809912898503,0.,0.981627005099017));
#90084=DIRECTION('center_axis',(0.,-1.,0.));
#90085=DIRECTION('ref_axis',(-0.627819040820256,0.,0.778359333459511));
#90086=DIRECTION('center_axis',(0.981627005099017,0.,0.190809912898503));
#90087=DIRECTION('ref_axis',(0.,-1.,0.));
#90088=DIRECTION('',(-0.190809912898503,0.,0.981627005099017));
#90089=DIRECTION('center_axis',(0.981627005099017,5.73837492917797E-17,
0.190809912898504));
#90090=DIRECTION('ref_axis',(-0.187027825861746,0.198115061199294,0.962169951141392));
#90091=DIRECTION('center_axis',(0.981627005099017,6.37337320690617E-17,
0.190809912898504));
#90092=DIRECTION('ref_axis',(-0.187211139464168,0.193301094495603,0.963113013164774));
#90093=DIRECTION('center_axis',(0.,1.,0.));
#90094=DIRECTION('ref_axis',(1.,0.,0.));
#90095=DIRECTION('',(-0.190809912898513,0.,0.981627005099015));
#90096=DIRECTION('center_axis',(0.,1.,0.));
#90097=DIRECTION('ref_axis',(-0.666833013553189,0.,0.74520717390238));
#90098=DIRECTION('center_axis',(0.,1.,0.));
#90099=DIRECTION('ref_axis',(-0.658095710086924,0.,0.752934284227506));
#90100=DIRECTION('center_axis',(-0.981627005099017,0.,-0.190809912898503));
#90101=DIRECTION('ref_axis',(-0.190809912898503,0.,0.981627005099017));
#90102=DIRECTION('center_axis',(-0.981627005099017,-9.96920048502059E-17,
-0.190809912898504));
#90103=DIRECTION('ref_axis',(-0.188200600434938,0.164811586339199,0.96820332317354));
#90104=DIRECTION('center_axis',(-0.981627005099017,-3.78853616018271E-17,
-0.190809912898503));
#90105=DIRECTION('ref_axis',(-0.188331766656967,0.160643551642793,0.968878111520461));
#90106=DIRECTION('center_axis',(0.981627005099017,0.,0.190809912898503));
#90107=DIRECTION('ref_axis',(0.,-1.,0.));
#90108=DIRECTION('',(-0.190809912898493,0.,0.981627005099019));
#90109=DIRECTION('center_axis',(0.981627005099017,-3.82558328611865E-17,
0.190809912898503));
#90110=DIRECTION('ref_axis',(-0.183643278732954,0.271491009791614,0.944758052507911));
#90111=DIRECTION('',(-0.190809912898503,0.,0.981627005099017));
#90112=DIRECTION('center_axis',(0.981627005099017,2.45830109409238E-16,
0.190809912898504));
#90113=DIRECTION('ref_axis',(-0.183993708038349,0.264894092456889,0.946560846001851));
#90114=DIRECTION('center_axis',(0.,1.,0.));
#90115=DIRECTION('ref_axis',(1.,0.,0.));
#90116=DIRECTION('',(-0.190809912898503,0.,0.981627005099017));
#90117=DIRECTION('center_axis',(0.,1.,0.));
#90118=DIRECTION('ref_axis',(-0.673095267236959,0.,0.739555786417229));
#90119=DIRECTION('center_axis',(0.,1.,0.));
#90120=DIRECTION('ref_axis',(-0.664012722407567,0.,0.747721274594278));
#90121=DIRECTION('center_axis',(-0.981627005099017,0.,-0.190809912898503));
#90122=DIRECTION('ref_axis',(-0.190809912898503,0.,0.981627005099017));
#90123=DIRECTION('',(-0.190809912898503,0.,0.981627005099017));
#90124=DIRECTION('center_axis',(-0.981627005099017,-1.99384009700412E-16,
-0.190809912898504));
#90125=DIRECTION('ref_axis',(-0.185246010449827,0.2397259437662,0.953003351252149));
#90126=DIRECTION('center_axis',(-0.981627005099017,-1.65748457007993E-16,
-0.190809912898504));
#90127=DIRECTION('ref_axis',(-0.185527829167789,0.233663347844097,0.954453175634392));
#90128=DIRECTION('center_axis',(0.,-1.,0.));
#90129=DIRECTION('ref_axis',(0.,0.,-1.));
#90130=DIRECTION('center_axis',(0.,-1.,0.));
#90131=DIRECTION('ref_axis',(-0.640873994377488,0.,0.767646092500081));
#90132=DIRECTION('center_axis',(0.,-1.,0.));
#90133=DIRECTION('ref_axis',(-0.632459259128942,0.,0.774593626065997));
#90134=DIRECTION('center_axis',(-0.981627005099017,0.,-0.190809912898503));
#90135=DIRECTION('ref_axis',(-0.190809912898503,0.,0.981627005099017));
#90136=DIRECTION('center_axis',(-0.981627005099017,-1.70484127208222E-16,
-0.190809912898504));
#90137=DIRECTION('ref_axis',(-0.181615101248095,0.306683144045398,0.9343240359517));
#90138=DIRECTION('',(-0.190809912898503,0.,0.981627005099017));
#90139=DIRECTION('',(0.,-1.,0.));
#90140=DIRECTION('',(-0.190809912898503,0.,0.981627005099017));
#90141=DIRECTION('center_axis',(0.,1.,0.));
#90142=DIRECTION('ref_axis',(1.,0.,0.));
#90143=DIRECTION('center_axis',(0.,1.,0.));
#90144=DIRECTION('ref_axis',(-0.655547712408208,0.,0.755153757029895));
#90145=DIRECTION('',(-0.190809912898503,0.,0.981627005099017));
#90146=DIRECTION('center_axis',(0.,1.,0.));
#90147=DIRECTION('ref_axis',(-0.672133847791218,0.,0.74042966624344));
#90148=DIRECTION('',(-0.981627005099017,0.,-0.190809912898503));
#90149=DIRECTION('center_axis',(0.981627005099017,0.,0.190809912898503));
#90150=DIRECTION('ref_axis',(0.,-1.,0.));
#90151=DIRECTION('center_axis',(0.981627005099017,-1.82096377340177E-17,
0.190809912898503));
#90152=DIRECTION('ref_axis',(-0.179683420316472,0.336487090418195,0.924386448648654));
#90153=DIRECTION('center_axis',(0.981627005099017,2.10407080736525E-16,
0.190809912898504));
#90154=DIRECTION('ref_axis',(-0.179104025447188,0.344866958383991,0.921405735321627));
#90155=DIRECTION('',(-0.190809912898503,0.,0.981627005099017));
#90156=DIRECTION('center_axis',(0.,-1.,0.));
#90157=DIRECTION('ref_axis',(0.,0.,-1.));
#90158=DIRECTION('center_axis',(0.,-1.,0.));
#90159=DIRECTION('ref_axis',(-0.63906727483693,0.,0.769150842314107));
#90160=DIRECTION('center_axis',(0.,-1.,0.));
#90161=DIRECTION('ref_axis',(-0.647876541765181,0.,0.761745355502999));
#90162=DIRECTION('',(0.981627005099017,-1.201910499755E-14,0.190809912898503));
#90163=DIRECTION('center_axis',(-0.190809912898503,0.,0.981627005099017));
#90164=DIRECTION('ref_axis',(0.,1.,0.));
#90165=DIRECTION('center_axis',(0.190809912898504,-2.79755002021787E-16,
-0.981627005099017));
#90166=DIRECTION('ref_axis',(-0.860530616782567,0.481152217157524,-0.167271042037209));
#90167=DIRECTION('center_axis',(0.,-1.,0.));
#90168=DIRECTION('ref_axis',(0.,0.,-1.));
#90169=DIRECTION('',(-0.190809912898503,0.,0.981627005099017));
#90170=DIRECTION('center_axis',(0.,-1.,0.));
#90171=DIRECTION('ref_axis',(-0.36010817800382,0.,0.932910553126488));
#90172=DIRECTION('',(-0.190809912898503,0.,0.981627005099017));
#90173=DIRECTION('center_axis',(0.,-1.,0.));
#90174=DIRECTION('ref_axis',(-0.355750051979793,0.,0.934581136400888));
#90175=DIRECTION('center_axis',(0.981627005099017,0.,0.190809912898503));
#90176=DIRECTION('ref_axis',(0.,-1.,0.));
#90177=DIRECTION('',(-0.190809912898503,0.,0.981627005099017));
#90178=DIRECTION('',(0.,1.,0.));
#90179=DIRECTION('center_axis',(0.981627005099017,1.36798056621695E-16,
0.190809912898504));
#90180=DIRECTION('ref_axis',(-0.159259150209648,0.550783426949693,0.819313212191805));
#90181=DIRECTION('center_axis',(0.981627005099017,5.99180671853892E-16,
0.190809912898504));
#90182=DIRECTION('ref_axis',(-0.158343211241182,0.557989617362613,0.814601138207746));
#90183=DIRECTION('center_axis',(0.,1.,0.));
#90184=DIRECTION('ref_axis',(1.,0.,0.));
#90185=DIRECTION('',(-0.190809912898481,-2.237399193409E-14,0.981627005099021));
#90186=DIRECTION('',(-0.981627005099017,0.,-0.190809912898503));
#90187=DIRECTION('center_axis',(0.,1.,0.));
#90188=DIRECTION('ref_axis',(-0.39557835715531,0.,0.918432231223571));
#90189=DIRECTION('center_axis',(-0.981627005099017,0.,-0.190809912898503));
#90190=DIRECTION('ref_axis',(-0.190809912898503,0.,0.981627005099017));
#90191=DIRECTION('center_axis',(-0.981627005099017,-1.9977671997632E-16,
-0.190809912898504));
#90192=DIRECTION('ref_axis',(-0.160683023926675,0.539305080265381,0.826638370886405));
#90193=DIRECTION('',(0.,-1.,0.));
#90194=DIRECTION('center_axis',(-0.981627005099017,-4.57841563969441E-16,
-0.190809912898504));
#90195=DIRECTION('ref_axis',(-0.161960951934984,0.528701459898722,0.833212707745912));
#90196=DIRECTION('center_axis',(-0.190809912898503,0.,0.981627005099017));
#90197=DIRECTION('ref_axis',(0.,1.,0.));
#90198=DIRECTION('center_axis',(0.190809912898503,-3.03067918856936E-16,
-0.981627005099017));
#90199=DIRECTION('ref_axis',(-0.314874673283405,0.94715774678758,-0.0612057417645015));
#90200=DIRECTION('center_axis',(0.,-1.,0.));
#90201=DIRECTION('ref_axis',(0.,0.,-1.));
#90202=DIRECTION('',(-0.190809912898503,0.,0.981627005099017));
#90203=DIRECTION('center_axis',(0.,-1.,0.));
#90204=DIRECTION('ref_axis',(-0.287232890231326,0.,0.957860776297557));
#90205=DIRECTION('',(-0.190809912898503,0.,0.981627005099017));
#90206=DIRECTION('center_axis',(0.,-1.,0.));
#90207=DIRECTION('ref_axis',(-0.284731188473297,0.,0.95860740155216));
#90208=DIRECTION('center_axis',(0.981627005099017,0.,0.190809912898503));
#90209=DIRECTION('ref_axis',(0.,-1.,0.));
#90210=DIRECTION('',(-0.190809912898503,0.,0.981627005099017));
#90211=DIRECTION('',(0.,1.,0.));
#90212=DIRECTION('center_axis',(0.981627005099017,-2.99384533280007E-17,
0.190809912898503));
#90213=DIRECTION('ref_axis',(-0.158046676310463,0.560293947206128,0.813075605851874));
#90214=DIRECTION('center_axis',(0.981627005099017,-3.45621705615262E-16,
0.190809912898503));
#90215=DIRECTION('ref_axis',(-0.158864696644741,0.553903401621509,0.817283934647009));
#90216=DIRECTION('center_axis',(0.,1.,0.));
#90217=DIRECTION('ref_axis',(1.,0.,0.));
#90218=DIRECTION('',(-0.190809912898503,0.,0.981627005099017));
#90219=DIRECTION('',(-0.981627005099017,0.,-0.190809912898503));
#90220=DIRECTION('center_axis',(0.,1.,0.));
#90221=DIRECTION('ref_axis',(-0.323465005201917,0.,0.946240133586461));
#90222=DIRECTION('center_axis',(-0.981627005099017,0.,-0.190809912898503));
#90223=DIRECTION('ref_axis',(-0.190809912898503,0.,0.981627005099017));
#90224=DIRECTION('center_axis',(-0.981627005099017,-1.35608682274755E-16,
-0.190809912898503));
#90225=DIRECTION('ref_axis',(-0.161324598799703,0.534018424990321,0.829938971005081));
#90226=DIRECTION('',(1.2372117882059E-14,-1.,2.40490809969879E-15));
#90227=DIRECTION('center_axis',(-0.981627005099017,-2.17379342169057E-16,
-0.190809912898504));
#90228=DIRECTION('ref_axis',(-0.162549414642268,0.52371770234561,0.836240070822543));
#90229=DIRECTION('center_axis',(-0.190809912898503,0.,0.981627005099017));
#90230=DIRECTION('ref_axis',(0.,1.,0.));
#90231=DIRECTION('center_axis',(0.190809912898503,-2.21472709933915E-16,
-0.981627005099017));
#90232=DIRECTION('ref_axis',(-0.202419432825034,0.978508161618217,-0.0393465482771771));
#90233=DIRECTION('center_axis',(0.,-1.,0.));
#90234=DIRECTION('ref_axis',(0.,0.,-1.));
#90235=DIRECTION('',(-0.190809912898503,0.,0.981627005099017));
#90236=DIRECTION('center_axis',(0.,-1.,0.));
#90237=DIRECTION('ref_axis',(-0.213228510768614,0.,0.977002355266045));
#90238=DIRECTION('',(-0.190809912898503,0.,0.981627005099017));
#90239=DIRECTION('center_axis',(0.,-1.,0.));
#90240=DIRECTION('ref_axis',(-0.212642527010119,0.,0.977130060793726));
#90241=DIRECTION('center_axis',(0.981627005099017,0.,0.190809912898503));
#90242=DIRECTION('ref_axis',(0.,-1.,0.));
#90243=DIRECTION('',(-0.190809912898503,0.,0.981627005099017));
#90244=DIRECTION('center_axis',(0.981627005099017,1.78427841472896E-16,
0.190809912898504));
#90245=DIRECTION('ref_axis',(-0.157717823102993,0.562833367160933,0.811383811205239));
#90246=DIRECTION('center_axis',(0.981627005099017,5.43708098996233E-16,
0.190809912898504));
#90247=DIRECTION('ref_axis',(-0.159091080364181,0.552115896314094,0.818448572108133));
#90248=DIRECTION('center_axis',(0.,1.,0.));
#90249=DIRECTION('ref_axis',(1.,0.,0.));
#90250=DIRECTION('',(-0.190809912898503,0.,0.981627005099017));
#90251=DIRECTION('',(-0.981627005099017,2.00746580949E-14,-0.190809912898503));
#90252=DIRECTION('center_axis',(0.,1.,0.));
#90253=DIRECTION('ref_axis',(-0.245163967178927,0.,0.969481629117896));
#90254=DIRECTION('center_axis',(0.,1.,0.));
#90255=DIRECTION('ref_axis',(-0.250213113485533,0.,0.968190785868093));
#90256=DIRECTION('center_axis',(-0.981627005099017,0.,-0.190809912898503));
#90257=DIRECTION('ref_axis',(-0.190809912898503,0.,0.981627005099017));
#90258=DIRECTION('center_axis',(-0.981627005099017,1.19226339786349E-16,
-0.190809912898503));
#90259=DIRECTION('ref_axis',(-0.161675195212823,0.531098237955401,0.831742624189457));
#90260=DIRECTION('',(0.,-1.,0.));
#90261=DIRECTION('center_axis',(-0.981627005099017,-2.00758200789695E-16,
-0.190809912898504));
#90262=DIRECTION('ref_axis',(-0.162871454312254,0.52096239795233,0.83789681303247));
#90263=DIRECTION('center_axis',(-0.190809912898503,0.,0.981627005099017));
#90264=DIRECTION('ref_axis',(0.,1.,0.));
#90265=DIRECTION('center_axis',(0.190809912898503,-2.68098543604213E-16,
-0.981627005099017));
#90266=DIRECTION('ref_axis',(-0.0899641923666874,0.995791462362609,-0.0174873547898578));
#90267=DIRECTION('center_axis',(0.,-1.,0.));
#90268=DIRECTION('ref_axis',(0.,0.,-1.));
#90269=DIRECTION('',(-0.190809912898503,0.,0.981627005099017));
#90270=DIRECTION('center_axis',(0.,-1.,0.));
#90271=DIRECTION('ref_axis',(-0.138110878477997,0.,0.99041677350802));
#90272=DIRECTION('',(-0.190809912898503,0.,0.981627005099017));
#90273=DIRECTION('center_axis',(0.,-1.,0.));
#90274=DIRECTION('ref_axis',(-0.139498295720707,0.,0.990222311145845));
#90275=DIRECTION('center_axis',(0.981627005099017,0.,0.190809912898503));
#90276=DIRECTION('ref_axis',(0.,-1.,0.));
#90277=DIRECTION('',(-0.190809912898503,0.,0.981627005099017));
#90278=DIRECTION('center_axis',(0.981627005099017,-1.04257444818754E-16,
0.190809912898503));
#90279=DIRECTION('ref_axis',(-0.15765649718869,0.563305078924996,0.811068318300929));
#90280=DIRECTION('center_axis',(0.981627005099017,2.86623894051664E-16,
0.190809912898504));
#90281=DIRECTION('ref_axis',(-0.159034788508833,0.552561149824621,0.818158977062798));
#90282=DIRECTION('center_axis',(0.,1.,0.));
#90283=DIRECTION('ref_axis',(1.,0.,0.));
#90284=DIRECTION('',(-0.190809912898503,0.,0.981627005099017));
#90285=DIRECTION('center_axis',(0.,1.,0.));
#90286=DIRECTION('ref_axis',(-0.175424908276315,0.,0.984492814375121));
#90287=DIRECTION('center_axis',(0.,1.,0.));
#90288=DIRECTION('ref_axis',(-0.17584854355869,0.,0.984417233559169));
#90289=DIRECTION('center_axis',(-0.981627005099017,0.,-0.190809912898503));
#90290=DIRECTION('ref_axis',(-0.190809912898503,0.,0.981627005099017));
#90291=DIRECTION('center_axis',(-0.981627005099017,-3.27049270256878E-16,
-0.190809912898504));
#90292=DIRECTION('ref_axis',(-0.161754912532506,0.5304311251837,0.832152732200018));
#90293=DIRECTION('center_axis',(-0.981627005099017,-2.14578408646104E-16,
-0.190809912898504));
#90294=DIRECTION('ref_axis',(-0.162944724580192,0.520332710947401,0.838273754002602));
#90295=DIRECTION('center_axis',(0.,-1.,0.));
#90296=DIRECTION('ref_axis',(0.,0.,-1.));
#90297=DIRECTION('',(-0.190809912898503,0.,0.981627005099017));
#90298=DIRECTION('center_axis',(0.,-1.,0.));
#90299=DIRECTION('ref_axis',(-0.0618760686472822,0.,0.998083840230247));
#90300=DIRECTION('',(-0.190809912898503,0.,0.981627005099017));
#90301=DIRECTION('center_axis',(0.,-1.,0.));
#90302=DIRECTION('ref_axis',(-0.0652949673712366,0.,0.997866006654195));
#90303=DIRECTION('center_axis',(0.981627005099017,0.,0.190809912898503));
#90304=DIRECTION('ref_axis',(0.,-1.,0.));
#90305=DIRECTION('',(-0.190809912898503,0.,0.981627005099017));
#90306=DIRECTION('',(0.,1.,0.));
#90307=DIRECTION('center_axis',(0.981627005099017,1.50452980269455E-16,
0.190809912898503));
#90308=DIRECTION('ref_axis',(-0.158447752147023,0.557173939626296,0.815138951860889));
#90309=DIRECTION('center_axis',(0.981627005099017,2.31540729222364E-16,
0.190809912898504));
#90310=DIRECTION('ref_axis',(-0.158692756981343,0.555255482759283,0.816399386175306));
#90311=DIRECTION('center_axis',(0.,1.,0.));
#90312=DIRECTION('ref_axis',(1.,0.,0.));
#90313=DIRECTION('',(-0.190809912898503,0.,0.981627005099017));
#90314=DIRECTION('',(-0.981627005099017,0.,-0.190809912898503));
#90315=DIRECTION('center_axis',(0.,1.,0.));
#90316=DIRECTION('ref_axis',(-0.100377124109986,0.,0.994949462513252));
#90317=DIRECTION('center_axis',(-0.981627005099017,0.,-0.190809912898503));
#90318=DIRECTION('ref_axis',(-0.190809912898503,0.,0.981627005099017));
#90319=DIRECTION('center_axis',(-0.981627005099017,1.04674326304966E-16,
-0.190809912898503));
#90320=DIRECTION('ref_axis',(-0.161568217374531,0.531991649679407,0.831192273668253));
#90321=DIRECTION('',(-1.21473334453955E-14,-1.,-2.36121421336731E-15));
#90322=DIRECTION('center_axis',(-0.981627005099017,5.75453027144371E-17,
-0.190809912898503));
#90323=DIRECTION('ref_axis',(-0.162773155018957,0.521805547768498,0.837391109531975));
#90324=DIRECTION('center_axis',(-0.190809912898503,0.,0.981627005099017));
#90325=DIRECTION('ref_axis',(0.,1.,0.));
#90326=DIRECTION('center_axis',(0.190809912898503,5.8865115008751E-16,-0.981627005099017));
#90327=DIRECTION('ref_axis',(0.134946288550026,0.990505644687143,0.0262310321847858));
#90328=DIRECTION('center_axis',(0.,-1.,0.));
#90329=DIRECTION('ref_axis',(0.,0.,-1.));
#90330=DIRECTION('',(-0.190809912898503,0.,0.981627005099017));
#90331=DIRECTION('center_axis',(0.,-1.,0.));
#90332=DIRECTION('ref_axis',(0.0154999611699387,0.,0.999879868386063));
#90333=DIRECTION('',(-0.190809912898503,0.,0.981627005099017));
#90334=DIRECTION('center_axis',(0.,-1.,0.));
#90335=DIRECTION('ref_axis',(0.00998904194942923,0.,0.999950108275874));
#90336=DIRECTION('center_axis',(0.981627005099017,0.,0.190809912898503));
#90337=DIRECTION('ref_axis',(0.,-1.,0.));
#90338=DIRECTION('',(-0.19080991289849,0.,0.98162700509902));
#90339=DIRECTION('',(0.,1.,0.));
#90340=DIRECTION('center_axis',(0.981627005099017,-4.59929004743199E-17,
0.190809912898503));
#90341=DIRECTION('ref_axis',(-0.159944922126264,0.545298088879797,0.822841185253913));
#90342=DIRECTION('center_axis',(0.981627005099017,3.8312017680401E-16,0.190809912898504));
#90343=DIRECTION('ref_axis',(-0.158046000911432,0.560299179896621,0.813072131242412));
#90344=DIRECTION('center_axis',(0.,1.,0.));
#90345=DIRECTION('ref_axis',(1.,0.,0.));
#90346=DIRECTION('',(-0.190809912898503,0.,0.981627005099017));
#90347=DIRECTION('',(-0.981627005099017,0.,-0.190809912898503));
#90348=DIRECTION('center_axis',(0.,1.,0.));
#90349=DIRECTION('ref_axis',(-0.0237851745823533,0.,0.999717092716778));
#90350=DIRECTION('center_axis',(-0.981627005099017,0.,-0.190809912898503));
#90351=DIRECTION('ref_axis',(-0.190809912898503,0.,0.981627005099017));
#90352=DIRECTION('center_axis',(-0.981627005099017,4.55117302256744E-17,
-0.190809912898503));
#90353=DIRECTION('ref_axis',(-0.1611045890806,0.535839585425286,0.828807124769345));
#90354=DIRECTION('',(0.,-1.,0.));
#90355=DIRECTION('center_axis',(-0.981627005099017,-2.33394570578009E-16,
-0.190809912898504));
#90356=DIRECTION('ref_axis',(-0.162347493712948,0.525435160950585,0.835201282878539));
#90357=DIRECTION('center_axis',(-0.190809912898503,0.,0.981627005099017));
#90358=DIRECTION('ref_axis',(0.,1.,0.));
#90359=DIRECTION('center_axis',(0.190809912898503,6.99387505054468E-17,
-0.981627005099017));
#90360=DIRECTION('ref_axis',(0.247401529008408,0.967718871180627,0.0480902256721118));
#90361=DIRECTION('center_axis',(-0.981627005099017,0.,-0.190809912898503));
#90362=DIRECTION('ref_axis',(-0.190809912898503,0.,0.981627005099017));
#90363=DIRECTION('',(-0.190809912898503,0.,0.981627005099017));
#90364=DIRECTION('center_axis',(-0.981627005099017,1.08576435036114E-16,
-0.190809912898503));
#90365=DIRECTION('ref_axis',(-0.188102688558877,0.167853620862203,0.967699612752));
#90366=DIRECTION('',(-0.190809912898503,0.,0.981627005099017));
#90367=DIRECTION('center_axis',(-0.981627005099017,-8.82536396353935E-17,
-0.190809912898504));
#90368=DIRECTION('ref_axis',(-0.188243617855828,0.163456664470504,0.968424627514566));
#90369=DIRECTION('center_axis',(0.,-1.,0.));
#90370=DIRECTION('ref_axis',(0.,0.,-1.));
#90371=DIRECTION('',(-0.190809912898503,0.,0.981627005099017));
#90372=DIRECTION('',(0.981627005099017,0.,0.190809912898503));
#90373=DIRECTION('center_axis',(0.,-1.,0.));
#90374=DIRECTION('ref_axis',(0.382749389888478,0.,0.923852209252107));
#90375=DIRECTION('center_axis',(0.,-1.,0.));
#90376=DIRECTION('ref_axis',(0.388822090405444,0.,0.921312857835351));
#90377=DIRECTION('center_axis',(0.981627005099017,0.,0.190809912898503));
#90378=DIRECTION('ref_axis',(0.,-1.,0.));
#90379=DIRECTION('',(-0.190809912898469,0.,0.981627005099024));
#90380=DIRECTION('',(0.,1.,0.));
#90381=DIRECTION('center_axis',(0.981627005099017,5.14287578091947E-17,
0.190809912898504));
#90382=DIRECTION('ref_axis',(-0.18673928257389,0.205454980260091,0.960685532018732));
#90383=DIRECTION('center_axis',(0.,1.,0.));
#90384=DIRECTION('ref_axis',(1.,0.,0.));
#90385=DIRECTION('center_axis',(0.,1.,0.));
#90386=DIRECTION('ref_axis',(0.36800660983366,0.,0.929823174113625));
#90387=DIRECTION('',(-0.981627005099017,0.,-0.190809912898503));
#90388=DIRECTION('center_axis',(0.,1.,0.));
#90389=DIRECTION('ref_axis',(0.356362726694326,0.,0.934347690649998));
#90390=DIRECTION('center_axis',(-0.190809912898503,0.,0.981627005099017));
#90391=DIRECTION('ref_axis',(0.,1.,0.));
#90392=DIRECTION('center_axis',(0.190809912898503,2.33129168351489E-17,
-0.981627005099017));
#90393=DIRECTION('ref_axis',(0.933488573509569,0.309312139601285,0.181452702989912));
#90394=DIRECTION('center_axis',(-0.981627005099017,0.,-0.190809912898503));
#90395=DIRECTION('ref_axis',(-0.190809912898503,0.,0.981627005099017));
#90396=DIRECTION('',(-0.190809912898503,0.,0.981627005099017));
#90397=DIRECTION('center_axis',(-0.981627005099017,-9.56506689603866E-17,
-0.190809912898504));
#90398=DIRECTION('ref_axis',(-0.19000848861158,0.0915565204702765,0.977504055139885));
#90399=DIRECTION('',(-0.190809912898503,0.,0.981627005099017));
#90400=DIRECTION('center_axis',(-0.981627005099017,-2.69663898885924E-17,
-0.190809912898504));
#90401=DIRECTION('ref_axis',(-0.190050008447378,0.0891581806202793,0.977717655111962));
#90402=DIRECTION('center_axis',(0.,-1.,0.));
#90403=DIRECTION('ref_axis',(0.,0.,-1.));
#90404=DIRECTION('',(-0.190809912898503,0.,0.981627005099017));
#90405=DIRECTION('',(0.981627005099017,0.,0.190809912898503));
#90406=DIRECTION('center_axis',(0.,-1.,0.));
#90407=DIRECTION('ref_axis',(0.392668203964276,0.,0.919680206156178));
#90408=DIRECTION('center_axis',(0.,-1.,0.));
#90409=DIRECTION('ref_axis',(0.384550963585417,0.,0.923103762534596));
#90410=DIRECTION('center_axis',(0.981627005099017,0.,0.190809912898503));
#90411=DIRECTION('ref_axis',(0.,-1.,0.));
#90412=DIRECTION('',(-0.190809912898503,0.,0.981627005099017));
#90413=DIRECTION('',(0.,1.,0.));
#90414=DIRECTION('center_axis',(0.981627005099017,4.11430062473557E-17,
0.190809912898504));
#90415=DIRECTION('ref_axis',(-0.189206656454335,0.129360543126695,0.97337900688033));
#90416=DIRECTION('center_axis',(0.,1.,0.));
#90417=DIRECTION('ref_axis',(1.,0.,0.));
#90418=DIRECTION('center_axis',(0.,1.,0.));
#90419=DIRECTION('ref_axis',(0.36244598286257,0.,0.932004779766062));
#90420=DIRECTION('',(-0.981627005099017,0.,-0.190809912898503));
#90421=DIRECTION('center_axis',(0.,1.,0.));
#90422=DIRECTION('ref_axis',(0.351135646025879,0.,0.936324600814263));
#90423=DIRECTION('center_axis',(-0.190809912898503,0.,0.981627005099017));
#90424=DIRECTION('ref_axis',(0.,1.,0.));
#90425=DIRECTION('center_axis',(0.190809912898504,1.57362188637255E-16,
-0.981627005099017));
#90426=DIRECTION('ref_axis',(0.962831300769634,0.194752087897094,0.187156379848449));
#90427=DIRECTION('center_axis',(0.,-1.,0.));
#90428=DIRECTION('ref_axis',(0.,0.,-1.));
#90429=DIRECTION('',(-0.190809912898503,0.,0.981627005099017));
#90430=DIRECTION('center_axis',(0.,-1.,0.));
#90431=DIRECTION('ref_axis',(0.394709160970064,0.,0.918806115699231));
#90432=DIRECTION('',(-0.190809912898493,0.,0.981627005099019));
#90433=DIRECTION('center_axis',(0.,-1.,0.));
#90434=DIRECTION('ref_axis',(0.382819211217212,0.,0.92382327937925));
#90435=DIRECTION('center_axis',(0.981627005099017,0.,0.190809912898503));
#90436=DIRECTION('ref_axis',(0.,-1.,0.));
#90437=DIRECTION('',(-0.190809912898503,0.,0.981627005099017));
#90438=DIRECTION('center_axis',(0.981627005099017,6.7972359589236E-18,0.190809912898503));
#90439=DIRECTION('ref_axis',(-0.190523485063913,0.0547720629017275,0.980153468985643));
#90440=DIRECTION('center_axis',(0.981627005099017,1.02857515618389E-17,
0.190809912898503));
#90441=DIRECTION('ref_axis',(-0.190539030231083,0.0532661059933524,0.980233441538751));
#90442=DIRECTION('center_axis',(0.,1.,0.));
#90443=DIRECTION('ref_axis',(1.,0.,0.));
#90444=DIRECTION('',(-0.190809912898503,0.,0.981627005099017));
#90445=DIRECTION('center_axis',(0.,1.,0.));
#90446=DIRECTION('ref_axis',(0.359481261317514,0.,0.933152304161314));
#90447=DIRECTION('center_axis',(0.,1.,0.));
#90448=DIRECTION('ref_axis',(0.34834621044521,0.,0.937365946505665));
#90449=DIRECTION('center_axis',(-0.981627005099017,0.,-0.190809912898503));
#90450=DIRECTION('ref_axis',(-0.190809912898503,0.,0.981627005099017));
#90451=DIRECTION('center_axis',(-0.981627005099017,-3.23144151893198E-18,
-0.190809912898503));
#90452=DIRECTION('ref_axis',(-0.190787696570484,0.0152594200783794,0.981512712569838));
#90453=DIRECTION('center_axis',(-0.981627005099017,2.45148998987204E-18,
-0.190809912898503));
#90454=DIRECTION('ref_axis',(-0.190788845310911,0.0148596967700502,0.981518622297525));
#90455=DIRECTION('center_axis',(0.,-1.,0.));
#90456=DIRECTION('ref_axis',(0.,0.,-1.));
#90457=DIRECTION('',(-0.190809912898503,0.,0.981627005099017));
#90458=DIRECTION('center_axis',(0.,-1.,0.));
#90459=DIRECTION('ref_axis',(-0.574285234822728,0.,0.81865528097277));
#90460=DIRECTION('',(-0.190809912898503,0.,0.981627005099017));
#90461=DIRECTION('center_axis',(0.,-1.,0.));
#90462=DIRECTION('ref_axis',(-0.567322385194415,0.,0.823495787030705));
#90463=DIRECTION('center_axis',(0.981627005099017,0.,0.190809912898503));
#90464=DIRECTION('ref_axis',(0.,-1.,0.));
#90465=DIRECTION('',(-0.190809912898503,0.,0.981627005099017));
#90466=DIRECTION('center_axis',(0.981627005099017,2.11646646347863E-17,
0.190809912898504));
#90467=DIRECTION('ref_axis',(-0.190575246060068,0.049580034247521,0.980419754897441));
#90468=DIRECTION('center_axis',(0.981627005099017,1.06393782711632E-17,
0.190809912898504));
#90469=DIRECTION('ref_axis',(-0.190585783831876,0.0484547159815876,0.980473966763184));
#90470=DIRECTION('center_axis',(0.,1.,0.));
#90471=DIRECTION('ref_axis',(1.,0.,0.));
#90472=DIRECTION('',(-0.190809912898503,0.,0.981627005099017));
#90473=DIRECTION('center_axis',(0.,1.,0.));
#90474=DIRECTION('ref_axis',(-0.603515359960136,0.,0.797351371913404));
#90475=DIRECTION('center_axis',(0.,1.,0.));
#90476=DIRECTION('ref_axis',(-0.59604858216218,0.,0.802948371754035));
#90477=DIRECTION('center_axis',(-0.981627005099017,0.,-0.190809912898503));
#90478=DIRECTION('ref_axis',(-0.190809912898503,0.,0.981627005099017));
#90479=DIRECTION('center_axis',(-0.981627005099017,6.33476981587151E-18,
-0.190809912898503));
#90480=DIRECTION('ref_axis',(-0.190790116719056,0.0144043596890905,0.981525163092764));
#90481=DIRECTION('center_axis',(-0.981627005099017,-4.39364430834196E-18,
-0.190809912898504));
#90482=DIRECTION('ref_axis',(-0.190791033980825,0.0140667035476899,0.981529881971929));
#90483=DIRECTION('center_axis',(0.,-1.,0.));
#90484=DIRECTION('ref_axis',(0.,0.,-1.));
#90485=DIRECTION('',(-0.190809912898503,0.,0.981627005099017));
#90486=DIRECTION('center_axis',(0.,-1.,0.));
#90487=DIRECTION('ref_axis',(-0.575359874209948,0.,0.817900369940687));
#90488=DIRECTION('',(-0.190809912898503,0.,0.981627005099017));
#90489=DIRECTION('center_axis',(0.,-1.,0.));
#90490=DIRECTION('ref_axis',(-0.568338838106609,0.,0.822794606873204));
#90491=DIRECTION('center_axis',(0.981627005099017,0.,0.190809912898503));
#90492=DIRECTION('ref_axis',(0.,-1.,0.));
#90493=DIRECTION('',(-0.190809912898503,0.,0.981627005099017));
#90494=DIRECTION('center_axis',(0.981627005099017,2.22785943524066E-17,
0.190809912898503));
#90495=DIRECTION('ref_axis',(-0.189421658366475,0.120408654601104,0.97448509031121));
#90496=DIRECTION('center_axis',(0.981627005099017,4.25575130846527E-17,
0.190809912898504));
#90497=DIRECTION('ref_axis',(-0.189484179630181,0.1176757388124,0.974806732724407));
#90498=DIRECTION('center_axis',(0.,1.,0.));
#90499=DIRECTION('ref_axis',(1.,0.,0.));
#90500=DIRECTION('',(-0.190809912898503,0.,0.981627005099017));
#90501=DIRECTION('center_axis',(0.,1.,0.));
#90502=DIRECTION('ref_axis',(-0.605496675700037,0.,0.795847834523789));
#90503=DIRECTION('center_axis',(0.,1.,0.));
#90504=DIRECTION('ref_axis',(-0.597922812738481,0.,0.801553685043555));
#90505=DIRECTION('center_axis',(-0.981627005099017,0.,-0.190809912898503));
#90506=DIRECTION('ref_axis',(-0.190809912898503,0.,0.981627005099017));
#90507=DIRECTION('center_axis',(-0.981627005099017,-2.30355266031692E-18,
-0.190809912898503));
#90508=DIRECTION('ref_axis',(-0.190095951678253,0.0864261581345065,0.977954011365386));
#90509=DIRECTION('center_axis',(-0.981627005099017,-3.51491544667356E-17,
-0.190809912898504));
#90510=DIRECTION('ref_axis',(-0.190129090875907,0.0844002212861198,0.978124496906991));
#90511=DIRECTION('center_axis',(0.,-1.,0.));
#90512=DIRECTION('ref_axis',(0.,0.,-1.));
#90513=DIRECTION('',(-0.190809912898503,0.,0.981627005099017));
#90514=DIRECTION('center_axis',(0.,-1.,0.));
#90515=DIRECTION('ref_axis',(-0.578008173140809,0.,0.816030974768988));
#90516=DIRECTION('',(-0.190809912898503,0.,0.981627005099017));
#90517=DIRECTION('center_axis',(0.,-1.,0.));
#90518=DIRECTION('ref_axis',(-0.570842395473156,0.,0.82105965649913));
#90519=DIRECTION('center_axis',(0.981627005099017,0.,0.190809912898503));
#90520=DIRECTION('ref_axis',(0.,-1.,0.));
#90521=DIRECTION('',(-0.190809912898503,0.,0.981627005099017));
#90522=DIRECTION('center_axis',(0.981627005099017,7.12915019277012E-17,
0.190809912898504));
#90523=DIRECTION('ref_axis',(-0.187288294113551,0.191237274954706,0.963509937445346));
#90524=DIRECTION('center_axis',(0.981627005099017,-4.25575130846527E-18,
0.190809912898503));
#90525=DIRECTION('ref_axis',(-0.187447758333338,0.186896761643308,0.964330305643793));
#90526=DIRECTION('center_axis',(0.,1.,0.));
#90527=DIRECTION('ref_axis',(1.,0.,0.));
#90528=DIRECTION('',(-0.190809912898503,0.,0.981627005099017));
#90529=DIRECTION('center_axis',(0.,1.,0.));
#90530=DIRECTION('ref_axis',(-0.609205159578384,0.,0.793012656609638));
#90531=DIRECTION('center_axis',(0.,1.,0.));
#90532=DIRECTION('ref_axis',(-0.601428192999473,0.,0.798926860648325));
#90533=DIRECTION('center_axis',(-0.981627005099017,0.,-0.190809912898503));
#90534=DIRECTION('ref_axis',(-0.190809912898503,0.,0.981627005099017));
#90535=DIRECTION('center_axis',(-0.981627005099017,-7.37136851301412E-17,
-0.190809912898504));
#90536=DIRECTION('ref_axis',(-0.188399474304184,0.158447956579895,0.969226435430629));
#90537=DIRECTION('center_axis',(-0.981627005099017,-1.31809329250259E-17,
-0.190809912898503));
#90538=DIRECTION('ref_axis',(-0.188511838100476,0.154733739024593,0.969804494165421));
#90539=DIRECTION('center_axis',(0.,-1.,0.));
#90540=DIRECTION('ref_axis',(0.,0.,-1.));
#90541=DIRECTION('',(-0.190809912898514,0.,0.981627005099015));
#90542=DIRECTION('center_axis',(0.,-1.,0.));
#90543=DIRECTION('ref_axis',(-0.58233026870445,0.,0.812952309886996));
#90544=DIRECTION('',(-0.190809912898503,0.,0.981627005099017));
#90545=DIRECTION('center_axis',(0.,-1.,0.));
#90546=DIRECTION('ref_axis',(-0.574924123248839,0.,0.818206729687891));
#90547=DIRECTION('center_axis',(0.981627005099017,0.,0.190809912898503));
#90548=DIRECTION('ref_axis',(0.,-1.,0.));
#90549=DIRECTION('',(-0.190809912898503,0.,0.981627005099017));
#90550=DIRECTION('center_axis',(0.981627005099017,3.56457509638507E-17,
0.190809912898503));
#90551=DIRECTION('ref_axis',(-0.184141102885343,0.26206589530831,0.94731912296988));
#90552=DIRECTION('center_axis',(0.981627005099017,1.70230052338611E-16,
0.190809912898504));
#90553=DIRECTION('ref_axis',(-0.184445559233683,0.256117784474097,0.948885407283226));
#90554=DIRECTION('center_axis',(0.,1.,0.));
#90555=DIRECTION('ref_axis',(1.,0.,0.));
#90556=DIRECTION('',(-0.190809912898503,0.,0.981627005099017));
#90557=DIRECTION('center_axis',(0.,1.,0.));
#90558=DIRECTION('ref_axis',(-0.614783199716477,0.,0.788696150203847));
#90559=DIRECTION('center_axis',(0.,1.,0.));
#90560=DIRECTION('ref_axis',(-0.606694140002808,0.,0.794935356168194));
#90561=DIRECTION('center_axis',(-0.981627005099017,0.,-0.190809912898503));
#90562=DIRECTION('ref_axis',(-0.190809912898503,0.,0.981627005099017));
#90563=DIRECTION('center_axis',(-0.981627005099017,-6.44994744888736E-17,
-0.190809912898504));
#90564=DIRECTION('ref_axis',(-0.185673212549806,0.230469755025396,0.955201104563834));
#90565=DIRECTION('center_axis',(-0.981627005099017,-6.15110203167874E-17,
-0.190809912898503));
#90566=DIRECTION('ref_axis',(-0.185914346858001,0.225067256763002,0.956441626846897));
#90567=DIRECTION('center_axis',(0.,-1.,0.));
#90568=DIRECTION('ref_axis',(0.,0.,-1.));
#90569=DIRECTION('',(-0.190809912898503,0.,0.981627005099017));
#90570=DIRECTION('center_axis',(0.,-1.,0.));
#90571=DIRECTION('ref_axis',(-0.588497763347602,0.,0.808498845104228));
#90572=DIRECTION('',(-0.190809912898503,0.,0.981627005099017));
#90573=DIRECTION('center_axis',(0.,-1.,0.));
#90574=DIRECTION('ref_axis',(-0.580739637394756,0.,0.814089352318655));
#90575=DIRECTION('center_axis',(0.981627005099017,0.,0.190809912898503));
#90576=DIRECTION('ref_axis',(0.,-1.,0.));
#90577=DIRECTION('',(-0.190809912898503,0.,0.981627005099017));
#90578=DIRECTION('center_axis',(0.981627005099017,1.3367156611444E-16,0.190809912898504));
#90579=DIRECTION('ref_axis',(-0.179926892481102,0.332894515661892,0.925638998100409));
#90580=DIRECTION('center_axis',(0.981627005099017,-1.36184041870889E-16,
0.190809912898503));
#90581=DIRECTION('ref_axis',(-0.180429379482987,0.325338807305,0.928224056723776));
#90582=DIRECTION('center_axis',(0.,1.,0.));
#90583=DIRECTION('ref_axis',(1.,0.,0.));
#90584=DIRECTION('',(-0.190809912898503,0.,0.981627005099017));
#90585=DIRECTION('center_axis',(0.,1.,0.));
#90586=DIRECTION('ref_axis',(-0.622458164940441,0.,0.782653073142232));
#90587=DIRECTION('center_axis',(0.,1.,0.));
#90588=DIRECTION('ref_axis',(-0.613926597176052,0.,0.789363118773504));
#90589=DIRECTION('center_axis',(-0.981627005099017,0.,-0.190809912898503));
#90590=DIRECTION('ref_axis',(-0.190809912898503,0.,0.981627005099017));
#90591=DIRECTION('center_axis',(-0.981627005099017,-2.11926844749156E-16,
-0.190809912898504));
#90592=DIRECTION('ref_axis',(-0.181870862608285,0.302491553470801,0.935639807518331));
#90593=DIRECTION('center_axis',(-0.981627005099017,-3.33916967433989E-16,
-0.190809912898504));
#90594=DIRECTION('ref_axis',(-0.182294720132399,0.295400774501413,0.937820354564677));
#90595=DIRECTION('center_axis',(0.,-1.,0.));
#90596=DIRECTION('ref_axis',(0.,0.,-1.));
#90597=DIRECTION('center_axis',(0.,-1.,0.));
#90598=DIRECTION('ref_axis',(-0.588526570035615,0.,0.808477876235407));
#90599=DIRECTION('',(-0.190809912898503,0.,0.981627005099017));
#90600=DIRECTION('center_axis',(0.,-1.,0.));
#90601=DIRECTION('ref_axis',(-0.596773820946327,0.,0.802409500587525));
#90602=DIRECTION('',(-0.190809912898503,0.,0.981627005099017));
#90603=DIRECTION('center_axis',(0.981627005099017,0.,0.190809912898503));
#90604=DIRECTION('ref_axis',(0.,-1.,0.));
#90605=DIRECTION('center_axis',(0.981627005099017,1.70230052338611E-16,
0.190809912898504));
#90606=DIRECTION('ref_axis',(-0.175329552794068,0.394559830135812,0.901987853776442));
#90607=DIRECTION('',(-0.190809912898503,0.,0.981627005099017));
#90608=DIRECTION('center_axis',(0.981627005099017,3.0298888319273E-16,0.190809912898504));
#90609=DIRECTION('ref_axis',(-0.174568404100475,0.403723136015587,0.898072102748745));
#90610=DIRECTION('center_axis',(0.,1.,0.));
#90611=DIRECTION('ref_axis',(1.,0.,0.));
#90612=DIRECTION('',(-0.981627005099017,0.,-0.190809912898503));
#90613=DIRECTION('center_axis',(0.,1.,0.));
#90614=DIRECTION('ref_axis',(-0.620988661056824,0.,0.783819547369707));
#90615=DIRECTION('center_axis',(0.,1.,0.));
#90616=DIRECTION('ref_axis',(-0.623432047557978,0.,0.781877536496392));
#90617=DIRECTION('',(-0.190809912898503,0.,0.981627005099017));
#90618=DIRECTION('center_axis',(-0.981627005099017,0.,-0.190809912898503));
#90619=DIRECTION('ref_axis',(-0.190809912898503,0.,0.981627005099017));
#90620=DIRECTION('center_axis',(-0.981627005099017,-2.81193235733885E-16,
-0.190809912898504));
#90621=DIRECTION('ref_axis',(-0.177590469804984,0.365734292239907,0.913619205421066));
#90622=DIRECTION('center_axis',(-0.981627005099017,-9.21421064126765E-17,
-0.190809912898504));
#90623=DIRECTION('ref_axis',(-0.176923057683389,0.374513351916211,0.910185684844826));
#90624=DIRECTION('',(0.,-1.,0.));
#90625=DIRECTION('center_axis',(-0.190809912898503,0.,0.981627005099017));
#90626=DIRECTION('ref_axis',(0.,1.,0.));
#90627=DIRECTION('center_axis',(0.190809912898504,-5.12884170373276E-16,
-0.981627005099017));
#90628=DIRECTION('ref_axis',(-0.764695635116802,0.627013547027167,-0.148642515713782));
#90629=DIRECTION('center_axis',(0.,-1.,0.));
#90630=DIRECTION('ref_axis',(0.,0.,-1.));
#90631=DIRECTION('',(-0.190809912898503,0.,0.981627005099017));
#90632=DIRECTION('center_axis',(0.,-1.,0.));
#90633=DIRECTION('ref_axis',(-0.489658531934886,0.,0.87191428598422));
#90634=DIRECTION('',(-0.190809912898503,0.,0.981627005099017));
#90635=DIRECTION('center_axis',(0.,-1.,0.));
#90636=DIRECTION('ref_axis',(-0.482690338571901,0.,0.875791092127194));
#90637=DIRECTION('center_axis',(0.981627005099017,0.,0.190809912898503));
#90638=DIRECTION('ref_axis',(0.,-1.,0.));
#90639=DIRECTION('',(-0.190809912898503,0.,0.981627005099017));
#90640=DIRECTION('',(0.,1.,0.));
#90641=DIRECTION('center_axis',(0.981627005099017,1.44986047536651E-16,
0.190809912898504));
#90642=DIRECTION('ref_axis',(-0.163956083486876,0.511532430965294,0.843476718563341));
#90643=DIRECTION('center_axis',(0.981627005099017,2.00892259541186E-16,
0.190809912898504));
#90644=DIRECTION('ref_axis',(-0.164374305125881,0.507832564945586,0.845628271639005));
#90645=DIRECTION('center_axis',(0.,1.,0.));
#90646=DIRECTION('ref_axis',(1.,0.,0.));
#90647=DIRECTION('',(-0.190809912898503,0.,0.981627005099017));
#90648=DIRECTION('',(-0.981627005099017,0.,-0.190809912898503));
#90649=DIRECTION('center_axis',(0.,1.,0.));
#90650=DIRECTION('ref_axis',(-0.521450772443428,0.,0.853281367380158));
#90651=DIRECTION('center_axis',(-0.981627005099017,0.,-0.190809912898503));
#90652=DIRECTION('ref_axis',(-0.190809912898503,0.,0.981627005099017));
#90653=DIRECTION('center_axis',(-0.981627005099017,4.93467903960143E-17,
-0.190809912898503));
#90654=DIRECTION('ref_axis',(-0.166342338650152,0.489915545565209,0.855752875885288));
#90655=DIRECTION('',(0.,-1.,0.));
#90656=DIRECTION('center_axis',(-0.981627005099017,-4.72957903022569E-17,
-0.190809912898503));
#90657=DIRECTION('ref_axis',(-0.167430516953427,0.479626321074999,0.861351040009107));
#90658=DIRECTION('center_axis',(-0.190809912898503,0.,0.981627005099017));
#90659=DIRECTION('ref_axis',(0.,1.,0.));
#90660=DIRECTION('center_axis',(0.190809912898503,-8.15952089230212E-17,
-0.981627005099017));
#90661=DIRECTION('ref_axis',(-0.539785154200082,0.835238238177304,-0.104924128739137));
#90662=DIRECTION('center_axis',(0.,-1.,0.));
#90663=DIRECTION('ref_axis',(0.,0.,-1.));
#90664=DIRECTION('',(-0.190809912898503,0.,0.981627005099017));
#90665=DIRECTION('center_axis',(0.,-1.,0.));
#90666=DIRECTION('ref_axis',(-0.42194565501119,0.,0.906621124956383));
#90667=DIRECTION('',(-0.190809912898503,0.,0.981627005099017));
#90668=DIRECTION('center_axis',(0.,-1.,0.));
#90669=DIRECTION('ref_axis',(-0.416507743824211,0.,0.909132168243136));
#90670=DIRECTION('center_axis',(0.981627005099017,0.,0.190809912898503));
#90671=DIRECTION('ref_axis',(0.,-1.,0.));
#90672=DIRECTION('',(-0.190809912898503,0.,0.981627005099017));
#90673=DIRECTION('center_axis',(0.981627005099017,-7.78644601242735E-17,
0.190809912898503));
#90674=DIRECTION('ref_axis',(-0.1641530299532,0.509794631015901,0.84448991524147));
#90675=DIRECTION('center_axis',(0.981627005099017,1.4958748237708E-16,0.190809912898503));
#90676=DIRECTION('ref_axis',(-0.165285739249462,0.499641205524799,0.850317170320866));
#90677=DIRECTION('center_axis',(0.,1.,0.));
#90678=DIRECTION('ref_axis',(1.,0.,0.));
#90679=DIRECTION('',(-0.190809912898503,0.,0.981627005099017));
#90680=DIRECTION('center_axis',(0.,1.,0.));
#90681=DIRECTION('ref_axis',(-0.461221229340861,0.,0.887285172650431));
#90682=DIRECTION('center_axis',(0.,1.,0.));
#90683=DIRECTION('ref_axis',(-0.45463858135335,0.,0.890676013118695));
#90684=DIRECTION('center_axis',(-0.981627005099017,0.,-0.190809912898503));
#90685=DIRECTION('ref_axis',(-0.190809912898503,0.,0.981627005099017));
#90686=DIRECTION('center_axis',(-0.981627005099017,3.1638104497012E-17,
-0.190809912898503));
#90687=DIRECTION('ref_axis',(-0.167345158855712,0.480443832419612,0.860911912856079));
#90688=DIRECTION('center_axis',(-0.981627005099017,1.21485874416176E-16,
-0.190809912898503));
#90689=DIRECTION('ref_axis',(-0.16834743337274,0.470728280640113,0.86606814251675));
#90690=DIRECTION('center_axis',(0.,-1.,0.));
#90691=DIRECTION('ref_axis',(0.,0.,-1.));
#90692=DIRECTION('',(-0.190809912898503,0.,0.981627005099017));
#90693=DIRECTION('center_axis',(0.,-1.,0.));
#90694=DIRECTION('ref_axis',(-0.353115435082057,0.,0.935579761167806));
#90695=DIRECTION('',(-0.190809912898503,0.,0.981627005099017));
#90696=DIRECTION('center_axis',(0.,-1.,0.));
#90697=DIRECTION('ref_axis',(-0.349265854344674,0.,0.937023672587243));
#90698=DIRECTION('center_axis',(0.981627005099017,0.,0.190809912898503));
#90699=DIRECTION('ref_axis',(0.,-1.,0.));
#90700=DIRECTION('',(-0.190809912898503,0.,0.981627005099017));
#90701=DIRECTION('center_axis',(0.981627005099017,2.7359611324339E-16,0.190809912898504));
#90702=DIRECTION('ref_axis',(-0.164842107563918,0.503650570550101,0.848034894540575));
#90703=DIRECTION('center_axis',(0.981627005099017,8.76849763688622E-17,
0.190809912898503));
#90704=DIRECTION('ref_axis',(-0.165917896355328,0.493852879734794,0.853569320469447));
#90705=DIRECTION('center_axis',(0.,1.,0.));
#90706=DIRECTION('ref_axis',(1.,0.,0.));
#90707=DIRECTION('',(-0.190809912898503,0.,0.981627005099017));
#90708=DIRECTION('center_axis',(0.,1.,0.));
#90709=DIRECTION('ref_axis',(-0.391618463739157,0.,0.920127697039157));
#90710=DIRECTION('center_axis',(0.,1.,0.));
#90711=DIRECTION('ref_axis',(-0.386687356930034,0.,0.922210869590282));
#90712=DIRECTION('center_axis',(-0.981627005099017,0.,-0.190809912898503));
#90713=DIRECTION('ref_axis',(-0.190809912898503,0.,0.981627005099017));
#90714=DIRECTION('center_axis',(-0.981627005099017,-4.76390639943534E-16,
-0.190809912898504));
#90715=DIRECTION('ref_axis',(-0.168060481549877,0.473536168037885,0.864591910730848));
#90716=DIRECTION('center_axis',(-0.981627005099017,-8.86144962521498E-17,
-0.190809912898503));
#90717=DIRECTION('ref_axis',(-0.169003575142171,0.464225672106184,0.869443682446843));
#90718=DIRECTION('center_axis',(0.,-1.,0.));
#90719=DIRECTION('ref_axis',(0.,0.,-1.));
#90720=DIRECTION('',(-0.190809912898503,0.,0.981627005099017));
#90721=DIRECTION('center_axis',(0.,-1.,0.));
#90722=DIRECTION('ref_axis',(-0.283219375007823,0.,0.95905515254347));
#90723=DIRECTION('',(-0.190809912898503,0.,0.981627005099017));
#90724=DIRECTION('center_axis',(0.,-1.,0.));
#90725=DIRECTION('ref_axis',(-0.281011109742765,0.,0.959704515046761));
#90726=DIRECTION('center_axis',(0.981627005099017,0.,0.190809912898503));
#90727=DIRECTION('ref_axis',(0.,-1.,0.));
#90728=DIRECTION('',(-0.190809912898503,0.,0.981627005099017));
#90729=DIRECTION('center_axis',(0.981627005099017,1.64661493304004E-16,
0.190809912898504));
#90730=DIRECTION('ref_axis',(-0.165266478237664,0.499816171268802,0.85021808149975));
#90731=DIRECTION('center_axis',(0.981627005099017,2.88018088012718E-16,
0.190809912898504));
#90732=DIRECTION('ref_axis',(-0.166307924300349,0.490236343963907,0.855575830287305));
#90733=DIRECTION('center_axis',(0.,1.,0.));
#90734=DIRECTION('ref_axis',(1.,0.,0.));
#90735=DIRECTION('',(-0.190809912898503,0.,0.981627005099017));
#90736=DIRECTION('center_axis',(0.,1.,0.));
#90737=DIRECTION('ref_axis',(-0.320878589892636,0.,0.947120335833052));
#90738=DIRECTION('center_axis',(0.,1.,0.));
#90739=DIRECTION('ref_axis',(-0.317659115433943,0.,0.948204981204868));
#90740=DIRECTION('center_axis',(-0.981627005099017,0.,-0.190809912898503));
#90741=DIRECTION('ref_axis',(-0.190809912898503,0.,0.981627005099017));
#90742=DIRECTION('center_axis',(-0.981627005099017,-4.97231835007436E-16,
-0.190809912898504));
#90743=DIRECTION('ref_axis',(-0.168533680974174,0.468894226820799,0.867026298581202));
#90744=DIRECTION('center_axis',(-0.981627005099017,-5.79678245784151E-17,
-0.190809912898503));
#90745=DIRECTION('ref_axis',(-0.169438586252028,0.459849689864406,0.871681609431175));
#90746=DIRECTION('center_axis',(0.,-1.,0.));
#90747=DIRECTION('ref_axis',(0.,0.,-1.));
#90748=DIRECTION('',(-0.190809912898503,0.,0.981627005099017));
#90749=DIRECTION('center_axis',(0.,-1.,0.));
#90750=DIRECTION('ref_axis',(-0.212288523804663,0.,0.977207031626787));
#90751=DIRECTION('',(-0.190809912898503,0.,0.981627005099017));
#90752=DIRECTION('center_axis',(0.,-1.,0.));
#90753=DIRECTION('ref_axis',(-0.211771596214555,0.,0.977319185853189));
#90754=DIRECTION('center_axis',(0.981627005099017,0.,0.190809912898503));
#90755=DIRECTION('ref_axis',(0.,-1.,0.));
#90756=DIRECTION('',(-0.190809912898503,0.,0.981627005099017));
#90757=DIRECTION('center_axis',(0.981627005099017,5.94759471576322E-17,
0.190809912898503));
#90758=DIRECTION('ref_axis',(-0.165450643172752,0.498139876682696,0.851165523228162));
#90759=DIRECTION('center_axis',(0.981627005099017,7.15405393416096E-17,
0.190809912898503));
#90760=DIRECTION('ref_axis',(-0.166477354471641,0.488654299036596,0.856447468605738));
#90761=DIRECTION('center_axis',(0.,1.,0.));
#90762=DIRECTION('ref_axis',(1.,0.,0.));
#90763=DIRECTION('',(-0.190809912898503,0.,0.981627005099017));
#90764=DIRECTION('center_axis',(0.,1.,0.));
#90765=DIRECTION('ref_axis',(-0.249046035387048,0.,0.968491648006318));
#90766=DIRECTION('center_axis',(0.,1.,0.));
#90767=DIRECTION('ref_axis',(-0.247593816860215,0.,0.968863923289845));
#90768=DIRECTION('center_axis',(-0.981627005099017,0.,-0.190809912898503));
#90769=DIRECTION('ref_axis',(-0.190809912898503,0.,0.981627005099017));
#90770=DIRECTION('center_axis',(-0.981627005099017,-1.19226339786349E-16,
-0.190809912898503));
#90771=DIRECTION('ref_axis',(-0.168792500449209,0.466330160156009,0.868357802706335));
#90772=DIRECTION('center_axis',(-0.981627005099017,4.30196144549347E-17,
-0.190809912898503));
#90773=DIRECTION('ref_axis',(-0.169676842617203,0.457430398202074,0.872907326054805));
#90774=DIRECTION('center_axis',(0.,-1.,0.));
#90775=DIRECTION('ref_axis',(0.,0.,-1.));
#90776=DIRECTION('',(-0.190809912898503,0.,0.981627005099017));
#90777=DIRECTION('center_axis',(0.,-1.,0.));
#90778=DIRECTION('ref_axis',(-0.140336198717109,0.,0.990103909359837));
#90779=DIRECTION('',(-0.190809912898503,0.,0.981627005099017));
#90780=DIRECTION('center_axis',(0.,-1.,0.));
#90781=DIRECTION('ref_axis',(-0.141559381142733,0.,0.989929765998824));
#90782=DIRECTION('center_axis',(0.981627005099017,0.,0.190809912898503));
#90783=DIRECTION('ref_axis',(0.,-1.,0.));
#90784=DIRECTION('',(-0.190809912898503,0.,0.981627005099017));
#90785=DIRECTION('center_axis',(0.981627005099017,3.12772334456263E-16,
0.190809912898504));
#90786=DIRECTION('ref_axis',(-0.165404852718561,0.498557368703801,0.850929952938721));
#90787=DIRECTION('center_axis',(0.981627005099017,3.1528628345683E-16,0.190809912898504));
#90788=DIRECTION('ref_axis',(-0.166435218084341,0.48904837398272,0.856230696766984));
#90789=DIRECTION('center_axis',(0.,1.,0.));
#90790=DIRECTION('ref_axis',(1.,0.,0.));
#90791=DIRECTION('',(-0.190809912898503,0.,0.981627005099017));
#90792=DIRECTION('center_axis',(0.,1.,0.));
#90793=DIRECTION('ref_axis',(-0.176144643249429,0.,0.984364294686947));
#90794=DIRECTION('center_axis',(0.,1.,0.));
#90795=DIRECTION('ref_axis',(-0.176512963578363,0.,0.984298315394669));
#90796=DIRECTION('center_axis',(-0.981627005099017,0.,-0.190809912898503));
#90797=DIRECTION('ref_axis',(-0.190809912898503,0.,0.981627005099017));
#90798=DIRECTION('center_axis',(-0.981627005099017,-2.0812226289074E-16,
-0.190809912898504));
#90799=DIRECTION('ref_axis',(-0.168851372823095,0.465744402600315,0.868660673302431));
#90800=DIRECTION('center_axis',(-0.981627005099017,-3.5763068107684E-16,
-0.190809912898504));
#90801=DIRECTION('ref_axis',(-0.169731069638787,0.456877502295317,0.873186298504314));
#90802=DIRECTION('center_axis',(0.,-1.,0.));
#90803=DIRECTION('ref_axis',(0.,0.,-1.));
#90804=DIRECTION('',(-0.190809912898503,0.,0.981627005099017));
#90805=DIRECTION('center_axis',(0.,-1.,0.));
#90806=DIRECTION('ref_axis',(-0.0673590974157918,0.,0.997728796815713));
#90807=DIRECTION('',(-0.190809912898503,0.,0.981627005099017));
#90808=DIRECTION('center_axis',(0.,-1.,0.));
#90809=DIRECTION('ref_axis',(-0.0703714709533455,0.,0.997520854957861));
#90810=DIRECTION('center_axis',(0.981627005099017,0.,0.190809912898503));
#90811=DIRECTION('ref_axis',(0.,-1.,0.));
#90812=DIRECTION('',(-0.190809912898503,0.,0.981627005099017));
#90813=DIRECTION('center_axis',(0.981627005099017,1.654982782964E-16,0.190809912898504));
#90814=DIRECTION('ref_axis',(-0.165126579629839,0.501084557252584,0.849498369146599));
#90815=DIRECTION('center_axis',(0.981627005099017,1.73655546916773E-16,
0.190809912898504));
#90816=DIRECTION('ref_axis',(-0.166179287158349,0.491433013476625,0.854914052864279));
#90817=DIRECTION('center_axis',(0.,1.,0.));
#90818=DIRECTION('ref_axis',(1.,0.,0.));
#90819=DIRECTION('',(-0.190809912898503,0.,0.981627005099017));
#90820=DIRECTION('center_axis',(0.,1.,0.));
#90821=DIRECTION('ref_axis',(-0.102179792300205,0.,0.994765947369273));
#90822=DIRECTION('center_axis',(0.,1.,0.));
#90823=DIRECTION('ref_axis',(-0.104421411927276,0.,0.994533141092399));
#90824=DIRECTION('center_axis',(-0.981627005099017,0.,-0.190809912898503));
#90825=DIRECTION('ref_axis',(-0.190809912898503,0.,0.981627005099017));
#90826=DIRECTION('center_axis',(-0.981627005099017,-7.47673759321185E-17,
-0.190809912898503));
#90827=DIRECTION('ref_axis',(-0.16871350914603,0.467114619230688,0.867951429708254));
#90828=DIRECTION('center_axis',(-0.981627005099017,8.63179540716556E-17,
-0.190809912898503));
#90829=DIRECTION('ref_axis',(-0.169604102816414,0.458170724869904,0.872533114087956));
#90830=DIRECTION('center_axis',(0.,-1.,0.));
#90831=DIRECTION('ref_axis',(0.,0.,-1.));
#90832=DIRECTION('',(-0.190809912898503,0.,0.981627005099017));
#90833=DIRECTION('center_axis',(0.,-1.,0.));
#90834=DIRECTION('ref_axis',(0.00666297473127236,0.,0.999977802137493));
#90835=DIRECTION('',(-0.190809912898503,0.,0.981627005099017));
#90836=DIRECTION('center_axis',(0.,-1.,0.));
#90837=DIRECTION('ref_axis',(0.00181042398919864,0.,0.999998361181147));
#90838=DIRECTION('center_axis',(0.981627005099017,0.,0.190809912898503));
#90839=DIRECTION('ref_axis',(0.,-1.,0.));
#90840=DIRECTION('',(-0.190809912898503,0.,0.981627005099017));
#90841=DIRECTION('center_axis',(0.981627005099017,-3.37281270145013E-16,
0.190809912898503));
#90842=DIRECTION('ref_axis',(-0.164600160397928,0.505819296281817,0.846790190487552));
#90843=DIRECTION('center_axis',(0.981627005099017,2.65237045479699E-16,
0.190809912898504));
#90844=DIRECTION('ref_axis',(-0.165695772046853,0.495896975310785,0.852426595668748));
#90845=DIRECTION('center_axis',(0.,1.,0.));
#90846=DIRECTION('ref_axis',(1.,0.,0.));
#90847=DIRECTION('',(-0.190809912898503,0.,0.981627005099017));
#90848=DIRECTION('center_axis',(0.,1.,0.));
#90849=DIRECTION('ref_axis',(-0.027138860824711,0.,0.999631673284284));
#90850=DIRECTION('center_axis',(0.,1.,0.));
#90851=DIRECTION('ref_axis',(-0.0313077694633037,0.,0.999509791633495));
#90852=DIRECTION('center_axis',(-0.981627005099017,0.,-0.190809912898503));
#90853=DIRECTION('ref_axis',(-0.190809912898503,0.,0.981627005099017));
#90854=DIRECTION('center_axis',(-0.981627005099017,4.55117302256744E-17,
-0.190809912898503));
#90855=DIRECTION('ref_axis',(-0.168371348274985,0.470493294519803,0.866191173409177));
#90856=DIRECTION('center_axis',(-0.981627005099017,-2.77156052561386E-16,
-0.190809912898504));
#90857=DIRECTION('ref_axis',(-0.169289267864162,0.461357702298085,0.870913436752613));
#90858=DIRECTION('center_axis',(0.,-1.,0.));
#90859=DIRECTION('ref_axis',(0.,0.,-1.));
#90860=DIRECTION('',(-0.190809912898503,0.,0.981627005099017));
#90861=DIRECTION('center_axis',(0.,-1.,0.));
#90862=DIRECTION('ref_axis',(0.081768816582179,0.,0.996651323500225));
#90863=DIRECTION('',(-0.190809912898503,0.,0.981627005099017));
#90864=DIRECTION('center_axis',(0.,-1.,0.));
#90865=DIRECTION('ref_axis',(0.0750213618657929,0.,0.9971819268638));
#90866=DIRECTION('center_axis',(0.981627005099017,0.,0.190809912898503));
#90867=DIRECTION('ref_axis',(0.,-1.,0.));
#90868=DIRECTION('',(-0.190809912898503,0.,0.981627005099017));
#90869=DIRECTION('center_axis',(0.981627005099017,-9.45984020779368E-17,
0.190809912898503));
#90870=DIRECTION('ref_axis',(-0.163794505829796,0.512952199260781,0.842645477726844));
#90871=DIRECTION('center_axis',(0.981627005099017,4.54116221843461E-17,
0.190809912898503));
#90872=DIRECTION('ref_axis',(-0.164957395957987,0.502612750449379,0.848627998951525));
#90873=DIRECTION('center_axis',(0.,1.,0.));
#90874=DIRECTION('ref_axis',(1.,0.,0.));
#90875=DIRECTION('',(-0.190809912898503,0.,0.981627005099017));
#90876=DIRECTION('center_axis',(0.,1.,0.));
#90877=DIRECTION('ref_axis',(0.0490098699559957,0.,0.998798294275124));
#90878=DIRECTION('center_axis',(0.,1.,0.));
#90879=DIRECTION('ref_axis',(0.0428565438402263,0.,0.999081236261632));
#90880=DIRECTION('center_axis',(-0.981627005099017,0.,-0.190809912898503));
#90881=DIRECTION('ref_axis',(-0.190809912898503,0.,0.981627005099017));
#90882=DIRECTION('center_axis',(-0.981627005099017,1.08700534976828E-16,
-0.190809912898503));
#90883=DIRECTION('ref_axis',(-0.167805489378009,0.476013437950482,0.863280096275345));
#90884=DIRECTION('center_axis',(-0.981627005099017,-3.87865929651451E-16,
-0.190809912898504));
#90885=DIRECTION('ref_axis',(-0.168769478873421,0.466558960501992,0.868239367557182));
#90886=DIRECTION('center_axis',(0.,-1.,0.));
#90887=DIRECTION('ref_axis',(0.,0.,-1.));
#90888=DIRECTION('',(-0.190809912898503,0.,0.981627005099017));
#90889=DIRECTION('center_axis',(0.,-1.,0.));
#90890=DIRECTION('ref_axis',(0.158019336155245,0.,0.987436017877136));
#90891=DIRECTION('',(-0.190809912898503,0.,0.981627005099017));
#90892=DIRECTION('center_axis',(0.,-1.,0.));
#90893=DIRECTION('ref_axis',(0.149316167640555,0.,0.988789503423827));
#90894=DIRECTION('center_axis',(0.981627005099017,0.,0.190809912898503));
#90895=DIRECTION('ref_axis',(0.,-1.,0.));
#90896=DIRECTION('',(-0.190809912898493,0.,0.981627005099019));
#90897=DIRECTION('',(0.,1.,0.));
#90898=DIRECTION('center_axis',(0.981627005099017,2.45653454077401E-16,
0.190809912898504));
#90899=DIRECTION('ref_axis',(-0.165310900973356,0.499412515026929,0.850446615522606));
#90900=DIRECTION('center_axis',(0.981627005099017,1.72689897470369E-16,
0.190809912898504));
#90901=DIRECTION('ref_axis',(-0.163919320156954,0.511855936218513,0.843287588570561));
#90902=DIRECTION('center_axis',(0.,1.,0.));
#90903=DIRECTION('ref_axis',(1.,0.,0.));
#90904=DIRECTION('',(-0.190809912898503,0.,0.981627005099017));
#90905=DIRECTION('',(-0.981627005099017,0.,-0.190809912898503));
#90906=DIRECTION('center_axis',(0.,1.,0.));
#90907=DIRECTION('ref_axis',(0.118119757483604,0.,0.992999356944411));
#90908=DIRECTION('center_axis',(-0.981627005099017,0.,-0.190809912898503));
#90909=DIRECTION('ref_axis',(-0.190809912898503,0.,0.981627005099017));
#90910=DIRECTION('center_axis',(-0.981627005099017,3.04906463307191E-16,
-0.190809912898503));
#90911=DIRECTION('ref_axis',(-0.166981814435774,0.483903660262205,0.85904267718931));
#90912=DIRECTION('',(1.82418708658322E-14,-1.,3.54587819297421E-15));
#90913=DIRECTION('center_axis',(-0.981627005099017,-7.69816334883557E-17,
-0.190809912898503));
#90914=DIRECTION('ref_axis',(-0.168014818177704,0.473981020103497,0.864356994218455));
#90915=DIRECTION('center_axis',(-0.190809912898503,0.,0.981627005099017));
#90916=DIRECTION('ref_axis',(0.,1.,0.));
#90917=DIRECTION('center_axis',(0.190809912898503,3.96319586197532E-16,
-0.981627005099017));
#90918=DIRECTION('ref_axis',(0.472312009925091,0.876637065109843,0.091808612646749));
#90919=DIRECTION('center_axis',(-0.981627005099017,0.,-0.190809912898503));
#90920=DIRECTION('ref_axis',(-0.190809912898503,0.,0.981627005099017));
#90921=DIRECTION('',(-0.190809912898503,0.,0.981627005099017));
#90922=DIRECTION('center_axis',(-0.981627005099017,-1.8030757312937E-16,
-0.190809912898504));
#90923=DIRECTION('ref_axis',(-0.181596654085648,0.306983029510506,0.934229134001637));
#90924=DIRECTION('',(-0.190809912898503,0.,0.981627005099017));
#90925=DIRECTION('center_axis',(-0.981627005099017,9.94141557488341E-17,
-0.190809912898503));
#90926=DIRECTION('ref_axis',(-0.182046275027808,0.299579406426393,0.936542221682349));
#90927=DIRECTION('center_axis',(0.,-1.,0.));
#90928=DIRECTION('ref_axis',(0.,0.,-1.));
#90929=DIRECTION('',(-0.190809912898493,0.,0.981627005099019));
#90930=DIRECTION('',(0.981627005099017,-1.858330177458E-14,0.190809912898503));
#90931=DIRECTION('center_axis',(0.,-1.,0.));
#90932=DIRECTION('ref_axis',(0.341205688802883,0.,0.939988658404212));
#90933=DIRECTION('center_axis',(0.,-1.,0.));
#90934=DIRECTION('ref_axis',(0.33310368336774,0.,0.942890203643481));
#90935=DIRECTION('center_axis',(0.981627005099017,0.,0.190809912898503));
#90936=DIRECTION('ref_axis',(0.,-1.,0.));
#90937=DIRECTION('',(-0.190809912898487,0.,0.98162700509902));
#90938=DIRECTION('',(0.,1.,0.));
#90939=DIRECTION('center_axis',(0.981627005099017,-1.87874135277778E-16,
0.190809912898503));
#90940=DIRECTION('ref_axis',(-0.179319086707495,0.341783624658495,0.922512124070839));
#90941=DIRECTION('center_axis',(0.,1.,0.));
#90942=DIRECTION('ref_axis',(1.,0.,0.));
#90943=DIRECTION('center_axis',(0.,1.,0.));
#90944=DIRECTION('ref_axis',(0.313402836107741,0.,0.949620272698316));
#90945=DIRECTION('',(-0.981627005099017,0.,-0.190809912898503));
#90946=DIRECTION('center_axis',(0.,1.,0.));
#90947=DIRECTION('ref_axis',(0.302289399785084,0.,0.953216197290821));
#90948=DIRECTION('center_axis',(-0.190809912898503,0.,0.981627005099017));
#90949=DIRECTION('ref_axis',(0.,1.,0.));
#90950=DIRECTION('center_axis',(0.190809912898503,0.,-0.981627005099017));
#90951=DIRECTION('ref_axis',(0.827186458119361,0.538432243009611,0.160789561824102));
#90952=DIRECTION('center_axis',(0.,-1.,0.));
#90953=DIRECTION('ref_axis',(0.,0.,-1.));
#90954=DIRECTION('',(-0.190809912898493,0.,0.981627005099019));
#90955=DIRECTION('center_axis',(0.,-1.,0.));
#90956=DIRECTION('ref_axis',(0.335481893758792,0.,0.942046654343624));
#90957=DIRECTION('',(-0.190809912898503,0.,0.981627005099017));
#90958=DIRECTION('center_axis',(0.,-1.,0.));
#90959=DIRECTION('ref_axis',(0.324430753252009,0.,0.945909449336634));
#90960=DIRECTION('center_axis',(0.981627005099017,0.,0.190809912898503));
#90961=DIRECTION('ref_axis',(0.,-1.,0.));
#90962=DIRECTION('',(-0.190809912898503,0.,0.981627005099017));
#90963=DIRECTION('center_axis',(0.981627005099017,1.97664555486468E-16,
0.190809912898504));
#90964=DIRECTION('ref_axis',(-0.183399207679054,0.275985344180091,0.943502422053326));
#90965=DIRECTION('center_axis',(0.981627005099017,1.87874135277778E-17,
0.190809912898503));
#90966=DIRECTION('ref_axis',(-0.183773297839977,0.2690637045184,0.945426939489168));
#90967=DIRECTION('center_axis',(0.,1.,0.));
#90968=DIRECTION('ref_axis',(1.,0.,0.));
#90969=DIRECTION('',(-0.190809912898503,0.,0.981627005099017));
#90970=DIRECTION('center_axis',(0.,1.,0.));
#90971=DIRECTION('ref_axis',(0.303402411978182,0.,0.952862517053652));
#90972=DIRECTION('center_axis',(0.,1.,0.));
#90973=DIRECTION('ref_axis',(0.292916715383648,0.,0.956137959631796));
#90974=DIRECTION('center_axis',(-0.981627005099017,0.,-0.190809912898503));
#90975=DIRECTION('ref_axis',(-0.190809912898503,0.,0.981627005099017));
#90976=DIRECTION('center_axis',(-0.981627005099017,-1.56582892454453E-16,
-0.190809912898504));
#90977=DIRECTION('ref_axis',(-0.185517346687496,0.233891832008005,0.954399248217417));
#90978=DIRECTION('center_axis',(-0.981627005099017,7.23012041809702E-17,
-0.190809912898503));
#90979=DIRECTION('ref_axis',(-0.185772975278006,0.228250976324805,0.955714336746672));
#90980=DIRECTION('center_axis',(0.,-1.,0.));
#90981=DIRECTION('ref_axis',(0.,0.,-1.));
#90982=DIRECTION('',(-0.190809912898503,0.,0.981627005099017));
#90983=DIRECTION('center_axis',(0.,-1.,0.));
#90984=DIRECTION('ref_axis',(0.329025837701854,0.,0.944320919033669));
#90985=DIRECTION('',(-0.190809912898503,0.,0.981627005099017));
#90986=DIRECTION('center_axis',(0.,-1.,0.));
#90987=DIRECTION('ref_axis',(0.318363930413136,0.,0.947968568999996));
#90988=DIRECTION('center_axis',(0.981627005099017,0.,0.190809912898503));
#90989=DIRECTION('ref_axis',(0.,-1.,0.));
#90990=DIRECTION('',(-0.190809912898503,0.,0.981627005099017));
#90991=DIRECTION('center_axis',(0.981627005099017,1.23540347179043E-16,
0.190809912898504));
#90992=DIRECTION('ref_axis',(-0.186900249967823,0.201394710617895,0.961513633339174));
#90993=DIRECTION('center_axis',(0.981627005099017,1.17421334548611E-16,
0.190809912898504));
#90994=DIRECTION('ref_axis',(-0.187095820528074,0.196343784378293,0.962519751629512));
#90995=DIRECTION('center_axis',(0.,1.,0.));
#90996=DIRECTION('ref_axis',(1.,0.,0.));
#90997=DIRECTION('',(-0.190809912898503,0.,0.981627005099017));
#90998=DIRECTION('center_axis',(0.,1.,0.));
#90999=DIRECTION('ref_axis',(0.296165820896561,0.,0.955136538162302));
#91000=DIRECTION('center_axis',(0.,1.,0.));
#91001=DIRECTION('ref_axis',(0.286119870298458,0.,0.958193832071775));
#91002=DIRECTION('center_axis',(-0.981627005099017,0.,-0.190809912898503));
#91003=DIRECTION('ref_axis',(-0.190809912898503,0.,0.981627005099017));
#91004=DIRECTION('center_axis',(-0.981627005099017,4.27044252148508E-17,
-0.190809912898503));
#91005=DIRECTION('ref_axis',(-0.188326885887437,0.160800634505503,0.968853002263278));
#91006=DIRECTION('center_axis',(-0.981627005099017,3.16317768291745E-17,
-0.190809912898503));
#91007=DIRECTION('ref_axis',(-0.188445952191515,0.156922546223307,0.969465542239345));
#91008=DIRECTION('center_axis',(0.,-1.,0.));
#91009=DIRECTION('ref_axis',(0.,0.,-1.));
#91010=DIRECTION('',(-0.190809912898503,0.,0.981627005099017));
#91011=DIRECTION('center_axis',(0.,-1.,0.));
#91012=DIRECTION('ref_axis',(0.325079416156572,0.,0.945686720426644));
#91013=DIRECTION('',(-0.190809912898503,0.,0.981627005099017));
#91014=DIRECTION('center_axis',(0.,-1.,0.));
#91015=DIRECTION('ref_axis',(0.314651032875617,0.,0.949207420699136));
#91016=DIRECTION('center_axis',(0.981627005099017,0.,0.190809912898503));
#91017=DIRECTION('ref_axis',(0.,-1.,0.));
#91018=DIRECTION('',(-0.190809912898513,0.,0.981627005099015));
#91019=DIRECTION('center_axis',(0.981627005099017,5.43577527587787E-17,
0.190809912898504));
#91020=DIRECTION('ref_axis',(-0.189269653813775,0.126804077055707,0.973703098581525));
#91021=DIRECTION('center_axis',(0.981627005099017,7.98465074930554E-17,
0.190809912898504));
#91022=DIRECTION('ref_axis',(-0.189346238510002,0.123623864238198,0.974097090721931));
#91023=DIRECTION('center_axis',(0.,1.,0.));
#91024=DIRECTION('ref_axis',(1.,0.,0.));
#91025=DIRECTION('',(-0.190809912898503,0.,0.981627005099017));
#91026=DIRECTION('center_axis',(0.,1.,0.));
#91027=DIRECTION('ref_axis',(0.291369117343108,0.,0.956610703190539));
#91028=DIRECTION('center_axis',(0.,1.,0.));
#91029=DIRECTION('ref_axis',(0.281608014703448,0.,0.95952953370638));
#91030=DIRECTION('center_axis',(-0.981627005099017,0.,-0.190809912898503));
#91031=DIRECTION('ref_axis',(-0.190809912898503,0.,0.981627005099017));
#91032=DIRECTION('center_axis',(-0.981627005099017,-5.45667655523093E-17,
-0.190809912898504));
#91033=DIRECTION('ref_axis',(-0.190074550777785,0.0877094370030095,0.977843913826352));
#91034=DIRECTION('center_axis',(-0.981627005099017,-7.68200294422809E-17,
-0.190809912898504));
#91035=DIRECTION('ref_axis',(-0.190109657599699,0.0855941161218201,0.978024521866732));
#91036=DIRECTION('center_axis',(0.,-1.,0.));
#91037=DIRECTION('ref_axis',(0.,0.,-1.));
#91038=DIRECTION('',(-0.190809912898503,0.,0.981627005099017));
#91039=DIRECTION('center_axis',(0.,-1.,0.));
#91040=DIRECTION('ref_axis',(0.323480044633156,0.,0.946234992337597));
#91041=DIRECTION('',(-0.190809912898503,0.,0.981627005099017));
#91042=DIRECTION('center_axis',(0.,-1.,0.));
#91043=DIRECTION('ref_axis',(0.313145356260713,0.,0.949705209974312));
#91044=DIRECTION('center_axis',(0.981627005099017,0.,0.190809912898503));
#91045=DIRECTION('ref_axis',(0.,-1.,0.));
#91046=DIRECTION('',(-0.190809912898503,0.,0.981627005099017));
#91047=DIRECTION('center_axis',(0.981627005099017,2.96496833229702E-17,
0.190809912898504));
#91048=DIRECTION('ref_axis',(-0.190549638224689,0.0522134434935414,0.980288014662521));
#91049=DIRECTION('center_axis',(0.981627005099017,4.22716804374999E-17,
0.190809912898504));
#91050=DIRECTION('ref_axis',(-0.190562538121797,0.0509039440980811,0.980354378548817));
#91051=DIRECTION('center_axis',(0.,1.,0.));
#91052=DIRECTION('ref_axis',(1.,0.,0.));
#91053=DIRECTION('',(-0.190809912898503,0.,0.981627005099017));
#91054=DIRECTION('center_axis',(0.,1.,0.));
#91055=DIRECTION('ref_axis',(0.288811078038997,0.,0.957386108736675));
#91056=DIRECTION('center_axis',(0.,1.,0.));
#91057=DIRECTION('ref_axis',(0.27919973712564,0.,0.960233048165378));
#91058=DIRECTION('center_axis',(-0.981627005099017,0.,-0.190809912898503));
#91059=DIRECTION('ref_axis',(-0.190809912898503,0.,0.981627005099017));
#91060=DIRECTION('center_axis',(-0.981627005099017,-8.89675525309391E-18,
-0.190809912898504));
#91061=DIRECTION('ref_axis',(-0.190789524444921,0.0146182395004994,0.981522116121683));
#91062=DIRECTION('center_axis',(-0.981627005099017,-1.35564757839319E-17,
-0.190809912898504));
#91063=DIRECTION('ref_axis',(-0.190790496067195,0.0142656860203004,0.98152711466001));
#91064=DIRECTION('center_axis',(0.,-1.,0.));
#91065=DIRECTION('ref_axis',(0.,0.,-1.));
#91066=DIRECTION('',(-0.190809912898503,0.,0.981627005099017));
#91067=DIRECTION('center_axis',(0.,-1.,0.));
#91068=DIRECTION('ref_axis',(-0.51578631619443,0.,0.856717267262998));
#91069=DIRECTION('',(-0.190809912898503,0.,0.981627005099017));
#91070=DIRECTION('center_axis',(0.,-1.,0.));
#91071=DIRECTION('ref_axis',(-0.509828849403992,0.,0.860275853616386));
#91072=DIRECTION('center_axis',(0.981627005099017,0.,0.190809912898503));
#91073=DIRECTION('ref_axis',(0.,-1.,0.));
#91074=DIRECTION('',(-0.190809912898503,0.,0.981627005099017));
#91075=DIRECTION('center_axis',(0.981627005099017,4.73701931306098E-17,
0.190809912898504));
#91076=DIRECTION('ref_axis',(-0.190588158690433,0.0481974707091998,0.980486184290338));
#91077=DIRECTION('center_axis',(0.981627005099017,1.61266538800991E-17,
0.190809912898504));
#91078=DIRECTION('ref_axis',(-0.19059759198742,0.047161767008978,0.980534714154062));
#91079=DIRECTION('center_axis',(0.,1.,0.));
#91080=DIRECTION('ref_axis',(1.,0.,0.));
#91081=DIRECTION('',(-0.190809912898503,0.,0.981627005099017));
#91082=DIRECTION('center_axis',(0.,1.,0.));
#91083=DIRECTION('ref_axis',(-0.54548104653432,0.,0.838123157937915));
#91084=DIRECTION('center_axis',(0.,1.,0.));
#91085=DIRECTION('ref_axis',(-0.538997674779873,0.,0.842307251887273));
#91086=DIRECTION('center_axis',(-0.981627005099017,0.,-0.190809912898503));
#91087=DIRECTION('ref_axis',(-0.190809912898503,0.,0.981627005099017));
#91088=DIRECTION('center_axis',(-0.981627005099017,-1.45950760997372E-17,
-0.190809912898504));
#91089=DIRECTION('ref_axis',(-0.190791331241222,0.0139555250478298,0.981531411236463));
#91090=DIRECTION('center_axis',(-0.981627005099017,-5.16982180453677E-18,
-0.190809912898504));
#91091=DIRECTION('ref_axis',(-0.190792141709014,0.0136478005707896,0.981535580710994));
#91092=DIRECTION('center_axis',(0.,-1.,0.));
#91093=DIRECTION('ref_axis',(0.,0.,-1.));
#91094=DIRECTION('',(-0.190809912898503,0.,0.981627005099017));
#91095=DIRECTION('center_axis',(0.,-1.,0.));
#91096=DIRECTION('ref_axis',(-0.516706060412873,0.,0.856162862504914));
#91097=DIRECTION('',(-0.190809912898503,0.,0.981627005099017));
#91098=DIRECTION('center_axis',(0.,-1.,0.));
#91099=DIRECTION('ref_axis',(-0.510698343921526,0.,0.85975996738381));
#91100=DIRECTION('center_axis',(0.981627005099017,0.,0.190809912898503));
#91101=DIRECTION('ref_axis',(0.,-1.,0.));
#91102=DIRECTION('',(-0.190809912898503,0.,0.981627005099017));
#91103=DIRECTION('center_axis',(0.981627005099017,8.84243605104716E-17,
0.190809912898504));
#91104=DIRECTION('ref_axis',(-0.18949826744453,0.117051000293799,0.974879207884619));
#91105=DIRECTION('center_axis',(0.981627005099017,5.24116251103221E-17,
0.190809912898504));
#91106=DIRECTION('ref_axis',(-0.189554217765144,0.114535719878902,0.975167045894838));
#91107=DIRECTION('center_axis',(0.,1.,0.));
#91108=DIRECTION('ref_axis',(1.,0.,0.));
#91109=DIRECTION('',(-0.190809912898503,0.,0.981627005099017));
#91110=DIRECTION('center_axis',(0.,1.,0.));
#91111=DIRECTION('ref_axis',(-0.547202057128739,0.,0.837000542815879));
#91112=DIRECTION('center_axis',(0.,1.,0.));
#91113=DIRECTION('ref_axis',(-0.540624705795703,0.,0.841263886948269));
#91114=DIRECTION('center_axis',(-0.981627005099017,0.,-0.190809912898503));
#91115=DIRECTION('ref_axis',(-0.190809912898503,0.,0.981627005099017));
#91116=DIRECTION('center_axis',(-0.981627005099017,-3.67579694363753E-17,
-0.190809912898504));
#91117=DIRECTION('ref_axis',(-0.190139829212612,0.0837331502869717,0.97817974058453));
#91118=DIRECTION('center_axis',(-0.981627005099017,-2.06792872181471E-18,
-0.190809912898503));
#91119=DIRECTION('ref_axis',(-0.190169103834306,0.081886803424733,0.978330344705578));
#91120=DIRECTION('center_axis',(0.,-1.,0.));
#91121=DIRECTION('ref_axis',(0.,0.,-1.));
#91122=DIRECTION('',(-0.190809912898503,0.,0.981627005099017));
#91123=DIRECTION('center_axis',(0.,-1.,0.));
#91124=DIRECTION('ref_axis',(-0.518972960090495,0.,0.854790656649281));
#91125=DIRECTION('',(-0.190809912898503,0.,0.981627005099017));
#91126=DIRECTION('center_axis',(0.,-1.,0.));
#91127=DIRECTION('ref_axis',(-0.512840213950635,0.,0.858484079616545));
#91128=DIRECTION('center_axis',(0.981627005099017,0.,0.190809912898503));
#91129=DIRECTION('ref_axis',(0.,-1.,0.));
#91130=DIRECTION('',(-0.190809912898493,0.,0.981627005099019));
#91131=DIRECTION('center_axis',(0.981627005099017,1.34741882682623E-16,
0.190809912898504));
#91132=DIRECTION('ref_axis',(-0.187483678682097,0.185904529878394,0.964515098896083));
#91133=DIRECTION('center_axis',(0.981627005099017,4.03166347002478E-17,
0.190809912898503));
#91134=DIRECTION('ref_axis',(-0.187626296241583,0.181909672748906,0.965248798973121));
#91135=DIRECTION('center_axis',(0.,1.,0.));
#91136=DIRECTION('ref_axis',(1.,0.,0.));
#91137=DIRECTION('',(-0.190809912898503,0.,0.981627005099017));
#91138=DIRECTION('center_axis',(0.,1.,0.));
#91139=DIRECTION('ref_axis',(-0.550424059915763,0.,0.834885234188417));
#91140=DIRECTION('center_axis',(0.,1.,0.));
#91141=DIRECTION('ref_axis',(-0.543668385334357,0.,0.839300117233361));
#91142=DIRECTION('center_axis',(-0.981627005099017,0.,-0.190809912898503));
#91143=DIRECTION('ref_axis',(-0.190809912898503,0.,0.981627005099017));
#91144=DIRECTION('center_axis',(-0.981627005099017,-5.18936039101769E-17,
-0.190809912898504));
#91145=DIRECTION('ref_axis',(-0.188548237998538,0.153510775526106,0.969991754472696));
#91146=DIRECTION('center_axis',(-0.981627005099017,-1.61298440301547E-16,
-0.190809912898504));
#91147=DIRECTION('ref_axis',(-0.188647445377018,0.150125806278706,0.970502129643152));
#91148=DIRECTION('center_axis',(0.,-1.,0.));
#91149=DIRECTION('ref_axis',(0.,0.,-1.));
#91150=DIRECTION('',(-0.190809912898503,0.,0.981627005099017));
#91151=DIRECTION('center_axis',(0.,-1.,0.));
#91152=DIRECTION('ref_axis',(-0.522673585683894,0.,0.85253288665502));
#91153=DIRECTION('',(-0.190809912898503,0.,0.981627005099017));
#91154=DIRECTION('center_axis',(0.,-1.,0.));
#91155=DIRECTION('ref_axis',(-0.516333108288111,0.,0.856387833452541));
#91156=DIRECTION('center_axis',(0.981627005099017,0.,0.190809912898503));
#91157=DIRECTION('ref_axis',(0.,-1.,0.));
#91158=DIRECTION('',(-0.190809912898503,0.,0.981627005099017));
#91159=DIRECTION('center_axis',(0.981627005099017,2.18955559359263E-16,
0.190809912898504));
#91160=DIRECTION('ref_axis',(-0.184514106387807,0.254758059462899,0.949238050060472));
#91161=DIRECTION('center_axis',(0.981627005099017,1.20949904100743E-16,
0.190809912898504));
#91162=DIRECTION('ref_axis',(-0.184786143359668,0.249283625618896,0.950637551972653));
#91163=DIRECTION('center_axis',(0.,1.,0.));
#91164=DIRECTION('ref_axis',(1.,0.,0.));
#91165=DIRECTION('',(-0.190809912898514,0.,0.981627005099015));
#91166=DIRECTION('center_axis',(0.,1.,0.));
#91167=DIRECTION('ref_axis',(-0.555272217382648,0.,0.831668662751553));
#91168=DIRECTION('center_axis',(0.,1.,0.));
#91169=DIRECTION('ref_axis',(-0.548242331478566,0.,0.836319523851348));
#91170=DIRECTION('center_axis',(-0.981627005099017,0.,-0.190809912898503));
#91171=DIRECTION('ref_axis',(-0.190809912898503,0.,0.981627005099017));
#91172=DIRECTION('center_axis',(-0.981627005099017,-5.18936039101769E-17,
-0.190809912898504));
#91173=DIRECTION('ref_axis',(-0.185992425315799,0.223288400765293,0.956843303686045));
#91174=DIRECTION('center_axis',(-0.981627005099017,-8.27171488725884E-17,
-0.190809912898504));
#91175=DIRECTION('ref_axis',(-0.186205137201712,0.218364809132596,0.957937606012091));
#91176=DIRECTION('center_axis',(0.,-1.,0.));
#91177=DIRECTION('ref_axis',(0.,0.,-1.));
#91178=DIRECTION('',(-0.190809912898503,0.,0.981627005099017));
#91179=DIRECTION('center_axis',(0.,-1.,0.));
#91180=DIRECTION('ref_axis',(-0.527956416002256,0.,0.849271465905957));
#91181=DIRECTION('',(-0.190809912898503,0.,0.981627005099017));
#91182=DIRECTION('center_axis',(0.,-1.,0.));
#91183=DIRECTION('ref_axis',(-0.521311526714744,0.,0.853366446559942));
#91184=DIRECTION('center_axis',(0.981627005099017,0.,0.190809912898503));
#91185=DIRECTION('ref_axis',(0.,-1.,0.));
#91186=DIRECTION('',(-0.190809912898503,0.,0.981627005099017));
#91187=DIRECTION('center_axis',(0.981627005099017,7.57923090089757E-17,
0.190809912898503));
#91188=DIRECTION('ref_axis',(-0.180542433838233,0.323611589047495,0.928805668058675));
#91189=DIRECTION('center_axis',(0.981627005099017,1.93519846561189E-16,
0.190809912898504));
#91190=DIRECTION('ref_axis',(-0.180990819330081,0.316657578488792,0.931112399930234));
#91191=DIRECTION('center_axis',(0.,1.,0.));
#91192=DIRECTION('ref_axis',(1.,0.,0.));
#91193=DIRECTION('',(-0.190809912898503,0.,0.981627005099017));
#91194=DIRECTION('center_axis',(0.,1.,0.));
#91195=DIRECTION('ref_axis',(-0.561946648451831,0.,0.827173478959374));
#91196=DIRECTION('center_axis',(0.,1.,0.));
#91197=DIRECTION('ref_axis',(-0.554527554446219,0.,0.83216536298977));
#91198=DIRECTION('center_axis',(-0.981627005099017,0.,-0.190809912898503));
#91199=DIRECTION('ref_axis',(-0.190809912898503,0.,0.981627005099017));
#91200=DIRECTION('center_axis',(-0.981627005099017,1.29734009775442E-16,
-0.190809912898503));
#91201=DIRECTION('ref_axis',(-0.182431870353022,0.293066026004411,0.938525927761977));
#91202=DIRECTION('center_axis',(-0.981627005099017,-4.13585744362942E-17,
-0.190809912898503));
#91203=DIRECTION('ref_axis',(-0.18280528294402,0.286603811986498,0.940446959420128));
#91204=DIRECTION('center_axis',(0.,-1.,0.));
#91205=DIRECTION('ref_axis',(0.,0.,-1.));
#91206=DIRECTION('',(-0.190809912898503,0.,0.981627005099017));
#91207=DIRECTION('center_axis',(0.,-1.,0.));
#91208=DIRECTION('ref_axis',(-0.53504944924277,0.,0.844820742444815));
#91209=DIRECTION('',(-0.190809912898503,0.,0.981627005099017));
#91210=DIRECTION('center_axis',(0.,-1.,0.));
#91211=DIRECTION('ref_axis',(-0.52798109669905,0.,0.849256122455687));
#91212=DIRECTION('center_axis',(0.981627005099017,0.,0.190809912898503));
#91213=DIRECTION('ref_axis',(0.,-1.,0.));
#91214=DIRECTION('',(-0.190809912898503,0.,0.981627005099017));
#91215=DIRECTION('center_axis',(0.981627005099017,1.26320515014959E-16,
0.190809912898504));
#91216=DIRECTION('ref_axis',(-0.175500640034728,0.392465118632079,0.902868016935205));
#91217=DIRECTION('center_axis',(0.981627005099017,-8.06332694004955E-17,
0.190809912898503));
#91218=DIRECTION('ref_axis',(-0.176178604698278,0.38403153135881,0.906355825362631));
#91219=DIRECTION('center_axis',(0.,1.,0.));
#91220=DIRECTION('ref_axis',(1.,0.,0.));
#91221=DIRECTION('',(-0.190809912898503,0.,0.981627005099017));
#91222=DIRECTION('center_axis',(0.,1.,0.));
#91223=DIRECTION('ref_axis',(-0.570747207818219,0.,0.821125827609695));
#91224=DIRECTION('center_axis',(0.,1.,0.));
#91225=DIRECTION('ref_axis',(-0.562793888599892,0.,0.826597265271676));
#91226=DIRECTION('center_axis',(-0.981627005099017,0.,-0.190809912898503));
#91227=DIRECTION('ref_axis',(-0.190809912898503,0.,0.981627005099017));
#91228=DIRECTION('center_axis',(-0.981627005099017,-1.5568081173053E-16,
-0.190809912898504));
#91229=DIRECTION('ref_axis',(-0.177806223707996,0.362843651243595,0.914729157490302));
#91230=DIRECTION('center_axis',(-0.981627005099017,3.30868595490354E-17,
-0.190809912898503));
#91231=DIRECTION('ref_axis',(-0.178393143654898,0.3548428148405,0.917748583792421));
#91232=DIRECTION('center_axis',(-0.190809912898503,0.,0.981627005099017));
#91233=DIRECTION('ref_axis',(0.,1.,0.));
#91234=DIRECTION('',(-0.981627005099017,0.,-0.190809912898503));
#91235=DIRECTION('',(0.,-1.,0.));
#91236=DIRECTION('center_axis',(0.190809912898504,-4.66258336702978E-16,
-0.981627005099017));
#91237=DIRECTION('ref_axis',(-0.652240394658444,0.747334233647181,-0.12678332222646));
#91238=DIRECTION('center_axis',(0.,-1.,0.));
#91239=DIRECTION('ref_axis',(0.,0.,-1.));
#91240=DIRECTION('',(-0.190809912898503,0.,0.981627005099017));
#91241=DIRECTION('center_axis',(0.,-1.,0.));
#91242=DIRECTION('ref_axis',(-0.544290275892155,0.,0.838896951698623));
#91243=DIRECTION('',(-0.190809912898503,0.,0.981627005099017));
#91244=DIRECTION('center_axis',(0.,-1.,0.));
#91245=DIRECTION('ref_axis',(-0.536644442339821,0.,0.843808475014196));
#91246=DIRECTION('center_axis',(0.981627005099017,0.,0.190809912898503));
#91247=DIRECTION('ref_axis',(0.,-1.,0.));
#91248=DIRECTION('',(-0.190809912898503,0.,0.981627005099017));
#91249=DIRECTION('center_axis',(0.981627005099017,3.36854706706558E-17,
0.190809912898503));
#91250=DIRECTION('ref_axis',(-0.169293142699848,0.461318648216628,0.870933370954628));
#91251=DIRECTION('center_axis',(0.981627005099017,1.61266538800991E-16,
0.190809912898504));
#91252=DIRECTION('ref_axis',(-0.17026329901866,0.451405484228805,0.875924367634238));
#91253=DIRECTION('center_axis',(0.,1.,0.));
#91254=DIRECTION('ref_axis',(1.,0.,0.));
#91255=DIRECTION('',(-0.190809912898503,0.,0.981627005099017));
#91256=DIRECTION('center_axis',(0.,1.,0.));
#91257=DIRECTION('ref_axis',(-0.568943506648922,0.,0.822376608520712));
#91258=DIRECTION('center_axis',(0.,1.,0.));
#91259=DIRECTION('ref_axis',(-0.573435895591197,0.,0.819250434023395));
#91260=DIRECTION('center_axis',(-0.981627005099017,0.,-0.190809912898503));
#91261=DIRECTION('ref_axis',(-0.190809912898503,0.,0.981627005099017));
#91262=DIRECTION('center_axis',(-0.981627005099017,-7.78404058652653E-17,
-0.190809912898503));
#91263=DIRECTION('ref_axis',(-0.172029590132755,0.432621276482712,0.885011102333313));
#91264=DIRECTION('center_axis',(-0.981627005099017,-2.8951002105406E-16,
-0.190809912898504));
#91265=DIRECTION('ref_axis',(-0.172891236946279,0.423081817694416,0.889443868787443));
#91266=DIRECTION('center_axis',(0.,-1.,0.));
#91267=DIRECTION('ref_axis',(0.,0.,-1.));
#91268=DIRECTION('',(-0.190809912898503,1.036699112927E-14,0.981627005099017));
#91269=DIRECTION('center_axis',(0.,-1.,0.));
#91270=DIRECTION('ref_axis',(-0.479837164377971,0.,0.877357564326944));
#91271=DIRECTION('',(-0.190809912898503,0.,0.981627005099017));
#91272=DIRECTION('center_axis',(0.,-1.,0.));
#91273=DIRECTION('ref_axis',(-0.473524725918971,0.,0.880780525411049));
#91274=DIRECTION('center_axis',(0.981627005099017,0.,0.190809912898503));
#91275=DIRECTION('ref_axis',(0.,-1.,0.));
#91276=DIRECTION('',(-0.190809912898503,0.,0.981627005099017));
#91277=DIRECTION('center_axis',(0.981627005099017,3.86629460097736E-16,
0.190809912898504));
#91278=DIRECTION('ref_axis',(-0.170286389349438,0.451166192838008,0.87604315649538));
#91279=DIRECTION('center_axis',(0.981627005099017,-2.31798761009061E-16,
0.190809912898503));
#91280=DIRECTION('ref_axis',(-0.17117061747492,0.44188028378381,0.880592093148919));
#91281=DIRECTION('center_axis',(0.,1.,0.));
#91282=DIRECTION('ref_axis',(1.,0.,0.));
#91283=DIRECTION('',(-0.190809912898503,0.,0.981627005099017));
#91284=DIRECTION('center_axis',(0.,1.,0.));
#91285=DIRECTION('ref_axis',(-0.517300722376421,0.,0.855803693979427));
#91286=DIRECTION('center_axis',(0.,1.,0.));
#91287=DIRECTION('ref_axis',(-0.509981045434312,0.,0.860185638858105));
#91288=DIRECTION('center_axis',(-0.981627005099017,0.,-0.190809912898503));
#91289=DIRECTION('ref_axis',(-0.190809912898503,0.,0.981627005099017));
#91290=DIRECTION('center_axis',(-0.981627005099017,1.64489301320048E-17,
-0.190809912898503));
#91291=DIRECTION('ref_axis',(-0.172998862914491,0.421871719792196,0.889997553631395));
#91292=DIRECTION('center_axis',(-0.981627005099017,0.,-0.190809912898503));
#91293=DIRECTION('ref_axis',(-0.173775507771522,0.413011554259003,0.893993025111109));
#91294=DIRECTION('center_axis',(0.,-1.,0.));
#91295=DIRECTION('ref_axis',(0.,0.,-1.));
#91296=DIRECTION('',(-0.190809912898503,0.,0.981627005099017));
#91297=DIRECTION('center_axis',(0.,-1.,0.));
#91298=DIRECTION('ref_axis',(-0.414281988925668,0.,0.910148577789249));
#91299=DIRECTION('',(-0.190809912898503,0.,0.981627005099017));
#91300=DIRECTION('center_axis',(0.,-1.,0.));
#91301=DIRECTION('ref_axis',(-0.409359365296299,0.,0.912373229574504));
#91302=DIRECTION('center_axis',(0.981627005099017,0.,0.190809912898503));
#91303=DIRECTION('ref_axis',(0.,-1.,0.));
#91304=DIRECTION('',(-0.190809912898503,0.,0.981627005099017));
#91305=DIRECTION('center_axis',(0.981627005099017,-9.34373521491282E-17,
0.190809912898503));
#91306=DIRECTION('ref_axis',(-0.171009768890973,0.443587536078797,0.879764603049814));
#91307=DIRECTION('center_axis',(0.981627005099017,1.94463727090204E-16,
0.190809912898504));
#91308=DIRECTION('ref_axis',(-0.171833841098054,0.434752737274877,0.884004065876108));
#91309=DIRECTION('center_axis',(0.,1.,0.));
#91310=DIRECTION('ref_axis',(1.,0.,0.));
#91311=DIRECTION('',(-0.190809912898503,0.,0.981627005099017));
#91312=DIRECTION('center_axis',(0.,1.,0.));
#91313=DIRECTION('ref_axis',(-0.451295175740691,0.,0.892374733143638));
#91314=DIRECTION('center_axis',(0.,1.,0.));
#91315=DIRECTION('ref_axis',(-0.445400813995018,0.,0.895331287788255));
#91316=DIRECTION('center_axis',(-0.981627005099017,0.,-0.190809912898503));
#91317=DIRECTION('ref_axis',(-0.190809912898503,0.,0.981627005099017));
#91318=DIRECTION('center_axis',(-0.981627005099017,-3.32200097218626E-16,
-0.190809912898504));
#91319=DIRECTION('ref_axis',(-0.173714529564319,0.413715522361311,0.893679320995823));
#91320=DIRECTION('center_axis',(-0.981627005099017,-1.67043077322241E-16,
-0.190809912898504));
#91321=DIRECTION('ref_axis',(-0.174431144456715,0.405349352773424,0.897365966621025));
#91322=DIRECTION('center_axis',(0.,-1.,0.));
#91323=DIRECTION('ref_axis',(0.,0.,-1.));
#91324=DIRECTION('',(-0.190809912898503,0.,0.981627005099017));
#91325=DIRECTION('center_axis',(0.,-1.,0.));
#91326=DIRECTION('ref_axis',(-0.347690702172142,0.,0.937609287295643));
#91327=DIRECTION('',(-0.190809912898503,0.,0.981627005099017));
#91328=DIRECTION('center_axis',(0.,-1.,0.));
#91329=DIRECTION('ref_axis',(-0.344208002633843,0.,0.938893418297743));
#91330=DIRECTION('center_axis',(0.981627005099017,0.,0.190809912898503));
#91331=DIRECTION('ref_axis',(0.,-1.,0.));
#91332=DIRECTION('',(-0.190809912898503,0.,0.981627005099017));
#91333=DIRECTION('center_axis',(0.981627005099017,-7.5998920345386E-17,
0.190809912898503));
#91334=DIRECTION('ref_axis',(-0.171510885743259,0.43824140554361,0.882342612899731));
#91335=DIRECTION('center_axis',(0.981627005099017,2.77669091834731E-16,
0.190809912898504));
#91336=DIRECTION('ref_axis',(-0.172294487675883,0.429716142106888,0.886373875252017));
#91337=DIRECTION('center_axis',(0.,1.,0.));
#91338=DIRECTION('ref_axis',(1.,0.,0.));
#91339=DIRECTION('',(-0.190809912898503,0.,0.981627005099017));
#91340=DIRECTION('center_axis',(0.,1.,0.));
#91341=DIRECTION('ref_axis',(-0.384183769154313,0.,0.923256644448544));
#91342=DIRECTION('center_axis',(0.,1.,0.));
#91343=DIRECTION('ref_axis',(-0.379771576195477,0.,0.9250802937659));
#91344=DIRECTION('center_axis',(-0.981627005099017,0.,-0.190809912898503));
#91345=DIRECTION('ref_axis',(-0.190809912898503,0.,0.981627005099017));
#91346=DIRECTION('center_axis',(-0.981627005099017,-3.53451119958106E-16,
-0.190809912898504));
#91347=DIRECTION('ref_axis',(-0.174225841498191,0.40776725581042,0.896309779731922));
#91348=DIRECTION('center_axis',(-0.981627005099017,-2.95381654173833E-17,
-0.190809912898503));
#91349=DIRECTION('ref_axis',(-0.174900994791868,0.399749884313687,0.899783124987354));
#91350=DIRECTION('center_axis',(0.,-1.,0.));
#91351=DIRECTION('ref_axis',(0.,0.,-1.));
#91352=DIRECTION('',(-0.190809912898503,0.,0.981627005099017));
#91353=DIRECTION('center_axis',(0.,-1.,0.));
#91354=DIRECTION('ref_axis',(-0.280107790543359,0.,0.959968554525052));
#91355=DIRECTION('',(-0.190809912898503,0.,0.981627005099017));
#91356=DIRECTION('center_axis',(0.,-1.,0.));
#91357=DIRECTION('ref_axis',(-0.278111038185117,0.,0.960548931829918));
#91358=DIRECTION('center_axis',(0.981627005099017,0.,0.190809912898503));
#91359=DIRECTION('ref_axis',(0.,-1.,0.));
#91360=DIRECTION('',(-0.190809912898503,0.,0.981627005099017));
#91361=DIRECTION('center_axis',(0.981627005099017,4.1913834659201E-16,0.190809912898504));
#91362=DIRECTION('ref_axis',(-0.171819814047587,0.434904980194897,0.883931903317404));
#91363=DIRECTION('center_axis',(0.981627005099017,7.20045220031795E-17,
0.190809912898503));
#91364=DIRECTION('ref_axis',(-0.172578958352769,0.426569286306185,0.887837342712113));
#91365=DIRECTION('center_axis',(0.,1.,0.));
#91366=DIRECTION('ref_axis',(1.,0.,0.));
#91367=DIRECTION('',(-0.190809912898503,0.,0.981627005099017));
#91368=DIRECTION('center_axis',(0.,1.,0.));
#91369=DIRECTION('ref_axis',(-0.31602509005927,0.,0.948750832649453));
#91370=DIRECTION('center_axis',(0.,1.,0.));
#91371=DIRECTION('ref_axis',(-0.313146253749265,0.,0.949704914045832));
#91372=DIRECTION('center_axis',(-0.981627005099017,0.,-0.190809912898503));
#91373=DIRECTION('ref_axis',(-0.190809912898503,0.,0.981627005099017));
#91374=DIRECTION('center_axis',(-0.981627005099017,-1.20541050910893E-16,
-0.190809912898504));
#91375=DIRECTION('ref_axis',(-0.174564455395936,0.403770028651194,0.898051788526327));
#91376=DIRECTION('center_axis',(-0.981627005099017,-5.79678245784151E-17,
-0.190809912898503));
#91377=DIRECTION('ref_axis',(-0.175212807608716,0.395981677383196,0.90138725486145));
#91378=DIRECTION('center_axis',(0.,-1.,0.));
#91379=DIRECTION('ref_axis',(0.,0.,-1.));
#91380=DIRECTION('',(-0.190809912898503,1.086578613169E-14,0.981627005099017));
#91381=DIRECTION('center_axis',(0.,-1.,0.));
#91382=DIRECTION('ref_axis',(-0.211560193439188,0.,0.977364969984076));
#91383=DIRECTION('',(-0.190809912898503,0.,0.981627005099017));
#91384=DIRECTION('center_axis',(0.,-1.,0.));
#91385=DIRECTION('ref_axis',(-0.211093004899912,0.,0.977465980626603));
#91386=DIRECTION('center_axis',(0.981627005099017,0.,0.190809912898503));
#91387=DIRECTION('ref_axis',(0.,-1.,0.));
#91388=DIRECTION('',(-0.190809912898503,0.,0.981627005099017));
#91389=DIRECTION('center_axis',(0.981627005099017,-1.4868986789408E-17,
0.190809912898503));
#91390=DIRECTION('ref_axis',(-0.171953954276685,0.433446386204417,0.884621991527988));
#91391=DIRECTION('center_axis',(0.981627005099017,0.,0.190809912898503));
#91392=DIRECTION('ref_axis',(-0.172702595687313,0.425192701759105,0.888473398483971));
#91393=DIRECTION('center_axis',(0.,1.,0.));
#91394=DIRECTION('ref_axis',(1.,0.,0.));
#91395=DIRECTION('',(-0.190809912898503,0.,0.981627005099017));
#91396=DIRECTION('center_axis',(0.,1.,0.));
#91397=DIRECTION('ref_axis',(-0.24685697062186,0.,0.969051926397857));
#91398=DIRECTION('center_axis',(0.,1.,0.));
#91399=DIRECTION('ref_axis',(-0.245559147376533,0.,0.969381609656233));
#91400=DIRECTION('center_axis',(-0.981627005099017,0.,-0.190809912898503));
#91401=DIRECTION('ref_axis',(-0.190809912898503,0.,0.981627005099017));
#91402=DIRECTION('center_axis',(-0.981627005099017,-1.04323047313055E-16,
-0.190809912898503));
#91403=DIRECTION('ref_axis',(-0.174749786833802,0.401562082356488,0.899005231361343));
#91404=DIRECTION('center_axis',(-0.981627005099017,-1.5773858633476E-16,
-0.190809912898504));
#91405=DIRECTION('ref_axis',(-0.175383692187236,0.393898398451778,0.902266375419087));
#91406=DIRECTION('center_axis',(0.,-1.,0.));
#91407=DIRECTION('ref_axis',(0.,0.,-1.));
#91408=DIRECTION('',(-0.190809912898503,0.,0.981627005099017));
#91409=DIRECTION('center_axis',(0.,-1.,0.));
#91410=DIRECTION('ref_axis',(-0.142059493577032,0.,0.989858121290439));
#91411=DIRECTION('',(-0.190809912898503,0.,0.981627005099017));
#91412=DIRECTION('center_axis',(0.,-1.,0.));
#91413=DIRECTION('ref_axis',(-0.14316446678366,0.,0.989698911513269));
#91414=DIRECTION('center_axis',(0.981627005099017,0.,0.190809912898503));
#91415=DIRECTION('ref_axis',(0.,-1.,0.));
#91416=DIRECTION('',(-0.190809912898503,0.,0.981627005099017));
#91417=DIRECTION('center_axis',(0.981627005099017,-8.93635241303609E-17,
0.190809912898503));
#91418=DIRECTION('ref_axis',(-0.171920597703966,0.433809658482487,0.884450387694199));
#91419=DIRECTION('center_axis',(0.981627005099017,2.86623894051663E-16,
0.190809912898504));
#91420=DIRECTION('ref_axis',(-0.172671844247454,0.425535598140786,0.888315196830014));
#91421=DIRECTION('center_axis',(0.,1.,0.));
#91422=DIRECTION('ref_axis',(1.,0.,0.));
#91423=DIRECTION('',(-0.190809912898503,0.,0.981627005099017));
#91424=DIRECTION('center_axis',(0.,1.,0.));
#91425=DIRECTION('ref_axis',(-0.176699795052451,0.,0.984264792842059));
#91426=DIRECTION('center_axis',(0.,1.,0.));
#91427=DIRECTION('ref_axis',(-0.177028780540981,0.,0.984205675080251));
#91428=DIRECTION('center_axis',(-0.981627005099017,0.,-0.190809912898503));
#91429=DIRECTION('ref_axis',(-0.190809912898503,0.,0.981627005099017));
#91430=DIRECTION('center_axis',(-0.981627005099017,0.,-0.190809912898503));
#91431=DIRECTION('ref_axis',(-0.174791955489963,0.401057680016923,0.899222169208165));
#91432=DIRECTION('center_axis',(-0.981627005099017,-8.58313634584417E-17,
-0.190809912898503));
#91433=DIRECTION('ref_axis',(-0.175422595692249,0.393422293643184,0.902466515603283));
#91434=DIRECTION('center_axis',(0.,-1.,0.));
#91435=DIRECTION('ref_axis',(0.,0.,-1.));
#91436=DIRECTION('',(-0.190809912898503,0.,0.981627005099017));
#91437=DIRECTION('center_axis',(0.,-1.,0.));
#91438=DIRECTION('ref_axis',(-0.0716028171606353,0.,0.997433224118116));
#91439=DIRECTION('',(-0.190809912898503,0.,0.981627005099017));
#91440=DIRECTION('center_axis',(0.,-1.,0.));
#91441=DIRECTION('ref_axis',(-0.0743228018941379,0.,0.99723423583359));
#91442=DIRECTION('center_axis',(0.981627005099017,0.,0.190809912898503));
#91443=DIRECTION('ref_axis',(0.,-1.,0.));
#91444=DIRECTION('',(-0.190809912898503,0.,0.981627005099017));
#91445=DIRECTION('center_axis',(0.981627005099017,3.00905960538911E-17,
0.190809912898503));
#91446=DIRECTION('ref_axis',(-0.171717946000204,0.436008640726291,0.883407840260365));
#91447=DIRECTION('center_axis',(0.981627005099017,2.6048332037516E-16,0.190809912898504));
#91448=DIRECTION('ref_axis',(-0.172485113654947,0.427610544193976,0.887354556004291));
#91449=DIRECTION('center_axis',(0.,1.,0.));
#91450=DIRECTION('ref_axis',(1.,0.,0.));
#91451=DIRECTION('',(-0.190809912898503,0.,0.981627005099017));
#91452=DIRECTION('center_axis',(0.,1.,0.));
#91453=DIRECTION('ref_axis',(-0.105558169770634,0.,0.994413129838235));
#91454=DIRECTION('center_axis',(0.,1.,0.));
#91455=DIRECTION('ref_axis',(-0.107559343282833,0.,0.994198666098766));
#91456=DIRECTION('center_axis',(-0.981627005099017,0.,-0.190809912898503));
#91457=DIRECTION('ref_axis',(-0.190809912898503,0.,0.981627005099017));
#91458=DIRECTION('center_axis',(-0.981627005099017,-2.09348652609932E-16,
-0.190809912898504));
#91459=DIRECTION('ref_axis',(-0.174693214665051,0.402237588782009,0.898714194235757));
#91460=DIRECTION('center_axis',(-0.981627005099017,-1.00704279750265E-16,
-0.190809912898503));
#91461=DIRECTION('ref_axis',(-0.17533151323336,0.394535901971296,0.901997939311946));
#91462=DIRECTION('center_axis',(0.,-1.,0.));
#91463=DIRECTION('ref_axis',(0.,0.,-1.));
#91464=DIRECTION('',(-0.190809912898503,0.,0.981627005099017));
#91465=DIRECTION('center_axis',(0.,-1.,0.));
#91466=DIRECTION('ref_axis',(-0.000172612850318695,0.,0.999999985102402));
#91467=DIRECTION('',(-0.190809912898503,-1.073924094398E-14,0.981627005099017));
#91468=DIRECTION('center_axis',(0.,-1.,0.));
#91469=DIRECTION('ref_axis',(-0.00455200992318091,0.,0.99998963954916));
#91470=DIRECTION('center_axis',(0.981627005099017,0.,0.190809912898503));
#91471=DIRECTION('ref_axis',(0.,-1.,0.));
#91472=DIRECTION('',(-0.190809912898503,0.,0.981627005099017));
#91473=DIRECTION('center_axis',(0.981627005099017,-7.66548341238665E-17,
0.190809912898503));
#91474=DIRECTION('ref_axis',(-0.171334862813509,0.440128478582875,0.881437057948552));
#91475=DIRECTION('center_axis',(0.981627005099017,1.76824696986466E-16,
0.190809912898504));
#91476=DIRECTION('ref_axis',(-0.172132568081392,0.431494770724981,0.885540875308814));
#91477=DIRECTION('center_axis',(0.,1.,0.));
#91478=DIRECTION('ref_axis',(1.,0.,0.));
#91479=DIRECTION('',(-0.190809912898503,0.,0.981627005099017));
#91480=DIRECTION('center_axis',(0.,1.,0.));
#91481=DIRECTION('ref_axis',(-0.0334212901421124,0.,0.999441352639182));
#91482=DIRECTION('center_axis',(0.,1.,0.));
#91483=DIRECTION('ref_axis',(-0.0371410100073943,0.,0.999310034661731));
#91484=DIRECTION('center_axis',(-0.981627005099017,0.,-0.190809912898503));
#91485=DIRECTION('ref_axis',(-0.190809912898503,0.,0.981627005099017));
#91486=DIRECTION('center_axis',(-0.981627005099017,-1.66876344160806E-16,
-0.190809912898504));
#91487=DIRECTION('ref_axis',(-0.174448259539567,0.405147003614198,0.897454015649856));
#91488=DIRECTION('center_axis',(-0.981627005099017,5.83486426445023E-17,
-0.190809912898503));
#91489=DIRECTION('ref_axis',(-0.175105749529825,0.397280243645616,0.900836491540212));
#91490=DIRECTION('center_axis',(0.,-1.,0.));
#91491=DIRECTION('ref_axis',(0.,0.,-1.));
#91492=DIRECTION('',(-0.190809912898503,-1.312424708425E-14,0.981627005099017));
#91493=DIRECTION('center_axis',(0.,-1.,0.));
#91494=DIRECTION('ref_axis',(0.0722647313333386,0.,0.99738548646214));
#91495=DIRECTION('',(-0.190809912898503,0.,0.981627005099017));
#91496=DIRECTION('center_axis',(0.,-1.,0.));
#91497=DIRECTION('ref_axis',(0.0661784895354501,0.,0.997807800892941));
#91498=DIRECTION('center_axis',(0.981627005099017,0.,0.190809912898503));
#91499=DIRECTION('ref_axis',(0.,-1.,0.));
#91500=DIRECTION('',(-0.190809912898503,0.,0.981627005099017));
#91501=DIRECTION('center_axis',(0.981627005099017,-1.57664003463228E-17,
0.190809912898503));
#91502=DIRECTION('ref_axis',(-0.170749290996154,0.446335030525624,0.8784245671371));
#91503=DIRECTION('center_axis',(0.981627005099017,1.21097659158256E-16,
0.190809912898504));
#91504=DIRECTION('ref_axis',(-0.171594788424947,0.437338367274091,0.882774252623755));
#91505=DIRECTION('center_axis',(0.,1.,0.));
#91506=DIRECTION('ref_axis',(1.,0.,0.));
#91507=DIRECTION('',(-0.190809912898503,0.,0.981627005099017));
#91508=DIRECTION('center_axis',(0.,1.,0.));
#91509=DIRECTION('ref_axis',(0.0397379259201496,0.,0.99921013667975));
#91510=DIRECTION('center_axis',(0.,1.,0.));
#91511=DIRECTION('ref_axis',(0.034250810833452,0.,0.999413268851905));
#91512=DIRECTION('center_axis',(-0.981627005099017,0.,-0.190809912898503));
#91513=DIRECTION('ref_axis',(-0.190809912898503,0.,0.981627005099017));
#91514=DIRECTION('center_axis',(-0.981627005099017,-3.26101604930485E-16,
-0.190809912898504));
#91515=DIRECTION('ref_axis',(-0.17404349559963,0.409900460457291,0.895371696088481));
#91516=DIRECTION('center_axis',(-0.981627005099017,-1.34261283340887E-16,
-0.190809912898504));
#91517=DIRECTION('ref_axis',(-0.174733298347147,0.401759104876689,0.898920405874407));
#91518=DIRECTION('center_axis',(0.,-1.,0.));
#91519=DIRECTION('ref_axis',(0.,0.,-1.));
#91520=DIRECTION('',(-0.190809912898503,0.,0.981627005099017));
#91521=DIRECTION('center_axis',(0.,-1.,0.));
#91522=DIRECTION('ref_axis',(0.14576169806305,0.,0.98931972960099));
#91523=DIRECTION('',(-0.190809912898503,0.,0.981627005099017));
#91524=DIRECTION('center_axis',(0.,-1.,0.));
#91525=DIRECTION('ref_axis',(0.137916286966303,0.,0.990443889268558));
#91526=DIRECTION('center_axis',(0.981627005099017,0.,0.190809912898503));
#91527=DIRECTION('ref_axis',(0.,-1.,0.));
#91528=DIRECTION('',(-0.190809912898503,0.,0.981627005099017));
#91529=DIRECTION('center_axis',(0.981627005099017,1.63768969384934E-17,
0.190809912898503));
#91530=DIRECTION('ref_axis',(-0.169924896128147,0.454894312187821,0.874183444372523));
#91531=DIRECTION('center_axis',(0.981627005099017,4.70972447646461E-17,
0.190809912898503));
#91532=DIRECTION('ref_axis',(-0.170839952553044,0.445381139307003,0.878890978086173));
#91533=DIRECTION('center_axis',(0.,1.,0.));
#91534=DIRECTION('ref_axis',(1.,0.,0.));
#91535=DIRECTION('',(-0.190809912898503,0.,0.981627005099017));
#91536=DIRECTION('center_axis',(0.,1.,0.));
#91537=DIRECTION('ref_axis',(0.113965105299485,0.,0.993484753166387));
#91538=DIRECTION('center_axis',(0.,1.,0.));
#91539=DIRECTION('ref_axis',(0.10665743332964,0.,0.994295827163895));
#91540=DIRECTION('center_axis',(-0.981627005099017,0.,-0.190809912898503));
#91541=DIRECTION('ref_axis',(-0.190809912898503,0.,0.981627005099017));
#91542=DIRECTION('center_axis',(-0.981627005099017,-1.52453231653595E-16,
-0.190809912898504));
#91543=DIRECTION('ref_axis',(-0.173455071838668,0.416694818559092,0.892344533372311));
#91544=DIRECTION('center_axis',(-0.981627005099017,-2.6173755386041E-16,
-0.190809912898504));
#91545=DIRECTION('ref_axis',(-0.174193181128001,0.408150322866915,0.896141757531776));
#91546=DIRECTION('center_axis',(-0.981627005099017,0.,-0.190809912898503));
#91547=DIRECTION('ref_axis',(-0.190809912898503,0.,0.981627005099017));
#91548=DIRECTION('',(-0.190809912898503,0.,0.981627005099017));
#91549=DIRECTION('center_axis',(-0.981627005099017,6.70372400852628E-17,
-0.190809912898503));
#91550=DIRECTION('ref_axis',(-0.172645118482797,0.425833332110878,0.888177705376243));
#91551=DIRECTION('',(-0.190809912898503,0.,0.981627005099017));
#91552=DIRECTION('center_axis',(-0.981627005099017,-3.37053264169227E-16,
-0.190809912898504));
#91553=DIRECTION('ref_axis',(-0.173452293294153,0.416726584693078,0.892330239071299));
#91554=DIRECTION('center_axis',(0.,-1.,0.));
#91555=DIRECTION('ref_axis',(0.,0.,-1.));
#91556=DIRECTION('',(-0.190809912898503,0.,0.981627005099017));
#91557=DIRECTION('center_axis',(0.,-1.,0.));
#91558=DIRECTION('ref_axis',(0.22039446301111,0.,0.975410826613097));
#91559=DIRECTION('center_axis',(0.,-1.,0.));
#91560=DIRECTION('ref_axis',(0.210730120697371,0.,0.977544278399128));
#91561=DIRECTION('center_axis',(0.981627005099017,0.,0.190809912898503));
#91562=DIRECTION('ref_axis',(0.,-1.,0.));
#91563=DIRECTION('',(-0.190809912898503,0.,0.981627005099017));
#91564=DIRECTION('',(0.,1.,0.));
#91565=DIRECTION('center_axis',(0.981627005099017,4.38639578588372E-16,
0.190809912898504));
#91566=DIRECTION('ref_axis',(-0.169421882294232,0.460018699991902,0.871595675446844));
#91567=DIRECTION('center_axis',(0.981627005099017,2.79740284150959E-16,
0.190809912898504));
#91568=DIRECTION('ref_axis',(-0.169818718509315,0.455982046898394,0.873637210603008));
#91569=DIRECTION('center_axis',(0.,1.,0.));
#91570=DIRECTION('ref_axis',(1.,0.,0.));
#91571=DIRECTION('center_axis',(0.,1.,0.));
#91572=DIRECTION('ref_axis',(0.189328555217771,0.,0.981913793659684));
#91573=DIRECTION('',(-0.981627005099017,0.,-0.190809912898503));
#91574=DIRECTION('center_axis',(0.,1.,0.));
#91575=DIRECTION('ref_axis',(0.180140439134743,0.,0.983640901034693));
#91576=DIRECTION('center_axis',(-0.190809912898503,0.,0.981627005099017));
#91577=DIRECTION('ref_axis',(0.,1.,0.));
#91578=DIRECTION('center_axis',(0.190809912898503,-1.0490812575817E-16,
-0.981627005099017));
#91579=DIRECTION('ref_axis',(0.629209430370232,0.767552346417929,0.122306533928078));
#91580=DIRECTION('center_axis',(-0.981627005099017,0.,-0.190809912898503));
#91581=DIRECTION('ref_axis',(-0.190809912898503,0.,0.981627005099017));
#91582=DIRECTION('',(-0.190809912898503,0.,0.981627005099017));
#91583=DIRECTION('center_axis',(-0.981627005099017,1.77118070983608E-17,
-0.190809912898503));
#91584=DIRECTION('ref_axis',(-0.17748337255926,0.367159421047011,0.913068240604948));
#91585=DIRECTION('',(-0.190809912898503,0.,0.981627005099017));
#91586=DIRECTION('center_axis',(-0.981627005099017,-5.92257891558324E-17,
-0.190809912898503));
#91587=DIRECTION('ref_axis',(-0.178099143471772,0.358876189925692,0.916236091517377));
#91588=DIRECTION('center_axis',(0.,-1.,0.));
#91589=DIRECTION('ref_axis',(0.,0.,-1.));
#91590=DIRECTION('',(-0.190809912898503,0.,0.981627005099017));
#91591=DIRECTION('center_axis',(0.,-1.,0.));
#91592=DIRECTION('ref_axis',(0.282313487580406,0.,0.959322205898617));
#91593=DIRECTION('center_axis',(0.,-1.,0.));
#91594=DIRECTION('ref_axis',(0.27169297752195,0.,0.962383980521942));
#91595=DIRECTION('center_axis',(0.981627005099017,0.,0.190809912898503));
#91596=DIRECTION('ref_axis',(0.,-1.,0.));
#91597=DIRECTION('',(-0.190809912898503,0.,0.981627005099017));
#91598=DIRECTION('',(0.,1.,0.));
#91599=DIRECTION('center_axis',(0.981627005099017,2.74504066559155E-17,
0.190809912898503));
#91600=DIRECTION('ref_axis',(-0.174748898384523,0.40157270146071,0.899000660708847));
#91601=DIRECTION('center_axis',(0.981627005099017,5.23739686473236E-17,
0.190809912898503));
#91602=DIRECTION('ref_axis',(-0.174916036819089,0.399569073108612,0.899860509122735));
#91603=DIRECTION('center_axis',(0.,1.,0.));
#91604=DIRECTION('ref_axis',(1.,0.,0.));
#91605=DIRECTION('center_axis',(0.,1.,0.));
#91606=DIRECTION('ref_axis',(0.251348939241017,0.,0.967896539275978));
#91607=DIRECTION('',(-0.981627005099017,0.,-0.190809912898503));
#91608=DIRECTION('center_axis',(0.,1.,0.));
#91609=DIRECTION('ref_axis',(0.241209387750856,0.,0.970473096618787));
#91610=DIRECTION('center_axis',(-0.190809912898503,0.,0.981627005099017));
#91611=DIRECTION('ref_axis',(0.,1.,0.));
#91612=DIRECTION('center_axis',(0.190809912898504,2.21472709933915E-16,
-0.981627005099017));
#91613=DIRECTION('ref_axis',(0.743449495922876,0.652992294713776,0.144512664000285));
#91614=DIRECTION('center_axis',(0.,-1.,0.));
#91615=DIRECTION('ref_axis',(0.,0.,-1.));
#91616=DIRECTION('',(-0.190809912898503,0.,0.981627005099017));
#91617=DIRECTION('center_axis',(0.,-1.,0.));
#91618=DIRECTION('ref_axis',(0.271655976778535,0.,0.962394425524431));
#91619=DIRECTION('',(-0.190809912898503,0.,0.981627005099017));
#91620=DIRECTION('center_axis',(0.,-1.,0.));
#91621=DIRECTION('ref_axis',(0.261714879697109,0.,0.965145233498631));
#91622=DIRECTION('center_axis',(0.981627005099017,0.,0.190809912898503));
#91623=DIRECTION('ref_axis',(0.,-1.,0.));
#91624=DIRECTION('',(-0.190809912898513,0.,0.981627005099015));
#91625=DIRECTION('center_axis',(0.981627005099017,3.56855286526902E-16,
0.190809912898504));
#91626=DIRECTION('ref_axis',(-0.179626317633374,0.337323436149387,0.92409268227697));
#91627=DIRECTION('center_axis',(0.981627005099017,-1.39663916392863E-16,
0.190809912898503));
#91628=DIRECTION('ref_axis',(-0.180156291552091,0.32946923572111,0.926819148123055));
#91629=DIRECTION('center_axis',(0.,1.,0.));
#91630=DIRECTION('ref_axis',(1.,0.,0.));
#91631=DIRECTION('',(-0.190809912898503,0.,0.981627005099017));
#91632=DIRECTION('center_axis',(0.,1.,0.));
#91633=DIRECTION('ref_axis',(0.24013206200696,0.,0.970740229307659));
#91634=DIRECTION('center_axis',(0.,1.,0.));
#91635=DIRECTION('ref_axis',(0.2307209198917,0.,0.973019967484906));
#91636=DIRECTION('center_axis',(-0.981627005099017,0.,-0.190809912898503));
#91637=DIRECTION('ref_axis',(-0.190809912898503,0.,0.981627005099017));
#91638=DIRECTION('center_axis',(-0.981627005099017,-3.01100720672133E-16,
-0.190809912898504));
#91639=DIRECTION('ref_axis',(-0.182226664219433,0.296551840076391,0.937470238991492));
#91640=DIRECTION('center_axis',(-0.981627005099017,-8.46082702226177E-18,
-0.190809912898503));
#91641=DIRECTION('ref_axis',(-0.182618174576295,0.289861538016888,0.939484375119089));
#91642=DIRECTION('center_axis',(0.,-1.,0.));
#91643=DIRECTION('ref_axis',(0.,0.,-1.));
#91644=DIRECTION('',(-0.190809912898503,0.,0.981627005099017));
#91645=DIRECTION('center_axis',(0.,-1.,0.));
#91646=DIRECTION('ref_axis',(0.263749234009829,0.,0.964591282128979));
#91647=DIRECTION('',(-0.190809912898503,0.,0.981627005099017));
#91648=DIRECTION('center_axis',(0.,-1.,0.));
#91649=DIRECTION('ref_axis',(0.254293746183647,0.,0.96712702922206));
#91650=DIRECTION('center_axis',(0.981627005099017,0.,0.190809912898503));
#91651=DIRECTION('ref_axis',(0.,-1.,0.));
#91652=DIRECTION('',(-0.190809912898503,0.,0.981627005099017));
#91653=DIRECTION('center_axis',(0.981627005099017,1.0065149107169E-16,0.190809912898504));
#91654=DIRECTION('ref_axis',(-0.183959150638866,0.265552492287812,0.946383064480741));
#91655=DIRECTION('center_axis',(0.981627005099017,-8.72899477455393E-18,
0.190809912898503));
#91656=DIRECTION('ref_axis',(-0.184280052602452,0.259369398333688,0.948033953727849));
#91657=DIRECTION('center_axis',(0.,1.,0.));
#91658=DIRECTION('ref_axis',(1.,0.,0.));
#91659=DIRECTION('',(-0.190809912898514,0.,0.981627005099015));
#91660=DIRECTION('center_axis',(0.,1.,0.));
#91661=DIRECTION('ref_axis',(0.231663694247404,0.,0.972795935830144));
#91662=DIRECTION('center_axis',(0.,1.,0.));
#91663=DIRECTION('ref_axis',(0.222779670595217,0.,0.974868821108505));
#91664=DIRECTION('center_axis',(-0.981627005099017,0.,-0.190809912898503));
#91665=DIRECTION('ref_axis',(-0.190809912898503,0.,0.981627005099017));
#91666=DIRECTION('center_axis',(-0.981627005099017,-2.21397588729509E-16,
-0.190809912898504));
#91667=DIRECTION('ref_axis',(-0.185875612836097,0.225944259105799,0.956242358573357));
#91668=DIRECTION('center_axis',(-0.981627005099017,-1.69216540445236E-17,
-0.190809912898503));
#91669=DIRECTION('ref_axis',(-0.186098528244237,0.220846886108093,0.957389153208709));
#91670=DIRECTION('center_axis',(0.,-1.,0.));
#91671=DIRECTION('ref_axis',(0.,0.,-1.));
#91672=DIRECTION('',(-0.190809912898503,0.,0.981627005099017));
#91673=DIRECTION('center_axis',(0.,-1.,0.));
#91674=DIRECTION('ref_axis',(0.258226029723844,0.,0.966084529206974));
#91675=DIRECTION('',(-0.190809912898503,0.,0.981627005099017));
#91676=DIRECTION('center_axis',(0.,-1.,0.));
#91677=DIRECTION('ref_axis',(0.249100565290067,0.,0.968477624094728));
#91678=DIRECTION('center_axis',(0.981627005099017,0.,0.190809912898503));
#91679=DIRECTION('ref_axis',(0.,-1.,0.));
#91680=DIRECTION('',(-0.190809912898503,0.,0.981627005099017));
#91681=DIRECTION('center_axis',(0.981627005099017,1.28101897727606E-16,
0.190809912898504));
#91682=DIRECTION('ref_axis',(-0.187193054543419,0.193781548426199,0.963019974777392));
#91683=DIRECTION('center_axis',(0.981627005099017,9.60189425200933E-17,
0.190809912898504));
#91684=DIRECTION('ref_axis',(-0.187361055560064,0.189269560946194,0.963884260769235));
#91685=DIRECTION('center_axis',(0.,1.,0.));
#91686=DIRECTION('ref_axis',(1.,0.,0.));
#91687=DIRECTION('',(-0.190809912898503,0.,0.981627005099017));
#91688=DIRECTION('center_axis',(0.,1.,0.));
#91689=DIRECTION('ref_axis',(0.22553298929724,0.,0.97423553144948));
#91690=DIRECTION('center_axis',(0.,1.,0.));
#91691=DIRECTION('ref_axis',(0.217018515201224,0.,0.976167487708875));
#91692=DIRECTION('center_axis',(-0.981627005099017,0.,-0.190809912898503));
#91693=DIRECTION('ref_axis',(-0.190809912898503,0.,0.981627005099017));
#91694=DIRECTION('center_axis',(-0.981627005099017,-2.21397588729509E-17,
-0.190809912898503));
#91695=DIRECTION('ref_axis',(-0.18849378350218,0.155336678135299,0.96971161177276));
#91696=DIRECTION('center_axis',(-0.981627005099017,-5.92257891558324E-17,
-0.190809912898504));
#91697=DIRECTION('ref_axis',(-0.188597716032453,0.151832234199303,0.970246295620545));
#91698=DIRECTION('center_axis',(0.,-1.,0.));
#91699=DIRECTION('ref_axis',(0.,0.,-1.));
#91700=DIRECTION('',(-0.190809912898503,0.,0.981627005099017));
#91701=DIRECTION('center_axis',(0.,-1.,0.));
#91702=DIRECTION('ref_axis',(0.254848902675841,0.,0.966980887507566));
#91703=DIRECTION('',(-0.190809912898503,0.,0.981627005099017));
#91704=DIRECTION('center_axis',(0.,-1.,0.));
#91705=DIRECTION('ref_axis',(0.245921538009721,0.,0.969289738490475));
#91706=DIRECTION('center_axis',(0.981627005099017,0.,0.190809912898503));
#91707=DIRECTION('ref_axis',(0.,-1.,0.));
#91708=DIRECTION('',(-0.190809912898503,0.,0.981627005099017));
#91709=DIRECTION('center_axis',(0.981627005099017,7.77761521917607E-17,
0.190809912898504));
#91710=DIRECTION('ref_axis',(-0.189384333256716,0.122010604564695,0.974293070226134));
#91711=DIRECTION('center_axis',(0.981627005099017,-2.61869843236618E-17,
0.190809912898503));
#91712=DIRECTION('ref_axis',(-0.18945018196364,0.119169723558698,0.974631830765283));
#91713=DIRECTION('center_axis',(0.,1.,0.));
#91714=DIRECTION('ref_axis',(1.,0.,0.));
#91715=DIRECTION('',(-0.190809912898503,0.,0.981627005099017));
#91716=DIRECTION('center_axis',(0.,1.,0.));
#91717=DIRECTION('ref_axis',(0.22146806454091,0.,0.975167624764329));
#91718=DIRECTION('center_axis',(0.,1.,0.));
#91719=DIRECTION('ref_axis',(0.213193096245038,0.,0.977010083731716));
#91720=DIRECTION('center_axis',(-0.981627005099017,0.,-0.190809912898503));
#91721=DIRECTION('ref_axis',(-0.190809912898503,0.,0.981627005099017));
#91722=DIRECTION('center_axis',(-0.981627005099017,-9.29869872663939E-17,
-0.190809912898504));
#91723=DIRECTION('ref_axis',(-0.190123765131721,0.0847290971646923,0.978097098465073));
#91724=DIRECTION('center_axis',(-0.981627005099017,8.46082702226177E-18,
-0.190809912898503));
#91725=DIRECTION('ref_axis',(-0.190154428082908,0.0828175822905362,0.978254844886552));
#91726=DIRECTION('center_axis',(0.,-1.,0.));
#91727=DIRECTION('ref_axis',(0.,0.,-1.));
#91728=DIRECTION('',(-0.190809912898503,0.,0.981627005099017));
#91729=DIRECTION('center_axis',(0.,-1.,0.));
#91730=DIRECTION('ref_axis',(0.253480050643459,0.,0.967340614223237));
#91731=DIRECTION('',(-0.190809912898503,0.,0.981627005099017));
#91732=DIRECTION('center_axis',(0.,-1.,0.));
#91733=DIRECTION('ref_axis',(0.244632188793599,0.,0.969615950882643));
#91734=DIRECTION('center_axis',(0.981627005099017,0.,0.190809912898503));
#91735=DIRECTION('ref_axis',(0.,-1.,0.));
#91736=DIRECTION('',(-0.190809912898503,0.,0.981627005099017));
#91737=DIRECTION('center_axis',(0.981627005099017,1.02939024959683E-17,
0.190809912898504));
#91738=DIRECTION('ref_axis',(-0.190568956404661,0.0502396607031005,0.980387397586931));
#91739=DIRECTION('center_axis',(0.981627005099017,1.30934921618309E-17,
0.190809912898504));
#91740=DIRECTION('ref_axis',(-0.190580053267881,0.0490698861712299,0.980444485714288));
#91741=DIRECTION('center_axis',(0.,1.,0.));
#91742=DIRECTION('ref_axis',(1.,0.,0.));
#91743=DIRECTION('',(-0.190809912898503,0.,0.981627005099017));
#91744=DIRECTION('center_axis',(0.,1.,0.));
#91745=DIRECTION('ref_axis',(0.219299875562532,0.,0.975657503726722));
#91746=DIRECTION('center_axis',(0.,1.,0.));
#91747=DIRECTION('ref_axis',(0.211150870270054,0.,0.977453482261022));
#91748=DIRECTION('center_axis',(-0.981627005099017,0.,-0.190809912898503));
#91749=DIRECTION('ref_axis',(-0.190809912898503,0.,0.981627005099017));
#91750=DIRECTION('center_axis',(-0.981627005099017,-4.42795177459018E-18,
-0.190809912898504));
#91751=DIRECTION('ref_axis',(-0.190790886558758,0.0141215161941199,0.981529123554926));
#91752=DIRECTION('center_axis',(-0.981627005099017,-5.81681857780497E-18,
-0.190809912898504));
#91753=DIRECTION('ref_axis',(-0.190791735395725,0.0138029303817604,0.981533490420762));
#91754=DIRECTION('center_axis',(0.,-1.,0.));
#91755=DIRECTION('ref_axis',(0.,0.,-1.));
#91756=DIRECTION('',(-0.190809912898503,0.,0.981627005099017));
#91757=DIRECTION('center_axis',(0.,-1.,0.));
#91758=DIRECTION('ref_axis',(-0.456322349908717,0.,0.88981453852687));
#91759=DIRECTION('',(-0.190809912898503,0.,0.981627005099017));
#91760=DIRECTION('center_axis',(0.,-1.,0.));
#91761=DIRECTION('ref_axis',(-0.451413722984057,0.,0.892314771087912));
#91762=DIRECTION('center_axis',(0.981627005099017,0.,0.190809912898503));
#91763=DIRECTION('ref_axis',(0.,-1.,0.));
#91764=DIRECTION('',(-0.190809912898503,0.,0.981627005099017));
#91765=DIRECTION('center_axis',(0.981627005099017,-5.03423776168928E-18,
0.190809912898503));
#91766=DIRECTION('ref_axis',(-0.190597817156863,0.0471367664159099,0.980535872544646));
#91767=DIRECTION('center_axis',(0.981627005099017,3.86331268348434E-17,
0.190809912898504));
#91768=DIRECTION('ref_axis',(-0.190606462635872,0.0461665968132409,0.980580349456445));
#91769=DIRECTION('center_axis',(0.,1.,0.));
#91770=DIRECTION('ref_axis',(1.,0.,0.));
#91771=DIRECTION('',(-0.190809912898503,0.,0.981627005099017));
#91772=DIRECTION('center_axis',(0.,1.,0.));
#91773=DIRECTION('ref_axis',(-0.486439685574001,0.,0.873714159378608));
#91774=DIRECTION('center_axis',(0.,1.,0.));
#91775=DIRECTION('ref_axis',(-0.480986849771355,0.,0.87672780858544));
#91776=DIRECTION('center_axis',(-0.981627005099017,0.,-0.190809912898503));
#91777=DIRECTION('ref_axis',(-0.190809912898503,0.,0.981627005099017));
#91778=DIRECTION('center_axis',(-0.981627005099017,-8.22446506600238E-18,
-0.190809912898504));
#91779=DIRECTION('ref_axis',(-0.190792243226586,0.0136087651545897,0.981536102971019));
#91780=DIRECTION('center_axis',(-0.981627005099017,-8.86796068167317E-18,
-0.190809912898504));
#91781=DIRECTION('ref_axis',(-0.190792977663555,0.0133229533631895,0.981539881302821));
#91782=DIRECTION('center_axis',(0.,-1.,0.));
#91783=DIRECTION('ref_axis',(0.,0.,-1.));
#91784=DIRECTION('',(-0.190809912898503,0.,0.981627005099017));
#91785=DIRECTION('center_axis',(0.,-1.,0.));
#91786=DIRECTION('ref_axis',(-0.457080350189202,0.,0.889425406355652));
#91787=DIRECTION('',(-0.190809912898503,0.,0.981627005099017));
#91788=DIRECTION('center_axis',(0.,-1.,0.));
#91789=DIRECTION('ref_axis',(-0.452130012986409,0.,0.891952045435689));
#91790=DIRECTION('center_axis',(0.981627005099017,0.,0.190809912898503));
#91791=DIRECTION('ref_axis',(0.,-1.,0.));
#91792=DIRECTION('',(-0.190809912898503,0.,0.981627005099017));
#91793=DIRECTION('center_axis',(0.981627005099017,4.02739020935142E-18,
0.190809912898503));
#91794=DIRECTION('ref_axis',(-0.189555553111424,0.114475004152895,0.975173915621627));
#91795=DIRECTION('center_axis',(0.981627005099017,3.09065014678748E-17,
0.190809912898504));
#91796=DIRECTION('ref_axis',(-0.189606818394553,0.112118877975005,0.975437651323713));
#91797=DIRECTION('center_axis',(0.,1.,0.));
#91798=DIRECTION('ref_axis',(1.,0.,0.));
#91799=DIRECTION('',(-0.190809912898503,0.,0.981627005099017));
#91800=DIRECTION('center_axis',(0.,1.,0.));
#91801=DIRECTION('ref_axis',(-0.487887564638898,0.,0.872906480827543));
#91802=DIRECTION('center_axis',(0.,1.,0.));
#91803=DIRECTION('ref_axis',(-0.482355027838568,0.,0.87597581423168));
#91804=DIRECTION('center_axis',(-0.981627005099017,0.,-0.190809912898503));
#91805=DIRECTION('ref_axis',(-0.190809912898503,0.,0.981627005099017));
#91806=DIRECTION('center_axis',(-0.981627005099017,-1.23366975990036E-17,
-0.190809912898503));
#91807=DIRECTION('ref_axis',(-0.190172770405938,0.0816525909275333,0.978349207487261));
#91808=DIRECTION('center_axis',(-0.981627005099017,-2.36478951511284E-17,
-0.190809912898504));
#91809=DIRECTION('ref_axis',(-0.190199294463509,0.0799377201791571,0.978485661253215));
#91810=DIRECTION('center_axis',(0.,-1.,0.));
#91811=DIRECTION('ref_axis',(0.,0.,-1.));
#91812=DIRECTION('',(-0.190809912898503,0.,0.981627005099017));
#91813=DIRECTION('center_axis',(0.,-1.,0.));
#91814=DIRECTION('ref_axis',(-0.458948807817462,0.,0.888462712668872));
#91815=DIRECTION('',(-0.190809912898503,0.,0.981627005099017));
#91816=DIRECTION('center_axis',(0.,-1.,0.));
#91817=DIRECTION('ref_axis',(-0.45389466954082,0.,0.891055345622498));
#91818=DIRECTION('center_axis',(0.981627005099017,0.,0.190809912898503));
#91819=DIRECTION('ref_axis',(0.,-1.,0.));
#91820=DIRECTION('',(-0.190809912898503,0.,0.981627005099017));
#91821=DIRECTION('center_axis',(0.981627005099017,3.62465118841628E-17,
0.190809912898503));
#91822=DIRECTION('ref_axis',(-0.187629699233558,0.181813241889893,0.965266305761789));
#91823=DIRECTION('center_axis',(0.981627005099017,1.93165634174218E-17,
0.190809912898503));
#91824=DIRECTION('ref_axis',(-0.187760314987319,0.178071159136799,0.965938262209102));
#91825=DIRECTION('center_axis',(0.,1.,0.));
#91826=DIRECTION('ref_axis',(1.,0.,0.));
#91827=DIRECTION('',(-0.190809912898503,0.,0.981627005099017));
#91828=DIRECTION('center_axis',(0.,1.,0.));
#91829=DIRECTION('ref_axis',(-0.490598707770679,0.,0.871385625273759));
#91830=DIRECTION('center_axis',(0.,1.,0.));
#91831=DIRECTION('ref_axis',(-0.484914894814882,0.,0.874561344210154));
#91832=DIRECTION('center_axis',(-0.981627005099017,0.,-0.190809912898503));
#91833=DIRECTION('ref_axis',(-0.190809912898503,0.,0.981627005099017));
#91834=DIRECTION('center_axis',(-0.981627005099017,-6.5795720528019E-17,
-0.190809912898504));
#91835=DIRECTION('ref_axis',(-0.188659868247639,0.149696416700501,0.970566039453171));
#91836=DIRECTION('center_axis',(-0.981627005099017,-3.94131585852141E-18,
-0.190809912898503));
#91837=DIRECTION('ref_axis',(-0.188749718337979,0.146552486995096,0.971028275789581));
#91838=DIRECTION('center_axis',(0.,-1.,0.));
#91839=DIRECTION('ref_axis',(0.,0.,-1.));
#91840=DIRECTION('',(-0.190809912898514,0.,0.981627005099015));
#91841=DIRECTION('center_axis',(0.,-1.,0.));
#91842=DIRECTION('ref_axis',(-0.461999637342515,0.,0.886880113146858));
#91843=DIRECTION('',(-0.190809912898503,0.,0.981627005099017));
#91844=DIRECTION('center_axis',(0.,-1.,0.));
#91845=DIRECTION('ref_axis',(-0.45677297861006,0.,0.889583299085416));
#91846=DIRECTION('center_axis',(0.981627005099017,0.,0.190809912898503));
#91847=DIRECTION('ref_axis',(0.,-1.,0.));
#91848=DIRECTION('',(-0.190809912898503,0.,0.981627005099017));
#91849=DIRECTION('center_axis',(0.981627005099017,1.04712145443137E-16,
0.190809912898504));
#91850=DIRECTION('ref_axis',(-0.184792632056183,0.249151479626997,0.950670933255786));
#91851=DIRECTION('center_axis',(0.981627005099017,1.54532507339374E-17,
0.190809912898503));
#91852=DIRECTION('ref_axis',(-0.185041602094931,0.244023440298493,0.951951766676773));
#91853=DIRECTION('center_axis',(0.,1.,0.));
#91854=DIRECTION('ref_axis',(1.,0.,0.));
#91855=DIRECTION('',(-0.190809912898503,0.,0.981627005099017));
#91856=DIRECTION('center_axis',(0.,1.,0.));
#91857=DIRECTION('ref_axis',(-0.494679381455157,0.,0.869075548823659));
#91858=DIRECTION('center_axis',(0.,1.,0.));
#91859=DIRECTION('ref_axis',(-0.48876283045677,0.,0.872416698352276));
#91860=DIRECTION('center_axis',(-0.981627005099017,0.,-0.190809912898503));
#91861=DIRECTION('ref_axis',(-0.190809912898503,0.,0.981627005099017));
#91862=DIRECTION('center_axis',(-0.981627005099017,-4.11223253300119E-17,
-0.190809912898503));
#91863=DIRECTION('ref_axis',(-0.186231764007846,0.217740242473403,0.958074588370942));
#91864=DIRECTION('center_axis',(-0.981627005099017,-7.88263171704282E-18,
-0.190809912898503));
#91865=DIRECTION('ref_axis',(-0.186424284899994,0.213167253811106,0.959065017557286));
#91866=DIRECTION('center_axis',(0.,-1.,0.));
#91867=DIRECTION('ref_axis',(0.,0.,-1.));
#91868=DIRECTION('',(-0.190809912898503,0.,0.981627005099017));
#91869=DIRECTION('center_axis',(0.,-1.,0.));
#91870=DIRECTION('ref_axis',(-0.466356255895842,0.,0.884596994448213));
#91871=DIRECTION('',(-0.190809912898503,0.,0.981627005099017));
#91872=DIRECTION('center_axis',(0.,-1.,0.));
#91873=DIRECTION('ref_axis',(-0.46087664993961,0.,0.887464204089631));
#91874=DIRECTION('center_axis',(0.981627005099017,0.,0.190809912898503));
#91875=DIRECTION('ref_axis',(0.,-1.,0.));
#91876=DIRECTION('',(-0.190809912898503,0.,0.981627005099017));
#91877=DIRECTION('center_axis',(0.981627005099017,2.41643412561085E-17,
0.190809912898503));
#91878=DIRECTION('ref_axis',(-0.181001508829926,0.316489717364005,0.931167392365166));
#91879=DIRECTION('center_axis',(0.981627005099017,-4.63597522018122E-17,
0.190809912898503));
#91880=DIRECTION('ref_axis',(-0.181411469998084,0.30997572146031,0.93327644921443));
#91881=DIRECTION('center_axis',(0.,1.,0.));
#91882=DIRECTION('ref_axis',(1.,0.,0.));
#91883=DIRECTION('',(-0.190809912898503,0.,0.981627005099017));
#91884=DIRECTION('center_axis',(0.,1.,0.));
#91885=DIRECTION('ref_axis',(-0.500299644059964,0.,0.865852335074217));
#91886=DIRECTION('center_axis',(0.,1.,0.));
#91887=DIRECTION('ref_axis',(-0.494052506517587,0.,0.869432067963731));
#91888=DIRECTION('center_axis',(-0.981627005099017,0.,-0.190809912898503));
#91889=DIRECTION('ref_axis',(-0.190809912898503,0.,0.981627005099017));
#91890=DIRECTION('center_axis',(-0.981627005099017,-2.30285021848067E-16,
-0.190809912898504));
#91891=DIRECTION('ref_axis',(-0.1828520022276,0.285784068246309,0.940687308098683));
#91892=DIRECTION('center_axis',(-0.981627005099017,-4.72957903022569E-17,
-0.190809912898503));
#91893=DIRECTION('ref_axis',(-0.183189642441488,0.279782020627107,0.942424307748889));
#91894=DIRECTION('center_axis',(0.,-1.,0.));
#91895=DIRECTION('ref_axis',(0.,0.,-1.));
#91896=DIRECTION('',(-0.190809912898503,0.,0.981627005099017));
#91897=DIRECTION('center_axis',(0.,-1.,0.));
#91898=DIRECTION('ref_axis',(-0.472208353495432,0.,0.881486965807852));
#91899=DIRECTION('',(-0.190809912898503,0.,0.981627005099017));
#91900=DIRECTION('center_axis',(0.,-1.,0.));
#91901=DIRECTION('ref_axis',(-0.466376613371833,0.,0.884586261762989));
#91902=DIRECTION('center_axis',(0.981627005099017,0.,0.190809912898503));
#91903=DIRECTION('ref_axis',(0.,-1.,0.));
#91904=DIRECTION('',(-0.190809912898503,0.,0.981627005099017));
#91905=DIRECTION('center_axis',(0.981627005099017,1.20821706280543E-16,
0.190809912898504));
#91906=DIRECTION('ref_axis',(-0.176194756005532,0.383827955100998,0.906438916220579));
#91907=DIRECTION('center_axis',(0.981627005099017,8.49928790366556E-17,
0.190809912898504));
#91908=DIRECTION('ref_axis',(-0.176813791054772,0.375928002622107,0.909623559576923));
#91909=DIRECTION('center_axis',(0.,1.,0.));
#91910=DIRECTION('ref_axis',(1.,0.,0.));
#91911=DIRECTION('',(-0.190809912898503,0.,0.981627005099017));
#91912=DIRECTION('center_axis',(0.,1.,0.));
#91913=DIRECTION('ref_axis',(-0.507714640295235,0.,0.861525300864624));
#91914=DIRECTION('center_axis',(0.,1.,0.));
#91915=DIRECTION('ref_axis',(-0.501013274042692,0.,0.865439598835772));
#91916=DIRECTION('center_axis',(-0.981627005099017,0.,-0.190809912898503));
#91917=DIRECTION('ref_axis',(-0.190809912898503,0.,0.981627005099017));
#91918=DIRECTION('center_axis',(-0.981627005099017,-2.79631812244081E-16,
-0.190809912898504));
#91919=DIRECTION('ref_axis',(-0.178466524218741,0.353827894019299,0.918126092182958));
#91920=DIRECTION('center_axis',(-0.981627005099017,-3.94131585852141E-17,
-0.190809912898503));
#91921=DIRECTION('ref_axis',(-0.178996506850741,0.346396787442996,0.92085260285477));
#91922=DIRECTION('center_axis',(0.,-1.,0.));
#91923=DIRECTION('ref_axis',(0.,0.,-1.));
#91924=DIRECTION('',(-0.190809912898503,0.,0.981627005099017));
#91925=DIRECTION('center_axis',(0.,-1.,0.));
#91926=DIRECTION('ref_axis',(-0.408333110934888,0.,0.912832991578545));
#91927=DIRECTION('',(-0.190809912898503,0.,0.981627005099017));
#91928=DIRECTION('center_axis',(0.,-1.,0.));
#91929=DIRECTION('ref_axis',(-0.403787833181439,0.,0.914852657958995));
#91930=DIRECTION('center_axis',(0.981627005099017,0.,0.190809912898503));
#91931=DIRECTION('ref_axis',(0.,-1.,0.));
#91932=DIRECTION('',(-0.190809912898503,0.,0.981627005099017));
#91933=DIRECTION('center_axis',(0.981627005099017,-7.78644601242735E-17,
0.190809912898503));
#91934=DIRECTION('ref_axis',(-0.176701106409977,0.377380441141686,0.909043850227917));
#91935=DIRECTION('center_axis',(0.981627005099017,1.79504978852495E-16,
0.190809912898504));
#91936=DIRECTION('ref_axis',(-0.177278780443546,0.369864269024907,0.912015710666829));
#91937=DIRECTION('center_axis',(0.,1.,0.));
#91938=DIRECTION('ref_axis',(1.,0.,0.));
#91939=DIRECTION('',(-0.190809912898503,1.064097794141E-14,0.981627005099017));
#91940=DIRECTION('center_axis',(0.,1.,0.));
#91941=DIRECTION('ref_axis',(-0.44357639185695,0.,0.896236567311985));
#91942=DIRECTION('center_axis',(0.,1.,0.));
#91943=DIRECTION('ref_axis',(-0.438183684981793,0.,0.89888545333417));
#91944=DIRECTION('center_axis',(-0.981627005099017,0.,-0.190809912898503));
#91945=DIRECTION('ref_axis',(-0.190809912898503,0.,0.981627005099017));
#91946=DIRECTION('center_axis',(-0.981627005099017,-2.76833414348855E-16,
-0.190809912898504));
#91947=DIRECTION('ref_axis',(-0.178954866317258,0.34698721230299,0.920638381950031));
#91948=DIRECTION('center_axis',(-0.981627005099017,3.03714686040439E-17,
-0.190809912898503));
#91949=DIRECTION('ref_axis',(-0.179444535603438,0.339970424906788,0.923157499471658));
#91950=DIRECTION('center_axis',(0.,-1.,0.));
#91951=DIRECTION('ref_axis',(0.,0.,-1.));
#91952=DIRECTION('',(-0.190809912898503,0.,0.981627005099017));
#91953=DIRECTION('center_axis',(0.,-1.,0.));
#91954=DIRECTION('ref_axis',(-0.343482113457155,0.,0.939159218522081));
#91955=DIRECTION('',(-0.190809912898503,0.,0.981627005099017));
#91956=DIRECTION('center_axis',(0.,-1.,0.));
#91957=DIRECTION('ref_axis',(-0.340267868241483,0.,0.940328547818472));
#91958=DIRECTION('center_axis',(0.981627005099017,0.,0.190809912898503));
#91959=DIRECTION('ref_axis',(0.,-1.,0.));
#91960=DIRECTION('',(-0.190809912898503,0.,0.981627005099017));
#91961=DIRECTION('center_axis',(0.981627005099017,-1.51997840690772E-17,
0.190809912898503));
#91962=DIRECTION('ref_axis',(-0.177052282767594,0.372832240537104,0.910850486953192));
#91963=DIRECTION('center_axis',(0.981627005099017,1.82677034101796E-16,
0.190809912898504));
#91964=DIRECTION('ref_axis',(-0.177602080516299,0.365579404478994,0.913678937054514));
#91965=DIRECTION('center_axis',(0.,1.,0.));
#91966=DIRECTION('ref_axis',(1.,0.,0.));
#91967=DIRECTION('',(-0.190809912898503,0.,0.981627005099017));
#91968=DIRECTION('center_axis',(0.,1.,0.));
#91969=DIRECTION('ref_axis',(-0.378406320814813,0.,0.925639593128663));
#91970=DIRECTION('center_axis',(0.,1.,0.));
#91971=DIRECTION('ref_axis',(-0.374371948525926,0.,0.927278622721834));
#91972=DIRECTION('center_axis',(-0.981627005099017,0.,-0.190809912898503));
#91973=DIRECTION('ref_axis',(-0.190809912898503,0.,0.981627005099017));
#91974=DIRECTION('center_axis',(-0.981627005099017,-1.69041839979963E-16,
-0.190809912898504));
#91975=DIRECTION('ref_axis',(-0.179304181042026,0.34199834358291,0.922435441452351));
#91976=DIRECTION('center_axis',(-0.981627005099017,-1.47690827086916E-17,
-0.190809912898503));
#91977=DIRECTION('ref_axis',(-0.179765955221612,0.335274096521094,0.924811051807463));
#91978=DIRECTION('center_axis',(0.,-1.,0.));
#91979=DIRECTION('ref_axis',(0.,0.,-1.));
#91980=DIRECTION('',(-0.190809912898503,0.,0.981627005099017));
#91981=DIRECTION('center_axis',(0.,-1.,0.));
#91982=DIRECTION('ref_axis',(-0.277694948631048,0.,0.960669306007431));
#91983=DIRECTION('',(-0.190809912898503,0.,0.981627005099017));
#91984=DIRECTION('center_axis',(0.,-1.,0.));
#91985=DIRECTION('ref_axis',(-0.275852862378494,0.,0.961199874280886));
#91986=DIRECTION('center_axis',(0.981627005099017,0.,0.190809912898503));
#91987=DIRECTION('ref_axis',(0.,-1.,0.));
#91988=DIRECTION('',(-0.190809912898503,0.,0.981627005099017));
#91989=DIRECTION('center_axis',(0.981627005099017,8.23307466520019E-17,
0.190809912898503));
#91990=DIRECTION('ref_axis',(-0.17726894004393,0.369993789121012,0.911965086452095));
#91991=DIRECTION('center_axis',(0.981627005099017,2.16013566009539E-17,
0.190809912898503));
#91992=DIRECTION('ref_axis',(-0.177801871146302,0.362902228648605,0.914706765613303));
#91993=DIRECTION('center_axis',(0.,1.,0.));
#91994=DIRECTION('ref_axis',(1.,0.,0.));
#91995=DIRECTION('',(-0.190809912898503,0.,0.981627005099017));
#91996=DIRECTION('center_axis',(0.,1.,0.));
#91997=DIRECTION('ref_axis',(-0.312255689172483,0.,0.949998097145156));
#91998=DIRECTION('center_axis',(0.,1.,0.));
#91999=DIRECTION('ref_axis',(-0.309624667518334,0.,0.950858856647064));
#92000=DIRECTION('center_axis',(-0.981627005099017,0.,-0.190809912898503));
#92001=DIRECTION('ref_axis',(-0.190809912898503,0.,0.981627005099017));
#92002=DIRECTION('center_axis',(-0.981627005099017,7.53381568193085E-17,
-0.190809912898503));
#92003=DIRECTION('ref_axis',(-0.179535702780267,0.338645830481712,0.92362651159684));
#92004=DIRECTION('center_axis',(-0.981627005099017,1.01443693012226E-16,
-0.190809912898503));
#92005=DIRECTION('ref_axis',(-0.179979422483989,0.332113664902088,0.925909240189141));
#92006=DIRECTION('center_axis',(0.,-1.,0.));
#92007=DIRECTION('ref_axis',(0.,0.,-1.));
#92008=DIRECTION('',(-0.190809912898503,0.,0.981627005099017));
#92009=DIRECTION('center_axis',(0.,-1.,0.));
#92010=DIRECTION('ref_axis',(-0.210995669584697,0.,0.977486996034477));
#92011=DIRECTION('',(-0.190809912898503,0.,0.981627005099017));
#92012=DIRECTION('center_axis',(0.,-1.,0.));
#92013=DIRECTION('ref_axis',(-0.21056483084966,0.,0.977579895460854));
#92014=DIRECTION('center_axis',(0.981627005099017,0.,0.190809912898503));
#92015=DIRECTION('ref_axis',(0.,-1.,0.));
#92016=DIRECTION('',(-0.190809912898503,0.,0.981627005099017));
#92017=DIRECTION('center_axis',(0.981627005099017,1.04082907525856E-16,
0.190809912898504));
#92018=DIRECTION('ref_axis',(-0.177363053987237,0.368752895726096,0.912449258300942));
#92019=DIRECTION('center_axis',(0.981627005099017,-5.72324314732877E-17,
0.190809912898503));
#92020=DIRECTION('ref_axis',(-0.177888737325384,0.361731104481622,0.91515365113367));
#92021=DIRECTION('center_axis',(0.,1.,0.));
#92022=DIRECTION('ref_axis',(1.,0.,0.));
#92023=DIRECTION('',(-0.190809912898503,0.,0.981627005099017));
#92024=DIRECTION('center_axis',(0.,1.,0.));
#92025=DIRECTION('ref_axis',(-0.245157759371825,0.,0.969483198936313));
#92026=DIRECTION('center_axis',(0.,1.,0.));
#92027=DIRECTION('ref_axis',(-0.24397218016453,0.,0.969782230867202));
#92028=DIRECTION('center_axis',(-0.981627005099017,0.,-0.190809912898503));
#92029=DIRECTION('ref_axis',(-0.190809912898503,0.,0.981627005099017));
#92030=DIRECTION('center_axis',(-0.981627005099017,-4.47098774198808E-17,
-0.190809912898503));
#92031=DIRECTION('ref_axis',(-0.179662483893508,0.336794004557109,0.924278740627307));
#92032=DIRECTION('center_axis',(-0.981627005099017,-7.16993574248911E-17,
-0.190809912898503));
#92033=DIRECTION('ref_axis',(-0.180096463940407,0.330366398701499,0.926511363279028));
#92034=DIRECTION('center_axis',(0.,-1.,0.));
#92035=DIRECTION('ref_axis',(0.,0.,-1.));
#92036=DIRECTION('',(-0.190809912898503,0.,0.981627005099017));
#92037=DIRECTION('center_axis',(0.,-1.,0.));
#92038=DIRECTION('ref_axis',(-0.143394636922443,0.,0.989665589025849));
#92039=DIRECTION('',(-0.190809912898503,0.,0.981627005099017));
#92040=DIRECTION('center_axis',(0.,-1.,0.));
#92041=DIRECTION('ref_axis',(-0.144413269309557,0.,0.989517462022437));
#92042=DIRECTION('center_axis',(0.981627005099017,0.,0.190809912898503));
#92043=DIRECTION('ref_axis',(0.,-1.,0.));
#92044=DIRECTION('',(-0.190809912898503,0.,0.981627005099017));
#92045=DIRECTION('center_axis',(0.981627005099017,3.79794977554034E-16,
0.190809912898504));
#92046=DIRECTION('ref_axis',(-0.177339648533324,0.369061948261209,0.912328848279894));
#92047=DIRECTION('center_axis',(0.981627005099017,5.73247788103327E-17,
0.190809912898503));
#92048=DIRECTION('ref_axis',(-0.177867129867076,0.36202282229889,0.915042490951975));
#92049=DIRECTION('center_axis',(0.,1.,0.));
#92050=DIRECTION('ref_axis',(1.,0.,0.));
#92051=DIRECTION('',(-0.190809912898503,0.,0.981627005099017));
#92052=DIRECTION('center_axis',(0.,1.,0.));
#92053=DIRECTION('ref_axis',(-0.177130506572721,0.,0.984187372222023));
#92054=DIRECTION('center_axis',(0.,1.,0.));
#92055=DIRECTION('ref_axis',(-0.177430914250361,0.,0.984133258592697));
#92056=DIRECTION('center_axis',(-0.981627005099017,0.,-0.190809912898503));
#92057=DIRECTION('ref_axis',(-0.190809912898503,0.,0.981627005099017));
#92058=DIRECTION('center_axis',(-0.981627005099017,-1.56091697168055E-16,
-0.190809912898504));
#92059=DIRECTION('ref_axis',(-0.179691336818671,0.336370957433608,0.924427175318595));
#92060=DIRECTION('center_axis',(-0.981627005099017,-1.85967954159957E-16,
-0.190809912898504));
#92061=DIRECTION('ref_axis',(-0.180123114853572,0.329967084990994,0.92664846965718));
#92062=DIRECTION('center_axis',(0.,-1.,0.));
#92063=DIRECTION('ref_axis',(0.,0.,-1.));
#92064=DIRECTION('',(-0.190809912898503,0.,0.981627005099017));
#92065=DIRECTION('center_axis',(0.,-1.,0.));
#92066=DIRECTION('ref_axis',(-0.0748892790042022,0.,0.997191855106243));
#92067=DIRECTION('',(-0.190809912898503,0.,0.981627005099017));
#92068=DIRECTION('center_axis',(0.,-1.,0.));
#92069=DIRECTION('ref_axis',(-0.0773958200853973,0.,0.997000444851109));
#92070=DIRECTION('center_axis',(0.981627005099017,0.,0.190809912898503));
#92071=DIRECTION('ref_axis',(0.,-1.,0.));
#92072=DIRECTION('',(-0.190809912898503,0.,0.981627005099017));
#92073=DIRECTION('center_axis',(0.981627005099017,-6.77038411212549E-17,
0.190809912898503));
#92074=DIRECTION('ref_axis',(-0.1771974842477,0.370932724200007,0.911597480083094));
#92075=DIRECTION('center_axis',(0.981627005099017,1.15770364611182E-16,
0.190809912898504));
#92076=DIRECTION('ref_axis',(-0.177735950146979,0.363788074911298,0.914367633163862));
#92077=DIRECTION('center_axis',(0.,1.,0.));
#92078=DIRECTION('ref_axis',(1.,0.,0.));
#92079=DIRECTION('',(-0.190809912898503,0.,0.981627005099017));
#92080=DIRECTION('center_axis',(0.,1.,0.));
#92081=DIRECTION('ref_axis',(-0.108177998002504,0.,0.994131540968382));
#92082=DIRECTION('center_axis',(0.,1.,0.));
#92083=DIRECTION('ref_axis',(-0.110004590107985,0.,0.993931079177613));
#92084=DIRECTION('center_axis',(-0.981627005099017,0.,-0.190809912898503));
#92085=DIRECTION('ref_axis',(-0.190809912898503,0.,0.981627005099017));
#92086=DIRECTION('center_axis',(-0.981627005099017,-3.43929929287745E-16,
-0.190809912898504));
#92087=DIRECTION('ref_axis',(-0.179623779357055,0.337360558333296,0.924079624042504));
#92088=DIRECTION('center_axis',(-0.981627005099017,-2.08601722339834E-16,
-0.190809912898504));
#92089=DIRECTION('ref_axis',(-0.180060721748086,0.330901079072703,0.926327486557578));
#92090=DIRECTION('center_axis',(0.,-1.,0.));
#92091=DIRECTION('ref_axis',(0.,0.,-1.));
#92092=DIRECTION('',(-0.190809912898503,0.,0.981627005099017));
#92093=DIRECTION('center_axis',(0.,-1.,0.));
#92094=DIRECTION('ref_axis',(-0.00546390507844353,0.,0.999985072759236));
#92095=DIRECTION('',(-0.190809912898503,0.,0.981627005099017));
#92096=DIRECTION('center_axis',(0.,-1.,0.));
#92097=DIRECTION('ref_axis',(-0.00949810829374728,0.,0.999954891952052));
#92098=DIRECTION('center_axis',(0.981627005099017,0.,0.190809912898503));
#92099=DIRECTION('ref_axis',(0.,-1.,0.));
#92100=DIRECTION('',(-0.190809912898503,0.,0.981627005099017));
#92101=DIRECTION('center_axis',(0.981627005099017,-1.07316767773413E-16,
0.190809912898503));
#92102=DIRECTION('ref_axis',(-0.176928890497236,0.374437660883914,0.910215691920986));
#92103=DIRECTION('center_axis',(0.981627005099017,1.76824696986466E-16,
0.190809912898504));
#92104=DIRECTION('ref_axis',(-0.177488407408411,0.367092566139198,0.913094142529107));
#92105=DIRECTION('center_axis',(0.,1.,0.));
#92106=DIRECTION('ref_axis',(1.,0.,0.));
#92107=DIRECTION('',(-0.190809912898503,0.,0.981627005099017));
#92108=DIRECTION('center_axis',(0.,1.,0.));
#92109=DIRECTION('ref_axis',(-0.038290696769099,0.,0.999266642363757));
#92110=DIRECTION('center_axis',(0.,1.,0.));
#92111=DIRECTION('ref_axis',(-0.0416844861317351,0.,0.999130824074572));
#92112=DIRECTION('center_axis',(-0.981627005099017,0.,-0.190809912898503));
#92113=DIRECTION('ref_axis',(-0.190809912898503,0.,0.981627005099017));
#92114=DIRECTION('center_axis',(-0.981627005099017,-7.58528837094573E-17,
-0.190809912898503));
#92115=DIRECTION('ref_axis',(-0.179456238766349,0.339800712708702,0.92321770672496));
#92116=DIRECTION('center_axis',(-0.981627005099017,-2.55275311569698E-16,
-0.190809912898504));
#92117=DIRECTION('ref_axis',(-0.179906116149876,0.333202784993083,0.925532113675544));
#92118=DIRECTION('center_axis',(0.,-1.,0.));
#92119=DIRECTION('ref_axis',(0.,0.,-1.));
#92120=DIRECTION('',(-0.190809912898503,0.,0.981627005099017));
#92121=DIRECTION('center_axis',(0.,-1.,0.));
#92122=DIRECTION('ref_axis',(0.0649114613199094,0.,0.997891027211546));
#92123=DIRECTION('',(-0.190809912898503,0.,0.981627005099017));
#92124=DIRECTION('center_axis',(0.,-1.,0.));
#92125=DIRECTION('ref_axis',(0.059307279506297,0.,0.998239774101174));
#92126=DIRECTION('center_axis',(0.981627005099017,0.,0.190809912898503));
#92127=DIRECTION('ref_axis',(0.,-1.,0.));
#92128=DIRECTION('',(-0.190809912898503,-1.06612429401E-14,0.981627005099017));
#92129=DIRECTION('center_axis',(0.981627005099017,2.36496005194842E-17,
0.190809912898503));
#92130=DIRECTION('ref_axis',(-0.17651869753264,0.379717861790502,0.908105442588376));
#92131=DIRECTION('center_axis',(0.981627005099017,-7.56860369739101E-17,
0.190809912898503));
#92132=DIRECTION('ref_axis',(-0.177111112947321,0.372063984098908,0.911153140480243));
#92133=DIRECTION('center_axis',(0.,1.,0.));
#92134=DIRECTION('ref_axis',(1.,0.,0.));
#92135=DIRECTION('',(-0.190809912898503,0.,0.981627005099017));
#92136=DIRECTION('center_axis',(0.,1.,0.));
#92137=DIRECTION('ref_axis',(0.0325552553334085,0.,0.999469937191798));
#92138=DIRECTION('center_axis',(0.,1.,0.));
#92139=DIRECTION('ref_axis',(0.0275511876846893,0.,0.999620393978216));
#92140=DIRECTION('center_axis',(-0.981627005099017,0.,-0.190809912898503));
#92141=DIRECTION('ref_axis',(-0.190809912898503,0.,0.981627005099017));
#92142=DIRECTION('center_axis',(-0.981627005099017,-2.25165393880573E-16,
-0.190809912898504));
#92143=DIRECTION('ref_axis',(-0.179179567547627,0.343787482964193,0.92179436379845));
#92144=DIRECTION('center_axis',(-0.981627005099017,-4.47537611136289E-17,
-0.190809912898503));
#92145=DIRECTION('ref_axis',(-0.179651202662149,0.336959249251399,0.924220704012833));
#92146=DIRECTION('center_axis',(0.,-1.,0.));
#92147=DIRECTION('ref_axis',(0.,0.,-1.));
#92148=DIRECTION('',(-0.190809912898503,0.,0.981627005099017));
#92149=DIRECTION('center_axis',(0.,-1.,0.));
#92150=DIRECTION('ref_axis',(0.136283439011562,0.,0.990669886617728));
#92151=DIRECTION('',(-0.190809912898503,0.,0.981627005099017));
#92152=DIRECTION('center_axis',(0.,-1.,0.));
#92153=DIRECTION('ref_axis',(0.129062849770344,0.,0.991636415632846));
#92154=DIRECTION('center_axis',(0.981627005099017,0.,0.190809912898503));
#92155=DIRECTION('ref_axis',(0.,-1.,0.));
#92156=DIRECTION('',(-0.190809912898503,0.,0.981627005099017));
#92157=DIRECTION('center_axis',(0.981627005099017,-3.27537938769868E-17,
0.190809912898503));
#92158=DIRECTION('ref_axis',(-0.175941978952378,0.386999638726905,0.905138497506081));
#92159=DIRECTION('center_axis',(0.981627005099017,-1.020440303234E-16,0.190809912898503));
#92160=DIRECTION('ref_axis',(-0.176582176327467,0.378906342395489,0.908432011047567));
#92161=DIRECTION('center_axis',(0.,1.,0.));
#92162=DIRECTION('ref_axis',(1.,0.,0.));
#92163=DIRECTION('',(-0.190809912898503,0.,0.981627005099017));
#92164=DIRECTION('center_axis',(0.,1.,0.));
#92165=DIRECTION('ref_axis',(0.104399906013785,0.,0.994535398879453));
#92166=DIRECTION('center_axis',(0.,1.,0.));
#92167=DIRECTION('ref_axis',(0.0977389164793506,0.,0.995212090061934));
#92168=DIRECTION('center_axis',(-0.981627005099017,0.,-0.190809912898503));
#92169=DIRECTION('ref_axis',(-0.190809912898503,0.,0.981627005099017));
#92170=DIRECTION('center_axis',(-0.981627005099017,-2.80834900414518E-16,
-0.190809912898504));
#92171=DIRECTION('ref_axis',(-0.178777744086074,0.349485976856103,0.919727171611467));
#92172=DIRECTION('center_axis',(-0.981627005099017,-4.31097147534792E-16,
-0.190809912898504));
#92173=DIRECTION('ref_axis',(-0.179281858024905,0.342319625630313,0.92232060005806));
#92174=DIRECTION('center_axis',(0.,-1.,0.));
#92175=DIRECTION('ref_axis',(0.,0.,-1.));
#92176=DIRECTION('',(-0.190809912898503,0.,0.981627005099017));
#92177=DIRECTION('center_axis',(0.,-1.,0.));
#92178=DIRECTION('ref_axis',(0.208719295675094,0.,0.977975590499524));
#92179=DIRECTION('',(-0.190809912898503,0.,0.981627005099017));
#92180=DIRECTION('center_axis',(0.,-1.,0.));
#92181=DIRECTION('ref_axis',(0.19982967058625,0.,0.979830650037745));
#92182=DIRECTION('center_axis',(0.981627005099017,0.,0.190809912898503));
#92183=DIRECTION('ref_axis',(0.,-1.,0.));
#92184=DIRECTION('',(-0.190809912898503,0.,0.981627005099017));
#92185=DIRECTION('center_axis',(0.981627005099017,-5.16046563045143E-17,
0.190809912898503));
#92186=DIRECTION('ref_axis',(-0.175159936094969,0.396623615588896,0.901115255860424));
#92187=DIRECTION('center_axis',(0.981627005099017,3.53789182896801E-16,
0.190809912898504));
#92188=DIRECTION('ref_axis',(-0.17586776654416,0.387925024973219,0.90475670966857));
#92189=DIRECTION('center_axis',(0.,1.,0.));
#92190=DIRECTION('ref_axis',(1.,0.,0.));
#92191=DIRECTION('',(-0.190809912898503,0.,0.981627005099017));
#92192=DIRECTION('center_axis',(0.,1.,0.));
#92193=DIRECTION('ref_axis',(0.177302870499554,0.,0.984156335199148));
#92194=DIRECTION('center_axis',(0.,1.,0.));
#92195=DIRECTION('ref_axis',(0.168932804716011,0.,0.985627570378783));
#92196=DIRECTION('center_axis',(-0.981627005099017,0.,-0.190809912898503));
#92197=DIRECTION('ref_axis',(-0.190809912898503,0.,0.981627005099017));
#92198=DIRECTION('center_axis',(-0.981627005099017,1.25694825159868E-16,
-0.190809912898503));
#92199=DIRECTION('ref_axis',(-0.178225395661155,0.357150536609089,0.916885599484071));
#92200=DIRECTION('center_axis',(-0.981627005099017,2.24702176112819E-16,
-0.190809912898503));
#92201=DIRECTION('ref_axis',(-0.178775847759892,0.349512619419995,0.919717415907683));
#92202=DIRECTION('center_axis',(0.,-1.,0.));
#92203=DIRECTION('ref_axis',(0.,0.,-1.));
#92204=DIRECTION('',(-0.190809912898503,0.,0.981627005099017));
#92205=DIRECTION('center_axis',(0.,-1.,0.));
#92206=DIRECTION('ref_axis',(0.199798691632371,0.,0.979836967470606));
#92207=DIRECTION('',(-0.190809912898503,0.,0.981627005099017));
#92208=DIRECTION('center_axis',(0.,-1.,0.));
#92209=DIRECTION('ref_axis',(0.191473403991459,0.,0.981497802118743));
#92210=DIRECTION('center_axis',(0.981627005099017,0.,0.190809912898503));
#92211=DIRECTION('ref_axis',(0.,-1.,0.));
#92212=DIRECTION('',(-0.190809912898503,0.,0.981627005099017));
#92213=DIRECTION('center_axis',(0.981627005099017,1.46213192862791E-16,
0.190809912898504));
#92214=DIRECTION('ref_axis',(-0.180317335839146,0.327040525134698,0.92764764502234));
#92215=DIRECTION('center_axis',(0.981627005099017,2.46829662486141E-17,
0.190809912898503));
#92216=DIRECTION('ref_axis',(-0.180785163765237,0.31986800304809,0.930054399047929));
#92217=DIRECTION('center_axis',(0.,1.,0.));
#92218=DIRECTION('ref_axis',(1.,0.,0.));
#92219=DIRECTION('',(-0.190809912898503,0.,0.981627005099017));
#92220=DIRECTION('center_axis',(0.,1.,0.));
#92221=DIRECTION('ref_axis',(0.168043234904274,0.,0.985779626084302));
#92222=DIRECTION('center_axis',(0.,1.,0.));
#92223=DIRECTION('ref_axis',(0.160270242051786,0.,0.987073173332485));
#92224=DIRECTION('center_axis',(-0.981627005099017,0.,-0.190809912898503));
#92225=DIRECTION('ref_axis',(-0.190809912898503,0.,0.981627005099017));
#92226=DIRECTION('center_axis',(-0.981627005099017,-9.21762051172364E-17,
-0.190809912898504));
#92227=DIRECTION('ref_axis',(-0.182698509990304,0.288467741107384,0.939897662933431));
#92228=DIRECTION('center_axis',(-0.981627005099017,-2.72852642422708E-16,
-0.190809912898504));
#92229=DIRECTION('ref_axis',(-0.183049019457732,0.282298654146891,0.941700868823225));
#92230=DIRECTION('center_axis',(0.,-1.,0.));
#92231=DIRECTION('ref_axis',(0.,0.,-1.));
#92232=DIRECTION('',(-0.190809912898514,0.,0.981627005099015));
#92233=DIRECTION('center_axis',(0.,-1.,0.));
#92234=DIRECTION('ref_axis',(0.193177433003047,0.,0.981163839212572));
#92235=DIRECTION('',(-0.190809912898503,0.,0.981627005099017));
#92236=DIRECTION('center_axis',(0.,-1.,0.));
#92237=DIRECTION('ref_axis',(0.185255825677008,0.,0.982690327139089));
#92238=DIRECTION('center_axis',(0.981627005099017,0.,0.190809912898503));
#92239=DIRECTION('ref_axis',(0.,-1.,0.));
#92240=DIRECTION('',(-0.190809912898503,0.,0.981627005099017));
#92241=DIRECTION('center_axis',(0.981627005099017,1.97817849167305E-16,
0.190809912898504));
#92242=DIRECTION('ref_axis',(-0.184377642137556,0.257457434680497,0.948536005857201));
#92243=DIRECTION('center_axis',(0.981627005099017,2.71512628734755E-16,
0.190809912898504));
#92244=DIRECTION('ref_axis',(-0.184661337429699,0.25181098112299,0.949995484328506));
#92245=DIRECTION('center_axis',(0.,1.,0.));
#92246=DIRECTION('ref_axis',(1.,0.,0.));
#92247=DIRECTION('',(-0.190809912898503,0.,0.981627005099017));
#92248=DIRECTION('center_axis',(0.,1.,0.));
#92249=DIRECTION('ref_axis',(0.161049074723182,0.,0.986946399522693));
#92250=DIRECTION('center_axis',(0.,1.,0.));
#92251=DIRECTION('ref_axis',(0.153708505209598,0.,0.988116235787183));
#92252=DIRECTION('center_axis',(-0.981627005099017,0.,-0.190809912898503));
#92253=DIRECTION('ref_axis',(-0.190809912898503,0.,0.981627005099017));
#92254=DIRECTION('center_axis',(-0.981627005099017,1.00555860127894E-16,
-0.190809912898503));
#92255=DIRECTION('ref_axis',(-0.186144295153646,0.219784945605611,0.957624602371352));
#92256=DIRECTION('center_axis',(-0.981627005099017,0.,-0.190809912898503));
#92257=DIRECTION('ref_axis',(-0.186344083339142,0.215084688873812,0.958652418354301));
#92258=DIRECTION('center_axis',(0.,-1.,0.));
#92259=DIRECTION('ref_axis',(0.,0.,-1.));
#92260=DIRECTION('',(-0.190809912898503,0.,0.981627005099017));
#92261=DIRECTION('center_axis',(0.,-1.,0.));
#92262=DIRECTION('ref_axis',(0.188550653993909,0.,0.982063465809857));
#92263=DIRECTION('',(-0.190809912898503,0.,0.981627005099017));
#92264=DIRECTION('center_axis',(0.,-1.,0.));
#92265=DIRECTION('ref_axis',(0.180903544065996,0.,0.983500842777657));
#92266=DIRECTION('center_axis',(0.981627005099017,0.,0.190809912898503));
#92267=DIRECTION('ref_axis',(0.,-1.,0.));
#92268=DIRECTION('',(-0.190809912898503,0.,0.981627005099017));
#92269=DIRECTION('center_axis',(0.981627005099017,6.45058203806429E-17,
0.190809912898504));
#92270=DIRECTION('ref_axis',(-0.18741217452723,0.187874344226309,0.964147243744704));
#92271=DIRECTION('center_axis',(0.981627005099017,7.81627264539445E-17,
0.190809912898504));
#92272=DIRECTION('ref_axis',(-0.187560853112628,0.183753959197796,0.964912124941333));
#92273=DIRECTION('center_axis',(0.,1.,0.));
#92274=DIRECTION('ref_axis',(1.,0.,0.));
#92275=DIRECTION('',(-0.190809912898503,0.,0.981627005099017));
#92276=DIRECTION('center_axis',(0.,1.,0.));
#92277=DIRECTION('ref_axis',(0.155983816576654,0.,0.987759610920684));
#92278=DIRECTION('center_axis',(0.,1.,0.));
#92279=DIRECTION('ref_axis',(0.148946583935359,0.,0.98884524326812));
#92280=DIRECTION('center_axis',(-0.981627005099017,0.,-0.190809912898503));
#92281=DIRECTION('ref_axis',(-0.190809912898503,0.,0.981627005099017));
#92282=DIRECTION('center_axis',(-0.981627005099017,5.02779300639471E-17,
-0.190809912898503));
#92283=DIRECTION('ref_axis',(-0.1886190628099,0.151102150103899,0.970356114722164));
#92284=DIRECTION('center_axis',(-0.981627005099017,8.02507771831495E-18,
-0.190809912898503));
#92285=DIRECTION('ref_axis',(-0.188712281941248,0.147870723600793,0.970835683185525));
#92286=DIRECTION('center_axis',(0.,-1.,0.));
#92287=DIRECTION('ref_axis',(0.,0.,-1.));
#92288=DIRECTION('',(-0.190809912898503,0.,0.981627005099017));
#92289=DIRECTION('center_axis',(0.,-1.,0.));
#92290=DIRECTION('ref_axis',(0.185721024850239,0.,0.982602514208353));
#92291=DIRECTION('',(-0.190809912898503,0.,0.981627005099017));
#92292=DIRECTION('center_axis',(0.,-1.,0.));
#92293=DIRECTION('ref_axis',(0.178238744550302,0.,0.983987271229223));
#92294=DIRECTION('center_axis',(0.981627005099017,0.,0.190809912898503));
#92295=DIRECTION('ref_axis',(0.,-1.,0.));
#92296=DIRECTION('',(-0.190809912898514,0.,0.981627005099015));
#92297=DIRECTION('center_axis',(0.981627005099017,-4.30038802537619E-18,
0.190809912898503));
#92298=DIRECTION('ref_axis',(-0.189470225435526,0.118291253772098,0.974734944974497));
#92299=DIRECTION('center_axis',(0.981627005099017,5.34797602053305E-17,
0.190809912898504));
#92300=DIRECTION('ref_axis',(-0.189528540527954,0.115696937272697,0.975034948620336));
#92301=DIRECTION('center_axis',(0.,1.,0.));
#92302=DIRECTION('ref_axis',(1.,0.,0.));
#92303=DIRECTION('',(-0.190809912898503,0.,0.981627005099017));
#92304=DIRECTION('center_axis',(0.,1.,0.));
#92305=DIRECTION('ref_axis',(0.152624503283608,0.,0.988284251112721));
#92306=DIRECTION('center_axis',(0.,1.,0.));
#92307=DIRECTION('ref_axis',(0.145783941845035,0.,0.98931645205168));
#92308=DIRECTION('center_axis',(-0.981627005099017,0.,-0.190809912898503));
#92309=DIRECTION('ref_axis',(-0.190809912898503,0.,0.981627005099017));
#92310=DIRECTION('center_axis',(-0.981627005099017,-2.93287925373025E-17,
-0.190809912898504));
#92311=DIRECTION('ref_axis',(-0.190160727448627,0.0824193546021032,0.978287252152036));
#92312=DIRECTION('center_axis',(-0.981627005099017,-2.00626942957873E-17,
-0.190809912898504));
#92313=DIRECTION('ref_axis',(-0.190188242024429,0.0806567583276901,0.978428801667104));
#92314=DIRECTION('center_axis',(0.,-1.,0.));
#92315=DIRECTION('ref_axis',(0.,0.,-1.));
#92316=DIRECTION('',(-0.190809912898503,0.,0.981627005099017));
#92317=DIRECTION('center_axis',(0.,-1.,0.));
#92318=DIRECTION('ref_axis',(0.184573958484037,0.,0.982818627138056));
#92319=DIRECTION('',(-0.190809912898503,0.,0.981627005099017));
#92320=DIRECTION('center_axis',(0.,-1.,0.));
#92321=DIRECTION('ref_axis',(0.177157841455015,0.,0.984182452196238));
#92322=DIRECTION('center_axis',(0.981627005099017,0.,0.190809912898503));
#92323=DIRECTION('ref_axis',(0.,-1.,0.));
#92324=DIRECTION('',(-0.190809912898503,0.,0.981627005099017));
#92325=DIRECTION('center_axis',(0.981627005099017,2.58023281522571E-17,
0.190809912898504));
#92326=DIRECTION('ref_axis',(-0.190583431643196,0.0487081633179298,0.980461865861848));
#92327=DIRECTION('center_axis',(0.981627005099017,4.2166734008049E-17,0.190809912898504));
#92328=DIRECTION('ref_axis',(-0.190593262483975,0.0476399153475881,0.980512440900874));
#92329=DIRECTION('center_axis',(0.,1.,0.));
#92330=DIRECTION('ref_axis',(1.,0.,0.));
#92331=DIRECTION('',(-0.190809912898503,0.,0.981627005099017));
#92332=DIRECTION('center_axis',(0.,1.,0.));
#92333=DIRECTION('ref_axis',(0.150832413364278,0.,0.988559347271932));
#92334=DIRECTION('center_axis',(0.,1.,0.));
#92335=DIRECTION('ref_axis',(0.144095311729787,0.,0.989563813575201));
#92336=DIRECTION('center_axis',(-0.981627005099017,0.,-0.190809912898503));
#92337=DIRECTION('ref_axis',(-0.190809912898503,0.,0.981627005099017));
#92338=DIRECTION('center_axis',(-0.981627005099017,-3.1423706289967E-18,
-0.190809912898504));
#92339=DIRECTION('ref_axis',(-0.190791909796416,0.0137365591003498,0.981534387630061));
#92340=DIRECTION('center_axis',(-0.981627005099017,-6.52037564613089E-18,
-0.190809912898504));
#92341=DIRECTION('ref_axis',(-0.190792671615323,0.0134427930546203,0.981538306829019));
#92342=DIRECTION('center_axis',(0.981627005099017,0.,0.190809912898503));
#92343=DIRECTION('ref_axis',(0.,-1.,0.));
#92344=DIRECTION('',(-0.190809912898503,0.,0.981627005099017));
#92345=DIRECTION('center_axis',(0.981627005099017,1.45995862733013E-17,
0.190809912898504));
#92346=DIRECTION('ref_axis',(-0.190604886647506,0.046344966455992,0.98057224173963));
#92347=DIRECTION('',(-0.190809912898493,0.,0.981627005099019));
#92348=DIRECTION('center_axis',(0.981627005099017,-7.47937411885398E-18,
0.190809912898503));
#92349=DIRECTION('ref_axis',(-0.19061297638741,0.0454219277749919,0.980613859635859));
#92350=DIRECTION('center_axis',(0.,1.,0.));
#92351=DIRECTION('ref_axis',(1.,0.,0.));
#92352=DIRECTION('',(-0.190809912898503,0.,0.981627005099017));
#92353=DIRECTION('center_axis',(0.,1.,0.));
#92354=DIRECTION('ref_axis',(-0.426465074644572,0.,0.904504029901691));
#92355=DIRECTION('center_axis',(0.,1.,0.));
#92356=DIRECTION('ref_axis',(-0.422083537818967,0.,0.906556940904555));
#92357=DIRECTION('center_axis',(-0.981627005099017,0.,-0.190809912898503));
#92358=DIRECTION('ref_axis',(-0.190809912898503,0.,0.981627005099017));
#92359=DIRECTION('',(-0.190809912898503,0.,0.981627005099017));
#92360=DIRECTION('center_axis',(-0.981627005099017,-1.48303614829744E-18,
-0.190809912898503));
#92361=DIRECTION('ref_axis',(-0.190792919880392,0.0133456620116604,0.981539584035705));
#92362=DIRECTION('center_axis',(-0.981627005099017,-9.01652974182553E-18,
-0.190809912898504));
#92363=DIRECTION('ref_axis',(-0.190793600227308,0.01307578557334,0.981543084099696));
#92364=DIRECTION('center_axis',(0.,-1.,0.));
#92365=DIRECTION('ref_axis',(0.,0.,-1.));
#92366=DIRECTION('center_axis',(0.,-1.,0.));
#92367=DIRECTION('ref_axis',(-0.395956002292056,0.,0.918269483457277));
#92368=DIRECTION('center_axis',(0.,-1.,0.));
#92369=DIRECTION('ref_axis',(-0.3921344237022,0.,0.919907926777318));
#92370=DIRECTION('center_axis',(0.,-1.,0.));
#92371=DIRECTION('ref_axis',(0.,0.,-1.));
#92372=DIRECTION('',(-0.190809912898503,0.,0.981627005099017));
#92373=DIRECTION('center_axis',(0.,-1.,0.));
#92374=DIRECTION('ref_axis',(-0.396546255825506,0.,0.918014742251328));
#92375=DIRECTION('',(-0.190809912898503,0.,0.981627005099017));
#92376=DIRECTION('center_axis',(0.,-1.,0.));
#92377=DIRECTION('ref_axis',(-0.39269200471537,0.,0.919670043783434));
#92378=DIRECTION('center_axis',(0.981627005099017,0.,0.190809912898503));
#92379=DIRECTION('ref_axis',(0.,-1.,0.));
#92380=DIRECTION('',(-0.190809912898503,0.,0.981627005099017));
#92381=DIRECTION('center_axis',(0.981627005099017,1.01223798161555E-16,
0.190809912898504));
#92382=DIRECTION('ref_axis',(-0.18959747408221,0.112552061393099,0.975389579244011));
#92383=DIRECTION('center_axis',(0.981627005099017,1.4958748237708E-17,0.190809912898503));
#92384=DIRECTION('ref_axis',(-0.189645435508974,0.110310396025003,0.975636318163392));
#92385=DIRECTION('center_axis',(0.,1.,0.));
#92386=DIRECTION('ref_axis',(1.,0.,0.));
#92387=DIRECTION('',(-0.190809912898503,0.,0.981627005099017));
#92388=DIRECTION('center_axis',(0.,1.,0.));
#92389=DIRECTION('ref_axis',(-0.427628772377974,0.,0.903954441902083));
#92390=DIRECTION('center_axis',(0.,1.,0.));
#92391=DIRECTION('ref_axis',(-0.423182760142292,0.,0.906044343019894));
#92392=DIRECTION('center_axis',(-0.981627005099017,0.,-0.190809912898503));
#92393=DIRECTION('ref_axis',(-0.190809912898503,0.,0.981627005099017));
#92394=DIRECTION('center_axis',(-0.981627005099017,-6.12988274629607E-17,
-0.190809912898504));
#92395=DIRECTION('ref_axis',(-0.190197207765472,0.0800739720699311,0.978474926176017));
#92396=DIRECTION('center_axis',(-0.981627005099017,-3.41679021795494E-17,
-0.190809912898504));
#92397=DIRECTION('ref_axis',(-0.190221775423882,0.0784547134400175,0.978601315191039));
#92398=DIRECTION('center_axis',(0.,-1.,0.));
#92399=DIRECTION('ref_axis',(0.,0.,-1.));
#92400=DIRECTION('',(-0.190809912898503,0.,0.981627005099017));
#92401=DIRECTION('center_axis',(0.,-1.,0.));
#92402=DIRECTION('ref_axis',(-0.398001355800204,0.,0.917384826984401));
#92403=DIRECTION('',(-0.190809912898503,0.,0.981627005099017));
#92404=DIRECTION('center_axis',(0.,-1.,0.));
#92405=DIRECTION('ref_axis',(-0.394065783747253,0.,0.919082236842636));
#92406=DIRECTION('center_axis',(0.981627005099017,0.,0.190809912898503));
#92407=DIRECTION('ref_axis',(0.,-1.,0.));
#92408=DIRECTION('',(-0.190809912898503,0.,0.981627005099017));
#92409=DIRECTION('center_axis',(0.981627005099017,2.33593380372821E-17,
0.190809912898503));
#92410=DIRECTION('ref_axis',(-0.187736511312627,0.178759156330292,0.965815803529972));
#92411=DIRECTION('center_axis',(0.981627005099017,1.60806543555361E-16,
0.190809912898504));
#92412=DIRECTION('ref_axis',(-0.18785866856038,0.1751988642749,0.966444244953379));
#92413=DIRECTION('center_axis',(0.,1.,0.));
#92414=DIRECTION('ref_axis',(1.,0.,0.));
#92415=DIRECTION('',(-0.190809912898503,0.,0.981627005099017));
#92416=DIRECTION('center_axis',(0.,1.,0.));
#92417=DIRECTION('ref_axis',(-0.429808105205998,0.,0.902920258217319));
#92418=DIRECTION('center_axis',(0.,1.,0.));
#92419=DIRECTION('ref_axis',(-0.425239687746592,0.,0.905080774276628));
#92420=DIRECTION('center_axis',(-0.981627005099017,0.,-0.190809912898503));
#92421=DIRECTION('ref_axis',(-0.190809912898503,0.,0.981627005099017));
#92422=DIRECTION('center_axis',(-0.981627005099017,-1.18642891863795E-17,
-0.190809912898503));
#92423=DIRECTION('ref_axis',(-0.188742650756643,0.146802282128194,0.970991916417078));
#92424=DIRECTION('center_axis',(-0.981627005099017,-7.59286715101097E-18,
-0.190809912898503));
#92425=DIRECTION('ref_axis',(-0.188825848790083,0.1438336413067,0.971419931058222));
#92426=DIRECTION('center_axis',(0.,-1.,0.));
#92427=DIRECTION('ref_axis',(0.,0.,-1.));
#92428=DIRECTION('',(-0.190809912898503,0.,0.981627005099017));
#92429=DIRECTION('center_axis',(0.,-1.,0.));
#92430=DIRECTION('ref_axis',(-0.400377667961243,0.,0.916350218528875));
#92431=DIRECTION('',(-0.190809912898503,0.,0.981627005099017));
#92432=DIRECTION('center_axis',(0.,-1.,0.));
#92433=DIRECTION('ref_axis',(-0.396306902290058,0.,0.918118096541648));
#92434=DIRECTION('center_axis',(0.981627005099017,0.,0.190809912898503));
#92435=DIRECTION('ref_axis',(0.,-1.,0.));
#92436=DIRECTION('',(-0.190809912898503,0.,0.981627005099017));
#92437=DIRECTION('center_axis',(0.981627005099017,2.56952718410103E-16,
0.190809912898504));
#92438=DIRECTION('ref_axis',(-0.184996241362783,0.244966251267409,0.951718407104557));
#92439=DIRECTION('center_axis',(0.981627005099017,1.34628734139372E-16,
0.190809912898504));
#92440=DIRECTION('ref_axis',(-0.185228969653602,0.240087332524911,0.952915684392978));
#92441=DIRECTION('center_axis',(0.,1.,0.));
#92442=DIRECTION('ref_axis',(1.,0.,0.));
#92443=DIRECTION('',(-0.190809912898503,0.,0.981627005099017));
#92444=DIRECTION('center_axis',(0.,1.,0.));
#92445=DIRECTION('ref_axis',(-0.4330891117883,0.,0.901351108753088));
#92446=DIRECTION('center_axis',(0.,1.,0.));
#92447=DIRECTION('ref_axis',(-0.428332303170954,0.,0.903621291283171));
#92448=DIRECTION('center_axis',(-0.981627005099017,0.,-0.190809912898503));
#92449=DIRECTION('ref_axis',(-0.190809912898503,0.,0.981627005099017));
#92450=DIRECTION('center_axis',(-0.981627005099017,-3.1638104497012E-17,
-0.190809912898503));
#92451=DIRECTION('ref_axis',(-0.186409145148707,0.213530592186508,0.958987130677679));
#92452=DIRECTION('center_axis',(-0.981627005099017,3.79643357550549E-17,
-0.190809912898503));
#92453=DIRECTION('ref_axis',(-0.186587325039356,0.209212569173405,0.959903782175339));
#92454=DIRECTION('center_axis',(0.,-1.,0.));
#92455=DIRECTION('ref_axis',(0.,0.,-1.));
#92456=DIRECTION('',(-0.190809912898503,0.,0.981627005099017));
#92457=DIRECTION('center_axis',(0.,-1.,0.));
#92458=DIRECTION('ref_axis',(-0.403771969882212,0.,0.914859659367183));
#92459=DIRECTION('',(-0.190809912898503,0.,0.981627005099017));
#92460=DIRECTION('center_axis',(0.,-1.,0.));
#92461=DIRECTION('ref_axis',(-0.399502905152937,0.,0.916731928523472));
#92462=DIRECTION('center_axis',(0.981627005099017,0.,0.190809912898503));
#92463=DIRECTION('ref_axis',(0.,-1.,0.));
#92464=DIRECTION('',(-0.190809912898503,0.,0.981627005099017));
#92465=DIRECTION('center_axis',(0.981627005099017,1.40156028223692E-16,
0.190809912898504));
#92466=DIRECTION('ref_axis',(-0.181336805679145,0.311173346204495,0.932892336509408));
#92467=DIRECTION('center_axis',(0.981627005099017,8.22731153073938E-17,
0.190809912898504));
#92468=DIRECTION('ref_axis',(-0.181719747816134,0.304975800774901,0.934862393187013));
#92469=DIRECTION('center_axis',(0.,1.,0.));
#92470=DIRECTION('ref_axis',(1.,0.,0.));
#92471=DIRECTION('',(-0.190809912898503,0.,0.981627005099017));
#92472=DIRECTION('center_axis',(0.,1.,0.));
#92473=DIRECTION('ref_axis',(-0.437609570560575,0.,0.899165092601903));
#92474=DIRECTION('center_axis',(0.,1.,0.));
#92475=DIRECTION('ref_axis',(-0.432585020225244,0.,0.901593145646486));
#92476=DIRECTION('center_axis',(-0.981627005099017,0.,-0.190809912898503));
#92477=DIRECTION('ref_axis',(-0.190809912898503,0.,0.981627005099017));
#92478=DIRECTION('center_axis',(-0.981627005099017,-2.45195309851843E-16,
-0.190809912898504));
#92479=DIRECTION('ref_axis',(-0.183163100495339,0.280258902244805,0.942287761954633));
#92480=DIRECTION('center_axis',(-0.981627005099017,1.13893007265165E-16,
-0.190809912898503));
#92481=DIRECTION('ref_axis',(-0.183475365996515,0.274591497040088,0.943894220676093));
#92482=DIRECTION('center_axis',(0.,-1.,0.));
#92483=DIRECTION('ref_axis',(0.,0.,-1.));
#92484=DIRECTION('',(-0.190809912898503,0.,0.981627005099017));
#92485=DIRECTION('center_axis',(0.,-1.,0.));
#92486=DIRECTION('ref_axis',(-0.340256652364869,0.,0.940332606326853));
#92487=DIRECTION('',(-0.190809912898503,0.,0.981627005099017));
#92488=DIRECTION('center_axis',(0.,-1.,0.));
#92489=DIRECTION('ref_axis',(-0.337238794243498,0.,0.941419139202721));
#92490=DIRECTION('center_axis',(0.981627005099017,0.,0.190809912898503));
#92491=DIRECTION('ref_axis',(0.,-1.,0.));
#92492=DIRECTION('',(-0.190809912898503,0.,0.981627005099017));
#92493=DIRECTION('center_axis',(0.981627005099017,-7.5998920345386E-18,
0.190809912898503));
#92494=DIRECTION('ref_axis',(-0.181569549045125,0.307423075530589,0.934089691352422));
#92495=DIRECTION('center_axis',(0.981627005099017,7.30708136407185E-17,
0.190809912898503));
#92496=DIRECTION('ref_axis',(-0.181934257059101,0.301442666851091,0.935965942067368));
#92497=DIRECTION('center_axis',(0.,1.,0.));
#92498=DIRECTION('ref_axis',(1.,0.,0.));
#92499=DIRECTION('',(-0.190809912898503,0.,0.981627005099017));
#92500=DIRECTION('center_axis',(0.,1.,0.));
#92501=DIRECTION('ref_axis',(-0.37394254111531,0.,0.927451872575728));
#92502=DIRECTION('center_axis',(0.,1.,0.));
#92503=DIRECTION('ref_axis',(-0.370185230514857,0.,0.928957961970649));
#92504=DIRECTION('center_axis',(-0.981627005099017,0.,-0.190809912898503));
#92505=DIRECTION('ref_axis',(-0.190809912898503,0.,0.981627005099017));
#92506=DIRECTION('center_axis',(-0.981627005099017,-1.45990679982696E-16,
-0.190809912898504));
#92507=DIRECTION('ref_axis',(-0.183385828075594,0.276229431355416,0.943433590304104));
#92508=DIRECTION('center_axis',(-0.981627005099017,-1.03383578960841E-16,
-0.190809912898504));
#92509=DIRECTION('ref_axis',(-0.183680511877257,0.270798308728604,0.944949599474087));
#92510=DIRECTION('center_axis',(0.,-1.,0.));
#92511=DIRECTION('ref_axis',(0.,0.,-1.));
#92512=DIRECTION('',(-0.190809912898503,0.,0.981627005099017));
#92513=DIRECTION('center_axis',(0.,-1.,0.));
#92514=DIRECTION('ref_axis',(-0.275846435585838,0.,0.961201718670222));
#92515=DIRECTION('',(-0.190809912898503,1.132361187045E-14,0.981627005099017));
#92516=DIRECTION('center_axis',(0.,-1.,0.));
#92517=DIRECTION('ref_axis',(-0.274117437734562,0.,0.961696225598208));
#92518=DIRECTION('center_axis',(0.981627005099017,0.,0.190809912898503));
#92519=DIRECTION('ref_axis',(0.,-1.,0.));
#92520=DIRECTION('',(-0.190809912898503,0.,0.981627005099017));
#92521=DIRECTION('center_axis',(0.981627005099017,3.74230666600009E-17,
0.190809912898503));
#92522=DIRECTION('ref_axis',(-0.181713220883714,0.305082598047195,0.934828815198184));
#92523=DIRECTION('center_axis',(0.981627005099017,-9.36058786041334E-17,
0.190809912898503));
#92524=DIRECTION('ref_axis',(-0.182066886709518,0.299235170990892,0.93664825906311));
#92525=DIRECTION('center_axis',(0.,1.,0.));
#92526=DIRECTION('ref_axis',(1.,0.,0.));
#92527=DIRECTION('',(-0.190809912898503,0.,0.981627005099017));
#92528=DIRECTION('center_axis',(0.,1.,0.));
#92529=DIRECTION('ref_axis',(-0.309344683605792,0.,0.950949981189774));
#92530=DIRECTION('center_axis',(0.,1.,0.));
#92531=DIRECTION('ref_axis',(-0.306895274081955,0.,0.951743290360464));
#92532=DIRECTION('center_axis',(-0.981627005099017,0.,-0.190809912898503));
#92533=DIRECTION('ref_axis',(-0.190809912898503,0.,0.981627005099017));
#92534=DIRECTION('center_axis',(-0.981627005099017,-9.04057881831701E-17,
-0.190809912898504));
#92535=DIRECTION('ref_axis',(-0.183533539382005,0.273521632312099,0.944193495306571));
#92536=DIRECTION('center_axis',(-0.981627005099017,-1.95641407952151E-16,
-0.190809912898504));
#92537=DIRECTION('ref_axis',(-0.18381683332523,0.268245652420898,0.945650909026989));
#92538=DIRECTION('center_axis',(0.,-1.,0.));
#92539=DIRECTION('ref_axis',(0.,0.,-1.));
#92540=DIRECTION('',(-0.190809912898503,0.,0.981627005099017));
#92541=DIRECTION('center_axis',(0.,-1.,0.));
#92542=DIRECTION('ref_axis',(-0.210563327934167,0.,0.977580219178605));
#92543=DIRECTION('',(-0.190809912898503,0.,0.981627005099017));
#92544=DIRECTION('center_axis',(0.,-1.,0.));
#92545=DIRECTION('ref_axis',(-0.210159055405375,0.,0.977667208937234));
#92546=DIRECTION('center_axis',(0.981627005099017,0.,0.190809912898503));
#92547=DIRECTION('ref_axis',(0.,-1.,0.));
#92548=DIRECTION('',(-0.190809912898503,0.,0.981627005099017));
#92549=DIRECTION('center_axis',(0.981627005099017,2.60207268814641E-16,
0.190809912898504));
#92550=DIRECTION('ref_axis',(-0.181775649940103,0.304059405247896,0.935149983248222));
#92551=DIRECTION('center_axis',(0.981627005099017,3.43394588839726E-16,
0.190809912898504));
#92552=DIRECTION('ref_axis',(-0.182124568584603,0.298269507204199,0.936945005104375));
#92553=DIRECTION('center_axis',(0.,1.,0.));
#92554=DIRECTION('ref_axis',(1.,0.,0.));
#92555=DIRECTION('',(-0.190809912898503,0.,0.981627005099017));
#92556=DIRECTION('center_axis',(0.,1.,0.));
#92557=DIRECTION('ref_axis',(-0.24384603732277,0.,0.969813956427717));
#92558=DIRECTION('center_axis',(0.,1.,0.));
#92559=DIRECTION('ref_axis',(-0.242742672216863,0.,0.970090714874138));
#92560=DIRECTION('center_axis',(-0.981627005099017,0.,-0.190809912898503));
#92561=DIRECTION('ref_axis',(-0.190809912898503,0.,0.981627005099017));
#92562=DIRECTION('center_axis',(-0.981627005099017,-5.96131698931744E-17,
-0.190809912898504));
#92563=DIRECTION('ref_axis',(-0.183614456317799,0.272025926757612,0.94460977477622));
#92564=DIRECTION('center_axis',(-0.981627005099017,-7.88692931673802E-17,
-0.190809912898504));
#92565=DIRECTION('ref_axis',(-0.183891602408533,0.266834398951196,0.94603556069525));
#92566=DIRECTION('center_axis',(0.,-1.,0.));
#92567=DIRECTION('ref_axis',(0.,0.,-1.));
#92568=DIRECTION('',(-0.190809912898503,0.,0.981627005099017));
#92569=DIRECTION('center_axis',(0.,-1.,0.));
#92570=DIRECTION('ref_axis',(-0.144416822146308,0.,0.98951694350383));
#92571=DIRECTION('',(-0.190809912898503,0.,0.981627005099017));
#92572=DIRECTION('center_axis',(0.,-1.,0.));
#92573=DIRECTION('ref_axis',(-0.14537237934921,0.,0.989377011721189));
#92574=DIRECTION('center_axis',(0.981627005099017,0.,0.190809912898503));
#92575=DIRECTION('ref_axis',(0.,-1.,0.));
#92576=DIRECTION('',(-0.190809912898503,0.,0.981627005099017));
#92577=DIRECTION('center_axis',(0.981627005099017,-1.19151365507148E-16,
0.190809912898503));
#92578=DIRECTION('ref_axis',(-0.181760123195241,0.304314238039989,0.935070105469206));
#92579=DIRECTION('center_axis',(0.981627005099017,7.16559735129159E-18,
0.190809912898503));
#92580=DIRECTION('ref_axis',(-0.182110219627529,0.298510046456984,0.936871186488016));
#92581=DIRECTION('center_axis',(0.,1.,0.));
#92582=DIRECTION('ref_axis',(1.,0.,0.));
#92583=DIRECTION('',(-0.190809912898503,0.,0.981627005099017));
#92584=DIRECTION('center_axis',(0.,1.,0.));
#92585=DIRECTION('ref_axis',(-0.177462871614912,0.,0.984127496414052));
#92586=DIRECTION('center_axis',(0.,1.,0.));
#92587=DIRECTION('ref_axis',(-0.177742357598668,0.,0.984077057102373));
#92588=DIRECTION('center_axis',(-0.981627005099017,0.,-0.190809912898503));
#92589=DIRECTION('ref_axis',(-0.190809912898503,0.,0.981627005099017));
#92590=DIRECTION('center_axis',(-0.981627005099017,-1.0406113144537E-16,
-0.190809912898504));
#92591=DIRECTION('ref_axis',(-0.183632874440486,0.271684234850208,0.944704527330414));
#92592=DIRECTION('center_axis',(-0.981627005099017,-1.43052272430736E-16,
-0.190809912898504));
#92593=DIRECTION('ref_axis',(-0.183908630238396,0.266511876338901,0.946123160848605));
#92594=DIRECTION('center_axis',(0.,-1.,0.));
#92595=DIRECTION('ref_axis',(0.,0.,-1.));
#92596=DIRECTION('',(-0.190809912898503,0.,0.981627005099017));
#92597=DIRECTION('center_axis',(0.,-1.,0.));
#92598=DIRECTION('ref_axis',(-0.0774045612714574,0.,0.996999766245897));
#92599=DIRECTION('',(-0.190809912898503,0.,0.981627005099017));
#92600=DIRECTION('center_axis',(0.,-1.,0.));
#92601=DIRECTION('ref_axis',(-0.0797552408636643,0.,0.996814476998995));
#92602=DIRECTION('center_axis',(0.981627005099017,0.,0.190809912898503));
#92603=DIRECTION('ref_axis',(0.,-1.,0.));
#92604=DIRECTION('',(-0.190809912898503,0.,0.981627005099017));
#92605=DIRECTION('center_axis',(0.981627005099017,0.,0.190809912898503));
#92606=DIRECTION('ref_axis',(-0.181665829576745,0.305856807673619,0.934585009276254));
#92607=DIRECTION('center_axis',(0.981627005099017,5.06495345173922E-17,
0.190809912898503));
#92608=DIRECTION('ref_axis',(-0.182023119703858,0.299965605628596,0.936423098461985));
#92609=DIRECTION('center_axis',(0.,1.,0.));
#92610=DIRECTION('ref_axis',(1.,0.,0.));
#92611=DIRECTION('',(-0.190809912898503,0.,0.981627005099017));
#92612=DIRECTION('center_axis',(0.,1.,0.));
#92613=DIRECTION('ref_axis',(-0.110198871269438,0.,0.993909557641409));
#92614=DIRECTION('center_axis',(0.,1.,0.));
#92615=DIRECTION('ref_axis',(-0.111897714940647,0.,0.99371972979863));
#92616=DIRECTION('center_axis',(-0.981627005099017,0.,-0.190809912898503));
#92617=DIRECTION('ref_axis',(-0.190809912898503,0.,0.981627005099017));
#92618=DIRECTION('center_axis',(-0.981627005099017,-2.0187191501672E-16,
-0.190809912898504));
#92619=DIRECTION('ref_axis',(-0.183589751211426,0.272483527884585,0.944482678656256));
#92620=DIRECTION('center_axis',(-0.981627005099017,-2.87726513572186E-16,
-0.190809912898504));
#92621=DIRECTION('ref_axis',(-0.183868767449469,0.267266256174104,0.945918085601122));
#92622=DIRECTION('center_axis',(0.,-1.,0.));
#92623=DIRECTION('ref_axis',(0.,0.,-1.));
#92624=DIRECTION('',(-0.190809912898503,0.,0.981627005099017));
#92625=DIRECTION('center_axis',(0.,-1.,0.));
#92626=DIRECTION('ref_axis',(-0.00951217486443362,0.,0.999954758241266));
#92627=DIRECTION('',(-0.190809912898503,0.,0.981627005099017));
#92628=DIRECTION('center_axis',(0.,-1.,0.));
#92629=DIRECTION('ref_axis',(-0.0132944259954453,0.,0.999911625213674));
#92630=DIRECTION('center_axis',(0.981627005099017,0.,0.190809912898503));
#92631=DIRECTION('ref_axis',(0.,-1.,0.));
#92632=DIRECTION('',(-0.190809912898503,0.,0.981627005099017));
#92633=DIRECTION('center_axis',(0.981627005099017,1.30313218010573E-16,
0.190809912898504));
#92634=DIRECTION('ref_axis',(-0.181487751748704,0.308746843185004,0.933668882842571));
#92635=DIRECTION('center_axis',(0.981627005099017,3.38914002557394E-16,
0.190809912898504));
#92636=DIRECTION('ref_axis',(-0.181858819374924,0.302690361553391,0.935577850762958));
#92637=DIRECTION('center_axis',(0.,1.,0.));
#92638=DIRECTION('ref_axis',(1.,0.,0.));
#92639=DIRECTION('',(-0.190809912898503,0.,0.981627005099017));
#92640=DIRECTION('center_axis',(0.,1.,0.));
#92641=DIRECTION('ref_axis',(-0.0420453982044825,0.,0.999115701252776));
#92642=DIRECTION('center_axis',(0.,1.,0.));
#92643=DIRECTION('ref_axis',(-0.0452008111636282,0.,0.998977921012347));
#92644=DIRECTION('center_axis',(-0.981627005099017,0.,-0.190809912898503));
#92645=DIRECTION('ref_axis',(-0.190809912898503,0.,0.981627005099017));
#92646=DIRECTION('center_axis',(-0.981627005099017,-6.82675953385116E-17,
-0.190809912898503));
#92647=DIRECTION('ref_axis',(-0.183482833113299,0.274454421803195,0.943932635470027));
#92648=DIRECTION('center_axis',(-0.981627005099017,0.,-0.190809912898503));
#92649=DIRECTION('ref_axis',(-0.183770012633108,0.269125326340587,0.945410038649315));
#92650=DIRECTION('center_axis',(0.,-1.,0.));
#92651=DIRECTION('ref_axis',(0.,0.,-1.));
#92652=DIRECTION('',(-0.190809912898503,0.,0.981627005099017));
#92653=DIRECTION('center_axis',(0.,-1.,0.));
#92654=DIRECTION('ref_axis',(0.0592877418835069,0.,0.99824093467577));
#92655=DIRECTION('',(-0.190809912898503,0.,0.981627005099017));
#92656=DIRECTION('center_axis',(0.,-1.,0.));
#92657=DIRECTION('ref_axis',(0.0540352232974096,0.,0.998539030105083));
#92658=DIRECTION('center_axis',(0.981627005099017,0.,0.190809912898503));
#92659=DIRECTION('ref_axis',(0.,-1.,0.));
#92660=DIRECTION('',(-0.190809912898503,0.,0.981627005099017));
#92661=DIRECTION('center_axis',(0.981627005099017,3.46860807619102E-16,
0.190809912898504));
#92662=DIRECTION('ref_axis',(-0.181215978183,0.313100693055305,0.93227073603083));
#92663=DIRECTION('center_axis',(0.981627005099017,3.55724373777378E-16,
0.190809912898504));
#92664=DIRECTION('ref_axis',(-0.181608554935483,0.306789600923706,0.93429035826092));
#92665=DIRECTION('center_axis',(0.,1.,0.));
#92666=DIRECTION('ref_axis',(1.,0.,0.));
#92667=DIRECTION('',(-0.190809912898503,0.,0.981627005099017));
#92668=DIRECTION('center_axis',(0.,1.,0.));
#92669=DIRECTION('ref_axis',(0.0270191259379464,0.,0.999634916773894));
#92670=DIRECTION('center_axis',(0.,1.,0.));
#92671=DIRECTION('ref_axis',(0.0223681473937496,0.,0.999749801691489));
#92672=DIRECTION('center_axis',(-0.981627005099017,0.,-0.190809912898503));
#92673=DIRECTION('ref_axis',(-0.190809912898503,0.,0.981627005099017));
#92674=DIRECTION('center_axis',(-0.981627005099017,-3.88216196345816E-17,
-0.190809912898503));
#92675=DIRECTION('ref_axis',(-0.183306354127305,0.277674505471101,0.943024734324575));
#92676=DIRECTION('center_axis',(-0.981627005099017,-1.19343362969677E-16,
-0.190809912898504));
#92677=DIRECTION('ref_axis',(-0.183607255301246,0.272159393626116,0.944572728942461));
#92678=DIRECTION('center_axis',(0.,-1.,0.));
#92679=DIRECTION('ref_axis',(0.,0.,-1.));
#92680=DIRECTION('',(-0.190809912898503,0.,0.981627005099017));
#92681=DIRECTION('center_axis',(0.,-1.,0.));
#92682=DIRECTION('ref_axis',(0.129037681608313,0.,0.991639690979114));
#92683=DIRECTION('',(-0.190809912898493,0.,0.981627005099019));
#92684=DIRECTION('center_axis',(0.,-1.,0.));
#92685=DIRECTION('ref_axis',(0.122272610118709,0.,0.992496553553088));
#92686=DIRECTION('center_axis',(0.981627005099017,0.,0.190809912898503));
#92687=DIRECTION('ref_axis',(0.,-1.,0.));
#92688=DIRECTION('',(-0.190809912898503,0.,0.981627005099017));
#92689=DIRECTION('center_axis',(0.981627005099017,-8.1884484692467E-18,
0.190809912898503));
#92690=DIRECTION('ref_axis',(-0.180834252140125,0.319104965266087,0.93030693558387));
#92691=DIRECTION('center_axis',(0.981627005099017,7.84954079410769E-18,
0.190809912898503));
#92692=DIRECTION('ref_axis',(-0.181258021464907,0.312431545483989,0.932487028886254));
#92693=DIRECTION('center_axis',(0.,1.,0.));
#92694=DIRECTION('ref_axis',(1.,0.,0.));
#92695=DIRECTION('',(-0.190809912898503,0.,0.981627005099017));
#92696=DIRECTION('center_axis',(0.,1.,0.));
#92697=DIRECTION('ref_axis',(0.0970308224791404,0.,0.995281377043207));
#92698=DIRECTION('center_axis',(0.,1.,0.));
#92699=DIRECTION('ref_axis',(0.0908422199685957,0.,0.995865297653843));
#92700=DIRECTION('center_axis',(-0.981627005099017,0.,-0.190809912898503));
#92701=DIRECTION('ref_axis',(-0.190809912898503,0.,0.981627005099017));
#92702=DIRECTION('center_axis',(-0.981627005099017,-4.81431257853459E-17,
-0.190809912898503));
#92703=DIRECTION('ref_axis',(-0.183050227681134,0.28227713515299,0.941707084562767));
#92704=DIRECTION('center_axis',(-0.981627005099017,9.23779601860268E-17,
-0.190809912898503));
#92705=DIRECTION('ref_axis',(-0.183371589738963,0.2764889283937,0.943360340777748));
#92706=DIRECTION('center_axis',(0.,-1.,0.));
#92707=DIRECTION('ref_axis',(0.,0.,-1.));
#92708=DIRECTION('',(-0.190809912898503,0.,0.981627005099017));
#92709=DIRECTION('center_axis',(0.,-1.,0.));
#92710=DIRECTION('ref_axis',(0.123657514606589,0.,0.99232495639348));
#92711=DIRECTION('',(-0.190809912898503,0.,0.981627005099017));
#92712=DIRECTION('center_axis',(0.,-1.,0.));
#92713=DIRECTION('ref_axis',(0.117218477629797,0.,0.993106151678738));
#92714=DIRECTION('center_axis',(0.981627005099017,0.,0.190809912898503));
#92715=DIRECTION('ref_axis',(0.,-1.,0.));
#92716=DIRECTION('',(-0.190809912898503,0.,0.981627005099017));
#92717=DIRECTION('center_axis',(0.981627005099017,1.228267270387E-16,0.190809912898504));
#92718=DIRECTION('ref_axis',(-0.184691122397272,0.251210291805195,0.950148713938394));
#92719=DIRECTION('center_axis',(0.981627005099017,1.56990815882154E-16,
0.190809912898504));
#92720=DIRECTION('ref_axis',(-0.184948385867005,0.245956748572503,0.951472213150144));
#92721=DIRECTION('center_axis',(0.,1.,0.));
#92722=DIRECTION('ref_axis',(1.,0.,0.));
#92723=DIRECTION('',(-0.190809912898503,0.,0.981627005099017));
#92724=DIRECTION('center_axis',(0.,1.,0.));
#92725=DIRECTION('ref_axis',(0.0914624082264752,0.,0.995808529729191));
#92726=DIRECTION('center_axis',(0.,1.,0.));
#92727=DIRECTION('ref_axis',(0.0856161376277009,0.,0.996328197421771));
#92728=DIRECTION('center_axis',(-0.981627005099017,0.,-0.190809912898503));
#92729=DIRECTION('ref_axis',(-0.190809912898503,0.,0.981627005099017));
#92730=DIRECTION('center_axis',(-0.981627005099017,-2.32691774629172E-16,
-0.190809912898504));
#92731=DIRECTION('ref_axis',(-0.186344772310312,0.215068293449893,0.958655962786008));
#92732=DIRECTION('center_axis',(-0.981627005099017,-1.00076123534862E-16,
-0.190809912898504));
#92733=DIRECTION('ref_axis',(-0.186528095125347,0.210658231157109,0.959599072203943));
#92734=DIRECTION('center_axis',(0.,-1.,0.));
#92735=DIRECTION('ref_axis',(0.,0.,-1.));
#92736=DIRECTION('',(-0.190809912898503,0.,0.981627005099017));
#92737=DIRECTION('center_axis',(0.,-1.,0.));
#92738=DIRECTION('ref_axis',(0.119896958150858,0.,0.992786341277));
#92739=DIRECTION('',(-0.190809912898503,0.,0.981627005099017));
#92740=DIRECTION('center_axis',(0.,-1.,0.));
#92741=DIRECTION('ref_axis',(0.113679714473517,0.,0.993517449528301));
#92742=DIRECTION('center_axis',(0.981627005099017,0.,0.190809912898503));
#92743=DIRECTION('ref_axis',(0.,-1.,0.));
#92744=DIRECTION('',(-0.190809912898503,0.,0.981627005099017));
#92745=DIRECTION('center_axis',(0.981627005099017,1.51486296681064E-16,
0.190809912898504));
#92746=DIRECTION('ref_axis',(-0.187576469189326,0.183315618344298,0.964992462290516));
#92747=DIRECTION('center_axis',(0.981627005099017,1.33442193499831E-16,
0.190809912898504));
#92748=DIRECTION('ref_axis',(-0.187711401531336,0.179481951661004,0.965686625548422));
#92749=DIRECTION('center_axis',(0.,1.,0.));
#92750=DIRECTION('ref_axis',(1.,0.,0.));
#92751=DIRECTION('',(-0.190809912898503,0.,0.981627005099017));
#92752=DIRECTION('center_axis',(0.,1.,0.));
#92753=DIRECTION('ref_axis',(0.0874284944613751,0.,0.9961707977833));
#92754=DIRECTION('center_axis',(0.,1.,0.));
#92755=DIRECTION('ref_axis',(0.0818224711015746,0.,0.996646920038803));
#92756=DIRECTION('center_axis',(-0.981627005099017,0.,-0.190809912898503));
#92757=DIRECTION('ref_axis',(-0.190809912898503,0.,0.981627005099017));
#92758=DIRECTION('center_axis',(-0.981627005099017,-8.42504701243554E-17,
-0.190809912898504));
#92759=DIRECTION('ref_axis',(-0.188712603501478,0.147859451746807,0.970837337461239));
#92760=DIRECTION('center_axis',(-0.981627005099017,-1.07774286883698E-16,
-0.190809912898504));
#92761=DIRECTION('ref_axis',(-0.188798187650067,0.144827533920497,0.971277627539396));
#92762=DIRECTION('center_axis',(0.,-1.,0.));
#92763=DIRECTION('ref_axis',(0.,0.,-1.));
#92764=DIRECTION('',(-0.190809912898503,0.,0.981627005099017));
#92765=DIRECTION('center_axis',(0.,-1.,0.));
#92766=DIRECTION('ref_axis',(0.117596679694482,0.,0.993061438645582));
#92767=DIRECTION('',(-0.190809912898503,0.,0.981627005099017));
#92768=DIRECTION('center_axis',(0.,-1.,0.));
#92769=DIRECTION('ref_axis',(0.111512654940727,0.,0.993763013896206));
#92770=DIRECTION('center_axis',(0.981627005099017,0.,0.190809912898503));
#92771=DIRECTION('ref_axis',(0.,-1.,0.));
#92772=DIRECTION('',(-0.190809912898492,0.,0.981627005099019));
#92773=DIRECTION('center_axis',(0.981627005099017,3.27537938769868E-17,
0.190809912898504));
#92774=DIRECTION('ref_axis',(-0.189534667147167,0.115420944883498,0.975066467186526));
#92775=DIRECTION('center_axis',(0.981627005099017,3.92477039705384E-17,
0.190809912898504));
#92776=DIRECTION('ref_axis',(-0.189587617832801,0.113007154749503,0.975338873489571));
#92777=DIRECTION('center_axis',(0.,1.,0.));
#92778=DIRECTION('ref_axis',(1.,0.,0.));
#92779=DIRECTION('',(-0.190809912898503,0.,0.981627005099017));
#92780=DIRECTION('center_axis',(0.,1.,0.));
#92781=DIRECTION('ref_axis',(0.0847526256525639,0.,0.996402023505069));
#92782=DIRECTION('center_axis',(0.,1.,0.));
#92783=DIRECTION('ref_axis',(0.0793024169710135,0.,0.996850603983644));
#92784=DIRECTION('center_axis',(-0.981627005099017,0.,-0.190809912898503));
#92785=DIRECTION('ref_axis',(-0.190809912898503,0.,0.981627005099017));
#92786=DIRECTION('center_axis',(-0.981627005099017,2.00596357438942E-17,
-0.190809912898503));
#92787=DIRECTION('ref_axis',(-0.190188336952842,0.0806506100437121,0.978429290029019));
#92788=DIRECTION('center_axis',(-0.981627005099017,-9.62270418604446E-18,
-0.190809912898503));
#92789=DIRECTION('ref_axis',(-0.190213606479589,0.0789968366839196,0.97855928982559));
#92790=DIRECTION('center_axis',(0.,-1.,0.));
#92791=DIRECTION('ref_axis',(0.,0.,-1.));
#92792=DIRECTION('',(-0.190809912898503,0.,0.981627005099017));
#92793=DIRECTION('center_axis',(0.,-1.,0.));
#92794=DIRECTION('ref_axis',(0.116664111632625,0.,0.993171427829542));
#92795=DIRECTION('',(-0.190809912898503,0.,0.981627005099017));
#92796=DIRECTION('center_axis',(0.,-1.,0.));
#92797=DIRECTION('ref_axis',(0.110633569332503,0.,0.993861264632419));
#92798=DIRECTION('center_axis',(0.981627005099017,0.,0.190809912898503));
#92799=DIRECTION('ref_axis',(0.,-1.,0.));
#92800=DIRECTION('',(-0.190809912898503,0.,0.981627005099017));
#92801=DIRECTION('center_axis',(0.981627005099017,1.12591166452142E-17,
0.190809912898504));
#92802=DIRECTION('ref_axis',(-0.190594295464282,0.0475262714226105,0.980517755097346));
#92803=DIRECTION('center_axis',(0.981627005099017,-2.551100758085E-17,0.190809912898503));
#92804=DIRECTION('ref_axis',(-0.190603224387164,0.0465323578380378,0.980563690194191));
#92805=DIRECTION('center_axis',(0.,1.,0.));
#92806=DIRECTION('ref_axis',(1.,0.,0.));
#92807=DIRECTION('',(-0.190809912898503,0.,0.981627005099017));
#92808=DIRECTION('center_axis',(0.,1.,0.));
#92809=DIRECTION('ref_axis',(0.083324953951956,0.,0.99652242927538));
#92810=DIRECTION('center_axis',(0.,1.,0.));
#92811=DIRECTION('ref_axis',(0.0779567276864901,0.,0.996956743599447));
#92812=DIRECTION('center_axis',(-0.981627005099017,0.,-0.190809912898503));
#92813=DIRECTION('ref_axis',(-0.190809912898503,0.,0.981627005099017));
#92814=DIRECTION('center_axis',(-0.981627005099017,-2.50745446798676E-18,
-0.190809912898504));
#92815=DIRECTION('ref_axis',(-0.19079267424387,0.0134417683406195,0.981538320351656));
#92816=DIRECTION('center_axis',(-0.981627005099017,-9.62270418604446E-19,
-0.190809912898503));
#92817=DIRECTION('ref_axis',(-0.190793373996996,0.0131661394473206,0.981541920251446));
#92818=DIRECTION('center_axis',(0.,-1.,0.));
#92819=DIRECTION('ref_axis',(0.,0.,-1.));
#92820=DIRECTION('',(-0.190809912898515,0.,0.981627005099015));
#92821=DIRECTION('center_axis',(0.,-1.,0.));
#92822=DIRECTION('ref_axis',(-0.334732212895843,0.,0.942313294849358));
#92823=DIRECTION('',(-0.190809912898516,0.,0.981627005099015));
#92824=DIRECTION('center_axis',(0.,-1.,0.));
#92825=DIRECTION('ref_axis',(-0.332032295999667,0.,0.943268018334762));
#92826=DIRECTION('center_axis',(0.981627005099017,0.,0.190809912898503));
#92827=DIRECTION('ref_axis',(0.,-1.,0.));
#92828=DIRECTION('',(-0.190809912898503,0.,0.981627005099017));
#92829=DIRECTION('center_axis',(0.981627005099017,1.51997840690772E-17,
0.190809912898504));
#92830=DIRECTION('ref_axis',(-0.190609801410987,0.0457864155045494,0.980597525879659));
#92831=DIRECTION('center_axis',(0.981627005099017,2.74015551152694E-17,
0.190809912898504));
#92832=DIRECTION('ref_axis',(-0.190617515250888,0.0448957163395215,0.980637209947664));
#92833=DIRECTION('center_axis',(0.,1.,0.));
#92834=DIRECTION('ref_axis',(1.,0.,0.));
#92835=DIRECTION('',(-0.190809912898503,0.,0.981627005099017));
#92836=DIRECTION('center_axis',(0.,1.,0.));
#92837=DIRECTION('ref_axis',(-0.365610687831021,0.,0.930767868452563));
#92838=DIRECTION('center_axis',(0.,1.,0.));
#92839=DIRECTION('ref_axis',(-0.362336833871464,0.,0.932047219200832));
#92840=DIRECTION('center_axis',(-0.981627005099017,0.,-0.190809912898503));
#92841=DIRECTION('ref_axis',(-0.190809912898503,0.,0.981627005099017));
#92842=DIRECTION('center_axis',(-0.981627005099017,9.60464999886156E-19,
-0.190809912898503));
#92843=DIRECTION('ref_axis',(-0.190793405028745,0.0131537824454998,0.981542079895159));
#92844=DIRECTION('center_axis',(-0.981627005099017,-6.46147368505259E-18,
-0.190809912898504));
#92845=DIRECTION('ref_axis',(-0.190794047817322,0.0128951575585105,0.981545386739209));
#92846=DIRECTION('center_axis',(0.,-1.,0.));
#92847=DIRECTION('ref_axis',(0.,0.,-1.));
#92848=DIRECTION('',(-0.190809912898503,0.,0.981627005099017));
#92849=DIRECTION('center_axis',(0.,-1.,0.));
#92850=DIRECTION('ref_axis',(-0.335149294303462,0.,0.942165033594376));
#92851=DIRECTION('',(-0.190809912898503,0.,0.981627005099017));
#92852=DIRECTION('center_axis',(0.,-1.,0.));
#92853=DIRECTION('ref_axis',(-0.332426172894225,0.,0.943129280414355));
#92854=DIRECTION('center_axis',(0.981627005099017,0.,0.190809912898503));
#92855=DIRECTION('ref_axis',(0.,-1.,0.));
#92856=DIRECTION('',(-0.190809912898503,0.,0.981627005099017));
#92857=DIRECTION('center_axis',(0.981627005099017,7.5998920345386E-18,0.190809912898503));
#92858=DIRECTION('ref_axis',(-0.189626613313853,0.111195580511101,0.975539486847107));
#92859=DIRECTION('center_axis',(0.981627005099017,1.82677034101797E-17,
0.190809912898503));
#92860=DIRECTION('ref_axis',(-0.189672340528791,0.109032453967399,0.975774731800418));
#92861=DIRECTION('center_axis',(0.,1.,0.));
#92862=DIRECTION('ref_axis',(1.,0.,0.));
#92863=DIRECTION('',(-0.190809912898503,0.,0.981627005099017));
#92864=DIRECTION('center_axis',(0.,1.,0.));
#92865=DIRECTION('ref_axis',(-0.366480370880962,0.,0.930425783047177));
#92866=DIRECTION('center_axis',(0.,1.,0.));
#92867=DIRECTION('ref_axis',(-0.363158067036044,0.,0.931727545126065));
#92868=DIRECTION('center_axis',(-0.981627005099017,0.,-0.190809912898503));
#92869=DIRECTION('ref_axis',(-0.190809912898503,0.,0.981627005099017));
#92870=DIRECTION('center_axis',(-0.981627005099017,-3.45767399959016E-17,
-0.190809912898504));
#92871=DIRECTION('ref_axis',(-0.190214727024376,0.0789226946729824,0.978565054500005));
#92872=DIRECTION('center_axis',(-0.981627005099017,-5.53840601575937E-17,
-0.190809912898504));
#92873=DIRECTION('ref_axis',(-0.19023793643477,0.0773709453510314,0.978684455969608));
#92874=DIRECTION('center_axis',(0.,-1.,0.));
#92875=DIRECTION('ref_axis',(0.,0.,-1.));
#92876=DIRECTION('',(-0.190809912898493,0.,0.981627005099019));
#92877=DIRECTION('center_axis',(0.,-1.,0.));
#92878=DIRECTION('ref_axis',(-0.336177570564712,0.,0.941798620220484));
#92879=DIRECTION('',(-0.190809912898503,0.,0.981627005099017));
#92880=DIRECTION('center_axis',(0.,-1.,0.));
#92881=DIRECTION('ref_axis',(-0.333396687233972,0.,0.942786640200959));
#92882=DIRECTION('center_axis',(0.981627005099017,0.,0.190809912898503));
#92883=DIRECTION('ref_axis',(0.,-1.,0.));
#92884=DIRECTION('',(-0.190809912898503,0.,0.981627005099017));
#92885=DIRECTION('center_axis',(0.981627005099017,4.17994061899623E-17,
0.190809912898504));
#92886=DIRECTION('ref_axis',(-0.187810734417079,0.176604745517606,0.966197646394556));
#92887=DIRECTION('center_axis',(0.981627005099017,1.13259761143114E-16,
0.190809912898504));
#92888=DIRECTION('ref_axis',(-0.187927174114397,0.173169191595305,0.966796673717698));
#92889=DIRECTION('center_axis',(0.,1.,0.));
#92890=DIRECTION('ref_axis',(1.,0.,0.));
#92891=DIRECTION('',(-0.190809912898503,-1.576961924456E-14,0.981627005099017));
#92892=DIRECTION('center_axis',(0.,1.,0.));
#92893=DIRECTION('ref_axis',(-0.36810928335472,0.,0.929782531298623));
#92894=DIRECTION('center_axis',(0.,1.,0.));
#92895=DIRECTION('ref_axis',(-0.364694981855002,0.,0.931127043002071));
#92896=DIRECTION('center_axis',(-0.981627005099017,0.,-0.190809912898503));
#92897=DIRECTION('ref_axis',(-0.190809912898503,0.,0.981627005099017));
#92898=DIRECTION('center_axis',(-0.981627005099017,-3.84185999954462E-17,
-0.190809912898504));
#92899=DIRECTION('ref_axis',(-0.188801982134388,0.144691606900499,0.971297148371536));
#92900=DIRECTION('center_axis',(-0.981627005099017,-3.69227067717291E-18,
-0.190809912898503));
#92901=DIRECTION('ref_axis',(-0.188880563702572,0.141846733143594,0.971701413476325));
#92902=DIRECTION('center_axis',(0.,-1.,0.));
#92903=DIRECTION('ref_axis',(0.,0.,-1.));
#92904=DIRECTION('',(-0.190809912898503,0.,0.981627005099017));
#92905=DIRECTION('center_axis',(0.,-1.,0.));
#92906=DIRECTION('ref_axis',(-0.337857092755181,0.,0.941197420775799));
#92907=DIRECTION('',(-0.190809912898503,-1.139455022803E-14,0.981627005099017));
#92908=DIRECTION('center_axis',(0.,-1.,0.));
#92909=DIRECTION('ref_axis',(-0.334980161426978,0.,0.942225180861961));
#92910=DIRECTION('center_axis',(0.981627005099017,0.,0.190809912898503));
#92911=DIRECTION('ref_axis',(0.,-1.,0.));
#92912=DIRECTION('',(-0.190809912898503,0.,0.981627005099017));
#92913=DIRECTION('center_axis',(0.981627005099017,2.65996221208851E-16,
0.190809912898504));
#92914=DIRECTION('ref_axis',(-0.18513766459081,0.242013910524089,0.95244596290955));
#92915=DIRECTION('center_axis',(0.981627005099017,-5.1149569548503E-17,
0.190809912898503));
#92916=DIRECTION('ref_axis',(-0.185359421522839,0.237305929223209,0.953586797731716));
#92917=DIRECTION('center_axis',(0.,1.,0.));
#92918=DIRECTION('ref_axis',(1.,0.,0.));
#92919=DIRECTION('',(-0.190809912898503,0.,0.981627005099017));
#92920=DIRECTION('center_axis',(0.,1.,0.));
#92921=DIRECTION('ref_axis',(-0.370562121723774,0.,0.928807684046366));
#92922=DIRECTION('center_axis',(0.,1.,0.));
#92923=DIRECTION('ref_axis',(-0.367006186766544,0.,0.930218500608906));
#92924=DIRECTION('center_axis',(-0.981627005099017,0.,-0.190809912898503));
#92925=DIRECTION('ref_axis',(-0.190809912898503,0.,0.981627005099017));
#92926=DIRECTION('center_axis',(-0.981627005099017,-4.61023199945355E-17,
-0.190809912898503));
#92927=DIRECTION('ref_axis',(-0.186536220732626,0.210460519128004,0.959640874620897));
#92928=DIRECTION('center_axis',(-0.981627005099017,-5.16917894804207E-17,
-0.190809912898504));
#92929=DIRECTION('ref_axis',(-0.186704454524913,0.206322520936108,0.960506358133627));
#92930=DIRECTION('center_axis',(0.,-1.,0.));
#92931=DIRECTION('ref_axis',(0.,0.,-1.));
#92932=DIRECTION('',(-0.190809912898503,0.,0.981627005099017));
#92933=DIRECTION('center_axis',(0.,-1.,0.));
#92934=DIRECTION('ref_axis',(-0.274471632436799,0.,0.961595197048882));
#92935=DIRECTION('',(-0.190809912898503,0.,0.981627005099017));
#92936=DIRECTION('center_axis',(0.,-1.,0.));
#92937=DIRECTION('ref_axis',(-0.272823755605811,0.,0.962064030289638));
#92938=DIRECTION('center_axis',(0.981627005099017,0.,0.190809912898503));
#92939=DIRECTION('ref_axis',(0.,-1.,0.));
#92940=DIRECTION('',(-0.190809912898503,0.,0.981627005099017));
#92941=DIRECTION('center_axis',(0.981627005099017,5.23922933240012E-17,
0.190809912898503));
#92942=DIRECTION('ref_axis',(-0.185225001331504,0.240171406973301,0.952895269247471));
#92943=DIRECTION('center_axis',(0.981627005099017,1.44009044006359E-17,
0.190809912898503));
#92944=DIRECTION('ref_axis',(-0.185440110076089,0.235568113333292,0.954001902280892));
#92945=DIRECTION('center_axis',(0.,1.,0.));
#92946=DIRECTION('ref_axis',(1.,0.,0.));
#92947=DIRECTION('',(-0.190809912898503,1.142355795319E-14,0.981627005099017));
#92948=DIRECTION('center_axis',(0.,1.,0.));
#92949=DIRECTION('ref_axis',(-0.307140935229151,0.,0.951664040461004));
#92950=DIRECTION('center_axis',(0.,1.,0.));
#92951=DIRECTION('ref_axis',(-0.304823463240135,0.,0.952408870316888));
#92952=DIRECTION('center_axis',(-0.981627005099017,0.,-0.190809912898503));
#92953=DIRECTION('ref_axis',(-0.190809912898503,0.,0.981627005099017));
#92954=DIRECTION('center_axis',(-0.981627005099017,-7.53381568193084E-17,
-0.190809912898504));
#92955=DIRECTION('ref_axis',(-0.186620533713518,0.208397434142596,0.960074625140809));
#92956=DIRECTION('center_axis',(-0.981627005099017,-2.17379342169057E-17,
-0.190809912898503));
#92957=DIRECTION('ref_axis',(-0.18678231992954,0.204377639939707,0.960906938914698));
#92958=DIRECTION('center_axis',(0.,-1.,0.));
#92959=DIRECTION('ref_axis',(0.,0.,-1.));
#92960=DIRECTION('',(-0.190809912898503,0.,0.981627005099017));
#92961=DIRECTION('center_axis',(0.,-1.,0.));
#92962=DIRECTION('ref_axis',(-0.210241863716573,0.,0.977649404817996));
#92963=DIRECTION('',(-0.190809912898503,0.,0.981627005099017));
#92964=DIRECTION('center_axis',(0.,-1.,0.));
#92965=DIRECTION('ref_axis',(-0.209856641284083,0.,0.977732166858063));
#92966=DIRECTION('center_axis',(0.981627005099017,0.,0.190809912898503));
#92967=DIRECTION('ref_axis',(0.,-1.,0.));
#92968=DIRECTION('',(-0.190809912898503,0.,0.981627005099017));
#92969=DIRECTION('center_axis',(0.981627005099017,1.41255374499376E-16,
0.190809912898504));
#92970=DIRECTION('ref_axis',(-0.185262960048131,0.239365914769592,0.953090548941034));
#92971=DIRECTION('center_axis',(0.981627005099017,-1.21618916880736E-16,
0.190809912898503));
#92972=DIRECTION('ref_axis',(-0.185475209669276,0.234807909926708,0.954182473132885));
#92973=DIRECTION('center_axis',(0.,1.,0.));
#92974=DIRECTION('ref_axis',(1.,0.,0.));
#92975=DIRECTION('',(-0.190809912898503,0.,0.981627005099017));
#92976=DIRECTION('center_axis',(0.,1.,0.));
#92977=DIRECTION('ref_axis',(-0.242853318412819,0.,0.970063021527922));
#92978=DIRECTION('center_axis',(0.,1.,0.));
#92979=DIRECTION('ref_axis',(-0.241809655546285,0.,0.970323703969241));
#92980=DIRECTION('center_axis',(-0.981627005099017,0.,-0.190809912898503));
#92981=DIRECTION('ref_axis',(-0.190809912898503,0.,0.981627005099017));
#92982=DIRECTION('center_axis',(-0.981627005099017,6.70648161298212E-17,
-0.190809912898503));
#92983=DIRECTION('ref_axis',(-0.186666733374594,0.207257848958206,0.96031230060667));
#92984=DIRECTION('center_axis',(-0.981627005099017,3.58496787124456E-17,
-0.190809912898503));
#92985=DIRECTION('ref_axis',(-0.186825037997708,0.203302399200895,0.961126703227163));
#92986=DIRECTION('center_axis',(0.,-1.,0.));
#92987=DIRECTION('ref_axis',(0.,0.,-1.));
#92988=DIRECTION('',(-0.190809912898503,0.,0.981627005099017));
#92989=DIRECTION('center_axis',(0.,-1.,0.));
#92990=DIRECTION('ref_axis',(-0.145176670594025,0.,0.989405748070646));
#92991=DIRECTION('',(-0.190809912898503,0.,0.981627005099017));
#92992=DIRECTION('center_axis',(0.,-1.,0.));
#92993=DIRECTION('ref_axis',(-0.146087012429917,0.,0.989271744668421));
#92994=DIRECTION('center_axis',(0.981627005099017,0.,0.190809912898503));
#92995=DIRECTION('ref_axis',(0.,-1.,0.));
#92996=DIRECTION('',(-0.190809912898503,0.,0.981627005099017));
#92997=DIRECTION('center_axis',(0.981627005099017,-4.46817620651805E-17,
0.190809912898503));
#92998=DIRECTION('ref_axis',(-0.185253518835601,0.239566527818698,0.953041978355581));
#92999=DIRECTION('center_axis',(0.981627005099017,1.14649557620665E-16,
0.190809912898504));
#93000=DIRECTION('ref_axis',(-0.185466477867897,0.234997270615096,0.954137552133199));
#93001=DIRECTION('center_axis',(0.,1.,0.));
#93002=DIRECTION('ref_axis',(1.,0.,0.));
#93003=DIRECTION('',(-0.190809912898503,0.,0.981627005099017));
#93004=DIRECTION('center_axis',(0.,1.,0.));
#93005=DIRECTION('ref_axis',(-0.177714334075482,0.,0.984082118252388));
#93006=DIRECTION('center_axis',(0.,1.,0.));
#93007=DIRECTION('ref_axis',(-0.177978632904428,0.,0.984034352159248));
#93008=DIRECTION('center_axis',(-0.981627005099017,0.,-0.190809912898503));
#93009=DIRECTION('ref_axis',(-0.190809912898503,0.,0.981627005099017));
#93010=DIRECTION('center_axis',(-0.981627005099017,-6.68964416434522E-17,
-0.190809912898504));
#93011=DIRECTION('ref_axis',(-0.186677250480035,0.206997512266798,0.960366406153699));
#93012=DIRECTION('center_axis',(-0.981627005099017,-1.14441817944589E-16,
-0.190809912898504));
#93013=DIRECTION('ref_axis',(-0.186834767627011,0.203056667686805,0.961176757580879));
#93014=DIRECTION('center_axis',(0.,-1.,0.));
#93015=DIRECTION('ref_axis',(0.,0.,-1.));
#93016=DIRECTION('',(-0.190809912898503,0.,0.981627005099017));
#93017=DIRECTION('center_axis',(0.,-1.,0.));
#93018=DIRECTION('ref_axis',(-0.0792738467656748,0.,0.99685287641606));
#93019=DIRECTION('',(-0.190809912898503,0.,0.981627005099017));
#93020=DIRECTION('center_axis',(0.,-1.,0.));
#93021=DIRECTION('ref_axis',(-0.0815128335683136,0.,0.996672292162105));
#93022=DIRECTION('center_axis',(0.981627005099017,0.,0.190809912898503));
#93023=DIRECTION('ref_axis',(0.,-1.,0.));
#93024=DIRECTION('',(-0.190809912898503,0.,0.981627005099017));
#93025=DIRECTION('center_axis',(0.981627005099017,2.25679470404183E-17,
0.190809912898503));
#93026=DIRECTION('ref_axis',(-0.185196189525605,0.240780891147295,0.9527470460954));
#93027=DIRECTION('center_axis',(0.981627005099017,-1.44712955763978E-17,
0.190809912898503));
#93028=DIRECTION('ref_axis',(-0.185413480709429,0.236143136345897,0.953864906749345));
#93029=DIRECTION('center_axis',(0.,1.,0.));
#93030=DIRECTION('ref_axis',(1.,0.,0.));
#93031=DIRECTION('',(-0.190809912898503,0.,0.981627005099017));
#93032=DIRECTION('center_axis',(0.,1.,0.));
#93033=DIRECTION('ref_axis',(-0.111727396157644,0.,0.993738893748168));
#93034=DIRECTION('center_axis',(0.,1.,0.));
#93035=DIRECTION('ref_axis',(-0.113333541028712,0.,0.993556998102219));
#93036=DIRECTION('center_axis',(-0.981627005099017,0.,-0.190809912898503));
#93037=DIRECTION('ref_axis',(-0.190809912898503,0.,0.981627005099017));
#93038=DIRECTION('center_axis',(-0.981627005099017,-1.12151063898178E-16,
-0.190809912898504));
#93039=DIRECTION('ref_axis',(-0.186652627005605,0.207606497435908,0.960239729991579));
#93040=DIRECTION('center_axis',(-0.981627005099017,-1.43863256786093E-16,
-0.190809912898504));
#93041=DIRECTION('ref_axis',(-0.186811990818403,0.203631433275501,0.961059581643423));
#93042=DIRECTION('center_axis',(0.,-1.,0.));
#93043=DIRECTION('ref_axis',(0.,0.,-1.));
#93044=DIRECTION('',(-0.190809912898503,0.,0.981627005099017));
#93045=DIRECTION('center_axis',(0.,-1.,0.));
#93046=DIRECTION('ref_axis',(-0.0125199473708714,0.,0.99992162238739));
#93047=DIRECTION('',(-0.190809912898503,0.,0.981627005099017));
#93048=DIRECTION('center_axis',(0.,-1.,0.));
#93049=DIRECTION('ref_axis',(-0.0161217085140551,0.,0.999870036812079));
#93050=DIRECTION('center_axis',(0.981627005099017,0.,0.190809912898503));
#93051=DIRECTION('ref_axis',(0.,-1.,0.));
#93052=DIRECTION('',(-0.190809912898503,0.,0.981627005099017));
#93053=DIRECTION('center_axis',(0.981627005099017,-4.59929004743199E-17,
0.190809912898503));
#93054=DIRECTION('ref_axis',(-0.185087953259993,0.243056025486103,0.952190221559183));
#93055=DIRECTION('center_axis',(0.981627005099017,0.,0.190809912898503));
#93056=DIRECTION('ref_axis',(-0.18531353769894,0.238288156967503,0.953350747099164));
#93057=DIRECTION('center_axis',(0.,1.,0.));
#93058=DIRECTION('ref_axis',(1.,0.,0.));
#93059=DIRECTION('',(-0.190809912898503,0.,0.981627005099017));
#93060=DIRECTION('center_axis',(0.,1.,0.));
#93061=DIRECTION('ref_axis',(-0.0448845029220051,0.,0.998992182851019));
#93062=DIRECTION('center_axis',(0.,1.,0.));
#93063=DIRECTION('ref_axis',(-0.0478670082003263,0.,0.998853717781513));
#93064=DIRECTION('center_axis',(-0.981627005099017,0.,-0.190809912898503));
#93065=DIRECTION('ref_axis',(-0.190809912898503,0.,0.981627005099017));
#93066=DIRECTION('center_axis',(-0.981627005099017,-8.3438172080403E-17,
-0.190809912898504));
#93067=DIRECTION('ref_axis',(-0.1865915874356,0.209108130897699,0.959925710193624));
#93068=DIRECTION('center_axis',(-0.981627005099017,-1.09403704958442E-16,
-0.190809912898504));
#93069=DIRECTION('ref_axis',(-0.186755573580884,0.205047867688004,0.960769341565955));
#93070=DIRECTION('center_axis',(0.,-1.,0.));
#93071=DIRECTION('ref_axis',(0.,0.,-1.));
#93072=DIRECTION('',(-0.190809912898503,0.,0.981627005099017));
#93073=DIRECTION('center_axis',(0.,-1.,0.));
#93074=DIRECTION('ref_axis',(0.0551106337815708,0.,0.998480254208461));
#93075=DIRECTION('',(-0.190809912898503,0.,0.981627005099017));
#93076=DIRECTION('center_axis',(0.,-1.,0.));
#93077=DIRECTION('ref_axis',(0.0501099354614011,0.,0.998743708049294));
#93078=DIRECTION('center_axis',(0.981627005099017,0.,0.190809912898503));
#93079=DIRECTION('ref_axis',(0.,-1.,0.));
#93080=DIRECTION('',(-0.190809912898503,0.,0.981627005099017));
#93081=DIRECTION('center_axis',(0.981627005099017,1.7343040380955E-16,0.190809912898504));
#93082=DIRECTION('ref_axis',(-0.184922851173921,0.246483524320091,0.951340849197834));
#93083=DIRECTION('center_axis',(0.981627005099017,-6.05488295791281E-17,
0.190809912898503));
#93084=DIRECTION('ref_axis',(-0.185161373141239,0.241515217748391,0.952567932219219));
#93085=DIRECTION('center_axis',(0.,1.,0.));
#93086=DIRECTION('ref_axis',(1.,0.,0.));
#93087=DIRECTION('',(-0.190809912898503,0.,0.981627005099017));
#93088=DIRECTION('center_axis',(0.,1.,0.));
#93089=DIRECTION('ref_axis',(0.0228343129577635,0.,0.999739263084004));
#93090=DIRECTION('center_axis',(0.,1.,0.));
#93091=DIRECTION('ref_axis',(0.018439340499448,0.,0.999829980907727));
#93092=DIRECTION('center_axis',(-0.981627005099017,0.,-0.190809912898503));
#93093=DIRECTION('ref_axis',(-0.190809912898503,0.,0.981627005099017));
#93094=DIRECTION('center_axis',(-0.981627005099017,-6.21145914153305E-17,
-0.190809912898504));
#93095=DIRECTION('ref_axis',(-0.186490869672513,0.211561527977992,0.959407564806744));
#93096=DIRECTION('center_axis',(-0.981627005099017,-1.8647400464012E-16,
-0.190809912898504));
#93097=DIRECTION('ref_axis',(-0.186662621580147,0.207359538000907,0.960291147363589));
#93098=DIRECTION('center_axis',(0.,-1.,0.));
#93099=DIRECTION('ref_axis',(0.,0.,-1.));
#93100=DIRECTION('',(-0.190809912898503,0.,0.981627005099017));
#93101=DIRECTION('center_axis',(0.,-1.,0.));
#93102=DIRECTION('ref_axis',(0.0521902993854495,0.,0.9986371576554));
#93103=DIRECTION('',(-0.190809912898503,0.,0.981627005099017));
#93104=DIRECTION('center_axis',(0.,-1.,0.));
#93105=DIRECTION('ref_axis',(0.047360966192575,0.,0.998877839818917));
#93106=DIRECTION('center_axis',(0.981627005099017,0.,0.190809912898503));
#93107=DIRECTION('ref_axis',(0.,-1.,0.));
#93108=DIRECTION('',(-0.190809912898503,0.,0.981627005099017));
#93109=DIRECTION('center_axis',(0.981627005099017,-3.9416000865807E-18,
0.190809912898503));
#93110=DIRECTION('ref_axis',(-0.187698004760385,0.179866355585003,0.965617705480559));
#93111=DIRECTION('center_axis',(0.981627005099017,8.32546406713011E-17,
0.190809912898504));
#93112=DIRECTION('ref_axis',(-0.187823180046607,0.176240834573197,0.966261673288413));
#93113=DIRECTION('center_axis',(0.,1.,0.));
#93114=DIRECTION('ref_axis',(1.,0.,0.));
#93115=DIRECTION('',(-0.190809912898503,0.,0.981627005099017));
#93116=DIRECTION('center_axis',(0.,1.,0.));
#93117=DIRECTION('ref_axis',(0.0198019381976702,0.,0.999803922398595));
#93118=DIRECTION('center_axis',(0.,1.,0.));
#93119=DIRECTION('ref_axis',(0.015586695628152,0.,0.999878520081012));
#93120=DIRECTION('center_axis',(-0.981627005099017,0.,-0.190809912898503));
#93121=DIRECTION('ref_axis',(-0.190809912898503,0.,0.981627005099017));
#93122=DIRECTION('center_axis',(-0.981627005099017,-1.08700534976828E-16,
-0.190809912898504));
#93123=DIRECTION('ref_axis',(-0.188780805300353,0.145448550484899,0.971188203548618));
#93124=DIRECTION('center_axis',(-0.981627005099017,-7.45896018560482E-17,
-0.190809912898504));
#93125=DIRECTION('ref_axis',(-0.188861020080131,0.142559682375593,0.971600870756744));
#93126=DIRECTION('center_axis',(0.,-1.,0.));
#93127=DIRECTION('ref_axis',(0.,0.,-1.));
#93128=DIRECTION('',(-0.190809912898503,0.,0.981627005099017));
#93129=DIRECTION('center_axis',(0.,-1.,0.));
#93130=DIRECTION('ref_axis',(0.0504037002691461,0.,0.998728925684631));
#93131=DIRECTION('',(-0.190809912898503,0.,0.981627005099017));
#93132=DIRECTION('center_axis',(0.,-1.,0.));
#93133=DIRECTION('ref_axis',(0.0456773194928813,0.,0.998956246531321));
#93134=DIRECTION('center_axis',(0.981627005099017,0.,0.190809912898503));
#93135=DIRECTION('ref_axis',(0.,-1.,0.));
#93136=DIRECTION('',(-0.190809912898503,0.,0.981627005099017));
#93137=DIRECTION('center_axis',(0.981627005099017,2.75912006060649E-17,
0.190809912898504));
#93138=DIRECTION('ref_axis',(-0.189582359577673,0.113249186849803,0.975311822247029));
#93139=DIRECTION('center_axis',(0.981627005099017,3.0274414789564E-17,0.190809912898504));
#93140=DIRECTION('ref_axis',(-0.189631500029847,0.110966451397898,0.975564626696042));
#93141=DIRECTION('center_axis',(0.,1.,0.));
#93142=DIRECTION('ref_axis',(1.,0.,0.));
#93143=DIRECTION('',(-0.190809912898503,0.,0.981627005099017));
#93144=DIRECTION('center_axis',(0.,1.,0.));
#93145=DIRECTION('ref_axis',(0.0177900737106688,0.,0.999841744116222));
#93146=DIRECTION('center_axis',(0.,1.,0.));
#93147=DIRECTION('ref_axis',(0.0136914263007247,0.,0.999906268030085));
#93148=DIRECTION('center_axis',(-0.981627005099017,0.,-0.190809912898503));
#93149=DIRECTION('ref_axis',(-0.190809912898503,0.,0.981627005099017));
#93150=DIRECTION('center_axis',(-0.981627005099017,3.29983766893944E-17,
-0.190809912898503));
#93151=DIRECTION('ref_axis',(-0.190208473521459,0.0793355729917432,0.978532883177008));
#93152=DIRECTION('center_axis',(-0.981627005099017,-3.17005807888205E-17,
-0.190809912898504));
#93153=DIRECTION('ref_axis',(-0.190232163502544,0.077759826750329,0.97865475695615));
#93154=DIRECTION('center_axis',(0.,-1.,0.));
#93155=DIRECTION('ref_axis',(0.,0.,-1.));
#93156=DIRECTION('',(-0.190809912898503,0.,0.981627005099017));
#93157=DIRECTION('center_axis',(0.,-1.,0.));
#93158=DIRECTION('ref_axis',(0.049679326965256,0.,0.998765219895186));
#93159=DIRECTION('',(-0.190809912898503,0.,0.981627005099017));
#93160=DIRECTION('center_axis',(0.,-1.,0.));
#93161=DIRECTION('ref_axis',(0.0449942826424662,0.,0.99898724442782));
#93162=DIRECTION('center_axis',(0.981627005099017,0.,0.190809912898503));
#93163=DIRECTION('ref_axis',(0.,-1.,0.));
#93164=DIRECTION('',(-0.190809912898503,0.,0.981627005099017));
#93165=DIRECTION('center_axis',(0.981627005099017,-9.85400021645174E-19,
0.190809912898503));
#93166=DIRECTION('ref_axis',(-0.190602337609787,0.0466320181146215,0.980559128142838));
#93167=DIRECTION('center_axis',(0.981627005099017,1.70293583191298E-17,
0.190809912898504));
#93168=DIRECTION('ref_axis',(-0.190610625689641,0.0456920682226691,0.980601766404558));
#93169=DIRECTION('center_axis',(0.,1.,0.));
#93170=DIRECTION('ref_axis',(1.,0.,0.));
#93171=DIRECTION('',(-0.190809912898503,0.,0.981627005099017));
#93172=DIRECTION('center_axis',(0.,1.,0.));
#93173=DIRECTION('ref_axis',(0.0167165551221656,0.,0.999860268629996));
#93174=DIRECTION('center_axis',(0.,1.,0.));
#93175=DIRECTION('ref_axis',(0.0126792641246964,0.,0.999919614899746));
#93176=DIRECTION('center_axis',(-0.981627005099017,0.,-0.190809912898503));
#93177=DIRECTION('ref_axis',(-0.190809912898503,0.,0.981627005099017));
#93178=DIRECTION('center_axis',(-0.981627005099017,-1.45581073629681E-18,
-0.190809912898503));
#93179=DIRECTION('ref_axis',(-0.190793231849958,0.0132225954986201,0.98154118897198));
#93180=DIRECTION('center_axis',(-0.981627005099017,3.26329508120211E-18,
-0.190809912898503));
#93181=DIRECTION('ref_axis',(-0.190793887927854,0.0129599711250496,0.981544564183314));
#93182=DIRECTION('center_axis',(0.,-1.,0.));
#93183=DIRECTION('ref_axis',(0.,0.,-1.));
#93184=DIRECTION('',(-0.190809912898503,0.,0.981627005099017));
#93185=DIRECTION('center_axis',(0.,-1.,0.));
#93186=DIRECTION('ref_axis',(-0.272681755189035,0.,0.962104287687685));
#93187=DIRECTION('',(-0.190809912898503,0.,0.981627005099017));
#93188=DIRECTION('center_axis',(0.,-1.,0.));
#93189=DIRECTION('ref_axis',(-0.271135734555198,0.,0.962541122990188));
#93190=DIRECTION('center_axis',(0.981627005099017,0.,0.190809912898503));
#93191=DIRECTION('ref_axis',(0.,-1.,0.));
#93192=DIRECTION('',(-0.190809912898503,0.,0.981627005099017));
#93193=DIRECTION('center_axis',(0.981627005099017,3.36807599940008E-17,
0.190809912898504));
#93194=DIRECTION('ref_axis',(-0.190612838364399,0.0454378337517089,0.980613149572562));
#93195=DIRECTION('center_axis',(0.981627005099017,0.,0.190809912898503));
#93196=DIRECTION('ref_axis',(-0.190620324225006,0.0445669403603487,0.980651660794632));
#93197=DIRECTION('center_axis',(0.,1.,0.));
#93198=DIRECTION('ref_axis',(1.,0.,0.));
#93199=DIRECTION('',(-0.190809912898503,0.,0.981627005099017));
#93200=DIRECTION('center_axis',(0.,1.,0.));
#93201=DIRECTION('ref_axis',(-0.303914183891769,0.,0.952699411582373));
#93202=DIRECTION('center_axis',(0.,1.,0.));
#93203=DIRECTION('ref_axis',(-0.301781433815546,0.,0.95337713744574));
#93204=DIRECTION('center_axis',(-0.981627005099017,0.,-0.190809912898503));
#93205=DIRECTION('ref_axis',(-0.190809912898503,0.,0.981627005099017));
#93206=DIRECTION('center_axis',(-0.981627005099017,-5.17949828132746E-18,
-0.190809912898504));
#93207=DIRECTION('ref_axis',(-0.190793727100074,0.0130248396339095,0.981543736800237));
#93208=DIRECTION('center_axis',(-0.981627005099017,3.17011540663208E-18,
-0.190809912898503));
#93209=DIRECTION('ref_axis',(-0.190794345521308,0.0127736024962302,0.981546918285807));
#93210=DIRECTION('center_axis',(0.,-1.,0.));
#93211=DIRECTION('ref_axis',(0.,0.,-1.));
#93212=DIRECTION('',(-0.190809912898503,0.,0.981627005099017));
#93213=DIRECTION('center_axis',(0.,-1.,0.));
#93214=DIRECTION('ref_axis',(-0.272920620201063,0.,0.962036555994141));
#93215=DIRECTION('',(-0.190809912898515,0.,0.981627005099015));
#93216=DIRECTION('center_axis',(0.,-1.,0.));
#93217=DIRECTION('ref_axis',(-0.271361249859389,0.,0.9624775696476));
#93218=DIRECTION('center_axis',(0.981627005099017,0.,0.190809912898503));
#93219=DIRECTION('ref_axis',(0.,-1.,0.));
#93220=DIRECTION('',(-0.190809912898503,0.,0.981627005099017));
#93221=DIRECTION('center_axis',(0.981627005099017,1.12269199980003E-17,
0.190809912898503));
#93222=DIRECTION('ref_axis',(-0.18964461730024,0.110349024825598,0.975632108865368));
#93223=DIRECTION('center_axis',(0.981627005099017,5.40033915023846E-17,
0.190809912898504));
#93224=DIRECTION('ref_axis',(-0.189688989693149,0.108233998017997,0.975860383898349));
#93225=DIRECTION('center_axis',(0.,1.,0.));
#93226=DIRECTION('ref_axis',(1.,0.,0.));
#93227=DIRECTION('',(-0.190809912898503,0.,0.981627005099017));
#93228=DIRECTION('center_axis',(0.,1.,0.));
#93229=DIRECTION('ref_axis',(-0.304480839231191,0.,0.952518460997512));
#93230=DIRECTION('center_axis',(0.,1.,0.));
#93231=DIRECTION('ref_axis',(-0.302316369370631,0.,0.953207644120923));
#93232=DIRECTION('center_axis',(-0.981627005099017,0.,-0.190809912898503));
#93233=DIRECTION('ref_axis',(-0.190809912898503,0.,0.981627005099017));
#93234=DIRECTION('center_axis',(-0.981627005099017,-4.70863480120678E-17,
-0.190809912898504));
#93235=DIRECTION('ref_axis',(-0.190226356519923,0.0781490378034625,0.978624882769465));
#93236=DIRECTION('center_axis',(-0.981627005099017,9.05747259037737E-18,
-0.190809912898503));
#93237=DIRECTION('ref_axis',(-0.190248684812419,0.0766416149774004,0.978739751303073));
#93238=DIRECTION('center_axis',(0.,-1.,0.));
#93239=DIRECTION('ref_axis',(0.,0.,-1.));
#93240=DIRECTION('',(-0.190809912898503,1.022228972926E-14,0.981627005099017));
#93241=DIRECTION('center_axis',(0.,-1.,0.));
#93242=DIRECTION('ref_axis',(-0.273509562255009,0.,0.961869283923275));
#93243=DIRECTION('',(-0.190809912898503,0.,0.981627005099017));
#93244=DIRECTION('center_axis',(0.,-1.,0.));
#93245=DIRECTION('ref_axis',(-0.271916957880207,0.,0.962320719935497));
#93246=DIRECTION('center_axis',(0.981627005099017,0.,0.190809912898503));
#93247=DIRECTION('ref_axis',(0.,-1.,0.));
#93248=DIRECTION('',(-0.190809912898503,0.,0.981627005099017));
#93249=DIRECTION('center_axis',(0.981627005099017,5.61345999900013E-17,
0.190809912898504));
#93250=DIRECTION('ref_axis',(-0.187856584998405,0.175260215899398,0.966433526009748));
#93251=DIRECTION('center_axis',(0.981627005099017,-1.80011305007949E-17,
0.190809912898503));
#93252=DIRECTION('ref_axis',(-0.187969558572489,0.171901055675604,0.967014721763674));
#93253=DIRECTION('center_axis',(0.,1.,0.));
#93254=DIRECTION('ref_axis',(1.,0.,0.));
#93255=DIRECTION('',(-0.190809912898503,0.,0.981627005099017));
#93256=DIRECTION('center_axis',(0.,1.,0.));
#93257=DIRECTION('ref_axis',(-0.305542296483778,0.,0.95217850482954));
#93258=DIRECTION('center_axis',(0.,1.,0.));
#93259=DIRECTION('ref_axis',(-0.303317587437942,0.,0.952889522007051));
#93260=DIRECTION('center_axis',(-0.981627005099017,0.,-0.190809912898503));
#93261=DIRECTION('ref_axis',(-0.190809912898503,0.,0.981627005099017));
#93262=DIRECTION('center_axis',(-0.981627005099017,-7.53381568193085E-17,
-0.190809912898504));
#93263=DIRECTION('ref_axis',(-0.18884135974173,0.143273235972994,0.971499727588599));
#93264=DIRECTION('center_axis',(-0.981627005099017,-1.44919561446038E-17,
-0.190809912898503));
#93265=DIRECTION('ref_axis',(-0.188916947337466,0.140509627458605,0.971888590117271));
#93266=DIRECTION('center_axis',(0.,-1.,0.));
#93267=DIRECTION('ref_axis',(0.,0.,-1.));
#93268=DIRECTION('',(-0.190809912898503,0.,0.981627005099017));
#93269=DIRECTION('center_axis',(0.,-1.,0.));
#93270=DIRECTION('ref_axis',(-0.210016949218452,0.,0.977697745236724));
#93271=DIRECTION('',(-0.190809912898503,0.,0.981627005099017));
#93272=DIRECTION('center_axis',(0.,-1.,0.));
#93273=DIRECTION('ref_axis',(-0.209644703523565,0.,0.977777632329824));
#93274=DIRECTION('center_axis',(0.981627005099017,0.,0.190809912898503));
#93275=DIRECTION('ref_axis',(0.,-1.,0.));
#93276=DIRECTION('',(-0.190809912898503,0.,0.981627005099017));
#93277=DIRECTION('center_axis',(0.981627005099017,4.08897136708722E-17,
0.190809912898503));
#93278=DIRECTION('ref_axis',(-0.187876516051428,0.1746724242913,0.966536061876937));
#93279=DIRECTION('center_axis',(0.981627005099017,2.11044591057748E-16,
0.190809912898504));
#93280=DIRECTION('ref_axis',(-0.187987998623376,0.1713463126492,0.967109587128108));
#93281=DIRECTION('center_axis',(0.,1.,0.));
#93282=DIRECTION('ref_axis',(1.,0.,0.));
#93283=DIRECTION('',(-0.190809912898503,0.,0.981627005099017));
#93284=DIRECTION('center_axis',(0.,1.,0.));
#93285=DIRECTION('ref_axis',(-0.242133347595446,0.,0.970242980898199));
#93286=DIRECTION('center_axis',(0.,1.,0.));
#93287=DIRECTION('ref_axis',(-0.241131647472688,0.,0.970492415522712));
#93288=DIRECTION('center_axis',(-0.981627005099017,0.,-0.190809912898503));
#93289=DIRECTION('ref_axis',(-0.190809912898503,0.,0.981627005099017));
#93290=DIRECTION('center_axis',(-0.981627005099017,2.60807618282638E-17,
-0.190809912898503));
#93291=DIRECTION('ref_axis',(-0.188862940934346,0.142489771158805,0.971610752645699));
#93292=DIRECTION('center_axis',(-0.981627005099017,-7.88692931673802E-17,
-0.190809912898504));
#93293=DIRECTION('ref_axis',(-0.188936911383774,0.139770399450607,0.971991295719348));
#93294=DIRECTION('center_axis',(0.,-1.,0.));
#93295=DIRECTION('ref_axis',(0.,0.,-1.));
#93296=DIRECTION('',(-0.190809912898503,1.171213937656E-14,0.981627005099017));
#93297=DIRECTION('center_axis',(0.,-1.,0.));
#93298=DIRECTION('ref_axis',(-0.145708207453926,0.,0.989327609177346));
#93299=DIRECTION('',(-0.190809912898503,0.,0.981627005099017));
#93300=DIRECTION('center_axis',(0.,-1.,0.));
#93301=DIRECTION('ref_axis',(-0.146587756234231,0.,0.989197669691055));
#93302=DIRECTION('center_axis',(0.981627005099017,0.,0.190809912898503));
#93303=DIRECTION('ref_axis',(0.,-1.,0.));
#93304=DIRECTION('',(-0.190809912898503,0.,0.981627005099017));
#93305=DIRECTION('center_axis',(0.981627005099017,3.35113215488854E-17,
0.190809912898503));
#93306=DIRECTION('ref_axis',(-0.187871558552619,0.174818817597398,0.966510557883802));
#93307=DIRECTION('center_axis',(0.981627005099017,-3.5827986756458E-18,
0.190809912898503));
#93308=DIRECTION('ref_axis',(-0.187983411095129,0.171484494773204,0.967085986459022));
#93309=DIRECTION('center_axis',(0.,1.,0.));
#93310=DIRECTION('ref_axis',(1.,0.,0.));
#93311=DIRECTION('',(-0.190809912898503,-1.31207553052E-14,0.981627005099017));
#93312=DIRECTION('center_axis',(0.,1.,0.));
#93313=DIRECTION('ref_axis',(-0.177896668082247,0.,0.984049173306515));
#93314=DIRECTION('center_axis',(0.,1.,0.));
#93315=DIRECTION('ref_axis',(-0.178150295368446,0.,0.984003288744573));
#93316=DIRECTION('center_axis',(-0.981627005099017,0.,-0.190809912898503));
#93317=DIRECTION('ref_axis',(-0.190809912898503,0.,0.981627005099017));
#93318=DIRECTION('center_axis',(-0.981627005099017,5.94635036830686E-17,
-0.190809912898503));
#93319=DIRECTION('ref_axis',(-0.188867854179084,0.142310789683404,0.971636028972513));
#93320=DIRECTION('center_axis',(-0.981627005099017,-3.5763068107684E-17,
-0.190809912898504));
#93321=DIRECTION('ref_axis',(-0.18894145881405,0.139601459034696,0.972014690103294));
#93322=DIRECTION('center_axis',(0.,-1.,0.));
#93323=DIRECTION('ref_axis',(0.,0.,-1.));
#93324=DIRECTION('',(-0.190809912898503,0.,0.981627005099017));
#93325=DIRECTION('center_axis',(0.,-1.,0.));
#93326=DIRECTION('ref_axis',(-0.080581231656937,0.,0.99674804494649));
#93327=DIRECTION('',(-0.190809912898503,0.,0.981627005099017));
#93328=DIRECTION('center_axis',(0.,-1.,0.));
#93329=DIRECTION('ref_axis',(-0.0827441701585023,0.,0.996570821519866));
#93330=DIRECTION('center_axis',(0.981627005099017,0.,0.190809912898503));
#93331=DIRECTION('ref_axis',(0.,-1.,0.));
#93332=DIRECTION('',(-0.190809912898503,1.014331218259E-14,0.981627005099017));
#93333=DIRECTION('center_axis',(0.981627005099017,3.38519205606274E-17,
0.190809912898503));
#93334=DIRECTION('ref_axis',(-0.187841458045623,0.175704974621005,0.966355704972412));
#93335=DIRECTION('center_axis',(0.981627005099017,1.01299069034784E-16,
0.190809912898504));
#93336=DIRECTION('ref_axis',(-0.187955569592477,0.172320667063197,0.966942755059503));
#93337=DIRECTION('center_axis',(0.,1.,0.));
#93338=DIRECTION('ref_axis',(1.,0.,0.));
#93339=DIRECTION('',(-0.190809912898503,0.,0.981627005099017));
#93340=DIRECTION('center_axis',(0.,1.,0.));
#93341=DIRECTION('ref_axis',(-0.11283548507849,0.,0.993613684138409));
#93342=DIRECTION('center_axis',(0.,1.,0.));
#93343=DIRECTION('ref_axis',(-0.11437651133568,0.,0.99343747344998));
#93344=DIRECTION('center_axis',(-0.981627005099017,0.,-0.190809912898503));
#93345=DIRECTION('ref_axis',(-0.190809912898503,0.,0.981627005099017));
#93346=DIRECTION('center_axis',(-0.981627005099017,-7.10290071355126E-17,
-0.190809912898504));
#93347=DIRECTION('ref_axis',(-0.188856351138037,0.142729466987203,0.971576851251807));
#93348=DIRECTION('center_axis',(-0.981627005099017,-1.11494024009222E-16,
-0.190809912898504));
#93349=DIRECTION('ref_axis',(-0.188930813598223,0.1399966103769,0.971959925488748));
#93350=DIRECTION('center_axis',(0.,-1.,0.));
#93351=DIRECTION('ref_axis',(0.,0.,-1.));
#93352=DIRECTION('',(-0.190809912898503,0.,0.981627005099017));
#93353=DIRECTION('center_axis',(0.,-1.,0.));
#93354=DIRECTION('ref_axis',(-0.0146231970935999,0.,0.999893075336939));
#93355=DIRECTION('',(-0.190809912898503,0.,0.981627005099017));
#93356=DIRECTION('center_axis',(0.,-1.,0.));
#93357=DIRECTION('ref_axis',(-0.0181020988785695,0.,0.999836143583633));
#93358=DIRECTION('center_axis',(0.981627005099017,0.,0.190809912898503));
#93359=DIRECTION('ref_axis',(0.,-1.,0.));
#93360=DIRECTION('',(-0.190809912898503,0.,0.981627005099017));
#93361=DIRECTION('center_axis',(0.981627005099017,3.83274170619332E-18,
0.190809912898503));
#93362=DIRECTION('ref_axis',(-0.187784641315811,0.177365207787101,0.966063409695518));
#93363=DIRECTION('center_axis',(0.981627005099017,-9.57800442010027E-17,
0.190809912898503));
#93364=DIRECTION('ref_axis',(-0.187903076011377,0.173885952381692,0.966672700343697));
#93365=DIRECTION('center_axis',(0.,1.,0.));
#93366=DIRECTION('ref_axis',(1.,0.,0.));
#93367=DIRECTION('',(-0.190809912898503,0.,0.981627005099017));
#93368=DIRECTION('center_axis',(0.,1.,0.));
#93369=DIRECTION('ref_axis',(-0.0469422356412144,0.,0.998897605619818));
#93370=DIRECTION('center_axis',(0.,1.,0.));
#93371=DIRECTION('ref_axis',(-0.049803312308202,0.,0.998759045056981));
#93372=DIRECTION('center_axis',(-0.981627005099017,0.,-0.190809912898503));
#93373=DIRECTION('ref_axis',(-0.190809912898503,0.,0.981627005099017));
#93374=DIRECTION('center_axis',(-0.981627005099017,-3.79264418547286E-18,
-0.190809912898503));
#93375=DIRECTION('ref_axis',(-0.18882783956697,0.143761839992095,0.971430172666341));
#93376=DIRECTION('center_axis',(-0.981627005099017,4.74082721486581E-17,
-0.190809912898503));
#93377=DIRECTION('ref_axis',(-0.188904448833758,0.140970409035506,0.971824291210698));
#93378=DIRECTION('center_axis',(0.,-1.,0.));
#93379=DIRECTION('ref_axis',(0.,0.,-1.));
#93380=DIRECTION('',(-0.190809912898503,0.,0.981627005099017));
#93381=DIRECTION('center_axis',(0.,-1.,0.));
#93382=DIRECTION('ref_axis',(-0.0159100952935859,0.,0.999873426423439));
#93383=DIRECTION('',(-0.190809912898503,0.,0.981627005099017));
#93384=DIRECTION('center_axis',(0.,-1.,0.));
#93385=DIRECTION('ref_axis',(-0.0193151720218505,0.,0.999813444663436));
#93386=DIRECTION('center_axis',(0.981627005099017,0.,0.190809912898503));
#93387=DIRECTION('ref_axis',(0.,-1.,0.));
#93388=DIRECTION('',(-0.190809912898503,0.,0.981627005099017));
#93389=DIRECTION('center_axis',(0.981627005099017,8.04875758300598E-17,
0.190809912898504));
#93390=DIRECTION('ref_axis',(-0.18961636862676,0.111674390088199,0.975486782763985));
#93391=DIRECTION('center_axis',(0.981627005099017,7.36769570776943E-18,
0.190809912898503));
#93392=DIRECTION('ref_axis',(-0.189662875504316,0.109483747795895,0.975726038713736));
#93393=DIRECTION('center_axis',(0.,1.,0.));
#93394=DIRECTION('ref_axis',(1.,0.,0.));
#93395=DIRECTION('',(-0.190809912898503,0.,0.981627005099017));
#93396=DIRECTION('center_axis',(0.,1.,0.));
#93397=DIRECTION('ref_axis',(-0.0483076832324515,0.,0.998832502344969));
#93398=DIRECTION('center_axis',(0.,1.,0.));
#93399=DIRECTION('ref_axis',(-0.051089968923592,0.,0.998694054791249));
#93400=DIRECTION('center_axis',(-0.981627005099017,0.,-0.190809912898503));
#93401=DIRECTION('ref_axis',(-0.190809912898503,0.,0.981627005099017));
#93402=DIRECTION('center_axis',(-0.981627005099017,-4.93043744111472E-17,
-0.190809912898504));
#93403=DIRECTION('ref_axis',(-0.190222363376804,0.0784155490866333,0.978604339931509));
#93404=DIRECTION('center_axis',(-0.981627005099017,-9.11697541320348E-18,
-0.190809912898503));
#93405=DIRECTION('ref_axis',(-0.190244992365523,0.0768929503830163,0.978720755405359));
#93406=DIRECTION('center_axis',(0.,-1.,0.));
#93407=DIRECTION('ref_axis',(0.,0.,-1.));
#93408=DIRECTION('',(-0.190809912898503,0.,0.981627005099017));
#93409=DIRECTION('center_axis',(0.,-1.,0.));
#93410=DIRECTION('ref_axis',(-0.0164319034129535,0.,0.99986498716088));
#93411=DIRECTION('',(-0.190809912898503,0.,0.981627005099017));
#93412=DIRECTION('center_axis',(0.,-1.,0.));
#93413=DIRECTION('ref_axis',(-0.0198073356643245,0.,0.999803815482758));
#93414=DIRECTION('center_axis',(0.981627005099017,0.,0.190809912898503));
#93415=DIRECTION('ref_axis',(0.,-1.,0.));
#93416=DIRECTION('',(-0.190809912898503,0.,0.981627005099017));
#93417=DIRECTION('center_axis',(0.981627005099017,2.20382648106116E-17,
0.190809912898504));
#93418=DIRECTION('ref_axis',(-0.190608073420958,0.0459835723892488,0.980588636185977));
#93419=DIRECTION('center_axis',(0.981627005099017,2.5786934977193E-17,0.190809912898504));
#93420=DIRECTION('ref_axis',(-0.19061591844487,0.0450815432100714,0.980628995133846));
#93421=DIRECTION('center_axis',(0.,1.,0.));
#93422=DIRECTION('ref_axis',(1.,0.,0.));
#93423=DIRECTION('',(-0.190809912898492,0.,0.981627005099019));
#93424=DIRECTION('center_axis',(0.,1.,0.));
#93425=DIRECTION('ref_axis',(-0.0490363496574017,0.,0.998796994595136));
#93426=DIRECTION('center_axis',(0.,1.,0.));
#93427=DIRECTION('ref_axis',(-0.0517771672578115,0.,0.998658662882747));
#93428=DIRECTION('center_axis',(-0.981627005099017,0.,-0.190809912898503));
#93429=DIRECTION('ref_axis',(-0.190809912898503,0.,0.981627005099017));
#93430=DIRECTION('center_axis',(-0.981627005099017,-1.09038520332345E-17,
-0.190809912898504));
#93431=DIRECTION('ref_axis',(-0.19079361651041,0.0130692581810996,0.981543167868573));
#93432=DIRECTION('center_axis',(-0.981627005099017,-8.20527787188313E-18,
-0.190809912898504));
#93433=DIRECTION('ref_axis',(-0.190794243247643,0.0128154917304995,0.981546392136034));
#93434=DIRECTION('center_axis',(0.,-1.,0.));
#93435=DIRECTION('ref_axis',(0.,0.,-1.));
#93436=DIRECTION('',(-0.190809912898503,0.,0.981627005099017));
#93437=DIRECTION('center_axis',(0.,-1.,0.));
#93438=DIRECTION('ref_axis',(-0.209823450757741,0.,0.977739290154647));
#93439=DIRECTION('',(-0.190809912898503,0.,0.981627005099017));
#93440=DIRECTION('center_axis',(0.,-1.,0.));
#93441=DIRECTION('ref_axis',(-0.209462139823336,0.,0.97781675787472));
#93442=DIRECTION('center_axis',(0.981627005099017,0.,0.190809912898503));
#93443=DIRECTION('ref_axis',(0.,-1.,0.));
#93444=DIRECTION('',(-0.190809912898503,0.,0.981627005099017));
#93445=DIRECTION('center_axis',(0.981627005099017,2.78793502301401E-17,
0.190809912898504));
#93446=DIRECTION('ref_axis',(-0.190614158731227,0.0452854433347916,0.980619942237133));
#93447=DIRECTION('center_axis',(0.981627005099017,1.60966213518621E-17,
0.190809912898504));
#93448=DIRECTION('ref_axis',(-0.190621546499908,0.0444231180942404,0.980657948822508));
#93449=DIRECTION('center_axis',(0.,1.,0.));
#93450=DIRECTION('ref_axis',(1.,0.,0.));
#93451=DIRECTION('',(-0.190809912898503,0.,0.981627005099017));
#93452=DIRECTION('center_axis',(0.,1.,0.));
#93453=DIRECTION('ref_axis',(-0.241400245375673,0.,0.970425639362731));
#93454=DIRECTION('center_axis',(0.,1.,0.));
#93455=DIRECTION('ref_axis',(-0.240440133543875,0.,0.970663969755447));
#93456=DIRECTION('center_axis',(-0.981627005099017,0.,-0.190809912898503));
#93457=DIRECTION('ref_axis',(-0.190809912898503,0.,0.981627005099017));
#93458=DIRECTION('center_axis',(-0.981627005099017,-9.3145577958085E-18,
-0.190809912898504));
#93459=DIRECTION('ref_axis',(-0.19079390364194,0.0129536155598903,0.981544645024869));
#93460=DIRECTION('center_axis',(-0.981627005099017,-2.24060491952785E-18,
-0.190809912898503));
#93461=DIRECTION('ref_axis',(-0.190794508898482,0.0127063999500603,0.981547758784307));
#93462=DIRECTION('center_axis',(0.,-1.,0.));
#93463=DIRECTION('ref_axis',(0.,0.,-1.));
#93464=DIRECTION('',(-0.190809912898503,0.,0.981627005099017));
#93465=DIRECTION('center_axis',(0.,-1.,0.));
#93466=DIRECTION('ref_axis',(-0.209879282403704,0.,0.97772730698171));
#93467=DIRECTION('',(-0.190809912898503,0.,0.981627005099017));
#93468=DIRECTION('center_axis',(0.,-1.,0.));
#93469=DIRECTION('ref_axis',(-0.209514838041807,0.,0.977805467687881));
#93470=DIRECTION('center_axis',(0.981627005099017,0.,0.190809912898503));
#93471=DIRECTION('ref_axis',(0.,-1.,0.));
#93472=DIRECTION('',(-0.190809912898503,0.,0.981627005099017));
#93473=DIRECTION('center_axis',(0.981627005099017,7.80621806443923E-17,
0.190809912898504));
#93474=DIRECTION('ref_axis',(-0.189652444394023,0.109978933813099,0.975672375571178));
#93475=DIRECTION('center_axis',(0.981627005099017,-1.07310809012414E-17,
0.190809912898503));
#93476=DIRECTION('ref_axis',(-0.189696233899903,0.107884715371704,0.975897651925323));
#93477=DIRECTION('center_axis',(0.,1.,0.));
#93478=DIRECTION('ref_axis',(1.,0.,0.));
#93479=DIRECTION('',(-0.190809912898503,0.,0.981627005099017));
#93480=DIRECTION('center_axis',(0.,1.,0.));
#93481=DIRECTION('ref_axis',(-0.241655381132283,0.,0.970362136920959));
#93482=DIRECTION('center_axis',(0.,1.,0.));
#93483=DIRECTION('ref_axis',(-0.240680925308484,0.,0.970604292280151));
#93484=DIRECTION('center_axis',(-0.981627005099017,0.,-0.190809912898503));
#93485=DIRECTION('ref_axis',(-0.190809912898503,0.,0.981627005099017));
#93486=DIRECTION('center_axis',(-0.981627005099017,1.11774693549702E-17,
-0.190809912898503));
#93487=DIRECTION('ref_axis',(-0.190232730879222,0.0777216933593315,0.978657675841554));
#93488=DIRECTION('center_axis',(-0.981627005099017,-4.66045823261792E-17,
-0.190809912898504));
#93489=DIRECTION('ref_axis',(-0.190254583170978,0.0762383997003401,0.978770095575855));
#93490=DIRECTION('center_axis',(0.,-1.,0.));
#93491=DIRECTION('ref_axis',(0.,0.,-1.));
#93492=DIRECTION('',(-0.190809912898503,0.,0.981627005099017));
#93493=DIRECTION('center_axis',(0.,-1.,0.));
#93494=DIRECTION('ref_axis',(-0.146033514275245,0.,0.989279643330652));
#93495=DIRECTION('',(-0.190809912898503,0.,0.981627005099017));
#93496=DIRECTION('center_axis',(0.,-1.,0.));
#93497=DIRECTION('ref_axis',(-0.146894553814633,0.,0.989152157182908));
#93498=DIRECTION('center_axis',(0.981627005099017,0.,0.190809912898503));
#93499=DIRECTION('ref_axis',(0.,-1.,0.));
#93500=DIRECTION('',(-0.190809912898503,0.,0.981627005099017));
#93501=DIRECTION('center_axis',(0.981627005099017,4.46817620651804E-17,
0.190809912898504));
#93502=DIRECTION('ref_axis',(-0.189650497494737,0.110071107376204,0.975662359692622));
#93503=DIRECTION('center_axis',(0.981627005099017,3.94107854321037E-17,
0.190809912898504));
#93504=DIRECTION('ref_axis',(-0.18969443164073,0.107971718931196,0.975888380151922));
#93505=DIRECTION('center_axis',(0.,1.,0.));
#93506=DIRECTION('ref_axis',(1.,0.,0.));
#93507=DIRECTION('',(-0.190809912898503,0.,0.981627005099017));
#93508=DIRECTION('center_axis',(0.,1.,0.));
#93509=DIRECTION('ref_axis',(-0.178017695683024,0.,0.98402728621909));
#93510=DIRECTION('center_axis',(0.,1.,0.));
#93511=DIRECTION('ref_axis',(-0.178264395839964,0.,0.983982624427796));
#93512=DIRECTION('center_axis',(-0.981627005099017,0.,-0.190809912898503));
#93513=DIRECTION('ref_axis',(-0.190809912898503,0.,0.981627005099017));
#93514=DIRECTION('center_axis',(-0.981627005099017,-7.43293796038357E-18,
-0.190809912898503));
#93515=DIRECTION('ref_axis',(-0.190234182158607,0.0776240671000532,0.978665141989482));
#93516=DIRECTION('center_axis',(-0.981627005099017,-1.43052272430736E-17,
-0.190809912898503));
#93517=DIRECTION('ref_axis',(-0.190255926766526,0.0761462503825465,0.978777007741237));
#93518=DIRECTION('center_axis',(0.,-1.,0.));
#93519=DIRECTION('ref_axis',(0.,0.,-1.));
#93520=DIRECTION('',(-0.190809912898503,0.,0.981627005099017));
#93521=DIRECTION('center_axis',(0.,-1.,0.));
#93522=DIRECTION('ref_axis',(-0.081381270585825,0.,0.996683043298037));
#93523=DIRECTION('',(-0.190809912898503,0.,0.981627005099017));
#93524=DIRECTION('center_axis',(0.,-1.,0.));
#93525=DIRECTION('ref_axis',(-0.0834985047492355,0.,0.996507902479776));
#93526=DIRECTION('center_axis',(0.981627005099017,0.,0.190809912898503));
#93527=DIRECTION('ref_axis',(0.,-1.,0.));
#93528=DIRECTION('',(-0.190809912898503,0.,0.981627005099017));
#93529=DIRECTION('center_axis',(0.981627005099017,6.77038411212548E-17,
0.190809912898504));
#93530=DIRECTION('ref_axis',(-0.189638677156094,0.110629058094703,0.975601549625443));
#93531=DIRECTION('center_axis',(0.981627005099017,-7.23564778819888E-18,
0.190809912898503));
#93532=DIRECTION('ref_axis',(-0.189683494387,0.108498197780605,0.975832113140113));
#93533=DIRECTION('center_axis',(0.,1.,0.));
#93534=DIRECTION('ref_axis',(1.,0.,0.));
#93535=DIRECTION('',(-0.190809912898503,0.,0.981627005099017));
#93536=DIRECTION('center_axis',(0.,1.,0.));
#93537=DIRECTION('ref_axis',(-0.113570890342994,0.,0.993529895305974));
#93538=DIRECTION('center_axis',(0.,1.,0.));
#93539=DIRECTION('ref_axis',(-0.115069654854028,0.,0.99335742536701));
#93540=DIRECTION('center_axis',(-0.981627005099017,0.,-0.190809912898503));
#93541=DIRECTION('ref_axis',(-0.190809912898503,0.,0.981627005099017));
#93542=DIRECTION('center_axis',(-0.981627005099017,-4.67296099575741E-17,
-0.190809912898504));
#93543=DIRECTION('ref_axis',(-0.19023078442017,0.0778524365384534,0.978647662227787));
#93544=DIRECTION('center_axis',(-0.981627005099017,-7.19316283930464E-18,
-0.190809912898503));
#93545=DIRECTION('ref_axis',(-0.1902527815393,0.0763617874783217,0.978760827030626));
#93546=DIRECTION('center_axis',(0.,-1.,0.));
#93547=DIRECTION('ref_axis',(0.,0.,-1.));
#93548=DIRECTION('',(-0.190809912898503,0.,0.981627005099017));
#93549=DIRECTION('center_axis',(0.,-1.,0.));
#93550=DIRECTION('ref_axis',(-0.0817056899061984,0.,0.996656500624439));
#93551=DIRECTION('',(-0.190809912898503,0.,0.981627005099017));
#93552=DIRECTION('center_axis',(0.,-1.,0.));
#93553=DIRECTION('ref_axis',(-0.0838045698468043,0.,0.996482209611788));
#93554=DIRECTION('center_axis',(0.981627005099017,0.,0.190809912898503));
#93555=DIRECTION('ref_axis',(0.,-1.,0.));
#93556=DIRECTION('',(-0.190809912898503,0.,0.981627005099017));
#93557=DIRECTION('center_axis',(0.981627005099017,3.38519205606274E-17,
0.190809912898504));
#93558=DIRECTION('ref_axis',(-0.190611836340838,0.0455531415684199,0.980607994633952));
#93559=DIRECTION('center_axis',(0.981627005099017,1.08534716822983E-17,
0.190809912898504));
#93560=DIRECTION('ref_axis',(-0.190619397058329,0.0446757284978794,0.980646890959382));
#93561=DIRECTION('center_axis',(0.,1.,0.));
#93562=DIRECTION('ref_axis',(1.,0.,0.));
#93563=DIRECTION('',(-0.190809912898503,0.,0.981627005099017));
#93564=DIRECTION('center_axis',(0.,1.,0.));
#93565=DIRECTION('ref_axis',(-0.113963373338753,0.,0.993484951842378));
#93566=DIRECTION('center_axis',(0.,1.,0.));
#93567=DIRECTION('ref_axis',(-0.115439892558234,0.,0.993314467430201));
#93568=DIRECTION('center_axis',(-0.981627005099017,0.,-0.190809912898503));
#93569=DIRECTION('ref_axis',(-0.190809912898503,0.,0.981627005099017));
#93570=DIRECTION('center_axis',(-0.981627005099017,-1.86918439830296E-18,
-0.190809912898503));
#93571=DIRECTION('ref_axis',(-0.190793849732929,0.0129754060897403,0.981544367688438));
#93572=DIRECTION('center_axis',(-0.981627005099017,-6.7435901618481E-18,
-0.190809912898504));
#93573=DIRECTION('ref_axis',(-0.19079445899501,0.0127269645797202,0.981547502054479));
#93574=DIRECTION('center_axis',(0.,1.,0.));
#93575=DIRECTION('ref_axis',(1.,0.,0.));
#93576=DIRECTION('',(-0.190809912898503,0.,0.981627005099017));
#93577=DIRECTION('center_axis',(0.,1.,0.));
#93578=DIRECTION('ref_axis',(-0.0225095378912939,0.,0.999746628253339));
#93579=DIRECTION('',(-0.190809912898503,0.,0.981627005099017));
#93580=DIRECTION('center_axis',(0.,1.,0.));
#93581=DIRECTION('ref_axis',(-0.0270306194594231,0.,0.99963460604945));
#93582=DIRECTION('center_axis',(-0.981627005099017,0.,-0.190809912898503));
#93583=DIRECTION('ref_axis',(-0.190809912898503,0.,0.981627005099017));
#93584=DIRECTION('',(-0.190809912898503,1.388010436138E-14,0.981627005099017));
#93585=DIRECTION('',(0.,-1.,0.));
#93586=DIRECTION('center_axis',(-0.981627005099017,-1.66876344160806E-16,
-0.190809912898503));
#93587=DIRECTION('ref_axis',(-0.159106063468809,-0.551997296878187,0.81852565311457));
#93588=DIRECTION('center_axis',(-0.981627005099017,-7.29358033056278E-17,
-0.190809912898503));
#93589=DIRECTION('ref_axis',(-0.157581438380154,-0.563881636142117,0.810682176132997));
#93590=DIRECTION('center_axis',(0.,-1.,0.));
#93591=DIRECTION('ref_axis',(0.,0.,-1.));
#93592=DIRECTION('',(-0.190809912898477,5.452489903615E-14,0.981627005099022));
#93593=DIRECTION('',(0.981627005099017,0.,0.190809912898503));
#93594=DIRECTION('center_axis',(0.,-1.,0.));
#93595=DIRECTION('ref_axis',(0.0160126619219826,0.,0.99987178911007));
#93596=DIRECTION('center_axis',(0.981627005099017,0.,0.190809912898503));
#93597=DIRECTION('ref_axis',(0.,-1.,0.));
#93598=DIRECTION('',(0.,1.,0.));
#93599=DIRECTION('center_axis',(0.981627005099017,-3.09443219726316E-16,
0.190809912898504));
#93600=DIRECTION('ref_axis',(-0.161261901248062,-0.534538298062307,0.829616421673603));
#93601=DIRECTION('center_axis',(-0.190809912898503,0.,0.981627005099017));
#93602=DIRECTION('ref_axis',(0.,1.,0.));
#93603=DIRECTION('center_axis',(0.190809912898503,-6.64418129801744E-16,
-0.981627005099017));
#93604=DIRECTION('ref_axis',(0.303629149237578,-0.950960567161055,0.0590198224157714));
#93605=DIRECTION('center_axis',(0.,1.,0.));
#93606=DIRECTION('ref_axis',(1.,0.,0.));
#93607=DIRECTION('',(-0.190809912898503,0.,0.981627005099017));
#93608=DIRECTION('center_axis',(0.,1.,0.));
#93609=DIRECTION('ref_axis',(-0.0996915880567629,0.,0.995018385393316));
#93610=DIRECTION('',(-0.190809912898503,0.,0.981627005099017));
#93611=DIRECTION('center_axis',(0.,1.,0.));
#93612=DIRECTION('ref_axis',(-0.102121602116587,0.,0.99477192279494));
#93613=DIRECTION('center_axis',(-0.981627005099017,0.,-0.190809912898503));
#93614=DIRECTION('ref_axis',(-0.190809912898503,0.,0.981627005099017));
#93615=DIRECTION('',(-0.190809912898503,0.,0.981627005099017));
#93616=DIRECTION('',(0.,-1.,0.));
#93617=DIRECTION('center_axis',(-0.981627005099017,2.69162553355626E-16,
-0.190809912898504));
#93618=DIRECTION('ref_axis',(-0.157963501542323,-0.5609378130862,0.812647710899723));
#93619=DIRECTION('center_axis',(-0.981627005099017,8.63179540716556E-17,
-0.190809912898503));
#93620=DIRECTION('ref_axis',(-0.158086350850289,-0.559986441507683,0.813279712646517));
#93621=DIRECTION('center_axis',(0.,-1.,0.));
#93622=DIRECTION('ref_axis',(0.,0.,-1.));
#93623=DIRECTION('',(-0.190809912898503,0.,0.981627005099017));
#93624=DIRECTION('',(0.981627005099017,0.,0.190809912898503));
#93625=DIRECTION('center_axis',(0.,-1.,0.));
#93626=DIRECTION('ref_axis',(-0.0615580680962634,0.,0.998103503777166));
#93627=DIRECTION('center_axis',(0.981627005099017,0.,0.190809912898503));
#93628=DIRECTION('ref_axis',(0.,-1.,0.));
#93629=DIRECTION('center_axis',(0.981627005099017,-1.80543576323346E-16,
0.190809912898504));
#93630=DIRECTION('ref_axis',(-0.160582097948044,-0.540130107168397,0.826119154328757));
#93631=DIRECTION('',(0.,1.,0.));
#93632=DIRECTION('center_axis',(0.981627005099017,-4.63081458444729E-16,
0.190809912898504));
#93633=DIRECTION('ref_axis',(-0.161838961663713,-0.529726495046211,0.832585125337745));
#93634=DIRECTION('center_axis',(-0.190809912898503,0.,0.981627005099017));
#93635=DIRECTION('ref_axis',(0.,1.,0.));
#93636=DIRECTION('center_axis',(0.190809912898503,5.18712399582064E-16,
-0.981627005099017));
#93637=DIRECTION('ref_axis',(0.191173908779205,-0.980852498727369,0.0371606289284456));
#93638=DIRECTION('center_axis',(0.,1.,0.));
#93639=DIRECTION('ref_axis',(1.,0.,0.));
#93640=DIRECTION('',(-0.190809912898503,0.,0.981627005099017));
#93641=DIRECTION('center_axis',(0.,1.,0.));
#93642=DIRECTION('ref_axis',(-0.175735962495432,0.,0.984437337511029));
#93643=DIRECTION('',(-0.190809912898503,0.,0.981627005099017));
#93644=DIRECTION('center_axis',(0.,1.,0.));
#93645=DIRECTION('ref_axis',(-0.176135083798187,0.,0.984366005231492));
#93646=DIRECTION('center_axis',(-0.981627005099017,0.,-0.190809912898503));
#93647=DIRECTION('ref_axis',(-0.190809912898503,0.,0.981627005099017));
#93648=DIRECTION('',(-0.190809912898503,0.,0.981627005099017));
#93649=DIRECTION('',(0.,-1.,0.));
#93650=DIRECTION('center_axis',(-0.981627005099017,8.91952555246029E-17,
-0.190809912898503));
#93651=DIRECTION('ref_axis',(-0.157500137288895,-0.564505169249368,0.810263920364668));
#93652=DIRECTION('center_axis',(-0.981627005099017,8.58313634584417E-17,
-0.190809912898503));
#93653=DIRECTION('ref_axis',(-0.158289781209933,-0.558405836138714,0.814326265897604));
#93654=DIRECTION('center_axis',(0.,-1.,0.));
#93655=DIRECTION('ref_axis',(0.,0.,-1.));
#93656=DIRECTION('',(-0.190809912898503,0.,0.981627005099017));
#93657=DIRECTION('',(0.981627005099017,0.,0.190809912898503));
#93658=DIRECTION('center_axis',(0.,-1.,0.));
#93659=DIRECTION('ref_axis',(-0.137981858751738,0.,0.990434756385001));
#93660=DIRECTION('center_axis',(0.981627005099017,0.,0.190809912898503));
#93661=DIRECTION('ref_axis',(0.,-1.,0.));
#93662=DIRECTION('center_axis',(0.981627005099017,-1.04257444818754E-16,
0.190809912898503));
#93663=DIRECTION('ref_axis',(-0.160914514245377,-0.537405994836492,0.827829279392179));
#93664=DIRECTION('',(0.,1.,0.));
#93665=DIRECTION('center_axis',(0.981627005099017,-4.58598230482662E-16,
0.190809912898504));
#93666=DIRECTION('ref_axis',(-0.162144254191831,-0.527156039487894,0.834155711401662));
#93667=DIRECTION('center_axis',(-0.190809912898503,0.,0.981627005099017));
#93668=DIRECTION('ref_axis',(0.,1.,0.));
#93669=DIRECTION('center_axis',(0.190809912898503,-5.91565264691904E-16,
-0.981627005099017));
#93670=DIRECTION('ref_axis',(0.0787186683208446,-0.996779432638552,0.0153014354411246));
#93671=DIRECTION('center_axis',(0.,1.,0.));
#93672=DIRECTION('ref_axis',(1.,0.,0.));
#93673=DIRECTION('',(-0.190809912898503,0.,0.981627005099017));
#93674=DIRECTION('center_axis',(0.,1.,0.));
#93675=DIRECTION('ref_axis',(-0.250656761475531,0.,0.968076023836247));
#93676=DIRECTION('',(-0.190809912898503,0.,0.981627005099017));
#93677=DIRECTION('center_axis',(0.,1.,0.));
#93678=DIRECTION('ref_axis',(-0.249083719402477,0.,0.968481956842061));
#93679=DIRECTION('center_axis',(-0.981627005099017,0.,-0.190809912898503));
#93680=DIRECTION('ref_axis',(-0.190809912898503,0.,0.981627005099017));
#93681=DIRECTION('',(-0.190809912898503,0.,0.981627005099017));
#93682=DIRECTION('',(0.,-1.,0.));
#93683=DIRECTION('center_axis',(-0.981627005099017,-1.6393621720623E-16,
-0.190809912898503));
#93684=DIRECTION('ref_axis',(-0.157698222107343,-0.562984198653009,0.811282973327564));
#93685=DIRECTION('center_axis',(-0.981627005099017,2.72457558214586E-16,
-0.190809912898504));
#93686=DIRECTION('ref_axis',(-0.1582029102982,-0.559081597802509,0.813879356029979));
#93687=DIRECTION('center_axis',(0.,-1.,0.));
#93688=DIRECTION('ref_axis',(0.,0.,-1.));
#93689=DIRECTION('',(-0.190809912898503,0.,0.981627005099017));
#93690=DIRECTION('',(0.981627005099017,0.,0.190809912898503));
#93691=DIRECTION('center_axis',(0.,-1.,0.));
#93692=DIRECTION('ref_axis',(-0.21328299146488,0.,0.976990463388355));
#93693=DIRECTION('center_axis',(0.981627005099017,0.,0.190809912898503));
#93694=DIRECTION('ref_axis',(0.,-1.,0.));
#93695=DIRECTION('center_axis',(0.981627005099017,-1.48689867894081E-16,
0.190809912898503));
#93696=DIRECTION('ref_axis',(-0.160969201866504,-0.536955970969592,0.828110621409098));
#93697=DIRECTION('',(0.,1.,0.));
#93698=DIRECTION('center_axis',(0.981627005099017,4.29243236049658E-17,
0.190809912898503));
#93699=DIRECTION('ref_axis',(-0.162194507351624,-0.526731257403113,0.834414240206565));
#93700=DIRECTION('center_axis',(-0.190809912898503,0.,0.981627005099017));
#93701=DIRECTION('ref_axis',(0.,1.,0.));
#93702=DIRECTION('center_axis',(0.190809912898503,1.62461889194944E-16,
-0.981627005099017));
#93703=DIRECTION('ref_axis',(-0.0337365721375064,-0.999409245259327,-0.00655775804619647));
#93704=DIRECTION('center_axis',(0.,1.,0.));
#93705=DIRECTION('ref_axis',(1.,0.,0.));
#93706=DIRECTION('',(-0.190809912898503,0.,0.981627005099017));
#93707=DIRECTION('center_axis',(0.,1.,0.));
#93708=DIRECTION('ref_axis',(-0.324447978030139,0.,0.945903541357233));
#93709=DIRECTION('',(-0.190809912898503,0.,0.981627005099017));
#93710=DIRECTION('center_axis',(0.,1.,0.));
#93711=DIRECTION('ref_axis',(-0.320962116007901,0.,0.947092033588991));
#93712=DIRECTION('center_axis',(-0.981627005099017,0.,-0.190809912898503));
#93713=DIRECTION('ref_axis',(-0.190809912898503,0.,0.981627005099017));
#93714=DIRECTION('',(-0.190809912898503,0.,0.981627005099017));
#93715=DIRECTION('',(0.,-1.,0.));
#93716=DIRECTION('center_axis',(-0.981627005099017,3.76690784096542E-16,
-0.190809912898504));
#93717=DIRECTION('ref_axis',(-0.158565308967581,-0.556254632219511,0.815743726256201));
#93718=DIRECTION('center_axis',(-0.981627005099017,-3.33314991325887E-16,
-0.190809912898503));
#93719=DIRECTION('ref_axis',(-0.157820990225955,-0.562038509834281,0.811914557393424));
#93720=DIRECTION('center_axis',(0.,-1.,0.));
#93721=DIRECTION('ref_axis',(0.,0.,-1.));
#93722=DIRECTION('',(-0.190809912898503,0.,0.981627005099017));
#93723=DIRECTION('',(0.981627005099017,0.,0.190809912898503));
#93724=DIRECTION('center_axis',(0.,-1.,0.));
#93725=DIRECTION('ref_axis',(-0.287465429548881,0.,0.957791014164508));
#93726=DIRECTION('center_axis',(0.981627005099017,0.,0.190809912898503));
#93727=DIRECTION('ref_axis',(0.,-1.,0.));
#93728=DIRECTION('center_axis',(0.981627005099017,-3.89199893264009E-16,
0.190809912898504));
#93729=DIRECTION('ref_axis',(-0.160749232394967,-0.538762885913093,0.8269789822281));
#93730=DIRECTION('',(0.,1.,0.));
#93731=DIRECTION('center_axis',(0.981627005099017,-4.32027132019077E-17,
0.190809912898503));
#93732=DIRECTION('ref_axis',(-0.161992422346658,-0.528436578558402,0.83337460817075));
#93733=DIRECTION('center_axis',(-0.190809912898503,0.,0.981627005099017));
#93734=DIRECTION('ref_axis',(0.,1.,0.));
#93735=DIRECTION('center_axis',(0.190809912898503,5.2454062879085E-17,-0.981627005099017));
#93736=DIRECTION('ref_axis',(-0.146191812595837,-0.988848032204891,-0.0284169515335126));
#93737=DIRECTION('center_axis',(0.,1.,0.));
#93738=DIRECTION('ref_axis',(1.,0.,0.));
#93739=DIRECTION('',(-0.190809912898503,0.,0.981627005099017));
#93740=DIRECTION('',(-0.981627005099017,0.,-0.190809912898503));
#93741=DIRECTION('center_axis',(0.,1.,0.));
#93742=DIRECTION('ref_axis',(-0.390089733402804,0.,0.920776845871859));
#93743=DIRECTION('',(-0.190809912898503,0.,0.981627005099017));
#93744=DIRECTION('center_axis',(0.,1.,0.));
#93745=DIRECTION('ref_axis',(-0.391746367360933,0.,0.920073249072873));
#93746=DIRECTION('center_axis',(-0.981627005099017,0.,-0.190809912898503));
#93747=DIRECTION('ref_axis',(-0.190809912898503,0.,0.981627005099017));
#93748=DIRECTION('',(-0.190809912898503,1.605442884968E-13,0.981627005099017));
#93749=DIRECTION('',(0.,-1.,0.));
#93750=DIRECTION('center_axis',(-0.981627005099017,-8.86144962521498E-17,
-0.190809912898503));
#93751=DIRECTION('ref_axis',(-0.157122673757211,-0.567386932574192,0.808322048527339));
#93752=DIRECTION('center_axis',(0.,-1.,0.));
#93753=DIRECTION('ref_axis',(0.,0.,-1.));
#93754=DIRECTION('',(-0.190809912898503,-1.607428443784E-14,0.981627005099017));
#93755=DIRECTION('',(0.981627005099017,0.,0.190809912898503));
#93756=DIRECTION('center_axis',(0.,-1.,0.));
#93757=DIRECTION('ref_axis',(-0.360513177655806,0.,0.93275412019273));
#93758=DIRECTION('center_axis',(0.981627005099017,0.,0.190809912898503));
#93759=DIRECTION('ref_axis',(0.,-1.,0.));
#93760=DIRECTION('center_axis',(0.981627005099017,-3.03995681381544E-17,
0.190809912898503));
#93761=DIRECTION('ref_axis',(-0.160242144137859,-0.542896069554004,0.824370252316831));
#93762=DIRECTION('',(0.,1.,0.));
#93763=DIRECTION('center_axis',(0.981627005099017,-4.67653207300599E-16,
0.190809912898504));
#93764=DIRECTION('ref_axis',(-0.161527046948701,-0.532334922311487,0.830980471245657));
#93765=DIRECTION('center_axis',(-0.190809912898503,0.,0.981627005099017));
#93766=DIRECTION('ref_axis',(0.,1.,0.));
#93767=DIRECTION('center_axis',(0.190809912898503,2.0981625151634E-16,-0.981627005099017));
#93768=DIRECTION('ref_axis',(-0.258647053054216,-0.964662641128085,-0.0502761450208387));
#93769=DIRECTION('center_axis',(0.,1.,0.));
#93770=DIRECTION('ref_axis',(1.,0.,0.));
#93771=DIRECTION('',(-0.190809912898488,0.,0.98162700509902));
#93772=DIRECTION('',(-0.981627005099017,0.,-0.190809912898503));
#93773=DIRECTION('center_axis',(0.,1.,0.));
#93774=DIRECTION('ref_axis',(-0.699923036064448,0.,0.714218274469595));
#93775=DIRECTION('',(-0.190809912898503,0.,0.981627005099017));
#93776=DIRECTION('center_axis',(0.,1.,0.));
#93777=DIRECTION('ref_axis',(-0.711546942295925,0.,0.702638562071083));
#93778=DIRECTION('center_axis',(-0.981627005099017,0.,-0.190809912898503));
#93779=DIRECTION('ref_axis',(-0.190809912898503,0.,0.981627005099017));
#93780=DIRECTION('',(-0.190809912898503,4.013607212418E-14,0.981627005099017));
#93781=DIRECTION('',(0.,-1.,0.));
#93782=DIRECTION('center_axis',(-0.981627005099017,2.5977613593094E-17,
-0.190809912898503));
#93783=DIRECTION('ref_axis',(-0.186383180917028,-0.214152203332011,0.958853556951892));
#93784=DIRECTION('center_axis',(0.,-1.,0.));
#93785=DIRECTION('ref_axis',(0.,0.,-1.));
#93786=DIRECTION('',(-0.190809912898503,0.,0.981627005099017));
#93787=DIRECTION('',(0.981627005099017,0.,0.190809912898503));
#93788=DIRECTION('center_axis',(0.,-1.,0.));
#93789=DIRECTION('ref_axis',(-0.686504883900775,0.,0.727125191683236));
#93790=DIRECTION('center_axis',(0.981627005099017,0.,0.190809912898503));
#93791=DIRECTION('ref_axis',(0.,-1.,0.));
#93792=DIRECTION('center_axis',(0.981627005099017,-3.65431440454912E-17,
0.190809912898503));
#93793=DIRECTION('ref_axis',(-0.187820057364573,-0.1763322148272,0.966245608562183));
#93794=DIRECTION('',(0.,1.,0.));
#93795=DIRECTION('center_axis',(0.981627005099017,-4.94804897087551E-17,
0.190809912898504));
#93796=DIRECTION('ref_axis',(-0.187977242348303,-0.171670124543093,0.967054251166131));
#93797=DIRECTION('center_axis',(-0.190809912898503,0.,0.981627005099017));
#93798=DIRECTION('ref_axis',(0.,1.,0.));
#93799=DIRECTION('center_axis',(0.190809912898504,2.44785626769064E-16,
-0.981627005099017));
#93800=DIRECTION('ref_axis',(-0.933378495804326,-0.309656688597602,-0.181431305944762));
#93801=DIRECTION('center_axis',(0.981627005099017,0.,0.190809912898503));
#93802=DIRECTION('ref_axis',(0.,-1.,0.));
#93803=DIRECTION('',(-0.190809912898503,0.,0.981627005099017));
#93804=DIRECTION('center_axis',(0.981627005099017,-6.00351652175927E-17,
0.190809912898504));
#93805=DIRECTION('ref_axis',(-0.189859859903711,-0.0996660344675376,0.976739430539619));
#93806=DIRECTION('',(-0.190809912898503,0.,0.981627005099017));
#93807=DIRECTION('center_axis',(0.981627005099017,-1.23701224271888E-17,
0.190809912898503));
#93808=DIRECTION('ref_axis',(-0.189909550677726,-0.0970309399591574,0.976995066134946));
#93809=DIRECTION('center_axis',(0.,1.,0.));
#93810=DIRECTION('ref_axis',(1.,0.,0.));
#93811=DIRECTION('',(-0.190809912898503,0.,0.981627005099017));
#93812=DIRECTION('',(-0.981627005099017,0.,-0.190809912898503));
#93813=DIRECTION('center_axis',(0.,1.,0.));
#93814=DIRECTION('ref_axis',(-0.708046345681522,0.,0.706165966587914));
#93815=DIRECTION('center_axis',(0.,1.,0.));
#93816=DIRECTION('ref_axis',(-0.708026020831984,0.,0.706186344971939));
#93817=DIRECTION('center_axis',(-0.981627005099017,0.,-0.190809912898503));
#93818=DIRECTION('ref_axis',(-0.190809912898503,0.,0.981627005099017));
#93819=DIRECTION('',(-0.190809912898503,0.,0.981627005099017));
#93820=DIRECTION('',(0.,-1.,0.));
#93821=DIRECTION('center_axis',(-0.981627005099017,2.5977613593094E-17,
-0.190809912898503));
#93822=DIRECTION('ref_axis',(-0.188993069322325,-0.137669273570596,0.97228020182593));
#93823=DIRECTION('center_axis',(0.,-1.,0.));
#93824=DIRECTION('ref_axis',(0.,0.,-1.));
#93825=DIRECTION('center_axis',(0.,-1.,0.));
#93826=DIRECTION('ref_axis',(-0.691132671254374,0.,0.722727909191829));
#93827=DIRECTION('',(0.981627005099017,0.,0.190809912898503));
#93828=DIRECTION('center_axis',(0.,-1.,0.));
#93829=DIRECTION('ref_axis',(-0.682158787921673,0.,0.731204067317212));
#93830=DIRECTION('center_axis',(-0.190809912898503,0.,0.981627005099017));
#93831=DIRECTION('ref_axis',(0.,1.,0.));
#93832=DIRECTION('center_axis',(0.190809912898503,-8.74234381318085E-17,
-0.981627005099017));
#93833=DIRECTION('ref_axis',(-0.960530036154236,-0.206208093067504,-0.186709057088846));
#93834=DIRECTION('center_axis',(0.981627005099017,0.,0.190809912898503));
#93835=DIRECTION('ref_axis',(0.,-1.,0.));
#93836=DIRECTION('',(-0.190809912898503,0.,0.981627005099017));
#93837=DIRECTION('center_axis',(0.981627005099017,5.22044914935589E-18,
0.190809912898503));
#93838=DIRECTION('ref_axis',(-0.190759437640654,-0.0229998541078904,0.981367333704377));
#93839=DIRECTION('',(-0.190809912898503,0.,0.981627005099017));
#93840=DIRECTION('center_axis',(0.981627005099017,-3.71103672815663E-18,
0.190809912898503));
#93841=DIRECTION('ref_axis',(-0.190762071742238,-0.0223917553751911,0.981380884914632));
#93842=DIRECTION('center_axis',(0.,1.,0.));
#93843=DIRECTION('ref_axis',(1.,0.,0.));
#93844=DIRECTION('',(-0.190809912898503,0.,0.981627005099017));
#93845=DIRECTION('',(-0.981627005099013,0.,-0.190809912898526));
#93846=DIRECTION('center_axis',(0.,1.,0.));
#93847=DIRECTION('ref_axis',(-0.711526155446024,0.,0.702659611843601));
#93848=DIRECTION('center_axis',(0.,1.,0.));
#93849=DIRECTION('ref_axis',(-0.706483995353756,0.,0.707729018981837));
#93850=DIRECTION('center_axis',(-0.981627005099017,0.,-0.190809912898503));
#93851=DIRECTION('ref_axis',(-0.190809912898503,0.,0.981627005099017));
#93852=DIRECTION('',(-0.190809912898515,0.,0.981627005099015));
#93853=DIRECTION('',(0.,-1.,0.));
#93854=DIRECTION('center_axis',(-0.981627005099017,3.50697783506769E-17,
-0.190809912898504));
#93855=DIRECTION('ref_axis',(-0.19045240389019,-0.0611863438091478,0.979787789872744));
#93856=DIRECTION('center_axis',(0.,-1.,0.));
#93857=DIRECTION('ref_axis',(0.,0.,-1.));
#93858=DIRECTION('center_axis',(0.,-1.,0.));
#93859=DIRECTION('ref_axis',(-0.688592136426526,0.,0.725148860339415));
#93860=DIRECTION('',(0.981627005099017,0.,0.190809912898503));
#93861=DIRECTION('center_axis',(0.,-1.,0.));
#93862=DIRECTION('ref_axis',(-0.679752594529884,0.,0.733441483848501));
#93863=DIRECTION('center_axis',(-0.190809912898503,0.,0.981627005099017));
#93864=DIRECTION('ref_axis',(0.,1.,0.));
#93865=DIRECTION('center_axis',(0.190809912898504,6.41105212966596E-17,
-0.981627005099017));
#93866=DIRECTION('ref_axis',(-0.977495790902178,-0.0916480413633408,-0.190006882198483));
#93867=DIRECTION('center_axis',(0.,1.,0.));
#93868=DIRECTION('ref_axis',(1.,0.,0.));
#93869=DIRECTION('',(-0.190809912898503,0.,0.981627005099017));
#93870=DIRECTION('center_axis',(0.,1.,0.));
#93871=DIRECTION('ref_axis',(0.120993925133802,0.,0.992653247655351));
#93872=DIRECTION('',(-0.190809912898503,0.,0.981627005099017));
#93873=DIRECTION('center_axis',(0.,1.,0.));
#93874=DIRECTION('ref_axis',(0.113186441507845,0.,0.993573766490839));
#93875=DIRECTION('center_axis',(-0.981627005099017,0.,-0.190809912898503));
#93876=DIRECTION('ref_axis',(-0.190809912898503,0.,0.981627005099017));
#93877=DIRECTION('',(-0.190809912898503,0.,0.981627005099017));
#93878=DIRECTION('',(0.,-1.,0.));
#93879=DIRECTION('center_axis',(-0.981627005099017,5.1352667504369E-16,
-0.190809912898504));
#93880=DIRECTION('ref_axis',(-0.16364102821286,-0.51429587245801,0.841855907776439));
#93881=DIRECTION('center_axis',(-0.981627005099017,-2.15548573767396E-16,
-0.190809912898503));
#93882=DIRECTION('ref_axis',(-0.163734348297844,-0.513479438445504,0.842335995598651));
#93883=DIRECTION('center_axis',(0.,-1.,0.));
#93884=DIRECTION('ref_axis',(0.,0.,-1.));
#93885=DIRECTION('',(-0.190809912898486,-1.729025838123E-14,0.98162700509902));
#93886=DIRECTION('',(0.981627005099017,0.,0.190809912898503));
#93887=DIRECTION('center_axis',(0.,-1.,0.));
#93888=DIRECTION('ref_axis',(0.157666506055977,0.,0.987492416612958));
#93889=DIRECTION('center_axis',(0.981627005099017,0.,0.190809912898503));
#93890=DIRECTION('ref_axis',(0.,-1.,0.));
#93891=DIRECTION('center_axis',(0.981627005099017,1.31015175507947E-16,
0.190809912898503));
#93892=DIRECTION('ref_axis',(-0.165724730740096,-0.495631116264313,0.852575574486927));
#93893=DIRECTION('',(0.,1.,0.));
#93894=DIRECTION('center_axis',(0.981627005099017,-2.040880606468E-16,0.190809912898504));
#93895=DIRECTION('ref_axis',(-0.166837808361562,-0.485266017453878,0.858301833858907));
#93896=DIRECTION('center_axis',(-0.190809912898503,0.,0.981627005099017));
#93897=DIRECTION('ref_axis',(0.,1.,0.));
#93898=DIRECTION('center_axis',(0.190809912898504,-3.73006669362382E-16,
-0.981627005099017));
#93899=DIRECTION('ref_axis',(0.528539630154271,-0.842668807828817,0.10273820939041));
#93900=DIRECTION('center_axis',(0.,-1.,0.));
#93901=DIRECTION('ref_axis',(0.,0.,-1.));
#93902=DIRECTION('',(-0.190809912898503,0.,0.981627005099017));
#93903=DIRECTION('center_axis',(0.,-1.,0.));
#93904=DIRECTION('ref_axis',(0.0887570095372046,0.,0.996053308441879));
#93905=DIRECTION('',(-0.190809912898503,0.,0.981627005099017));
#93906=DIRECTION('center_axis',(0.,-1.,0.));
#93907=DIRECTION('ref_axis',(0.0814953329512814,0.,0.996673723295222));
#93908=DIRECTION('center_axis',(0.981627005099017,0.,0.190809912898503));
#93909=DIRECTION('ref_axis',(0.,-1.,0.));
#93910=DIRECTION('',(-0.190809912898503,0.,0.981627005099017));
#93911=DIRECTION('center_axis',(0.981627005099017,3.15328006926456E-17,
0.190809912898503));
#93912=DIRECTION('ref_axis',(-0.16672759291197,-0.486305331766721,0.857734827354608));
#93913=DIRECTION('center_axis',(0.981627005099017,-1.66509281342602E-16,
0.190809912898504));
#93914=DIRECTION('ref_axis',(-0.16775489422609,-0.476502997179297,0.86301980808226));
#93915=DIRECTION('center_axis',(0.,1.,0.));
#93916=DIRECTION('ref_axis',(1.,0.,0.));
#93917=DIRECTION('',(-0.190809912898503,0.,0.981627005099017));
#93918=DIRECTION('center_axis',(0.,1.,0.));
#93919=DIRECTION('ref_axis',(0.0450135661808758,0.,0.998986375712742));
#93920=DIRECTION('center_axis',(0.,1.,0.));
#93921=DIRECTION('ref_axis',(0.0391533554628644,0.,0.999233213397152));
#93922=DIRECTION('center_axis',(-0.981627005099017,0.,-0.190809912898503));
#93923=DIRECTION('ref_axis',(-0.190809912898503,0.,0.981627005099017));
#93924=DIRECTION('center_axis',(-0.981627005099017,4.50330787761146E-16,
-0.190809912898504));
#93925=DIRECTION('ref_axis',(-0.163482218098267,-0.515681224446299,0.841038904640705));
#93926=DIRECTION('center_axis',(-0.981627005099017,-1.19343362969677E-16,
-0.190809912898503));
#93927=DIRECTION('ref_axis',(-0.164642701979114,-0.505438873877122,0.847009046857732));
#93928=DIRECTION('center_axis',(0.,-1.,0.));
#93929=DIRECTION('ref_axis',(0.,0.,-1.));
#93930=DIRECTION('',(-0.190809912898503,0.,0.981627005099017));
#93931=DIRECTION('center_axis',(0.,-1.,0.));
#93932=DIRECTION('ref_axis',(0.0116866005388723,0.,0.999931709352116));
#93933=DIRECTION('',(-0.190809912898503,1.012116632187E-14,0.981627005099017));
#93934=DIRECTION('center_axis',(0.,-1.,0.));
#93935=DIRECTION('ref_axis',(0.00646633198153377,0.,0.999979093056802));
#93936=DIRECTION('center_axis',(0.981627005099017,0.,0.190809912898503));
#93937=DIRECTION('ref_axis',(0.,-1.,0.));
#93938=DIRECTION('',(-0.190809912898503,0.,0.981627005099017));
#93939=DIRECTION('center_axis',(0.981627005099017,-1.22647734598186E-16,
0.190809912898504));
#93940=DIRECTION('ref_axis',(-0.167439209291461,-0.479542969202221,0.861395757988492));
#93941=DIRECTION('center_axis',(0.981627005099017,-2.35766262648622E-16,
0.190809912898504));
#93942=DIRECTION('ref_axis',(-0.168407671809334,-0.470136093476487,0.866378040861163));
#93943=DIRECTION('center_axis',(0.,1.,0.));
#93944=DIRECTION('ref_axis',(1.,0.,0.));
#93945=DIRECTION('',(-0.190809912898503,0.,0.981627005099017));
#93946=DIRECTION('center_axis',(0.,1.,0.));
#93947=DIRECTION('ref_axis',(-0.0298461846255247,0.,0.999554503398038));
#93948=DIRECTION('center_axis',(0.,1.,0.));
#93949=DIRECTION('ref_axis',(-0.033817507686259,0.,0.999428024508964));
#93950=DIRECTION('center_axis',(-0.981627005099017,0.,-0.190809912898503));
#93951=DIRECTION('ref_axis',(-0.190809912898503,0.,0.981627005099017));
#93952=DIRECTION('center_axis',(-0.981627005099017,3.03411534837829E-17,
-0.190809912898503));
#93953=DIRECTION('ref_axis',(-0.164163607711793,-0.509701069063094,0.84454433282036));
#93954=DIRECTION('center_axis',(-0.981627005099017,2.04220249255758E-16,
-0.190809912898504));
#93955=DIRECTION('ref_axis',(-0.165267798853502,-0.499804177489587,0.850224875445359));
#93956=DIRECTION('center_axis',(0.,-1.,0.));
#93957=DIRECTION('ref_axis',(0.,0.,-1.));
#93958=DIRECTION('',(-0.190809912898503,0.,0.981627005099017));
#93959=DIRECTION('center_axis',(0.,-1.,0.));
#93960=DIRECTION('ref_axis',(-0.0642416745920277,0.,0.99793437020959));
#93961=DIRECTION('',(-0.190809912898503,0.,0.981627005099017));
#93962=DIRECTION('center_axis',(0.,-1.,0.));
#93963=DIRECTION('ref_axis',(-0.0674811483731083,0.,0.997720549359512));
#93964=DIRECTION('center_axis',(0.981627005099017,0.,0.190809912898503));
#93965=DIRECTION('ref_axis',(0.,-1.,0.));
#93966=DIRECTION('',(-0.190809912898503,0.,0.981627005099017));
#93967=DIRECTION('center_axis',(0.981627005099017,-2.40724768431128E-16,
0.190809912898504));
#93968=DIRECTION('ref_axis',(-0.167904431149187,-0.475054190642086,0.86378910502151));
#93969=DIRECTION('center_axis',(0.981627005099017,-1.01299069034784E-16,
0.190809912898503));
#93970=DIRECTION('ref_axis',(-0.168835339045174,-0.465904025763593,0.868578187077467));
#93971=DIRECTION('center_axis',(0.,1.,0.));
#93972=DIRECTION('ref_axis',(1.,0.,0.));
#93973=DIRECTION('',(-0.190809912898503,0.,0.981627005099017));
#93974=DIRECTION('center_axis',(0.,1.,0.));
#93975=DIRECTION('ref_axis',(-0.103635423533207,0.,0.994615352279007));
#93976=DIRECTION('center_axis',(0.,1.,0.));
#93977=DIRECTION('ref_axis',(-0.105771299395389,0.,0.994390482770331));
#93978=DIRECTION('center_axis',(-0.981627005099017,0.,-0.190809912898503));
#93979=DIRECTION('ref_axis',(-0.190809912898503,0.,0.981627005099017));
#93980=DIRECTION('center_axis',(-0.981627005099017,2.99069503728474E-16,
-0.190809912898504));
#93981=DIRECTION('ref_axis',(-0.164575366240622,-0.506040837499906,0.846662636242535));
#93982=DIRECTION('center_axis',(-0.981627005099017,1.72635908143311E-16,
-0.190809912898504));
#93983=DIRECTION('ref_axis',(-0.165646202300485,-0.496351618609119,0.852171582703586));
#93984=DIRECTION('center_axis',(0.,-1.,0.));
#93985=DIRECTION('ref_axis',(0.,0.,-1.));
#93986=DIRECTION('',(-0.190809912898503,0.,0.981627005099017));
#93987=DIRECTION('center_axis',(0.,-1.,0.));
#93988=DIRECTION('ref_axis',(-0.139070803150795,0.,0.990282440372944));
#93989=DIRECTION('',(-0.190809912898503,0.,0.981627005099017));
#93990=DIRECTION('center_axis',(0.,-1.,0.));
#93991=DIRECTION('ref_axis',(-0.14038574967161,0.,0.99009688479923));
#93992=DIRECTION('center_axis',(0.981627005099017,0.,0.190809912898503));
#93993=DIRECTION('ref_axis',(0.,-1.,0.));
#93994=DIRECTION('',(-0.190809912898503,0.,0.981627005099017));
#93995=DIRECTION('center_axis',(0.981627005099017,-2.9787841376787E-16,
0.190809912898504));
#93996=DIRECTION('ref_axis',(-0.168150432820926,-0.472658284615304,0.865054667594282));
#93997=DIRECTION('center_axis',(0.981627005099017,1.43311947025832E-17,
0.190809912898503));
#93998=DIRECTION('ref_axis',(-0.169061774141528,-0.463643263645911,0.869743088848591));
#93999=DIRECTION('center_axis',(0.,1.,0.));
#94000=DIRECTION('ref_axis',(1.,0.,0.));
#94001=DIRECTION('',(-0.190809912898503,0.,0.981627005099017));
#94002=DIRECTION('center_axis',(0.,1.,0.));
#94003=DIRECTION('ref_axis',(-0.176383802734287,0.,0.984321468897734));
#94004=DIRECTION('center_axis',(0.,1.,0.));
#94005=DIRECTION('ref_axis',(-0.176734827717815,0.,0.984258502971427));
#94006=DIRECTION('center_axis',(-0.981627005099017,0.,-0.190809912898503));
#94007=DIRECTION('ref_axis',(-0.190809912898503,0.,0.981627005099017));
#94008=DIRECTION('center_axis',(-0.981627005099017,-8.91952555246029E-17,
-0.190809912898503));
#94009=DIRECTION('ref_axis',(-0.164741217100846,-0.504556436150305,0.847515860693731));
#94010=DIRECTION('center_axis',(-0.981627005099017,2.00273181403031E-16,
-0.190809912898504));
#94011=DIRECTION('ref_axis',(-0.165798759222807,-0.494950627486599,0.852956416114446));
#94012=DIRECTION('center_axis',(0.,-1.,0.));
#94013=DIRECTION('ref_axis',(0.,0.,-1.));
#94014=DIRECTION('',(-0.190809912898503,0.,0.981627005099017));
#94015=DIRECTION('center_axis',(0.,-1.,0.));
#94016=DIRECTION('ref_axis',(-0.212823105190621,0.,0.977090745988837));
#94017=DIRECTION('',(-0.190809912898503,0.,0.981627005099017));
#94018=DIRECTION('center_axis',(0.,-1.,0.));
#94019=DIRECTION('ref_axis',(-0.212267586570765,0.,0.977211579798061));
#94020=DIRECTION('center_axis',(0.981627005099017,0.,0.190809912898503));
#94021=DIRECTION('ref_axis',(0.,-1.,0.));
#94022=DIRECTION('',(-0.190809912898503,0.,0.981627005099017));
#94023=DIRECTION('center_axis',(0.981627005099017,-2.08165815051713E-16,
0.190809912898504));
#94024=DIRECTION('ref_axis',(-0.168190918116109,-0.472262480491401,0.865262945342842));
#94025=DIRECTION('center_axis',(0.981627005099017,-2.14621618024828E-16,
0.190809912898504));
#94026=DIRECTION('ref_axis',(-0.169099058653206,-0.463269660125623,0.869934900075684));
#94027=DIRECTION('center_axis',(0.,1.,0.));
#94028=DIRECTION('ref_axis',(1.,0.,0.));
#94029=DIRECTION('',(-0.190809912898503,0.,0.981627005099017));
#94030=DIRECTION('center_axis',(0.,1.,0.));
#94031=DIRECTION('ref_axis',(-0.248103134940545,0.,0.968733624084905));
#94032=DIRECTION('center_axis',(0.,1.,0.));
#94033=DIRECTION('ref_axis',(-0.246718789670631,0.,0.969087116219929));
#94034=DIRECTION('center_axis',(-0.981627005099017,0.,-0.190809912898503));
#94035=DIRECTION('ref_axis',(-0.190809912898503,0.,0.981627005099017));
#94036=DIRECTION('center_axis',(-0.981627005099017,1.49032924732936E-16,
-0.190809912898503));
#94037=DIRECTION('ref_axis',(-0.164670397132728,-0.505191006835612,0.84715152536047));
#94038=DIRECTION('center_axis',(-0.981627005099017,1.43398714849782E-17,
-0.190809912898503));
#94039=DIRECTION('ref_axis',(-0.165733605986292,-0.495549598052214,0.852621233442535));
#94040=DIRECTION('center_axis',(0.,-1.,0.));
#94041=DIRECTION('ref_axis',(0.,0.,-1.));
#94042=DIRECTION('',(-0.190809912898503,0.,0.981627005099017));
#94043=DIRECTION('center_axis',(0.,-1.,0.));
#94044=DIRECTION('ref_axis',(-0.285502227028518,0.,0.95837804563844));
#94045=DIRECTION('',(-0.190809912898503,0.,0.981627005099017));
#94046=DIRECTION('center_axis',(0.,-1.,0.));
#94047=DIRECTION('ref_axis',(-0.28312994844639,0.,0.959081556642992));
#94048=DIRECTION('center_axis',(0.981627005099017,0.,0.190809912898503));
#94049=DIRECTION('ref_axis',(0.,-1.,0.));
#94050=DIRECTION('',(-0.190809912898503,0.,0.981627005099017));
#94051=DIRECTION('center_axis',(0.981627005099017,-7.48461333200017E-17,
0.190809912898503));
#94052=DIRECTION('ref_axis',(-0.168028098915109,-0.473851694839214,0.864425317348456));
#94053=DIRECTION('center_axis',(0.981627005099017,-2.73617183612082E-16,
0.190809912898504));
#94054=DIRECTION('ref_axis',(-0.168949145239597,-0.46476952090078,0.869163666270323));
#94055=DIRECTION('center_axis',(0.,1.,0.));
#94056=DIRECTION('ref_axis',(1.,0.,0.));
#94057=DIRECTION('',(-0.190809912898503,0.,0.981627005099017));
#94058=DIRECTION('center_axis',(0.,1.,0.));
#94059=DIRECTION('ref_axis',(-0.318788385159717,0.,0.94782591518024));
#94060=DIRECTION('center_axis',(0.,1.,0.));
#94061=DIRECTION('ref_axis',(-0.315718624595745,0.,0.948852860080724));
#94062=DIRECTION('center_axis',(-0.981627005099017,0.,-0.190809912898503));
#94063=DIRECTION('ref_axis',(-0.190809912898503,0.,0.981627005099017));
#94064=DIRECTION('center_axis',(-0.981627005099017,4.52028940915851E-17,
-0.190809912898503));
#94065=DIRECTION('ref_axis',(-0.164358984279519,-0.50796874572249,0.845549453110653));
#94066=DIRECTION('center_axis',(-0.981627005099017,1.30427605301434E-16,
-0.190809912898504));
#94067=DIRECTION('ref_axis',(-0.165447286436924,-0.498170497353102,0.851148254405554));
#94068=DIRECTION('center_axis',(0.,-1.,0.));
#94069=DIRECTION('ref_axis',(0.,0.,-1.));
#94070=DIRECTION('',(-0.190809912898503,0.,0.981627005099017));
#94071=DIRECTION('center_axis',(0.,-1.,0.));
#94072=DIRECTION('ref_axis',(-0.357093458083529,0.,0.934068660321042));
#94073=DIRECTION('',(-0.190809912898503,0.,0.981627005099017));
#94074=DIRECTION('center_axis',(0.,-1.,0.));
#94075=DIRECTION('ref_axis',(-0.352959570505503,0.,0.935638574230761));
#94076=DIRECTION('center_axis',(0.981627005099017,0.,0.190809912898503));
#94077=DIRECTION('ref_axis',(0.,-1.,0.));
#94078=DIRECTION('',(-0.190809912898503,0.,0.981627005099017));
#94079=DIRECTION('center_axis',(0.981627005099017,-4.40793738003239E-16,
0.190809912898504));
#94080=DIRECTION('ref_axis',(-0.167653005397309,-0.477486904547474,0.862495638114722));
#94081=DIRECTION('center_axis',(0.981627005099017,1.46141627281437E-16,
0.190809912898503));
#94082=DIRECTION('ref_axis',(-0.168604119842488,-0.468198184683616,0.867388673335724));
#94083=DIRECTION('center_axis',(0.,1.,0.));
#94084=DIRECTION('ref_axis',(1.,0.,0.));
#94085=DIRECTION('',(-0.190809912898503,0.,0.981627005099017));
#94086=DIRECTION('center_axis',(0.,1.,0.));
#94087=DIRECTION('ref_axis',(-0.388417251131186,0.,0.921483607571884));
#94088=DIRECTION('center_axis',(0.,1.,0.));
#94089=DIRECTION('ref_axis',(-0.38371415291867,0.,0.923451920161471));
#94090=DIRECTION('center_axis',(-0.981627005099017,0.,-0.190809912898503));
#94091=DIRECTION('ref_axis',(-0.190809912898503,0.,0.981627005099017));
#94092=DIRECTION('center_axis',(-0.981627005099017,3.22716239961749E-16,
-0.190809912898504));
#94093=DIRECTION('ref_axis',(-0.163789338595868,-0.512997515374394,0.84261889474544));
#94094=DIRECTION('center_axis',(-0.981627005099017,3.39688902299908E-16,
-0.190809912898504));
#94095=DIRECTION('ref_axis',(-0.164924280814687,-0.502911144781707,0.848457637158221));
#94096=DIRECTION('center_axis',(0.,-1.,0.));
#94097=DIRECTION('ref_axis',(0.,0.,-1.));
#94098=DIRECTION('',(-0.190809912898503,0.,0.981627005099017));
#94099=DIRECTION('center_axis',(0.,-1.,0.));
#94100=DIRECTION('ref_axis',(-0.427562437492918,0.,0.903985819603999));
#94101=DIRECTION('',(-0.190809912898503,0.,0.981627005099017));
#94102=DIRECTION('center_axis',(0.,-1.,0.));
#94103=DIRECTION('ref_axis',(-0.421725528224158,0.,0.906723540470884));
#94104=DIRECTION('center_axis',(0.981627005099017,0.,0.190809912898503));
#94105=DIRECTION('ref_axis',(0.,-1.,0.));
#94106=DIRECTION('',(-0.190809912898503,0.,0.981627005099017));
#94107=DIRECTION('center_axis',(0.981627005099017,-4.20468084671077E-16,
0.190809912898504));
#94108=DIRECTION('ref_axis',(-0.167044212206533,-0.483311793041112,0.859363684289535));
#94109=DIRECTION('center_axis',(0.981627005099017,4.48762447131239E-17,
0.190809912898503));
#94110=DIRECTION('ref_axis',(-0.168045126361751,-0.473685818224829,0.864512915530322));
#94111=DIRECTION('center_axis',(0.,1.,0.));
#94112=DIRECTION('ref_axis',(1.,0.,0.));
#94113=DIRECTION('',(-0.190809912898503,0.,0.981627005099017));
#94114=DIRECTION('center_axis',(0.,1.,0.));
#94115=DIRECTION('ref_axis',(-0.456948248125761,0.,0.889493281894134));
#94116=DIRECTION('center_axis',(0.,1.,0.));
#94117=DIRECTION('ref_axis',(-0.450667931431808,0.,0.892691668819069));
#94118=DIRECTION('center_axis',(-0.981627005099017,0.,-0.190809912898503));
#94119=DIRECTION('ref_axis',(-0.190809912898503,0.,0.981627005099017));
#94120=DIRECTION('center_axis',(-0.981627005099017,1.5819052248506E-17,
-0.190809912898503));
#94121=DIRECTION('ref_axis',(-0.162927501749981,-0.520480818454586,0.838185150664431));
#94122=DIRECTION('center_axis',(-0.981627005099017,1.21485874416176E-16,
-0.190809912898503));
#94123=DIRECTION('ref_axis',(-0.164134821046406,-0.509955637360102,0.844396239004365));
#94124=DIRECTION('center_axis',(0.,1.,0.));
#94125=DIRECTION('ref_axis',(1.,0.,0.));
#94126=DIRECTION('',(-0.190809912898503,0.,0.981627005099017));
#94127=DIRECTION('',(-0.981627005099017,0.,-0.190809912898503));
#94128=DIRECTION('center_axis',(0.,1.,0.));
#94129=DIRECTION('ref_axis',(-0.523385314028976,0.,0.852096129001177));
#94130=DIRECTION('',(-0.190809912898503,0.,0.981627005099017));
#94131=DIRECTION('center_axis',(0.,1.,0.));
#94132=DIRECTION('ref_axis',(-0.516521998262274,0.,0.856273919555622));
#94133=DIRECTION('center_axis',(-0.981627005099017,0.,-0.190809912898503));
#94134=DIRECTION('ref_axis',(-0.190809912898503,0.,0.981627005099017));
#94135=DIRECTION('',(-0.19080991289849,0.,0.98162700509902));
#94136=DIRECTION('',(0.,-1.,0.));
#94137=DIRECTION('center_axis',(-0.981627005099017,2.04948424643113E-16,
-0.190809912898504));
#94138=DIRECTION('ref_axis',(-0.163030388947302,-0.519595181164497,0.838714456767215));
#94139=DIRECTION('center_axis',(0.,-1.,0.));
#94140=DIRECTION('ref_axis',(0.,0.,-1.));
#94141=DIRECTION('',(-0.190809912898503,0.,0.981627005099017));
#94142=DIRECTION('',(0.981627005099017,0.,0.190809912898503));
#94143=DIRECTION('center_axis',(0.,-1.,0.));
#94144=DIRECTION('ref_axis',(-0.489376531975999,0.,0.87207259442729));
#94145=DIRECTION('center_axis',(0.981627005099017,0.,0.190809912898503));
#94146=DIRECTION('ref_axis',(0.,-1.,0.));
#94147=DIRECTION('center_axis',(0.981627005099017,3.22191216748114E-17,
0.190809912898503));
#94148=DIRECTION('ref_axis',(-0.166164628408473,-0.491569135480225,0.854838640510066));
#94149=DIRECTION('',(0.,1.,0.));
#94150=DIRECTION('center_axis',(0.981627005099017,2.00892259541186E-16,
0.190809912898503));
#94151=DIRECTION('ref_axis',(-0.167239670018067,-0.481451652480913,0.860369222540908));
#94152=DIRECTION('center_axis',(-0.190809912898503,0.,0.981627005099017));
#94153=DIRECTION('ref_axis',(0.,1.,0.));
#94154=DIRECTION('center_axis',(0.190809912898503,-3.49693752527234E-17,
-0.981627005099017));
#94155=DIRECTION('ref_axis',(-0.483557533970894,-0.870251193216613,-0.0939945319954744));
#94156=DIRECTION('center_axis',(0.,1.,0.));
#94157=DIRECTION('ref_axis',(1.,0.,0.));
#94158=DIRECTION('',(-0.190809912898503,0.,0.981627005099017));
#94159=DIRECTION('',(-0.981627005099017,0.,-0.190809912898503));
#94160=DIRECTION('center_axis',(0.,1.,0.));
#94161=DIRECTION('ref_axis',(-0.666090131706357,0.,0.745871259966094));
#94162=DIRECTION('',(-0.190809912898503,0.,0.981627005099017));
#94163=DIRECTION('center_axis',(0.,1.,0.));
#94164=DIRECTION('ref_axis',(-0.668602144346241,0.,0.743620314794861));
#94165=DIRECTION('center_axis',(-0.981627005099017,0.,-0.190809912898503));
#94166=DIRECTION('ref_axis',(-0.190809912898503,0.,0.981627005099017));
#94167=DIRECTION('',(-0.19080991289849,0.,0.98162700509902));
#94168=DIRECTION('',(0.,-1.,0.));
#94169=DIRECTION('center_axis',(-0.981627005099017,1.42070106006851E-16,
-0.190809912898504));
#94170=DIRECTION('ref_axis',(-0.178705808705077,-0.350495021766094,0.91935709800504));
#94171=DIRECTION('center_axis',(0.,-1.,0.));
#94172=DIRECTION('ref_axis',(0.,0.,-1.));
#94173=DIRECTION('',(-0.190809912898503,0.,0.981627005099017));
#94174=DIRECTION('',(0.981627005099017,0.,0.190809912898503));
#94175=DIRECTION('center_axis',(0.,-1.,0.));
#94176=DIRECTION('ref_axis',(-0.644082689417421,0.,0.76495587401681));
#94177=DIRECTION('center_axis',(0.981627005099017,0.,0.190809912898503));
#94178=DIRECTION('ref_axis',(0.,-1.,0.));
#94179=DIRECTION('center_axis',(0.981627005099017,-7.65116657223729E-17,
0.190809912898504));
#94180=DIRECTION('ref_axis',(-0.181063354814559,-0.315516578947016,0.931485560786032));
#94181=DIRECTION('',(-2.42927638559096E-14,1.,1.24974812195102E-13));
#94182=DIRECTION('center_axis',(0.981627005099017,-5.46289132020529E-17,
0.190809912898503));
#94183=DIRECTION('ref_axis',(-0.181543217971292,-0.307849891233687,0.933954230396776));
#94184=DIRECTION('center_axis',(-0.190809912898503,0.,0.981627005099017));
#94185=DIRECTION('ref_axis',(0.,1.,0.));
#94186=DIRECTION('center_axis',(0.190809912898504,3.26380835692085E-16,
-0.981627005099017));
#94187=DIRECTION('ref_axis',(-0.820923255345953,-0.548289841013012,-0.159572112457437));
#94188=DIRECTION('center_axis',(0.981627005099017,0.,0.190809912898503));
#94189=DIRECTION('ref_axis',(0.,-1.,0.));
#94190=DIRECTION('',(-0.190809912898503,0.,0.981627005099017));
#94191=DIRECTION('center_axis',(0.981627005099017,-1.24331456798856E-16,
0.190809912898504));
#94192=DIRECTION('ref_axis',(-0.185131631876501,-0.242140630354711,0.952414927439804));
#94193=DIRECTION('',(-0.190809912898503,0.,0.981627005099017));
#94194=DIRECTION('center_axis',(0.981627005099017,-1.18362645271115E-16,
0.190809912898504));
#94195=DIRECTION('ref_axis',(-0.185408204469832,-0.236256893272313,0.953837762985188));
#94196=DIRECTION('center_axis',(0.,1.,0.));
#94197=DIRECTION('ref_axis',(1.,0.,0.));
#94198=DIRECTION('',(-0.190809912898503,0.,0.981627005099017));
#94199=DIRECTION('center_axis',(0.,1.,0.));
#94200=DIRECTION('ref_axis',(-0.670325070726556,0.,0.742067584223591));
#94201=DIRECTION('center_axis',(0.,1.,0.));
#94202=DIRECTION('ref_axis',(-0.661396304967786,0.,0.75003661762274));
#94203=DIRECTION('center_axis',(-0.981627005099017,0.,-0.190809912898503));
#94204=DIRECTION('ref_axis',(-0.190809912898503,0.,0.981627005099017));
#94205=DIRECTION('',(-0.190809912898503,0.,0.981627005099017));
#94206=DIRECTION('center_axis',(-0.981627005099017,1.29599606305268E-16,
-0.190809912898504));
#94207=DIRECTION('ref_axis',(-0.18291500399328,-0.284674558222307,0.941011422467906));
#94208=DIRECTION('center_axis',(-0.981627005099017,3.78853616018271E-17,
-0.190809912898503));
#94209=DIRECTION('ref_axis',(-0.183317340516521,-0.277475225564888,0.943081254115288));
#94210=DIRECTION('center_axis',(0.,-1.,0.));
#94211=DIRECTION('ref_axis',(0.,0.,-1.));
#94212=DIRECTION('center_axis',(0.,-1.,0.));
#94213=DIRECTION('ref_axis',(-0.644808210944829,0.,0.76434440607499));
#94214=DIRECTION('center_axis',(0.,-1.,0.));
#94215=DIRECTION('ref_axis',(-0.636173251407937,0.,0.771546235939917));
#94216=DIRECTION('center_axis',(0.,-1.,0.));
#94217=DIRECTION('ref_axis',(0.,0.,-1.));
#94218=DIRECTION('',(-0.190809912898503,0.,0.981627005099017));
#94219=DIRECTION('center_axis',(0.,-1.,0.));
#94220=DIRECTION('ref_axis',(-0.638671662809062,0.,0.769479374073606));
#94221=DIRECTION('',(-0.190809912898503,0.,0.981627005099017));
#94222=DIRECTION('center_axis',(0.,-1.,0.));
#94223=DIRECTION('ref_axis',(-0.630378608858621,0.,0.776287839331178));
#94224=DIRECTION('center_axis',(0.981627005099017,0.,0.190809912898503));
#94225=DIRECTION('ref_axis',(0.,-1.,0.));
#94226=DIRECTION('',(-0.190809912898503,0.,0.981627005099017));
#94227=DIRECTION('center_axis',(0.981627005099017,-9.56395821529661E-17,
0.190809912898504));
#94228=DIRECTION('ref_axis',(-0.188073006346447,-0.168764681762398,0.967546911768854));
#94229=DIRECTION('center_axis',(0.981627005099017,-2.23068062241716E-16,
0.190809912898504));
#94230=DIRECTION('ref_axis',(-0.18820530720141,-0.164663895310999,0.968227537267057));
#94231=DIRECTION('center_axis',(0.,1.,0.));
#94232=DIRECTION('ref_axis',(1.,0.,0.));
#94233=DIRECTION('',(-0.190809912898503,0.,0.981627005099017));
#94234=DIRECTION('center_axis',(0.,1.,0.));
#94235=DIRECTION('ref_axis',(-0.664925875210949,0.,0.746909352247616));
#94236=DIRECTION('center_axis',(0.,1.,0.));
#94237=DIRECTION('ref_axis',(-0.656292015446062,0.,0.75450698503178));
#94238=DIRECTION('center_axis',(-0.981627005099017,0.,-0.190809912898503));
#94239=DIRECTION('ref_axis',(-0.190809912898503,0.,0.981627005099017));
#94240=DIRECTION('center_axis',(-0.981627005099017,4.48614021825927E-17,
-0.190809912898503));
#94241=DIRECTION('ref_axis',(-0.186564938338183,-0.209760200795403,0.959788613156638));
#94242=DIRECTION('center_axis',(-0.981627005099017,-2.84140212013703E-17,
-0.190809912898503));
#94243=DIRECTION('ref_axis',(-0.186779220325047,-0.204455429363609,0.960890992911532));
#94244=DIRECTION('center_axis',(0.,-1.,0.));
#94245=DIRECTION('ref_axis',(0.,0.,-1.));
#94246=DIRECTION('',(-0.190809912898503,0.,0.981627005099017));
#94247=DIRECTION('center_axis',(0.,-1.,0.));
#94248=DIRECTION('ref_axis',(-0.634540109712014,0.,0.772889933410098));
#94249=DIRECTION('',(-0.190809912898503,0.,0.981627005099017));
#94250=DIRECTION('center_axis',(0.,-1.,0.));
#94251=DIRECTION('ref_axis',(-0.626472251574789,0.,0.779443723437949));
#94252=DIRECTION('center_axis',(0.981627005099017,0.,0.190809912898503));
#94253=DIRECTION('ref_axis',(0.,-1.,0.));
#94254=DIRECTION('',(-0.190809912898503,0.,0.981627005099017));
#94255=DIRECTION('center_axis',(0.981627005099017,2.15189059844174E-17,
0.190809912898503));
#94256=DIRECTION('ref_axis',(-0.189939838479203,-0.0953887331700394,0.977150882588103));
#94257=DIRECTION('center_axis',(0.981627005099017,-2.95906613177786E-17,
0.190809912898504));
#94258=DIRECTION('ref_axis',(-0.189981699417399,-0.0930708973497062,0.977366237371129));
#94259=DIRECTION('center_axis',(0.,1.,0.));
#94260=DIRECTION('ref_axis',(1.,0.,0.));
#94261=DIRECTION('',(-0.190809912898513,0.,0.981627005099015));
#94262=DIRECTION('center_axis',(0.,1.,0.));
#94263=DIRECTION('ref_axis',(-0.661550435497198,0.,0.749900674285246));
#94264=DIRECTION('center_axis',(0.,1.,0.));
#94265=DIRECTION('ref_axis',(-0.653097727316854,0.,0.757273635202996));
#94266=DIRECTION('center_axis',(-0.981627005099017,0.,-0.190809912898503));
#94267=DIRECTION('ref_axis',(-0.190809912898503,0.,0.981627005099017));
#94268=DIRECTION('center_axis',(-0.981627005099017,1.14645805577737E-16,
-0.190809912898504));
#94269=DIRECTION('ref_axis',(-0.189067167669161,-0.1348458433685,0.97266140287142));
#94270=DIRECTION('center_axis',(-0.981627005099017,9.47134040045677E-17,
-0.190809912898504));
#94271=DIRECTION('ref_axis',(-0.189154580960868,-0.131435633162295,0.973111103028192));
#94272=DIRECTION('center_axis',(0.,-1.,0.));
#94273=DIRECTION('ref_axis',(0.,0.,-1.));
#94274=DIRECTION('',(-0.190809912898503,0.,0.981627005099017));
#94275=DIRECTION('center_axis',(0.,-1.,0.));
#94276=DIRECTION('ref_axis',(-0.632255301211611,0.,0.774760113899661));
#94277=DIRECTION('',(-0.190809912898503,0.,0.981627005099017));
#94278=DIRECTION('center_axis',(0.,-1.,0.));
#94279=DIRECTION('ref_axis',(-0.624310263777235,0.,0.781176481047912));
#94280=DIRECTION('center_axis',(0.981627005099017,0.,0.190809912898503));
#94281=DIRECTION('ref_axis',(0.,-1.,0.));
#94282=DIRECTION('',(-0.190809912898503,0.,0.981627005099017));
#94283=DIRECTION('center_axis',(0.981627005099017,-6.57522127301642E-18,
0.190809912898504));
#94284=DIRECTION('ref_axis',(-0.190763677615005,-0.0220127845777007,0.981389146372597));
#94285=DIRECTION('center_axis',(0.981627005099017,1.1381023583761E-18,0.190809912898503));
#94286=DIRECTION('ref_axis',(-0.190765897499961,-0.0214778993883992,0.981400566633674));
#94287=DIRECTION('center_axis',(0.,1.,0.));
#94288=DIRECTION('ref_axis',(1.,0.,0.));
#94289=DIRECTION('',(-0.190809912898503,0.,0.981627005099017));
#94290=DIRECTION('center_axis',(0.,1.,0.));
#94291=DIRECTION('ref_axis',(-0.660073373181361,0.,0.751201132864548));
#94292=DIRECTION('center_axis',(0.,1.,0.));
#94293=DIRECTION('ref_axis',(-0.651699160648413,0.,0.758477556695091));
#94294=DIRECTION('center_axis',(-0.981627005099017,0.,-0.190809912898503));
#94295=DIRECTION('ref_axis',(-0.190809912898503,0.,0.981627005099017));
#94296=DIRECTION('center_axis',(-0.981627005099017,1.99384009700412E-17,
-0.190809912898504));
#94297=DIRECTION('ref_axis',(-0.190466930740712,-0.0599314859415386,0.979862523666995));
#94298=DIRECTION('center_axis',(-0.981627005099017,-3.07818563014845E-17,
-0.190809912898503));
#94299=DIRECTION('ref_axis',(-0.19048407385867,-0.0584158369610204,0.979950716923228));
#94300=DIRECTION('center_axis',(0.,1.,0.));
#94301=DIRECTION('ref_axis',(1.,0.,0.));
#94302=DIRECTION('',(-0.190809912898503,0.,0.981627005099017));
#94303=DIRECTION('center_axis',(0.,1.,0.));
#94304=DIRECTION('ref_axis',(0.358991707710534,0.,0.933340749027425));
#94305=DIRECTION('',(-0.190809912898503,0.,0.981627005099017));
#94306=DIRECTION('center_axis',(0.,1.,0.));
#94307=DIRECTION('ref_axis',(0.347885431423932,0.,0.937537053456014));
#94308=DIRECTION('center_axis',(-0.981627005099017,0.,-0.190809912898503));
#94309=DIRECTION('ref_axis',(-0.190809912898503,0.,0.981627005099017));
#94310=DIRECTION('',(-0.190809912898503,0.,0.981627005099017));
#94311=DIRECTION('center_axis',(-0.981627005099017,2.58515321514558E-18,
-0.190809912898503));
#94312=DIRECTION('ref_axis',(-0.190454140668356,-0.0610376803135203,0.979796724777248));
#94313=DIRECTION('center_axis',(-0.981627005099017,4.65783098075688E-17,
-0.190809912898504));
#94314=DIRECTION('ref_axis',(-0.190472551870653,-0.0594387870801789,0.979891441729296));
#94315=DIRECTION('center_axis',(0.,-1.,0.));
#94316=DIRECTION('ref_axis',(0.,0.,-1.));
#94317=DIRECTION('',(-0.190809912898503,0.,0.981627005099017));
#94318=DIRECTION('',(0.981627005099017,-5.774756729131E-14,0.190809912898503));
#94319=DIRECTION('center_axis',(0.,-1.,0.));
#94320=DIRECTION('ref_axis',(0.394942270734479,0.,0.918705939235778));
#94321=DIRECTION('center_axis',(0.,-1.,0.));
#94322=DIRECTION('ref_axis',(0.383559494744058,0.,0.923516168776531));
#94323=DIRECTION('center_axis',(0.981627005099017,0.,0.190809912898503));
#94324=DIRECTION('ref_axis',(0.,-1.,0.));
#94325=DIRECTION('center_axis',(0.981627005099017,-8.15668315070832E-18,
0.190809912898504));
#94326=DIRECTION('ref_axis',(-0.190757335946959,-0.0234737412435989,0.98135652148159));
#94327=DIRECTION('',(0.,1.,0.));
#94328=DIRECTION('center_axis',(0.981627005099017,1.09286110344539E-17,
0.190809912898503));
#94329=DIRECTION('ref_axis',(-0.190760187776512,-0.0228283311400105,0.98137119279956));
#94330=DIRECTION('center_axis',(-0.190809912898503,0.,0.981627005099017));
#94331=DIRECTION('ref_axis',(0.,1.,0.));
#94332=DIRECTION('center_axis',(0.190809912898504,-6.70246359010532E-17,
-0.981627005099017));
#94333=DIRECTION('ref_axis',(0.978360591987681,-0.0815109057565992,0.190174983339693));
#94334=DIRECTION('center_axis',(-0.981627005099017,0.,-0.190809912898503));
#94335=DIRECTION('ref_axis',(-0.190809912898503,0.,0.981627005099017));
#94336=DIRECTION('',(-0.190809912898503,0.,0.981627005099017));
#94337=DIRECTION('center_axis',(-0.981627005099017,-5.17030643029117E-17,
-0.190809912898503));
#94338=DIRECTION('ref_axis',(-0.189001929486472,-0.137334780705401,0.972325783191514));
#94339=DIRECTION('',(-0.190809912898503,0.,0.981627005099017));
#94340=DIRECTION('center_axis',(-0.981627005099017,1.02962579574626E-16,
-0.190809912898504));
#94341=DIRECTION('ref_axis',(-0.189095833571211,-0.133737270930404,0.972808875417004));
#94342=DIRECTION('center_axis',(0.,-1.,0.));
#94343=DIRECTION('ref_axis',(0.,0.,-1.));
#94344=DIRECTION('',(-0.190809912898503,0.,0.981627005099017));
#94345=DIRECTION('',(0.981627005099017,0.,0.190809912898503));
#94346=DIRECTION('center_axis',(0.,-1.,0.));
#94347=DIRECTION('ref_axis',(0.387469259730511,0.,0.921882624179396));
#94348=DIRECTION('center_axis',(0.,-1.,0.));
#94349=DIRECTION('ref_axis',(0.386800467114359,0.,0.922163433801251));
#94350=DIRECTION('center_axis',(0.981627005099017,0.,0.190809912898503));
#94351=DIRECTION('ref_axis',(0.,-1.,0.));
#94352=DIRECTION('',(-0.190809912898503,0.,0.981627005099017));
#94353=DIRECTION('',(0.,1.,0.));
#94354=DIRECTION('center_axis',(0.981627005099017,1.28571894522987E-17,
0.190809912898503));
#94355=DIRECTION('ref_axis',(-0.189874012029069,-0.0989227682733557,0.976812236549646));
#94356=DIRECTION('center_axis',(0.,1.,0.));
#94357=DIRECTION('ref_axis',(1.,0.,0.));
#94358=DIRECTION('center_axis',(0.,1.,0.));
#94359=DIRECTION('ref_axis',(0.36095771605842,0.,0.932582182554379));
#94360=DIRECTION('',(-0.981627005099017,0.,-0.190809912898503));
#94361=DIRECTION('center_axis',(0.,1.,0.));
#94362=DIRECTION('ref_axis',(0.349735592176022,0.,0.93684844855787));
#94363=DIRECTION('center_axis',(-0.190809912898503,0.,0.981627005099017));
#94364=DIRECTION('ref_axis',(0.,1.,0.));
#94365=DIRECTION('center_axis',(0.190809912898504,-8.15952089230212E-17,
-0.981627005099017));
#94366=DIRECTION('ref_axis',(0.970679932351344,-0.148928067215399,0.188682006894872));
#94367=DIRECTION('center_axis',(-0.981627005099017,0.,-0.190809912898503));
#94368=DIRECTION('ref_axis',(-0.190809912898503,0.,0.981627005099017));
#94369=DIRECTION('',(-0.190809912898503,0.,0.981627005099017));
#94370=DIRECTION('center_axis',(-0.981627005099017,-5.17030643029117E-18,
-0.190809912898503));
#94371=DIRECTION('ref_axis',(-0.186404919780389,-0.213631881097296,0.958965393150607));
#94372=DIRECTION('',(-0.190809912898503,0.,0.981627005099017));
#94373=DIRECTION('center_axis',(-0.981627005099017,2.94178798784645E-17,
-0.190809912898503));
#94374=DIRECTION('ref_axis',(-0.186635225155084,-0.208035754780595,0.960150205678351));
#94375=DIRECTION('center_axis',(0.,-1.,0.));
#94376=DIRECTION('ref_axis',(0.,0.,-1.));
#94377=DIRECTION('',(-0.190809912898503,0.,0.981627005099017));
#94378=DIRECTION('',(0.981627005099017,0.,0.190809912898503));
#94379=DIRECTION('center_axis',(0.,-1.,0.));
#94380=DIRECTION('ref_axis',(0.373637525799342,0.,0.927574794458402));
#94381=DIRECTION('center_axis',(0.,-1.,0.));
#94382=DIRECTION('ref_axis',(0.392669915561929,0.,0.919679475367689));
#94383=DIRECTION('center_axis',(0.981627005099017,0.,0.190809912898503));
#94384=DIRECTION('ref_axis',(0.,-1.,0.));
#94385=DIRECTION('',(-0.190809912898503,0.,0.981627005099017));
#94386=DIRECTION('',(0.,1.,0.));
#94387=DIRECTION('center_axis',(0.981627005099017,4.11430062473558E-17,
0.190809912898503));
#94388=DIRECTION('ref_axis',(-0.187864833462401,-0.175017205406708,0.966475960466566));
#94389=DIRECTION('center_axis',(0.,1.,0.));
#94390=DIRECTION('ref_axis',(1.,0.,0.));
#94391=DIRECTION('center_axis',(0.,1.,0.));
#94392=DIRECTION('ref_axis',(0.365458588656494,0.,0.930827599492626));
#94393=DIRECTION('',(-0.981627005099017,0.,-0.190809912898503));
#94394=DIRECTION('center_axis',(0.,1.,0.));
#94395=DIRECTION('ref_axis',(0.353968321307143,0.,0.935257412433071));
#94396=DIRECTION('center_axis',(-0.190809912898503,0.,0.981627005099017));
#94397=DIRECTION('ref_axis',(0.,1.,0.));
#94398=DIRECTION('center_axis',(0.190809912898502,2.03988022307553E-16,
-0.981627005099017));
#94399=DIRECTION('ref_axis',(0.94693889934147,-0.263488118919596,0.184067194530089));
#94400=DIRECTION('center_axis',(0.,1.,0.));
#94401=DIRECTION('ref_axis',(1.,0.,0.));
#94402=DIRECTION('',(-0.190809912898503,0.,0.981627005099017));
#94403=DIRECTION('center_axis',(0.,1.,0.));
#94404=DIRECTION('ref_axis',(0.184145244684996,0.,0.982899043065921));
#94405=DIRECTION('',(-0.190809912898503,0.,0.981627005099017));
#94406=DIRECTION('center_axis',(0.,1.,0.));
#94407=DIRECTION('ref_axis',(0.175315692747643,0.,0.984512269032953));
#94408=DIRECTION('center_axis',(-0.981627005099017,0.,-0.190809912898503));
#94409=DIRECTION('ref_axis',(-0.190809912898503,0.,0.981627005099017));
#94410=DIRECTION('',(-0.190809912898503,0.,0.981627005099017));
#94411=DIRECTION('center_axis',(-0.981627005099017,-6.70372400852628E-17,
-0.190809912898503));
#94412=DIRECTION('ref_axis',(-0.168720726956303,-0.467043009411895,0.867988561937781));
#94413=DIRECTION('center_axis',(-0.981627005099017,3.04952953295968E-16,
-0.190809912898504));
#94414=DIRECTION('ref_axis',(-0.169713673567315,-0.457054963856906,0.873096803921564));
#94415=DIRECTION('center_axis',(0.,-1.,0.));
#94416=DIRECTION('ref_axis',(0.,0.,-1.));
#94417=DIRECTION('',(-0.190809912898503,0.,0.981627005099017));
#94418=DIRECTION('',(0.981627005099017,0.,0.190809912898503));
#94419=DIRECTION('center_axis',(0.,-1.,0.));
#94420=DIRECTION('ref_axis',(0.211589721837698,0.,0.977358577806859));
#94421=DIRECTION('center_axis',(0.,-1.,0.));
#94422=DIRECTION('ref_axis',(0.218730261134039,0.,0.975785362087501));
#94423=DIRECTION('center_axis',(0.981627005099017,0.,0.190809912898503));
#94424=DIRECTION('ref_axis',(0.,-1.,0.));
#94425=DIRECTION('center_axis',(0.981627005099017,-2.83825609674828E-16,
0.190809912898504));
#94426=DIRECTION('ref_axis',(-0.171498597492433,-0.43837346986139,0.882279395645061));
#94427=DIRECTION('',(0.,1.,0.));
#94428=DIRECTION('center_axis',(0.981627005099017,-3.12650905815778E-16,
0.190809912898504));
#94429=DIRECTION('ref_axis',(-0.172381261221582,-0.428759238128314,0.886820284217318));
#94430=DIRECTION('center_axis',(-0.190809912898503,0.,0.981627005099017));
#94431=DIRECTION('ref_axis',(0.,1.,0.));
#94432=DIRECTION('center_axis',(0.190809912898504,-6.87731046636893E-16,
-0.981627005099017));
#94433=DIRECTION('ref_axis',(0.640994870612618,-0.757364550955772,0.12459740287773));
#94434=DIRECTION('center_axis',(0.,-1.,0.));
#94435=DIRECTION('ref_axis',(0.,0.,-1.));
#94436=DIRECTION('',(-0.190809912898503,1.255691120406E-14,0.981627005099017));
#94437=DIRECTION('center_axis',(0.,-1.,0.));
#94438=DIRECTION('ref_axis',(0.152737602003591,0.,0.988266778220432));
#94439=DIRECTION('',(-0.190809912898503,0.,0.981627005099017));
#94440=DIRECTION('center_axis',(0.,-1.,0.));
#94441=DIRECTION('ref_axis',(0.144410991615934,0.,0.989517794433482));
#94442=DIRECTION('center_axis',(0.981627005099017,0.,0.190809912898503));
#94443=DIRECTION('ref_axis',(0.,-1.,0.));
#94444=DIRECTION('',(-0.190809912898503,0.,0.981627005099017));
#94445=DIRECTION('center_axis',(0.981627005099017,-1.31015175507947E-16,
0.190809912898504));
#94446=DIRECTION('ref_axis',(-0.172473747912141,-0.427736442803512,0.887296084618284));
#94447=DIRECTION('center_axis',(0.981627005099017,-2.82583468587877E-16,
0.190809912898504));
#94448=DIRECTION('ref_axis',(-0.173271151848023,-0.418791220542401,0.891398351767528));
#94449=DIRECTION('center_axis',(0.,1.,0.));
#94450=DIRECTION('ref_axis',(1.,0.,0.));
#94451=DIRECTION('',(-0.190809912898503,0.,0.981627005099017));
#94452=DIRECTION('center_axis',(0.,1.,0.));
#94453=DIRECTION('ref_axis',(0.10984303932686,0.,0.99394894572681));
#94454=DIRECTION('center_axis',(0.,1.,0.));
#94455=DIRECTION('ref_axis',(0.102818743046302,0.,0.994700108614842));
#94456=DIRECTION('center_axis',(-0.981627005099017,0.,-0.190809912898503));
#94457=DIRECTION('ref_axis',(-0.190809912898503,0.,0.981627005099017));
#94458=DIRECTION('center_axis',(-0.981627005099017,1.28381668760922E-16,
-0.190809912898504));
#94459=DIRECTION('ref_axis',(-0.169717089537917,-0.457020123580983,0.873114377479149));
#94460=DIRECTION('center_axis',(-0.981627005099017,3.38719187348766E-16,
-0.190809912898504));
#94461=DIRECTION('ref_axis',(-0.17062403409845,-0.447648741208883,0.877780179476658));
#94462=DIRECTION('center_axis',(0.,-1.,0.));
#94463=DIRECTION('ref_axis',(0.,0.,-1.));
#94464=DIRECTION('',(-0.190809912898503,0.,0.981627005099017));
#94465=DIRECTION('center_axis',(0.,-1.,0.));
#94466=DIRECTION('ref_axis',(0.0776743290905875,0.,0.996978785431429));
#94467=DIRECTION('',(-0.190809912898503,0.,0.981627005099017));
#94468=DIRECTION('center_axis',(0.,-1.,0.));
#94469=DIRECTION('ref_axis',(0.0712170703537014,0.,0.997460840780347));
#94470=DIRECTION('center_axis',(0.981627005099017,0.,0.190809912898503));
#94471=DIRECTION('ref_axis',(0.,-1.,0.));
#94472=DIRECTION('',(-0.190809912898503,0.,0.981627005099017));
#94473=DIRECTION('center_axis',(0.981627005099017,-2.8379520623381E-16,
0.190809912898504));
#94474=DIRECTION('ref_axis',(-0.173192120088612,-0.419688163031609,0.890991770641214));
#94475=DIRECTION('center_axis',(0.981627005099017,1.81646488737385E-16,
0.190809912898503));
#94476=DIRECTION('ref_axis',(-0.173929387576568,-0.411228614003993,0.894784664129641));
#94477=DIRECTION('center_axis',(0.,1.,0.));
#94478=DIRECTION('ref_axis',(1.,0.,0.));
#94479=DIRECTION('',(-0.190809912898503,0.,0.981627005099017));
#94480=DIRECTION('center_axis',(0.,1.,0.));
#94481=DIRECTION('ref_axis',(0.0366430595622812,0.,0.999328417581485));
#94482=DIRECTION('center_axis',(0.,1.,0.));
#94483=DIRECTION('ref_axis',(0.0313675707532251,0.,0.999507916679524));
#94484=DIRECTION('center_axis',(-0.981627005099017,0.,-0.190809912898503));
#94485=DIRECTION('ref_axis',(-0.190809912898503,0.,0.981627005099017));
#94486=DIRECTION('center_axis',(-0.981627005099017,2.3292971780749E-16,
-0.190809912898504));
#94487=DIRECTION('ref_axis',(-0.170440188767048,-0.449568246953191,0.876834381958468));
#94488=DIRECTION('center_axis',(-0.981627005099017,2.53604646310564E-16,
-0.190809912898504));
#94489=DIRECTION('ref_axis',(-0.171287079367587,-0.440639018251895,0.88119123465666));
#94490=DIRECTION('center_axis',(0.,-1.,0.));
#94491=DIRECTION('ref_axis',(0.,0.,-1.));
#94492=DIRECTION('',(-0.190809912898503,0.,0.981627005099017));
#94493=DIRECTION('center_axis',(0.,-1.,0.));
#94494=DIRECTION('ref_axis',(0.00371858367446118,0.,0.999993086043827));
#94495=DIRECTION('',(-0.190809912898503,0.,0.981627005099017));
#94496=DIRECTION('center_axis',(0.,-1.,0.));
#94497=DIRECTION('ref_axis',(-0.000926353014041966,0.,0.999999570934955));
#94498=DIRECTION('center_axis',(0.981627005099017,0.,0.190809912898503));
#94499=DIRECTION('ref_axis',(0.,-1.,0.));
#94500=DIRECTION('',(-0.190809912898503,0.,0.981627005099017));
#94501=DIRECTION('center_axis',(0.981627005099017,-3.2195030332024E-16,
0.190809912898504));
#94502=DIRECTION('ref_axis',(-0.17370268013601,-0.413852151503288,0.893618361276035));
#94503=DIRECTION('center_axis',(0.981627005099017,-1.03147739908772E-16,
0.190809912898504));
#94504=DIRECTION('ref_axis',(-0.174398591463139,-0.405733888890709,0.897198496822913));
#94505=DIRECTION('center_axis',(0.,1.,0.));
#94506=DIRECTION('ref_axis',(1.,0.,0.));
#94507=DIRECTION('',(-0.190809912898503,0.,0.981627005099017));
#94508=DIRECTION('center_axis',(0.,1.,0.));
#94509=DIRECTION('ref_axis',(-0.0355191393229559,0.,0.999368996288036));
#94510=DIRECTION('center_axis',(0.,1.,0.));
#94511=DIRECTION('ref_axis',(-0.0390960923094082,0.,0.999235455518935));
#94512=DIRECTION('center_axis',(-0.981627005099017,0.,-0.190809912898503));
#94513=DIRECTION('ref_axis',(-0.190809912898503,0.,0.981627005099017));
#94514=DIRECTION('center_axis',(-0.981627005099017,-2.27558651128372E-16,
-0.190809912898503));
#94515=DIRECTION('ref_axis',(-0.170937231783471,-0.444354778157526,0.879391433844326));
#94516=DIRECTION('center_axis',(-0.981627005099017,-1.02110124627879E-16,
-0.190809912898503));
#94517=DIRECTION('ref_axis',(-0.171743997738244,-0.435726718837086,0.883541864165107));
#94518=DIRECTION('center_axis',(0.,-1.,0.));
#94519=DIRECTION('ref_axis',(0.,0.,-1.));
#94520=DIRECTION('',(-0.190809912898503,0.,0.981627005099017));
#94521=DIRECTION('center_axis',(0.,-1.,0.));
#94522=DIRECTION('ref_axis',(-0.0691867906738412,0.,0.99760372292622));
#94523=DIRECTION('',(-0.190809912898503,0.,0.981627005099017));
#94524=DIRECTION('center_axis',(0.,-1.,0.));
#94525=DIRECTION('ref_axis',(-0.0720708919844832,0.,0.997399511995349));
#94526=DIRECTION('center_axis',(0.981627005099017,0.,0.190809912898503));
#94527=DIRECTION('ref_axis',(0.,-1.,0.));
#94528=DIRECTION('',(-0.190809912898503,0.,0.981627005099017));
#94529=DIRECTION('center_axis',(0.981627005099017,-1.50452980269455E-17,
0.190809912898503));
#94530=DIRECTION('ref_axis',(-0.174036822496206,-0.409978274115724,0.895337366118781));
#94531=DIRECTION('center_axis',(0.981627005099017,-2.02598138069568E-16,
0.190809912898504));
#94532=DIRECTION('ref_axis',(-0.174706292097902,-0.402081556480905,0.898781471459718));
#94533=DIRECTION('center_axis',(0.,1.,0.));
#94534=DIRECTION('ref_axis',(1.,0.,0.));
#94535=DIRECTION('',(-0.190809912898503,0.,0.981627005099017));
#94536=DIRECTION('center_axis',(0.,1.,0.));
#94537=DIRECTION('ref_axis',(-0.106686710809781,0.,0.994292686152619));
#94538=DIRECTION('center_axis',(0.,1.,0.));
#94539=DIRECTION('ref_axis',(-0.108611424892643,0.,0.99408428132769));
#94540=DIRECTION('center_axis',(-0.981627005099017,0.,-0.190809912898503));
#94541=DIRECTION('ref_axis',(-0.190809912898503,0.,0.981627005099017));
#94542=DIRECTION('center_axis',(-0.981627005099017,2.09348652609932E-16,
-0.190809912898504));
#94543=DIRECTION('ref_axis',(-0.171237890630439,-0.441163807051188,0.880938181804228));
#94544=DIRECTION('center_axis',(-0.981627005099017,-1.58249582464702E-16,
-0.190809912898503));
#94545=DIRECTION('ref_axis',(-0.172020843188232,-0.432716795710511,0.884966103429299));
#94546=DIRECTION('center_axis',(0.,-1.,0.));
#94547=DIRECTION('ref_axis',(0.,0.,-1.));
#94548=DIRECTION('',(-0.190809912898503,0.,0.981627005099017));
#94549=DIRECTION('center_axis',(0.,-1.,0.));
#94550=DIRECTION('ref_axis',(-0.141078288382398,0.,0.989998442699327));
#94551=DIRECTION('',(-0.190809912898503,0.,0.981627005099017));
#94552=DIRECTION('center_axis',(0.,-1.,0.));
#94553=DIRECTION('ref_axis',(-0.142249621027872,0.,0.98983081651231));
#94554=DIRECTION('center_axis',(0.981627005099017,0.,0.190809912898503));
#94555=DIRECTION('ref_axis',(0.,-1.,0.));
#94556=DIRECTION('',(-0.190809912898503,-1.082199615072E-14,0.981627005099017));
#94557=DIRECTION('center_axis',(0.981627005099017,-2.23408810325902E-16,
0.190809912898504));
#94558=DIRECTION('ref_axis',(-0.174213626435771,-0.407910574394006,0.896246938997088));
#94559=DIRECTION('center_axis',(0.981627005099017,2.43630309943914E-16,
0.190809912898503));
#94560=DIRECTION('ref_axis',(-0.174869305192863,-0.400130487804013,0.899620096947088));
#94561=DIRECTION('center_axis',(0.,1.,0.));
#94562=DIRECTION('ref_axis',(1.,0.,0.));
#94563=DIRECTION('',(-0.190809912898503,0.,0.981627005099017));
#94564=DIRECTION('center_axis',(0.,1.,0.));
#94565=DIRECTION('ref_axis',(-0.176885309946529,0.,0.98423147029808));
#94566=DIRECTION('center_axis',(0.,1.,0.));
#94567=DIRECTION('ref_axis',(-0.177201781451223,0.,0.98417454176102));
#94568=DIRECTION('center_axis',(-0.981627005099017,0.,-0.190809912898503));
#94569=DIRECTION('ref_axis',(-0.190809912898503,0.,0.981627005099017));
#94570=DIRECTION('center_axis',(-0.981627005099017,1.33792883286904E-16,
-0.190809912898504));
#94571=DIRECTION('ref_axis',(-0.171359055428295,-0.439869713566988,0.881561517541016));
#94572=DIRECTION('center_axis',(-0.981627005099017,1.85967954159957E-16,
-0.190809912898504));
#94573=DIRECTION('ref_axis',(-0.172132508930255,-0.431495418834412,0.885540571004113));
#94574=DIRECTION('center_axis',(0.,-1.,0.));
#94575=DIRECTION('ref_axis',(0.,0.,-1.));
#94576=DIRECTION('',(-0.190809912898503,0.,0.981627005099017));
#94577=DIRECTION('center_axis',(0.,-1.,0.));
#94578=DIRECTION('ref_axis',(-0.211974931298844,0.,0.9772751037967));
#94579=DIRECTION('',(-0.190809912898503,0.,0.981627005099017));
#94580=DIRECTION('center_axis',(0.,-1.,0.));
#94581=DIRECTION('ref_axis',(-0.211479816819108,0.,0.977382364828707));
#94582=DIRECTION('center_axis',(0.981627005099017,0.,0.190809912898503));
#94583=DIRECTION('ref_axis',(0.,-1.,0.));
#94584=DIRECTION('',(-0.190809912898503,0.,0.981627005099017));
#94585=DIRECTION('center_axis',(0.981627005099017,2.97379735788161E-17,
0.190809912898503));
#94586=DIRECTION('ref_axis',(-0.174242731231815,-0.407568990013114,0.896396669445267));
#94587=DIRECTION('center_axis',(0.981627005099017,0.,0.190809912898503));
#94588=DIRECTION('ref_axis',(-0.174896153086883,-0.399808062848099,0.899758216698831));
#94589=DIRECTION('center_axis',(0.,1.,0.));
#94590=DIRECTION('ref_axis',(1.,0.,0.));
#94591=DIRECTION('',(-0.190809912898503,0.,0.981627005099017));
#94592=DIRECTION('center_axis',(0.,1.,0.));
#94593=DIRECTION('ref_axis',(-0.24612518066157,0.,0.969238048904556));
#94594=DIRECTION('center_axis',(0.,1.,0.));
#94595=DIRECTION('ref_axis',(-0.244876500445944,0.,0.969554278794822));
#94596=DIRECTION('center_axis',(-0.981627005099017,0.,-0.190809912898503));
#94597=DIRECTION('ref_axis',(-0.190809912898503,0.,0.981627005099017));
#94598=DIRECTION('center_axis',(-0.981627005099017,1.04323047313055E-16,
-0.190809912898503));
#94599=DIRECTION('ref_axis',(-0.171307312408284,-0.440422929036202,0.881295324107999));
#94600=DIRECTION('center_axis',(-0.981627005099017,3.87176530094412E-16,
-0.190809912898504));
#94601=DIRECTION('ref_axis',(-0.172084815581002,-0.4320175983019,0.885295211217089));
#94602=DIRECTION('center_axis',(0.,-1.,0.));
#94603=DIRECTION('ref_axis',(0.,0.,-1.));
#94604=DIRECTION('',(-0.190809912898503,0.,0.981627005099017));
#94605=DIRECTION('center_axis',(0.,-1.,0.));
#94606=DIRECTION('ref_axis',(-0.28187983172236,0.,0.959449717529884));
#94607=DIRECTION('',(-0.190809912898503,0.,0.981627005099017));
#94608=DIRECTION('center_axis',(0.,-1.,0.));
#94609=DIRECTION('ref_axis',(-0.279764308576818,0.,0.960068711940211));
#94610=DIRECTION('center_axis',(0.981627005099017,0.,0.190809912898503));
#94611=DIRECTION('ref_axis',(0.,-1.,0.));
#94612=DIRECTION('',(-0.190809912898503,0.,0.981627005099017));
#94613=DIRECTION('center_axis',(0.981627005099017,-1.64661493304004E-16,
0.190809912898504));
#94614=DIRECTION('ref_axis',(-0.174125693879922,-0.408940503765383,0.89579456747122));
#94615=DIRECTION('center_axis',(0.981627005099017,-4.32027132019077E-17,
0.190809912898503));
#94616=DIRECTION('ref_axis',(-0.17478821411242,-0.401102463243196,0.899202921585352));
#94617=DIRECTION('center_axis',(0.,1.,0.));
#94618=DIRECTION('ref_axis',(1.,0.,0.));
#94619=DIRECTION('',(-0.190809912898503,0.,0.981627005099017));
#94620=DIRECTION('center_axis',(0.,1.,0.));
#94621=DIRECTION('ref_axis',(-0.314401954981219,0.,0.949289950807438));
#94622=DIRECTION('center_axis',(0.,1.,0.));
#94623=DIRECTION('ref_axis',(-0.311631599069456,0.,0.950203002763838));
#94624=DIRECTION('center_axis',(-0.981627005099017,0.,-0.190809912898503));
#94625=DIRECTION('ref_axis',(-0.190809912898503,0.,0.981627005099017));
#94626=DIRECTION('center_axis',(-0.981627005099017,2.86284995913372E-16,
-0.190809912898504));
#94627=DIRECTION('ref_axis',(-0.171079864292319,-0.442844547552897,0.880125210828773));
#94628=DIRECTION('center_axis',(-0.981627005099017,2.17379342169057E-16,
-0.190809912898504));
#94629=DIRECTION('ref_axis',(-0.171875290112581,-0.434302484871899,0.884217301506146));
#94630=DIRECTION('center_axis',(0.,-1.,0.));
#94631=DIRECTION('ref_axis',(0.,0.,-1.));
#94632=DIRECTION('',(-0.190809912898503,0.,0.981627005099017));
#94633=DIRECTION('center_axis',(0.,-1.,0.));
#94634=DIRECTION('ref_axis',(-0.350780441750461,0.,0.936457730858874));
#94635=DIRECTION('',(-0.190809912898503,0.,0.981627005099017));
#94636=DIRECTION('center_axis',(0.,-1.,0.));
#94637=DIRECTION('ref_axis',(-0.347091693931338,0.,0.937831198032926));
#94638=DIRECTION('center_axis',(0.981627005099017,0.,0.190809912898503));
#94639=DIRECTION('ref_axis',(0.,-1.,0.));
#94640=DIRECTION('',(-0.190809912898503,0.,0.981627005099017));
#94641=DIRECTION('center_axis',(0.981627005099017,-7.5998920345386E-17,
0.190809912898503));
#94642=DIRECTION('ref_axis',(-0.173856202311149,-0.412077739540977,0.894408160457374));
#94643=DIRECTION('center_axis',(0.981627005099017,-2.338266036503E-16,0.190809912898504));
#94644=DIRECTION('ref_axis',(-0.174539903539162,-0.404061447055713,0.89792548080327));
#94645=DIRECTION('center_axis',(0.,1.,0.));
#94646=DIRECTION('ref_axis',(1.,0.,0.));
#94647=DIRECTION('',(-0.190809912898503,0.,0.981627005099017));
#94648=DIRECTION('center_axis',(0.,1.,0.));
#94649=DIRECTION('ref_axis',(-0.381696314616838,0.,0.924287792523478));
#94650=DIRECTION('center_axis',(0.,1.,0.));
#94651=DIRECTION('ref_axis',(-0.377449478914398,0.,0.926030178162272));
#94652=DIRECTION('center_axis',(-0.981627005099017,0.,-0.190809912898503));
#94653=DIRECTION('ref_axis',(-0.190809912898503,0.,0.981627005099017));
#94654=DIRECTION('center_axis',(-0.981627005099017,1.38306959983606E-16,
-0.190809912898504));
#94655=DIRECTION('ref_axis',(-0.170664142574815,-0.447228603146884,0.877986518670128));
#94656=DIRECTION('center_axis',(-0.981627005099017,1.47690827086916E-16,
-0.190809912898504));
#94657=DIRECTION('ref_axis',(-0.171492837474547,-0.438435356989177,0.882249763069791));
#94658=DIRECTION('center_axis',(0.,-1.,0.));
#94659=DIRECTION('ref_axis',(0.,0.,-1.));
#94660=DIRECTION('',(-0.190809912898503,0.,0.981627005099017));
#94661=DIRECTION('center_axis',(0.,-1.,0.));
#94662=DIRECTION('ref_axis',(-0.418647537023905,0.,0.908148798239483));
#94663=DIRECTION('',(-0.190809912898503,0.,0.981627005099017));
#94664=DIRECTION('center_axis',(0.,-1.,0.));
#94665=DIRECTION('ref_axis',(-0.413435459905699,0.,0.910533426345548));
#94666=DIRECTION('center_axis',(0.981627005099017,0.,0.190809912898503));
#94667=DIRECTION('ref_axis',(0.,-1.,0.));
#94668=DIRECTION('',(-0.190809912898503,0.,0.981627005099017));
#94669=DIRECTION('center_axis',(0.981627005099017,-1.24583136198838E-16,
0.190809912898504));
#94670=DIRECTION('ref_axis',(-0.173419200493624,-0.417104698103898,0.892159992221019));
#94671=DIRECTION('center_axis',(0.981627005099017,-4.03886202418115E-16,
0.190809912898504));
#94672=DIRECTION('ref_axis',(-0.174137931887097,-0.408797349974888,0.895857526245995));
#94673=DIRECTION('center_axis',(0.,1.,0.));
#94674=DIRECTION('ref_axis',(1.,0.,0.));
#94675=DIRECTION('',(-0.190809912898503,1.305554049207E-14,0.981627005099017));
#94676=DIRECTION('center_axis',(0.,1.,0.));
#94677=DIRECTION('ref_axis',(-0.447972451854823,0.,0.894047360255136));
#94678=DIRECTION('center_axis',(0.,1.,0.));
#94679=DIRECTION('ref_axis',(-0.442297590336883,0.,0.896868352425364));
#94680=DIRECTION('center_axis',(-0.981627005099017,0.,-0.190809912898503));
#94681=DIRECTION('ref_axis',(-0.190809912898503,0.,0.981627005099017));
#94682=DIRECTION('center_axis',(-0.981627005099017,-9.49143134910359E-17,
-0.190809912898503));
#94683=DIRECTION('ref_axis',(-0.170036007749122,-0.45375250839628,0.874755061255906));
#94684=DIRECTION('center_axis',(-0.981627005099017,-1.67043077322242E-16,
-0.190809912898503));
#94685=DIRECTION('ref_axis',(-0.170916220682317,-0.444576709493399,0.879283341638914));
#94686=DIRECTION('center_axis',(0.,-1.,0.));
#94687=DIRECTION('ref_axis',(0.,0.,-1.));
#94688=DIRECTION('',(-0.190809912898503,0.,0.981627005099017));
#94689=DIRECTION('center_axis',(0.,-1.,0.));
#94690=DIRECTION('ref_axis',(-0.485432735772008,0.,0.874274018280827));
#94691=DIRECTION('',(-0.190809912898503,0.,0.981627005099017));
#94692=DIRECTION('center_axis',(0.,-1.,0.));
#94693=DIRECTION('ref_axis',(-0.47875184538002,0.,0.877950266555701));
#94694=DIRECTION('center_axis',(0.981627005099017,0.,0.190809912898503));
#94695=DIRECTION('ref_axis',(0.,-1.,0.));
#94696=DIRECTION('',(-0.190809912898503,0.,0.981627005099017));
#94697=DIRECTION('center_axis',(0.981627005099017,0.,0.190809912898503));
#94698=DIRECTION('ref_axis',(-0.172788690240708,-0.424230897743185,0.88891631435412));
#94699=DIRECTION('center_axis',(0.981627005099017,-2.47252011742998E-16,
0.190809912898504));
#94700=DIRECTION('ref_axis',(-0.173559449920186,-0.415499371319114,0.892881509371105));
#94701=DIRECTION('center_axis',(0.,1.,0.));
#94702=DIRECTION('ref_axis',(1.,0.,0.));
#94703=DIRECTION('',(-0.190809912898503,0.,0.981627005099017));
#94704=DIRECTION('center_axis',(0.,1.,0.));
#94705=DIRECTION('ref_axis',(-0.513175031076331,0.,0.85828397834272));
#94706=DIRECTION('center_axis',(0.,1.,0.));
#94707=DIRECTION('ref_axis',(-0.506125809124676,0.,0.862459660122079));
#94708=DIRECTION('center_axis',(-0.981627005099017,0.,-0.190809912898503));
#94709=DIRECTION('ref_axis',(-0.190809912898503,0.,0.981627005099017));
#94710=DIRECTION('center_axis',(-0.981627005099017,0.,-0.190809912898503));
#94711=DIRECTION('ref_axis',(-0.169156033040075,-0.462698015255998,0.870228006423779));
#94712=DIRECTION('center_axis',(-0.981627005099017,1.73417897774942E-16,
-0.190809912898504));
#94713=DIRECTION('ref_axis',(-0.170110942777143,-0.452980414348596,0.875140566631467));
#94714=DIRECTION('center_axis',(0.981627005099017,0.,0.190809912898503));
#94715=DIRECTION('ref_axis',(0.,-1.,0.));
#94716=DIRECTION('',(-0.190809912898503,0.,0.981627005099017));
#94717=DIRECTION('center_axis',(0.981627005099017,-2.69483765365246E-16,
0.190809912898504));
#94718=DIRECTION('ref_axis',(-0.171923576181418,-0.433777236382802,0.884465710555865));
#94719=DIRECTION('',(-0.190809912898503,0.,0.981627005099017));
#94720=DIRECTION('center_axis',(0.981627005099017,-7.2569942460446E-17,
0.190809912898503));
#94721=DIRECTION('ref_axis',(-0.172768570512372,-0.4244559030808,0.888812807841434));
#94722=DIRECTION('center_axis',(0.,1.,0.));
#94723=DIRECTION('ref_axis',(1.,0.,0.));
#94724=DIRECTION('',(-0.190809912898503,0.,0.981627005099017));
#94725=DIRECTION('center_axis',(0.,1.,0.));
#94726=DIRECTION('ref_axis',(-0.577224006242642,0.,0.816585847671385));
#94727=DIRECTION('center_axis',(0.,1.,0.));
#94728=DIRECTION('ref_axis',(-0.568861998611027,0.,0.822432992125357));
#94729=DIRECTION('center_axis',(-0.981627005099017,0.,-0.190809912898503));
#94730=DIRECTION('ref_axis',(-0.190809912898503,0.,0.981627005099017));
#94731=DIRECTION('',(-0.190809912898503,0.,0.981627005099017));
#94732=DIRECTION('',(0.,-1.,0.));
#94733=DIRECTION('center_axis',(-0.981627005099017,6.91914718802358E-17,
-0.190809912898503));
#94734=DIRECTION('ref_axis',(-0.169895538310713,-0.455195395847704,0.874032412248634));
#94735=DIRECTION('center_axis',(-0.981627005099017,1.65434297745177E-17,
-0.190809912898503));
#94736=DIRECTION('ref_axis',(-0.169023616517123,-0.464025219406811,0.869546785868324));
#94737=DIRECTION('center_axis',(0.,-1.,0.));
#94738=DIRECTION('ref_axis',(0.,0.,-1.));
#94739=DIRECTION('center_axis',(0.,-1.,0.));
#94740=DIRECTION('ref_axis',(-0.551064033121797,0.,0.834462959872719));
#94741=DIRECTION('',(0.981627005099017,0.,0.190809912898503));
#94742=DIRECTION('center_axis',(0.,-1.,0.));
#94743=DIRECTION('ref_axis',(-0.542976020742699,0.,0.839748200890257));
#94744=DIRECTION('center_axis',(-0.190809912898503,0.,0.981627005099017));
#94745=DIRECTION('ref_axis',(0.,1.,0.));
#94746=DIRECTION('center_axis',(0.190809912898503,1.16564584175745E-16,
-0.981627005099017));
#94747=DIRECTION('ref_axis',(-0.615493430324788,-0.779008351588359,-0.119640400294435));
#94748=DIRECTION('center_axis',(0.981627005099017,0.,0.190809912898503));
#94749=DIRECTION('ref_axis',(0.,-1.,0.));
#94750=DIRECTION('',(-0.190809912898503,0.,0.981627005099017));
#94751=DIRECTION('center_axis',(0.981627005099017,-1.78228754819253E-17,
0.190809912898503));
#94752=DIRECTION('ref_axis',(-0.176855272063147,-0.375391687874098,0.90983695980022));
#94753=DIRECTION('',(-0.190809912898503,0.,0.981627005099017));
#94754=DIRECTION('center_axis',(0.981627005099017,-3.064140942095E-16,0.190809912898504));
#94755=DIRECTION('ref_axis',(-0.177505054319294,-0.366871421003507,0.913179783033972));
#94756=DIRECTION('center_axis',(0.,1.,0.));
#94757=DIRECTION('ref_axis',(1.,0.,0.));
#94758=DIRECTION('',(-0.190809912898503,0.,0.981627005099017));
#94759=DIRECTION('center_axis',(0.,1.,0.));
#94760=DIRECTION('ref_axis',(-0.628205223222824,0.,0.778047683317393));
#94761=DIRECTION('center_axis',(0.,1.,0.));
#94762=DIRECTION('ref_axis',(-0.619332264144748,0.,0.785128999967101));
#94763=DIRECTION('center_axis',(-0.981627005099017,0.,-0.190809912898503));
#94764=DIRECTION('ref_axis',(-0.190809912898503,0.,0.981627005099017));
#94765=DIRECTION('',(-0.190809912898503,0.,0.981627005099017));
#94766=DIRECTION('',(0.,-1.,0.));
#94767=DIRECTION('center_axis',(-0.981627005099017,1.65855791542818E-16,
-0.190809912898504));
#94768=DIRECTION('ref_axis',(-0.175359682635441,-0.394191890059205,0.902142857599366));
#94769=DIRECTION('center_axis',(-0.981627005099017,2.10894926800414E-16,
-0.190809912898504));
#94770=DIRECTION('ref_axis',(-0.174211595031188,-0.407934402882895,0.896236488378634));
#94771=DIRECTION('center_axis',(0.,-1.,0.));
#94772=DIRECTION('ref_axis',(0.,0.,-1.));
#94773=DIRECTION('center_axis',(0.,-1.,0.));
#94774=DIRECTION('ref_axis',(-0.6029066307257,0.,0.797811753878685));
#94775=DIRECTION('',(0.981627005099017,0.,0.190809912898503));
#94776=DIRECTION('center_axis',(0.,-1.,0.));
#94777=DIRECTION('ref_axis',(-0.594284330901843,0.,0.804255018041261));
#94778=DIRECTION('center_axis',(-0.190809912898503,0.,0.981627005099017));
#94779=DIRECTION('ref_axis',(0.,1.,0.));
#94780=DIRECTION('center_axis',(0.190809912898503,-3.49693752527234E-17,
-0.981627005099017));
#94781=DIRECTION('ref_axis',(-0.733603465583051,-0.664448299884183,-0.142598780028288));
#94782=DIRECTION('center_axis',(0.,-1.,0.));
#94783=DIRECTION('ref_axis',(0.,0.,-1.));
#94784=DIRECTION('',(-0.190809912898503,0.,0.981627005099017));
#94785=DIRECTION('center_axis',(0.,-1.,0.));
#94786=DIRECTION('ref_axis',(-0.593188827435541,0.,0.805063360864005));
#94787=DIRECTION('',(-0.190809912898503,0.,0.981627005099017));
#94788=DIRECTION('center_axis',(0.,-1.,0.));
#94789=DIRECTION('ref_axis',(-0.585155835598189,0.,0.810920864243476));
#94790=DIRECTION('center_axis',(0.981627005099017,0.,0.190809912898503));
#94791=DIRECTION('ref_axis',(0.,-1.,0.));
#94792=DIRECTION('',(-0.190809912898503,0.,0.981627005099017));
#94793=DIRECTION('center_axis',(0.981627005099017,-9.80258151505892E-17,
0.190809912898504));
#94794=DIRECTION('ref_axis',(-0.181744948393978,-0.304563067520509,0.934992038274));
#94795=DIRECTION('center_axis',(0.981627005099017,-7.66035235523749E-17,
0.190809912898504));
#94796=DIRECTION('ref_axis',(-0.182161442088192,-0.297650398172597,0.937134701888712));
#94797=DIRECTION('center_axis',(0.,1.,0.));
#94798=DIRECTION('ref_axis',(1.,0.,0.));
#94799=DIRECTION('',(-0.190809912898503,0.,0.981627005099017));
#94800=DIRECTION('center_axis',(0.,1.,0.));
#94801=DIRECTION('ref_axis',(-0.619117740094101,0.,0.785298175154363));
#94802=DIRECTION('center_axis',(0.,1.,0.));
#94803=DIRECTION('ref_axis',(-0.610780642463143,0.,0.791799852735722));
#94804=DIRECTION('center_axis',(-0.981627005099017,0.,-0.190809912898503));
#94805=DIRECTION('ref_axis',(-0.190809912898503,0.,0.981627005099017));
#94806=DIRECTION('center_axis',(-0.981627005099017,1.28998948977747E-16,
-0.190809912898504));
#94807=DIRECTION('ref_axis',(-0.179045219445688,-0.345704632538082,0.921103206180152));
#94808=DIRECTION('center_axis',(-0.981627005099017,4.48151719450879E-16,
-0.190809912898504));
#94809=DIRECTION('ref_axis',(-0.179607339081024,-0.337600885144495,0.923995046576489));
#94810=DIRECTION('center_axis',(0.,-1.,0.));
#94811=DIRECTION('ref_axis',(0.,0.,-1.));
#94812=DIRECTION('',(-0.190809912898503,0.,0.981627005099017));
#94813=DIRECTION('center_axis',(0.,-1.,0.));
#94814=DIRECTION('ref_axis',(-0.585794842268511,0.,0.810459377619638));
#94815=DIRECTION('',(-0.190809912898503,0.,0.981627005099017));
#94816=DIRECTION('center_axis',(0.,-1.,0.));
#94817=DIRECTION('ref_axis',(-0.578192279907259,0.,0.815900537722366));
#94818=DIRECTION('center_axis',(0.981627005099017,0.,0.190809912898503));
#94819=DIRECTION('ref_axis',(0.,-1.,0.));
#94820=DIRECTION('',(-0.190809912898503,0.,0.981627005099017));
#94821=DIRECTION('center_axis',(0.981627005099017,9.80258151505892E-17,
0.190809912898503));
#94822=DIRECTION('ref_axis',(-0.185524568408441,-0.23373444716689,0.954436400565512));
#94823=DIRECTION('center_axis',(0.981627005099017,6.80920209354444E-17,
0.190809912898503));
#94824=DIRECTION('ref_axis',(-0.185764991591961,-0.228429375341796,0.955673264447528));
#94825=DIRECTION('center_axis',(0.,1.,0.));
#94826=DIRECTION('ref_axis',(1.,0.,0.));
#94827=DIRECTION('',(-0.190809912898493,0.,0.981627005099019));
#94828=DIRECTION('center_axis',(0.,1.,0.));
#94829=DIRECTION('ref_axis',(-0.612315243995724,0.,0.790613712232755));
#94830=DIRECTION('center_axis',(0.,1.,0.));
#94831=DIRECTION('ref_axis',(-0.604365249086077,0.,0.796707377709736));
#94832=DIRECTION('center_axis',(-0.981627005099017,0.,-0.190809912898503));
#94833=DIRECTION('ref_axis',(-0.190809912898503,0.,0.981627005099017));
#94834=DIRECTION('center_axis',(-0.981627005099017,6.44994744888736E-17,
-0.190809912898503));
#94835=DIRECTION('ref_axis',(-0.183524789821252,-0.273682834092602,0.944148482943285));
#94836=DIRECTION('center_axis',(-0.981627005099017,-5.27237317001035E-17,
-0.190809912898503));
#94837=DIRECTION('ref_axis',(-0.183868708640475,-0.267267367406098,0.945917783056592));
#94838=DIRECTION('center_axis',(0.,-1.,0.));
#94839=DIRECTION('ref_axis',(0.,0.,-1.));
#94840=DIRECTION('',(-0.190809912898503,0.,0.981627005099017));
#94841=DIRECTION('center_axis',(0.,-1.,0.));
#94842=DIRECTION('ref_axis',(-0.580391375879782,0.,0.814337676154293));
#94843=DIRECTION('',(-0.190809912898503,0.,0.981627005099017));
#94844=DIRECTION('center_axis',(0.,-1.,0.));
#94845=DIRECTION('ref_axis',(-0.573093697528526,0.,0.819489849755982));
#94846=DIRECTION('center_axis',(0.981627005099017,0.,0.190809912898503));
#94847=DIRECTION('ref_axis',(0.,-1.,0.));
#94848=DIRECTION('',(-0.190809912898503,0.,0.981627005099017));
#94849=DIRECTION('center_axis',(0.981627005099017,-3.56457509638507E-17,
0.190809912898503));
#94850=DIRECTION('ref_axis',(-0.188261002084221,-0.162905826813305,0.968514061170264));
#94851=DIRECTION('center_axis',(0.981627005099017,-6.38362696269791E-17,
0.190809912898504));
#94852=DIRECTION('ref_axis',(-0.188376133470869,-0.159208352510898,0.969106357852084));
#94853=DIRECTION('center_axis',(0.,1.,0.));
#94854=DIRECTION('ref_axis',(1.,0.,0.));
#94855=DIRECTION('',(-0.190809912898503,0.,0.981627005099017));
#94856=DIRECTION('center_axis',(0.,1.,0.));
#94857=DIRECTION('ref_axis',(-0.607507081583685,0.,0.794314261376235));
#94858=DIRECTION('center_axis',(0.,1.,0.));
#94859=DIRECTION('ref_axis',(-0.599823547083943,0.,0.800132309286181));
#94860=DIRECTION('center_axis',(-0.981627005099017,0.,-0.190809912898503));
#94861=DIRECTION('ref_axis',(-0.190809912898503,0.,0.981627005099017));
#94862=DIRECTION('center_axis',(-0.981627005099017,-4.14639478857045E-17,
-0.190809912898503));
#94863=DIRECTION('ref_axis',(-0.186889794312999,-0.201661035647202,0.96145984392659));
#94864=DIRECTION('center_axis',(-0.981627005099017,1.66958483716994E-16,
-0.190809912898504));
#94865=DIRECTION('ref_axis',(-0.187073240040802,-0.196933849667601,0.962403585672734));
#94866=DIRECTION('center_axis',(0.,-1.,0.));
#94867=DIRECTION('ref_axis',(0.,0.,-1.));
#94868=DIRECTION('',(-0.190809912898503,0.,0.981627005099017));
#94869=DIRECTION('center_axis',(0.,-1.,0.));
#94870=DIRECTION('ref_axis',(-0.576755053793433,0.,0.816917136510022));
#94871=DIRECTION('',(-0.190809912898503,0.,0.981627005099017));
#94872=DIRECTION('center_axis',(0.,-1.,0.));
#94873=DIRECTION('ref_axis',(-0.56965800443632,0.,0.821881839428047));
#94874=DIRECTION('center_axis',(0.981627005099017,0.,0.190809912898503));
#94875=DIRECTION('ref_axis',(0.,-1.,0.));
#94876=DIRECTION('',(-0.190809912898503,0.,0.981627005099017));
#94877=DIRECTION('center_axis',(0.981627005099017,2.45064537876473E-17,
0.190809912898503));
#94878=DIRECTION('ref_axis',(-0.18999932772139,-0.0920772064596915,0.977456926680659));
#94879=DIRECTION('center_axis',(0.981627005099017,-7.66035235523749E-17,
0.190809912898504));
#94880=DIRECTION('ref_axis',(-0.190035779958582,-0.0899873296801039,0.977644456248067));
#94881=DIRECTION('center_axis',(0.,1.,0.));
#94882=DIRECTION('ref_axis',(1.,0.,0.));
#94883=DIRECTION('',(-0.190809912898503,0.,0.981627005099017));
#94884=DIRECTION('center_axis',(0.,1.,0.));
#94885=DIRECTION('ref_axis',(-0.604502425562639,0.,0.796603299948529));
#94886=DIRECTION('center_axis',(0.,1.,0.));
#94887=DIRECTION('ref_axis',(-0.596982423120826,0.,0.802254315341954));
#94888=DIRECTION('center_axis',(-0.981627005099017,0.,-0.190809912898503));
#94889=DIRECTION('ref_axis',(-0.190809912898503,0.,0.981627005099017));
#94890=DIRECTION('center_axis',(-0.981627005099017,9.21421064126766E-17,
-0.190809912898504));
#94891=DIRECTION('ref_axis',(-0.18919971148133,-0.129639237201797,0.97334327826986));
#94892=DIRECTION('center_axis',(-0.981627005099017,4.83300873917615E-17,
-0.190809912898504));
#94893=DIRECTION('ref_axis',(-0.189274619583568,-0.126600331929198,0.973728645124971));
#94894=DIRECTION('center_axis',(0.,-1.,0.));
#94895=DIRECTION('ref_axis',(0.,0.,-1.));
#94896=DIRECTION('',(-0.190809912898503,0.,0.981627005099017));
#94897=DIRECTION('center_axis',(0.,-1.,0.));
#94898=DIRECTION('ref_axis',(-0.574744679387081,0.,0.818332788977835));
#94899=DIRECTION('',(-0.190809912898503,0.,0.981627005099017));
#94900=DIRECTION('center_axis',(0.,-1.,0.));
#94901=DIRECTION('ref_axis',(-0.567756991666042,0.,0.823196208940691));
#94902=DIRECTION('center_axis',(0.981627005099017,0.,0.190809912898503));
#94903=DIRECTION('ref_axis',(0.,-1.,0.));
#94904=DIRECTION('',(-0.190809912898503,0.,0.981627005099017));
#94905=DIRECTION('center_axis',(0.981627005099017,-3.89875401167116E-18,
0.190809912898503));
#94906=DIRECTION('ref_axis',(-0.190766832467318,-0.0212485861060798,0.981405376599741));
#94907=DIRECTION('center_axis',(0.981627005099017,4.25575130846528E-18,
0.190809912898503));
#94908=DIRECTION('ref_axis',(-0.190768766076259,-0.0207663068492494,0.981415324105745));
#94909=DIRECTION('center_axis',(0.,1.,0.));
#94910=DIRECTION('ref_axis',(1.,0.,0.));
#94911=DIRECTION('',(-0.190809912898503,0.,0.981627005099017));
#94912=DIRECTION('center_axis',(0.,1.,0.));
#94913=DIRECTION('ref_axis',(-0.60318791972257,0.,0.797599105754739));
#94914=DIRECTION('center_axis',(0.,1.,0.));
#94915=DIRECTION('ref_axis',(-0.595738743977029,0.,0.803178279664404));
#94916=DIRECTION('center_axis',(-0.981627005099017,0.,-0.190809912898503));
#94917=DIRECTION('ref_axis',(-0.190809912898503,0.,0.981627005099017));
#94918=DIRECTION('center_axis',(-0.981627005099017,-2.30355266031692E-18,
-0.190809912898503));
#94919=DIRECTION('ref_axis',(-0.190492927159314,-0.0576174387563383,0.979996262979322));
#94920=DIRECTION('center_axis',(-0.981627005099017,1.75745772333678E-17,
-0.190809912898504));
#94921=DIRECTION('ref_axis',(-0.190507625712308,-0.0562668141907479,0.980071880101803));
#94922=DIRECTION('center_axis',(0.,-1.,0.));
#94923=DIRECTION('ref_axis',(0.,0.,-1.));
#94924=DIRECTION('',(-0.190809912898503,0.,0.981627005099017));
#94925=DIRECTION('center_axis',(0.,-1.,0.));
#94926=DIRECTION('ref_axis',(0.324163687217122,0.,0.946001006283714));
#94927=DIRECTION('',(-0.190809912898493,0.,0.981627005099019));
#94928=DIRECTION('center_axis',(0.,-1.,0.));
#94929=DIRECTION('ref_axis',(0.313789016047043,0.,0.949492734784331));
#94930=DIRECTION('center_axis',(0.981627005099017,0.,0.190809912898503));
#94931=DIRECTION('ref_axis',(0.,-1.,0.));
#94932=DIRECTION('',(-0.190809912898503,0.,0.981627005099017));
#94933=DIRECTION('center_axis',(0.981627005099017,-1.7295648605066E-17,
0.190809912898504));
#94934=DIRECTION('ref_axis',(-0.190762133968866,-0.0223771900686593,0.98138120504128));
#94935=DIRECTION('center_axis',(0.981627005099017,-2.11358402187499E-17,
0.190809912898504));
#94936=DIRECTION('ref_axis',(-0.19076450076384,-0.021815976042031,0.981393381085106));
#94937=DIRECTION('center_axis',(0.,1.,0.));
#94938=DIRECTION('ref_axis',(1.,0.,0.));
#94939=DIRECTION('',(-0.190809912898503,0.,0.981627005099017));
#94940=DIRECTION('center_axis',(0.,1.,0.));
#94941=DIRECTION('ref_axis',(0.288388637747114,0.,0.95751344304838));
#94942=DIRECTION('center_axis',(0.,1.,0.));
#94943=DIRECTION('ref_axis',(0.278801885864545,0.,0.960348639004801));
#94944=DIRECTION('center_axis',(-0.981627005099017,0.,-0.190809912898503));
#94945=DIRECTION('ref_axis',(-0.190809912898503,0.,0.981627005099017));
#94946=DIRECTION('center_axis',(-0.981627005099017,2.13522126074254E-17,
-0.190809912898504));
#94947=DIRECTION('ref_axis',(-0.190483435767225,-0.0584729580020077,0.979947434243699));
#94948=DIRECTION('center_axis',(-0.981627005099017,-1.80753010452426E-17,
-0.190809912898503));
#94949=DIRECTION('ref_axis',(-0.190499006107751,-0.0570627440812116,0.980027536301854));
#94950=DIRECTION('center_axis',(0.,-1.,0.));
#94951=DIRECTION('ref_axis',(0.,0.,-1.));
#94952=DIRECTION('',(-0.190809912898503,0.,0.981627005099017));
#94953=DIRECTION('center_axis',(0.,-1.,0.));
#94954=DIRECTION('ref_axis',(0.327157586265152,0.,0.94496979515176));
#94955=DIRECTION('',(-0.190809912898514,0.,0.981627005099015));
#94956=DIRECTION('center_axis',(0.,-1.,0.));
#94957=DIRECTION('ref_axis',(0.31660664489919,0.,0.948556921015116));
#94958=DIRECTION('center_axis',(0.981627005099017,0.,0.190809912898503));
#94959=DIRECTION('ref_axis',(0.,-1.,0.));
#94960=DIRECTION('',(-0.190809912898503,0.,0.981627005099017));
#94961=DIRECTION('center_axis',(0.981627005099017,-6.17701735895213E-17,
0.190809912898504));
#94962=DIRECTION('ref_axis',(-0.189910724397473,-0.0969678236308587,0.977001104369448));
#94963=DIRECTION('center_axis',(0.981627005099017,2.58326936006944E-17,
0.190809912898503));
#94964=DIRECTION('ref_axis',(-0.189955361826545,-0.0945358961821438,0.977230742888488));
#94965=DIRECTION('center_axis',(0.,1.,0.));
#94966=DIRECTION('ref_axis',(1.,0.,0.));
#94967=DIRECTION('',(-0.190809912898503,0.,0.981627005099017));
#94968=DIRECTION('center_axis',(0.,1.,0.));
#94969=DIRECTION('ref_axis',(0.290085054729223,0.,0.957000867827581));
#94970=DIRECTION('center_axis',(0.,1.,0.));
#94971=DIRECTION('ref_axis',(0.280399314101408,0.,0.959883443263535));
#94972=DIRECTION('center_axis',(-0.981627005099017,0.,-0.190809912898503));
#94973=DIRECTION('ref_axis',(-0.190809912898503,0.,0.981627005099017));
#94974=DIRECTION('center_axis',(-0.981627005099017,-9.48987226996683E-18,
-0.190809912898503));
#94975=DIRECTION('ref_axis',(-0.189151327895628,-0.131564155504506,0.973094367541867));
#94976=DIRECTION('center_axis',(-0.981627005099017,9.94141557488341E-17,
-0.190809912898504));
#94977=DIRECTION('ref_axis',(-0.189230694466041,-0.128391174182701,0.973502671112867));
#94978=DIRECTION('center_axis',(0.,-1.,0.));
#94979=DIRECTION('ref_axis',(0.,0.,-1.));
#94980=DIRECTION('',(-0.190809912898503,0.,0.981627005099017));
#94981=DIRECTION('center_axis',(0.,-1.,0.));
#94982=DIRECTION('ref_axis',(0.332583332787186,0.,0.943073871312406));
#94983=DIRECTION('',(-0.190809912898503,0.,0.981627005099017));
#94984=DIRECTION('center_axis',(0.,-1.,0.));
#94985=DIRECTION('ref_axis',(0.321708056003748,0.,0.946838912752475));
#94986=DIRECTION('center_axis',(0.981627005099017,0.,0.190809912898503));
#94987=DIRECTION('ref_axis',(0.,-1.,0.));
#94988=DIRECTION('',(-0.190809912898503,0.,0.981627005099017));
#94989=DIRECTION('center_axis',(0.981627005099017,-4.44745249844553E-17,
0.190809912898503));
#94990=DIRECTION('ref_axis',(-0.187980954040593,-0.171558457193103,0.967073346072319));
#94991=DIRECTION('center_axis',(0.981627005099017,-7.98465074930554E-17,
0.190809912898504));
#94992=DIRECTION('ref_axis',(-0.18812207510112,-0.167255816322301,0.967799347368043));
#94993=DIRECTION('center_axis',(0.,1.,0.));
#94994=DIRECTION('ref_axis',(1.,0.,0.));
#94995=DIRECTION('',(-0.190809912898503,0.,0.981627005099017));
#94996=DIRECTION('center_axis',(0.,1.,0.));
#94997=DIRECTION('ref_axis',(0.293968036548532,0.,0.955815250708944));
#94998=DIRECTION('center_axis',(0.,1.,0.));
#94999=DIRECTION('ref_axis',(0.284053252507605,0.,0.958808505250058));
#95000=DIRECTION('center_axis',(-0.981627005099017,0.,-0.190809912898503));
#95001=DIRECTION('ref_axis',(-0.190809912898503,0.,0.981627005099017));
#95002=DIRECTION('center_axis',(-0.981627005099017,-9.01537865646849E-17,
-0.190809912898503));
#95003=DIRECTION('ref_axis',(-0.186771248501737,-0.204655353007008,0.960849981640568));
#95004=DIRECTION('center_axis',(-0.981627005099017,9.03765052262128E-18,
-0.190809912898503));
#95005=DIRECTION('ref_axis',(-0.186965682920001,-0.1997196042842,0.961850255016247));
#95006=DIRECTION('center_axis',(0.,-1.,0.));
#95007=DIRECTION('ref_axis',(0.,0.,-1.));
#95008=DIRECTION('',(-0.190809912898503,0.,0.981627005099017));
#95009=DIRECTION('center_axis',(0.,-1.,0.));
#95010=DIRECTION('ref_axis',(0.340670977220966,0.,0.94018258082104));
#95011=DIRECTION('',(-0.190809912898503,0.,0.981627005099017));
#95012=DIRECTION('center_axis',(0.,-1.,0.));
#95013=DIRECTION('ref_axis',(0.329300453690895,0.,0.944225190936448));
#95014=DIRECTION('center_axis',(0.981627005099017,0.,0.190809912898503));
#95015=DIRECTION('ref_axis',(0.,-1.,0.));
#95016=DIRECTION('',(-0.190809912898503,0.,0.981627005099017));
#95017=DIRECTION('center_axis',(0.981627005099017,3.95329110972936E-17,
0.190809912898503));
#95018=DIRECTION('ref_axis',(-0.184939069098101,-0.246149090755304,0.951424282768453));
#95019=DIRECTION('center_axis',(0.981627005099017,5.63622405833332E-17,
0.190809912898503));
#95020=DIRECTION('ref_axis',(-0.185234234721259,-0.239975736462394,0.952942770682773));
#95021=DIRECTION('center_axis',(0.,1.,0.));
#95022=DIRECTION('ref_axis',(1.,0.,0.));
#95023=DIRECTION('',(-0.190809912898503,0.,0.981627005099017));
#95024=DIRECTION('center_axis',(0.,1.,0.));
#95025=DIRECTION('ref_axis',(0.300197402785575,0.,0.953877098666697));
#95026=DIRECTION('center_axis',(0.,1.,0.));
#95027=DIRECTION('ref_axis',(0.289907957000668,0.,0.957054531606062));
#95028=DIRECTION('center_axis',(-0.981627005099017,0.,-0.190809912898503));
#95029=DIRECTION('ref_axis',(-0.190809912898503,0.,0.981627005099017));
#95030=DIRECTION('center_axis',(-0.981627005099017,1.04388594969635E-16,
-0.190809912898504));
#95031=DIRECTION('ref_axis',(-0.183302380149146,-0.277746550509493,0.943004290081299));
#95032=DIRECTION('center_axis',(-0.981627005099017,9.94141557488341E-17,
-0.190809912898504));
#95033=DIRECTION('ref_axis',(-0.183667100790987,-0.271048034385807,0.944880605760656));
#95034=DIRECTION('center_axis',(-0.981627005099017,0.,-0.190809912898503));
#95035=DIRECTION('ref_axis',(-0.190809912898503,0.,0.981627005099017));
#95036=DIRECTION('',(-0.190809912898503,0.,0.981627005099017));
#95037=DIRECTION('center_axis',(-0.981627005099017,2.84696168099005E-17,
-0.190809912898503));
#95038=DIRECTION('ref_axis',(-0.178681321768697,-0.350837748012096,0.919231124266793));
#95039=DIRECTION('',(-0.190809912898503,0.,0.981627005099017));
#95040=DIRECTION('center_axis',(-0.981627005099017,-1.08451806271455E-16,
-0.190809912898503));
#95041=DIRECTION('ref_axis',(-0.179277906329184,-0.342376464487307,0.922300270447427));
#95042=DIRECTION('center_axis',(0.,-1.,0.));
#95043=DIRECTION('ref_axis',(0.,0.,-1.));
#95044=DIRECTION('',(-0.190809912898483,0.,0.981627005099021));
#95045=DIRECTION('',(0.981627005099017,0.,0.190809912898503));
#95046=DIRECTION('center_axis',(0.,-1.,0.));
#95047=DIRECTION('ref_axis',(0.321307357956275,0.,0.946974963620031));
#95048=DIRECTION('center_axis',(0.,-1.,0.));
#95049=DIRECTION('ref_axis',(0.339712961600918,0.,0.940529161547016));
#95050=DIRECTION('center_axis',(0.981627005099017,0.,0.190809912898503));
#95051=DIRECTION('ref_axis',(0.,-1.,0.));
#95052=DIRECTION('',(-0.190809912898503,0.,0.981627005099017));
#95053=DIRECTION('',(0.,1.,0.));
#95054=DIRECTION('center_axis',(0.981627005099017,-1.40905601458333E-16,
0.190809912898504));
#95055=DIRECTION('ref_axis',(-0.181241438981021,-0.3126956566025,0.932401719827897));
#95056=DIRECTION('center_axis',(0.,1.,0.));
#95057=DIRECTION('ref_axis',(1.,0.,0.));
#95058=DIRECTION('center_axis',(0.,1.,0.));
#95059=DIRECTION('ref_axis',(0.30904404227791,0.,0.951047727473511));
#95060=DIRECTION('',(-0.981627005099017,0.,-0.190809912898503));
#95061=DIRECTION('center_axis',(0.,1.,0.));
#95062=DIRECTION('ref_axis',(0.298207091960414,0.,0.954501194501355));
#95063=DIRECTION('center_axis',(-0.190809912898503,0.,0.981627005099017));
#95064=DIRECTION('ref_axis',(0.,1.,0.));
#95065=DIRECTION('center_axis',(0.190809912898504,-3.49693752527234E-16,
-0.981627005099017));
#95066=DIRECTION('ref_axis',(0.85426207248107,-0.492608222327907,0.166052554377481));
#95067=DIRECTION('center_axis',(0.,1.,0.));
#95068=DIRECTION('ref_axis',(1.,0.,0.));
#95069=DIRECTION('',(-0.190809912898503,0.,0.981627005099017));
#95070=DIRECTION('center_axis',(0.,1.,0.));
#95071=DIRECTION('ref_axis',(0.246498687235726,0.,0.969143125235413));
#95072=DIRECTION('',(-0.190809912898503,0.,0.981627005099017));
#95073=DIRECTION('center_axis',(0.,1.,0.));
#95074=DIRECTION('ref_axis',(0.236678365804582,0.,0.971588056307853));
#95075=DIRECTION('center_axis',(-0.981627005099017,0.,-0.190809912898503));
#95076=DIRECTION('ref_axis',(-0.190809912898503,0.,0.981627005099017));
#95077=DIRECTION('',(-0.190809912898503,0.,0.981627005099017));
#95078=DIRECTION('center_axis',(-0.981627005099017,1.77118070983607E-16,
-0.190809912898504));
#95079=DIRECTION('ref_axis',(-0.174075761005115,-0.409523969629305,0.895537686381509));
#95080=DIRECTION('center_axis',(-0.981627005099017,-1.69216540445236E-17,
-0.190809912898503));
#95081=DIRECTION('ref_axis',(-0.174856431613847,-0.40028498107098,0.899553868454957));
#95082=DIRECTION('center_axis',(0.,-1.,0.));
#95083=DIRECTION('ref_axis',(0.,0.,-1.));
#95084=DIRECTION('',(-0.190809912898503,0.,0.981627005099017));
#95085=DIRECTION('',(0.981627005099017,0.,0.190809912898503));
#95086=DIRECTION('center_axis',(0.,-1.,0.));
#95087=DIRECTION('ref_axis',(0.27693655485013,0.,0.960888206082134));
#95088=DIRECTION('center_axis',(0.,-1.,0.));
#95089=DIRECTION('ref_axis',(0.279101841281133,0.,0.960261507191391));
#95090=DIRECTION('center_axis',(0.981627005099017,0.,0.190809912898503));
#95091=DIRECTION('ref_axis',(0.,-1.,0.));
#95092=DIRECTION('center_axis',(0.981627005099017,-1.0065149107169E-16,
0.190809912898504));
#95093=DIRECTION('ref_axis',(-0.176466315004732,-0.38038600246631,0.907835959188856));
#95094=DIRECTION('',(0.,1.,0.));
#95095=DIRECTION('center_axis',(0.981627005099017,0.,0.190809912898503));
#95096=DIRECTION('ref_axis',(-0.177151986277243,-0.371529138153602,0.911363414484513));
#95097=DIRECTION('center_axis',(-0.190809912898503,0.,0.981627005099017));
#95098=DIRECTION('ref_axis',(0.,1.,0.));
#95099=DIRECTION('center_axis',(0.190809912898503,4.4294541986783E-16,-0.981627005099017));
#95100=DIRECTION('ref_axis',(0.753450111070955,-0.640986267800124,0.146456596365046));
#95101=DIRECTION('center_axis',(0.,-1.,0.));
#95102=DIRECTION('ref_axis',(0.,0.,-1.));
#95103=DIRECTION('',(-0.190809912898503,0.,0.981627005099017));
#95104=DIRECTION('center_axis',(0.,-1.,0.));
#95105=DIRECTION('ref_axis',(0.215356558023971,0.,0.976535484719356));
#95106=DIRECTION('',(-0.190809912898503,0.,0.981627005099017));
#95107=DIRECTION('center_axis',(0.,-1.,0.));
#95108=DIRECTION('ref_axis',(0.206031581908636,0.,0.9785453424631));
#95109=DIRECTION('center_axis',(0.981627005099017,0.,0.190809912898503));
#95110=DIRECTION('ref_axis',(0.,-1.,0.));
#95111=DIRECTION('',(-0.190809912898503,0.,0.981627005099017));
#95112=DIRECTION('center_axis',(0.981627005099017,-8.60077605075239E-17,
0.190809912898503));
#95113=DIRECTION('ref_axis',(-0.177360216447652,-0.368790379407218,0.912434660498121));
#95114=DIRECTION('center_axis',(0.981627005099017,-9.05042095782515E-17,
0.190809912898503));
#95115=DIRECTION('ref_axis',(-0.177964786864002,-0.360702216203213,0.915544890140588));
#95116=DIRECTION('center_axis',(0.,1.,0.));
#95117=DIRECTION('ref_axis',(1.,0.,0.));
#95118=DIRECTION('',(-0.190809912898503,0.,0.981627005099017));
#95119=DIRECTION('center_axis',(0.,1.,0.));
#95120=DIRECTION('ref_axis',(0.173299588604038,0.,0.984869155060545));
#95121=DIRECTION('center_axis',(0.,1.,0.));
#95122=DIRECTION('ref_axis',(0.165191125635383,0.,0.986261573828827));
#95123=DIRECTION('center_axis',(-0.981627005099017,0.,-0.190809912898503));
#95124=DIRECTION('ref_axis',(-0.190809912898503,0.,0.981627005099017));
#95125=DIRECTION('center_axis',(-0.981627005099017,4.10603095522234E-16,
-0.190809912898504));
#95126=DIRECTION('ref_axis',(-0.175016396158809,-0.398360213910187,0.90037681059044));
#95127=DIRECTION('center_axis',(-0.981627005099017,4.01253885915747E-17,
-0.190809912898503));
#95128=DIRECTION('ref_axis',(-0.17571344921673,-0.38984099858382,0.90396281980374));
#95129=DIRECTION('center_axis',(0.,-1.,0.));
#95130=DIRECTION('ref_axis',(0.,0.,-1.));
#95131=DIRECTION('',(-0.190809912898503,0.,0.981627005099017));
#95132=DIRECTION('center_axis',(0.,-1.,0.));
#95133=DIRECTION('ref_axis',(0.141672460290673,0.,0.989913589155734));
#95134=DIRECTION('',(-0.190809912898503,0.,0.981627005099017));
#95135=DIRECTION('center_axis',(0.,-1.,0.));
#95136=DIRECTION('ref_axis',(0.134100681649831,0.,0.990967712481618));
#95137=DIRECTION('center_axis',(0.981627005099017,0.,0.190809912898503));
#95138=DIRECTION('ref_axis',(0.,-1.,0.));
#95139=DIRECTION('',(-0.190809912898503,0.,0.981627005099017));
#95140=DIRECTION('center_axis',(0.981627005099017,-1.14638278569454E-16,
0.190809912898504));
#95141=DIRECTION('ref_axis',(-0.178028194999365,-0.359841769342607,0.915871095090161));
#95142=DIRECTION('center_axis',(0.981627005099017,-3.53229335734846E-16,
0.190809912898504));
#95143=DIRECTION('ref_axis',(-0.178575361030583,-0.352316423630891,0.918686006246277));
#95144=DIRECTION('center_axis',(0.,1.,0.));
#95145=DIRECTION('ref_axis',(1.,0.,0.));
#95146=DIRECTION('',(-0.190809912898503,0.,0.981627005099017));
#95147=DIRECTION('center_axis',(0.,1.,0.));
#95148=DIRECTION('ref_axis',(0.101214401296622,0.,0.994864636505975));
#95149=DIRECTION('center_axis',(0.,1.,0.));
#95150=DIRECTION('ref_axis',(0.0947603432797819,0.,0.995500114184573));
#95151=DIRECTION('center_axis',(-0.981627005099017,0.,-0.190809912898503));
#95152=DIRECTION('ref_axis',(-0.190809912898503,0.,0.981627005099017));
#95153=DIRECTION('center_axis',(-0.981627005099017,2.56763337521845E-16,
-0.190809912898504));
#95154=DIRECTION('ref_axis',(-0.175715849516705,-0.389811281877913,0.903975168214991));
#95155=DIRECTION('center_axis',(-0.981627005099017,3.77210004092943E-16,
-0.190809912898504));
#95156=DIRECTION('ref_axis',(-0.176353679441912,-0.381818043972282,0.907256502343455));
#95157=DIRECTION('center_axis',(0.,-1.,0.));
#95158=DIRECTION('ref_axis',(0.,0.,-1.));
#95159=DIRECTION('',(-0.190809912898503,-1.328769267093E-14,0.981627005099017));
#95160=DIRECTION('center_axis',(0.,-1.,0.));
#95161=DIRECTION('ref_axis',(0.0690927304182998,0.,0.997610241829616));
#95162=DIRECTION('',(-0.190809912898503,0.,0.981627005099017));
#95163=DIRECTION('center_axis',(0.,-1.,0.));
#95164=DIRECTION('ref_axis',(0.063217557275382,0.,0.997999769765572));
#95165=DIRECTION('center_axis',(0.981627005099017,0.,0.190809912898503));
#95166=DIRECTION('ref_axis',(0.,-1.,0.));
#95167=DIRECTION('',(-0.190809912898503,0.,0.981627005099017));
#95168=DIRECTION('center_axis',(0.981627005099017,-3.15328006926456E-17,
0.190809912898503));
#95169=DIRECTION('ref_axis',(-0.178521093013203,-0.353070994296397,0.918406822892734));
#95170=DIRECTION('center_axis',(0.981627005099017,-3.33018562685204E-16,
0.190809912898504));
#95171=DIRECTION('ref_axis',(-0.179027665935153,-0.34595423082879,0.921012901647676));
#95172=DIRECTION('center_axis',(0.,1.,0.));
#95173=DIRECTION('ref_axis',(1.,0.,0.));
#95174=DIRECTION('',(-0.190809912898503,0.,0.981627005099017));
#95175=DIRECTION('center_axis',(0.,1.,0.));
#95176=DIRECTION('ref_axis',(0.0301623710479701,0.,0.999545012179424));
#95177=DIRECTION('center_axis',(0.,1.,0.));
#95178=DIRECTION('ref_axis',(0.0253129510981065,0.,0.999679575917556));
#95179=DIRECTION('center_axis',(-0.981627005099017,0.,-0.190809912898503));
#95180=DIRECTION('ref_axis',(-0.190809912898503,0.,0.981627005099017));
#95181=DIRECTION('center_axis',(-0.981627005099017,0.,-0.190809912898503));
#95182=DIRECTION('ref_axis',(-0.176224298070495,-0.383455269460088,0.906590896211104));
#95183=DIRECTION('center_axis',(-0.981627005099017,1.41720243526492E-16,
-0.190809912898504));
#95184=DIRECTION('ref_axis',(-0.176820667107078,-0.375839162626588,0.909658933622901));
#95185=DIRECTION('center_axis',(0.,-1.,0.));
#95186=DIRECTION('ref_axis',(0.,0.,-1.));
#95187=DIRECTION('',(-0.190809912898503,0.,0.981627005099017));
#95188=DIRECTION('center_axis',(0.,-1.,0.));
#95189=DIRECTION('ref_axis',(-0.00245485281101381,0.,0.999996986844299));
#95190=DIRECTION('',(-0.190809912898503,0.,0.981627005099017));
#95191=DIRECTION('center_axis',(0.,-1.,0.));
#95192=DIRECTION('ref_axis',(-0.00668313312353966,0.,0.999977667616459));
#95193=DIRECTION('center_axis',(0.981627005099017,0.,0.190809912898503));
#95194=DIRECTION('ref_axis',(0.,-1.,0.));
#95195=DIRECTION('',(-0.190809912898503,0.,0.981627005099017));
#95196=DIRECTION('center_axis',(0.981627005099017,0.,0.190809912898503));
#95197=DIRECTION('ref_axis',(-0.178871820110591,-0.348161333804301,0.920211148386029));
#95198=DIRECTION('center_axis',(0.981627005099017,-2.43133958356391E-16,
0.190809912898504));
#95199=DIRECTION('ref_axis',(-0.179350425520556,-0.341331684304794,0.922673347482872));
#95200=DIRECTION('center_axis',(0.,1.,0.));
#95201=DIRECTION('ref_axis',(1.,0.,0.));
#95202=DIRECTION('',(-0.190809912898503,0.,0.981627005099017));
#95203=DIRECTION('center_axis',(0.,1.,0.));
#95204=DIRECTION('ref_axis',(-0.0399134285534144,0.,0.999203141618916));
#95205=DIRECTION('center_axis',(0.,1.,0.));
#95206=DIRECTION('ref_axis',(-0.0432028268842918,0.,0.999066321997297));
#95207=DIRECTION('center_axis',(-0.981627005099017,0.,-0.190809912898503));
#95208=DIRECTION('ref_axis',(-0.190809912898503,0.,0.981627005099017));
#95209=DIRECTION('center_axis',(-0.981627005099017,4.55117302256744E-17,
-0.190809912898503));
#95210=DIRECTION('ref_axis',(-0.176574195062516,-0.379008487252018,0.908390951203809));
#95211=DIRECTION('center_axis',(-0.981627005099017,3.20917534544763E-16,
-0.190809912898504));
#95212=DIRECTION('ref_axis',(-0.177142812401908,-0.371649260184588,0.911316219222829));
#95213=DIRECTION('center_axis',(0.,-1.,0.));
#95214=DIRECTION('ref_axis',(0.,0.,-1.));
#95215=DIRECTION('',(-0.190809912898503,0.,0.981627005099017));
#95216=DIRECTION('center_axis',(0.,-1.,0.));
#95217=DIRECTION('ref_axis',(-0.0730201753284488,0.,0.997330463785702));
#95218=DIRECTION('',(-0.190809912898503,0.,0.981627005099017));
#95219=DIRECTION('center_axis',(0.,-1.,0.));
#95220=DIRECTION('ref_axis',(-0.0756467337952682,0.,0.997134680806012));
#95221=DIRECTION('center_axis',(0.981627005099017,0.,0.190809912898503));
#95222=DIRECTION('ref_axis',(0.,-1.,0.));
#95223=DIRECTION('',(-0.190809912898503,0.,0.981627005099017));
#95224=DIRECTION('center_axis',(0.981627005099017,-3.00905960538911E-17,
0.190809912898503));
#95225=DIRECTION('ref_axis',(-0.179101543646402,-0.344902357589395,0.921392967627143));
#95226=DIRECTION('center_axis',(0.981627005099017,-1.01299069034784E-16,
0.190809912898504));
#95227=DIRECTION('ref_axis',(-0.179562245131546,-0.338259087198216,0.92376305947529));
#95228=DIRECTION('center_axis',(0.,1.,0.));
#95229=DIRECTION('ref_axis',(1.,0.,0.));
#95230=DIRECTION('',(-0.190809912898503,0.,0.981627005099017));
#95231=DIRECTION('center_axis',(0.,1.,0.));
#95232=DIRECTION('ref_axis',(-0.109051309513976,0.,0.994036122026401));
#95233=DIRECTION('center_axis',(0.,1.,0.));
#95234=DIRECTION('ref_axis',(-0.110821964250551,0.,0.993840275013872));
#95235=DIRECTION('center_axis',(-0.981627005099017,0.,-0.190809912898503));
#95236=DIRECTION('ref_axis',(-0.190809912898503,0.,0.981627005099017));
#95237=DIRECTION('center_axis',(-0.981627005099017,3.06546241321686E-16,
-0.190809912898504));
#95238=DIRECTION('ref_axis',(-0.176786003350799,-0.376286776602481,0.909480604946233));
#95239=DIRECTION('center_axis',(-0.981627005099017,-2.15794885179139E-17,
-0.190809912898503));
#95240=DIRECTION('ref_axis',(-0.177338131232431,-0.369081972811902,0.91232104248245));
#95241=DIRECTION('center_axis',(0.,-1.,0.));
#95242=DIRECTION('ref_axis',(0.,0.,-1.));
#95243=DIRECTION('',(-0.190809912898503,0.,0.981627005099017));
#95244=DIRECTION('center_axis',(0.,-1.,0.));
#95245=DIRECTION('ref_axis',(-0.142635241858787,0.,0.989775321868496));
#95246=DIRECTION('',(-0.190809912898503,0.,0.981627005099017));
#95247=DIRECTION('center_axis',(0.,-1.,0.));
#95248=DIRECTION('ref_axis',(-0.143702428046443,0.,0.98962094368175));
#95249=DIRECTION('center_axis',(0.981627005099017,0.,0.190809912898503));
#95250=DIRECTION('ref_axis',(0.,-1.,0.));
#95251=DIRECTION('',(-0.190809912898503,0.,0.981627005099017));
#95252=DIRECTION('center_axis',(0.981627005099017,-9.68104844745577E-17,
0.190809912898503));
#95253=DIRECTION('ref_axis',(-0.179223155950715,-0.343162864172706,0.922018605573581));
#95254=DIRECTION('center_axis',(0.981627005099017,-1.71974336430998E-16,
0.190809912898504));
#95255=DIRECTION('ref_axis',(-0.179674512482127,-0.336617711962109,0.924340622042386));
#95256=DIRECTION('center_axis',(0.,1.,0.));
#95257=DIRECTION('ref_axis',(1.,0.,0.));
#95258=DIRECTION('',(-0.190809912898503,0.,0.981627005099017));
#95259=DIRECTION('center_axis',(0.,1.,0.));
#95260=DIRECTION('ref_axis',(-0.177274123368118,0.,0.984161513768988));
#95261=DIRECTION('center_axis',(0.,1.,0.));
#95262=DIRECTION('ref_axis',(-0.1775653711205,0.,0.984109007670817));
#95263=DIRECTION('center_axis',(-0.981627005099017,0.,-0.190809912898503));
#95264=DIRECTION('ref_axis',(-0.190809912898503,0.,0.981627005099017));
#95265=DIRECTION('center_axis',(-0.981627005099017,3.56781022098411E-16,
-0.190809912898504));
#95266=DIRECTION('ref_axis',(-0.176871394992535,-0.375182990983614,0.90991990466743));
#95267=DIRECTION('center_axis',(-0.981627005099017,1.71662726916883E-16,
-0.190809912898504));
#95268=DIRECTION('ref_axis',(-0.177416941265172,-0.368040210182297,0.912726482929624));
#95269=DIRECTION('center_axis',(0.,-1.,0.));
#95270=DIRECTION('ref_axis',(0.,0.,-1.));
#95271=DIRECTION('',(-0.190809912898503,0.,0.981627005099017));
#95272=DIRECTION('center_axis',(0.,-1.,0.));
#95273=DIRECTION('ref_axis',(-0.21131678201032,0.,0.97741762703606));
#95274=DIRECTION('',(-0.190809912898503,1.372221714061E-14,0.981627005099017));
#95275=DIRECTION('center_axis',(0.,-1.,0.));
#95276=DIRECTION('ref_axis',(-0.210865499794873,0.,0.977515084792178));
#95277=DIRECTION('center_axis',(0.981627005099017,0.,0.190809912898503));
#95278=DIRECTION('ref_axis',(0.,-1.,0.));
#95279=DIRECTION('',(-0.190809912898503,0.,0.981627005099017));
#95280=DIRECTION('center_axis',(0.981627005099017,-3.56855682945794E-16,
0.190809912898504));
#95281=DIRECTION('ref_axis',(-0.179243179230579,-0.342875499534802,0.922121615904364));
#95282=DIRECTION('center_axis',(0.981627005099017,-1.43081078683219E-16,
0.190809912898504));
#95283=DIRECTION('ref_axis',(-0.179693005975761,-0.336346465570606,0.924435762344554));
#95284=DIRECTION('center_axis',(0.,1.,0.));
#95285=DIRECTION('ref_axis',(1.,0.,0.));
#95286=DIRECTION('',(-0.190809912898503,0.,0.981627005099017));
#95287=DIRECTION('center_axis',(0.,1.,0.));
#95288=DIRECTION('ref_axis',(-0.244591010378231,0.,0.969626339185439));
#95289=DIRECTION('center_axis',(0.,1.,0.));
#95290=DIRECTION('ref_axis',(-0.243441421751623,0.,0.96991560157343));
#95291=DIRECTION('center_axis',(-0.981627005099017,0.,-0.190809912898503));
#95292=DIRECTION('ref_axis',(-0.190809912898503,0.,0.981627005099017));
#95293=DIRECTION('center_axis',(-0.981627005099017,2.98065849465872E-17,
-0.190809912898503));
#95294=DIRECTION('ref_axis',(-0.176834926434283,-0.375654851236703,0.909732291135866));
#95295=DIRECTION('center_axis',(-0.981627005099017,-5.01895501974238E-17,
-0.190809912898503));
#95296=DIRECTION('ref_axis',(-0.177383278884452,-0.368485598551699,0.912553305857908));
#95297=DIRECTION('center_axis',(0.,-1.,0.));
#95298=DIRECTION('ref_axis',(0.,0.,-1.));
#95299=DIRECTION('',(-0.190809912898503,0.,0.981627005099017));
#95300=DIRECTION('center_axis',(0.,-1.,0.));
#95301=DIRECTION('ref_axis',(-0.279067536185833,0.,0.960271477368337));
#95302=DIRECTION('',(-0.190809912898503,0.,0.981627005099017));
#95303=DIRECTION('center_axis',(0.,-1.,0.));
#95304=DIRECTION('ref_axis',(-0.277138454551981,0.,0.960829993811881));
#95305=DIRECTION('center_axis',(0.981627005099017,0.,0.190809912898503));
#95306=DIRECTION('ref_axis',(0.,-1.,0.));
#95307=DIRECTION('',(-0.190809912898503,0.,0.981627005099017));
#95308=DIRECTION('center_axis',(0.981627005099017,-1.94599946632004E-16,
0.190809912898504));
#95309=DIRECTION('ref_axis',(-0.179162667562163,-0.344029312691491,0.92170742134423));
#95310=DIRECTION('center_axis',(0.981627005099017,-1.94412209408584E-16,
0.190809912898504));
#95311=DIRECTION('ref_axis',(-0.179618660622996,-0.337435405585499,0.924053290570057));
#95312=DIRECTION('center_axis',(0.,1.,0.));
#95313=DIRECTION('ref_axis',(1.,0.,0.));
#95314=DIRECTION('',(-0.190809912898503,0.,0.981627005099017));
#95315=DIRECTION('center_axis',(0.,1.,0.));
#95316=DIRECTION('ref_axis',(-0.310998072064368,0.,0.950410542435345));
#95317=DIRECTION('center_axis',(0.,1.,0.));
#95318=DIRECTION('ref_axis',(-0.308446543639216,0.,0.951241677870046));
#95319=DIRECTION('center_axis',(-0.981627005099017,0.,-0.190809912898503));
#95320=DIRECTION('ref_axis',(-0.190809912898503,0.,0.981627005099017));
#95321=DIRECTION('center_axis',(-0.981627005099017,9.04057881831701E-17,
-0.190809912898503));
#95322=DIRECTION('ref_axis',(-0.176674662131589,-0.377720349383403,0.908907806888228));
#95323=DIRECTION('center_axis',(-0.981627005099017,5.79678245784152E-17,
-0.190809912898503));
#95324=DIRECTION('ref_axis',(-0.177235428855869,-0.370434472390808,0.911792687195297));
#95325=DIRECTION('center_axis',(0.,-1.,0.));
#95326=DIRECTION('ref_axis',(0.,0.,-1.));
#95327=DIRECTION('',(-0.190809912898503,0.,0.981627005099017));
#95328=DIRECTION('center_axis',(0.,-1.,0.));
#95329=DIRECTION('ref_axis',(-0.345876461290101,0.,0.938280061349189));
#95330=DIRECTION('',(-0.190809912898503,0.,0.981627005099017));
#95331=DIRECTION('center_axis',(0.,-1.,0.));
#95332=DIRECTION('ref_axis',(-0.342511199077206,0.,0.939513745778471));
#95333=DIRECTION('center_axis',(0.981627005099017,0.,0.190809912898503));
#95334=DIRECTION('ref_axis',(0.,-1.,0.));
#95335=DIRECTION('',(-0.190809912898503,-1.100134239348E-14,0.981627005099017));
#95336=DIRECTION('center_axis',(0.981627005099017,-1.51997840690772E-17,
0.190809912898503));
#95337=DIRECTION('ref_axis',(-0.178977348700373,-0.346668574534505,0.920754043207196));
#95338=DIRECTION('center_axis',(0.981627005099017,-6.57637322766467E-17,
0.190809912898503));
#95339=DIRECTION('ref_axis',(-0.179447688741777,-0.339924709427799,0.923173720881212));
#95340=DIRECTION('center_axis',(0.,1.,0.));
#95341=DIRECTION('ref_axis',(1.,0.,0.));
#95342=DIRECTION('',(-0.190809912898503,0.,0.981627005099017));
#95343=DIRECTION('center_axis',(0.,1.,0.));
#95344=DIRECTION('ref_axis',(-0.376478086240433,0.,0.926425523493789));
#95345=DIRECTION('center_axis',(0.,1.,0.));
#95346=DIRECTION('ref_axis',(-0.372564967779079,0.,0.928006112471127));
#95347=DIRECTION('center_axis',(-0.981627005099017,0.,-0.190809912898503));
#95348=DIRECTION('ref_axis',(-0.190809912898503,0.,0.981627005099017));
#95349=DIRECTION('center_axis',(-0.981627005099017,-1.07572079987249E-16,
-0.190809912898503));
#95350=DIRECTION('ref_axis',(-0.176381911743642,-0.381459690919397,0.907401744219911));
#95351=DIRECTION('center_axis',(-0.981627005099017,1.25537203023879E-16,
-0.190809912898504));
#95352=DIRECTION('ref_axis',(-0.176965700962373,-0.373959569196591,0.910405064402212));
#95353=DIRECTION('center_axis',(0.,-1.,0.));
#95354=DIRECTION('ref_axis',(0.,0.,-1.));
#95355=DIRECTION('',(-0.190809912898503,0.,0.981627005099017));
#95356=DIRECTION('center_axis',(0.,-1.,0.));
#95357=DIRECTION('ref_axis',(-0.4117178933269,0.,0.911311349822035));
#95358=DIRECTION('',(-0.190809912898503,0.,0.981627005099017));
#95359=DIRECTION('center_axis',(0.,-1.,0.));
#95360=DIRECTION('ref_axis',(-0.406960310608449,0.,0.913445841629089));
#95361=DIRECTION('center_axis',(0.981627005099017,0.,0.190809912898503));
#95362=DIRECTION('ref_axis',(0.,-1.,0.));
#95363=DIRECTION('',(-0.190809912898503,0.,0.981627005099017));
#95364=DIRECTION('center_axis',(0.981627005099017,-2.18020488347966E-16,
0.190809912898504));
#95365=DIRECTION('ref_axis',(-0.178677042467767,-0.350897603166811,0.919209109281865));
#95366=DIRECTION('center_axis',(0.981627005099017,4.48762447131239E-17,
0.190809912898503));
#95367=DIRECTION('ref_axis',(-0.179171085423017,-0.343908881724904,0.921750727267987));
#95368=DIRECTION('center_axis',(0.,1.,0.));
#95369=DIRECTION('ref_axis',(1.,0.,0.));
#95370=DIRECTION('',(-0.190809912898503,-1.075932076554E-14,0.981627005099017));
#95371=DIRECTION('center_axis',(0.,1.,0.));
#95372=DIRECTION('ref_axis',(-0.440999214539524,0.,0.897507488980189));
#95373=DIRECTION('center_axis',(0.,1.,0.));
#95374=DIRECTION('ref_axis',(-0.435767598225736,0.,0.900059220460839));
#95375=DIRECTION('center_axis',(-0.981627005099017,0.,-0.190809912898503));
#95376=DIRECTION('ref_axis',(-0.190809912898503,0.,0.981627005099017));
#95377=DIRECTION('center_axis',(-0.981627005099017,3.9547630621265E-16,
-0.190809912898504));
#95378=DIRECTION('ref_axis',(-0.175940012059776,-0.38702419833801,0.905128378771336));
#95379=DIRECTION('center_axis',(-0.981627005099017,1.67043077322241E-16,
-0.190809912898504));
#95380=DIRECTION('ref_axis',(-0.17655939757736,-0.379197781626803,0.908314825122012));
#95381=DIRECTION('center_axis',(0.,-1.,0.));
#95382=DIRECTION('ref_axis',(0.,0.,-1.));
#95383=DIRECTION('',(-0.190809912898503,0.,0.981627005099017));
#95384=DIRECTION('center_axis',(0.,-1.,0.));
#95385=DIRECTION('ref_axis',(-0.476549513638056,0.,0.879147633251283));
#95386=DIRECTION('',(-0.190809912898503,0.,0.981627005099017));
#95387=DIRECTION('center_axis',(0.,-1.,0.));
#95388=DIRECTION('ref_axis',(-0.470447268182042,0.,0.882428109173803));
#95389=DIRECTION('center_axis',(0.981627005099017,0.,0.190809912898503));
#95390=DIRECTION('ref_axis',(0.,-1.,0.));
#95391=DIRECTION('',(-0.190809912898503,0.,0.981627005099017));
#95392=DIRECTION('center_axis',(0.981627005099017,9.66573650244341E-17,
0.190809912898503));
#95393=DIRECTION('ref_axis',(-0.178244202499692,-0.35689266000621,0.916982351797972));
#95394=DIRECTION('center_axis',(0.981627005099017,-2.16345510275123E-16,
0.190809912898504));
#95395=DIRECTION('ref_axis',(-0.178773394006849,-0.3495470901574,0.919704792505599));
#95396=DIRECTION('center_axis',(0.,1.,0.));
#95397=DIRECTION('ref_axis',(1.,0.,0.));
#95398=DIRECTION('',(-0.190809912898503,0.,0.981627005099017));
#95399=DIRECTION('center_axis',(0.,1.,0.));
#95400=DIRECTION('ref_axis',(-0.504512466774432,0.,0.863404407487695));
#95401=DIRECTION('center_axis',(0.,1.,0.));
#95402=DIRECTION('ref_axis',(-0.498009804424277,0.,0.867171398684997));
#95403=DIRECTION('center_axis',(-0.981627005099017,0.,-0.190809912898503));
#95404=DIRECTION('ref_axis',(-0.190809912898503,0.,0.981627005099017));
#95405=DIRECTION('center_axis',(-0.981627005099017,2.46733951980072E-17,
-0.190809912898503));
#95406=DIRECTION('ref_axis',(-0.175321820541314,-0.394654189483089,0.901948074982992));
#95407=DIRECTION('center_axis',(-0.981627005099017,1.26122107472685E-16,
-0.190809912898504));
#95408=DIRECTION('ref_axis',(-0.175992702275721,-0.386365647532587,0.905399445080686));
#95409=DIRECTION('center_axis',(0.,-1.,0.));
#95410=DIRECTION('ref_axis',(0.,0.,-1.));
#95411=DIRECTION('',(-0.190809912898503,0.,0.981627005099017));
#95412=DIRECTION('center_axis',(0.,-1.,0.));
#95413=DIRECTION('ref_axis',(-0.540308722347473,0.,0.841466864799346));
#95414=DIRECTION('',(-0.190809912898503,0.,0.981627005099017));
#95415=DIRECTION('center_axis',(0.,-1.,0.));
#95416=DIRECTION('ref_axis',(-0.53291531834023,0.,0.84616857864041));
#95417=DIRECTION('center_axis',(0.981627005099017,0.,0.190809912898503));
#95418=DIRECTION('ref_axis',(0.,-1.,0.));
#95419=DIRECTION('',(-0.190809912898503,0.,0.981627005099017));
#95420=DIRECTION('center_axis',(0.981627005099017,-4.29489751050862E-16,
0.190809912898504));
#95421=DIRECTION('ref_axis',(-0.177651170119724,-0.364923706798204,0.913931479910694));
#95422=DIRECTION('center_axis',(0.981627005099017,-8.06332694004955E-18,
0.190809912898503));
#95423=DIRECTION('ref_axis',(-0.178230399159777,-0.35708195021081,0.916911340124546));
#95424=DIRECTION('center_axis',(0.,1.,0.));
#95425=DIRECTION('ref_axis',(1.,0.,0.));
#95426=DIRECTION('',(-0.190809912898503,0.,0.981627005099017));
#95427=DIRECTION('center_axis',(0.,1.,0.));
#95428=DIRECTION('ref_axis',(-0.566947419293269,0.,0.823753982543758));
#95429=DIRECTION('center_axis',(0.,1.,0.));
#95430=DIRECTION('ref_axis',(-0.559227720460236,0.,0.829014087135344));
#95431=DIRECTION('center_axis',(-0.981627005099017,0.,-0.190809912898503));
#95432=DIRECTION('ref_axis',(-0.190809912898503,0.,0.981627005099017));
#95433=DIRECTION('center_axis',(-0.981627005099017,-8.64893398502948E-18,
-0.190809912898503));
#95434=DIRECTION('ref_axis',(-0.174485168153884,-0.404710226387007,0.897643893062326));
#95435=DIRECTION('center_axis',(-0.981627005099017,1.65434297745177E-16,
-0.190809912898504));
#95436=DIRECTION('ref_axis',(-0.175228886041806,-0.395786216552817,0.901469970816197));
#95437=DIRECTION('center_axis',(0.,-1.,0.));
#95438=DIRECTION('ref_axis',(0.,0.,-1.));
#95439=DIRECTION('',(-0.190809912898503,0.,0.981627005099017));
#95440=DIRECTION('center_axis',(0.,-1.,0.));
#95441=DIRECTION('ref_axis',(-0.531976328976784,0.,0.846759225168752));
#95442=DIRECTION('',(-0.190809912898503,0.,0.981627005099017));
#95443=DIRECTION('center_axis',(0.,-1.,0.));
#95444=DIRECTION('ref_axis',(-0.525093536093152,0.,0.8510445219571));
#95445=DIRECTION('center_axis',(0.981627005099017,0.,0.190809912898503));
#95446=DIRECTION('ref_axis',(0.,-1.,0.));
#95447=DIRECTION('',(-0.190809912898503,0.,0.981627005099017));
#95448=DIRECTION('center_axis',(0.981627005099017,-1.68427353353279E-16,
0.190809912898504));
#95449=DIRECTION('ref_axis',(-0.182255177482091,-0.296070177213685,0.937616926279399));
#95450=DIRECTION('center_axis',(0.981627005099017,2.41899808201487E-17,
0.190809912898503));
#95451=DIRECTION('ref_axis',(-0.182627045040003,-0.289707997340905,0.939530009471054));
#95452=DIRECTION('center_axis',(0.,1.,0.));
#95453=DIRECTION('ref_axis',(1.,0.,0.));
#95454=DIRECTION('',(-0.190809912898493,0.,0.981627005099019));
#95455=DIRECTION('center_axis',(0.,1.,0.));
#95456=DIRECTION('ref_axis',(-0.559041153008243,0.,0.829139909329671));
#95457=DIRECTION('center_axis',(0.,1.,0.));
#95458=DIRECTION('ref_axis',(-0.551793165097242,0.,0.833980996757101));
#95459=DIRECTION('center_axis',(-0.981627005099017,0.,-0.190809912898503));
#95460=DIRECTION('ref_axis',(-0.190809912898503,0.,0.981627005099017));
#95461=DIRECTION('center_axis',(-0.981627005099017,2.68116953535914E-16,
-0.190809912898504));
#95462=DIRECTION('ref_axis',(-0.179789130769917,-0.33493260114791,0.924930279072587));
#95463=DIRECTION('center_axis',(-0.981627005099017,7.44454339853295E-17,
-0.190809912898503));
#95464=DIRECTION('ref_axis',(-0.180283848265106,-0.327547213698889,0.927475367248542));
#95465=DIRECTION('center_axis',(0.,-1.,0.));
#95466=DIRECTION('ref_axis',(0.,0.,-1.));
#95467=DIRECTION('',(-0.190809912898517,0.,0.981627005099014));
#95468=DIRECTION('center_axis',(0.,-1.,0.));
#95469=DIRECTION('ref_axis',(-0.525640886100688,0.,0.85070656448583));
#95470=DIRECTION('',(-0.190809912898503,0.,0.981627005099017));
#95471=DIRECTION('center_axis',(0.,-1.,0.));
#95472=DIRECTION('ref_axis',(-0.51913056933854,0.,0.854694946737281));
#95473=DIRECTION('center_axis',(0.981627005099017,0.,0.190809912898503));
#95474=DIRECTION('ref_axis',(0.,-1.,0.));
#95475=DIRECTION('',(-0.190809912898503,0.,0.981627005099017));
#95476=DIRECTION('center_axis',(0.981627005099017,-1.43163250350287E-16,
0.190809912898504));
#95477=DIRECTION('ref_axis',(-0.185819133754778,-0.227216647629105,0.955951800338707));
#95478=DIRECTION('center_axis',(0.981627005099017,-1.12886577160694E-16,
0.190809912898504));
#95479=DIRECTION('ref_axis',(-0.186034045655795,-0.222334044470899,0.957057420704813));
#95480=DIRECTION('center_axis',(0.,1.,0.));
#95481=DIRECTION('ref_axis',(1.,0.,0.));
#95482=DIRECTION('',(-0.190809912898503,0.,0.981627005099017));
#95483=DIRECTION('center_axis',(0.,1.,0.));
#95484=DIRECTION('ref_axis',(-0.553126915130717,0.,0.833097002610126));
#95485=DIRECTION('center_axis',(0.,1.,0.));
#95486=DIRECTION('ref_axis',(-0.546219243843012,0.,0.837642249206407));
#95487=DIRECTION('center_axis',(-0.981627005099017,0.,-0.190809912898503));
#95488=DIRECTION('ref_axis',(-0.190809912898503,0.,0.981627005099017));
#95489=DIRECTION('center_axis',(-0.981627005099017,1.47031877745501E-16,
-0.190809912898504));
#95490=DIRECTION('ref_axis',(-0.183980026099205,-0.265154975908797,0.946490458878134));
#95491=DIRECTION('center_axis',(-0.981627005099017,-8.27171488725884E-18,
-0.190809912898503));
#95492=DIRECTION('ref_axis',(-0.184283187692203,-0.259308210845006,0.948050082285932));
#95493=DIRECTION('center_axis',(0.,-1.,0.));
#95494=DIRECTION('ref_axis',(0.,0.,-1.));
#95495=DIRECTION('',(-0.190809912898503,0.,0.981627005099017));
#95496=DIRECTION('center_axis',(0.,-1.,0.));
#95497=DIRECTION('ref_axis',(-0.521013332380248,0.,0.853548538445254));
#95498=DIRECTION('',(-0.190809912898503,0.,0.981627005099017));
#95499=DIRECTION('center_axis',(0.,-1.,0.));
#95500=DIRECTION('ref_axis',(-0.514766609928991,0.,0.857330354823748));
#95501=DIRECTION('center_axis',(0.981627005099017,0.,0.190809912898503));
#95502=DIRECTION('ref_axis',(0.,-1.,0.));
#95503=DIRECTION('',(-0.190809912898517,0.,0.981627005099014));
#95504=DIRECTION('center_axis',(0.981627005099017,-7.57923090089756E-17,
0.190809912898504));
#95505=DIRECTION('ref_axis',(-0.188402071368518,-0.158363118044504,0.969239796101705));
#95506=DIRECTION('center_axis',(0.981627005099017,-4.03166347002478E-18,
0.190809912898503));
#95507=DIRECTION('ref_axis',(-0.18850506856238,-0.154960091600897,0.969769668084816));
#95508=DIRECTION('center_axis',(0.,1.,0.));
#95509=DIRECTION('ref_axis',(1.,0.,0.));
#95510=DIRECTION('',(-0.190809912898503,0.,0.981627005099017));
#95511=DIRECTION('center_axis',(0.,1.,0.));
#95512=DIRECTION('ref_axis',(-0.548948616419421,0.,0.83585609798051));
#95513=DIRECTION('center_axis',(0.,1.,0.));
#95514=DIRECTION('ref_axis',(-0.542274986861829,0.,0.840201070353998));
#95515=DIRECTION('center_axis',(-0.981627005099017,0.,-0.190809912898503));
#95516=DIRECTION('ref_axis',(-0.190809912898503,0.,0.981627005099017));
#95517=DIRECTION('center_axis',(-0.981627005099017,9.08138068428095E-17,
-0.190809912898504));
#95518=DIRECTION('ref_axis',(-0.187132651579236,-0.195377350669603,0.962709230016131));
#95519=DIRECTION('center_axis',(-0.981627005099017,6.20378616544413E-17,
-0.190809912898504));
#95520=DIRECTION('ref_axis',(-0.187294539337449,-0.191069207991,0.9635420661767));
#95521=DIRECTION('center_axis',(0.,-1.,0.));
#95522=DIRECTION('ref_axis',(0.,0.,-1.));
#95523=DIRECTION('',(-0.190809912898503,0.,0.981627005099017));
#95524=DIRECTION('center_axis',(0.,-1.,0.));
#95525=DIRECTION('ref_axis',(-0.517900254205494,0.,0.855441012983294));
#95526=DIRECTION('',(-0.190809912898503,0.,0.981627005099017));
#95527=DIRECTION('center_axis',(0.,-1.,0.));
#95528=DIRECTION('ref_axis',(-0.511826882023824,0.,0.859088611749551));
#95529=DIRECTION('center_axis',(0.981627005099017,0.,0.190809912898503));
#95530=DIRECTION('ref_axis',(0.,-1.,0.));
#95531=DIRECTION('',(-0.190809912898503,0.,0.981627005099017));
#95532=DIRECTION('center_axis',(0.981627005099017,4.21068383383198E-18,
0.190809912898503));
#95533=DIRECTION('ref_axis',(-0.190043994376944,-0.0895095884599529,0.977686715556157));
#95534=DIRECTION('center_axis',(0.981627005099017,-4.23324664352601E-17,
0.190809912898504));
#95535=DIRECTION('ref_axis',(-0.190076620792719,-0.0875861387309634,0.977854563076852));
#95536=DIRECTION('center_axis',(0.,1.,0.));
#95537=DIRECTION('ref_axis',(1.,0.,0.));
#95538=DIRECTION('',(-0.190809912898503,0.,0.981627005099017));
#95539=DIRECTION('center_axis',(0.,1.,0.));
#95540=DIRECTION('ref_axis',(-0.546338397386211,0.,0.837564538135102));
#95541=DIRECTION('center_axis',(0.,1.,0.));
#95542=DIRECTION('ref_axis',(-0.539808318337868,0.,0.841787965851997));
#95543=DIRECTION('center_axis',(-0.981627005099017,0.,-0.190809912898503));
#95544=DIRECTION('ref_axis',(-0.190809912898503,0.,0.981627005099017));
#95545=DIRECTION('center_axis',(-0.981627005099017,-7.35159388727506E-17,
-0.190809912898503));
#95546=DIRECTION('ref_axis',(-0.18929888904543,-0.125599725430494,0.973853500059403));
#95547=DIRECTION('center_axis',(-0.981627005099017,4.13585744362942E-18,
-0.190809912898503));
#95548=DIRECTION('ref_axis',(-0.189365043089146,-0.122830205137097,0.974193831412325));
#95549=DIRECTION('center_axis',(0.,-1.,0.));
#95550=DIRECTION('ref_axis',(0.,0.,-1.));
#95551=DIRECTION('',(-0.190809912898503,0.,0.981627005099017));
#95552=DIRECTION('center_axis',(0.,-1.,0.));
#95553=DIRECTION('ref_axis',(-0.51617952877047,0.,0.85648041079659));
#95554=DIRECTION('',(-0.190809912898503,0.,0.981627005099017));
#95555=DIRECTION('center_axis',(0.,-1.,0.));
#95556=DIRECTION('ref_axis',(-0.510200612741185,0.,0.860055425399154));
#95557=DIRECTION('center_axis',(0.981627005099017,0.,0.190809912898503));
#95558=DIRECTION('ref_axis',(0.,-1.,0.));
#95559=DIRECTION('',(-0.190809912898503,0.,0.981627005099017));
#95560=DIRECTION('center_axis',(0.981627005099017,-1.0000374105351E-17,
0.190809912898504));
#95561=DIRECTION('ref_axis',(-0.190769201858593,-0.0206560588753701,0.98141756600031));
#95562=DIRECTION('center_axis',(0.981627005099017,1.10870745425681E-17,
0.190809912898503));
#95563=DIRECTION('ref_axis',(-0.190770932895652,-0.020212185860989,0.981426471369528));
#95564=DIRECTION('center_axis',(0.,1.,0.));
#95565=DIRECTION('ref_axis',(1.,0.,0.));
#95566=DIRECTION('',(-0.190809912898503,0.,0.981627005099017));
#95567=DIRECTION('center_axis',(0.,1.,0.));
#95568=DIRECTION('ref_axis',(-0.545196651612185,0.,0.838308183826725));
#95569=DIRECTION('center_axis',(0.,1.,0.));
#95570=DIRECTION('ref_axis',(-0.538728725034813,0.,0.842479294002152));
#95571=DIRECTION('center_axis',(-0.981627005099017,0.,-0.190809912898503));
#95572=DIRECTION('ref_axis',(-0.190809912898503,0.,0.981627005099017));
#95573=DIRECTION('center_axis',(-0.981627005099017,3.89202029326326E-17,
-0.190809912898504));
#95574=DIRECTION('ref_axis',(-0.190512388898313,-0.0558221001913178,0.980096384447207));
#95575=DIRECTION('center_axis',(-0.981627005099017,2.68830733835912E-17,
-0.190809912898504));
#95576=DIRECTION('ref_axis',(-0.190525374954579,-0.0545912022831507,0.980163191581737));
#95577=DIRECTION('center_axis',(0.,-1.,0.));
#95578=DIRECTION('ref_axis',(0.,0.,-1.));
#95579=DIRECTION('',(-0.190809912898503,0.,0.981627005099017));
#95580=DIRECTION('center_axis',(0.,-1.,0.));
#95581=DIRECTION('ref_axis',(0.254065172927508,0.,0.967187100774879));
#95582=DIRECTION('',(-0.190809912898503,0.,0.981627005099017));
#95583=DIRECTION('center_axis',(0.,-1.,0.));
#95584=DIRECTION('ref_axis',(0.245183383065688,0.,0.969476718992501));
#95585=DIRECTION('center_axis',(0.981627005099017,0.,0.190809912898503));
#95586=DIRECTION('ref_axis',(0.,-1.,0.));
#95587=DIRECTION('',(-0.190809912898503,0.,0.981627005099017));
#95588=DIRECTION('center_axis',(0.981627005099017,-9.15013555197185E-18,
0.190809912898504));
#95589=DIRECTION('ref_axis',(-0.190765678400248,-0.0215312831584694,0.981399439468988));
#95590=DIRECTION('center_axis',(0.981627005099017,-8.18343260114431E-18,
0.190809912898504));
#95591=DIRECTION('ref_axis',(-0.190767714546191,-0.02102995121624,0.981409914479503));
#95592=DIRECTION('center_axis',(0.,1.,0.));
#95593=DIRECTION('ref_axis',(1.,0.,0.));
#95594=DIRECTION('',(-0.19080991289849,0.,0.98162700509902));
#95595=DIRECTION('center_axis',(0.,1.,0.));
#95596=DIRECTION('ref_axis',(0.218941789395062,0.,0.975737922219121));
#95597=DIRECTION('center_axis',(0.,1.,0.));
#95598=DIRECTION('ref_axis',(0.210813468337157,0.,0.977526307353239));
#95599=DIRECTION('center_axis',(-0.981627005099017,0.,-0.190809912898503));
#95600=DIRECTION('ref_axis',(-0.190809912898503,0.,0.981627005099017));
#95601=DIRECTION('center_axis',(-0.981627005099017,-1.54978312110657E-17,
-0.190809912898503));
#95602=DIRECTION('ref_axis',(-0.190505263436507,-0.0564860647764627,0.980059727306992));
#95603=DIRECTION('center_axis',(-0.981627005099017,4.86497553780052E-17,
-0.190809912898504));
#95604=DIRECTION('ref_axis',(-0.190518864735177,-0.0552117215270287,0.980129699573501));
#95605=DIRECTION('center_axis',(0.,-1.,0.));
#95606=DIRECTION('ref_axis',(0.,0.,-1.));
#95607=DIRECTION('',(-0.190809912898503,0.,0.981627005099017));
#95608=DIRECTION('center_axis',(0.,-1.,0.));
#95609=DIRECTION('ref_axis',(0.256627372086269,0.,0.966510419962504));
#95610=DIRECTION('',(-0.190809912898503,0.,0.981627005099017));
#95611=DIRECTION('center_axis',(0.,-1.,0.));
#95612=DIRECTION('ref_axis',(0.247596031419092,0.,0.968863357355162));
#95613=DIRECTION('center_axis',(0.981627005099017,0.,0.190809912898503));
#95614=DIRECTION('ref_axis',(0.,-1.,0.));
#95615=DIRECTION('',(-0.190809912898503,0.,0.981627005099017));
#95616=DIRECTION('center_axis',(0.981627005099017,1.37252033279578E-17,
0.190809912898503));
#95617=DIRECTION('ref_axis',(-0.189977568186684,-0.0933022270200431,0.977344984137625));
#95618=DIRECTION('center_axis',(0.981627005099017,2.18224869363849E-17,
0.190809912898503));
#95619=DIRECTION('ref_axis',(-0.190015957421534,-0.0911297886037193,0.977542478644391));
#95620=DIRECTION('center_axis',(0.,1.,0.));
#95621=DIRECTION('ref_axis',(1.,0.,0.));
#95622=DIRECTION('',(-0.190809912898503,0.,0.981627005099017));
#95623=DIRECTION('center_axis',(0.,1.,0.));
#95624=DIRECTION('ref_axis',(0.220379730294923,0.,0.975414155359218));
#95625=DIRECTION('center_axis',(0.,1.,0.));
#95626=DIRECTION('ref_axis',(0.212168144710188,0.,0.977233175025407));
#95627=DIRECTION('center_axis',(-0.981627005099017,0.,-0.190809912898503));
#95628=DIRECTION('ref_axis',(-0.190809912898503,0.,0.981627005099017));
#95629=DIRECTION('center_axis',(-0.981627005099017,-4.42795177459019E-17,
-0.190809912898503));
#95630=DIRECTION('ref_axis',(-0.189262582348626,-0.127093645746998,0.973666719228641));
#95631=DIRECTION('center_axis',(-0.981627005099017,2.53824810667853E-17,
-0.190809912898503));
#95632=DIRECTION('ref_axis',(-0.189331880816577,-0.124226373435802,0.974023227161163));
#95633=DIRECTION('center_axis',(0.,-1.,0.));
#95634=DIRECTION('ref_axis',(0.,0.,-1.));
#95635=DIRECTION('',(-0.190809912898493,0.,0.981627005099019));
#95636=DIRECTION('center_axis',(0.,-1.,0.));
#95637=DIRECTION('ref_axis',(0.261269729827485,0.,0.965265832957882));
#95638=DIRECTION('',(-0.190809912898503,0.,0.981627005099017));
#95639=DIRECTION('center_axis',(0.,-1.,0.));
#95640=DIRECTION('ref_axis',(0.251963327850453,0.,0.967736783127791));
#95641=DIRECTION('center_axis',(0.981627005099017,0.,0.190809912898503));
#95642=DIRECTION('ref_axis',(0.,-1.,0.));
#95643=DIRECTION('',(-0.190809912898503,0.,0.981627005099017));
#95644=DIRECTION('center_axis',(0.981627005099017,-9.60764232957044E-17,
0.190809912898504));
#95645=DIRECTION('ref_axis',(-0.188192253350186,-0.165073170881603,0.968160381359448));
#95646=DIRECTION('center_axis',(0.981627005099017,-6.11029634218775E-17,
0.190809912898504));
#95647=DIRECTION('ref_axis',(-0.188313531612905,-0.1612296259912,0.968784300819441));
#95648=DIRECTION('center_axis',(0.,1.,0.));
#95649=DIRECTION('ref_axis',(1.,0.,0.));
#95650=DIRECTION('',(-0.190809912898503,0.,0.981627005099017));
#95651=DIRECTION('center_axis',(0.,1.,0.));
#95652=DIRECTION('ref_axis',(0.223670618325374,0.,0.974664790837314));
#95653=DIRECTION('center_axis',(0.,1.,0.));
#95654=DIRECTION('ref_axis',(0.215266419163362,0.,0.976555358789548));
#95655=DIRECTION('center_axis',(-0.981627005099017,0.,-0.190809912898503));
#95656=DIRECTION('ref_axis',(-0.190809912898503,0.,0.981627005099017));
#95657=DIRECTION('center_axis',(-0.981627005099017,2.21397588729509E-17,
-0.190809912898503));
#95658=DIRECTION('ref_axis',(-0.187043768767229,-0.197701226717603,0.962251969870525));
#95659=DIRECTION('center_axis',(-0.981627005099017,1.35373232356188E-16,
-0.190809912898504));
#95660=DIRECTION('ref_axis',(-0.187213397266324,-0.193241025344597,0.963124628491957));
#95661=DIRECTION('center_axis',(0.,-1.,0.));
#95662=DIRECTION('ref_axis',(0.,0.,-1.));
#95663=DIRECTION('',(-0.190809912898503,0.,0.981627005099017));
#95664=DIRECTION('center_axis',(0.,-1.,0.));
#95665=DIRECTION('ref_axis',(0.268187136288328,0.,0.963366835597669));
#95666=DIRECTION('',(-0.190809912898503,0.,0.981627005099017));
#95667=DIRECTION('center_axis',(0.,-1.,0.));
#95668=DIRECTION('ref_axis',(0.25846100454496,0.,0.966021691852523));
#95669=DIRECTION('center_axis',(0.981627005099017,0.,0.190809912898503));
#95670=DIRECTION('ref_axis',(0.,-1.,0.));
#95671=DIRECTION('',(-0.190809912898503,0.,0.981627005099017));
#95672=DIRECTION('center_axis',(0.981627005099017,-2.19603253247325E-16,
0.190809912898504));
#95673=DIRECTION('ref_axis',(-0.185380925329951,-0.236844114743192,0.953697424676886));
#95674=DIRECTION('center_axis',(0.981627005099017,3.49159790982158E-17,
0.190809912898503));
#95675=DIRECTION('ref_axis',(-0.185634283617771,-0.231329463378695,0.955000833569606));
#95676=DIRECTION('center_axis',(0.,1.,0.));
#95677=DIRECTION('ref_axis',(1.,0.,0.));
#95678=DIRECTION('',(-0.190809912898503,0.,0.981627005099017));
#95679=DIRECTION('center_axis',(0.,1.,0.));
#95680=DIRECTION('ref_axis',(0.228948751797627,0.,0.973438477280567));
#95681=DIRECTION('center_axis',(0.,1.,0.));
#95682=DIRECTION('ref_axis',(0.220229621907956,0.,0.975448057886364));
#95683=DIRECTION('center_axis',(-0.981627005099017,0.,-0.190809912898503));
#95684=DIRECTION('ref_axis',(-0.190809912898503,0.,0.981627005099017));
#95685=DIRECTION('center_axis',(-0.981627005099017,2.21397588729509E-16,
-0.190809912898504));
#95686=DIRECTION('ref_axis',(-0.183813477387126,-0.268308807688208,0.945633644308294));
#95687=DIRECTION('center_axis',(-0.981627005099017,1.18451578311665E-16,
-0.190809912898504));
#95688=DIRECTION('ref_axis',(-0.184131265371603,-0.262255677253399,0.947268513601615));
#95689=DIRECTION('center_axis',(0.,-1.,0.));
#95690=DIRECTION('ref_axis',(0.,0.,-1.));
#95691=DIRECTION('',(-0.190809912898503,0.,0.981627005099017));
#95692=DIRECTION('center_axis',(0.,-1.,0.));
#95693=DIRECTION('ref_axis',(0.277690140407669,0.,0.960670695878858));
#95694=DIRECTION('',(-0.190809912898503,0.,0.981627005099017));
#95695=DIRECTION('center_axis',(0.,-1.,0.));
#95696=DIRECTION('ref_axis',(0.26736789956837,0.,0.963594523791204));
#95697=DIRECTION('center_axis',(0.981627005099017,0.,0.190809912898503));
#95698=DIRECTION('ref_axis',(0.,-1.,0.));
#95699=DIRECTION('',(-0.190809912898503,0.,0.981627005099017));
#95700=DIRECTION('center_axis',(0.981627005099017,9.15013555197185E-18,
0.190809912898503));
#95701=DIRECTION('ref_axis',(-0.181495912294555,-0.308615058604696,0.933710865002002));
#95702=DIRECTION('center_axis',(0.981627005099017,-6.11029634218775E-17,
0.190809912898504));
#95703=DIRECTION('ref_axis',(-0.181935063338814,-0.301429300766198,0.935970089996204));
#95704=DIRECTION('center_axis',(0.,1.,0.));
#95705=DIRECTION('ref_axis',(1.,0.,0.));
#95706=DIRECTION('',(-0.190809912898503,0.,0.981627005099017));
#95707=DIRECTION('center_axis',(0.,1.,0.));
#95708=DIRECTION('ref_axis',(0.236441581346834,0.,0.97164570632006));
#95709=DIRECTION('center_axis',(0.,1.,0.));
#95710=DIRECTION('ref_axis',(0.227262546686523,0.,0.97383352523599));
#95711=DIRECTION('center_axis',(-0.981627005099017,0.,-0.190809912898503));
#95712=DIRECTION('ref_axis',(-0.190809912898503,0.,0.981627005099017));
#95713=DIRECTION('center_axis',(-0.981627005099017,1.85973974532787E-16,
-0.190809912898504));
#95714=DIRECTION('ref_axis',(-0.179517113893821,-0.338916388658794,0.923530880543642));
#95715=DIRECTION('center_axis',(-0.981627005099017,-1.52294886400712E-16,
-0.190809912898503));
#95716=DIRECTION('ref_axis',(-0.180036000309911,-0.331270329162208,0.926200306418203));
#95717=DIRECTION('center_axis',(0.,-1.,0.));
#95718=DIRECTION('ref_axis',(0.,0.,-1.));
#95719=DIRECTION('',(-0.190809912898503,0.,0.981627005099017));
#95720=DIRECTION('center_axis',(0.,-1.,0.));
#95721=DIRECTION('ref_axis',(0.204850037849769,0.,0.978793370427563));
#95722=DIRECTION('',(-0.190809912898503,0.,0.981627005099017));
#95723=DIRECTION('center_axis',(0.,-1.,0.));
#95724=DIRECTION('ref_axis',(0.196208098272871,0.,0.980562278579053));
#95725=DIRECTION('center_axis',(0.981627005099017,0.,0.190809912898503));
#95726=DIRECTION('ref_axis',(0.,-1.,0.));
#95727=DIRECTION('',(-0.190809912898503,0.,0.981627005099017));
#95728=DIRECTION('center_axis',(0.981627005099017,-2.40821729421067E-16,
0.190809912898504));
#95729=DIRECTION('ref_axis',(-0.182068555054379,-0.299207288953005,0.936656841910528));
#95730=DIRECTION('center_axis',(0.981627005099017,-2.13919040821322E-16,
0.190809912898504));
#95731=DIRECTION('ref_axis',(-0.182456464621202,-0.292645194278013,0.938652453671707));
#95732=DIRECTION('center_axis',(0.,1.,0.));
#95733=DIRECTION('ref_axis',(1.,0.,0.));
#95734=DIRECTION('',(-0.190809912898503,0.,0.981627005099017));
#95735=DIRECTION('center_axis',(0.,1.,0.));
#95736=DIRECTION('ref_axis',(0.164995567902462,0.,0.986294308293698));
#95737=DIRECTION('center_axis',(0.,1.,0.));
#95738=DIRECTION('ref_axis',(0.15741294900624,0.,0.987532867040464));
#95739=DIRECTION('center_axis',(-0.981627005099017,0.,-0.190809912898503));
#95740=DIRECTION('ref_axis',(-0.190809912898503,0.,0.981627005099017));
#95741=DIRECTION('center_axis',(-0.981627005099017,2.93287925373025E-16,
-0.190809912898504));
#95742=DIRECTION('ref_axis',(-0.180142425085377,-0.329677418408388,0.926747811692016));
#95743=DIRECTION('center_axis',(-0.981627005099017,-1.60501554366299E-17,
-0.190809912898503));
#95744=DIRECTION('ref_axis',(-0.180606576747544,-0.322627033310802,0.929135653073653));
#95745=DIRECTION('center_axis',(0.,-1.,0.));
#95746=DIRECTION('ref_axis',(0.,0.,-1.));
#95747=DIRECTION('',(-0.190809912898503,0.,0.981627005099017));
#95748=DIRECTION('center_axis',(0.,-1.,0.));
#95749=DIRECTION('ref_axis',(0.133141028786344,0.,0.991097102434324));
#95750=DIRECTION('',(-0.190809912898503,0.,0.981627005099017));
#95751=DIRECTION('center_axis',(0.,-1.,0.));
#95752=DIRECTION('ref_axis',(0.126120325699543,0.,0.992014951220717));
#95753=DIRECTION('center_axis',(0.981627005099017,0.,0.190809912898503));
#95754=DIRECTION('ref_axis',(0.,-1.,0.));
#95755=DIRECTION('',(-0.190809912898514,0.,0.981627005099015));
#95756=DIRECTION('center_axis',(0.981627005099017,-1.63768969384934E-16,
0.190809912898504));
#95757=DIRECTION('ref_axis',(-0.182497177694581,-0.291947095881692,0.938861903231651));
#95758=DIRECTION('center_axis',(0.981627005099017,-1.25592652705723E-16,
0.190809912898504));
#95759=DIRECTION('ref_axis',(-0.182848726580948,-0.285841626719414,0.940670456441641));
#95760=DIRECTION('center_axis',(0.,1.,0.));
#95761=DIRECTION('ref_axis',(1.,0.,0.));
#95762=DIRECTION('',(-0.190809912898503,0.,0.981627005099017));
#95763=DIRECTION('center_axis',(0.,1.,0.));
#95764=DIRECTION('ref_axis',(0.0946046538042337,0.,0.995514921775953));
#95765=DIRECTION('center_axis',(0.,1.,0.));
#95766=DIRECTION('ref_axis',(0.0885667405097263,0.,0.996070244749577));
#95767=DIRECTION('center_axis',(-0.981627005099017,0.,-0.190809912898503));
#95768=DIRECTION('ref_axis',(-0.190809912898503,0.,0.981627005099017));
#95769=DIRECTION('center_axis',(-0.981627005099017,1.3640552305848E-16,
-0.190809912898504));
#95770=DIRECTION('ref_axis',(-0.180608176174812,-0.3226024401748,0.929143881372564));
#95771=DIRECTION('center_axis',(-0.981627005099017,-1.53963266976712E-17,
-0.190809912898503));
#95772=DIRECTION('ref_axis',(-0.181033462471816,-0.315987346735709,0.931331778781543));
#95773=DIRECTION('center_axis',(0.,-1.,0.));
#95774=DIRECTION('ref_axis',(0.,0.,-1.));
#95775=DIRECTION('',(-0.190809912898503,0.,0.981627005099017));
#95776=DIRECTION('center_axis',(0.,-1.,0.));
#95777=DIRECTION('ref_axis',(0.0624727692896659,0.,0.998046668797246));
#95778=DIRECTION('',(-0.190809912898503,-1.10039580182E-14,0.981627005099017));
#95779=DIRECTION('center_axis',(0.,-1.,0.));
#95780=DIRECTION('ref_axis',(0.0570228775206296,0.,0.998372871946783));
#95781=DIRECTION('center_axis',(0.981627005099017,0.,0.190809912898503));
#95782=DIRECTION('ref_axis',(0.,-1.,0.));
#95783=DIRECTION('',(-0.190809912898503,0.,0.981627005099017));
#95784=DIRECTION('center_axis',(0.981627005099017,1.57664003463228E-17,
0.190809912898503));
#95785=DIRECTION('ref_axis',(-0.182813841947861,-0.286453825561204,0.94049099145798));
#95786=DIRECTION('center_axis',(0.981627005099017,-4.54116221843461E-17,
0.190809912898503));
#95787=DIRECTION('ref_axis',(-0.183139631044442,-0.280679847653606,0.942167022699295));
#95788=DIRECTION('center_axis',(0.,1.,0.));
#95789=DIRECTION('ref_axis',(1.,0.,0.));
#95790=DIRECTION('',(-0.190809912898503,0.,0.981627005099017));
#95791=DIRECTION('center_axis',(0.,1.,0.));
#95792=DIRECTION('ref_axis',(0.0251959490043322,0.,0.99968253168382));
#95793=DIRECTION('center_axis',(0.,1.,0.));
#95794=DIRECTION('ref_axis',(0.0206576469622491,0.,0.999786608042928));
#95795=DIRECTION('center_axis',(-0.981627005099017,0.,-0.190809912898503));
#95796=DIRECTION('ref_axis',(-0.190809912898503,0.,0.981627005099017));
#95797=DIRECTION('center_axis',(-0.981627005099017,1.31993506757577E-16,
-0.190809912898504));
#95798=DIRECTION('ref_axis',(-0.180947151082311,-0.317342291967003,0.930887747391878));
#95799=DIRECTION('center_axis',(-0.981627005099017,3.72948009280241E-17,
-0.190809912898503));
#95800=DIRECTION('ref_axis',(-0.18134517801343,-0.311039307001288,0.932935408220438));
#95801=DIRECTION('center_axis',(0.,-1.,0.));
#95802=DIRECTION('ref_axis',(0.,0.,-1.));
#95803=DIRECTION('',(-0.190809912898503,0.,0.981627005099017));
#95804=DIRECTION('center_axis',(0.,-1.,0.));
#95805=DIRECTION('ref_axis',(-0.00721925021943933,0.,0.999973940873596));
#95806=DIRECTION('',(-0.190809912898503,0.,0.981627005099017));
#95807=DIRECTION('center_axis',(0.,-1.,0.));
#95808=DIRECTION('ref_axis',(-0.0111429250982784,0.,0.999937915682896));
#95809=DIRECTION('center_axis',(0.981627005099017,0.,0.190809912898503));
#95810=DIRECTION('ref_axis',(0.,-1.,0.));
#95811=DIRECTION('',(-0.190809912898503,0.,0.981627005099017));
#95812=DIRECTION('center_axis',(0.981627005099017,-7.66548341238665E-18,
0.190809912898503));
#95813=DIRECTION('ref_axis',(-0.183039366361104,-0.28247051610541,0.941651208194026));
#95814=DIRECTION('center_axis',(0.981627005099017,-1.2525082703208E-16,
0.190809912898504));
#95815=DIRECTION('ref_axis',(-0.183347383985879,-0.276929479719012,0.943235813594931));
#95816=DIRECTION('center_axis',(0.,1.,0.));
#95817=DIRECTION('ref_axis',(1.,0.,0.));
#95818=DIRECTION('',(-0.190809912898503,0.,0.981627005099017));
#95819=DIRECTION('center_axis',(0.,1.,0.));
#95820=DIRECTION('ref_axis',(-0.0432822030002458,0.,0.999062886360736));
#95821=DIRECTION('center_axis',(0.,1.,0.));
#95822=DIRECTION('ref_axis',(-0.0463615215085348,0.,0.998924726555216));
#95823=DIRECTION('center_axis',(-0.981627005099017,0.,-0.190809912898503));
#95824=DIRECTION('ref_axis',(-0.190809912898503,0.,0.981627005099017));
#95825=DIRECTION('center_axis',(-0.981627005099017,1.51705767418914E-16,
-0.190809912898504));
#95826=DIRECTION('ref_axis',(-0.181180621351987,-0.313662196346486,0.932088841811555));
#95827=DIRECTION('center_axis',(-0.981627005099017,-1.23990865619567E-16,
-0.190809912898503));
#95828=DIRECTION('ref_axis',(-0.181560378435138,-0.307571801532109,0.93404251288942));
#95829=DIRECTION('center_axis',(0.,-1.,0.));
#95830=DIRECTION('ref_axis',(0.,0.,-1.));
#95831=DIRECTION('',(-0.190809912898503,0.,0.981627005099017));
#95832=DIRECTION('center_axis',(0.,-1.,0.));
#95833=DIRECTION('ref_axis',(-0.0759798223257543,0.,0.997109355386533));
#95834=DIRECTION('',(-0.190809912898503,0.,0.981627005099017));
#95835=DIRECTION('center_axis',(0.,-1.,0.));
#95836=DIRECTION('ref_axis',(-0.0784179965065422,0.,0.996920567459564));
#95837=DIRECTION('center_axis',(0.981627005099017,0.,0.190809912898503));
#95838=DIRECTION('ref_axis',(0.,-1.,0.));
#95839=DIRECTION('',(-0.190809912898503,0.,0.981627005099017));
#95840=DIRECTION('center_axis',(0.981627005099017,-1.88066225336819E-16,
0.190809912898504));
#95841=DIRECTION('ref_axis',(-0.183187172191114,-0.27982644106311,0.942411599475822));
#95842=DIRECTION('center_axis',(0.981627005099017,-1.51948603552176E-16,
0.190809912898504));
#95843=DIRECTION('ref_axis',(-0.183483802676835,-0.274436617915494,0.943937623417116));
#95844=DIRECTION('center_axis',(0.,1.,0.));
#95845=DIRECTION('ref_axis',(1.,0.,0.));
#95846=DIRECTION('',(-0.190809912898503,0.,0.981627005099017));
#95847=DIRECTION('center_axis',(0.,1.,0.));
#95848=DIRECTION('ref_axis',(-0.110864698133628,0.,0.993835508878476));
#95849=DIRECTION('center_axis',(0.,1.,0.));
#95850=DIRECTION('ref_axis',(-0.112522750034819,0.,0.993649148706223));
#95851=DIRECTION('center_axis',(-0.981627005099017,0.,-0.190809912898503));
#95852=DIRECTION('ref_axis',(-0.190809912898503,0.,0.981627005099017));
#95853=DIRECTION('center_axis',(-0.981627005099017,2.39255602982779E-16,
-0.190809912898504));
#95854=DIRECTION('ref_axis',(-0.18132202997097,-0.311409746153812,0.932816322459907));
#95855=DIRECTION('center_axis',(-0.981627005099017,4.31589770358279E-17,
-0.190809912898503));
#95856=DIRECTION('ref_axis',(-0.181690922255445,-0.305447149913308,0.934714099273036));
#95857=DIRECTION('center_axis',(0.,-1.,0.));
#95858=DIRECTION('ref_axis',(0.,0.,-1.));
#95859=DIRECTION('',(-0.190809912898503,0.,0.981627005099017));
#95860=DIRECTION('center_axis',(0.,-1.,0.));
#95861=DIRECTION('ref_axis',(-0.143837786703644,0.,0.989601278857398));
#95862=DIRECTION('',(-0.190809912898503,0.,0.981627005099017));
#95863=DIRECTION('center_axis',(0.,-1.,0.));
#95864=DIRECTION('ref_axis',(-0.1448287547547,0.,0.989456735686914));
#95865=DIRECTION('center_axis',(0.981627005099017,0.,0.190809912898503));
#95866=DIRECTION('ref_axis',(0.,-1.,0.));
#95867=DIRECTION('',(-0.190809912898503,1.137179689376E-14,0.981627005099017));
#95868=DIRECTION('center_axis',(0.981627005099017,-1.19151365507148E-16,
0.190809912898504));
#95869=DIRECTION('ref_axis',(-0.183265446925925,-0.278415153951492,0.942814286067626));
#95870=DIRECTION('center_axis',(0.981627005099017,-1.43311947025832E-17,
0.190809912898503));
#95871=DIRECTION('ref_axis',(-0.183556130616892,-0.273104936120213,0.944309716554759));
#95872=DIRECTION('center_axis',(0.,1.,0.));
#95873=DIRECTION('ref_axis',(1.,0.,0.));
#95874=DIRECTION('',(-0.190809912898503,0.,0.981627005099017));
#95875=DIRECTION('center_axis',(0.,1.,0.));
#95876=DIRECTION('ref_axis',(-0.177572401270701,0.,0.984107739176437));
#95877=DIRECTION('center_axis',(0.,1.,0.));
#95878=DIRECTION('ref_axis',(-0.177845204798666,0.,0.984058475462775));
#95879=DIRECTION('center_axis',(-0.981627005099017,0.,-0.190809912898503));
#95880=DIRECTION('ref_axis',(-0.190809912898503,0.,0.981627005099017));
#95881=DIRECTION('center_axis',(-0.981627005099017,2.45286952692658E-16,
-0.190809912898504));
#95882=DIRECTION('ref_axis',(-0.181379056342926,-0.310496268400187,0.933109696246754));
#95883=DIRECTION('center_axis',(-0.981627005099017,6.43735225938313E-17,
-0.190809912898503));
#95884=DIRECTION('ref_axis',(-0.181743610098458,-0.304585001530188,0.934985153374766));
#95885=DIRECTION('center_axis',(0.,-1.,0.));
#95886=DIRECTION('ref_axis',(0.,0.,-1.));
#95887=DIRECTION('',(-0.190809912898503,0.,0.981627005099017));
#95888=DIRECTION('center_axis',(0.,-1.,0.));
#95889=DIRECTION('ref_axis',(-0.210808250907887,0.,0.977527432530237));
#95890=DIRECTION('',(-0.190809912898503,0.,0.981627005099017));
#95891=DIRECTION('center_axis',(0.,-1.,0.));
#95892=DIRECTION('ref_axis',(-0.210389062719221,0.,0.977617738325225));
#95893=DIRECTION('center_axis',(0.981627005099017,0.,0.190809912898503));
#95894=DIRECTION('ref_axis',(0.,-1.,0.));
#95895=DIRECTION('',(-0.190809912898503,0.,0.981627005099017));
#95896=DIRECTION('center_axis',(0.981627005099017,-1.41255374499376E-16,
0.190809912898504));
#95897=DIRECTION('ref_axis',(-0.183278336628812,-0.278182009056604,0.942880597509466));
#95898=DIRECTION('center_axis',(0.981627005099017,-9.30027011440924E-17,
0.190809912898504));
#95899=DIRECTION('ref_axis',(-0.183568046602459,-0.272884868293189,0.944371018680246));
#95900=DIRECTION('center_axis',(0.,1.,0.));
#95901=DIRECTION('ref_axis',(1.,0.,0.));
#95902=DIRECTION('',(-0.190809912898503,0.,0.981627005099017));
#95903=DIRECTION('center_axis',(0.,1.,0.));
#95904=DIRECTION('ref_axis',(-0.243413668799643,0.,0.969922566930731));
#95905=DIRECTION('center_axis',(0.,1.,0.));
#95906=DIRECTION('ref_axis',(-0.242336570704233,0.,0.97019224203212));
#95907=DIRECTION('center_axis',(-0.981627005099017,0.,-0.190809912898503));
#95908=DIRECTION('ref_axis',(-0.190809912898503,0.,0.981627005099017));
#95909=DIRECTION('center_axis',(-0.981627005099017,6.70648161298212E-17,
-0.190809912898503));
#95910=DIRECTION('ref_axis',(-0.181354700681431,-0.31088677343731,0.932984397855874));
#95911=DIRECTION('center_axis',(-0.981627005099017,1.50568650592271E-16,
-0.190809912898504));
#95912=DIRECTION('ref_axis',(-0.181721104376961,-0.304953598801405,0.934869372052636));
#95913=DIRECTION('center_axis',(0.,-1.,0.));
#95914=DIRECTION('ref_axis',(0.,0.,-1.));
#95915=DIRECTION('',(-0.190809912898503,0.,0.981627005099017));
#95916=DIRECTION('center_axis',(0.,-1.,0.));
#95917=DIRECTION('ref_axis',(-0.276893691776251,0.,0.960900558567076));
#95918=DIRECTION('',(-0.190809912898503,0.,0.981627005099017));
#95919=DIRECTION('center_axis',(0.,-1.,0.));
#95920=DIRECTION('ref_axis',(-0.275101194754168,0.,0.961415275853691));
#95921=DIRECTION('center_axis',(0.981627005099017,0.,0.190809912898503));
#95922=DIRECTION('ref_axis',(0.,-1.,0.));
#95923=DIRECTION('',(-0.190809912898503,0.,0.981627005099017));
#95924=DIRECTION('center_axis',(0.981627005099017,-7.48461333200017E-17,
0.190809912898504));
#95925=DIRECTION('ref_axis',(-0.183226511622911,-0.279118121617608,0.942613982297715));
#95926=DIRECTION('center_axis',(0.981627005099017,-1.94412209408584E-16,
0.190809912898504));
#95927=DIRECTION('ref_axis',(-0.183520146118496,-0.273768347927886,0.944124593282837));
#95928=DIRECTION('center_axis',(0.,1.,0.));
#95929=DIRECTION('ref_axis',(1.,0.,0.));
#95930=DIRECTION('',(-0.190809912898503,0.,0.981627005099017));
#95931=DIRECTION('center_axis',(0.,1.,0.));
#95932=DIRECTION('ref_axis',(-0.308384935821295,0.,0.951261652416671));
#95933=DIRECTION('center_axis',(0.,1.,0.));
#95934=DIRECTION('ref_axis',(-0.305993568691603,0.,0.952033579197382));
#95935=DIRECTION('center_axis',(-0.981627005099017,0.,-0.190809912898503));
#95936=DIRECTION('ref_axis',(-0.190809912898503,0.,0.981627005099017));
#95937=DIRECTION('center_axis',(-0.981627005099017,5.27367097735159E-17,
-0.190809912898503));
#95938=DIRECTION('ref_axis',(-0.181247688350776,-0.312596151213815,0.932433869887731));
#95939=DIRECTION('center_axis',(-0.981627005099017,-2.17379342169057E-17,
-0.190809912898503));
#95940=DIRECTION('ref_axis',(-0.181622273580826,-0.306566459909599,0.934360934220726));
#95941=DIRECTION('center_axis',(0.,-1.,0.));
#95942=DIRECTION('ref_axis',(0.,0.,-1.));
#95943=DIRECTION('',(-0.190809912898503,0.,0.981627005099017));
#95944=DIRECTION('center_axis',(0.,-1.,0.));
#95945=DIRECTION('ref_axis',(-0.342084131986487,0.,0.939669328350698));
#95946=DIRECTION('',(-0.190809912898503,0.,0.981627005099017));
#95947=DIRECTION('center_axis',(0.,-1.,0.));
#95948=DIRECTION('ref_axis',(-0.338955991905877,0.,0.940802229775793));
#95949=DIRECTION('center_axis',(0.981627005099017,0.,0.190809912898503));
#95950=DIRECTION('ref_axis',(0.,-1.,0.));
#95951=DIRECTION('',(-0.190809912898503,0.,0.981627005099017));
#95952=DIRECTION('center_axis',(0.981627005099017,6.83990283108474E-17,
0.190809912898503));
#95953=DIRECTION('ref_axis',(-0.183107255498057,-0.281259409527999,0.942000465783287));
#95954=DIRECTION('center_axis',(0.981627005099017,-1.82677034101796E-16,
0.190809912898504));
#95955=DIRECTION('ref_axis',(-0.183410017255811,-0.275787971799909,0.943558032227332));
#95956=DIRECTION('center_axis',(0.,1.,0.));
#95957=DIRECTION('ref_axis',(1.,0.,0.));
#95958=DIRECTION('',(-0.190809912898503,0.,0.981627005099017));
#95959=DIRECTION('center_axis',(0.,1.,0.));
#95960=DIRECTION('ref_axis',(-0.372470467214768,0.,0.928044045858176));
#95961=DIRECTION('center_axis',(0.,1.,0.));
#95962=DIRECTION('ref_axis',(-0.368801736329265,0.,0.929508084569746));
#95963=DIRECTION('center_axis',(-0.981627005099017,0.,-0.190809912898503));
#95964=DIRECTION('ref_axis',(-0.190809912898503,0.,0.981627005099017));
#95965=DIRECTION('center_axis',(-0.981627005099017,2.68930199968124E-16,
-0.190809912898504));
#95966=DIRECTION('ref_axis',(-0.181052299422872,-0.315690778691902,0.931428686010148));
#95967=DIRECTION('center_axis',(-0.981627005099017,1.40306285732571E-16,
-0.190809912898504));
#95968=DIRECTION('ref_axis',(-0.181442047051767,-0.309483781404091,0.933433753733755));
#95969=DIRECTION('center_axis',(0.,-1.,0.));
#95970=DIRECTION('ref_axis',(0.,0.,-1.));
#95971=DIRECTION('',(-0.190809912898503,0.,0.981627005099017));
#95972=DIRECTION('center_axis',(0.,-1.,0.));
#95973=DIRECTION('ref_axis',(-0.406356421956365,0.,0.913714648199765));
#95974=DIRECTION('',(-0.190809912898503,0.,0.981627005099017));
#95975=DIRECTION('center_axis',(0.,-1.,0.));
#95976=DIRECTION('ref_axis',(-0.40193223106788,0.,0.915669417218243));
#95977=DIRECTION('center_axis',(0.981627005099017,0.,0.190809912898503));
#95978=DIRECTION('ref_axis',(0.,-1.,0.));
#95979=DIRECTION('',(-0.190809912898503,0.,0.981627005099017));
#95980=DIRECTION('center_axis',(0.981627005099017,8.56509061367008E-17,
0.190809912898503));
#95981=DIRECTION('ref_axis',(-0.182914100187073,-0.284690508229704,0.941006772811262));
#95982=DIRECTION('center_axis',(0.981627005099017,-2.61778094159889E-16,
0.190809912898504));
#95983=DIRECTION('ref_axis',(-0.18323192975892,-0.279020413474902,0.942641856051977));
#95984=DIRECTION('center_axis',(0.,1.,0.));
#95985=DIRECTION('ref_axis',(1.,0.,0.));
#95986=DIRECTION('',(-0.190809912898503,0.,0.981627005099017));
#95987=DIRECTION('center_axis',(0.,1.,0.));
#95988=DIRECTION('ref_axis',(-0.435641230883273,0.,0.900120390811422));
#95989=DIRECTION('center_axis',(0.,1.,0.));
#95990=DIRECTION('ref_axis',(-0.430734436520186,0.,0.902478722849263));
#95991=DIRECTION('center_axis',(-0.981627005099017,0.,-0.190809912898503));
#95992=DIRECTION('ref_axis',(-0.190809912898503,0.,0.981627005099017));
#95993=DIRECTION('center_axis',(-0.981627005099017,-7.90952612425299E-18,
-0.190809912898503));
#95994=DIRECTION('ref_axis',(-0.180757579546461,-0.320295888279689,0.929912491252607));
#95995=DIRECTION('center_axis',(-0.981627005099017,5.31500700570768E-17,
-0.190809912898503));
#95996=DIRECTION('ref_axis',(-0.181170744386621,-0.313818853760112,0.932038029483286));
#95997=DIRECTION('center_axis',(0.,-1.,0.));
#95998=DIRECTION('ref_axis',(0.,0.,-1.));
#95999=DIRECTION('',(-0.190809912898503,0.,0.981627005099017));
#96000=DIRECTION('center_axis',(0.,-1.,0.));
#96001=DIRECTION('ref_axis',(-0.469672502576099,0.,0.882840721944737));
#96002=DIRECTION('',(-0.190809912898503,0.,0.981627005099017));
#96003=DIRECTION('center_axis',(0.,-1.,0.));
#96004=DIRECTION('ref_axis',(-0.463995103545157,0.,0.88583776386318));
#96005=DIRECTION('center_axis',(0.981627005099017,0.,0.190809912898503));
#96006=DIRECTION('ref_axis',(0.,-1.,0.));
#96007=DIRECTION('',(-0.190809912898503,0.,0.981627005099017));
#96008=DIRECTION('center_axis',(0.981627005099017,0.,0.190809912898503));
#96009=DIRECTION('ref_axis',(-0.182635912358673,-0.2895544222692,0.939575627643281));
#96010=DIRECTION('center_axis',(0.981627005099017,-2.16345510275123E-16,
0.190809912898504));
#96011=DIRECTION('ref_axis',(-0.18297605983338,-0.283594808995592,0.941325525967826));
#96012=DIRECTION('center_axis',(0.,1.,0.));
#96013=DIRECTION('ref_axis',(1.,0.,0.));
#96014=DIRECTION('',(-0.190809912898503,0.,0.981627005099017));
#96015=DIRECTION('center_axis',(0.,1.,0.));
#96016=DIRECTION('ref_axis',(-0.497852697527391,0.,0.867261605033164));
#96017=DIRECTION('center_axis',(0.,1.,0.));
#96018=DIRECTION('ref_axis',(-0.491750929833315,0.,0.870735908877123));
#96019=DIRECTION('center_axis',(-0.981627005099017,0.,-0.190809912898503));
#96020=DIRECTION('ref_axis',(-0.190809912898503,0.,0.981627005099017));
#96021=DIRECTION('center_axis',(-0.981627005099017,1.97387161584057E-16,
-0.190809912898504));
#96022=DIRECTION('ref_axis',(-0.180345720095873,-0.326610363710094,0.927793668635576));
#96023=DIRECTION('center_axis',(-0.981627005099017,1.57652634340856E-16,
-0.190809912898504));
#96024=DIRECTION('ref_axis',(-0.180792707058803,-0.319750880716613,0.930093205735479));
#96025=DIRECTION('center_axis',(0.,-1.,0.));
#96026=DIRECTION('ref_axis',(0.,0.,-1.));
#96027=DIRECTION('',(-0.190809912898503,0.,0.981627005099017));
#96028=DIRECTION('center_axis',(0.,-1.,0.));
#96029=DIRECTION('ref_axis',(-0.464446491029698,0.,0.885601183925474));
#96030=DIRECTION('',(-0.190809912898503,0.,0.981627005099017));
#96031=DIRECTION('center_axis',(0.,-1.,0.));
#96032=DIRECTION('ref_axis',(-0.459078725961924,0.,0.888395589458422));
#96033=DIRECTION('center_axis',(0.981627005099017,0.,0.190809912898503));
#96034=DIRECTION('ref_axis',(0.,-1.,0.));
#96035=DIRECTION('',(-0.190809912898503,0.,0.981627005099017));
#96036=DIRECTION('center_axis',(0.981627005099017,8.05478041870284E-18,
0.190809912898503));
#96037=DIRECTION('ref_axis',(-0.186039172622593,-0.222216184532195,0.957083796530823));
#96038=DIRECTION('center_axis',(0.981627005099017,-1.08172755137562E-16,
0.190809912898504));
#96039=DIRECTION('ref_axis',(-0.186235922579013,-0.217642527833793,0.958095982258177));
#96040=DIRECTION('center_axis',(0.,1.,0.));
#96041=DIRECTION('ref_axis',(1.,0.,0.));
#96042=DIRECTION('',(-0.190809912898503,0.,0.981627005099017));
#96043=DIRECTION('center_axis',(0.,1.,0.));
#96044=DIRECTION('ref_axis',(-0.492873509125509,0.,0.870100973452108));
#96045=DIRECTION('center_axis',(0.,1.,0.));
#96046=DIRECTION('ref_axis',(-0.487060705905151,0.,0.873368117555923));
#96047=DIRECTION('center_axis',(-0.981627005099017,0.,-0.190809912898503));
#96048=DIRECTION('ref_axis',(-0.190809912898503,0.,0.981627005099017));
#96049=DIRECTION('center_axis',(-0.981627005099017,5.75712554620167E-17,
-0.190809912898503));
#96050=DIRECTION('ref_axis',(-0.184321126056631,-0.258566537937205,0.948245257277031));
#96051=DIRECTION('center_axis',(-0.981627005099017,3.94131585852141E-17,
-0.190809912898503));
#96052=DIRECTION('ref_axis',(-0.184595362527196,-0.253136113900701,0.949656074572634));
#96053=DIRECTION('center_axis',(0.,-1.,0.));
#96054=DIRECTION('ref_axis',(0.,0.,-1.));
#96055=DIRECTION('',(-0.190809912898503,0.,0.981627005099017));
#96056=DIRECTION('center_axis',(0.,-1.,0.));
#96057=DIRECTION('ref_axis',(-0.460630809902228,0.,0.887591830161149));
#96058=DIRECTION('',(-0.190809912898503,0.,0.981627005099017));
#96059=DIRECTION('center_axis',(0.,-1.,0.));
#96060=DIRECTION('ref_axis',(-0.455482023679629,0.,0.890244980948901));
#96061=DIRECTION('center_axis',(0.981627005099017,0.,0.190809912898503));
#96062=DIRECTION('ref_axis',(0.,-1.,0.));
#96063=DIRECTION('',(-0.190809912898503,0.,0.981627005099017));
#96064=DIRECTION('center_axis',(0.981627005099017,4.83286825122171E-17,
0.190809912898503));
#96065=DIRECTION('ref_axis',(-0.188507526443361,-0.154877946795105,0.969782312723189));
#96066=DIRECTION('center_axis',(0.981627005099017,-3.86331268348435E-17,
0.190809912898503));
#96067=DIRECTION('ref_axis',(-0.188601875825374,-0.151690246672095,0.97026769579313));
#96068=DIRECTION('center_axis',(0.,1.,0.));
#96069=DIRECTION('ref_axis',(1.,0.,0.));
#96070=DIRECTION('',(-0.190809912898503,0.,0.981627005099017));
#96071=DIRECTION('center_axis',(0.,1.,0.));
#96072=DIRECTION('ref_axis',(-0.489357122006741,0.,0.872083486336761));
#96073=DIRECTION('center_axis',(0.,1.,0.));
#96074=DIRECTION('ref_axis',(-0.483742917424828,0.,0.875210140389905));
#96075=DIRECTION('center_axis',(-0.981627005099017,0.,-0.190809912898503));
#96076=DIRECTION('ref_axis',(-0.190809912898503,0.,0.981627005099017));
#96077=DIRECTION('center_axis',(-0.981627005099017,1.64489301320047E-16,
-0.190809912898504));
#96078=DIRECTION('ref_axis',(-0.187314807261953,-0.190522712164197,0.963646335088769));
#96079=DIRECTION('center_axis',(-0.981627005099017,1.65535266057899E-16,
-0.190809912898504));
#96080=DIRECTION('ref_axis',(-0.187461372226399,-0.186521347084696,0.964400342702503));
#96081=DIRECTION('center_axis',(0.,-1.,0.));
#96082=DIRECTION('ref_axis',(0.,0.,-1.));
#96083=DIRECTION('',(-0.190809912898503,0.,0.981627005099017));
#96084=DIRECTION('center_axis',(0.,-1.,0.));
#96085=DIRECTION('ref_axis',(-0.458064609075315,0.,0.888918901763642));
#96086=DIRECTION('',(-0.190809912898517,0.,0.981627005099014));
#96087=DIRECTION('center_axis',(0.,-1.,0.));
#96088=DIRECTION('ref_axis',(-0.453059767116766,0.,0.891480144153588));
#96089=DIRECTION('center_axis',(0.981627005099017,0.,0.190809912898503));
#96090=DIRECTION('ref_axis',(0.,-1.,0.));
#96091=DIRECTION('',(-0.190809912898503,0.,0.981627005099017));
#96092=DIRECTION('center_axis',(0.981627005099017,-8.05478041870284E-18,
0.190809912898503));
#96093=DIRECTION('ref_axis',(-0.190077399524955,-0.087539709058116,0.977858569286914));
#96094=DIRECTION('center_axis',(0.981627005099017,-2.51115324426482E-17,
0.190809912898504));
#96095=DIRECTION('ref_axis',(-0.190107297572009,-0.0857379655103025,0.978012380637393));
#96096=DIRECTION('center_axis',(0.,1.,0.));
#96097=DIRECTION('ref_axis',(1.,0.,0.));
#96098=DIRECTION('',(-0.190809912898503,0.,0.981627005099017));
#96099=DIRECTION('center_axis',(0.,1.,0.));
#96100=DIRECTION('ref_axis',(-0.48716094882944,0.,0.873312206450591));
#96101=DIRECTION('center_axis',(0.,1.,0.));
#96102=DIRECTION('ref_axis',(-0.481668504198278,0.,0.876353497204977));
#96103=DIRECTION('center_axis',(-0.981627005099017,0.,-0.190809912898503));
#96104=DIRECTION('ref_axis',(-0.190809912898503,0.,0.981627005099017));
#96105=DIRECTION('center_axis',(-0.981627005099017,-2.0561162665006E-17,
-0.190809912898503));
#96106=DIRECTION('ref_axis',(-0.18937332780328,-0.122478886391301,0.974236452359004));
#96107=DIRECTION('center_axis',(-0.981627005099017,-1.97065792926071E-17,
-0.190809912898503));
#96108=DIRECTION('ref_axis',(-0.189433253567106,-0.119906580268704,0.974544742149505));
#96109=DIRECTION('center_axis',(0.,-1.,0.));
#96110=DIRECTION('ref_axis',(0.,0.,-1.));
#96111=DIRECTION('',(-0.190809912898503,0.,0.981627005099017));
#96112=DIRECTION('center_axis',(0.,-1.,0.));
#96113=DIRECTION('ref_axis',(-0.456646407116791,0.,0.889648278179262));
#96114=DIRECTION('',(-0.190809912898503,0.,0.981627005099017));
#96115=DIRECTION('center_axis',(0.,-1.,0.));
#96116=DIRECTION('ref_axis',(-0.451719976566491,0.,0.892159774239328));
#96117=DIRECTION('center_axis',(0.981627005099017,0.,0.190809912898503));
#96118=DIRECTION('ref_axis',(0.,-1.,0.));
#96119=DIRECTION('',(-0.190809912898503,0.,0.981627005099017));
#96120=DIRECTION('center_axis',(0.981627005099017,-1.56061370612367E-17,
0.190809912898504));
#96121=DIRECTION('ref_axis',(-0.190770974215747,-0.0202014713211108,0.981426683941922));
#96122=DIRECTION('center_axis',(0.981627005099017,0.,0.190809912898503));
#96123=DIRECTION('ref_axis',(-0.190772560748925,-0.0197856843485292,0.981434845906827));
#96124=DIRECTION('center_axis',(0.,1.,0.));
#96125=DIRECTION('ref_axis',(1.,0.,0.));
#96126=DIRECTION('',(-0.190809912898503,0.,0.981627005099017));
#96127=DIRECTION('center_axis',(0.,1.,0.));
#96128=DIRECTION('ref_axis',(-0.486200442577545,0.,0.873847314831029));
#96129=DIRECTION('center_axis',(0.,1.,0.));
#96130=DIRECTION('ref_axis',(-0.480760703718784,0.,0.87685183797482));
#96131=DIRECTION('center_axis',(-0.981627005099017,0.,-0.190809912898503));
#96132=DIRECTION('ref_axis',(-0.190809912898503,0.,0.981627005099017));
#96133=DIRECTION('center_axis',(-0.981627005099017,4.11223253300119E-18,
-0.190809912898503));
#96134=DIRECTION('ref_axis',(-0.190527001503476,-0.0544350606183517,0.980171559408643));
#96135=DIRECTION('center_axis',(-0.981627005099017,1.18239475755642E-17,
-0.190809912898504));
#96136=DIRECTION('ref_axis',(-0.190538768513374,-0.05329181345277,0.980232095124579));
#96137=DIRECTION('center_axis',(0.,-1.,0.));
#96138=DIRECTION('ref_axis',(0.,0.,-1.));
#96139=DIRECTION('',(-0.190809912898503,0.,0.981627005099017));
#96140=DIRECTION('center_axis',(0.,-1.,0.));
#96141=DIRECTION('ref_axis',(0.185064286707852,0.,0.982726416550056));
#96142=DIRECTION('',(-0.190809912898503,0.,0.981627005099017));
#96143=DIRECTION('center_axis',(0.,-1.,0.));
#96144=DIRECTION('ref_axis',(0.177619933460537,0.,0.984099161282782));
#96145=DIRECTION('center_axis',(0.981627005099017,0.,0.190809912898503));
#96146=DIRECTION('ref_axis',(0.,-1.,0.));
#96147=DIRECTION('',(-0.190809912898503,0.,0.981627005099017));
#96148=DIRECTION('center_axis',(0.981627005099017,-1.66640035983327E-17,
0.190809912898504));
#96149=DIRECTION('ref_axis',(-0.19076833445818,-0.0208749271362605,0.981413103634299));
#96150=DIRECTION('center_axis',(0.981627005099017,4.62805617161513E-18,
0.190809912898503));
#96151=DIRECTION('ref_axis',(-0.190770138410662,-0.0204171065775405,0.981422384118978));
#96152=DIRECTION('center_axis',(0.,1.,0.));
#96153=DIRECTION('ref_axis',(1.,0.,0.));
#96154=DIRECTION('',(-0.190809912898503,0.,0.981627005099017));
#96155=DIRECTION('center_axis',(0.,1.,0.));
#96156=DIRECTION('ref_axis',(0.150536423879934,0.,0.988604463415698));
#96157=DIRECTION('center_axis',(0.,1.,0.));
#96158=DIRECTION('ref_axis',(0.143816312892431,0.,0.989604399821477));
#96159=DIRECTION('center_axis',(-0.981627005099017,0.,-0.190809912898503));
#96160=DIRECTION('ref_axis',(-0.190809912898503,0.,0.981627005099017));
#96161=DIRECTION('center_axis',(-0.981627005099017,0.,-0.190809912898503));
#96162=DIRECTION('ref_axis',(-0.190521659123586,-0.0549462364013984,0.980144075383878));
#96163=DIRECTION('center_axis',(-0.981627005099017,2.80877720141023E-17,
-0.190809912898504));
#96164=DIRECTION('ref_axis',(-0.190533865149434,-0.0537711722184585,0.980206869629809));
#96165=DIRECTION('center_axis',(0.,-1.,0.));
#96166=DIRECTION('ref_axis',(0.,0.,-1.));
#96167=DIRECTION('',(-0.190809912898503,0.,0.981627005099017));
#96168=DIRECTION('center_axis',(0.,-1.,0.));
#96169=DIRECTION('ref_axis',(0.187211227674096,0.,0.982319681281383));
#96170=DIRECTION('',(-0.190809912898503,0.,0.981627005099017));
#96171=DIRECTION('center_axis',(0.,-1.,0.));
#96172=DIRECTION('ref_axis',(0.179642428155144,0.,0.983731974679345));
#96173=DIRECTION('center_axis',(0.981627005099017,0.,0.190809912898503));
#96174=DIRECTION('ref_axis',(0.,-1.,0.));
#96175=DIRECTION('',(-0.190809912898503,0.,0.981627005099017));
#96176=DIRECTION('center_axis',(0.981627005099017,-2.1501940126881E-18,
0.190809912898503));
#96177=DIRECTION('ref_axis',(-0.190027643704127,-0.0904580175904463,0.977602599056418));
#96178=DIRECTION('center_axis',(0.981627005099017,-2.05691385405117E-18,
0.190809912898503));
#96179=DIRECTION('ref_axis',(-0.190061647076601,-0.0884741285026728,0.97777753036988));
#96180=DIRECTION('center_axis',(0.,1.,0.));
#96181=DIRECTION('ref_axis',(1.,0.,0.));
#96182=DIRECTION('',(-0.190809912898503,0.,0.981627005099017));
#96183=DIRECTION('center_axis',(0.,1.,0.));
#96184=DIRECTION('ref_axis',(0.151724977115547,0.,0.988422749292673));
#96185=DIRECTION('center_axis',(0.,1.,0.));
#96186=DIRECTION('ref_axis',(0.144936472974812,0.,0.989440962767169));
#96187=DIRECTION('center_axis',(-0.981627005099017,0.,-0.190809912898503));
#96188=DIRECTION('ref_axis',(-0.190809912898503,0.,0.981627005099017));
#96189=DIRECTION('center_axis',(-0.981627005099017,2.51389650319736E-17,
-0.190809912898503));
#96190=DIRECTION('ref_axis',(-0.189346115666816,-0.123629031903203,0.974096458751681));
#96191=DIRECTION('center_axis',(-0.981627005099017,6.01880828873621E-17,
-0.190809912898504));
#96192=DIRECTION('ref_axis',(-0.189408284096429,-0.120985137491496,0.974416285999885));
#96193=DIRECTION('center_axis',(0.,-1.,0.));
#96194=DIRECTION('ref_axis',(0.,0.,-1.));
#96195=DIRECTION('',(-0.190809912898503,0.,0.981627005099017));
#96196=DIRECTION('center_axis',(0.,-1.,0.));
#96197=DIRECTION('ref_axis',(0.191100511883499,0.,0.981570473454588));
#96198=DIRECTION('',(-0.190809912898503,0.,0.981627005099017));
#96199=DIRECTION('center_axis',(0.,-1.,0.));
#96200=DIRECTION('ref_axis',(0.18330289149611,0.,0.983056483610767));
#96201=DIRECTION('center_axis',(0.981627005099017,0.,0.190809912898503));
#96202=DIRECTION('ref_axis',(0.,-1.,0.));
#96203=DIRECTION('',(-0.190809912898503,0.,0.981627005099017));
#96204=DIRECTION('center_axis',(0.981627005099017,-1.29011640761286E-16,
0.190809912898504));
#96205=DIRECTION('ref_axis',(-0.188350439968379,-0.160041108044595,0.968974176900281));
#96206=DIRECTION('center_axis',(0.981627005099017,-4.11382770810234E-17,
0.190809912898504));
#96207=DIRECTION('ref_axis',(-0.188457803354032,-0.156531150427793,0.969526510880814));
#96208=DIRECTION('center_axis',(0.,1.,0.));
#96209=DIRECTION('ref_axis',(1.,0.,0.));
#96210=DIRECTION('',(-0.190809912898503,0.,0.981627005099017));
#96211=DIRECTION('center_axis',(0.,1.,0.));
#96212=DIRECTION('ref_axis',(0.154444807220379,0.,0.988001417773608));
#96213=DIRECTION('center_axis',(0.,1.,0.));
#96214=DIRECTION('ref_axis',(0.147498119662627,0.,0.989062336102224));
#96215=DIRECTION('center_axis',(-0.981627005099017,0.,-0.190809912898503));
#96216=DIRECTION('ref_axis',(-0.190809912898503,0.,0.981627005099017));
#96217=DIRECTION('center_axis',(-0.981627005099017,1.63403272707828E-16,
-0.190809912898504));
#96218=DIRECTION('ref_axis',(-0.18724822993152,-0.192311827404893,0.963303826125332));
#96219=DIRECTION('center_axis',(-0.981627005099017,1.00313471478937E-16,
-0.190809912898504));
#96220=DIRECTION('ref_axis',(-0.187400310802369,-0.188199102764594,0.964086210475898));
#96221=DIRECTION('center_axis',(0.,-1.,0.));
#96222=DIRECTION('ref_axis',(0.,0.,-1.));
#96223=DIRECTION('',(-0.190809912898503,0.,0.981627005099017));
#96224=DIRECTION('center_axis',(0.,-1.,0.));
#96225=DIRECTION('ref_axis',(0.196894140539301,0.,0.980424753574332));
#96226=DIRECTION('',(-0.190809912898503,0.,0.981627005099017));
#96227=DIRECTION('center_axis',(0.,-1.,0.));
#96228=DIRECTION('ref_axis',(0.188747517532452,0.,0.982025648659615));
#96229=DIRECTION('center_axis',(0.981627005099017,0.,0.190809912898503));
#96230=DIRECTION('ref_axis',(0.,-1.,0.));
#96231=DIRECTION('',(-0.190809912898503,0.,0.981627005099017));
#96232=DIRECTION('center_axis',(0.981627005099017,-6.88062084060191E-17,
0.190809912898504));
#96233=DIRECTION('ref_axis',(-0.185711351364325,-0.229624198498799,0.955397310776109));
#96234=DIRECTION('center_axis',(0.981627005099017,-9.05042095782515E-17,
0.190809912898504));
#96235=DIRECTION('ref_axis',(-0.185935439268292,-0.224588172352909,0.956550137349469));
#96236=DIRECTION('center_axis',(0.,1.,0.));
#96237=DIRECTION('ref_axis',(1.,0.,0.));
#96238=DIRECTION('',(-0.190809912898503,0.,0.981627005099017));
#96239=DIRECTION('center_axis',(0.,1.,0.));
#96240=DIRECTION('ref_axis',(0.158806144368473,0.,0.987309783457462));
#96241=DIRECTION('center_axis',(0.,1.,0.));
#96242=DIRECTION('ref_axis',(0.15160090640473,0.,0.988441786438263));
#96243=DIRECTION('center_axis',(-0.981627005099017,0.,-0.190809912898503));
#96244=DIRECTION('ref_axis',(-0.190809912898503,0.,0.981627005099017));
#96245=DIRECTION('center_axis',(-0.981627005099017,1.00555860127894E-16,
-0.190809912898504));
#96246=DIRECTION('ref_axis',(-0.1841964898643,-0.260994622906685,0.947604062852977));
#96247=DIRECTION('center_axis',(-0.981627005099017,1.92601865239559E-16,
-0.190809912898504));
#96248=DIRECTION('ref_axis',(-0.184481134488586,-0.255413068037693,0.949068425190395));
#96249=DIRECTION('center_axis',(0.,-1.,0.));
#96250=DIRECTION('ref_axis',(0.,0.,-1.));
#96251=DIRECTION('',(-0.190809912898503,0.,0.981627005099017));
#96252=DIRECTION('center_axis',(0.,-1.,0.));
#96253=DIRECTION('ref_axis',(0.126677774296384,0.,0.991943920541537));
#96254=DIRECTION('',(-0.190809912898503,0.,0.981627005099017));
#96255=DIRECTION('center_axis',(0.,-1.,0.));
#96256=DIRECTION('ref_axis',(0.120056982034697,0.,0.992767002405258));
#96257=DIRECTION('center_axis',(0.981627005099017,0.,0.190809912898503));
#96258=DIRECTION('ref_axis',(0.,-1.,0.));
#96259=DIRECTION('',(-0.190809912898503,0.,0.981627005099017));
#96260=DIRECTION('center_axis',(0.981627005099017,0.,0.190809912898503));
#96261=DIRECTION('ref_axis',(-0.1859589704051,-0.224052422420893,0.956671193949732));
#96262=DIRECTION('center_axis',(0.981627005099017,-1.56990815882154E-16,
0.190809912898504));
#96263=DIRECTION('ref_axis',(-0.186162251270113,-0.219366829807895,0.957716978121448));
#96264=DIRECTION('center_axis',(0.,1.,0.));
#96265=DIRECTION('ref_axis',(1.,0.,0.));
#96266=DIRECTION('',(-0.190809912898503,0.,0.981627005099017));
#96267=DIRECTION('center_axis',(0.,1.,0.));
#96268=DIRECTION('ref_axis',(0.0896762875991086,0.,0.995970965160351));
#96269=DIRECTION('center_axis',(0.,1.,0.));
#96270=DIRECTION('ref_axis',(0.0839371904866857,0.,0.996471047272926));
#96271=DIRECTION('center_axis',(-0.981627005099017,0.,-0.190809912898503));
#96272=DIRECTION('ref_axis',(-0.190809912898503,0.,0.981627005099017));
#96273=DIRECTION('center_axis',(-0.981627005099017,-6.41908343804613E-17,
-0.190809912898503));
#96274=DIRECTION('ref_axis',(-0.184482115855883,-0.25539359847171,0.949073473862276));
#96275=DIRECTION('center_axis',(-0.981627005099017,6.15853067906846E-17,
-0.190809912898503));
#96276=DIRECTION('ref_axis',(-0.184743183521159,-0.250156649499107,0.950416543865819));
#96277=DIRECTION('center_axis',(0.,-1.,0.));
#96278=DIRECTION('ref_axis',(0.,0.,-1.));
#96279=DIRECTION('',(-0.190809912898503,0.,0.981627005099017));
#96280=DIRECTION('center_axis',(0.,-1.,0.));
#96281=DIRECTION('ref_axis',(0.057455673972295,0.,0.998348058308519));
#96282=DIRECTION('',(-0.190809912898503,0.,0.981627005099017));
#96283=DIRECTION('center_axis',(0.,-1.,0.));
#96284=DIRECTION('ref_axis',(0.0523145803672791,0.,0.998630654787342));
#96285=DIRECTION('center_axis',(0.981627005099017,0.,0.190809912898503));
#96286=DIRECTION('ref_axis',(0.,-1.,0.));
#96287=DIRECTION('',(-0.190809912898503,0.,0.981627005099017));
#96288=DIRECTION('center_axis',(0.981627005099017,-1.02481602251098E-16,
0.190809912898504));
#96289=DIRECTION('ref_axis',(-0.186142071902388,-0.219836656826109,0.957613164792238));
#96290=DIRECTION('center_axis',(0.981627005099017,3.78430184869551E-17,
0.190809912898503));
#96291=DIRECTION('ref_axis',(-0.186330592575348,-0.215405464478295,0.958583014737592));
#96292=DIRECTION('center_axis',(0.,1.,0.));
#96293=DIRECTION('ref_axis',(1.,0.,0.));
#96294=DIRECTION('',(-0.190809912898503,0.,0.981627005099017));
#96295=DIRECTION('center_axis',(0.,1.,0.));
#96296=DIRECTION('ref_axis',(0.0214917304669384,0.,0.999769026086294));
#96297=DIRECTION('center_axis',(0.,1.,0.));
#96298=DIRECTION('ref_axis',(0.0171769281236512,0.,0.999852465686931));
#96299=DIRECTION('center_axis',(-0.981627005099017,0.,-0.190809912898503));
#96300=DIRECTION('ref_axis',(-0.190809912898503,0.,0.981627005099017));
#96301=DIRECTION('center_axis',(-0.981627005099017,0.,-0.190809912898503));
#96302=DIRECTION('ref_axis',(-0.184690180329235,-0.251229314473896,0.950143867442679));
#96303=DIRECTION('center_axis',(-0.981627005099017,1.41720243526492E-16,
-0.190809912898504));
#96304=DIRECTION('ref_axis',(-0.184934689487586,-0.246239451375998,0.951401751738022));
#96305=DIRECTION('center_axis',(0.,-1.,0.));
#96306=DIRECTION('ref_axis',(0.,0.,-1.));
#96307=DIRECTION('',(-0.190809912898503,0.,0.981627005099017));
#96308=DIRECTION('center_axis',(0.,-1.,0.));
#96309=DIRECTION('ref_axis',(-0.0108312859749144,0.,0.999941339901561));
#96310=DIRECTION('',(-0.190809912898503,0.,0.981627005099017));
#96311=DIRECTION('center_axis',(0.,-1.,0.));
#96312=DIRECTION('ref_axis',(-0.0145336816644732,0.,0.999894380470895));
#96313=DIRECTION('center_axis',(0.981627005099017,0.,0.190809912898503));
#96314=DIRECTION('ref_axis',(0.,-1.,0.));
#96315=DIRECTION('',(-0.190809912898503,0.,0.981627005099017));
#96316=DIRECTION('center_axis',(0.981627005099017,-7.66548341238665E-18,
0.190809912898503));
#96317=DIRECTION('ref_axis',(-0.186272558126613,-0.216779698406492,0.958284454871182));
#96318=DIRECTION('center_axis',(0.981627005099017,0.,0.190809912898503));
#96319=DIRECTION('ref_axis',(-0.186450886145693,-0.212527275133194,0.959201868419753));
#96320=DIRECTION('center_axis',(0.,1.,0.));
#96321=DIRECTION('ref_axis',(1.,0.,0.));
#96322=DIRECTION('',(-0.190809912898503,0.,0.981627005099017));
#96323=DIRECTION('center_axis',(0.,1.,0.));
#96324=DIRECTION('ref_axis',(-0.0457955137113147,0.,0.998950835088453));
#96325=DIRECTION('center_axis',(0.,1.,0.));
#96326=DIRECTION('ref_axis',(-0.0487238586301981,0.,0.998812287469565));
#96327=DIRECTION('center_axis',(-0.981627005099017,0.,-0.190809912898503));
#96328=DIRECTION('ref_axis',(-0.190809912898503,0.,0.981627005099017));
#96329=DIRECTION('center_axis',(-0.981627005099017,-2.27558651128372E-17,
-0.190809912898503));
#96330=DIRECTION('ref_axis',(-0.184833575911802,-0.248315905441003,0.950881570081507));
#96331=DIRECTION('center_axis',(-0.981627005099017,1.3128444595013E-16,
-0.190809912898504));
#96332=DIRECTION('ref_axis',(-0.185066976672435,-0.243494342879606,0.95208230690994));
#96333=DIRECTION('center_axis',(0.,-1.,0.));
#96334=DIRECTION('ref_axis',(0.,0.,-1.));
#96335=DIRECTION('',(-0.190809912898503,0.,0.981627005099017));
#96336=DIRECTION('center_axis',(0.,-1.,0.));
#96337=DIRECTION('ref_axis',(-0.0782243178778391,0.,0.996935783334386));
#96338=DIRECTION('',(-0.190809912898503,0.,0.981627005099017));
#96339=DIRECTION('center_axis',(0.,-1.,0.));
#96340=DIRECTION('ref_axis',(-0.0805255845251147,0.,0.996752542127126));
#96341=DIRECTION('center_axis',(0.981627005099017,0.,0.190809912898503));
#96342=DIRECTION('ref_axis',(0.,-1.,0.));
#96343=DIRECTION('',(-0.190809912898503,0.,0.981627005099017));
#96344=DIRECTION('center_axis',(0.981627005099017,-1.50452980269455E-16,
0.190809912898504));
#96345=DIRECTION('ref_axis',(-0.186358114771361,-0.214750524536794,0.958724603455047));
#96346=DIRECTION('center_axis',(0.981627005099017,2.89425911527956E-17,
0.190809912898503));
#96347=DIRECTION('ref_axis',(-0.186529907529078,-0.210614148632799,0.959608396166308));
#96348=DIRECTION('center_axis',(0.,1.,0.));
#96349=DIRECTION('ref_axis',(1.,0.,0.));
#96350=DIRECTION('',(-0.190809912898503,0.,0.981627005099017));
#96351=DIRECTION('center_axis',(0.,1.,0.));
#96352=DIRECTION('ref_axis',(-0.11221795040211,0.,0.993683617459576));
#96353=DIRECTION('center_axis',(0.,1.,0.));
#96354=DIRECTION('ref_axis',(-0.113795052586422,0.,0.993504245590754));
#96355=DIRECTION('center_axis',(-0.981627005099017,0.,-0.190809912898503));
#96356=DIRECTION('ref_axis',(-0.190809912898503,0.,0.981627005099017));
#96357=DIRECTION('center_axis',(-0.981627005099017,1.57011489457449E-16,
-0.190809912898504));
#96358=DIRECTION('ref_axis',(-0.184920463723457,-0.246532715705106,0.951328566891254));
#96359=DIRECTION('center_axis',(-0.981627005099017,-1.00704279750265E-16,
-0.190809912898503));
#96360=DIRECTION('ref_axis',(-0.185147254406488,-0.241812327014693,0.95249529798812));
#96361=DIRECTION('center_axis',(0.,-1.,0.));
#96362=DIRECTION('ref_axis',(0.,0.,-1.));
#96363=DIRECTION('',(-0.190809912898503,0.,0.981627005099017));
#96364=DIRECTION('center_axis',(0.,-1.,0.));
#96365=DIRECTION('ref_axis',(-0.144750026222805,0.,0.989468256139881));
#96366=DIRECTION('',(-0.190809912898503,0.,0.981627005099017));
#96367=DIRECTION('center_axis',(0.,-1.,0.));
#96368=DIRECTION('ref_axis',(-0.145685581668177,0.,0.989330941239586));
#96369=DIRECTION('center_axis',(0.981627005099017,0.,0.190809912898503));
#96370=DIRECTION('ref_axis',(0.,-1.,0.));
#96371=DIRECTION('',(-0.190809912898503,-1.011721224396E-14,0.981627005099017));
#96372=DIRECTION('center_axis',(0.981627005099017,-8.93635241303609E-17,
0.190809912898504));
#96373=DIRECTION('ref_axis',(-0.186403435751544,-0.213667443730199,0.958957758522148));
#96374=DIRECTION('center_axis',(0.981627005099017,-8.59871682154991E-17,
0.190809912898504));
#96375=DIRECTION('ref_axis',(-0.186571814196846,-0.209592160278304,0.959823986206414));
#96376=DIRECTION('center_axis',(0.,1.,0.));
#96377=DIRECTION('ref_axis',(1.,0.,0.));
#96378=DIRECTION('',(-0.190809912898503,1.157372297933E-14,0.981627005099017));
#96379=DIRECTION('center_axis',(0.,1.,0.));
#96380=DIRECTION('ref_axis',(-0.177795049856396,0.,0.984067538457885));
#96381=DIRECTION('center_axis',(0.,1.,0.));
#96382=DIRECTION('ref_axis',(-0.178054589517587,0.,0.98402061114172));
#96383=DIRECTION('center_axis',(-0.981627005099017,0.,-0.190809912898503));
#96384=DIRECTION('ref_axis',(-0.190809912898503,0.,0.981627005099017));
#96385=DIRECTION('center_axis',(-0.981627005099017,2.22988138811507E-16,
-0.190809912898504));
#96386=DIRECTION('ref_axis',(-0.184955510912788,-0.245809545816807,0.951508868150121));
#96387=DIRECTION('center_axis',(-0.981627005099017,1.21594431566126E-16,
-0.190809912898504));
#96388=DIRECTION('ref_axis',(-0.185179661199109,-0.241129792878107,0.952662015651272));
#96389=DIRECTION('center_axis',(0.,-1.,0.));
#96390=DIRECTION('ref_axis',(0.,0.,-1.));
#96391=DIRECTION('',(-0.190809912898503,0.,0.981627005099017));
#96392=DIRECTION('center_axis',(0.,-1.,0.));
#96393=DIRECTION('ref_axis',(-0.210422369826518,0.,0.977610569847008));
#96394=DIRECTION('',(-0.190809912898503,0.,0.981627005099017));
#96395=DIRECTION('center_axis',(0.,-1.,0.));
#96396=DIRECTION('ref_axis',(-0.210026523774284,0.,0.977695688499898));
#96397=DIRECTION('center_axis',(0.981627005099017,0.,0.190809912898503));
#96398=DIRECTION('ref_axis',(0.,-1.,0.));
#96399=DIRECTION('',(-0.190809912898503,0.,0.981627005099017));
#96400=DIRECTION('center_axis',(0.981627005099017,-2.30469295235825E-16,
0.190809912898504));
#96401=DIRECTION('ref_axis',(-0.1864108996742,-0.213488518578295,0.958996156883801));
#96402=DIRECTION('center_axis',(0.981627005099017,-1.35927024749058E-16,
0.190809912898504));
#96403=DIRECTION('ref_axis',(-0.186578718977024,-0.209423271015703,0.959859508043743));
#96404=DIRECTION('center_axis',(0.,1.,0.));
#96405=DIRECTION('ref_axis',(1.,0.,0.));
#96406=DIRECTION('',(-0.190809912898503,1.155879430164E-14,0.981627005099017));
#96407=DIRECTION('center_axis',(0.,1.,0.));
#96408=DIRECTION('ref_axis',(-0.242534617261097,0.,0.970142752088585));
#96409=DIRECTION('center_axis',(0.,1.,0.));
#96410=DIRECTION('ref_axis',(-0.241509667213401,0.,0.970398413355294));
#96411=DIRECTION('center_axis',(-0.981627005099017,0.,-0.190809912898503));
#96412=DIRECTION('ref_axis',(-0.190809912898503,0.,0.981627005099017));
#96413=DIRECTION('center_axis',(-0.981627005099017,-1.49032924732936E-17,
-0.190809912898503));
#96414=DIRECTION('ref_axis',(-0.184940541908074,-0.246118695637908,0.951431859681103));
#96415=DIRECTION('center_axis',(-0.981627005099017,3.58496787124456E-17,
-0.190809912898503));
#96416=DIRECTION('ref_axis',(-0.185165818114719,-0.241421599051094,0.952590799511269));
#96417=DIRECTION('center_axis',(0.,-1.,0.));
#96418=DIRECTION('ref_axis',(0.,0.,-1.));
#96419=DIRECTION('',(-0.190809912898503,0.,0.981627005099017));
#96420=DIRECTION('center_axis',(0.,-1.,0.));
#96421=DIRECTION('ref_axis',(-0.275243638658276,0.,0.961374505267407));
#96422=DIRECTION('',(-0.190809912898503,0.,0.981627005099017));
#96423=DIRECTION('center_axis',(0.,-1.,0.));
#96424=DIRECTION('ref_axis',(-0.273550520375017,0.,0.961857636452795));
#96425=DIRECTION('center_axis',(0.981627005099017,0.,0.190809912898503));
#96426=DIRECTION('ref_axis',(0.,-1.,0.));
#96427=DIRECTION('',(-0.190809912898503,0.,0.981627005099017));
#96428=DIRECTION('center_axis',(0.981627005099017,-7.48461333200017E-17,
0.190809912898504));
#96429=DIRECTION('ref_axis',(-0.186380891213921,-0.214206930543801,0.958841777509359));
#96430=DIRECTION('center_axis',(0.981627005099017,-8.64054264038154E-17,
0.190809912898504));
#96431=DIRECTION('ref_axis',(-0.186550963960731,-0.210101290270208,0.959716721575755));
#96432=DIRECTION('center_axis',(0.,1.,0.));
#96433=DIRECTION('ref_axis',(1.,0.,0.));
#96434=DIRECTION('',(-0.190809912898503,0.,0.981627005099017));
#96435=DIRECTION('center_axis',(0.,1.,0.));
#96436=DIRECTION('ref_axis',(-0.306433322347889,0.,0.95189212569221));
#96437=DIRECTION('center_axis',(0.,1.,0.));
#96438=DIRECTION('ref_axis',(-0.304157214022129,0.,0.952621850031951));
#96439=DIRECTION('center_axis',(-0.981627005099017,0.,-0.190809912898503));
#96440=DIRECTION('ref_axis',(-0.190809912898503,0.,0.981627005099017));
#96441=DIRECTION('center_axis',(-0.981627005099017,-6.78043411373776E-17,
-0.190809912898503));
#96442=DIRECTION('ref_axis',(-0.184874781530203,-0.247471953044298,0.951093553553277));
#96443=DIRECTION('center_axis',(-0.981627005099017,-7.97057587953209E-17,
-0.190809912898503));
#96444=DIRECTION('ref_axis',(-0.185105036150056,-0.242698447428403,0.952278104971299));
#96445=DIRECTION('center_axis',(0.,-1.,0.));
#96446=DIRECTION('ref_axis',(0.,0.,-1.));
#96447=DIRECTION('',(-0.190809912898503,0.,0.981627005099017));
#96448=DIRECTION('center_axis',(0.,-1.,0.));
#96449=DIRECTION('ref_axis',(-0.339204610666547,0.,0.940712619295902));
#96450=DIRECTION('',(-0.190809912898503,0.,0.981627005099017));
#96451=DIRECTION('center_axis',(0.,-1.,0.));
#96452=DIRECTION('ref_axis',(-0.336249078397679,0.,0.941773092245001));
#96453=DIRECTION('center_axis',(0.981627005099017,0.,0.190809912898503));
#96454=DIRECTION('ref_axis',(0.,-1.,0.));
#96455=DIRECTION('',(-0.190809912898503,0.,0.981627005099017));
#96456=DIRECTION('center_axis',(0.981627005099017,-9.87985964490018E-17,
0.190809912898504));
#96457=DIRECTION('ref_axis',(-0.186311851707565,-0.215850244521505,0.958486601812099));
#96458=DIRECTION('center_axis',(0.981627005099017,-1.68062871373652E-16,
0.190809912898504));
#96459=DIRECTION('ref_axis',(-0.18648716372044,-0.211651234172008,0.959388499431263));
#96460=DIRECTION('center_axis',(0.,1.,0.));
#96461=DIRECTION('ref_axis',(1.,0.,0.));
#96462=DIRECTION('',(-0.190809912898503,0.,0.981627005099017));
#96463=DIRECTION('center_axis',(0.,1.,0.));
#96464=DIRECTION('ref_axis',(-0.369476474789942,0.,0.929240084465149));
#96465=DIRECTION('center_axis',(0.,1.,0.));
#96466=DIRECTION('ref_axis',(-0.365983690060656,0.,0.930621264859978));
#96467=DIRECTION('center_axis',(-0.981627005099017,0.,-0.190809912898503));
#96468=DIRECTION('ref_axis',(-0.190809912898503,0.,0.981627005099017));
#96469=DIRECTION('center_axis',(-0.981627005099017,-3.0734879996357E-17,
-0.190809912898503));
#96470=DIRECTION('ref_axis',(-0.184754752492854,-0.249921866464486,0.950476060768609));
#96471=DIRECTION('center_axis',(-0.981627005099017,-5.16917894804207E-17,
-0.190809912898503));
#96472=DIRECTION('ref_axis',(-0.184994228744489,-0.245007993611609,0.951708053132706));
#96473=DIRECTION('center_axis',(0.,-1.,0.));
#96474=DIRECTION('ref_axis',(0.,0.,-1.));
#96475=DIRECTION('',(-0.190809912898503,0.,0.981627005099017));
#96476=DIRECTION('center_axis',(0.,-1.,0.));
#96477=DIRECTION('ref_axis',(-0.402283914344989,0.,0.915514965611854));
#96478=DIRECTION('',(-0.190809912898503,0.,0.981627005099017));
#96479=DIRECTION('center_axis',(0.,-1.,0.));
#96480=DIRECTION('ref_axis',(-0.398102539409541,0.,0.917340922512277));
#96481=DIRECTION('center_axis',(0.981627005099017,0.,0.190809912898503));
#96482=DIRECTION('ref_axis',(0.,-1.,0.));
#96483=DIRECTION('',(-0.190809912898503,0.,0.981627005099017));
#96484=DIRECTION('center_axis',(0.981627005099017,-7.00780141118461E-17,
0.190809912898504));
#96485=DIRECTION('ref_axis',(-0.18620007176826,-0.218483413292492,0.957911546746127));
#96486=DIRECTION('center_axis',(0.981627005099017,-8.97524894262478E-17,
0.190809912898504));
#96487=DIRECTION('ref_axis',(-0.186384028329845,-0.214131945224895,0.958857916491146));
#96488=DIRECTION('center_axis',(0.,1.,0.));
#96489=DIRECTION('ref_axis',(1.,0.,0.));
#96490=DIRECTION('',(-0.190809912898503,0.,0.981627005099017));
#96491=DIRECTION('center_axis',(0.,1.,0.));
#96492=DIRECTION('ref_axis',(-0.431637009093733,0.,0.902047389210022));
#96493=DIRECTION('center_axis',(0.,1.,0.));
#96494=DIRECTION('ref_axis',(-0.426964190304545,0.,0.904268533234229));
#96495=DIRECTION('center_axis',(-0.981627005099017,0.,-0.190809912898503));
#96496=DIRECTION('ref_axis',(-0.190809912898503,0.,0.981627005099017));
#96497=DIRECTION('center_axis',(-0.981627005099017,-1.5819052248506E-17,
-0.190809912898503));
#96498=DIRECTION('ref_axis',(-0.184573801204179,-0.253567578221496,0.949545151735254));
#96499=DIRECTION('center_axis',(-0.981627005099017,-7.59286715101097E-18,
-0.190809912898503));
#96500=DIRECTION('ref_axis',(-0.184827508067632,-0.248439925893398,0.950850353885191));
#96501=DIRECTION('center_axis',(0.,-1.,0.));
#96502=DIRECTION('ref_axis',(0.,0.,-1.));
#96503=DIRECTION('',(-0.190809912898503,0.,0.981627005099017));
#96504=DIRECTION('center_axis',(0.,-1.,0.));
#96505=DIRECTION('ref_axis',(-0.399311414847207,0.,0.916815354350439));
#96506=DIRECTION('',(-0.190809912898503,0.,0.981627005099017));
#96507=DIRECTION('center_axis',(0.,-1.,0.));
#96508=DIRECTION('ref_axis',(-0.395301678561444,0.,0.918551350184901));
#96509=DIRECTION('center_axis',(0.981627005099017,0.,0.190809912898503));
#96510=DIRECTION('ref_axis',(0.,-1.,0.));
#96511=DIRECTION('',(-0.190809912898491,0.,0.981627005099019));
#96512=DIRECTION('center_axis',(0.981627005099017,7.78644601242735E-18,
0.190809912898503));
#96513=DIRECTION('ref_axis',(-0.188584680032072,-0.152276318355394,0.970179231547103));
#96514=DIRECTION('center_axis',(0.981627005099017,-1.00971550604529E-16,
0.190809912898504));
#96515=DIRECTION('ref_axis',(-0.188672933012422,-0.149243476974994,0.970633251505894));
#96516=DIRECTION('center_axis',(0.,1.,0.));
#96517=DIRECTION('ref_axis',(1.,0.,0.));
#96518=DIRECTION('',(-0.190809912898503,0.,0.981627005099017));
#96519=DIRECTION('center_axis',(0.,1.,0.));
#96520=DIRECTION('ref_axis',(-0.428810013970232,0.,0.903394693320062));
#96521=DIRECTION('center_axis',(0.,1.,0.));
#96522=DIRECTION('ref_axis',(-0.424297924716844,0.,0.90552265078295));
#96523=DIRECTION('center_axis',(-0.981627005099017,0.,-0.190809912898503));
#96524=DIRECTION('ref_axis',(-0.190809912898503,0.,0.981627005099017));
#96525=DIRECTION('center_axis',(-0.981627005099017,1.14688128801668E-16,
-0.190809912898504));
#96526=DIRECTION('ref_axis',(-0.187449845094609,-0.186839268163196,0.964341041046293));
#96527=DIRECTION('center_axis',(-0.981627005099017,1.25282307991681E-16,
-0.190809912898504));
#96528=DIRECTION('ref_axis',(-0.187585522425224,-0.183060998026701,0.965039036919193));
#96529=DIRECTION('center_axis',(0.,-1.,0.));
#96530=DIRECTION('ref_axis',(0.,0.,-1.));
#96531=DIRECTION('',(-0.190809912898503,0.,0.981627005099017));
#96532=DIRECTION('center_axis',(0.,-1.,0.));
#96533=DIRECTION('ref_axis',(-0.397312743751599,0.,0.91768326979006));
#96534=DIRECTION('',(-0.190809912898503,0.,0.981627005099017));
#96535=DIRECTION('center_axis',(0.,-1.,0.));
#96536=DIRECTION('ref_axis',(-0.393415793973014,0.,0.919360654505392));
#96537=DIRECTION('center_axis',(0.981627005099017,0.,0.190809912898503));
#96538=DIRECTION('ref_axis',(0.,-1.,0.));
#96539=DIRECTION('',(-0.190809912898503,0.,0.981627005099017));
#96540=DIRECTION('center_axis',(0.981627005099017,-6.42381796025256E-17,
0.190809912898504));
#96541=DIRECTION('ref_axis',(-0.190101847692576,-0.0860692234182736,0.97798434357818));
#96542=DIRECTION('center_axis',(0.981627005099017,-7.66635847182533E-17,
0.190809912898504));
#96543=DIRECTION('ref_axis',(-0.190129821407186,-0.0843550087249674,0.978128255145859));
#96544=DIRECTION('center_axis',(0.,1.,0.));
#96545=DIRECTION('ref_axis',(1.,0.,0.));
#96546=DIRECTION('',(-0.190809912898503,0.,0.981627005099017));
#96547=DIRECTION('center_axis',(0.,1.,0.));
#96548=DIRECTION('ref_axis',(-0.427044757829044,0.,0.904230487658281));
#96549=DIRECTION('center_axis',(0.,1.,0.));
#96550=DIRECTION('ref_axis',(-0.422631180074548,0.,0.906301763006558));
#96551=DIRECTION('center_axis',(-0.981627005099017,0.,-0.190809912898503));
#96552=DIRECTION('ref_axis',(-0.190809912898503,0.,0.981627005099017));
#96553=DIRECTION('center_axis',(-0.981627005099017,4.35023936833914E-17,
-0.190809912898504));
#96554=DIRECTION('ref_axis',(-0.189428539477533,-0.120110958104898,0.974520490382081));
#96555=DIRECTION('center_axis',(-0.981627005099017,1.48060909444714E-16,
-0.190809912898504));
#96556=DIRECTION('ref_axis',(-0.18948403646947,-0.117682070159998,0.974805996230067));
#96557=DIRECTION('center_axis',(0.981627005099017,0.,0.190809912898503));
#96558=DIRECTION('ref_axis',(0.,-1.,0.));
#96559=DIRECTION('',(-0.190809912898503,0.,0.981627005099017));
#96560=DIRECTION('center_axis',(0.981627005099017,-1.45995862733013E-17,
0.190809912898504));
#96561=DIRECTION('ref_axis',(-0.190772271534679,-0.0198621284811394,0.981433358035938));
#96562=DIRECTION('',(-0.190809912898492,0.,0.981627005099019));
#96563=DIRECTION('center_axis',(0.981627005099017,-5.60953058914049E-18,
0.190809912898504));
#96564=DIRECTION('ref_axis',(-0.190773756127288,-0.0194665404749907,0.981440995564696));
#96565=DIRECTION('center_axis',(0.,1.,0.));
#96566=DIRECTION('ref_axis',(1.,0.,0.));
#96567=DIRECTION('',(-0.190809912898503,0.,0.981627005099017));
#96568=DIRECTION('center_axis',(0.,1.,0.));
#96569=DIRECTION('ref_axis',(-0.426272800182109,0.,0.904594660510941));
#96570=DIRECTION('center_axis',(0.,1.,0.));
#96571=DIRECTION('ref_axis',(-0.42190185736574,0.,0.906641507295656));
#96572=DIRECTION('center_axis',(-0.981627005099017,0.,-0.190809912898503));
#96573=DIRECTION('ref_axis',(-0.190809912898503,0.,0.981627005099017));
#96574=DIRECTION('',(-0.190809912898503,0.,0.981627005099017));
#96575=DIRECTION('center_axis',(-0.981627005099017,2.17511968416957E-17,
-0.190809912898504));
#96576=DIRECTION('ref_axis',(-0.190537842747197,-0.053382648046619,0.980227332494241));
#96577=DIRECTION('center_axis',(-0.981627005099017,4.36589861183131E-17,
-0.190809912898504));
#96578=DIRECTION('ref_axis',(-0.190548742578238,-0.0523031422933503,0.980283406983967));
#96579=DIRECTION('center_axis',(0.,-1.,0.));
#96580=DIRECTION('ref_axis',(0.,0.,-1.));
#96581=DIRECTION('center_axis',(0.,-1.,0.));
#96582=DIRECTION('ref_axis',(-0.396208341225175,0.,0.918160634281167));
#96583=DIRECTION('center_axis',(0.,-1.,0.));
#96584=DIRECTION('ref_axis',(-0.392372817011327,0.,0.919806268988528));
#96585=DIRECTION('center_axis',(0.,-1.,0.));
#96586=DIRECTION('ref_axis',(0.,0.,-1.));
#96587=DIRECTION('',(-0.190809912898503,0.,0.981627005099017));
#96588=DIRECTION('center_axis',(0.,-1.,0.));
#96589=DIRECTION('ref_axis',(0.117062756021325,0.,0.993124519460018));
#96590=DIRECTION('',(-0.190809912898503,0.,0.981627005099017));
#96591=DIRECTION('center_axis',(0.,-1.,0.));
#96592=DIRECTION('ref_axis',(0.111009388690272,0.,0.993819357641323));
#96593=DIRECTION('center_axis',(0.981627005099017,0.,0.190809912898503));
#96594=DIRECTION('ref_axis',(0.,-1.,0.));
#96595=DIRECTION('',(-0.190809912898503,0.,0.981627005099017));
#96596=DIRECTION('center_axis',(0.981627005099017,-1.63768969384934E-17,
0.190809912898504));
#96597=DIRECTION('ref_axis',(-0.190770327966247,-0.0203684020382603,0.981423359293052));
#96598=DIRECTION('center_axis',(0.981627005099017,4.90596299631731E-18,
0.190809912898503));
#96599=DIRECTION('ref_axis',(-0.190771966490524,-0.0199424390734504,0.981431788727643));
#96600=DIRECTION('center_axis',(0.,1.,0.));
#96601=DIRECTION('ref_axis',(1.,0.,0.));
#96602=DIRECTION('',(-0.190809912898503,0.,0.981627005099017));
#96603=DIRECTION('center_axis',(0.,1.,0.));
#96604=DIRECTION('ref_axis',(0.0830891414914541,0.,0.996542118811951));
#96605=DIRECTION('center_axis',(0.,1.,0.));
#96606=DIRECTION('ref_axis',(0.0777343797762107,0.,0.996974105080372));
#96607=DIRECTION('center_axis',(-0.981627005099017,0.,-0.190809912898503));
#96608=DIRECTION('ref_axis',(-0.190809912898503,0.,0.981627005099017));
#96609=DIRECTION('center_axis',(-0.981627005099017,-6.01789072316824E-18,
-0.190809912898503));
#96610=DIRECTION('ref_axis',(-0.190533907263313,-0.0537670733624724,0.980207086285857));
#96611=DIRECTION('center_axis',(-0.981627005099017,7.69816334883557E-18,
-0.190809912898503));
#96612=DIRECTION('ref_axis',(-0.19054511820959,-0.0526645577892776,0.980264761316734));
#96613=DIRECTION('center_axis',(0.,-1.,0.));
#96614=DIRECTION('ref_axis',(0.,0.,-1.));
#96615=DIRECTION('',(-0.190809912898503,0.,0.981627005099017));
#96616=DIRECTION('center_axis',(0.,-1.,0.));
#96617=DIRECTION('ref_axis',(0.118808142662354,0.,0.99291722980172));
#96618=DIRECTION('',(-0.190809912898503,0.,0.981627005099017));
#96619=DIRECTION('center_axis',(0.,-1.,0.));
#96620=DIRECTION('ref_axis',(0.112654187705058,0.,0.993634255645664));
#96621=DIRECTION('center_axis',(0.981627005099017,0.,0.190809912898503));
#96622=DIRECTION('ref_axis',(0.,-1.,0.));
#96623=DIRECTION('',(-0.190809912898503,0.,0.981627005099017));
#96624=DIRECTION('center_axis',(0.981627005099017,-4.91306908154802E-17,
0.190809912898504));
#96625=DIRECTION('ref_axis',(-0.190065219745899,-0.0882630754991305,0.977795910068342));
#96626=DIRECTION('center_axis',(0.981627005099017,-1.96238519852693E-18,
0.190809912898503));
#96627=DIRECTION('ref_axis',(-0.190096099358061,-0.086417235984943,0.977954771108344));
#96628=DIRECTION('center_axis',(0.,1.,0.));
#96629=DIRECTION('ref_axis',(1.,0.,0.));
#96630=DIRECTION('',(-0.190809912898503,0.,0.981627005099017));
#96631=DIRECTION('center_axis',(0.,1.,0.));
#96632=DIRECTION('ref_axis',(0.0840360319589374,0.,0.996462716478944));
#96633=DIRECTION('center_axis',(0.,1.,0.));
#96634=DIRECTION('ref_axis',(0.0786270725857584,0.,0.996904099428122));
#96635=DIRECTION('center_axis',(-0.981627005099017,0.,-0.190809912898503));
#96636=DIRECTION('ref_axis',(-0.190809912898503,0.,0.981627005099017));
#96637=DIRECTION('center_axis',(-0.981627005099017,-2.00596357438942E-17,
-0.190809912898503));
#96638=DIRECTION('ref_axis',(-0.18940849856482,-0.120975915065594,0.974417389338605));
#96639=DIRECTION('center_axis',(-0.981627005099017,-6.54343884651024E-17,
-0.190809912898503));
#96640=DIRECTION('ref_axis',(-0.189465584281205,-0.118495255025902,0.97471106842455));
#96641=DIRECTION('center_axis',(0.,-1.,0.));
#96642=DIRECTION('ref_axis',(0.,0.,-1.));
#96643=DIRECTION('',(-0.190809912898503,0.,0.981627005099017));
#96644=DIRECTION('center_axis',(0.,-1.,0.));
#96645=DIRECTION('ref_axis',(0.121969536764593,0.,0.992533844310324));
#96646=DIRECTION('',(-0.190809912898503,0.,0.981627005099017));
#96647=DIRECTION('center_axis',(0.,-1.,0.));
#96648=DIRECTION('ref_axis',(0.115630671479797,0.,0.993292277133539));
#96649=DIRECTION('center_axis',(0.981627005099017,0.,0.190809912898503));
#96650=DIRECTION('ref_axis',(0.,-1.,0.));
#96651=DIRECTION('',(-0.190809912898492,0.,0.981627005099019));
#96652=DIRECTION('center_axis',(0.981627005099017,-3.68480181116102E-17,
0.190809912898503));
#96653=DIRECTION('ref_axis',(-0.188469081383788,-0.156157748959995,0.969584531024551));
#96654=DIRECTION('center_axis',(0.981627005099017,5.10220151617E-17,0.190809912898503));
#96655=DIRECTION('ref_axis',(-0.188566541370011,-0.152892032896403,0.970085916686021));
#96656=DIRECTION('center_axis',(0.,1.,0.));
#96657=DIRECTION('ref_axis',(1.,0.,0.));
#96658=DIRECTION('',(-0.190809912898503,0.,0.981627005099017));
#96659=DIRECTION('center_axis',(0.,1.,0.));
#96660=DIRECTION('ref_axis',(0.0862026472117667,0.,0.996277623764422));
#96661=DIRECTION('center_axis',(0.,1.,0.));
#96662=DIRECTION('ref_axis',(0.08066835433569,0.,0.996740997756574));
#96663=DIRECTION('center_axis',(-0.981627005099017,0.,-0.190809912898503));
#96664=DIRECTION('ref_axis',(-0.190809912898503,0.,0.981627005099017));
#96665=DIRECTION('center_axis',(-0.981627005099017,-2.80834900414518E-17,
-0.190809912898503));
#96666=DIRECTION('ref_axis',(-0.187400835323093,-0.18818475676861,0.964088908887633));
#96667=DIRECTION('center_axis',(-0.981627005099017,-3.46417350697601E-17,
-0.190809912898503));
#96668=DIRECTION('ref_axis',(-0.187540417568304,-0.184325952262508,0.96480699370435));
#96669=DIRECTION('center_axis',(0.,-1.,0.));
#96670=DIRECTION('ref_axis',(0.,0.,-1.));
#96671=DIRECTION('',(-0.190809912898503,0.,0.981627005099017));
#96672=DIRECTION('center_axis',(0.,-1.,0.));
#96673=DIRECTION('ref_axis',(0.0537998697696712,0.,0.998551738275372));
#96674=DIRECTION('',(-0.190809912898503,0.,0.981627005099017));
#96675=DIRECTION('center_axis',(0.,-1.,0.));
#96676=DIRECTION('ref_axis',(0.0488765616770635,0.,0.998804826639633));
#96677=DIRECTION('center_axis',(0.981627005099017,0.,0.190809912898503));
#96678=DIRECTION('ref_axis',(0.,-1.,0.));
#96679=DIRECTION('',(-0.190809912898503,0.,0.981627005099017));
#96680=DIRECTION('center_axis',(0.981627005099017,-1.65547203636389E-16,
0.190809912898504));
#96681=DIRECTION('ref_axis',(-0.188556864165061,-0.153219488090906,0.970036132030864));
#96682=DIRECTION('center_axis',(0.981627005099017,-3.78430184869551E-18,
0.190809912898503));
#96683=DIRECTION('ref_axis',(-0.188647292536475,-0.150131081303099,0.970501343350652));
#96684=DIRECTION('center_axis',(0.,1.,0.));
#96685=DIRECTION('ref_axis',(1.,0.,0.));
#96686=DIRECTION('',(-0.190809912898503,0.,0.981627005099017));
#96687=DIRECTION('center_axis',(0.,1.,0.));
#96688=DIRECTION('ref_axis',(0.0188803147301753,0.,0.999821750971487));
#96689=DIRECTION('center_axis',(0.,1.,0.));
#96690=DIRECTION('ref_axis',(0.0147187447196545,0.,0.999891673409614));
#96691=DIRECTION('center_axis',(-0.981627005099017,0.,-0.190809912898503));
#96692=DIRECTION('ref_axis',(-0.190809912898503,0.,0.981627005099017));
#96693=DIRECTION('center_axis',(-0.981627005099017,5.0468105524956E-17,
-0.190809912898504));
#96694=DIRECTION('ref_axis',(-0.187512071361184,-0.185116336980702,0.964661165838392));
#96695=DIRECTION('center_axis',(-0.981627005099017,3.35653208352217E-17,
-0.190809912898503));
#96696=DIRECTION('ref_axis',(-0.187642867377453,-0.181439595750803,0.965334049651287));
#96697=DIRECTION('center_axis',(0.,-1.,0.));
#96698=DIRECTION('ref_axis',(0.,0.,-1.));
#96699=DIRECTION('',(-0.190809912898503,0.,0.981627005099017));
#96700=DIRECTION('center_axis',(0.,-1.,0.));
#96701=DIRECTION('ref_axis',(-0.0134639270068732,0.,0.999909357226721));
#96702=DIRECTION('',(-0.190809912898503,0.,0.981627005099017));
#96703=DIRECTION('center_axis',(0.,-1.,0.));
#96704=DIRECTION('ref_axis',(-0.0170102071589267,0.,0.999855315959469));
#96705=DIRECTION('center_axis',(0.981627005099017,0.,0.190809912898503));
#96706=DIRECTION('ref_axis',(0.,-1.,0.));
#96707=DIRECTION('',(-0.190809912898503,0.,0.981627005099017));
#96708=DIRECTION('center_axis',(0.981627005099017,-1.149822511858E-16,0.190809912898504));
#96709=DIRECTION('ref_axis',(-0.188619449816688,-0.151088880707496,0.970358105689547));
#96710=DIRECTION('center_axis',(0.981627005099017,-6.99931092238096E-17,
0.190809912898504));
#96711=DIRECTION('ref_axis',(-0.188705019341167,-0.148125070547402,0.970798320533558));
#96712=DIRECTION('center_axis',(0.,1.,0.));
#96713=DIRECTION('ref_axis',(1.,0.,0.));
#96714=DIRECTION('',(-0.190809912898503,0.,0.981627005099017));
#96715=DIRECTION('center_axis',(0.,1.,0.));
#96716=DIRECTION('ref_axis',(-0.0475677174377644,0.,0.998868015434352));
#96717=DIRECTION('center_axis',(0.,1.,0.));
#96718=DIRECTION('ref_axis',(-0.0503925257524187,0.,0.998729489575777));
#96719=DIRECTION('center_axis',(-0.981627005099017,0.,-0.190809912898503));
#96720=DIRECTION('ref_axis',(-0.190809912898503,0.,0.981627005099017));
#96721=DIRECTION('center_axis',(-0.981627005099017,4.93043744111472E-17,
-0.190809912898503));
#96722=DIRECTION('ref_axis',(-0.187588768465847,-0.182969614535498,0.965055736267185));
#96723=DIRECTION('center_axis',(-0.981627005099017,-1.45871606611256E-17,
-0.190809912898503));
#96724=DIRECTION('ref_axis',(-0.187713666250361,-0.179416884227009,0.96569827645964));
#96725=DIRECTION('center_axis',(0.,-1.,0.));
#96726=DIRECTION('ref_axis',(0.,0.,-1.));
#96727=DIRECTION('',(-0.190809912898503,0.,0.981627005099017));
#96728=DIRECTION('center_axis',(0.,-1.,0.));
#96729=DIRECTION('ref_axis',(-0.0798606015889436,0.,0.996806041471385));
#96730=DIRECTION('',(-0.190809912898503,0.,0.981627005099017));
#96731=DIRECTION('center_axis',(0.,-1.,0.));
#96732=DIRECTION('ref_axis',(-0.0820652483437025,0.,0.996626958803687));
#96733=DIRECTION('center_axis',(0.981627005099017,0.,0.190809912898503));
#96734=DIRECTION('ref_axis',(0.,-1.,0.));
#96735=DIRECTION('',(-0.190809912898503,0.,0.981627005099017));
#96736=DIRECTION('center_axis',(0.981627005099017,-1.31646357735773E-16,
0.190809912898504));
#96737=DIRECTION('ref_axis',(-0.188660498233732,-0.149674608010496,0.97056928043448));
#96738=DIRECTION('center_axis',(0.981627005099017,-8.68277734583866E-17,
0.190809912898504));
#96739=DIRECTION('ref_axis',(-0.188742950996444,-0.146791679350195,0.97099346100924));
#96740=DIRECTION('center_axis',(0.,1.,0.));
#96741=DIRECTION('ref_axis',(1.,0.,0.));
#96742=DIRECTION('',(-0.190809912898503,0.,0.981627005099017));
#96743=DIRECTION('center_axis',(0.,1.,0.));
#96744=DIRECTION('ref_axis',(-0.113172347138354,0.,0.993575371999123));
#96745=DIRECTION('center_axis',(0.,1.,0.));
#96746=DIRECTION('ref_axis',(-0.114693920685021,0.,0.993400878073851));
#96747=DIRECTION('center_axis',(-0.981627005099017,0.,-0.190809912898503));
#96748=DIRECTION('ref_axis',(-0.190809912898503,0.,0.981627005099017));
#96749=DIRECTION('center_axis',(-0.981627005099017,1.12151063898178E-17,
-0.190809912898503));
#96750=DIRECTION('ref_axis',(-0.18763525530524,-0.181655685256397,0.965294889130035));
#96751=DIRECTION('center_axis',(-0.981627005099017,3.59658141965232E-17,
-0.190809912898503));
#96752=DIRECTION('ref_axis',(-0.187756641804466,-0.178177504116097,0.965919365415803));
#96753=DIRECTION('center_axis',(0.,-1.,0.));
#96754=DIRECTION('ref_axis',(0.,0.,-1.));
#96755=DIRECTION('',(-0.190809912898503,0.,0.981627005099017));
#96756=DIRECTION('center_axis',(0.,-1.,0.));
#96757=DIRECTION('ref_axis',(-0.145415214742479,0.,0.989370716830349));
#96758=DIRECTION('',(-0.190809912898503,-1.310547882E-14,0.981627005099017));
#96759=DIRECTION('center_axis',(0.,-1.,0.));
#96760=DIRECTION('ref_axis',(-0.146311652535326,0.,0.989238545717049));
#96761=DIRECTION('center_axis',(0.981627005099017,0.,0.190809912898503));
#96762=DIRECTION('ref_axis',(0.,-1.,0.));
#96763=DIRECTION('',(-0.190809912898503,1.170107715525E-14,0.981627005099017));
#96764=DIRECTION('center_axis',(0.981627005099017,-8.19165637861642E-17,
0.190809912898504));
#96765=DIRECTION('ref_axis',(-0.18868224637733,-0.148919733508905,0.970681164375636));
#96766=DIRECTION('center_axis',(0.981627005099017,-4.65763827833953E-17,
0.190809912898504));
#96767=DIRECTION('ref_axis',(-0.188763070362452,-0.146079384436406,0.971096965657921));
#96768=DIRECTION('center_axis',(0.,1.,0.));
#96769=DIRECTION('ref_axis',(1.,0.,0.));
#96770=DIRECTION('',(-0.190809912898503,-1.171213937656E-14,0.981627005099017));
#96771=DIRECTION('center_axis',(0.,1.,0.));
#96772=DIRECTION('ref_axis',(-0.177952104583987,0.,0.984039149868607));
#96773=DIRECTION('center_axis',(0.,1.,0.));
#96774=DIRECTION('ref_axis',(-0.178202543505702,0.,0.983993827972563));
#96775=DIRECTION('center_axis',(-0.981627005099017,0.,-0.190809912898503));
#96776=DIRECTION('ref_axis',(-0.190809912898503,0.,0.981627005099017));
#96777=DIRECTION('center_axis',(-0.981627005099017,5.2030565722685E-17,
-0.190809912898504));
#96778=DIRECTION('ref_axis',(-0.187654009224651,-0.181122823233507,0.965391369199994));
#96779=DIRECTION('center_axis',(-0.981627005099017,1.85967954159957E-16,
-0.190809912898504));
#96780=DIRECTION('ref_axis',(-0.187773992817113,-0.177674584225901,0.966008628192146));
#96781=DIRECTION('center_axis',(0.,-1.,0.));
#96782=DIRECTION('ref_axis',(0.,0.,-1.));
#96783=DIRECTION('',(-0.190809912898503,0.,0.981627005099017));
#96784=DIRECTION('center_axis',(0.,-1.,0.));
#96785=DIRECTION('ref_axis',(-0.210140930284338,0.,0.977671104932141));
#96786=DIRECTION('',(-0.190809912898503,0.,0.981627005099017));
#96787=DIRECTION('center_axis',(0.,-1.,0.));
#96788=DIRECTION('ref_axis',(-0.209761566952143,0.,0.977752568408686));
#96789=DIRECTION('center_axis',(0.981627005099017,0.,0.190809912898503));
#96790=DIRECTION('ref_axis',(0.,-1.,0.));
#96791=DIRECTION('',(-0.190809912898503,0.,0.981627005099017));
#96792=DIRECTION('center_axis',(0.981627005099017,-9.29311674338004E-17,
0.190809912898504));
#96793=DIRECTION('ref_axis',(-0.188685828350842,-0.1487950281,0.970699591939894));
#96794=DIRECTION('center_axis',(0.981627005099017,3.21932427037243E-17,
0.190809912898503));
#96795=DIRECTION('ref_axis',(-0.188766385571152,-0.145961673738203,0.971114020843045));
#96796=DIRECTION('center_axis',(0.,1.,0.));
#96797=DIRECTION('ref_axis',(1.,0.,0.));
#96798=DIRECTION('',(-0.190809912898503,0.,0.981627005099017));
#96799=DIRECTION('center_axis',(0.,1.,0.));
#96800=DIRECTION('ref_axis',(-0.241914422980073,0.,0.970297589378753));
#96801=DIRECTION('center_axis',(0.,1.,0.));
#96802=DIRECTION('ref_axis',(-0.240925262116702,0.,0.970543671389391));
#96803=DIRECTION('center_axis',(-0.981627005099017,0.,-0.190809912898503));
#96804=DIRECTION('ref_axis',(-0.190809912898503,0.,0.981627005099017));
#96805=DIRECTION('center_axis',(-0.981627005099017,-7.07906392481446E-17,
-0.190809912898503));
#96806=DIRECTION('ref_axis',(-0.187645999032811,-0.181350617838393,0.96535016054104));
#96807=DIRECTION('center_axis',(-0.981627005099017,2.22268008017162E-16,
-0.190809912898504));
#96808=DIRECTION('ref_axis',(-0.187766580876715,-0.177889599300794,0.965970497254689));
#96809=DIRECTION('center_axis',(0.,-1.,0.));
#96810=DIRECTION('ref_axis',(0.,0.,-1.));
#96811=DIRECTION('',(-0.190809912898503,0.,0.981627005099017));
#96812=DIRECTION('center_axis',(0.,-1.,0.));
#96813=DIRECTION('ref_axis',(-0.274039908751656,0.,0.961718320721501));
#96814=DIRECTION('',(-0.190809912898503,0.,0.981627005099017));
#96815=DIRECTION('center_axis',(0.,-1.,0.));
#96816=DIRECTION('ref_axis',(-0.272416986488902,0.,0.962179289671268));
#96817=DIRECTION('center_axis',(0.981627005099017,0.,0.190809912898503));
#96818=DIRECTION('ref_axis',(0.,-1.,0.));
#96819=DIRECTION('',(-0.190809912898503,0.,0.981627005099017));
#96820=DIRECTION('center_axis',(0.981627005099017,5.61345999900013E-17,
0.190809912898503));
#96821=DIRECTION('ref_axis',(-0.18867142759988,-0.149295739469903,0.97062550686841));
#96822=DIRECTION('center_axis',(0.981627005099017,-7.56047481033385E-17,
0.190809912898504));
#96823=DIRECTION('ref_axis',(-0.18875305987975,-0.146434232612596,0.971045466445929));
#96824=DIRECTION('center_axis',(0.,1.,0.));
#96825=DIRECTION('ref_axis',(1.,0.,0.));
#96826=DIRECTION('',(-0.190809912898503,0.,0.981627005099017));
#96827=DIRECTION('center_axis',(0.,1.,0.));
#96828=DIRECTION('ref_axis',(-0.305056130431757,0.,0.952334372626549));
#96829=DIRECTION('center_axis',(0.,1.,0.));
#96830=DIRECTION('ref_axis',(-0.30285914535448,0.,0.953035328870422));
#96831=DIRECTION('center_axis',(-0.981627005099017,0.,-0.190809912898503));
#96832=DIRECTION('ref_axis',(-0.190809912898503,0.,0.981627005099017));
#96833=DIRECTION('center_axis',(-0.981627005099017,9.04057881831701E-17,
-0.190809912898504));
#96834=DIRECTION('ref_axis',(-0.187610813066133,-0.18234775487471,0.965169145338172));
#96835=DIRECTION('center_axis',(-0.981627005099017,7.24597807230189E-17,
-0.190809912898504));
#96836=DIRECTION('ref_axis',(-0.187734039758534,-0.178830434947303,0.965803088549886));
#96837=DIRECTION('center_axis',(0.,-1.,0.));
#96838=DIRECTION('ref_axis',(0.,0.,-1.));
#96839=DIRECTION('',(-0.190809912898503,0.,0.981627005099017));
#96840=DIRECTION('center_axis',(0.,-1.,0.));
#96841=DIRECTION('ref_axis',(-0.337103451036581,0.,0.941467611391506));
#96842=DIRECTION('',(-0.190809912898503,0.,0.981627005099017));
#96843=DIRECTION('center_axis',(0.,-1.,0.));
#96844=DIRECTION('ref_axis',(-0.334269881053193,0.,0.942477398466766));
#96845=DIRECTION('center_axis',(0.981627005099017,0.,0.190809912898503));
#96846=DIRECTION('ref_axis',(0.,-1.,0.));
#96847=DIRECTION('',(-0.190809912898503,0.,0.981627005099017));
#96848=DIRECTION('center_axis',(0.981627005099017,-1.40598002638964E-16,
0.190809912898504));
#96849=DIRECTION('ref_axis',(-0.188638300882477,-0.150441079515,0.9704550855318));
#96850=DIRECTION('center_axis',(0.981627005099017,-8.03778950047904E-17,
0.190809912898504));
#96851=DIRECTION('ref_axis',(-0.188722432166707,-0.147514496544108,0.970887901308087));
#96852=DIRECTION('center_axis',(0.,1.,0.));
#96853=DIRECTION('ref_axis',(1.,0.,0.));
#96854=DIRECTION('',(-0.190809912898503,0.,0.981627005099017));
#96855=DIRECTION('center_axis',(0.,1.,0.));
#96856=DIRECTION('ref_axis',(-0.367363241275728,0.,0.930077549970641));
#96857=DIRECTION('center_axis',(0.,1.,0.));
#96858=DIRECTION('ref_axis',(-0.363991277767333,0.,0.931402356508348));
#96859=DIRECTION('center_axis',(-0.981627005099017,0.,-0.190809912898503));
#96860=DIRECTION('ref_axis',(-0.190809912898503,0.,0.981627005099017));
#96861=DIRECTION('center_axis',(-0.981627005099017,1.15255799986339E-17,
-0.190809912898503));
#96862=DIRECTION('ref_axis',(-0.187546605187899,-0.18415295423699,0.964838826088733));
#96863=DIRECTION('center_axis',(-0.981627005099017,1.69844451149954E-16,
-0.190809912898504));
#96864=DIRECTION('ref_axis',(-0.187674729274892,-0.180532205819094,0.965497964085729));
#96865=DIRECTION('center_axis',(0.,-1.,0.));
#96866=DIRECTION('ref_axis',(0.,0.,-1.));
#96867=DIRECTION('',(-0.190809912898503,0.,0.981627005099017));
#96868=DIRECTION('center_axis',(0.,-1.,0.));
#96869=DIRECTION('ref_axis',(-0.335690934126128,0.,0.941972184698427));
#96870=DIRECTION('',(-0.190809912898503,0.,0.981627005099017));
#96871=DIRECTION('center_axis',(0.,-1.,0.));
#96872=DIRECTION('ref_axis',(-0.332937485198635,0.,0.94294890155809));
#96873=DIRECTION('center_axis',(0.981627005099017,0.,0.190809912898503));
#96874=DIRECTION('ref_axis',(0.,-1.,0.));
#96875=DIRECTION('',(-0.190809912898503,0.,0.981627005099017));
#96876=DIRECTION('center_axis',(0.981627005099017,5.69991902590395E-18,
0.190809912898503));
#96877=DIRECTION('ref_axis',(-0.190118842925705,-0.0850319145084515,0.978071776036717));
#96878=DIRECTION('center_axis',(0.981627005099017,-3.65354068203592E-17,
0.190809912898504));
#96879=DIRECTION('ref_axis',(-0.190145515174684,-0.0833777589162615,0.978208992177569));
#96880=DIRECTION('center_axis',(0.,1.,0.));
#96881=DIRECTION('ref_axis',(1.,0.,0.));
#96882=DIRECTION('',(-0.190809912898503,0.,0.981627005099017));
#96883=DIRECTION('center_axis',(0.,1.,0.));
#96884=DIRECTION('ref_axis',(-0.366043901565332,0.,0.930597583344611));
#96885=DIRECTION('center_axis',(0.,1.,0.));
#96886=DIRECTION('ref_axis',(-0.362745971285859,0.,0.93188806211684));
#96887=DIRECTION('center_axis',(-0.981627005099017,0.,-0.190809912898503));
#96888=DIRECTION('ref_axis',(-0.190809912898503,0.,0.981627005099017));
#96889=DIRECTION('center_axis',(-0.981627005099017,5.76278999931694E-17,
-0.190809912898504));
#96890=DIRECTION('ref_axis',(-0.189468115451484,-0.118384042009503,0.974724090101786));
#96891=DIRECTION('center_axis',(-0.981627005099017,3.69227067717291E-18,
-0.190809912898503));
#96892=DIRECTION('ref_axis',(-0.189520538352024,-0.116056418026502,0.974993781199458));
#96893=DIRECTION('center_axis',(0.,-1.,0.));
#96894=DIRECTION('ref_axis',(0.,0.,-1.));
#96895=DIRECTION('',(-0.190809912898503,0.,0.981627005099017));
#96896=DIRECTION('center_axis',(0.,-1.,0.));
#96897=DIRECTION('ref_axis',(-0.334910516764006,0.,0.942249938052992));
#96898=DIRECTION('',(-0.190809912898503,0.,0.981627005099017));
#96899=DIRECTION('center_axis',(0.,-1.,0.));
#96900=DIRECTION('ref_axis',(-0.33220069566279,0.,0.94320872440895));
#96901=DIRECTION('center_axis',(0.981627005099017,0.,0.190809912898503));
#96902=DIRECTION('ref_axis',(0.,-1.,0.));
#96903=DIRECTION('',(-0.190809912898503,0.,0.981627005099017));
#96904=DIRECTION('center_axis',(0.981627005099017,-7.5998920345386E-18,
0.190809912898504));
#96905=DIRECTION('ref_axis',(-0.190773173463789,-0.0196227495019493,0.98143799803581));
#96906=DIRECTION('center_axis',(0.981627005099017,-9.59054429034431E-18,
0.190809912898504));
#96907=DIRECTION('ref_axis',(-0.190774589101592,-0.0192410212883709,0.981445280824611));
#96908=DIRECTION('center_axis',(0.,1.,0.));
#96909=DIRECTION('ref_axis',(1.,0.,0.));
#96910=DIRECTION('',(-0.190809912898503,0.,0.981627005099017));
#96911=DIRECTION('center_axis',(0.,1.,0.));
#96912=DIRECTION('ref_axis',(-0.365466999719524,0.,0.930824297123796));
#96913=DIRECTION('center_axis',(0.,1.,0.));
#96914=DIRECTION('ref_axis',(-0.362201106022701,0.,0.932099972532953));
#96915=DIRECTION('center_axis',(-0.981627005099017,0.,-0.190809912898503));
#96916=DIRECTION('ref_axis',(-0.190809912898503,0.,0.981627005099017));
#96917=DIRECTION('center_axis',(-0.981627005099017,-1.34465099984062E-17,
-0.190809912898503));
#96918=DIRECTION('ref_axis',(-0.190545615363852,-0.0526151297819897,0.980267318940928));
#96919=DIRECTION('center_axis',(-0.981627005099017,-1.29229473701052E-17,
-0.190809912898503));
#96920=DIRECTION('ref_axis',(-0.1905559130945,-0.0515806302340213,0.980320295908119));
#96921=DIRECTION('center_axis',(0.,-1.,0.));
#96922=DIRECTION('ref_axis',(0.,0.,-1.));
#96923=DIRECTION('',(-0.190809912898503,0.,0.981627005099017));
#96924=DIRECTION('center_axis',(0.,-1.,0.));
#96925=DIRECTION('ref_axis',(0.0499889785862565,0.,0.998749769471765));
#96926=DIRECTION('',(-0.190809912898503,0.,0.981627005099017));
#96927=DIRECTION('center_axis',(0.,-1.,0.));
#96928=DIRECTION('ref_axis',(0.0452862925115339,0.,0.998974049568136));
#96929=DIRECTION('center_axis',(0.981627005099017,0.,0.190809912898503));
#96930=DIRECTION('ref_axis',(0.,-1.,0.));
#96931=DIRECTION('',(-0.190809912898503,0.,0.981627005099017));
#96932=DIRECTION('center_axis',(0.981627005099017,-5.41970011904846E-18,
0.190809912898504));
#96933=DIRECTION('ref_axis',(-0.190771803757425,-0.0199851506205497,0.9814309515426));
#96934=DIRECTION('center_axis',(0.981627005099017,5.20341504195632E-18,
0.190809912898503));
#96935=DIRECTION('ref_axis',(-0.190773324732523,-0.019582314952569,0.981438776242104));
#96936=DIRECTION('center_axis',(0.,1.,0.));
#96937=DIRECTION('ref_axis',(1.,0.,0.));
#96938=DIRECTION('',(-0.190809912898503,0.,0.981627005099017));
#96939=DIRECTION('center_axis',(0.,1.,0.));
#96940=DIRECTION('ref_axis',(0.0165392312897058,0.,0.999863217559455));
#96941=DIRECTION('center_axis',(0.,1.,0.));
#96942=DIRECTION('ref_axis',(0.0125120179178436,0.,0.999921721640061));
#96943=DIRECTION('center_axis',(-0.981627005099017,0.,-0.190809912898503));
#96944=DIRECTION('ref_axis',(-0.190809912898503,0.,0.981627005099017));
#96945=DIRECTION('center_axis',(-0.981627005099017,2.91162147259362E-17,
-0.190809912898504));
#96946=DIRECTION('ref_axis',(-0.190542840881032,-0.0528903819944982,0.980253045535418));
#96947=DIRECTION('center_axis',(-0.981627005099017,2.42416206032157E-17,
-0.190809912898504));
#96948=DIRECTION('ref_axis',(-0.190553351649904,-0.0518398845002214,0.98030711848379));
#96949=DIRECTION('center_axis',(0.,-1.,0.));
#96950=DIRECTION('ref_axis',(0.,0.,-1.));
#96951=DIRECTION('',(-0.190809912898503,0.,0.981627005099017));
#96952=DIRECTION('center_axis',(0.,-1.,0.));
#96953=DIRECTION('ref_axis',(0.0513446549634899,0.,0.998680993314021));
#96954=DIRECTION('',(-0.190809912898503,0.,0.981627005099017));
#96955=DIRECTION('center_axis',(0.,-1.,0.));
#96956=DIRECTION('ref_axis',(0.0465642295325163,0.,0.99891529797478));
#96957=DIRECTION('center_axis',(0.981627005099017,0.,0.190809912898503));
#96958=DIRECTION('ref_axis',(0.,-1.,0.));
#96959=DIRECTION('',(-0.190809912898503,0.,0.981627005099017));
#96960=DIRECTION('center_axis',(0.981627005099017,-6.50364014285815E-17,
0.190809912898504));
#96961=DIRECTION('ref_axis',(-0.190093032704192,-0.086602319355716,0.977938994620592));
#96962=DIRECTION('center_axis',(0.981627005099017,-4.91959240330416E-17,
0.190809912898504));
#96963=DIRECTION('ref_axis',(-0.19012169317225,-0.0848566981278218,0.97808643921085));
#96964=DIRECTION('center_axis',(0.,1.,0.));
#96965=DIRECTION('ref_axis',(1.,0.,0.));
#96966=DIRECTION('',(-0.190809912898503,0.,0.981627005099017));
#96967=DIRECTION('center_axis',(0.,1.,0.));
#96968=DIRECTION('ref_axis',(0.0172512508492204,0.,0.99985118609928));
#96969=DIRECTION('center_axis',(0.,1.,0.));
#96970=DIRECTION('ref_axis',(0.0131834739886762,0.,0.999913094230489));
#96971=DIRECTION('center_axis',(-0.981627005099017,0.,-0.190809912898503));
#96972=DIRECTION('ref_axis',(-0.190809912898503,0.,0.981627005099017));
#96973=DIRECTION('center_axis',(-0.981627005099017,3.88216196345816E-18,
-0.190809912898503));
#96974=DIRECTION('ref_axis',(-0.189453989330261,-0.119003359487598,0.974651417870776));
#96975=DIRECTION('center_axis',(-0.981627005099017,1.11884402784072E-16,
-0.190809912898504));
#96976=DIRECTION('ref_axis',(-0.189507499835796,-0.116639740125495,0.974926704183162));
#96977=DIRECTION('center_axis',(0.,-1.,0.));
#96978=DIRECTION('ref_axis',(0.,0.,-1.));
#96979=DIRECTION('',(-0.190809912898503,0.,0.981627005099017));
#96980=DIRECTION('center_axis',(0.,-1.,0.));
#96981=DIRECTION('ref_axis',(-0.0152323034392406,0.,0.999883981735849));
#96982=DIRECTION('',(-0.190809912898513,0.,0.981627005099015));
#96983=DIRECTION('center_axis',(0.,-1.,0.));
#96984=DIRECTION('ref_axis',(-0.0186761357819992,0.,0.999825585765964));
#96985=DIRECTION('center_axis',(0.981627005099017,0.,0.190809912898503));
#96986=DIRECTION('ref_axis',(0.,-1.,0.));
#96987=DIRECTION('',(-0.190809912898503,0.,0.981627005099017));
#96988=DIRECTION('center_axis',(0.981627005099017,-2.68291919433533E-17,
0.190809912898504));
#96989=DIRECTION('ref_axis',(-0.19011286766609,-0.0853980630086089,0.978041036144268));
#96990=DIRECTION('center_axis',(0.981627005099017,-6.44673374429825E-17,
0.190809912898504));
#96991=DIRECTION('ref_axis',(-0.190139994095334,-0.0837228659615728,0.978180588828365));
#96992=DIRECTION('center_axis',(0.,1.,0.));
#96993=DIRECTION('ref_axis',(1.,0.,0.));
#96994=DIRECTION('',(-0.190809912898492,0.,0.981627005099019));
#96995=DIRECTION('center_axis',(0.,1.,0.));
#96996=DIRECTION('ref_axis',(-0.0486734108678654,0.,0.998814747125055));
#96997=DIRECTION('center_axis',(0.,1.,0.));
#96998=DIRECTION('ref_axis',(-0.0514348329990322,0.,0.998676352956433));
#96999=DIRECTION('center_axis',(-0.981627005099017,0.,-0.190809912898503));
#97000=DIRECTION('ref_axis',(-0.190809912898503,0.,0.981627005099017));
#97001=DIRECTION('center_axis',(-0.981627005099017,-1.89632209273643E-17,
-0.190809912898503));
#97002=DIRECTION('ref_axis',(-0.18948536451151,-0.117623323629904,0.97481282837999));
#97003=DIRECTION('center_axis',(-0.981627005099017,4.37614819833767E-17,
-0.190809912898504));
#97004=DIRECTION('ref_axis',(-0.189536473917127,-0.115339425574496,0.975075762165796));
#97005=DIRECTION('center_axis',(0.,-1.,0.));
#97006=DIRECTION('ref_axis',(0.,0.,-1.));
#97007=DIRECTION('',(-0.190809912898503,0.,0.981627005099017));
#97008=DIRECTION('center_axis',(0.,-1.,0.));
#97009=DIRECTION('ref_axis',(-0.0809598914546659,0.,0.996717360125552));
#97010=DIRECTION('',(-0.190809912898503,0.,0.981627005099017));
#97011=DIRECTION('center_axis',(0.,-1.,0.));
#97012=DIRECTION('ref_axis',(-0.0831011195422453,0.,0.996541120040124));
#97013=DIRECTION('center_axis',(0.981627005099017,0.,0.190809912898503));
#97014=DIRECTION('ref_axis',(0.,-1.,0.));
#97015=DIRECTION('',(-0.190809912898503,0.,0.981627005099017));
#97016=DIRECTION('center_axis',(0.981627005099017,-6.39425166145185E-17,
0.190809912898504));
#97017=DIRECTION('ref_axis',(-0.190125879388814,-0.0845986914841974,0.978107975320614));
#97018=DIRECTION('center_axis',(0.981627005099017,-3.79871508880441E-17,
0.190809912898504));
#97019=DIRECTION('ref_axis',(-0.190152021521919,-0.0829692100674824,0.97824246426533));
#97020=DIRECTION('center_axis',(0.,1.,0.));
#97021=DIRECTION('ref_axis',(1.,0.,0.));
#97022=DIRECTION('',(-0.190809912898503,0.,0.981627005099017));
#97023=DIRECTION('center_axis',(0.,1.,0.));
#97024=DIRECTION('ref_axis',(-0.113767879747049,0.,0.993507357566043));
#97025=DIRECTION('center_axis',(0.,1.,0.));
#97026=DIRECTION('ref_axis',(-0.115255452371297,0.,0.993335885135883));
#97027=DIRECTION('center_axis',(-0.981627005099017,0.,-0.190809912898503));
#97028=DIRECTION('ref_axis',(-0.190809912898503,0.,0.981627005099017));
#97029=DIRECTION('center_axis',(-0.981627005099017,2.24302127796356E-17,
-0.190809912898503));
#97030=DIRECTION('ref_axis',(-0.189504385020733,-0.116778654807704,0.974910679928791));
#97031=DIRECTION('center_axis',(-0.981627005099017,-3.59658141965232E-17,
-0.190809912898503));
#97032=DIRECTION('ref_axis',(-0.189554064615674,-0.114542681217505,0.975166258013054));
#97033=DIRECTION('center_axis',(0.,-1.,0.));
#97034=DIRECTION('ref_axis',(0.,0.,-1.));
#97035=DIRECTION('',(-0.190809912898503,0.,0.981627005099017));
#97036=DIRECTION('center_axis',(0.,-1.,0.));
#97037=DIRECTION('ref_axis',(-0.145862172035669,0.,0.989304921027403));
#97038=DIRECTION('',(-0.190809912898503,0.,0.981627005099017));
#97039=DIRECTION('center_axis',(0.,-1.,0.));
#97040=DIRECTION('ref_axis',(-0.146732928854605,0.,0.989176145885933));
#97041=DIRECTION('center_axis',(0.981627005099017,0.,0.190809912898503));
#97042=DIRECTION('ref_axis',(0.,-1.,0.));
#97043=DIRECTION('',(-0.190809912898503,0.,0.981627005099017));
#97044=DIRECTION('center_axis',(0.981627005099017,-2.42026211186394E-17,
0.190809912898504));
#97045=DIRECTION('ref_axis',(-0.190132774005443,-0.0841720232876468,0.978143444871282));
#97046=DIRECTION('center_axis',(0.981627005099017,-3.22451880808121E-17,
0.190809912898504));
#97047=DIRECTION('ref_axis',(-0.190158401673233,-0.0825666085944808,0.978275287134602));
#97048=DIRECTION('center_axis',(0.,1.,0.));
#97049=DIRECTION('ref_axis',(1.,0.,0.));
#97050=DIRECTION('',(-0.190809912898503,0.,0.981627005099017));
#97051=DIRECTION('center_axis',(0.,1.,0.));
#97052=DIRECTION('ref_axis',(-0.178050117193582,0.,0.984021420380345));
#97053=DIRECTION('center_axis',(0.,1.,0.));
#97054=DIRECTION('ref_axis',(-0.178294982707409,0.,0.983977082630162));
#97055=DIRECTION('center_axis',(-0.981627005099017,0.,-0.190809912898503));
#97056=DIRECTION('ref_axis',(-0.190809912898503,0.,0.981627005099017));
#97057=DIRECTION('center_axis',(-0.981627005099017,-5.94635036830686E-17,
-0.190809912898503));
#97058=DIRECTION('ref_axis',(-0.189512059149486,-0.116436100650099,0.974950159701675));
#97059=DIRECTION('center_axis',(-0.981627005099017,-2.86104544861472E-17,
-0.190809912898503));
#97060=DIRECTION('ref_axis',(-0.189561167388284,-0.114219375573802,0.975202798428061));
#97061=DIRECTION('center_axis',(0.,-1.,0.));
#97062=DIRECTION('ref_axis',(0.,0.,-1.));
#97063=DIRECTION('',(-0.190809912898503,0.,0.981627005099017));
#97064=DIRECTION('center_axis',(0.,-1.,0.));
#97065=DIRECTION('ref_axis',(-0.209951794403501,0.,0.977711738717885));
#97066=DIRECTION('',(-0.190809912898503,0.,0.981627005099017));
#97067=DIRECTION('center_axis',(0.,-1.,0.));
#97068=DIRECTION('ref_axis',(-0.209583254257496,0.,0.977790805609685));
#97069=DIRECTION('center_axis',(0.981627005099017,0.,0.190809912898503));
#97070=DIRECTION('ref_axis',(0.,-1.,0.));
#97071=DIRECTION('',(-0.190809912898503,0.,0.981627005099017));
#97072=DIRECTION('center_axis',(0.981627005099017,1.85862334867601E-17,
0.190809912898503));
#97073=DIRECTION('ref_axis',(-0.190133909618249,-0.0841015376217537,0.978149287063553));
#97074=DIRECTION('center_axis',(0.981627005099017,-1.60966213518622E-17,
0.190809912898503));
#97075=DIRECTION('ref_axis',(-0.190159453020121,-0.0825000764607267,0.978280695818466));
#97076=DIRECTION('center_axis',(0.,1.,0.));
#97077=DIRECTION('ref_axis',(1.,0.,0.));
#97078=DIRECTION('',(-0.190809912898503,0.,0.981627005099017));
#97079=DIRECTION('center_axis',(0.,1.,0.));
#97080=DIRECTION('ref_axis',(-0.2415273311514,0.,0.970394017039925));
#97081=DIRECTION('center_axis',(0.,1.,0.));
#97082=DIRECTION('ref_axis',(-0.240560091673225,0.,0.970634247435237));
#97083=DIRECTION('center_axis',(-0.981627005099017,0.,-0.190809912898503));
#97084=DIRECTION('ref_axis',(-0.190809912898503,0.,0.981627005099017));
#97085=DIRECTION('center_axis',(-0.981627005099017,1.15500516668025E-16,
-0.190809912898504));
#97086=DIRECTION('ref_axis',(-0.189508781312522,-0.116582540038997,0.974933296776502));
#97087=DIRECTION('center_axis',(-0.981627005099017,8.60392289098693E-17,
-0.190809912898504));
#97088=DIRECTION('ref_axis',(-0.189558133204824,-0.114357599550504,0.975187188985247));
#97089=DIRECTION('center_axis',(0.,-1.,0.));
#97090=DIRECTION('ref_axis',(0.,0.,-1.));
#97091=DIRECTION('',(-0.190809912898503,0.,0.981627005099017));
#97092=DIRECTION('center_axis',(0.,-1.,0.));
#97093=DIRECTION('ref_axis',(-0.273230835267042,0.,0.961948496884981));
#97094=DIRECTION('',(-0.190809912898503,0.,0.981627005099017));
#97095=DIRECTION('center_axis',(0.,-1.,0.));
#97096=DIRECTION('ref_axis',(-0.271654016185366,0.,0.962394978940747));
#97097=DIRECTION('center_axis',(0.981627005099017,0.,0.190809912898503));
#97098=DIRECTION('ref_axis',(0.,-1.,0.));
#97099=DIRECTION('',(-0.190809912898503,0.,0.981627005099017));
#97100=DIRECTION('center_axis',(0.981627005099017,-5.42634466570013E-17,
0.190809912898504));
#97101=DIRECTION('ref_axis',(-0.190129344158506,-0.0843845483960271,0.9781257999265));
#97102=DIRECTION('center_axis',(0.981627005099017,4.32027132019077E-17,
0.190809912898503));
#97103=DIRECTION('ref_axis',(-0.190155227141477,-0.0827671749549381,0.97825895566601));
#97104=DIRECTION('center_axis',(0.,1.,0.));
#97105=DIRECTION('ref_axis',(1.,0.,0.));
#97106=DIRECTION('',(-0.190809912898503,0.,0.981627005099017));
#97107=DIRECTION('center_axis',(0.,1.,0.));
#97108=DIRECTION('ref_axis',(-0.304196445644748,0.,0.952609323100032));
#97109=DIRECTION('center_axis',(0.,1.,0.));
#97110=DIRECTION('ref_axis',(-0.302047933389658,0.,0.953292738845228));
#97111=DIRECTION('center_axis',(-0.981627005099017,0.,-0.190809912898503));
#97112=DIRECTION('ref_axis',(-0.190809912898503,0.,0.981627005099017));
#97113=DIRECTION('center_axis',(-0.981627005099017,1.13007235228963E-17,
-0.190809912898503));
#97114=DIRECTION('ref_axis',(-0.189494383908818,-0.117223556705195,0.97485922892508));
#97115=DIRECTION('center_axis',(-0.981627005099017,3.62298903615095E-17,
-0.190809912898504));
#97116=DIRECTION('ref_axis',(-0.189544812876814,-0.114962422466095,0.97511866218026));
#97117=DIRECTION('center_axis',(0.,-1.,0.));
#97118=DIRECTION('ref_axis',(0.,0.,-1.));
#97119=DIRECTION('',(-0.190809912898503,0.,0.981627005099017));
#97120=DIRECTION('center_axis',(0.,-1.,0.));
#97121=DIRECTION('ref_axis',(-0.272783869673527,0.,0.96207534031693));
#97122=DIRECTION('',(-0.190809912898503,0.,0.981627005099017));
#97123=DIRECTION('center_axis',(0.,-1.,0.));
#97124=DIRECTION('ref_axis',(-0.271232151177082,0.,0.96251395842754));
#97125=DIRECTION('center_axis',(0.981627005099017,0.,0.190809912898503));
#97126=DIRECTION('ref_axis',(0.,-1.,0.));
#97127=DIRECTION('',(-0.190809912898503,0.,0.981627005099017));
#97128=DIRECTION('center_axis',(0.981627005099017,1.87115333300005E-18,
0.190809912898503));
#97129=DIRECTION('ref_axis',(-0.190773730797495,-0.0194733573221602,0.98144086525486));
#97130=DIRECTION('center_axis',(0.981627005099017,1.35008478755962E-18,
0.190809912898503));
#97131=DIRECTION('ref_axis',(-0.190775104613922,-0.0191001172972896,0.981447932892406));
#97132=DIRECTION('center_axis',(0.,1.,0.));
#97133=DIRECTION('ref_axis',(1.,0.,0.));
#97134=DIRECTION('',(-0.190809912898513,0.,0.981627005099015));
#97135=DIRECTION('center_axis',(0.,1.,0.));
#97136=DIRECTION('ref_axis',(-0.303820565781007,0.,0.952729270993869));
#97137=DIRECTION('center_axis',(0.,1.,0.));
#97138=DIRECTION('ref_axis',(-0.301693026915346,0.,0.953405117203939));
#97139=DIRECTION('center_axis',(-0.981627005099017,0.,-0.190809912898503));
#97140=DIRECTION('ref_axis',(-0.190809912898503,0.,0.981627005099017));
#97141=DIRECTION('center_axis',(-0.981627005099017,6.02705254554468E-17,
-0.190809912898504));
#97142=DIRECTION('ref_axis',(-0.190550775140863,-0.0520993585356409,0.98029386356));
#97143=DIRECTION('center_axis',(-0.981627005099017,1.99264396988302E-17,
-0.190809912898504));
#97144=DIRECTION('ref_axis',(-0.190560682254905,-0.0510944099849382,0.980344830988992));
#97145=DIRECTION('center_axis',(0.,-1.,0.));
#97146=DIRECTION('ref_axis',(0.,0.,-1.));
#97147=DIRECTION('',(-0.19080991289849,0.,0.98162700509902));
#97148=DIRECTION('center_axis',(0.,-1.,0.));
#97149=DIRECTION('ref_axis',(-0.0162088407295448,0.,0.999868628111816));
#97150=DIRECTION('',(-0.190809912898503,0.,0.981627005099017));
#97151=DIRECTION('center_axis',(0.,-1.,0.));
#97152=DIRECTION('ref_axis',(-0.0195969249883702,0.,0.99980796182617));
#97153=DIRECTION('center_axis',(0.981627005099017,0.,0.190809912898503));
#97154=DIRECTION('ref_axis',(0.,-1.,0.));
#97155=DIRECTION('',(-0.190809912898503,0.,0.981627005099017));
#97156=DIRECTION('center_axis',(0.981627005099017,-9.58185426548332E-19,
0.190809912898503));
#97157=DIRECTION('ref_axis',(-0.190772856350838,-0.0197072453096809,0.981436366639247));
#97158=DIRECTION('center_axis',(0.981627005099017,-1.93402012328947E-17,
0.190809912898504));
#97159=DIRECTION('ref_axis',(-0.190774296053174,-0.0193206613757493,0.981443773228716));
#97160=DIRECTION('center_axis',(0.,1.,0.));
#97161=DIRECTION('ref_axis',(1.,0.,0.));
#97162=DIRECTION('',(-0.190809912898503,0.,0.981627005099017));
#97163=DIRECTION('center_axis',(0.,1.,0.));
#97164=DIRECTION('ref_axis',(-0.0491567156126708,0.,0.998791077908776));
#97165=DIRECTION('center_axis',(0.,1.,0.));
#97166=DIRECTION('ref_axis',(-0.0518907218216088,0.,0.998652768978704));
#97167=DIRECTION('center_axis',(-0.981627005099017,0.,-0.190809912898503));
#97168=DIRECTION('ref_axis',(-0.190809912898503,0.,0.981627005099017));
#97169=DIRECTION('center_axis',(-0.981627005099017,-1.3274254649155E-17,
-0.190809912898503));
#97170=DIRECTION('ref_axis',(-0.190549003442479,-0.0522770327244192,0.980284749007454));
#97171=DIRECTION('center_axis',(-0.981627005099017,1.8233950826407E-18,
-0.190809912898503));
#97172=DIRECTION('ref_axis',(-0.190559043863139,-0.0512619669220116,0.980336402236117));
#97173=DIRECTION('center_axis',(0.,-1.,0.));
#97174=DIRECTION('ref_axis',(0.,0.,-1.));
#97175=DIRECTION('',(-0.190809912898503,0.,0.981627005099017));
#97176=DIRECTION('center_axis',(0.,-1.,0.));
#97177=DIRECTION('ref_axis',(-0.0815670055162436,0.,0.996667860227826));
#97178=DIRECTION('',(-0.190809912898503,0.,0.981627005099017));
#97179=DIRECTION('center_axis',(0.,-1.,0.));
#97180=DIRECTION('ref_axis',(-0.0836737189959334,0.,0.996493205571112));
#97181=DIRECTION('center_axis',(0.981627005099017,0.,0.190809912898503));
#97182=DIRECTION('ref_axis',(0.,-1.,0.));
#97183=DIRECTION('',(-0.190809912898503,0.,0.981627005099017));
#97184=DIRECTION('center_axis',(0.981627005099017,-2.30381126037603E-17,
0.190809912898504));
#97185=DIRECTION('ref_axis',(-0.190773546907965,-0.0195227749578894,0.981439919229954));
#97186=DIRECTION('center_axis',(0.981627005099017,-4.07005188086187E-18,
0.190809912898503));
#97187=DIRECTION('ref_axis',(-0.190774934456505,-0.0191467407848009,0.98144705751275));
#97188=DIRECTION('center_axis',(0.,1.,0.));
#97189=DIRECTION('ref_axis',(1.,0.,0.));
#97190=DIRECTION('',(-0.190809912898503,0.,0.981627005099017));
#97191=DIRECTION('center_axis',(0.,1.,0.));
#97192=DIRECTION('ref_axis',(-0.114028208728371,0.,0.993477512384754));
#97193=DIRECTION('center_axis',(0.,1.,0.));
#97194=DIRECTION('ref_axis',(-0.115501073839451,0.,0.993307355223917));
#97195=DIRECTION('center_axis',(-0.981627005099017,0.,-0.190809912898503));
#97196=DIRECTION('ref_axis',(-0.190809912898503,0.,0.981627005099017));
#97197=DIRECTION('center_axis',(-0.981627005099017,-1.86918439830296E-18,
-0.190809912898503));
#97198=DIRECTION('ref_axis',(-0.190552739758759,-0.0519016243589593,0.980303970592455));
#97199=DIRECTION('center_axis',(-0.981627005099017,-1.79829070982616E-17,
-0.190809912898503));
#97200=DIRECTION('ref_axis',(-0.190562500052238,-0.0509078583188802,0.980354182698899));
#97201=DIRECTION('center_axis',(0.,-1.,0.));
#97202=DIRECTION('ref_axis',(0.,0.,-1.));
#97203=DIRECTION('',(-0.190809912898503,0.,0.981627005099017));
#97204=DIRECTION('center_axis',(0.,-1.,0.));
#97205=DIRECTION('ref_axis',(-0.146109040889921,0.,0.989268491447204));
#97206=DIRECTION('',(-0.190809912898503,0.,0.981627005099017));
#97207=DIRECTION('center_axis',(0.,-1.,0.));
#97208=DIRECTION('ref_axis',(-0.146965819474498,0.,0.989141571215258));
#97209=DIRECTION('center_axis',(0.981627005099017,0.,0.190809912898503));
#97210=DIRECTION('ref_axis',(0.,-1.,0.));
#97211=DIRECTION('',(-0.190809912898503,0.,0.981627005099017));
#97212=DIRECTION('center_axis',(0.981627005099017,-7.91239536570904E-18,
0.190809912898504));
#97213=DIRECTION('ref_axis',(-0.190773912836659,-0.0194243130663802,0.981441801760497));
#97214=DIRECTION('center_axis',(0.981627005099017,-9.40484652357021E-18,
0.190809912898504));
#97215=DIRECTION('ref_axis',(-0.190775273123846,-0.0190538327525699,0.981448799796484));
#97216=DIRECTION('center_axis',(0.,1.,0.));
#97217=DIRECTION('ref_axis',(1.,0.,0.));
#97218=DIRECTION('',(-0.190809912898503,0.,0.981627005099017));
#97219=DIRECTION('center_axis',(0.,1.,0.));
#97220=DIRECTION('ref_axis',(-0.178092965033456,0.,0.984013666472977));
#97221=DIRECTION('center_axis',(0.,1.,0.));
#97222=DIRECTION('ref_axis',(-0.178335419485715,0.,0.983969754696177));
#97223=DIRECTION('center_axis',(-0.981627005099017,0.,-0.190809912898503));
#97224=DIRECTION('ref_axis',(-0.190809912898503,0.,0.981627005099017));
#97225=DIRECTION('center_axis',(-0.981627005099017,0.,-0.190809912898503));
#97226=DIRECTION('ref_axis',(-0.190554247320776,-0.0517493780667019,0.980311726287981));
#97227=DIRECTION('center_axis',(-0.981627005099017,2.50341476753788E-17,
-0.190809912898504));
#97228=DIRECTION('ref_axis',(-0.190563895665479,-0.0507641669217001,0.980361362470769));
#97229=DIRECTION('center_axis',(0.,-1.,0.));
#97230=DIRECTION('ref_axis',(0.,0.,-1.));
#97231=DIRECTION('',(-0.190809912898503,1.256366518269E-14,0.981627005099017));
#97232=DIRECTION('center_axis',(0.,-1.,0.));
#97233=DIRECTION('ref_axis',(-0.209847318452884,0.,0.977734167827909));
#97234=DIRECTION('',(-0.190809912898503,0.,0.981627005099017));
#97235=DIRECTION('center_axis',(0.,-1.,0.));
#97236=DIRECTION('ref_axis',(-0.209484670142235,0.,0.977811931291186));
#97237=DIRECTION('center_axis',(0.981627005099017,0.,0.190809912898503));
#97238=DIRECTION('ref_axis',(0.,-1.,0.));
#97239=DIRECTION('',(-0.190809912898503,0.,0.981627005099017));
#97240=DIRECTION('center_axis',(0.981627005099017,-1.5798298463746E-17,
0.190809912898504));
#97241=DIRECTION('ref_axis',(-0.190773973110007,-0.0194080471434809,0.981442111838441));
#97242=DIRECTION('center_axis',(0.981627005099017,2.2356418544253E-18,0.190809912898503));
#97243=DIRECTION('ref_axis',(-0.190775328931839,-0.0190384791832405,0.981449086902289));
#97244=DIRECTION('center_axis',(0.,1.,0.));
#97245=DIRECTION('ref_axis',(1.,0.,0.));
#97246=DIRECTION('',(-0.190809912898491,0.,0.981627005099019));
#97247=DIRECTION('center_axis',(0.,1.,0.));
#97248=DIRECTION('ref_axis',(-0.241358095629752,0.,0.970436123438312));
#97249=DIRECTION('center_axis',(0.,1.,0.));
#97250=DIRECTION('ref_axis',(-0.240400340232753,0.,0.97067382596626));
#97251=DIRECTION('center_axis',(-0.981627005099017,0.,-0.190809912898503));
#97252=DIRECTION('ref_axis',(-0.190809912898503,0.,0.981627005099017));
#97253=DIRECTION('center_axis',(-0.981627005099017,4.65727889790425E-17,
-0.190809912898504));
#97254=DIRECTION('ref_axis',(-0.190553603392484,-0.0518144622395518,0.980308413580627));
#97255=DIRECTION('center_axis',(-0.981627005099017,-2.33022911630896E-17,
-0.190809912898503));
#97256=DIRECTION('ref_axis',(-0.190563299478129,-0.0508255998002297,0.980358295368054));
#97257=DIRECTION('center_axis',(0.190809912898503,0.,-0.981627005099017));
#97258=DIRECTION('ref_axis',(0.,-1.,0.));
#97259=DIRECTION('center_axis',(0.,1.,0.));
#97260=DIRECTION('ref_axis',(1.,0.,0.));
#97261=DIRECTION('',(-0.190809912898503,0.,0.981627005099017));
#97262=DIRECTION('',(0.981627005099017,0.,0.190809912898503));
#97263=DIRECTION('',(-0.190809912898503,0.,0.981627005099017));
#97264=DIRECTION('',(0.981627005099017,0.,0.190809912898503));
#97265=DIRECTION('center_axis',(0.981627005099017,0.,0.190809912898503));
#97266=DIRECTION('ref_axis',(0.,-1.,0.));
#97267=DIRECTION('',(-0.190809912898503,0.,0.981627005099017));
#97268=DIRECTION('',(0.,-1.,0.));
#97269=DIRECTION('',(0.,-1.,0.));
#97270=DIRECTION('center_axis',(0.,-1.,0.));
#97271=DIRECTION('ref_axis',(0.,0.,-1.));
#97272=DIRECTION('',(-0.190809912898503,0.,0.981627005099017));
#97273=DIRECTION('',(-0.981627005099017,0.,-0.190809912898503));
#97274=DIRECTION('',(-0.981627005099017,0.,-0.190809912898503));
#97275=DIRECTION('center_axis',(-0.981627005099017,0.,-0.190809912898503));
#97276=DIRECTION('ref_axis',(-0.190809912898503,0.,0.981627005099017));
#97277=DIRECTION('',(0.,1.,0.));
#97278=DIRECTION('',(0.,1.,0.));
#97279=DIRECTION('center_axis',(0.,1.,0.));
#97280=DIRECTION('ref_axis',(1.,0.,0.));
#97281=DIRECTION('',(-0.190809912898503,0.,0.981627005099017));
#97282=DIRECTION('',(0.981627005099017,0.,0.190809912898503));
#97283=DIRECTION('',(-0.190809912898503,0.,0.981627005099017));
#97284=DIRECTION('',(0.981627005099017,0.,0.190809912898503));
#97285=DIRECTION('center_axis',(0.981627005099017,0.,0.190809912898503));
#97286=DIRECTION('ref_axis',(0.,-1.,0.));
#97287=DIRECTION('',(-0.190809912898503,0.,0.981627005099017));
#97288=DIRECTION('',(0.,-1.,0.));
#97289=DIRECTION('',(0.,-1.,0.));
#97290=DIRECTION('center_axis',(0.,-1.,0.));
#97291=DIRECTION('ref_axis',(0.,0.,-1.));
#97292=DIRECTION('',(-0.190809912898503,0.,0.981627005099017));
#97293=DIRECTION('',(-0.981627005099017,0.,-0.190809912898503));
#97294=DIRECTION('',(-0.981627005099017,0.,-0.190809912898503));
#97295=DIRECTION('center_axis',(-0.981627005099017,0.,-0.190809912898503));
#97296=DIRECTION('ref_axis',(-0.190809912898503,0.,0.981627005099017));
#97297=DIRECTION('',(0.,1.,0.));
#97298=DIRECTION('',(0.,1.,0.));
#97299=DIRECTION('center_axis',(0.,1.,0.));
#97300=DIRECTION('ref_axis',(1.,0.,0.));
#97301=DIRECTION('',(-0.190809912898503,0.,0.981627005099017));
#97302=DIRECTION('',(0.981627005099017,0.,0.190809912898503));
#97303=DIRECTION('',(-0.190809912898503,0.,0.981627005099017));
#97304=DIRECTION('',(0.981627005099017,0.,0.190809912898503));
#97305=DIRECTION('center_axis',(0.981627005099017,0.,0.190809912898503));
#97306=DIRECTION('ref_axis',(0.,-1.,0.));
#97307=DIRECTION('',(-0.190809912898503,0.,0.981627005099017));
#97308=DIRECTION('',(0.,-1.,0.));
#97309=DIRECTION('',(0.,-1.,0.));
#97310=DIRECTION('center_axis',(0.,-1.,0.));
#97311=DIRECTION('ref_axis',(0.,0.,-1.));
#97312=DIRECTION('',(-0.190809912898503,0.,0.981627005099017));
#97313=DIRECTION('',(-0.981627005099017,0.,-0.190809912898503));
#97314=DIRECTION('',(-0.981627005099017,0.,-0.190809912898503));
#97315=DIRECTION('center_axis',(-0.981627005099017,0.,-0.190809912898503));
#97316=DIRECTION('ref_axis',(-0.190809912898503,0.,0.981627005099017));
#97317=DIRECTION('',(0.,1.,0.));
#97318=DIRECTION('',(0.,1.,0.));
#97319=DIRECTION('center_axis',(0.,1.,0.));
#97320=DIRECTION('ref_axis',(1.,0.,0.));
#97321=DIRECTION('',(-0.190809912898503,0.,0.981627005099017));
#97322=DIRECTION('',(0.981627005099017,0.,0.190809912898503));
#97323=DIRECTION('',(-0.190809912898503,0.,0.981627005099017));
#97324=DIRECTION('',(0.981627005099017,0.,0.190809912898503));
#97325=DIRECTION('center_axis',(0.981627005099017,0.,0.190809912898503));
#97326=DIRECTION('ref_axis',(0.,-1.,0.));
#97327=DIRECTION('',(-0.190809912898503,0.,0.981627005099017));
#97328=DIRECTION('',(0.,-1.,0.));
#97329=DIRECTION('',(0.,-1.,0.));
#97330=DIRECTION('center_axis',(0.,-1.,0.));
#97331=DIRECTION('ref_axis',(0.,0.,-1.));
#97332=DIRECTION('',(-0.190809912898503,0.,0.981627005099017));
#97333=DIRECTION('',(-0.981627005099017,0.,-0.190809912898503));
#97334=DIRECTION('',(-0.981627005099017,0.,-0.190809912898503));
#97335=DIRECTION('center_axis',(-0.981627005099017,0.,-0.190809912898503));
#97336=DIRECTION('ref_axis',(-0.190809912898503,0.,0.981627005099017));
#97337=DIRECTION('',(0.,1.,0.));
#97338=DIRECTION('',(0.,1.,0.));
#97339=DIRECTION('center_axis',(0.,1.,0.));
#97340=DIRECTION('ref_axis',(1.,0.,0.));
#97341=DIRECTION('',(-0.190809912898503,0.,0.981627005099017));
#97342=DIRECTION('',(0.981627005099017,0.,0.190809912898503));
#97343=DIRECTION('',(-0.190809912898503,0.,0.981627005099017));
#97344=DIRECTION('',(0.981627005099017,0.,0.190809912898503));
#97345=DIRECTION('center_axis',(0.981627005099017,0.,0.190809912898503));
#97346=DIRECTION('ref_axis',(0.,-1.,0.));
#97347=DIRECTION('',(-0.190809912898503,0.,0.981627005099017));
#97348=DIRECTION('',(0.,-1.,0.));
#97349=DIRECTION('',(0.,-1.,0.));
#97350=DIRECTION('center_axis',(0.,-1.,0.));
#97351=DIRECTION('ref_axis',(0.,0.,-1.));
#97352=DIRECTION('',(-0.190809912898503,0.,0.981627005099017));
#97353=DIRECTION('',(-0.981627005099017,0.,-0.190809912898503));
#97354=DIRECTION('',(-0.981627005099017,0.,-0.190809912898503));
#97355=DIRECTION('center_axis',(-0.981627005099017,0.,-0.190809912898503));
#97356=DIRECTION('ref_axis',(-0.190809912898503,0.,0.981627005099017));
#97357=DIRECTION('',(0.,1.,0.));
#97358=DIRECTION('',(0.,1.,0.));
#97359=DIRECTION('center_axis',(0.,1.,0.));
#97360=DIRECTION('ref_axis',(1.,0.,0.));
#97361=DIRECTION('',(-0.190809912898503,0.,0.981627005099017));
#97362=DIRECTION('',(0.981627005099017,0.,0.190809912898503));
#97363=DIRECTION('',(-0.190809912898503,0.,0.981627005099017));
#97364=DIRECTION('',(0.981627005099017,0.,0.190809912898503));
#97365=DIRECTION('center_axis',(0.981627005099017,0.,0.190809912898503));
#97366=DIRECTION('ref_axis',(0.,-1.,0.));
#97367=DIRECTION('',(-0.190809912898503,0.,0.981627005099017));
#97368=DIRECTION('',(0.,-1.,0.));
#97369=DIRECTION('',(0.,-1.,0.));
#97370=DIRECTION('center_axis',(0.,-1.,0.));
#97371=DIRECTION('ref_axis',(0.,0.,-1.));
#97372=DIRECTION('',(-0.190809912898503,0.,0.981627005099017));
#97373=DIRECTION('',(-0.981627005099017,0.,-0.190809912898503));
#97374=DIRECTION('',(-0.981627005099017,0.,-0.190809912898503));
#97375=DIRECTION('center_axis',(-0.981627005099017,0.,-0.190809912898503));
#97376=DIRECTION('ref_axis',(-0.190809912898503,0.,0.981627005099017));
#97377=DIRECTION('',(0.,1.,0.));
#97378=DIRECTION('',(0.,1.,0.));
#97379=DIRECTION('center_axis',(0.,1.,0.));
#97380=DIRECTION('ref_axis',(1.,0.,0.));
#97381=DIRECTION('',(-0.190809912898503,0.,0.981627005099017));
#97382=DIRECTION('',(0.981627005099017,0.,0.190809912898503));
#97383=DIRECTION('',(-0.190809912898503,0.,0.981627005099017));
#97384=DIRECTION('',(0.981627005099017,0.,0.190809912898503));
#97385=DIRECTION('center_axis',(0.981627005099017,0.,0.190809912898503));
#97386=DIRECTION('ref_axis',(0.,-1.,0.));
#97387=DIRECTION('',(-0.190809912898503,0.,0.981627005099017));
#97388=DIRECTION('',(0.,-1.,0.));
#97389=DIRECTION('',(0.,-1.,0.));
#97390=DIRECTION('center_axis',(0.,-1.,0.));
#97391=DIRECTION('ref_axis',(0.,0.,-1.));
#97392=DIRECTION('',(-0.190809912898503,0.,0.981627005099017));
#97393=DIRECTION('',(-0.981627005099017,0.,-0.190809912898503));
#97394=DIRECTION('',(-0.981627005099017,0.,-0.190809912898503));
#97395=DIRECTION('center_axis',(-0.981627005099017,0.,-0.190809912898503));
#97396=DIRECTION('ref_axis',(-0.190809912898503,0.,0.981627005099017));
#97397=DIRECTION('',(0.,1.,0.));
#97398=DIRECTION('',(0.,1.,0.));
#97399=DIRECTION('center_axis',(0.,1.,0.));
#97400=DIRECTION('ref_axis',(1.,0.,0.));
#97401=DIRECTION('',(-0.190809912898503,0.,0.981627005099017));
#97402=DIRECTION('',(0.981627005099017,0.,0.190809912898503));
#97403=DIRECTION('',(-0.190809912898503,0.,0.981627005099017));
#97404=DIRECTION('',(0.981627005099017,0.,0.190809912898503));
#97405=DIRECTION('center_axis',(0.981627005099017,0.,0.190809912898503));
#97406=DIRECTION('ref_axis',(0.,-1.,0.));
#97407=DIRECTION('',(-0.190809912898503,0.,0.981627005099017));
#97408=DIRECTION('',(0.,-1.,0.));
#97409=DIRECTION('',(0.,-1.,0.));
#97410=DIRECTION('center_axis',(0.,-1.,0.));
#97411=DIRECTION('ref_axis',(0.,0.,-1.));
#97412=DIRECTION('',(-0.190809912898503,0.,0.981627005099017));
#97413=DIRECTION('',(-0.981627005099017,0.,-0.190809912898503));
#97414=DIRECTION('',(-0.981627005099017,0.,-0.190809912898503));
#97415=DIRECTION('center_axis',(-0.981627005099017,0.,-0.190809912898503));
#97416=DIRECTION('ref_axis',(-0.190809912898503,0.,0.981627005099017));
#97417=DIRECTION('',(0.,1.,0.));
#97418=DIRECTION('',(0.,1.,0.));
#97419=DIRECTION('center_axis',(0.,1.,0.));
#97420=DIRECTION('ref_axis',(1.,0.,0.));
#97421=DIRECTION('',(-0.190809912898503,0.,0.981627005099017));
#97422=DIRECTION('',(0.981627005099017,0.,0.190809912898503));
#97423=DIRECTION('',(-0.190809912898503,0.,0.981627005099017));
#97424=DIRECTION('',(0.981627005099017,0.,0.190809912898503));
#97425=DIRECTION('center_axis',(0.981627005099017,0.,0.190809912898503));
#97426=DIRECTION('ref_axis',(0.,-1.,0.));
#97427=DIRECTION('',(-0.190809912898503,0.,0.981627005099017));
#97428=DIRECTION('',(0.,-1.,0.));
#97429=DIRECTION('',(0.,-1.,0.));
#97430=DIRECTION('center_axis',(0.,-1.,0.));
#97431=DIRECTION('ref_axis',(0.,0.,-1.));
#97432=DIRECTION('',(-0.190809912898503,0.,0.981627005099017));
#97433=DIRECTION('',(-0.981627005099017,0.,-0.190809912898503));
#97434=DIRECTION('',(-0.981627005099017,0.,-0.190809912898503));
#97435=DIRECTION('center_axis',(-0.981627005099017,0.,-0.190809912898503));
#97436=DIRECTION('ref_axis',(-0.190809912898503,0.,0.981627005099017));
#97437=DIRECTION('',(0.,1.,0.));
#97438=DIRECTION('',(0.,1.,0.));
#97439=DIRECTION('center_axis',(0.,1.,0.));
#97440=DIRECTION('ref_axis',(1.,0.,0.));
#97441=DIRECTION('',(-0.190809912898503,0.,0.981627005099017));
#97442=DIRECTION('',(0.981627005099017,0.,0.190809912898503));
#97443=DIRECTION('',(-0.190809912898503,0.,0.981627005099017));
#97444=DIRECTION('',(0.981627005099017,0.,0.190809912898503));
#97445=DIRECTION('center_axis',(0.981627005099017,0.,0.190809912898503));
#97446=DIRECTION('ref_axis',(0.,-1.,0.));
#97447=DIRECTION('',(-0.190809912898503,0.,0.981627005099017));
#97448=DIRECTION('',(0.,-1.,0.));
#97449=DIRECTION('',(0.,-1.,0.));
#97450=DIRECTION('center_axis',(0.,-1.,0.));
#97451=DIRECTION('ref_axis',(0.,0.,-1.));
#97452=DIRECTION('',(-0.190809912898503,0.,0.981627005099017));
#97453=DIRECTION('',(-0.981627005099017,0.,-0.190809912898503));
#97454=DIRECTION('',(-0.981627005099017,0.,-0.190809912898503));
#97455=DIRECTION('center_axis',(-0.981627005099017,0.,-0.190809912898503));
#97456=DIRECTION('ref_axis',(-0.190809912898503,0.,0.981627005099017));
#97457=DIRECTION('',(0.,1.,0.));
#97458=DIRECTION('',(0.,1.,0.));
#97459=DIRECTION('center_axis',(0.,1.,0.));
#97460=DIRECTION('ref_axis',(1.,0.,0.));
#97461=DIRECTION('',(-0.190809912898503,0.,0.981627005099017));
#97462=DIRECTION('',(0.981627005099017,0.,0.190809912898503));
#97463=DIRECTION('',(-0.190809912898503,0.,0.981627005099017));
#97464=DIRECTION('',(0.981627005099017,0.,0.190809912898503));
#97465=DIRECTION('center_axis',(0.981627005099017,0.,0.190809912898503));
#97466=DIRECTION('ref_axis',(0.,-1.,0.));
#97467=DIRECTION('',(-0.190809912898503,0.,0.981627005099017));
#97468=DIRECTION('',(0.,-1.,0.));
#97469=DIRECTION('',(0.,-1.,0.));
#97470=DIRECTION('center_axis',(0.,-1.,0.));
#97471=DIRECTION('ref_axis',(0.,0.,-1.));
#97472=DIRECTION('',(-0.190809912898503,0.,0.981627005099017));
#97473=DIRECTION('',(-0.981627005099017,0.,-0.190809912898503));
#97474=DIRECTION('',(-0.981627005099017,0.,-0.190809912898503));
#97475=DIRECTION('center_axis',(-0.981627005099017,0.,-0.190809912898503));
#97476=DIRECTION('ref_axis',(-0.190809912898503,0.,0.981627005099017));
#97477=DIRECTION('',(0.,1.,0.));
#97478=DIRECTION('',(0.,1.,0.));
#97479=DIRECTION('center_axis',(0.,1.,0.));
#97480=DIRECTION('ref_axis',(1.,0.,0.));
#97481=DIRECTION('',(-0.190809912898503,0.,0.981627005099017));
#97482=DIRECTION('',(0.981627005099017,0.,0.190809912898503));
#97483=DIRECTION('',(-0.190809912898503,0.,0.981627005099017));
#97484=DIRECTION('',(0.981627005099017,0.,0.190809912898503));
#97485=DIRECTION('center_axis',(0.981627005099017,0.,0.190809912898503));
#97486=DIRECTION('ref_axis',(0.,-1.,0.));
#97487=DIRECTION('',(-0.190809912898503,0.,0.981627005099017));
#97488=DIRECTION('',(0.,-1.,0.));
#97489=DIRECTION('',(0.,-1.,0.));
#97490=DIRECTION('center_axis',(0.,-1.,0.));
#97491=DIRECTION('ref_axis',(0.,0.,-1.));
#97492=DIRECTION('',(-0.190809912898503,0.,0.981627005099017));
#97493=DIRECTION('',(-0.981627005099017,0.,-0.190809912898503));
#97494=DIRECTION('',(-0.981627005099017,0.,-0.190809912898503));
#97495=DIRECTION('center_axis',(-0.981627005099017,0.,-0.190809912898503));
#97496=DIRECTION('ref_axis',(-0.190809912898503,0.,0.981627005099017));
#97497=DIRECTION('',(0.,1.,0.));
#97498=DIRECTION('',(0.,1.,0.));
#97499=DIRECTION('center_axis',(0.,1.,0.));
#97500=DIRECTION('ref_axis',(1.,0.,0.));
#97501=DIRECTION('',(-0.190809912898503,0.,0.981627005099017));
#97502=DIRECTION('',(0.981627005099017,0.,0.190809912898503));
#97503=DIRECTION('',(-0.190809912898503,0.,0.981627005099017));
#97504=DIRECTION('',(0.981627005099017,0.,0.190809912898503));
#97505=DIRECTION('center_axis',(0.981627005099017,0.,0.190809912898503));
#97506=DIRECTION('ref_axis',(0.,-1.,0.));
#97507=DIRECTION('',(-0.190809912898503,0.,0.981627005099017));
#97508=DIRECTION('',(0.,-1.,0.));
#97509=DIRECTION('',(0.,-1.,0.));
#97510=DIRECTION('center_axis',(0.,-1.,0.));
#97511=DIRECTION('ref_axis',(0.,0.,-1.));
#97512=DIRECTION('',(-0.190809912898503,0.,0.981627005099017));
#97513=DIRECTION('',(-0.981627005099017,0.,-0.190809912898503));
#97514=DIRECTION('',(-0.981627005099017,0.,-0.190809912898503));
#97515=DIRECTION('center_axis',(-0.981627005099017,0.,-0.190809912898503));
#97516=DIRECTION('ref_axis',(-0.190809912898503,0.,0.981627005099017));
#97517=DIRECTION('',(0.,1.,0.));
#97518=DIRECTION('',(0.,1.,0.));
#97519=DIRECTION('center_axis',(0.,1.,0.));
#97520=DIRECTION('ref_axis',(1.,0.,0.));
#97521=DIRECTION('',(-0.190809912898503,0.,0.981627005099017));
#97522=DIRECTION('',(0.981627005099017,0.,0.190809912898503));
#97523=DIRECTION('',(-0.190809912898503,0.,0.981627005099017));
#97524=DIRECTION('',(0.981627005099017,0.,0.190809912898503));
#97525=DIRECTION('center_axis',(0.981627005099017,0.,0.190809912898503));
#97526=DIRECTION('ref_axis',(0.,-1.,0.));
#97527=DIRECTION('',(-0.190809912898503,0.,0.981627005099017));
#97528=DIRECTION('',(0.,-1.,0.));
#97529=DIRECTION('',(0.,-1.,0.));
#97530=DIRECTION('center_axis',(0.,-1.,0.));
#97531=DIRECTION('ref_axis',(0.,0.,-1.));
#97532=DIRECTION('',(-0.190809912898503,0.,0.981627005099017));
#97533=DIRECTION('',(-0.981627005099017,0.,-0.190809912898503));
#97534=DIRECTION('',(-0.981627005099017,0.,-0.190809912898503));
#97535=DIRECTION('center_axis',(-0.981627005099017,0.,-0.190809912898503));
#97536=DIRECTION('ref_axis',(-0.190809912898503,0.,0.981627005099017));
#97537=DIRECTION('',(0.,1.,0.));
#97538=DIRECTION('',(0.,1.,0.));
#97539=DIRECTION('center_axis',(0.,1.,0.));
#97540=DIRECTION('ref_axis',(1.,0.,0.));
#97541=DIRECTION('',(-0.190809912898503,0.,0.981627005099017));
#97542=DIRECTION('',(0.981627005099017,0.,0.190809912898503));
#97543=DIRECTION('',(-0.190809912898503,0.,0.981627005099017));
#97544=DIRECTION('',(0.981627005099017,0.,0.190809912898503));
#97545=DIRECTION('center_axis',(0.981627005099017,0.,0.190809912898503));
#97546=DIRECTION('ref_axis',(0.,-1.,0.));
#97547=DIRECTION('',(-0.190809912898503,0.,0.981627005099017));
#97548=DIRECTION('',(0.,-1.,0.));
#97549=DIRECTION('',(0.,-1.,0.));
#97550=DIRECTION('center_axis',(0.,-1.,0.));
#97551=DIRECTION('ref_axis',(0.,0.,-1.));
#97552=DIRECTION('',(-0.190809912898503,0.,0.981627005099017));
#97553=DIRECTION('',(-0.981627005099017,0.,-0.190809912898503));
#97554=DIRECTION('',(-0.981627005099017,0.,-0.190809912898503));
#97555=DIRECTION('center_axis',(-0.981627005099017,0.,-0.190809912898503));
#97556=DIRECTION('ref_axis',(-0.190809912898503,0.,0.981627005099017));
#97557=DIRECTION('',(0.,1.,0.));
#97558=DIRECTION('',(0.,1.,0.));
#97559=DIRECTION('center_axis',(0.,1.,0.));
#97560=DIRECTION('ref_axis',(1.,0.,0.));
#97561=DIRECTION('',(-0.190809912898503,0.,0.981627005099017));
#97562=DIRECTION('',(0.981627005099017,0.,0.190809912898503));
#97563=DIRECTION('',(-0.190809912898503,0.,0.981627005099017));
#97564=DIRECTION('',(0.981627005099017,0.,0.190809912898503));
#97565=DIRECTION('center_axis',(0.981627005099017,0.,0.190809912898503));
#97566=DIRECTION('ref_axis',(0.,-1.,0.));
#97567=DIRECTION('',(-0.190809912898503,0.,0.981627005099017));
#97568=DIRECTION('',(0.,-1.,0.));
#97569=DIRECTION('',(0.,-1.,0.));
#97570=DIRECTION('center_axis',(0.,-1.,0.));
#97571=DIRECTION('ref_axis',(0.,0.,-1.));
#97572=DIRECTION('',(-0.190809912898503,0.,0.981627005099017));
#97573=DIRECTION('',(-0.981627005099017,0.,-0.190809912898503));
#97574=DIRECTION('',(-0.981627005099017,0.,-0.190809912898503));
#97575=DIRECTION('center_axis',(-0.981627005099017,0.,-0.190809912898503));
#97576=DIRECTION('ref_axis',(-0.190809912898503,0.,0.981627005099017));
#97577=DIRECTION('',(0.,1.,0.));
#97578=DIRECTION('',(0.,1.,0.));
#97579=DIRECTION('center_axis',(0.,1.,0.));
#97580=DIRECTION('ref_axis',(1.,0.,0.));
#97581=DIRECTION('',(-0.190809912898503,0.,0.981627005099017));
#97582=DIRECTION('',(0.981627005099017,0.,0.190809912898503));
#97583=DIRECTION('',(-0.190809912898503,0.,0.981627005099017));
#97584=DIRECTION('',(0.981627005099017,0.,0.190809912898503));
#97585=DIRECTION('center_axis',(0.981627005099017,0.,0.190809912898503));
#97586=DIRECTION('ref_axis',(0.,-1.,0.));
#97587=DIRECTION('',(-0.190809912898503,0.,0.981627005099017));
#97588=DIRECTION('',(0.,-1.,0.));
#97589=DIRECTION('',(0.,-1.,0.));
#97590=DIRECTION('center_axis',(0.,-1.,0.));
#97591=DIRECTION('ref_axis',(0.,0.,-1.));
#97592=DIRECTION('',(-0.190809912898503,0.,0.981627005099017));
#97593=DIRECTION('',(-0.981627005099017,0.,-0.190809912898503));
#97594=DIRECTION('',(-0.981627005099017,0.,-0.190809912898503));
#97595=DIRECTION('center_axis',(-0.981627005099017,0.,-0.190809912898503));
#97596=DIRECTION('ref_axis',(-0.190809912898503,0.,0.981627005099017));
#97597=DIRECTION('',(0.,1.,0.));
#97598=DIRECTION('',(0.,1.,0.));
#97599=DIRECTION('center_axis',(0.,1.,0.));
#97600=DIRECTION('ref_axis',(1.,0.,0.));
#97601=DIRECTION('',(-0.190809912898503,0.,0.981627005099017));
#97602=DIRECTION('',(0.981627005099017,0.,0.190809912898503));
#97603=DIRECTION('',(-0.190809912898503,0.,0.981627005099017));
#97604=DIRECTION('',(0.981627005099017,0.,0.190809912898503));
#97605=DIRECTION('center_axis',(0.981627005099017,0.,0.190809912898503));
#97606=DIRECTION('ref_axis',(0.,-1.,0.));
#97607=DIRECTION('',(-0.190809912898503,0.,0.981627005099017));
#97608=DIRECTION('',(0.,-1.,0.));
#97609=DIRECTION('',(0.,-1.,0.));
#97610=DIRECTION('center_axis',(0.,-1.,0.));
#97611=DIRECTION('ref_axis',(0.,0.,-1.));
#97612=DIRECTION('',(-0.190809912898503,0.,0.981627005099017));
#97613=DIRECTION('',(-0.981627005099017,0.,-0.190809912898503));
#97614=DIRECTION('',(-0.981627005099017,0.,-0.190809912898503));
#97615=DIRECTION('center_axis',(-0.981627005099017,0.,-0.190809912898503));
#97616=DIRECTION('ref_axis',(-0.190809912898503,0.,0.981627005099017));
#97617=DIRECTION('',(0.,1.,0.));
#97618=DIRECTION('',(0.,1.,0.));
#97619=DIRECTION('center_axis',(0.,1.,0.));
#97620=DIRECTION('ref_axis',(1.,0.,0.));
#97621=DIRECTION('',(-0.190809912898503,0.,0.981627005099017));
#97622=DIRECTION('',(0.981627005099017,0.,0.190809912898503));
#97623=DIRECTION('',(-0.190809912898503,0.,0.981627005099017));
#97624=DIRECTION('',(0.981627005099017,0.,0.190809912898503));
#97625=DIRECTION('center_axis',(0.981627005099017,0.,0.190809912898503));
#97626=DIRECTION('ref_axis',(0.,-1.,0.));
#97627=DIRECTION('',(-0.190809912898503,0.,0.981627005099017));
#97628=DIRECTION('',(0.,-1.,0.));
#97629=DIRECTION('',(0.,-1.,0.));
#97630=DIRECTION('center_axis',(0.,-1.,0.));
#97631=DIRECTION('ref_axis',(0.,0.,-1.));
#97632=DIRECTION('',(-0.190809912898503,0.,0.981627005099017));
#97633=DIRECTION('',(-0.981627005099017,0.,-0.190809912898503));
#97634=DIRECTION('',(-0.981627005099017,0.,-0.190809912898503));
#97635=DIRECTION('center_axis',(-0.981627005099017,0.,-0.190809912898503));
#97636=DIRECTION('ref_axis',(-0.190809912898503,0.,0.981627005099017));
#97637=DIRECTION('',(0.,1.,0.));
#97638=DIRECTION('',(0.,1.,0.));
#97639=DIRECTION('center_axis',(0.,1.,0.));
#97640=DIRECTION('ref_axis',(1.,0.,0.));
#97641=DIRECTION('',(-0.190809912898503,0.,0.981627005099017));
#97642=DIRECTION('',(0.981627005099017,0.,0.190809912898503));
#97643=DIRECTION('',(-0.190809912898503,0.,0.981627005099017));
#97644=DIRECTION('',(0.981627005099017,0.,0.190809912898503));
#97645=DIRECTION('center_axis',(0.981627005099017,0.,0.190809912898503));
#97646=DIRECTION('ref_axis',(0.,-1.,0.));
#97647=DIRECTION('',(-0.190809912898503,0.,0.981627005099017));
#97648=DIRECTION('',(0.,-1.,0.));
#97649=DIRECTION('',(0.,-1.,0.));
#97650=DIRECTION('center_axis',(0.,-1.,0.));
#97651=DIRECTION('ref_axis',(0.,0.,-1.));
#97652=DIRECTION('',(-0.190809912898503,0.,0.981627005099017));
#97653=DIRECTION('',(-0.981627005099017,0.,-0.190809912898503));
#97654=DIRECTION('',(-0.981627005099017,0.,-0.190809912898503));
#97655=DIRECTION('center_axis',(-0.981627005099017,0.,-0.190809912898503));
#97656=DIRECTION('ref_axis',(-0.190809912898503,0.,0.981627005099017));
#97657=DIRECTION('',(0.,1.,0.));
#97658=DIRECTION('',(0.,1.,0.));
#97659=DIRECTION('center_axis',(0.,1.,0.));
#97660=DIRECTION('ref_axis',(1.,0.,0.));
#97661=DIRECTION('',(-0.190809912898503,0.,0.981627005099017));
#97662=DIRECTION('',(0.981627005099017,0.,0.190809912898503));
#97663=DIRECTION('',(-0.190809912898503,0.,0.981627005099017));
#97664=DIRECTION('',(0.981627005099017,0.,0.190809912898503));
#97665=DIRECTION('center_axis',(0.981627005099017,0.,0.190809912898503));
#97666=DIRECTION('ref_axis',(0.,-1.,0.));
#97667=DIRECTION('',(-0.190809912898503,0.,0.981627005099017));
#97668=DIRECTION('',(0.,-1.,0.));
#97669=DIRECTION('',(0.,-1.,0.));
#97670=DIRECTION('center_axis',(0.,-1.,0.));
#97671=DIRECTION('ref_axis',(0.,0.,-1.));
#97672=DIRECTION('',(-0.190809912898503,0.,0.981627005099017));
#97673=DIRECTION('',(-0.981627005099017,0.,-0.190809912898503));
#97674=DIRECTION('',(-0.981627005099017,0.,-0.190809912898503));
#97675=DIRECTION('center_axis',(-0.981627005099017,0.,-0.190809912898503));
#97676=DIRECTION('ref_axis',(-0.190809912898503,0.,0.981627005099017));
#97677=DIRECTION('',(0.,1.,0.));
#97678=DIRECTION('',(0.,1.,0.));
#97679=DIRECTION('center_axis',(0.,1.,0.));
#97680=DIRECTION('ref_axis',(1.,0.,0.));
#97681=DIRECTION('',(-0.190809912898503,0.,0.981627005099017));
#97682=DIRECTION('',(0.981627005099017,0.,0.190809912898503));
#97683=DIRECTION('',(-0.190809912898503,0.,0.981627005099017));
#97684=DIRECTION('',(0.981627005099017,0.,0.190809912898503));
#97685=DIRECTION('center_axis',(0.981627005099017,0.,0.190809912898503));
#97686=DIRECTION('ref_axis',(0.,-1.,0.));
#97687=DIRECTION('',(-0.190809912898503,0.,0.981627005099017));
#97688=DIRECTION('',(0.,-1.,0.));
#97689=DIRECTION('',(0.,-1.,0.));
#97690=DIRECTION('center_axis',(0.,-1.,0.));
#97691=DIRECTION('ref_axis',(0.,0.,-1.));
#97692=DIRECTION('',(-0.190809912898503,0.,0.981627005099017));
#97693=DIRECTION('',(-0.981627005099017,0.,-0.190809912898503));
#97694=DIRECTION('',(-0.981627005099017,0.,-0.190809912898503));
#97695=DIRECTION('center_axis',(-0.981627005099017,0.,-0.190809912898503));
#97696=DIRECTION('ref_axis',(-0.190809912898503,0.,0.981627005099017));
#97697=DIRECTION('',(0.,1.,0.));
#97698=DIRECTION('',(0.,1.,0.));
#97699=DIRECTION('center_axis',(0.,1.,0.));
#97700=DIRECTION('ref_axis',(1.,0.,0.));
#97701=DIRECTION('',(-0.190809912898503,0.,0.981627005099017));
#97702=DIRECTION('',(0.981627005099017,0.,0.190809912898503));
#97703=DIRECTION('',(-0.190809912898503,0.,0.981627005099017));
#97704=DIRECTION('',(0.981627005099017,0.,0.190809912898503));
#97705=DIRECTION('center_axis',(0.981627005099017,0.,0.190809912898503));
#97706=DIRECTION('ref_axis',(0.,-1.,0.));
#97707=DIRECTION('',(-0.190809912898503,0.,0.981627005099017));
#97708=DIRECTION('',(0.,-1.,0.));
#97709=DIRECTION('',(0.,-1.,0.));
#97710=DIRECTION('center_axis',(0.,-1.,0.));
#97711=DIRECTION('ref_axis',(0.,0.,-1.));
#97712=DIRECTION('',(-0.190809912898503,0.,0.981627005099017));
#97713=DIRECTION('',(-0.981627005099017,0.,-0.190809912898503));
#97714=DIRECTION('',(-0.981627005099017,0.,-0.190809912898503));
#97715=DIRECTION('center_axis',(-0.981627005099017,0.,-0.190809912898503));
#97716=DIRECTION('ref_axis',(-0.190809912898503,0.,0.981627005099017));
#97717=DIRECTION('',(0.,1.,0.));
#97718=DIRECTION('',(0.,1.,0.));
#97719=DIRECTION('center_axis',(0.,1.,0.));
#97720=DIRECTION('ref_axis',(1.,0.,0.));
#97721=DIRECTION('',(-0.190809912898503,0.,0.981627005099017));
#97722=DIRECTION('',(0.981627005099017,0.,0.190809912898503));
#97723=DIRECTION('',(-0.190809912898503,0.,0.981627005099017));
#97724=DIRECTION('',(0.981627005099017,0.,0.190809912898503));
#97725=DIRECTION('center_axis',(0.981627005099017,0.,0.190809912898503));
#97726=DIRECTION('ref_axis',(0.,-1.,0.));
#97727=DIRECTION('',(-0.190809912898503,0.,0.981627005099017));
#97728=DIRECTION('',(0.,-1.,0.));
#97729=DIRECTION('',(0.,-1.,0.));
#97730=DIRECTION('center_axis',(0.,-1.,0.));
#97731=DIRECTION('ref_axis',(0.,0.,-1.));
#97732=DIRECTION('',(-0.190809912898503,0.,0.981627005099017));
#97733=DIRECTION('',(-0.981627005099017,0.,-0.190809912898503));
#97734=DIRECTION('',(-0.981627005099017,0.,-0.190809912898503));
#97735=DIRECTION('center_axis',(-0.981627005099017,0.,-0.190809912898503));
#97736=DIRECTION('ref_axis',(-0.190809912898503,0.,0.981627005099017));
#97737=DIRECTION('',(0.,1.,0.));
#97738=DIRECTION('',(0.,1.,0.));
#97739=DIRECTION('center_axis',(0.,1.,0.));
#97740=DIRECTION('ref_axis',(1.,0.,0.));
#97741=DIRECTION('',(-0.190809912898503,0.,0.981627005099017));
#97742=DIRECTION('',(0.981627005099017,0.,0.190809912898503));
#97743=DIRECTION('',(-0.190809912898503,0.,0.981627005099017));
#97744=DIRECTION('',(0.981627005099017,0.,0.190809912898503));
#97745=DIRECTION('center_axis',(0.981627005099017,0.,0.190809912898503));
#97746=DIRECTION('ref_axis',(0.,-1.,0.));
#97747=DIRECTION('',(-0.190809912898503,0.,0.981627005099017));
#97748=DIRECTION('',(0.,-1.,0.));
#97749=DIRECTION('',(0.,-1.,0.));
#97750=DIRECTION('center_axis',(0.,-1.,0.));
#97751=DIRECTION('ref_axis',(0.,0.,-1.));
#97752=DIRECTION('',(-0.190809912898503,0.,0.981627005099017));
#97753=DIRECTION('',(-0.981627005099017,0.,-0.190809912898503));
#97754=DIRECTION('',(-0.981627005099017,0.,-0.190809912898503));
#97755=DIRECTION('center_axis',(-0.981627005099017,0.,-0.190809912898503));
#97756=DIRECTION('ref_axis',(-0.190809912898503,0.,0.981627005099017));
#97757=DIRECTION('',(0.,1.,0.));
#97758=DIRECTION('',(0.,1.,0.));
#97759=DIRECTION('center_axis',(0.,1.,0.));
#97760=DIRECTION('ref_axis',(1.,0.,0.));
#97761=DIRECTION('',(-0.190809912898503,0.,0.981627005099017));
#97762=DIRECTION('',(0.981627005099017,0.,0.190809912898503));
#97763=DIRECTION('',(-0.190809912898503,0.,0.981627005099017));
#97764=DIRECTION('',(0.981627005099017,0.,0.190809912898503));
#97765=DIRECTION('center_axis',(0.981627005099017,0.,0.190809912898503));
#97766=DIRECTION('ref_axis',(0.,-1.,0.));
#97767=DIRECTION('',(-0.190809912898503,0.,0.981627005099017));
#97768=DIRECTION('',(0.,-1.,0.));
#97769=DIRECTION('',(0.,-1.,0.));
#97770=DIRECTION('center_axis',(0.,-1.,0.));
#97771=DIRECTION('ref_axis',(0.,0.,-1.));
#97772=DIRECTION('',(-0.190809912898503,0.,0.981627005099017));
#97773=DIRECTION('',(-0.981627005099017,0.,-0.190809912898503));
#97774=DIRECTION('',(-0.981627005099017,0.,-0.190809912898503));
#97775=DIRECTION('center_axis',(-0.981627005099017,0.,-0.190809912898503));
#97776=DIRECTION('ref_axis',(-0.190809912898503,0.,0.981627005099017));
#97777=DIRECTION('',(0.,1.,0.));
#97778=DIRECTION('',(0.,1.,0.));
#97779=DIRECTION('center_axis',(0.,1.,0.));
#97780=DIRECTION('ref_axis',(1.,0.,0.));
#97781=DIRECTION('',(-0.190809912898503,0.,0.981627005099017));
#97782=DIRECTION('',(0.981627005099017,0.,0.190809912898503));
#97783=DIRECTION('',(-0.190809912898503,0.,0.981627005099017));
#97784=DIRECTION('',(0.981627005099017,0.,0.190809912898503));
#97785=DIRECTION('center_axis',(0.981627005099017,0.,0.190809912898503));
#97786=DIRECTION('ref_axis',(0.,-1.,0.));
#97787=DIRECTION('',(-0.190809912898503,0.,0.981627005099017));
#97788=DIRECTION('',(0.,-1.,0.));
#97789=DIRECTION('',(0.,-1.,0.));
#97790=DIRECTION('center_axis',(0.,-1.,0.));
#97791=DIRECTION('ref_axis',(0.,0.,-1.));
#97792=DIRECTION('',(-0.190809912898503,0.,0.981627005099017));
#97793=DIRECTION('',(-0.981627005099017,0.,-0.190809912898503));
#97794=DIRECTION('',(-0.981627005099017,0.,-0.190809912898503));
#97795=DIRECTION('center_axis',(-0.981627005099017,0.,-0.190809912898503));
#97796=DIRECTION('ref_axis',(-0.190809912898503,0.,0.981627005099017));
#97797=DIRECTION('',(0.,1.,0.));
#97798=DIRECTION('',(0.,1.,0.));
#97799=DIRECTION('center_axis',(0.,1.,0.));
#97800=DIRECTION('ref_axis',(1.,0.,0.));
#97801=DIRECTION('',(-0.190809912898503,0.,0.981627005099017));
#97802=DIRECTION('',(0.981627005099017,0.,0.190809912898503));
#97803=DIRECTION('',(-0.190809912898503,0.,0.981627005099017));
#97804=DIRECTION('',(0.981627005099017,0.,0.190809912898503));
#97805=DIRECTION('center_axis',(0.981627005099017,0.,0.190809912898503));
#97806=DIRECTION('ref_axis',(0.,-1.,0.));
#97807=DIRECTION('',(-0.190809912898503,0.,0.981627005099017));
#97808=DIRECTION('',(0.,-1.,0.));
#97809=DIRECTION('',(0.,-1.,0.));
#97810=DIRECTION('center_axis',(0.,-1.,0.));
#97811=DIRECTION('ref_axis',(0.,0.,-1.));
#97812=DIRECTION('',(-0.190809912898503,0.,0.981627005099017));
#97813=DIRECTION('',(-0.981627005099017,0.,-0.190809912898503));
#97814=DIRECTION('',(-0.981627005099017,0.,-0.190809912898503));
#97815=DIRECTION('center_axis',(-0.981627005099017,0.,-0.190809912898503));
#97816=DIRECTION('ref_axis',(-0.190809912898503,0.,0.981627005099017));
#97817=DIRECTION('',(0.,1.,0.));
#97818=DIRECTION('',(0.,1.,0.));
#97819=DIRECTION('center_axis',(0.,1.,0.));
#97820=DIRECTION('ref_axis',(1.,0.,0.));
#97821=DIRECTION('',(-0.190809912898503,0.,0.981627005099017));
#97822=DIRECTION('',(0.981627005099017,0.,0.190809912898503));
#97823=DIRECTION('',(-0.190809912898503,0.,0.981627005099017));
#97824=DIRECTION('',(0.981627005099017,0.,0.190809912898503));
#97825=DIRECTION('center_axis',(0.981627005099017,0.,0.190809912898503));
#97826=DIRECTION('ref_axis',(0.,-1.,0.));
#97827=DIRECTION('',(-0.190809912898503,0.,0.981627005099017));
#97828=DIRECTION('',(0.,-1.,0.));
#97829=DIRECTION('',(0.,-1.,0.));
#97830=DIRECTION('center_axis',(0.,-1.,0.));
#97831=DIRECTION('ref_axis',(0.,0.,-1.));
#97832=DIRECTION('',(-0.190809912898503,0.,0.981627005099017));
#97833=DIRECTION('',(-0.981627005099017,0.,-0.190809912898503));
#97834=DIRECTION('',(-0.981627005099017,0.,-0.190809912898503));
#97835=DIRECTION('center_axis',(-0.981627005099017,0.,-0.190809912898503));
#97836=DIRECTION('ref_axis',(-0.190809912898503,0.,0.981627005099017));
#97837=DIRECTION('',(0.,1.,0.));
#97838=DIRECTION('',(0.,1.,0.));
#97839=DIRECTION('center_axis',(0.,1.,0.));
#97840=DIRECTION('ref_axis',(1.,0.,0.));
#97841=DIRECTION('',(-0.190809912898503,0.,0.981627005099017));
#97842=DIRECTION('',(0.981627005099017,0.,0.190809912898503));
#97843=DIRECTION('',(-0.190809912898503,0.,0.981627005099017));
#97844=DIRECTION('',(0.981627005099017,0.,0.190809912898503));
#97845=DIRECTION('center_axis',(0.981627005099017,0.,0.190809912898503));
#97846=DIRECTION('ref_axis',(0.,-1.,0.));
#97847=DIRECTION('',(-0.190809912898503,0.,0.981627005099017));
#97848=DIRECTION('',(0.,-1.,0.));
#97849=DIRECTION('',(0.,-1.,0.));
#97850=DIRECTION('center_axis',(0.,-1.,0.));
#97851=DIRECTION('ref_axis',(0.,0.,-1.));
#97852=DIRECTION('',(-0.190809912898503,0.,0.981627005099017));
#97853=DIRECTION('',(-0.981627005099017,0.,-0.190809912898503));
#97854=DIRECTION('',(-0.981627005099017,0.,-0.190809912898503));
#97855=DIRECTION('center_axis',(-0.981627005099017,0.,-0.190809912898503));
#97856=DIRECTION('ref_axis',(-0.190809912898503,0.,0.981627005099017));
#97857=DIRECTION('',(0.,1.,0.));
#97858=DIRECTION('',(0.,1.,0.));
#97859=DIRECTION('center_axis',(0.,1.,0.));
#97860=DIRECTION('ref_axis',(1.,0.,0.));
#97861=DIRECTION('',(-0.190809912898503,0.,0.981627005099017));
#97862=DIRECTION('',(0.981627005099017,0.,0.190809912898503));
#97863=DIRECTION('',(-0.190809912898503,0.,0.981627005099017));
#97864=DIRECTION('',(0.981627005099017,0.,0.190809912898503));
#97865=DIRECTION('center_axis',(0.981627005099017,0.,0.190809912898503));
#97866=DIRECTION('ref_axis',(0.,-1.,0.));
#97867=DIRECTION('',(-0.190809912898503,0.,0.981627005099017));
#97868=DIRECTION('',(0.,-1.,0.));
#97869=DIRECTION('',(0.,-1.,0.));
#97870=DIRECTION('center_axis',(0.,-1.,0.));
#97871=DIRECTION('ref_axis',(0.,0.,-1.));
#97872=DIRECTION('',(-0.190809912898503,0.,0.981627005099017));
#97873=DIRECTION('',(-0.981627005099017,0.,-0.190809912898503));
#97874=DIRECTION('',(-0.981627005099017,0.,-0.190809912898503));
#97875=DIRECTION('center_axis',(-0.981627005099017,0.,-0.190809912898503));
#97876=DIRECTION('ref_axis',(-0.190809912898503,0.,0.981627005099017));
#97877=DIRECTION('',(0.,1.,0.));
#97878=DIRECTION('',(0.,1.,0.));
#97879=DIRECTION('center_axis',(0.,1.,0.));
#97880=DIRECTION('ref_axis',(1.,0.,0.));
#97881=DIRECTION('',(-0.190809912898503,0.,0.981627005099017));
#97882=DIRECTION('',(0.981627005099017,0.,0.190809912898503));
#97883=DIRECTION('',(-0.190809912898503,0.,0.981627005099017));
#97884=DIRECTION('',(0.981627005099017,0.,0.190809912898503));
#97885=DIRECTION('center_axis',(0.981627005099017,0.,0.190809912898503));
#97886=DIRECTION('ref_axis',(0.,-1.,0.));
#97887=DIRECTION('',(-0.190809912898503,0.,0.981627005099017));
#97888=DIRECTION('',(0.,-1.,0.));
#97889=DIRECTION('',(0.,-1.,0.));
#97890=DIRECTION('center_axis',(0.,-1.,0.));
#97891=DIRECTION('ref_axis',(0.,0.,-1.));
#97892=DIRECTION('',(-0.190809912898503,0.,0.981627005099017));
#97893=DIRECTION('',(-0.981627005099017,0.,-0.190809912898503));
#97894=DIRECTION('',(-0.981627005099017,0.,-0.190809912898503));
#97895=DIRECTION('center_axis',(-0.981627005099017,0.,-0.190809912898503));
#97896=DIRECTION('ref_axis',(-0.190809912898503,0.,0.981627005099017));
#97897=DIRECTION('',(0.,1.,0.));
#97898=DIRECTION('',(0.,1.,0.));
#97899=DIRECTION('center_axis',(0.,1.,0.));
#97900=DIRECTION('ref_axis',(1.,0.,0.));
#97901=DIRECTION('',(-0.190809912898503,0.,0.981627005099017));
#97902=DIRECTION('',(0.981627005099017,0.,0.190809912898503));
#97903=DIRECTION('',(-0.190809912898503,0.,0.981627005099017));
#97904=DIRECTION('',(0.981627005099017,0.,0.190809912898503));
#97905=DIRECTION('center_axis',(0.981627005099017,0.,0.190809912898503));
#97906=DIRECTION('ref_axis',(0.,-1.,0.));
#97907=DIRECTION('',(-0.190809912898503,0.,0.981627005099017));
#97908=DIRECTION('',(0.,-1.,0.));
#97909=DIRECTION('',(0.,-1.,0.));
#97910=DIRECTION('center_axis',(0.,-1.,0.));
#97911=DIRECTION('ref_axis',(0.,0.,-1.));
#97912=DIRECTION('',(-0.190809912898503,0.,0.981627005099017));
#97913=DIRECTION('',(-0.981627005099017,0.,-0.190809912898503));
#97914=DIRECTION('',(-0.981627005099017,0.,-0.190809912898503));
#97915=DIRECTION('center_axis',(-0.981627005099017,0.,-0.190809912898503));
#97916=DIRECTION('ref_axis',(-0.190809912898503,0.,0.981627005099017));
#97917=DIRECTION('',(0.,1.,0.));
#97918=DIRECTION('',(0.,1.,0.));
#97919=DIRECTION('center_axis',(0.,1.,0.));
#97920=DIRECTION('ref_axis',(1.,0.,0.));
#97921=DIRECTION('',(-0.190809912898503,0.,0.981627005099017));
#97922=DIRECTION('',(0.981627005099017,0.,0.190809912898503));
#97923=DIRECTION('',(-0.190809912898503,0.,0.981627005099017));
#97924=DIRECTION('',(0.981627005099017,0.,0.190809912898503));
#97925=DIRECTION('center_axis',(0.981627005099017,0.,0.190809912898503));
#97926=DIRECTION('ref_axis',(0.,-1.,0.));
#97927=DIRECTION('',(-0.190809912898503,0.,0.981627005099017));
#97928=DIRECTION('',(0.,-1.,0.));
#97929=DIRECTION('',(0.,-1.,0.));
#97930=DIRECTION('center_axis',(0.,-1.,0.));
#97931=DIRECTION('ref_axis',(0.,0.,-1.));
#97932=DIRECTION('',(-0.190809912898503,0.,0.981627005099017));
#97933=DIRECTION('',(-0.981627005099017,0.,-0.190809912898503));
#97934=DIRECTION('',(-0.981627005099017,0.,-0.190809912898503));
#97935=DIRECTION('center_axis',(-0.981627005099017,0.,-0.190809912898503));
#97936=DIRECTION('ref_axis',(-0.190809912898503,0.,0.981627005099017));
#97937=DIRECTION('',(0.,1.,0.));
#97938=DIRECTION('',(0.,1.,0.));
#97939=DIRECTION('center_axis',(0.,1.,0.));
#97940=DIRECTION('ref_axis',(1.,0.,0.));
#97941=DIRECTION('',(-0.190809912898503,0.,0.981627005099017));
#97942=DIRECTION('',(0.981627005099017,0.,0.190809912898503));
#97943=DIRECTION('',(-0.190809912898503,0.,0.981627005099017));
#97944=DIRECTION('',(0.981627005099017,0.,0.190809912898503));
#97945=DIRECTION('center_axis',(0.981627005099017,0.,0.190809912898503));
#97946=DIRECTION('ref_axis',(0.,-1.,0.));
#97947=DIRECTION('',(-0.190809912898503,0.,0.981627005099017));
#97948=DIRECTION('',(0.,-1.,0.));
#97949=DIRECTION('',(0.,-1.,0.));
#97950=DIRECTION('center_axis',(0.,-1.,0.));
#97951=DIRECTION('ref_axis',(0.,0.,-1.));
#97952=DIRECTION('',(-0.190809912898503,0.,0.981627005099017));
#97953=DIRECTION('',(-0.981627005099017,0.,-0.190809912898503));
#97954=DIRECTION('',(-0.981627005099017,0.,-0.190809912898503));
#97955=DIRECTION('center_axis',(-0.981627005099017,0.,-0.190809912898503));
#97956=DIRECTION('ref_axis',(-0.190809912898503,0.,0.981627005099017));
#97957=DIRECTION('',(0.,1.,0.));
#97958=DIRECTION('',(0.,1.,0.));
#97959=DIRECTION('center_axis',(0.,1.,0.));
#97960=DIRECTION('ref_axis',(1.,0.,0.));
#97961=DIRECTION('',(-0.190809912898503,0.,0.981627005099017));
#97962=DIRECTION('',(0.981627005099017,0.,0.190809912898503));
#97963=DIRECTION('',(-0.190809912898503,0.,0.981627005099017));
#97964=DIRECTION('',(0.981627005099017,0.,0.190809912898503));
#97965=DIRECTION('center_axis',(0.981627005099017,0.,0.190809912898503));
#97966=DIRECTION('ref_axis',(0.,-1.,0.));
#97967=DIRECTION('',(-0.190809912898503,0.,0.981627005099017));
#97968=DIRECTION('',(0.,-1.,0.));
#97969=DIRECTION('',(0.,-1.,0.));
#97970=DIRECTION('center_axis',(0.,-1.,0.));
#97971=DIRECTION('ref_axis',(0.,0.,-1.));
#97972=DIRECTION('',(-0.190809912898503,0.,0.981627005099017));
#97973=DIRECTION('',(-0.981627005099017,0.,-0.190809912898503));
#97974=DIRECTION('',(-0.981627005099017,0.,-0.190809912898503));
#97975=DIRECTION('center_axis',(-0.981627005099017,0.,-0.190809912898503));
#97976=DIRECTION('ref_axis',(-0.190809912898503,0.,0.981627005099017));
#97977=DIRECTION('',(0.,1.,0.));
#97978=DIRECTION('',(0.,1.,0.));
#97979=DIRECTION('center_axis',(0.,1.,0.));
#97980=DIRECTION('ref_axis',(1.,0.,0.));
#97981=DIRECTION('',(-0.190809912898503,0.,0.981627005099017));
#97982=DIRECTION('',(0.981627005099017,0.,0.190809912898503));
#97983=DIRECTION('',(-0.190809912898503,0.,0.981627005099017));
#97984=DIRECTION('',(0.981627005099017,0.,0.190809912898503));
#97985=DIRECTION('center_axis',(0.981627005099017,0.,0.190809912898503));
#97986=DIRECTION('ref_axis',(0.,-1.,0.));
#97987=DIRECTION('',(-0.190809912898503,0.,0.981627005099017));
#97988=DIRECTION('',(0.,-1.,0.));
#97989=DIRECTION('',(0.,-1.,0.));
#97990=DIRECTION('center_axis',(0.,-1.,0.));
#97991=DIRECTION('ref_axis',(0.,0.,-1.));
#97992=DIRECTION('',(-0.190809912898503,0.,0.981627005099017));
#97993=DIRECTION('',(-0.981627005099017,0.,-0.190809912898503));
#97994=DIRECTION('',(-0.981627005099017,0.,-0.190809912898503));
#97995=DIRECTION('center_axis',(-0.981627005099017,0.,-0.190809912898503));
#97996=DIRECTION('ref_axis',(-0.190809912898503,0.,0.981627005099017));
#97997=DIRECTION('',(0.,1.,0.));
#97998=DIRECTION('',(0.,1.,0.));
#97999=DIRECTION('center_axis',(0.,1.,0.));
#98000=DIRECTION('ref_axis',(1.,0.,0.));
#98001=DIRECTION('',(-0.190809912898503,0.,0.981627005099017));
#98002=DIRECTION('',(0.981627005099017,0.,0.190809912898503));
#98003=DIRECTION('',(-0.190809912898503,0.,0.981627005099017));
#98004=DIRECTION('',(0.981627005099017,0.,0.190809912898503));
#98005=DIRECTION('center_axis',(0.981627005099017,0.,0.190809912898503));
#98006=DIRECTION('ref_axis',(0.,-1.,0.));
#98007=DIRECTION('',(-0.190809912898503,0.,0.981627005099017));
#98008=DIRECTION('',(0.,-1.,0.));
#98009=DIRECTION('',(0.,-1.,0.));
#98010=DIRECTION('center_axis',(0.,-1.,0.));
#98011=DIRECTION('ref_axis',(0.,0.,-1.));
#98012=DIRECTION('',(-0.190809912898503,0.,0.981627005099017));
#98013=DIRECTION('',(-0.981627005099017,0.,-0.190809912898503));
#98014=DIRECTION('',(-0.981627005099017,0.,-0.190809912898503));
#98015=DIRECTION('center_axis',(-0.981627005099017,0.,-0.190809912898503));
#98016=DIRECTION('ref_axis',(-0.190809912898503,0.,0.981627005099017));
#98017=DIRECTION('',(0.,1.,0.));
#98018=DIRECTION('',(0.,1.,0.));
#98019=DIRECTION('center_axis',(0.,1.,0.));
#98020=DIRECTION('ref_axis',(1.,0.,0.));
#98021=DIRECTION('',(-0.190809912898503,0.,0.981627005099017));
#98022=DIRECTION('',(0.981627005099017,0.,0.190809912898503));
#98023=DIRECTION('',(-0.190809912898503,0.,0.981627005099017));
#98024=DIRECTION('',(0.981627005099017,0.,0.190809912898503));
#98025=DIRECTION('center_axis',(0.981627005099017,0.,0.190809912898503));
#98026=DIRECTION('ref_axis',(0.,-1.,0.));
#98027=DIRECTION('',(-0.190809912898503,0.,0.981627005099017));
#98028=DIRECTION('',(0.,-1.,0.));
#98029=DIRECTION('',(0.,-1.,0.));
#98030=DIRECTION('center_axis',(0.,-1.,0.));
#98031=DIRECTION('ref_axis',(0.,0.,-1.));
#98032=DIRECTION('',(-0.190809912898503,0.,0.981627005099017));
#98033=DIRECTION('',(-0.981627005099017,0.,-0.190809912898503));
#98034=DIRECTION('',(-0.981627005099017,0.,-0.190809912898503));
#98035=DIRECTION('center_axis',(-0.981627005099017,0.,-0.190809912898503));
#98036=DIRECTION('ref_axis',(-0.190809912898503,0.,0.981627005099017));
#98037=DIRECTION('',(0.,1.,0.));
#98038=DIRECTION('',(0.,1.,0.));
#98039=DIRECTION('center_axis',(0.,1.,0.));
#98040=DIRECTION('ref_axis',(1.,0.,0.));
#98041=DIRECTION('',(-0.190809912898503,0.,0.981627005099017));
#98042=DIRECTION('',(0.981627005099017,0.,0.190809912898503));
#98043=DIRECTION('',(-0.190809912898503,0.,0.981627005099017));
#98044=DIRECTION('',(0.981627005099017,0.,0.190809912898503));
#98045=DIRECTION('center_axis',(0.981627005099017,0.,0.190809912898503));
#98046=DIRECTION('ref_axis',(0.,-1.,0.));
#98047=DIRECTION('',(-0.190809912898503,0.,0.981627005099017));
#98048=DIRECTION('',(0.,-1.,0.));
#98049=DIRECTION('',(0.,-1.,0.));
#98050=DIRECTION('center_axis',(0.,-1.,0.));
#98051=DIRECTION('ref_axis',(0.,0.,-1.));
#98052=DIRECTION('',(-0.190809912898503,0.,0.981627005099017));
#98053=DIRECTION('',(-0.981627005099017,0.,-0.190809912898503));
#98054=DIRECTION('',(-0.981627005099017,0.,-0.190809912898503));
#98055=DIRECTION('center_axis',(-0.981627005099017,0.,-0.190809912898503));
#98056=DIRECTION('ref_axis',(-0.190809912898503,0.,0.981627005099017));
#98057=DIRECTION('',(0.,1.,0.));
#98058=DIRECTION('',(0.,1.,0.));
#98059=DIRECTION('center_axis',(0.,1.,0.));
#98060=DIRECTION('ref_axis',(1.,0.,0.));
#98061=DIRECTION('',(-0.190809912898503,0.,0.981627005099017));
#98062=DIRECTION('',(0.981627005099017,0.,0.190809912898503));
#98063=DIRECTION('',(-0.190809912898503,0.,0.981627005099017));
#98064=DIRECTION('',(0.981627005099017,0.,0.190809912898503));
#98065=DIRECTION('center_axis',(0.981627005099017,0.,0.190809912898503));
#98066=DIRECTION('ref_axis',(0.,-1.,0.));
#98067=DIRECTION('',(-0.190809912898503,0.,0.981627005099017));
#98068=DIRECTION('',(0.,-1.,0.));
#98069=DIRECTION('',(0.,-1.,0.));
#98070=DIRECTION('center_axis',(0.,-1.,0.));
#98071=DIRECTION('ref_axis',(0.,0.,-1.));
#98072=DIRECTION('',(-0.190809912898503,0.,0.981627005099017));
#98073=DIRECTION('',(-0.981627005099017,0.,-0.190809912898503));
#98074=DIRECTION('',(-0.981627005099017,0.,-0.190809912898503));
#98075=DIRECTION('center_axis',(-0.981627005099017,0.,-0.190809912898503));
#98076=DIRECTION('ref_axis',(-0.190809912898503,0.,0.981627005099017));
#98077=DIRECTION('',(0.,1.,0.));
#98078=DIRECTION('',(0.,1.,0.));
#98079=DIRECTION('center_axis',(0.,1.,0.));
#98080=DIRECTION('ref_axis',(1.,0.,0.));
#98081=DIRECTION('',(-0.190809912898503,0.,0.981627005099017));
#98082=DIRECTION('',(0.981627005099017,0.,0.190809912898503));
#98083=DIRECTION('',(-0.190809912898503,0.,0.981627005099017));
#98084=DIRECTION('',(0.981627005099017,0.,0.190809912898503));
#98085=DIRECTION('center_axis',(0.981627005099017,0.,0.190809912898503));
#98086=DIRECTION('ref_axis',(0.,-1.,0.));
#98087=DIRECTION('',(-0.190809912898503,0.,0.981627005099017));
#98088=DIRECTION('',(0.,-1.,0.));
#98089=DIRECTION('',(0.,-1.,0.));
#98090=DIRECTION('center_axis',(0.,-1.,0.));
#98091=DIRECTION('ref_axis',(0.,0.,-1.));
#98092=DIRECTION('',(-0.190809912898503,0.,0.981627005099017));
#98093=DIRECTION('',(-0.981627005099017,0.,-0.190809912898503));
#98094=DIRECTION('',(-0.981627005099017,0.,-0.190809912898503));
#98095=DIRECTION('center_axis',(-0.981627005099017,0.,-0.190809912898503));
#98096=DIRECTION('ref_axis',(-0.190809912898503,0.,0.981627005099017));
#98097=DIRECTION('',(0.,1.,0.));
#98098=DIRECTION('',(0.,1.,0.));
#98099=DIRECTION('center_axis',(0.,1.,0.));
#98100=DIRECTION('ref_axis',(1.,0.,0.));
#98101=DIRECTION('',(-0.190809912898503,0.,0.981627005099017));
#98102=DIRECTION('',(0.981627005099017,0.,0.190809912898503));
#98103=DIRECTION('',(-0.190809912898503,0.,0.981627005099017));
#98104=DIRECTION('',(0.981627005099017,0.,0.190809912898503));
#98105=DIRECTION('center_axis',(0.981627005099017,0.,0.190809912898503));
#98106=DIRECTION('ref_axis',(0.,-1.,0.));
#98107=DIRECTION('',(-0.190809912898503,0.,0.981627005099017));
#98108=DIRECTION('',(0.,-1.,0.));
#98109=DIRECTION('',(0.,-1.,0.));
#98110=DIRECTION('center_axis',(0.,-1.,0.));
#98111=DIRECTION('ref_axis',(0.,0.,-1.));
#98112=DIRECTION('',(-0.190809912898503,0.,0.981627005099017));
#98113=DIRECTION('',(-0.981627005099017,0.,-0.190809912898503));
#98114=DIRECTION('',(-0.981627005099017,0.,-0.190809912898503));
#98115=DIRECTION('center_axis',(-0.981627005099017,0.,-0.190809912898503));
#98116=DIRECTION('ref_axis',(-0.190809912898503,0.,0.981627005099017));
#98117=DIRECTION('',(0.,1.,0.));
#98118=DIRECTION('',(0.,1.,0.));
#98119=DIRECTION('center_axis',(0.,1.,0.));
#98120=DIRECTION('ref_axis',(1.,0.,0.));
#98121=DIRECTION('',(-0.190809912898503,0.,0.981627005099017));
#98122=DIRECTION('',(0.981627005099017,0.,0.190809912898503));
#98123=DIRECTION('',(-0.190809912898503,0.,0.981627005099017));
#98124=DIRECTION('',(0.981627005099017,0.,0.190809912898503));
#98125=DIRECTION('center_axis',(0.981627005099017,0.,0.190809912898503));
#98126=DIRECTION('ref_axis',(0.,-1.,0.));
#98127=DIRECTION('',(-0.190809912898503,0.,0.981627005099017));
#98128=DIRECTION('',(0.,-1.,0.));
#98129=DIRECTION('',(0.,-1.,0.));
#98130=DIRECTION('center_axis',(0.,-1.,0.));
#98131=DIRECTION('ref_axis',(0.,0.,-1.));
#98132=DIRECTION('',(-0.190809912898503,0.,0.981627005099017));
#98133=DIRECTION('',(-0.981627005099017,0.,-0.190809912898503));
#98134=DIRECTION('',(-0.981627005099017,0.,-0.190809912898503));
#98135=DIRECTION('center_axis',(-0.981627005099017,0.,-0.190809912898503));
#98136=DIRECTION('ref_axis',(-0.190809912898503,0.,0.981627005099017));
#98137=DIRECTION('',(0.,1.,0.));
#98138=DIRECTION('',(0.,1.,0.));
#98139=DIRECTION('center_axis',(0.,1.,0.));
#98140=DIRECTION('ref_axis',(1.,0.,0.));
#98141=DIRECTION('',(-0.190809912898503,0.,0.981627005099017));
#98142=DIRECTION('',(0.981627005099017,0.,0.190809912898503));
#98143=DIRECTION('',(-0.190809912898503,0.,0.981627005099017));
#98144=DIRECTION('',(0.981627005099017,0.,0.190809912898503));
#98145=DIRECTION('center_axis',(0.981627005099017,0.,0.190809912898503));
#98146=DIRECTION('ref_axis',(0.,-1.,0.));
#98147=DIRECTION('',(-0.190809912898503,0.,0.981627005099017));
#98148=DIRECTION('',(0.,-1.,0.));
#98149=DIRECTION('',(0.,-1.,0.));
#98150=DIRECTION('center_axis',(0.,-1.,0.));
#98151=DIRECTION('ref_axis',(0.,0.,-1.));
#98152=DIRECTION('',(-0.190809912898503,0.,0.981627005099017));
#98153=DIRECTION('',(-0.981627005099017,0.,-0.190809912898503));
#98154=DIRECTION('',(-0.981627005099017,0.,-0.190809912898503));
#98155=DIRECTION('center_axis',(-0.981627005099017,0.,-0.190809912898503));
#98156=DIRECTION('ref_axis',(-0.190809912898503,0.,0.981627005099017));
#98157=DIRECTION('',(0.,1.,0.));
#98158=DIRECTION('',(0.,1.,0.));
#98159=DIRECTION('center_axis',(0.,1.,0.));
#98160=DIRECTION('ref_axis',(1.,0.,0.));
#98161=DIRECTION('',(-0.190809912898503,0.,0.981627005099017));
#98162=DIRECTION('',(0.981627005099017,0.,0.190809912898503));
#98163=DIRECTION('',(-0.190809912898503,0.,0.981627005099017));
#98164=DIRECTION('',(0.981627005099017,0.,0.190809912898503));
#98165=DIRECTION('center_axis',(0.981627005099017,0.,0.190809912898503));
#98166=DIRECTION('ref_axis',(0.,-1.,0.));
#98167=DIRECTION('',(-0.190809912898503,0.,0.981627005099017));
#98168=DIRECTION('',(0.,-1.,0.));
#98169=DIRECTION('',(0.,-1.,0.));
#98170=DIRECTION('center_axis',(0.,-1.,0.));
#98171=DIRECTION('ref_axis',(0.,0.,-1.));
#98172=DIRECTION('',(-0.190809912898503,0.,0.981627005099017));
#98173=DIRECTION('',(-0.981627005099017,0.,-0.190809912898503));
#98174=DIRECTION('',(-0.981627005099017,0.,-0.190809912898503));
#98175=DIRECTION('center_axis',(-0.981627005099017,0.,-0.190809912898503));
#98176=DIRECTION('ref_axis',(-0.190809912898503,0.,0.981627005099017));
#98177=DIRECTION('',(0.,1.,0.));
#98178=DIRECTION('',(0.,1.,0.));
#98179=DIRECTION('center_axis',(0.,1.,0.));
#98180=DIRECTION('ref_axis',(1.,0.,0.));
#98181=DIRECTION('',(-0.190809912898503,0.,0.981627005099017));
#98182=DIRECTION('',(0.981627005099017,0.,0.190809912898503));
#98183=DIRECTION('',(-0.190809912898503,0.,0.981627005099017));
#98184=DIRECTION('',(0.981627005099017,0.,0.190809912898503));
#98185=DIRECTION('center_axis',(0.981627005099017,0.,0.190809912898503));
#98186=DIRECTION('ref_axis',(0.,-1.,0.));
#98187=DIRECTION('',(-0.190809912898503,0.,0.981627005099017));
#98188=DIRECTION('',(0.,-1.,0.));
#98189=DIRECTION('',(0.,-1.,0.));
#98190=DIRECTION('center_axis',(0.,-1.,0.));
#98191=DIRECTION('ref_axis',(0.,0.,-1.));
#98192=DIRECTION('',(-0.190809912898503,0.,0.981627005099017));
#98193=DIRECTION('',(-0.981627005099017,0.,-0.190809912898503));
#98194=DIRECTION('',(-0.981627005099017,0.,-0.190809912898503));
#98195=DIRECTION('center_axis',(-0.981627005099017,0.,-0.190809912898503));
#98196=DIRECTION('ref_axis',(-0.190809912898503,0.,0.981627005099017));
#98197=DIRECTION('',(0.,1.,0.));
#98198=DIRECTION('',(0.,1.,0.));
#98199=DIRECTION('center_axis',(0.,1.,0.));
#98200=DIRECTION('ref_axis',(1.,0.,0.));
#98201=DIRECTION('',(-0.190809912898503,0.,0.981627005099017));
#98202=DIRECTION('',(0.981627005099017,0.,0.190809912898503));
#98203=DIRECTION('',(-0.190809912898503,0.,0.981627005099017));
#98204=DIRECTION('',(0.981627005099017,0.,0.190809912898503));
#98205=DIRECTION('center_axis',(0.981627005099017,0.,0.190809912898503));
#98206=DIRECTION('ref_axis',(0.,-1.,0.));
#98207=DIRECTION('',(-0.190809912898503,0.,0.981627005099017));
#98208=DIRECTION('',(0.,-1.,0.));
#98209=DIRECTION('',(0.,-1.,0.));
#98210=DIRECTION('center_axis',(0.,-1.,0.));
#98211=DIRECTION('ref_axis',(0.,0.,-1.));
#98212=DIRECTION('',(-0.190809912898503,0.,0.981627005099017));
#98213=DIRECTION('',(-0.981627005099017,0.,-0.190809912898503));
#98214=DIRECTION('',(-0.981627005099017,0.,-0.190809912898503));
#98215=DIRECTION('center_axis',(-0.981627005099017,0.,-0.190809912898503));
#98216=DIRECTION('ref_axis',(-0.190809912898503,0.,0.981627005099017));
#98217=DIRECTION('',(0.,1.,0.));
#98218=DIRECTION('',(0.,1.,0.));
#98219=DIRECTION('center_axis',(0.,1.,0.));
#98220=DIRECTION('ref_axis',(1.,0.,0.));
#98221=DIRECTION('',(-0.190809912898503,0.,0.981627005099017));
#98222=DIRECTION('',(0.981627005099017,0.,0.190809912898503));
#98223=DIRECTION('',(-0.190809912898503,0.,0.981627005099017));
#98224=DIRECTION('',(0.981627005099017,0.,0.190809912898503));
#98225=DIRECTION('center_axis',(0.981627005099017,0.,0.190809912898503));
#98226=DIRECTION('ref_axis',(0.,-1.,0.));
#98227=DIRECTION('',(-0.190809912898503,0.,0.981627005099017));
#98228=DIRECTION('',(0.,-1.,0.));
#98229=DIRECTION('',(0.,-1.,0.));
#98230=DIRECTION('center_axis',(0.,-1.,0.));
#98231=DIRECTION('ref_axis',(0.,0.,-1.));
#98232=DIRECTION('',(-0.190809912898503,0.,0.981627005099017));
#98233=DIRECTION('',(-0.981627005099017,0.,-0.190809912898503));
#98234=DIRECTION('',(-0.981627005099017,0.,-0.190809912898503));
#98235=DIRECTION('center_axis',(-0.981627005099017,0.,-0.190809912898503));
#98236=DIRECTION('ref_axis',(-0.190809912898503,0.,0.981627005099017));
#98237=DIRECTION('',(0.,1.,0.));
#98238=DIRECTION('',(0.,1.,0.));
#98239=DIRECTION('center_axis',(0.,1.,0.));
#98240=DIRECTION('ref_axis',(1.,0.,0.));
#98241=DIRECTION('',(-0.190809912898503,0.,0.981627005099017));
#98242=DIRECTION('',(0.981627005099017,0.,0.190809912898503));
#98243=DIRECTION('',(-0.190809912898503,0.,0.981627005099017));
#98244=DIRECTION('',(0.981627005099017,0.,0.190809912898503));
#98245=DIRECTION('center_axis',(0.981627005099017,0.,0.190809912898503));
#98246=DIRECTION('ref_axis',(0.,-1.,0.));
#98247=DIRECTION('',(-0.190809912898503,0.,0.981627005099017));
#98248=DIRECTION('',(0.,-1.,0.));
#98249=DIRECTION('',(0.,-1.,0.));
#98250=DIRECTION('center_axis',(0.,-1.,0.));
#98251=DIRECTION('ref_axis',(0.,0.,-1.));
#98252=DIRECTION('',(-0.190809912898503,0.,0.981627005099017));
#98253=DIRECTION('',(-0.981627005099017,0.,-0.190809912898503));
#98254=DIRECTION('',(-0.981627005099017,0.,-0.190809912898503));
#98255=DIRECTION('center_axis',(-0.981627005099017,0.,-0.190809912898503));
#98256=DIRECTION('ref_axis',(-0.190809912898503,0.,0.981627005099017));
#98257=DIRECTION('',(0.,1.,0.));
#98258=DIRECTION('',(0.,1.,0.));
#98259=DIRECTION('center_axis',(0.,1.,0.));
#98260=DIRECTION('ref_axis',(1.,0.,0.));
#98261=DIRECTION('',(-0.190809912898503,0.,0.981627005099017));
#98262=DIRECTION('',(0.981627005099017,0.,0.190809912898503));
#98263=DIRECTION('',(-0.190809912898503,0.,0.981627005099017));
#98264=DIRECTION('',(0.981627005099017,0.,0.190809912898503));
#98265=DIRECTION('center_axis',(0.981627005099017,0.,0.190809912898503));
#98266=DIRECTION('ref_axis',(0.,-1.,0.));
#98267=DIRECTION('',(-0.190809912898503,0.,0.981627005099017));
#98268=DIRECTION('',(0.,-1.,0.));
#98269=DIRECTION('',(0.,-1.,0.));
#98270=DIRECTION('center_axis',(0.,-1.,0.));
#98271=DIRECTION('ref_axis',(0.,0.,-1.));
#98272=DIRECTION('',(-0.190809912898503,0.,0.981627005099017));
#98273=DIRECTION('',(-0.981627005099017,0.,-0.190809912898503));
#98274=DIRECTION('',(-0.981627005099017,0.,-0.190809912898503));
#98275=DIRECTION('center_axis',(-0.981627005099017,0.,-0.190809912898503));
#98276=DIRECTION('ref_axis',(-0.190809912898503,0.,0.981627005099017));
#98277=DIRECTION('',(0.,1.,0.));
#98278=DIRECTION('',(0.,1.,0.));
#98279=DIRECTION('center_axis',(0.,1.,0.));
#98280=DIRECTION('ref_axis',(1.,0.,0.));
#98281=DIRECTION('',(-0.190809912898503,0.,0.981627005099017));
#98282=DIRECTION('',(0.981627005099017,0.,0.190809912898503));
#98283=DIRECTION('',(-0.190809912898503,0.,0.981627005099017));
#98284=DIRECTION('',(0.981627005099017,0.,0.190809912898503));
#98285=DIRECTION('center_axis',(0.981627005099017,0.,0.190809912898503));
#98286=DIRECTION('ref_axis',(0.,-1.,0.));
#98287=DIRECTION('',(-0.190809912898503,0.,0.981627005099017));
#98288=DIRECTION('',(0.,-1.,0.));
#98289=DIRECTION('',(0.,-1.,0.));
#98290=DIRECTION('center_axis',(0.,-1.,0.));
#98291=DIRECTION('ref_axis',(0.,0.,-1.));
#98292=DIRECTION('',(-0.190809912898503,0.,0.981627005099017));
#98293=DIRECTION('',(-0.981627005099017,0.,-0.190809912898503));
#98294=DIRECTION('',(-0.981627005099017,0.,-0.190809912898503));
#98295=DIRECTION('center_axis',(-0.981627005099017,0.,-0.190809912898503));
#98296=DIRECTION('ref_axis',(-0.190809912898503,0.,0.981627005099017));
#98297=DIRECTION('',(0.,1.,0.));
#98298=DIRECTION('',(0.,1.,0.));
#98299=DIRECTION('center_axis',(0.,1.,0.));
#98300=DIRECTION('ref_axis',(1.,0.,0.));
#98301=DIRECTION('',(-0.190809912898503,0.,0.981627005099017));
#98302=DIRECTION('',(0.981627005099017,0.,0.190809912898503));
#98303=DIRECTION('',(-0.190809912898503,0.,0.981627005099017));
#98304=DIRECTION('',(0.981627005099017,0.,0.190809912898503));
#98305=DIRECTION('center_axis',(0.981627005099017,0.,0.190809912898503));
#98306=DIRECTION('ref_axis',(0.,-1.,0.));
#98307=DIRECTION('',(-0.190809912898503,0.,0.981627005099017));
#98308=DIRECTION('',(0.,-1.,0.));
#98309=DIRECTION('',(0.,-1.,0.));
#98310=DIRECTION('center_axis',(0.,-1.,0.));
#98311=DIRECTION('ref_axis',(0.,0.,-1.));
#98312=DIRECTION('',(-0.190809912898503,0.,0.981627005099017));
#98313=DIRECTION('',(-0.981627005099017,0.,-0.190809912898503));
#98314=DIRECTION('',(-0.981627005099017,0.,-0.190809912898503));
#98315=DIRECTION('center_axis',(-0.981627005099017,0.,-0.190809912898503));
#98316=DIRECTION('ref_axis',(-0.190809912898503,0.,0.981627005099017));
#98317=DIRECTION('',(0.,1.,0.));
#98318=DIRECTION('',(0.,1.,0.));
#98319=DIRECTION('center_axis',(0.,1.,0.));
#98320=DIRECTION('ref_axis',(1.,0.,0.));
#98321=DIRECTION('',(-0.190809912898503,0.,0.981627005099017));
#98322=DIRECTION('',(0.981627005099017,0.,0.190809912898503));
#98323=DIRECTION('',(-0.190809912898503,0.,0.981627005099017));
#98324=DIRECTION('',(0.981627005099017,0.,0.190809912898503));
#98325=DIRECTION('center_axis',(0.981627005099017,0.,0.190809912898503));
#98326=DIRECTION('ref_axis',(0.,-1.,0.));
#98327=DIRECTION('',(-0.190809912898503,0.,0.981627005099017));
#98328=DIRECTION('',(0.,-1.,0.));
#98329=DIRECTION('',(0.,-1.,0.));
#98330=DIRECTION('center_axis',(0.,-1.,0.));
#98331=DIRECTION('ref_axis',(0.,0.,-1.));
#98332=DIRECTION('',(-0.190809912898503,0.,0.981627005099017));
#98333=DIRECTION('',(-0.981627005099017,0.,-0.190809912898503));
#98334=DIRECTION('',(-0.981627005099017,0.,-0.190809912898503));
#98335=DIRECTION('center_axis',(-0.981627005099017,0.,-0.190809912898503));
#98336=DIRECTION('ref_axis',(-0.190809912898503,0.,0.981627005099017));
#98337=DIRECTION('',(0.,1.,0.));
#98338=DIRECTION('',(0.,1.,0.));
#98339=DIRECTION('center_axis',(0.,1.,0.));
#98340=DIRECTION('ref_axis',(1.,0.,0.));
#98341=DIRECTION('',(-0.190809912898503,0.,0.981627005099017));
#98342=DIRECTION('',(0.981627005099017,0.,0.190809912898503));
#98343=DIRECTION('',(-0.190809912898503,0.,0.981627005099017));
#98344=DIRECTION('',(0.981627005099017,0.,0.190809912898503));
#98345=DIRECTION('center_axis',(0.981627005099017,0.,0.190809912898503));
#98346=DIRECTION('ref_axis',(0.,-1.,0.));
#98347=DIRECTION('',(-0.190809912898503,0.,0.981627005099017));
#98348=DIRECTION('',(0.,-1.,0.));
#98349=DIRECTION('',(0.,-1.,0.));
#98350=DIRECTION('center_axis',(0.,-1.,0.));
#98351=DIRECTION('ref_axis',(0.,0.,-1.));
#98352=DIRECTION('',(-0.190809912898503,0.,0.981627005099017));
#98353=DIRECTION('',(-0.981627005099017,0.,-0.190809912898503));
#98354=DIRECTION('',(-0.981627005099017,0.,-0.190809912898503));
#98355=DIRECTION('center_axis',(-0.981627005099017,0.,-0.190809912898503));
#98356=DIRECTION('ref_axis',(-0.190809912898503,0.,0.981627005099017));
#98357=DIRECTION('',(0.,1.,0.));
#98358=DIRECTION('',(0.,1.,0.));
#98359=DIRECTION('center_axis',(0.,1.,0.));
#98360=DIRECTION('ref_axis',(1.,0.,0.));
#98361=DIRECTION('',(-0.190809912898503,0.,0.981627005099017));
#98362=DIRECTION('',(0.981627005099017,0.,0.190809912898503));
#98363=DIRECTION('',(-0.190809912898503,0.,0.981627005099017));
#98364=DIRECTION('',(0.981627005099017,0.,0.190809912898503));
#98365=DIRECTION('center_axis',(0.981627005099017,0.,0.190809912898503));
#98366=DIRECTION('ref_axis',(0.,-1.,0.));
#98367=DIRECTION('',(-0.190809912898503,0.,0.981627005099017));
#98368=DIRECTION('',(0.,-1.,0.));
#98369=DIRECTION('',(0.,-1.,0.));
#98370=DIRECTION('center_axis',(0.,-1.,0.));
#98371=DIRECTION('ref_axis',(0.,0.,-1.));
#98372=DIRECTION('',(-0.190809912898503,0.,0.981627005099017));
#98373=DIRECTION('',(-0.981627005099017,0.,-0.190809912898503));
#98374=DIRECTION('',(-0.981627005099017,0.,-0.190809912898503));
#98375=DIRECTION('center_axis',(-0.981627005099017,0.,-0.190809912898503));
#98376=DIRECTION('ref_axis',(-0.190809912898503,0.,0.981627005099017));
#98377=DIRECTION('',(0.,1.,0.));
#98378=DIRECTION('',(0.,1.,0.));
#98379=DIRECTION('center_axis',(0.,1.,0.));
#98380=DIRECTION('ref_axis',(1.,0.,0.));
#98381=DIRECTION('',(-0.190809912898503,0.,0.981627005099017));
#98382=DIRECTION('',(0.981627005099017,0.,0.190809912898503));
#98383=DIRECTION('',(-0.190809912898503,0.,0.981627005099017));
#98384=DIRECTION('',(0.981627005099017,0.,0.190809912898503));
#98385=DIRECTION('center_axis',(0.981627005099017,0.,0.190809912898503));
#98386=DIRECTION('ref_axis',(0.,-1.,0.));
#98387=DIRECTION('',(-0.190809912898503,0.,0.981627005099017));
#98388=DIRECTION('',(0.,-1.,0.));
#98389=DIRECTION('',(0.,-1.,0.));
#98390=DIRECTION('center_axis',(0.,-1.,0.));
#98391=DIRECTION('ref_axis',(0.,0.,-1.));
#98392=DIRECTION('',(-0.190809912898503,0.,0.981627005099017));
#98393=DIRECTION('',(-0.981627005099017,0.,-0.190809912898503));
#98394=DIRECTION('',(-0.981627005099017,0.,-0.190809912898503));
#98395=DIRECTION('center_axis',(-0.981627005099017,0.,-0.190809912898503));
#98396=DIRECTION('ref_axis',(-0.190809912898503,0.,0.981627005099017));
#98397=DIRECTION('',(0.,1.,0.));
#98398=DIRECTION('',(0.,1.,0.));
#98399=DIRECTION('center_axis',(0.,1.,0.));
#98400=DIRECTION('ref_axis',(1.,0.,0.));
#98401=DIRECTION('',(-0.190809912898503,0.,0.981627005099017));
#98402=DIRECTION('',(0.981627005099017,0.,0.190809912898503));
#98403=DIRECTION('',(-0.190809912898503,0.,0.981627005099017));
#98404=DIRECTION('',(0.981627005099017,0.,0.190809912898503));
#98405=DIRECTION('center_axis',(0.981627005099017,0.,0.190809912898503));
#98406=DIRECTION('ref_axis',(0.,-1.,0.));
#98407=DIRECTION('',(-0.190809912898503,0.,0.981627005099017));
#98408=DIRECTION('',(0.,-1.,0.));
#98409=DIRECTION('',(0.,-1.,0.));
#98410=DIRECTION('center_axis',(0.,-1.,0.));
#98411=DIRECTION('ref_axis',(0.,0.,-1.));
#98412=DIRECTION('',(-0.190809912898503,0.,0.981627005099017));
#98413=DIRECTION('',(-0.981627005099017,0.,-0.190809912898503));
#98414=DIRECTION('',(-0.981627005099017,0.,-0.190809912898503));
#98415=DIRECTION('center_axis',(-0.981627005099017,0.,-0.190809912898503));
#98416=DIRECTION('ref_axis',(-0.190809912898503,0.,0.981627005099017));
#98417=DIRECTION('',(0.,1.,0.));
#98418=DIRECTION('',(0.,1.,0.));
#98419=DIRECTION('center_axis',(0.,1.,0.));
#98420=DIRECTION('ref_axis',(1.,0.,0.));
#98421=DIRECTION('',(-0.190809912898503,0.,0.981627005099017));
#98422=DIRECTION('',(0.981627005099017,0.,0.190809912898503));
#98423=DIRECTION('',(-0.190809912898503,0.,0.981627005099017));
#98424=DIRECTION('',(0.981627005099017,0.,0.190809912898503));
#98425=DIRECTION('center_axis',(0.981627005099017,0.,0.190809912898503));
#98426=DIRECTION('ref_axis',(0.,-1.,0.));
#98427=DIRECTION('',(-0.190809912898503,0.,0.981627005099017));
#98428=DIRECTION('',(0.,-1.,0.));
#98429=DIRECTION('',(0.,-1.,0.));
#98430=DIRECTION('center_axis',(0.,-1.,0.));
#98431=DIRECTION('ref_axis',(0.,0.,-1.));
#98432=DIRECTION('',(-0.190809912898503,0.,0.981627005099017));
#98433=DIRECTION('',(-0.981627005099017,0.,-0.190809912898503));
#98434=DIRECTION('',(-0.981627005099017,0.,-0.190809912898503));
#98435=DIRECTION('center_axis',(-0.981627005099017,0.,-0.190809912898503));
#98436=DIRECTION('ref_axis',(-0.190809912898503,0.,0.981627005099017));
#98437=DIRECTION('',(0.,1.,0.));
#98438=DIRECTION('',(0.,1.,0.));
#98439=DIRECTION('center_axis',(0.,1.,0.));
#98440=DIRECTION('ref_axis',(1.,0.,0.));
#98441=DIRECTION('',(-0.190809912898503,0.,0.981627005099017));
#98442=DIRECTION('',(0.981627005099017,0.,0.190809912898503));
#98443=DIRECTION('',(-0.190809912898503,0.,0.981627005099017));
#98444=DIRECTION('',(0.981627005099017,0.,0.190809912898503));
#98445=DIRECTION('center_axis',(0.981627005099017,0.,0.190809912898503));
#98446=DIRECTION('ref_axis',(0.,-1.,0.));
#98447=DIRECTION('',(-0.190809912898503,0.,0.981627005099017));
#98448=DIRECTION('',(0.,-1.,0.));
#98449=DIRECTION('',(0.,-1.,0.));
#98450=DIRECTION('center_axis',(0.,-1.,0.));
#98451=DIRECTION('ref_axis',(0.,0.,-1.));
#98452=DIRECTION('',(-0.190809912898503,0.,0.981627005099017));
#98453=DIRECTION('',(-0.981627005099017,0.,-0.190809912898503));
#98454=DIRECTION('',(-0.981627005099017,0.,-0.190809912898503));
#98455=DIRECTION('center_axis',(-0.981627005099017,0.,-0.190809912898503));
#98456=DIRECTION('ref_axis',(-0.190809912898503,0.,0.981627005099017));
#98457=DIRECTION('',(0.,1.,0.));
#98458=DIRECTION('',(0.,1.,0.));
#98459=DIRECTION('center_axis',(0.,1.,0.));
#98460=DIRECTION('ref_axis',(1.,0.,0.));
#98461=DIRECTION('',(-0.190809912898503,0.,0.981627005099017));
#98462=DIRECTION('',(0.981627005099017,0.,0.190809912898503));
#98463=DIRECTION('',(-0.190809912898503,0.,0.981627005099017));
#98464=DIRECTION('',(0.981627005099017,0.,0.190809912898503));
#98465=DIRECTION('center_axis',(0.981627005099017,0.,0.190809912898503));
#98466=DIRECTION('ref_axis',(0.,-1.,0.));
#98467=DIRECTION('',(-0.190809912898503,0.,0.981627005099017));
#98468=DIRECTION('',(0.,-1.,0.));
#98469=DIRECTION('',(0.,-1.,0.));
#98470=DIRECTION('center_axis',(0.,-1.,0.));
#98471=DIRECTION('ref_axis',(0.,0.,-1.));
#98472=DIRECTION('',(-0.190809912898503,0.,0.981627005099017));
#98473=DIRECTION('',(-0.981627005099017,0.,-0.190809912898503));
#98474=DIRECTION('',(-0.981627005099017,0.,-0.190809912898503));
#98475=DIRECTION('center_axis',(-0.981627005099017,0.,-0.190809912898503));
#98476=DIRECTION('ref_axis',(-0.190809912898503,0.,0.981627005099017));
#98477=DIRECTION('',(0.,1.,0.));
#98478=DIRECTION('',(0.,1.,0.));
#98479=DIRECTION('center_axis',(0.,1.,0.));
#98480=DIRECTION('ref_axis',(1.,0.,0.));
#98481=DIRECTION('',(-0.190809912898503,0.,0.981627005099017));
#98482=DIRECTION('',(0.981627005099017,0.,0.190809912898503));
#98483=DIRECTION('',(-0.190809912898503,0.,0.981627005099017));
#98484=DIRECTION('',(0.981627005099017,0.,0.190809912898503));
#98485=DIRECTION('center_axis',(0.981627005099017,0.,0.190809912898503));
#98486=DIRECTION('ref_axis',(0.,-1.,0.));
#98487=DIRECTION('',(-0.190809912898503,0.,0.981627005099017));
#98488=DIRECTION('',(0.,-1.,0.));
#98489=DIRECTION('',(0.,-1.,0.));
#98490=DIRECTION('center_axis',(0.,-1.,0.));
#98491=DIRECTION('ref_axis',(0.,0.,-1.));
#98492=DIRECTION('',(-0.190809912898503,0.,0.981627005099017));
#98493=DIRECTION('',(-0.981627005099017,0.,-0.190809912898503));
#98494=DIRECTION('',(-0.981627005099017,0.,-0.190809912898503));
#98495=DIRECTION('center_axis',(-0.981627005099017,0.,-0.190809912898503));
#98496=DIRECTION('ref_axis',(-0.190809912898503,0.,0.981627005099017));
#98497=DIRECTION('',(0.,1.,0.));
#98498=DIRECTION('',(0.,1.,0.));
#98499=DIRECTION('center_axis',(0.,1.,0.));
#98500=DIRECTION('ref_axis',(1.,0.,0.));
#98501=DIRECTION('',(-0.190809912898503,0.,0.981627005099017));
#98502=DIRECTION('',(0.981627005099017,0.,0.190809912898503));
#98503=DIRECTION('',(-0.190809912898503,0.,0.981627005099017));
#98504=DIRECTION('',(0.981627005099017,0.,0.190809912898503));
#98505=DIRECTION('center_axis',(0.981627005099017,0.,0.190809912898503));
#98506=DIRECTION('ref_axis',(0.,-1.,0.));
#98507=DIRECTION('',(-0.190809912898503,0.,0.981627005099017));
#98508=DIRECTION('',(0.,-1.,0.));
#98509=DIRECTION('',(0.,-1.,0.));
#98510=DIRECTION('center_axis',(0.,-1.,0.));
#98511=DIRECTION('ref_axis',(0.,0.,-1.));
#98512=DIRECTION('',(-0.190809912898503,0.,0.981627005099017));
#98513=DIRECTION('',(-0.981627005099017,0.,-0.190809912898503));
#98514=DIRECTION('',(-0.981627005099017,0.,-0.190809912898503));
#98515=DIRECTION('center_axis',(-0.981627005099017,0.,-0.190809912898503));
#98516=DIRECTION('ref_axis',(-0.190809912898503,0.,0.981627005099017));
#98517=DIRECTION('',(0.,1.,0.));
#98518=DIRECTION('',(0.,1.,0.));
#98519=DIRECTION('center_axis',(0.,1.,0.));
#98520=DIRECTION('ref_axis',(1.,0.,0.));
#98521=DIRECTION('',(-0.190809912898503,0.,0.981627005099017));
#98522=DIRECTION('',(0.981627005099017,0.,0.190809912898503));
#98523=DIRECTION('',(-0.190809912898503,0.,0.981627005099017));
#98524=DIRECTION('',(0.981627005099017,0.,0.190809912898503));
#98525=DIRECTION('center_axis',(0.981627005099017,0.,0.190809912898503));
#98526=DIRECTION('ref_axis',(0.,-1.,0.));
#98527=DIRECTION('',(-0.190809912898503,0.,0.981627005099017));
#98528=DIRECTION('',(0.,-1.,0.));
#98529=DIRECTION('',(0.,-1.,0.));
#98530=DIRECTION('center_axis',(0.,-1.,0.));
#98531=DIRECTION('ref_axis',(0.,0.,-1.));
#98532=DIRECTION('',(-0.190809912898503,0.,0.981627005099017));
#98533=DIRECTION('',(-0.981627005099017,0.,-0.190809912898503));
#98534=DIRECTION('',(-0.981627005099017,0.,-0.190809912898503));
#98535=DIRECTION('center_axis',(-0.981627005099017,0.,-0.190809912898503));
#98536=DIRECTION('ref_axis',(-0.190809912898503,0.,0.981627005099017));
#98537=DIRECTION('',(0.,1.,0.));
#98538=DIRECTION('',(0.,1.,0.));
#98539=DIRECTION('center_axis',(0.,1.,0.));
#98540=DIRECTION('ref_axis',(1.,0.,0.));
#98541=DIRECTION('',(-0.190809912898503,0.,0.981627005099017));
#98542=DIRECTION('',(0.981627005099017,0.,0.190809912898503));
#98543=DIRECTION('',(-0.190809912898503,0.,0.981627005099017));
#98544=DIRECTION('',(0.981627005099017,0.,0.190809912898503));
#98545=DIRECTION('center_axis',(0.981627005099017,0.,0.190809912898503));
#98546=DIRECTION('ref_axis',(0.,-1.,0.));
#98547=DIRECTION('',(-0.190809912898503,0.,0.981627005099017));
#98548=DIRECTION('',(0.,-1.,0.));
#98549=DIRECTION('',(0.,-1.,0.));
#98550=DIRECTION('center_axis',(0.,-1.,0.));
#98551=DIRECTION('ref_axis',(0.,0.,-1.));
#98552=DIRECTION('',(-0.190809912898503,0.,0.981627005099017));
#98553=DIRECTION('',(-0.981627005099017,0.,-0.190809912898503));
#98554=DIRECTION('',(-0.981627005099017,0.,-0.190809912898503));
#98555=DIRECTION('center_axis',(-0.981627005099017,0.,-0.190809912898503));
#98556=DIRECTION('ref_axis',(-0.190809912898503,0.,0.981627005099017));
#98557=DIRECTION('',(0.,1.,0.));
#98558=DIRECTION('',(0.,1.,0.));
#98559=DIRECTION('center_axis',(0.,1.,0.));
#98560=DIRECTION('ref_axis',(1.,0.,0.));
#98561=DIRECTION('',(-0.190809912898503,0.,0.981627005099017));
#98562=DIRECTION('',(0.981627005099017,0.,0.190809912898503));
#98563=DIRECTION('',(-0.190809912898503,0.,0.981627005099017));
#98564=DIRECTION('',(0.981627005099017,0.,0.190809912898503));
#98565=DIRECTION('center_axis',(0.981627005099017,0.,0.190809912898503));
#98566=DIRECTION('ref_axis',(0.,-1.,0.));
#98567=DIRECTION('',(-0.190809912898503,0.,0.981627005099017));
#98568=DIRECTION('',(0.,-1.,0.));
#98569=DIRECTION('',(0.,-1.,0.));
#98570=DIRECTION('center_axis',(0.,-1.,0.));
#98571=DIRECTION('ref_axis',(0.,0.,-1.));
#98572=DIRECTION('',(-0.190809912898503,0.,0.981627005099017));
#98573=DIRECTION('',(-0.981627005099017,0.,-0.190809912898503));
#98574=DIRECTION('',(-0.981627005099017,0.,-0.190809912898503));
#98575=DIRECTION('center_axis',(-0.981627005099017,0.,-0.190809912898503));
#98576=DIRECTION('ref_axis',(-0.190809912898503,0.,0.981627005099017));
#98577=DIRECTION('',(0.,1.,0.));
#98578=DIRECTION('',(0.,1.,0.));
#98579=DIRECTION('center_axis',(0.,1.,0.));
#98580=DIRECTION('ref_axis',(1.,0.,0.));
#98581=DIRECTION('',(-0.190809912898503,0.,0.981627005099017));
#98582=DIRECTION('',(0.981627005099017,0.,0.190809912898503));
#98583=DIRECTION('',(-0.190809912898503,0.,0.981627005099017));
#98584=DIRECTION('',(0.981627005099017,0.,0.190809912898503));
#98585=DIRECTION('center_axis',(0.981627005099017,0.,0.190809912898503));
#98586=DIRECTION('ref_axis',(0.,-1.,0.));
#98587=DIRECTION('',(-0.190809912898503,0.,0.981627005099017));
#98588=DIRECTION('',(0.,-1.,0.));
#98589=DIRECTION('',(0.,-1.,0.));
#98590=DIRECTION('center_axis',(0.,-1.,0.));
#98591=DIRECTION('ref_axis',(0.,0.,-1.));
#98592=DIRECTION('',(-0.190809912898503,0.,0.981627005099017));
#98593=DIRECTION('',(-0.981627005099017,0.,-0.190809912898503));
#98594=DIRECTION('',(-0.981627005099017,0.,-0.190809912898503));
#98595=DIRECTION('center_axis',(-0.981627005099017,0.,-0.190809912898503));
#98596=DIRECTION('ref_axis',(-0.190809912898503,0.,0.981627005099017));
#98597=DIRECTION('',(0.,1.,0.));
#98598=DIRECTION('',(0.,1.,0.));
#98599=DIRECTION('center_axis',(0.,1.,0.));
#98600=DIRECTION('ref_axis',(1.,0.,0.));
#98601=DIRECTION('',(-0.190809912898503,0.,0.981627005099017));
#98602=DIRECTION('',(0.981627005099017,0.,0.190809912898503));
#98603=DIRECTION('',(-0.190809912898503,0.,0.981627005099017));
#98604=DIRECTION('',(0.981627005099017,0.,0.190809912898503));
#98605=DIRECTION('center_axis',(0.981627005099017,0.,0.190809912898503));
#98606=DIRECTION('ref_axis',(0.,-1.,0.));
#98607=DIRECTION('',(-0.190809912898503,0.,0.981627005099017));
#98608=DIRECTION('',(0.,-1.,0.));
#98609=DIRECTION('',(0.,-1.,0.));
#98610=DIRECTION('center_axis',(0.,-1.,0.));
#98611=DIRECTION('ref_axis',(0.,0.,-1.));
#98612=DIRECTION('',(-0.190809912898503,0.,0.981627005099017));
#98613=DIRECTION('',(-0.981627005099017,0.,-0.190809912898503));
#98614=DIRECTION('',(-0.981627005099017,0.,-0.190809912898503));
#98615=DIRECTION('center_axis',(-0.981627005099017,0.,-0.190809912898503));
#98616=DIRECTION('ref_axis',(-0.190809912898503,0.,0.981627005099017));
#98617=DIRECTION('',(0.,1.,0.));
#98618=DIRECTION('',(0.,1.,0.));
#98619=DIRECTION('center_axis',(0.,1.,0.));
#98620=DIRECTION('ref_axis',(1.,0.,0.));
#98621=DIRECTION('',(-0.190809912898503,0.,0.981627005099017));
#98622=DIRECTION('',(0.981627005099017,0.,0.190809912898503));
#98623=DIRECTION('',(-0.190809912898503,0.,0.981627005099017));
#98624=DIRECTION('',(0.981627005099017,0.,0.190809912898503));
#98625=DIRECTION('center_axis',(0.981627005099017,0.,0.190809912898503));
#98626=DIRECTION('ref_axis',(0.,-1.,0.));
#98627=DIRECTION('',(-0.190809912898503,0.,0.981627005099017));
#98628=DIRECTION('',(0.,-1.,0.));
#98629=DIRECTION('',(0.,-1.,0.));
#98630=DIRECTION('center_axis',(0.,-1.,0.));
#98631=DIRECTION('ref_axis',(0.,0.,-1.));
#98632=DIRECTION('',(-0.190809912898503,0.,0.981627005099017));
#98633=DIRECTION('',(-0.981627005099017,0.,-0.190809912898503));
#98634=DIRECTION('',(-0.981627005099017,0.,-0.190809912898503));
#98635=DIRECTION('center_axis',(-0.981627005099017,0.,-0.190809912898503));
#98636=DIRECTION('ref_axis',(-0.190809912898503,0.,0.981627005099017));
#98637=DIRECTION('',(0.,1.,0.));
#98638=DIRECTION('',(0.,1.,0.));
#98639=DIRECTION('center_axis',(0.,1.,0.));
#98640=DIRECTION('ref_axis',(1.,0.,0.));
#98641=DIRECTION('',(-0.190809912898503,0.,0.981627005099017));
#98642=DIRECTION('',(0.981627005099017,0.,0.190809912898503));
#98643=DIRECTION('',(-0.190809912898503,0.,0.981627005099017));
#98644=DIRECTION('',(0.981627005099017,0.,0.190809912898503));
#98645=DIRECTION('center_axis',(0.981627005099017,0.,0.190809912898503));
#98646=DIRECTION('ref_axis',(0.,-1.,0.));
#98647=DIRECTION('',(-0.190809912898503,0.,0.981627005099017));
#98648=DIRECTION('',(0.,-1.,0.));
#98649=DIRECTION('',(0.,-1.,0.));
#98650=DIRECTION('center_axis',(0.,-1.,0.));
#98651=DIRECTION('ref_axis',(0.,0.,-1.));
#98652=DIRECTION('',(-0.190809912898503,0.,0.981627005099017));
#98653=DIRECTION('',(-0.981627005099017,0.,-0.190809912898503));
#98654=DIRECTION('',(-0.981627005099017,0.,-0.190809912898503));
#98655=DIRECTION('center_axis',(-0.981627005099017,0.,-0.190809912898503));
#98656=DIRECTION('ref_axis',(-0.190809912898503,0.,0.981627005099017));
#98657=DIRECTION('',(0.,1.,0.));
#98658=DIRECTION('',(0.,1.,0.));
#98659=DIRECTION('center_axis',(0.,1.,0.));
#98660=DIRECTION('ref_axis',(1.,0.,0.));
#98661=DIRECTION('',(-0.190809912898503,0.,0.981627005099017));
#98662=DIRECTION('',(0.981627005099017,0.,0.190809912898503));
#98663=DIRECTION('',(-0.190809912898503,0.,0.981627005099017));
#98664=DIRECTION('',(0.981627005099017,0.,0.190809912898503));
#98665=DIRECTION('center_axis',(0.981627005099017,0.,0.190809912898503));
#98666=DIRECTION('ref_axis',(0.,-1.,0.));
#98667=DIRECTION('',(-0.190809912898503,0.,0.981627005099017));
#98668=DIRECTION('',(0.,-1.,0.));
#98669=DIRECTION('',(0.,-1.,0.));
#98670=DIRECTION('center_axis',(0.,-1.,0.));
#98671=DIRECTION('ref_axis',(0.,0.,-1.));
#98672=DIRECTION('',(-0.190809912898503,0.,0.981627005099017));
#98673=DIRECTION('',(-0.981627005099017,0.,-0.190809912898503));
#98674=DIRECTION('',(-0.981627005099017,0.,-0.190809912898503));
#98675=DIRECTION('center_axis',(-0.981627005099017,0.,-0.190809912898503));
#98676=DIRECTION('ref_axis',(-0.190809912898503,0.,0.981627005099017));
#98677=DIRECTION('',(0.,1.,0.));
#98678=DIRECTION('',(0.,1.,0.));
#98679=DIRECTION('center_axis',(0.,1.,0.));
#98680=DIRECTION('ref_axis',(1.,0.,0.));
#98681=DIRECTION('',(-0.190809912898503,0.,0.981627005099017));
#98682=DIRECTION('',(0.981627005099017,0.,0.190809912898503));
#98683=DIRECTION('',(-0.190809912898503,0.,0.981627005099017));
#98684=DIRECTION('',(0.981627005099017,0.,0.190809912898503));
#98685=DIRECTION('center_axis',(0.981627005099017,0.,0.190809912898503));
#98686=DIRECTION('ref_axis',(0.,-1.,0.));
#98687=DIRECTION('',(-0.190809912898503,0.,0.981627005099017));
#98688=DIRECTION('',(0.,-1.,0.));
#98689=DIRECTION('',(0.,-1.,0.));
#98690=DIRECTION('center_axis',(0.,-1.,0.));
#98691=DIRECTION('ref_axis',(0.,0.,-1.));
#98692=DIRECTION('',(-0.190809912898503,0.,0.981627005099017));
#98693=DIRECTION('',(-0.981627005099017,0.,-0.190809912898503));
#98694=DIRECTION('',(-0.981627005099017,0.,-0.190809912898503));
#98695=DIRECTION('center_axis',(-0.981627005099017,0.,-0.190809912898503));
#98696=DIRECTION('ref_axis',(-0.190809912898503,0.,0.981627005099017));
#98697=DIRECTION('',(0.,1.,0.));
#98698=DIRECTION('',(0.,1.,0.));
#98699=DIRECTION('center_axis',(0.,1.,0.));
#98700=DIRECTION('ref_axis',(1.,0.,0.));
#98701=DIRECTION('',(-0.190809912898503,0.,0.981627005099017));
#98702=DIRECTION('',(0.981627005099017,0.,0.190809912898503));
#98703=DIRECTION('',(-0.190809912898503,0.,0.981627005099017));
#98704=DIRECTION('',(0.981627005099017,0.,0.190809912898503));
#98705=DIRECTION('center_axis',(0.981627005099017,0.,0.190809912898503));
#98706=DIRECTION('ref_axis',(0.,-1.,0.));
#98707=DIRECTION('',(-0.190809912898503,0.,0.981627005099017));
#98708=DIRECTION('',(0.,-1.,0.));
#98709=DIRECTION('',(0.,-1.,0.));
#98710=DIRECTION('center_axis',(0.,-1.,0.));
#98711=DIRECTION('ref_axis',(0.,0.,-1.));
#98712=DIRECTION('',(-0.190809912898503,0.,0.981627005099017));
#98713=DIRECTION('',(-0.981627005099017,0.,-0.190809912898503));
#98714=DIRECTION('',(-0.981627005099017,0.,-0.190809912898503));
#98715=DIRECTION('center_axis',(-0.981627005099017,0.,-0.190809912898503));
#98716=DIRECTION('ref_axis',(-0.190809912898503,0.,0.981627005099017));
#98717=DIRECTION('',(0.,1.,0.));
#98718=DIRECTION('',(0.,1.,0.));
#98719=DIRECTION('center_axis',(0.,1.,0.));
#98720=DIRECTION('ref_axis',(1.,0.,0.));
#98721=DIRECTION('',(-0.190809912898503,0.,0.981627005099017));
#98722=DIRECTION('',(0.981627005099017,0.,0.190809912898503));
#98723=DIRECTION('',(-0.190809912898503,0.,0.981627005099017));
#98724=DIRECTION('',(0.981627005099017,0.,0.190809912898503));
#98725=DIRECTION('center_axis',(0.981627005099017,0.,0.190809912898503));
#98726=DIRECTION('ref_axis',(0.,-1.,0.));
#98727=DIRECTION('',(-0.190809912898503,0.,0.981627005099017));
#98728=DIRECTION('',(0.,-1.,0.));
#98729=DIRECTION('',(0.,-1.,0.));
#98730=DIRECTION('center_axis',(0.,-1.,0.));
#98731=DIRECTION('ref_axis',(0.,0.,-1.));
#98732=DIRECTION('',(-0.190809912898503,0.,0.981627005099017));
#98733=DIRECTION('',(-0.981627005099017,0.,-0.190809912898503));
#98734=DIRECTION('',(-0.981627005099017,0.,-0.190809912898503));
#98735=DIRECTION('center_axis',(-0.981627005099017,0.,-0.190809912898503));
#98736=DIRECTION('ref_axis',(-0.190809912898503,0.,0.981627005099017));
#98737=DIRECTION('',(0.,1.,0.));
#98738=DIRECTION('',(0.,1.,0.));
#98739=DIRECTION('center_axis',(0.,1.,0.));
#98740=DIRECTION('ref_axis',(1.,0.,0.));
#98741=DIRECTION('',(-0.190809912898503,0.,0.981627005099017));
#98742=DIRECTION('',(0.981627005099017,0.,0.190809912898503));
#98743=DIRECTION('',(-0.190809912898503,0.,0.981627005099017));
#98744=DIRECTION('',(0.981627005099017,0.,0.190809912898503));
#98745=DIRECTION('center_axis',(0.981627005099017,0.,0.190809912898503));
#98746=DIRECTION('ref_axis',(0.,-1.,0.));
#98747=DIRECTION('',(-0.190809912898503,0.,0.981627005099017));
#98748=DIRECTION('',(0.,-1.,0.));
#98749=DIRECTION('',(0.,-1.,0.));
#98750=DIRECTION('center_axis',(0.,-1.,0.));
#98751=DIRECTION('ref_axis',(0.,0.,-1.));
#98752=DIRECTION('',(-0.190809912898503,0.,0.981627005099017));
#98753=DIRECTION('',(-0.981627005099017,0.,-0.190809912898503));
#98754=DIRECTION('',(-0.981627005099017,0.,-0.190809912898503));
#98755=DIRECTION('center_axis',(-0.981627005099017,0.,-0.190809912898503));
#98756=DIRECTION('ref_axis',(-0.190809912898503,0.,0.981627005099017));
#98757=DIRECTION('',(0.,1.,0.));
#98758=DIRECTION('',(0.,1.,0.));
#98759=DIRECTION('center_axis',(0.,1.,0.));
#98760=DIRECTION('ref_axis',(1.,0.,0.));
#98761=DIRECTION('',(-0.190809912898503,0.,0.981627005099017));
#98762=DIRECTION('',(0.981627005099017,0.,0.190809912898503));
#98763=DIRECTION('',(-0.190809912898503,0.,0.981627005099017));
#98764=DIRECTION('',(0.981627005099017,0.,0.190809912898503));
#98765=DIRECTION('center_axis',(0.981627005099017,0.,0.190809912898503));
#98766=DIRECTION('ref_axis',(0.,-1.,0.));
#98767=DIRECTION('',(-0.190809912898503,0.,0.981627005099017));
#98768=DIRECTION('',(0.,-1.,0.));
#98769=DIRECTION('',(0.,-1.,0.));
#98770=DIRECTION('center_axis',(0.,-1.,0.));
#98771=DIRECTION('ref_axis',(0.,0.,-1.));
#98772=DIRECTION('',(-0.190809912898503,0.,0.981627005099017));
#98773=DIRECTION('',(-0.981627005099017,0.,-0.190809912898503));
#98774=DIRECTION('',(-0.981627005099017,0.,-0.190809912898503));
#98775=DIRECTION('center_axis',(-0.981627005099017,0.,-0.190809912898503));
#98776=DIRECTION('ref_axis',(-0.190809912898503,0.,0.981627005099017));
#98777=DIRECTION('',(0.,1.,0.));
#98778=DIRECTION('',(0.,1.,0.));
#98779=DIRECTION('center_axis',(0.,1.,0.));
#98780=DIRECTION('ref_axis',(1.,0.,0.));
#98781=DIRECTION('',(-0.190809912898503,0.,0.981627005099017));
#98782=DIRECTION('',(0.981627005099017,0.,0.190809912898503));
#98783=DIRECTION('',(-0.190809912898503,0.,0.981627005099017));
#98784=DIRECTION('',(0.981627005099017,0.,0.190809912898503));
#98785=DIRECTION('center_axis',(0.981627005099017,0.,0.190809912898503));
#98786=DIRECTION('ref_axis',(0.,-1.,0.));
#98787=DIRECTION('',(-0.190809912898503,0.,0.981627005099017));
#98788=DIRECTION('',(0.,-1.,0.));
#98789=DIRECTION('',(0.,-1.,0.));
#98790=DIRECTION('center_axis',(0.,-1.,0.));
#98791=DIRECTION('ref_axis',(0.,0.,-1.));
#98792=DIRECTION('',(-0.190809912898503,0.,0.981627005099017));
#98793=DIRECTION('',(-0.981627005099017,0.,-0.190809912898503));
#98794=DIRECTION('',(-0.981627005099017,0.,-0.190809912898503));
#98795=DIRECTION('center_axis',(-0.981627005099017,0.,-0.190809912898503));
#98796=DIRECTION('ref_axis',(-0.190809912898503,0.,0.981627005099017));
#98797=DIRECTION('',(0.,1.,0.));
#98798=DIRECTION('',(0.,1.,0.));
#98799=DIRECTION('center_axis',(0.,1.,0.));
#98800=DIRECTION('ref_axis',(1.,0.,0.));
#98801=DIRECTION('',(-0.190809912898503,0.,0.981627005099017));
#98802=DIRECTION('',(0.981627005099017,0.,0.190809912898503));
#98803=DIRECTION('',(-0.190809912898503,0.,0.981627005099017));
#98804=DIRECTION('',(0.981627005099017,0.,0.190809912898503));
#98805=DIRECTION('center_axis',(0.981627005099017,0.,0.190809912898503));
#98806=DIRECTION('ref_axis',(0.,-1.,0.));
#98807=DIRECTION('',(-0.190809912898503,0.,0.981627005099017));
#98808=DIRECTION('',(0.,-1.,0.));
#98809=DIRECTION('',(0.,-1.,0.));
#98810=DIRECTION('center_axis',(0.,-1.,0.));
#98811=DIRECTION('ref_axis',(0.,0.,-1.));
#98812=DIRECTION('',(-0.190809912898503,0.,0.981627005099017));
#98813=DIRECTION('',(-0.981627005099017,0.,-0.190809912898503));
#98814=DIRECTION('',(-0.981627005099017,0.,-0.190809912898503));
#98815=DIRECTION('center_axis',(-0.981627005099017,0.,-0.190809912898503));
#98816=DIRECTION('ref_axis',(-0.190809912898503,0.,0.981627005099017));
#98817=DIRECTION('',(0.,1.,0.));
#98818=DIRECTION('',(0.,1.,0.));
#98819=DIRECTION('center_axis',(0.,1.,0.));
#98820=DIRECTION('ref_axis',(1.,0.,0.));
#98821=DIRECTION('',(-0.190809912898503,0.,0.981627005099017));
#98822=DIRECTION('',(0.981627005099017,0.,0.190809912898503));
#98823=DIRECTION('',(-0.190809912898503,0.,0.981627005099017));
#98824=DIRECTION('',(0.981627005099017,0.,0.190809912898503));
#98825=DIRECTION('center_axis',(0.981627005099017,0.,0.190809912898503));
#98826=DIRECTION('ref_axis',(0.,-1.,0.));
#98827=DIRECTION('',(-0.190809912898503,0.,0.981627005099017));
#98828=DIRECTION('',(0.,-1.,0.));
#98829=DIRECTION('',(0.,-1.,0.));
#98830=DIRECTION('center_axis',(0.,-1.,0.));
#98831=DIRECTION('ref_axis',(0.,0.,-1.));
#98832=DIRECTION('',(-0.190809912898503,0.,0.981627005099017));
#98833=DIRECTION('',(-0.981627005099017,0.,-0.190809912898503));
#98834=DIRECTION('',(-0.981627005099017,0.,-0.190809912898503));
#98835=DIRECTION('center_axis',(-0.981627005099017,0.,-0.190809912898503));
#98836=DIRECTION('ref_axis',(-0.190809912898503,0.,0.981627005099017));
#98837=DIRECTION('',(0.,1.,0.));
#98838=DIRECTION('',(0.,1.,0.));
#98839=DIRECTION('center_axis',(0.,1.,0.));
#98840=DIRECTION('ref_axis',(1.,0.,0.));
#98841=DIRECTION('',(-0.190809912898503,0.,0.981627005099017));
#98842=DIRECTION('',(0.981627005099017,0.,0.190809912898503));
#98843=DIRECTION('',(-0.190809912898503,0.,0.981627005099017));
#98844=DIRECTION('',(0.981627005099017,0.,0.190809912898503));
#98845=DIRECTION('center_axis',(0.981627005099017,0.,0.190809912898503));
#98846=DIRECTION('ref_axis',(0.,-1.,0.));
#98847=DIRECTION('',(-0.190809912898503,0.,0.981627005099017));
#98848=DIRECTION('',(0.,-1.,0.));
#98849=DIRECTION('',(0.,-1.,0.));
#98850=DIRECTION('center_axis',(0.,-1.,0.));
#98851=DIRECTION('ref_axis',(0.,0.,-1.));
#98852=DIRECTION('',(-0.190809912898503,0.,0.981627005099017));
#98853=DIRECTION('',(-0.981627005099017,0.,-0.190809912898503));
#98854=DIRECTION('',(-0.981627005099017,0.,-0.190809912898503));
#98855=DIRECTION('center_axis',(-0.981627005099017,0.,-0.190809912898503));
#98856=DIRECTION('ref_axis',(-0.190809912898503,0.,0.981627005099017));
#98857=DIRECTION('',(0.,1.,0.));
#98858=DIRECTION('',(0.,1.,0.));
#98859=DIRECTION('center_axis',(0.,1.,0.));
#98860=DIRECTION('ref_axis',(1.,0.,0.));
#98861=DIRECTION('',(-0.190809912898503,0.,0.981627005099017));
#98862=DIRECTION('',(0.981627005099017,0.,0.190809912898503));
#98863=DIRECTION('',(-0.190809912898503,0.,0.981627005099017));
#98864=DIRECTION('',(0.981627005099017,0.,0.190809912898503));
#98865=DIRECTION('center_axis',(0.981627005099017,0.,0.190809912898503));
#98866=DIRECTION('ref_axis',(0.,-1.,0.));
#98867=DIRECTION('',(-0.190809912898503,0.,0.981627005099017));
#98868=DIRECTION('',(0.,-1.,0.));
#98869=DIRECTION('',(0.,-1.,0.));
#98870=DIRECTION('center_axis',(0.,-1.,0.));
#98871=DIRECTION('ref_axis',(0.,0.,-1.));
#98872=DIRECTION('',(-0.190809912898503,0.,0.981627005099017));
#98873=DIRECTION('',(-0.981627005099017,0.,-0.190809912898503));
#98874=DIRECTION('',(-0.981627005099017,0.,-0.190809912898503));
#98875=DIRECTION('center_axis',(-0.981627005099017,0.,-0.190809912898503));
#98876=DIRECTION('ref_axis',(-0.190809912898503,0.,0.981627005099017));
#98877=DIRECTION('',(0.,1.,0.));
#98878=DIRECTION('',(0.,1.,0.));
#98879=DIRECTION('center_axis',(0.,1.,0.));
#98880=DIRECTION('ref_axis',(1.,0.,0.));
#98881=DIRECTION('',(-0.190809912898503,0.,0.981627005099017));
#98882=DIRECTION('',(0.981627005099017,0.,0.190809912898503));
#98883=DIRECTION('',(-0.190809912898503,0.,0.981627005099017));
#98884=DIRECTION('',(0.981627005099017,0.,0.190809912898503));
#98885=DIRECTION('center_axis',(0.981627005099017,0.,0.190809912898503));
#98886=DIRECTION('ref_axis',(0.,-1.,0.));
#98887=DIRECTION('',(-0.190809912898503,0.,0.981627005099017));
#98888=DIRECTION('',(0.,-1.,0.));
#98889=DIRECTION('',(0.,-1.,0.));
#98890=DIRECTION('center_axis',(0.,-1.,0.));
#98891=DIRECTION('ref_axis',(0.,0.,-1.));
#98892=DIRECTION('',(-0.190809912898503,0.,0.981627005099017));
#98893=DIRECTION('',(-0.981627005099017,0.,-0.190809912898503));
#98894=DIRECTION('',(-0.981627005099017,0.,-0.190809912898503));
#98895=DIRECTION('center_axis',(-0.981627005099017,0.,-0.190809912898503));
#98896=DIRECTION('ref_axis',(-0.190809912898503,0.,0.981627005099017));
#98897=DIRECTION('',(0.,1.,0.));
#98898=DIRECTION('',(0.,1.,0.));
#98899=DIRECTION('center_axis',(0.,1.,0.));
#98900=DIRECTION('ref_axis',(1.,0.,0.));
#98901=DIRECTION('',(-0.190809912898503,0.,0.981627005099017));
#98902=DIRECTION('',(0.981627005099017,0.,0.190809912898503));
#98903=DIRECTION('',(-0.190809912898503,0.,0.981627005099017));
#98904=DIRECTION('',(0.981627005099017,0.,0.190809912898503));
#98905=DIRECTION('center_axis',(0.981627005099017,0.,0.190809912898503));
#98906=DIRECTION('ref_axis',(0.,-1.,0.));
#98907=DIRECTION('',(-0.190809912898503,0.,0.981627005099017));
#98908=DIRECTION('',(0.,-1.,0.));
#98909=DIRECTION('',(0.,-1.,0.));
#98910=DIRECTION('center_axis',(0.,-1.,0.));
#98911=DIRECTION('ref_axis',(0.,0.,-1.));
#98912=DIRECTION('',(-0.190809912898503,0.,0.981627005099017));
#98913=DIRECTION('',(-0.981627005099017,0.,-0.190809912898503));
#98914=DIRECTION('',(-0.981627005099017,0.,-0.190809912898503));
#98915=DIRECTION('center_axis',(-0.981627005099017,0.,-0.190809912898503));
#98916=DIRECTION('ref_axis',(-0.190809912898503,0.,0.981627005099017));
#98917=DIRECTION('',(0.,1.,0.));
#98918=DIRECTION('',(0.,1.,0.));
#98919=DIRECTION('center_axis',(0.,1.,0.));
#98920=DIRECTION('ref_axis',(1.,0.,0.));
#98921=DIRECTION('',(-0.190809912898503,0.,0.981627005099017));
#98922=DIRECTION('',(0.981627005099017,0.,0.190809912898503));
#98923=DIRECTION('',(-0.190809912898503,0.,0.981627005099017));
#98924=DIRECTION('',(0.981627005099017,0.,0.190809912898503));
#98925=DIRECTION('center_axis',(0.981627005099017,0.,0.190809912898503));
#98926=DIRECTION('ref_axis',(0.,-1.,0.));
#98927=DIRECTION('',(-0.190809912898503,0.,0.981627005099017));
#98928=DIRECTION('',(0.,-1.,0.));
#98929=DIRECTION('',(0.,-1.,0.));
#98930=DIRECTION('center_axis',(0.,-1.,0.));
#98931=DIRECTION('ref_axis',(0.,0.,-1.));
#98932=DIRECTION('',(-0.190809912898503,0.,0.981627005099017));
#98933=DIRECTION('',(-0.981627005099017,0.,-0.190809912898503));
#98934=DIRECTION('',(-0.981627005099017,0.,-0.190809912898503));
#98935=DIRECTION('center_axis',(-0.981627005099017,0.,-0.190809912898503));
#98936=DIRECTION('ref_axis',(-0.190809912898503,0.,0.981627005099017));
#98937=DIRECTION('',(0.,1.,0.));
#98938=DIRECTION('',(0.,1.,0.));
#98939=DIRECTION('center_axis',(0.,1.,0.));
#98940=DIRECTION('ref_axis',(1.,0.,0.));
#98941=DIRECTION('',(-0.190809912898503,0.,0.981627005099017));
#98942=DIRECTION('',(0.981627005099017,0.,0.190809912898503));
#98943=DIRECTION('',(-0.190809912898503,0.,0.981627005099017));
#98944=DIRECTION('',(0.981627005099017,0.,0.190809912898503));
#98945=DIRECTION('center_axis',(0.981627005099017,0.,0.190809912898503));
#98946=DIRECTION('ref_axis',(0.,-1.,0.));
#98947=DIRECTION('',(-0.190809912898503,0.,0.981627005099017));
#98948=DIRECTION('',(0.,-1.,0.));
#98949=DIRECTION('',(0.,-1.,0.));
#98950=DIRECTION('center_axis',(0.,-1.,0.));
#98951=DIRECTION('ref_axis',(0.,0.,-1.));
#98952=DIRECTION('',(-0.190809912898503,0.,0.981627005099017));
#98953=DIRECTION('',(-0.981627005099017,0.,-0.190809912898503));
#98954=DIRECTION('',(-0.981627005099017,0.,-0.190809912898503));
#98955=DIRECTION('center_axis',(-0.981627005099017,0.,-0.190809912898503));
#98956=DIRECTION('ref_axis',(-0.190809912898503,0.,0.981627005099017));
#98957=DIRECTION('',(0.,1.,0.));
#98958=DIRECTION('',(0.,1.,0.));
#98959=DIRECTION('center_axis',(0.,1.,0.));
#98960=DIRECTION('ref_axis',(1.,0.,0.));
#98961=DIRECTION('',(-0.190809912898503,0.,0.981627005099017));
#98962=DIRECTION('',(0.981627005099017,0.,0.190809912898503));
#98963=DIRECTION('',(-0.190809912898503,0.,0.981627005099017));
#98964=DIRECTION('',(0.981627005099017,0.,0.190809912898503));
#98965=DIRECTION('center_axis',(0.981627005099017,0.,0.190809912898503));
#98966=DIRECTION('ref_axis',(0.,-1.,0.));
#98967=DIRECTION('',(-0.190809912898503,0.,0.981627005099017));
#98968=DIRECTION('',(0.,-1.,0.));
#98969=DIRECTION('',(0.,-1.,0.));
#98970=DIRECTION('center_axis',(0.,-1.,0.));
#98971=DIRECTION('ref_axis',(0.,0.,-1.));
#98972=DIRECTION('',(-0.190809912898503,0.,0.981627005099017));
#98973=DIRECTION('',(-0.981627005099017,0.,-0.190809912898503));
#98974=DIRECTION('',(-0.981627005099017,0.,-0.190809912898503));
#98975=DIRECTION('center_axis',(-0.981627005099017,0.,-0.190809912898503));
#98976=DIRECTION('ref_axis',(-0.190809912898503,0.,0.981627005099017));
#98977=DIRECTION('',(0.,1.,0.));
#98978=DIRECTION('',(0.,1.,0.));
#98979=DIRECTION('center_axis',(0.,1.,0.));
#98980=DIRECTION('ref_axis',(1.,0.,0.));
#98981=DIRECTION('',(-0.190809912898503,0.,0.981627005099017));
#98982=DIRECTION('',(0.981627005099017,0.,0.190809912898503));
#98983=DIRECTION('',(-0.190809912898503,0.,0.981627005099017));
#98984=DIRECTION('',(0.981627005099017,0.,0.190809912898503));
#98985=DIRECTION('center_axis',(0.981627005099017,0.,0.190809912898503));
#98986=DIRECTION('ref_axis',(0.,-1.,0.));
#98987=DIRECTION('',(-0.190809912898503,0.,0.981627005099017));
#98988=DIRECTION('',(0.,-1.,0.));
#98989=DIRECTION('',(0.,-1.,0.));
#98990=DIRECTION('center_axis',(0.,-1.,0.));
#98991=DIRECTION('ref_axis',(0.,0.,-1.));
#98992=DIRECTION('',(-0.190809912898503,0.,0.981627005099017));
#98993=DIRECTION('',(-0.981627005099017,0.,-0.190809912898503));
#98994=DIRECTION('',(-0.981627005099017,0.,-0.190809912898503));
#98995=DIRECTION('center_axis',(-0.981627005099017,0.,-0.190809912898503));
#98996=DIRECTION('ref_axis',(-0.190809912898503,0.,0.981627005099017));
#98997=DIRECTION('',(0.,1.,0.));
#98998=DIRECTION('',(0.,1.,0.));
#98999=DIRECTION('center_axis',(0.,1.,0.));
#99000=DIRECTION('ref_axis',(1.,0.,0.));
#99001=DIRECTION('',(-0.190809912898503,0.,0.981627005099017));
#99002=DIRECTION('',(0.981627005099017,0.,0.190809912898503));
#99003=DIRECTION('',(-0.190809912898503,0.,0.981627005099017));
#99004=DIRECTION('',(0.981627005099017,0.,0.190809912898503));
#99005=DIRECTION('center_axis',(0.981627005099017,0.,0.190809912898503));
#99006=DIRECTION('ref_axis',(0.,-1.,0.));
#99007=DIRECTION('',(-0.190809912898503,0.,0.981627005099017));
#99008=DIRECTION('',(0.,-1.,0.));
#99009=DIRECTION('',(0.,-1.,0.));
#99010=DIRECTION('center_axis',(0.,-1.,0.));
#99011=DIRECTION('ref_axis',(0.,0.,-1.));
#99012=DIRECTION('',(-0.190809912898503,0.,0.981627005099017));
#99013=DIRECTION('',(-0.981627005099017,0.,-0.190809912898503));
#99014=DIRECTION('',(-0.981627005099017,0.,-0.190809912898503));
#99015=DIRECTION('center_axis',(-0.981627005099017,0.,-0.190809912898503));
#99016=DIRECTION('ref_axis',(-0.190809912898503,0.,0.981627005099017));
#99017=DIRECTION('',(0.,1.,0.));
#99018=DIRECTION('',(0.,1.,0.));
#99019=DIRECTION('center_axis',(0.,1.,0.));
#99020=DIRECTION('ref_axis',(1.,0.,0.));
#99021=DIRECTION('',(-0.190809912898503,0.,0.981627005099017));
#99022=DIRECTION('',(0.981627005099017,0.,0.190809912898503));
#99023=DIRECTION('',(-0.190809912898503,0.,0.981627005099017));
#99024=DIRECTION('',(0.981627005099017,0.,0.190809912898503));
#99025=DIRECTION('center_axis',(0.981627005099017,0.,0.190809912898503));
#99026=DIRECTION('ref_axis',(0.,-1.,0.));
#99027=DIRECTION('',(-0.190809912898503,0.,0.981627005099017));
#99028=DIRECTION('',(0.,-1.,0.));
#99029=DIRECTION('',(0.,-1.,0.));
#99030=DIRECTION('center_axis',(0.,-1.,0.));
#99031=DIRECTION('ref_axis',(0.,0.,-1.));
#99032=DIRECTION('',(-0.190809912898503,0.,0.981627005099017));
#99033=DIRECTION('',(-0.981627005099017,0.,-0.190809912898503));
#99034=DIRECTION('',(-0.981627005099017,0.,-0.190809912898503));
#99035=DIRECTION('center_axis',(-0.981627005099017,0.,-0.190809912898503));
#99036=DIRECTION('ref_axis',(-0.190809912898503,0.,0.981627005099017));
#99037=DIRECTION('',(0.,1.,0.));
#99038=DIRECTION('',(0.,1.,0.));
#99039=DIRECTION('center_axis',(0.,1.,0.));
#99040=DIRECTION('ref_axis',(1.,0.,0.));
#99041=DIRECTION('',(-0.190809912898503,0.,0.981627005099017));
#99042=DIRECTION('',(0.981627005099017,0.,0.190809912898503));
#99043=DIRECTION('',(-0.190809912898503,0.,0.981627005099017));
#99044=DIRECTION('',(0.981627005099017,0.,0.190809912898503));
#99045=DIRECTION('center_axis',(0.981627005099017,0.,0.190809912898503));
#99046=DIRECTION('ref_axis',(0.,-1.,0.));
#99047=DIRECTION('',(-0.190809912898503,0.,0.981627005099017));
#99048=DIRECTION('',(0.,-1.,0.));
#99049=DIRECTION('',(0.,-1.,0.));
#99050=DIRECTION('center_axis',(0.,-1.,0.));
#99051=DIRECTION('ref_axis',(0.,0.,-1.));
#99052=DIRECTION('',(-0.190809912898503,0.,0.981627005099017));
#99053=DIRECTION('',(-0.981627005099017,0.,-0.190809912898503));
#99054=DIRECTION('',(-0.981627005099017,0.,-0.190809912898503));
#99055=DIRECTION('center_axis',(-0.981627005099017,0.,-0.190809912898503));
#99056=DIRECTION('ref_axis',(-0.190809912898503,0.,0.981627005099017));
#99057=DIRECTION('',(0.,1.,0.));
#99058=DIRECTION('',(0.,1.,0.));
#99059=DIRECTION('center_axis',(0.,1.,0.));
#99060=DIRECTION('ref_axis',(1.,0.,0.));
#99061=DIRECTION('',(-0.190809912898503,0.,0.981627005099017));
#99062=DIRECTION('',(0.981627005099017,0.,0.190809912898503));
#99063=DIRECTION('',(-0.190809912898503,0.,0.981627005099017));
#99064=DIRECTION('',(0.981627005099017,0.,0.190809912898503));
#99065=DIRECTION('center_axis',(0.981627005099017,0.,0.190809912898503));
#99066=DIRECTION('ref_axis',(0.,-1.,0.));
#99067=DIRECTION('',(-0.190809912898503,0.,0.981627005099017));
#99068=DIRECTION('',(0.,-1.,0.));
#99069=DIRECTION('',(0.,-1.,0.));
#99070=DIRECTION('center_axis',(0.,-1.,0.));
#99071=DIRECTION('ref_axis',(0.,0.,-1.));
#99072=DIRECTION('',(-0.190809912898503,0.,0.981627005099017));
#99073=DIRECTION('',(-0.981627005099017,0.,-0.190809912898503));
#99074=DIRECTION('',(-0.981627005099017,0.,-0.190809912898503));
#99075=DIRECTION('center_axis',(-0.981627005099017,0.,-0.190809912898503));
#99076=DIRECTION('ref_axis',(-0.190809912898503,0.,0.981627005099017));
#99077=DIRECTION('',(0.,1.,0.));
#99078=DIRECTION('',(0.,1.,0.));
#99079=DIRECTION('center_axis',(0.,1.,0.));
#99080=DIRECTION('ref_axis',(1.,0.,0.));
#99081=DIRECTION('',(-0.190809912898503,0.,0.981627005099017));
#99082=DIRECTION('',(0.981627005099017,0.,0.190809912898503));
#99083=DIRECTION('',(-0.190809912898503,0.,0.981627005099017));
#99084=DIRECTION('',(0.981627005099017,0.,0.190809912898503));
#99085=DIRECTION('center_axis',(0.981627005099017,0.,0.190809912898503));
#99086=DIRECTION('ref_axis',(0.,-1.,0.));
#99087=DIRECTION('',(-0.190809912898503,0.,0.981627005099017));
#99088=DIRECTION('',(0.,-1.,0.));
#99089=DIRECTION('',(0.,-1.,0.));
#99090=DIRECTION('center_axis',(0.,-1.,0.));
#99091=DIRECTION('ref_axis',(0.,0.,-1.));
#99092=DIRECTION('',(-0.190809912898503,0.,0.981627005099017));
#99093=DIRECTION('',(-0.981627005099017,0.,-0.190809912898503));
#99094=DIRECTION('',(-0.981627005099017,0.,-0.190809912898503));
#99095=DIRECTION('center_axis',(-0.981627005099017,0.,-0.190809912898503));
#99096=DIRECTION('ref_axis',(-0.190809912898503,0.,0.981627005099017));
#99097=DIRECTION('',(0.,1.,0.));
#99098=DIRECTION('',(0.,1.,0.));
#99099=DIRECTION('center_axis',(0.,1.,0.));
#99100=DIRECTION('ref_axis',(1.,0.,0.));
#99101=DIRECTION('',(-0.190809912898503,0.,0.981627005099017));
#99102=DIRECTION('',(0.981627005099017,0.,0.190809912898503));
#99103=DIRECTION('',(-0.190809912898503,0.,0.981627005099017));
#99104=DIRECTION('',(0.981627005099017,0.,0.190809912898503));
#99105=DIRECTION('center_axis',(0.981627005099017,0.,0.190809912898503));
#99106=DIRECTION('ref_axis',(0.,-1.,0.));
#99107=DIRECTION('',(-0.190809912898503,0.,0.981627005099017));
#99108=DIRECTION('',(0.,-1.,0.));
#99109=DIRECTION('',(0.,-1.,0.));
#99110=DIRECTION('center_axis',(0.,-1.,0.));
#99111=DIRECTION('ref_axis',(0.,0.,-1.));
#99112=DIRECTION('',(-0.190809912898503,0.,0.981627005099017));
#99113=DIRECTION('',(-0.981627005099017,0.,-0.190809912898503));
#99114=DIRECTION('',(-0.981627005099017,0.,-0.190809912898503));
#99115=DIRECTION('center_axis',(-0.981627005099017,0.,-0.190809912898503));
#99116=DIRECTION('ref_axis',(-0.190809912898503,0.,0.981627005099017));
#99117=DIRECTION('',(0.,1.,0.));
#99118=DIRECTION('',(0.,1.,0.));
#99119=DIRECTION('center_axis',(0.,1.,0.));
#99120=DIRECTION('ref_axis',(1.,0.,0.));
#99121=DIRECTION('',(-0.190809912898503,0.,0.981627005099017));
#99122=DIRECTION('',(0.981627005099017,0.,0.190809912898503));
#99123=DIRECTION('',(-0.190809912898503,0.,0.981627005099017));
#99124=DIRECTION('',(0.981627005099017,0.,0.190809912898503));
#99125=DIRECTION('center_axis',(0.981627005099017,0.,0.190809912898503));
#99126=DIRECTION('ref_axis',(0.,-1.,0.));
#99127=DIRECTION('',(-0.190809912898503,0.,0.981627005099017));
#99128=DIRECTION('',(0.,-1.,0.));
#99129=DIRECTION('',(0.,-1.,0.));
#99130=DIRECTION('center_axis',(0.,-1.,0.));
#99131=DIRECTION('ref_axis',(0.,0.,-1.));
#99132=DIRECTION('',(-0.190809912898503,0.,0.981627005099017));
#99133=DIRECTION('',(-0.981627005099017,0.,-0.190809912898503));
#99134=DIRECTION('',(-0.981627005099017,0.,-0.190809912898503));
#99135=DIRECTION('center_axis',(-0.981627005099017,0.,-0.190809912898503));
#99136=DIRECTION('ref_axis',(-0.190809912898503,0.,0.981627005099017));
#99137=DIRECTION('',(0.,1.,0.));
#99138=DIRECTION('',(0.,1.,0.));
#99139=DIRECTION('center_axis',(0.,1.,0.));
#99140=DIRECTION('ref_axis',(1.,0.,0.));
#99141=DIRECTION('',(-0.190809912898503,0.,0.981627005099017));
#99142=DIRECTION('',(0.981627005099017,0.,0.190809912898503));
#99143=DIRECTION('',(-0.190809912898503,0.,0.981627005099017));
#99144=DIRECTION('',(0.981627005099017,0.,0.190809912898503));
#99145=DIRECTION('center_axis',(0.981627005099017,0.,0.190809912898503));
#99146=DIRECTION('ref_axis',(0.,-1.,0.));
#99147=DIRECTION('',(-0.190809912898503,0.,0.981627005099017));
#99148=DIRECTION('',(0.,-1.,0.));
#99149=DIRECTION('',(0.,-1.,0.));
#99150=DIRECTION('center_axis',(0.,-1.,0.));
#99151=DIRECTION('ref_axis',(0.,0.,-1.));
#99152=DIRECTION('',(-0.190809912898503,0.,0.981627005099017));
#99153=DIRECTION('',(-0.981627005099017,0.,-0.190809912898503));
#99154=DIRECTION('',(-0.981627005099017,0.,-0.190809912898503));
#99155=DIRECTION('center_axis',(-0.981627005099017,0.,-0.190809912898503));
#99156=DIRECTION('ref_axis',(-0.190809912898503,0.,0.981627005099017));
#99157=DIRECTION('',(0.,1.,0.));
#99158=DIRECTION('',(0.,1.,0.));
#99159=DIRECTION('center_axis',(0.,1.,0.));
#99160=DIRECTION('ref_axis',(1.,0.,0.));
#99161=DIRECTION('',(-0.190809912898503,0.,0.981627005099017));
#99162=DIRECTION('',(0.981627005099017,0.,0.190809912898503));
#99163=DIRECTION('',(-0.190809912898503,0.,0.981627005099017));
#99164=DIRECTION('',(0.981627005099017,0.,0.190809912898503));
#99165=DIRECTION('center_axis',(0.981627005099017,0.,0.190809912898503));
#99166=DIRECTION('ref_axis',(0.,-1.,0.));
#99167=DIRECTION('',(-0.190809912898503,0.,0.981627005099017));
#99168=DIRECTION('',(0.,-1.,0.));
#99169=DIRECTION('',(0.,-1.,0.));
#99170=DIRECTION('center_axis',(0.,-1.,0.));
#99171=DIRECTION('ref_axis',(0.,0.,-1.));
#99172=DIRECTION('',(-0.190809912898503,0.,0.981627005099017));
#99173=DIRECTION('',(-0.981627005099017,0.,-0.190809912898503));
#99174=DIRECTION('',(-0.981627005099017,0.,-0.190809912898503));
#99175=DIRECTION('center_axis',(-0.981627005099017,0.,-0.190809912898503));
#99176=DIRECTION('ref_axis',(-0.190809912898503,0.,0.981627005099017));
#99177=DIRECTION('',(0.,1.,0.));
#99178=DIRECTION('',(0.,1.,0.));
#99179=DIRECTION('center_axis',(0.,1.,0.));
#99180=DIRECTION('ref_axis',(1.,0.,0.));
#99181=DIRECTION('',(-0.190809912898503,0.,0.981627005099017));
#99182=DIRECTION('',(0.981627005099017,0.,0.190809912898503));
#99183=DIRECTION('',(-0.190809912898503,0.,0.981627005099017));
#99184=DIRECTION('',(0.981627005099017,0.,0.190809912898503));
#99185=DIRECTION('center_axis',(0.981627005099017,0.,0.190809912898503));
#99186=DIRECTION('ref_axis',(0.,-1.,0.));
#99187=DIRECTION('',(-0.190809912898503,0.,0.981627005099017));
#99188=DIRECTION('',(0.,-1.,0.));
#99189=DIRECTION('',(0.,-1.,0.));
#99190=DIRECTION('center_axis',(0.,-1.,0.));
#99191=DIRECTION('ref_axis',(0.,0.,-1.));
#99192=DIRECTION('',(-0.190809912898503,0.,0.981627005099017));
#99193=DIRECTION('',(-0.981627005099017,0.,-0.190809912898503));
#99194=DIRECTION('',(-0.981627005099017,0.,-0.190809912898503));
#99195=DIRECTION('center_axis',(-0.981627005099017,0.,-0.190809912898503));
#99196=DIRECTION('ref_axis',(-0.190809912898503,0.,0.981627005099017));
#99197=DIRECTION('',(0.,1.,0.));
#99198=DIRECTION('',(0.,1.,0.));
#99199=DIRECTION('center_axis',(0.,1.,0.));
#99200=DIRECTION('ref_axis',(1.,0.,0.));
#99201=DIRECTION('',(-0.190809912898503,0.,0.981627005099017));
#99202=DIRECTION('',(0.981627005099017,0.,0.190809912898503));
#99203=DIRECTION('',(-0.190809912898503,0.,0.981627005099017));
#99204=DIRECTION('',(0.981627005099017,0.,0.190809912898503));
#99205=DIRECTION('center_axis',(0.981627005099017,0.,0.190809912898503));
#99206=DIRECTION('ref_axis',(0.,-1.,0.));
#99207=DIRECTION('',(-0.190809912898503,0.,0.981627005099017));
#99208=DIRECTION('',(0.,-1.,0.));
#99209=DIRECTION('',(0.,-1.,0.));
#99210=DIRECTION('center_axis',(0.,-1.,0.));
#99211=DIRECTION('ref_axis',(0.,0.,-1.));
#99212=DIRECTION('',(-0.190809912898503,0.,0.981627005099017));
#99213=DIRECTION('',(-0.981627005099017,0.,-0.190809912898503));
#99214=DIRECTION('',(-0.981627005099017,0.,-0.190809912898503));
#99215=DIRECTION('center_axis',(-0.981627005099017,0.,-0.190809912898503));
#99216=DIRECTION('ref_axis',(-0.190809912898503,0.,0.981627005099017));
#99217=DIRECTION('',(0.,1.,0.));
#99218=DIRECTION('',(0.,1.,0.));
#99219=DIRECTION('center_axis',(0.,1.,0.));
#99220=DIRECTION('ref_axis',(1.,0.,0.));
#99221=DIRECTION('',(-0.190809912898503,0.,0.981627005099017));
#99222=DIRECTION('',(0.981627005099017,0.,0.190809912898503));
#99223=DIRECTION('',(-0.190809912898503,0.,0.981627005099017));
#99224=DIRECTION('',(0.981627005099017,0.,0.190809912898503));
#99225=DIRECTION('center_axis',(0.981627005099017,0.,0.190809912898503));
#99226=DIRECTION('ref_axis',(0.,-1.,0.));
#99227=DIRECTION('',(-0.190809912898503,0.,0.981627005099017));
#99228=DIRECTION('',(0.,-1.,0.));
#99229=DIRECTION('',(0.,-1.,0.));
#99230=DIRECTION('center_axis',(0.,-1.,0.));
#99231=DIRECTION('ref_axis',(0.,0.,-1.));
#99232=DIRECTION('',(-0.190809912898503,0.,0.981627005099017));
#99233=DIRECTION('',(-0.981627005099017,0.,-0.190809912898503));
#99234=DIRECTION('',(-0.981627005099017,0.,-0.190809912898503));
#99235=DIRECTION('center_axis',(-0.981627005099017,0.,-0.190809912898503));
#99236=DIRECTION('ref_axis',(-0.190809912898503,0.,0.981627005099017));
#99237=DIRECTION('',(0.,1.,0.));
#99238=DIRECTION('',(0.,1.,0.));
#99239=DIRECTION('center_axis',(0.,1.,0.));
#99240=DIRECTION('ref_axis',(1.,0.,0.));
#99241=DIRECTION('',(-0.190809912898503,0.,0.981627005099017));
#99242=DIRECTION('',(0.981627005099017,0.,0.190809912898503));
#99243=DIRECTION('',(-0.190809912898503,0.,0.981627005099017));
#99244=DIRECTION('',(0.981627005099017,0.,0.190809912898503));
#99245=DIRECTION('center_axis',(0.981627005099017,0.,0.190809912898503));
#99246=DIRECTION('ref_axis',(0.,-1.,0.));
#99247=DIRECTION('',(-0.190809912898503,0.,0.981627005099017));
#99248=DIRECTION('',(0.,-1.,0.));
#99249=DIRECTION('',(0.,-1.,0.));
#99250=DIRECTION('center_axis',(0.,-1.,0.));
#99251=DIRECTION('ref_axis',(0.,0.,-1.));
#99252=DIRECTION('',(-0.190809912898503,0.,0.981627005099017));
#99253=DIRECTION('',(-0.981627005099017,0.,-0.190809912898503));
#99254=DIRECTION('',(-0.981627005099017,0.,-0.190809912898503));
#99255=DIRECTION('center_axis',(-0.981627005099017,0.,-0.190809912898503));
#99256=DIRECTION('ref_axis',(-0.190809912898503,0.,0.981627005099017));
#99257=DIRECTION('',(0.,1.,0.));
#99258=DIRECTION('',(0.,1.,0.));
#99259=DIRECTION('center_axis',(0.,1.,0.));
#99260=DIRECTION('ref_axis',(1.,0.,0.));
#99261=DIRECTION('',(-0.190809912898503,0.,0.981627005099017));
#99262=DIRECTION('',(0.981627005099017,0.,0.190809912898503));
#99263=DIRECTION('',(-0.190809912898503,0.,0.981627005099017));
#99264=DIRECTION('',(0.981627005099017,0.,0.190809912898503));
#99265=DIRECTION('center_axis',(0.981627005099017,0.,0.190809912898503));
#99266=DIRECTION('ref_axis',(0.,-1.,0.));
#99267=DIRECTION('',(-0.190809912898503,0.,0.981627005099017));
#99268=DIRECTION('',(0.,-1.,0.));
#99269=DIRECTION('',(0.,-1.,0.));
#99270=DIRECTION('center_axis',(0.,-1.,0.));
#99271=DIRECTION('ref_axis',(0.,0.,-1.));
#99272=DIRECTION('',(-0.190809912898503,0.,0.981627005099017));
#99273=DIRECTION('',(-0.981627005099017,0.,-0.190809912898503));
#99274=DIRECTION('',(-0.981627005099017,0.,-0.190809912898503));
#99275=DIRECTION('center_axis',(-0.981627005099017,0.,-0.190809912898503));
#99276=DIRECTION('ref_axis',(-0.190809912898503,0.,0.981627005099017));
#99277=DIRECTION('',(0.,1.,0.));
#99278=DIRECTION('',(0.,1.,0.));
#99279=DIRECTION('center_axis',(0.,1.,0.));
#99280=DIRECTION('ref_axis',(1.,0.,0.));
#99281=DIRECTION('',(-0.190809912898503,0.,0.981627005099017));
#99282=DIRECTION('',(0.981627005099017,0.,0.190809912898503));
#99283=DIRECTION('',(-0.190809912898503,0.,0.981627005099017));
#99284=DIRECTION('',(0.981627005099017,0.,0.190809912898503));
#99285=DIRECTION('center_axis',(0.981627005099017,0.,0.190809912898503));
#99286=DIRECTION('ref_axis',(0.,-1.,0.));
#99287=DIRECTION('',(-0.190809912898503,0.,0.981627005099017));
#99288=DIRECTION('',(0.,-1.,0.));
#99289=DIRECTION('',(0.,-1.,0.));
#99290=DIRECTION('center_axis',(0.,-1.,0.));
#99291=DIRECTION('ref_axis',(0.,0.,-1.));
#99292=DIRECTION('',(-0.190809912898503,0.,0.981627005099017));
#99293=DIRECTION('',(-0.981627005099017,0.,-0.190809912898503));
#99294=DIRECTION('',(-0.981627005099017,0.,-0.190809912898503));
#99295=DIRECTION('center_axis',(-0.981627005099017,0.,-0.190809912898503));
#99296=DIRECTION('ref_axis',(-0.190809912898503,0.,0.981627005099017));
#99297=DIRECTION('',(0.,1.,0.));
#99298=DIRECTION('',(0.,1.,0.));
#99299=DIRECTION('center_axis',(0.,1.,0.));
#99300=DIRECTION('ref_axis',(1.,0.,0.));
#99301=DIRECTION('',(-0.190809912898503,0.,0.981627005099017));
#99302=DIRECTION('',(0.981627005099017,0.,0.190809912898503));
#99303=DIRECTION('',(-0.190809912898503,0.,0.981627005099017));
#99304=DIRECTION('',(0.981627005099017,0.,0.190809912898503));
#99305=DIRECTION('center_axis',(0.981627005099017,0.,0.190809912898503));
#99306=DIRECTION('ref_axis',(0.,-1.,0.));
#99307=DIRECTION('',(-0.190809912898503,0.,0.981627005099017));
#99308=DIRECTION('',(0.,-1.,0.));
#99309=DIRECTION('',(0.,-1.,0.));
#99310=DIRECTION('center_axis',(0.,-1.,0.));
#99311=DIRECTION('ref_axis',(0.,0.,-1.));
#99312=DIRECTION('',(-0.190809912898503,0.,0.981627005099017));
#99313=DIRECTION('',(-0.981627005099017,0.,-0.190809912898503));
#99314=DIRECTION('',(-0.981627005099017,0.,-0.190809912898503));
#99315=DIRECTION('center_axis',(-0.981627005099017,0.,-0.190809912898503));
#99316=DIRECTION('ref_axis',(-0.190809912898503,0.,0.981627005099017));
#99317=DIRECTION('',(0.,1.,0.));
#99318=DIRECTION('',(0.,1.,0.));
#99319=DIRECTION('center_axis',(0.,1.,0.));
#99320=DIRECTION('ref_axis',(1.,0.,0.));
#99321=DIRECTION('',(-0.190809912898503,0.,0.981627005099017));
#99322=DIRECTION('',(0.981627005099017,0.,0.190809912898503));
#99323=DIRECTION('',(-0.190809912898503,0.,0.981627005099017));
#99324=DIRECTION('',(0.981627005099017,0.,0.190809912898503));
#99325=DIRECTION('center_axis',(0.981627005099017,0.,0.190809912898503));
#99326=DIRECTION('ref_axis',(0.,-1.,0.));
#99327=DIRECTION('',(-0.190809912898503,0.,0.981627005099017));
#99328=DIRECTION('',(0.,-1.,0.));
#99329=DIRECTION('',(0.,-1.,0.));
#99330=DIRECTION('center_axis',(0.,-1.,0.));
#99331=DIRECTION('ref_axis',(0.,0.,-1.));
#99332=DIRECTION('',(-0.190809912898503,0.,0.981627005099017));
#99333=DIRECTION('',(-0.981627005099017,0.,-0.190809912898503));
#99334=DIRECTION('',(-0.981627005099017,0.,-0.190809912898503));
#99335=DIRECTION('center_axis',(-0.981627005099017,0.,-0.190809912898503));
#99336=DIRECTION('ref_axis',(-0.190809912898503,0.,0.981627005099017));
#99337=DIRECTION('',(0.,1.,0.));
#99338=DIRECTION('',(0.,1.,0.));
#99339=DIRECTION('center_axis',(0.,1.,0.));
#99340=DIRECTION('ref_axis',(1.,0.,0.));
#99341=DIRECTION('',(-0.190809912898503,0.,0.981627005099017));
#99342=DIRECTION('',(0.981627005099017,0.,0.190809912898503));
#99343=DIRECTION('',(-0.190809912898503,0.,0.981627005099017));
#99344=DIRECTION('',(0.981627005099017,0.,0.190809912898503));
#99345=DIRECTION('center_axis',(0.981627005099017,0.,0.190809912898503));
#99346=DIRECTION('ref_axis',(0.,-1.,0.));
#99347=DIRECTION('',(-0.190809912898503,0.,0.981627005099017));
#99348=DIRECTION('',(0.,-1.,0.));
#99349=DIRECTION('',(0.,-1.,0.));
#99350=DIRECTION('center_axis',(0.,-1.,0.));
#99351=DIRECTION('ref_axis',(0.,0.,-1.));
#99352=DIRECTION('',(-0.190809912898503,0.,0.981627005099017));
#99353=DIRECTION('',(-0.981627005099017,0.,-0.190809912898503));
#99354=DIRECTION('',(-0.981627005099017,0.,-0.190809912898503));
#99355=DIRECTION('center_axis',(-0.981627005099017,0.,-0.190809912898503));
#99356=DIRECTION('ref_axis',(-0.190809912898503,0.,0.981627005099017));
#99357=DIRECTION('',(0.,1.,0.));
#99358=DIRECTION('',(0.,1.,0.));
#99359=DIRECTION('center_axis',(0.,1.,0.));
#99360=DIRECTION('ref_axis',(1.,0.,0.));
#99361=DIRECTION('',(-0.190809912898503,0.,0.981627005099017));
#99362=DIRECTION('',(0.981627005099017,0.,0.190809912898503));
#99363=DIRECTION('',(-0.190809912898503,0.,0.981627005099017));
#99364=DIRECTION('',(0.981627005099017,0.,0.190809912898503));
#99365=DIRECTION('center_axis',(0.981627005099017,0.,0.190809912898503));
#99366=DIRECTION('ref_axis',(0.,-1.,0.));
#99367=DIRECTION('',(-0.190809912898503,0.,0.981627005099017));
#99368=DIRECTION('',(0.,-1.,0.));
#99369=DIRECTION('',(0.,-1.,0.));
#99370=DIRECTION('center_axis',(0.,-1.,0.));
#99371=DIRECTION('ref_axis',(0.,0.,-1.));
#99372=DIRECTION('',(-0.190809912898503,0.,0.981627005099017));
#99373=DIRECTION('',(-0.981627005099017,0.,-0.190809912898503));
#99374=DIRECTION('',(-0.981627005099017,0.,-0.190809912898503));
#99375=DIRECTION('center_axis',(-0.981627005099017,0.,-0.190809912898503));
#99376=DIRECTION('ref_axis',(-0.190809912898503,0.,0.981627005099017));
#99377=DIRECTION('',(0.,1.,0.));
#99378=DIRECTION('',(0.,1.,0.));
#99379=DIRECTION('center_axis',(0.,1.,0.));
#99380=DIRECTION('ref_axis',(1.,0.,0.));
#99381=DIRECTION('',(-0.190809912898503,0.,0.981627005099017));
#99382=DIRECTION('',(0.981627005099017,0.,0.190809912898503));
#99383=DIRECTION('',(-0.190809912898503,0.,0.981627005099017));
#99384=DIRECTION('',(0.981627005099017,0.,0.190809912898503));
#99385=DIRECTION('center_axis',(0.981627005099017,0.,0.190809912898503));
#99386=DIRECTION('ref_axis',(0.,-1.,0.));
#99387=DIRECTION('',(-0.190809912898503,0.,0.981627005099017));
#99388=DIRECTION('',(0.,-1.,0.));
#99389=DIRECTION('',(0.,-1.,0.));
#99390=DIRECTION('center_axis',(0.,-1.,0.));
#99391=DIRECTION('ref_axis',(0.,0.,-1.));
#99392=DIRECTION('',(-0.190809912898503,0.,0.981627005099017));
#99393=DIRECTION('',(-0.981627005099017,0.,-0.190809912898503));
#99394=DIRECTION('',(-0.981627005099017,0.,-0.190809912898503));
#99395=DIRECTION('center_axis',(-0.981627005099017,0.,-0.190809912898503));
#99396=DIRECTION('ref_axis',(-0.190809912898503,0.,0.981627005099017));
#99397=DIRECTION('',(0.,1.,0.));
#99398=DIRECTION('',(0.,1.,0.));
#99399=DIRECTION('center_axis',(0.,1.,0.));
#99400=DIRECTION('ref_axis',(1.,0.,0.));
#99401=DIRECTION('',(-0.190809912898503,0.,0.981627005099017));
#99402=DIRECTION('',(0.981627005099017,0.,0.190809912898503));
#99403=DIRECTION('',(-0.190809912898503,0.,0.981627005099017));
#99404=DIRECTION('',(0.981627005099017,0.,0.190809912898503));
#99405=DIRECTION('center_axis',(0.981627005099017,0.,0.190809912898503));
#99406=DIRECTION('ref_axis',(0.,-1.,0.));
#99407=DIRECTION('',(-0.190809912898503,0.,0.981627005099017));
#99408=DIRECTION('',(0.,-1.,0.));
#99409=DIRECTION('',(0.,-1.,0.));
#99410=DIRECTION('center_axis',(0.,-1.,0.));
#99411=DIRECTION('ref_axis',(0.,0.,-1.));
#99412=DIRECTION('',(-0.190809912898503,0.,0.981627005099017));
#99413=DIRECTION('',(-0.981627005099017,0.,-0.190809912898503));
#99414=DIRECTION('',(-0.981627005099017,0.,-0.190809912898503));
#99415=DIRECTION('center_axis',(-0.981627005099017,0.,-0.190809912898503));
#99416=DIRECTION('ref_axis',(-0.190809912898503,0.,0.981627005099017));
#99417=DIRECTION('',(0.,1.,0.));
#99418=DIRECTION('',(0.,1.,0.));
#99419=DIRECTION('center_axis',(0.,1.,0.));
#99420=DIRECTION('ref_axis',(1.,0.,0.));
#99421=DIRECTION('',(-0.190809912898503,0.,0.981627005099017));
#99422=DIRECTION('',(0.981627005099017,0.,0.190809912898503));
#99423=DIRECTION('',(-0.190809912898503,0.,0.981627005099017));
#99424=DIRECTION('',(0.981627005099017,0.,0.190809912898503));
#99425=DIRECTION('center_axis',(0.981627005099017,0.,0.190809912898503));
#99426=DIRECTION('ref_axis',(0.,-1.,0.));
#99427=DIRECTION('',(-0.190809912898503,0.,0.981627005099017));
#99428=DIRECTION('',(0.,-1.,0.));
#99429=DIRECTION('',(0.,-1.,0.));
#99430=DIRECTION('center_axis',(0.,-1.,0.));
#99431=DIRECTION('ref_axis',(0.,0.,-1.));
#99432=DIRECTION('',(-0.190809912898503,0.,0.981627005099017));
#99433=DIRECTION('',(-0.981627005099017,0.,-0.190809912898503));
#99434=DIRECTION('',(-0.981627005099017,0.,-0.190809912898503));
#99435=DIRECTION('center_axis',(-0.981627005099017,0.,-0.190809912898503));
#99436=DIRECTION('ref_axis',(-0.190809912898503,0.,0.981627005099017));
#99437=DIRECTION('',(0.,1.,0.));
#99438=DIRECTION('',(0.,1.,0.));
#99439=DIRECTION('center_axis',(0.,1.,0.));
#99440=DIRECTION('ref_axis',(1.,0.,0.));
#99441=DIRECTION('',(-0.190809912898503,0.,0.981627005099017));
#99442=DIRECTION('',(0.981627005099017,0.,0.190809912898503));
#99443=DIRECTION('',(-0.190809912898503,0.,0.981627005099017));
#99444=DIRECTION('',(0.981627005099017,0.,0.190809912898503));
#99445=DIRECTION('center_axis',(0.981627005099017,0.,0.190809912898503));
#99446=DIRECTION('ref_axis',(0.,-1.,0.));
#99447=DIRECTION('',(-0.190809912898503,0.,0.981627005099017));
#99448=DIRECTION('',(0.,-1.,0.));
#99449=DIRECTION('',(0.,-1.,0.));
#99450=DIRECTION('center_axis',(0.,-1.,0.));
#99451=DIRECTION('ref_axis',(0.,0.,-1.));
#99452=DIRECTION('',(-0.190809912898503,0.,0.981627005099017));
#99453=DIRECTION('',(-0.981627005099017,0.,-0.190809912898503));
#99454=DIRECTION('',(-0.981627005099017,0.,-0.190809912898503));
#99455=DIRECTION('center_axis',(-0.981627005099017,0.,-0.190809912898503));
#99456=DIRECTION('ref_axis',(-0.190809912898503,0.,0.981627005099017));
#99457=DIRECTION('',(0.,1.,0.));
#99458=DIRECTION('',(0.,1.,0.));
#99459=DIRECTION('center_axis',(0.,1.,0.));
#99460=DIRECTION('ref_axis',(1.,0.,0.));
#99461=DIRECTION('',(-0.190809912898503,0.,0.981627005099017));
#99462=DIRECTION('',(0.981627005099017,0.,0.190809912898503));
#99463=DIRECTION('',(-0.190809912898503,0.,0.981627005099017));
#99464=DIRECTION('',(0.981627005099017,0.,0.190809912898503));
#99465=DIRECTION('center_axis',(0.981627005099017,0.,0.190809912898503));
#99466=DIRECTION('ref_axis',(0.,-1.,0.));
#99467=DIRECTION('',(-0.190809912898503,0.,0.981627005099017));
#99468=DIRECTION('',(0.,-1.,0.));
#99469=DIRECTION('',(0.,-1.,0.));
#99470=DIRECTION('center_axis',(0.,-1.,0.));
#99471=DIRECTION('ref_axis',(0.,0.,-1.));
#99472=DIRECTION('',(-0.190809912898503,0.,0.981627005099017));
#99473=DIRECTION('',(-0.981627005099017,0.,-0.190809912898503));
#99474=DIRECTION('',(-0.981627005099017,0.,-0.190809912898503));
#99475=DIRECTION('center_axis',(-0.981627005099017,0.,-0.190809912898503));
#99476=DIRECTION('ref_axis',(-0.190809912898503,0.,0.981627005099017));
#99477=DIRECTION('',(0.,1.,0.));
#99478=DIRECTION('',(0.,1.,0.));
#99479=DIRECTION('center_axis',(0.,1.,0.));
#99480=DIRECTION('ref_axis',(1.,0.,0.));
#99481=DIRECTION('',(-0.190809912898503,0.,0.981627005099017));
#99482=DIRECTION('',(0.981627005099017,0.,0.190809912898503));
#99483=DIRECTION('',(-0.190809912898503,0.,0.981627005099017));
#99484=DIRECTION('',(0.981627005099017,0.,0.190809912898503));
#99485=DIRECTION('center_axis',(0.981627005099017,0.,0.190809912898503));
#99486=DIRECTION('ref_axis',(0.,-1.,0.));
#99487=DIRECTION('',(-0.190809912898503,0.,0.981627005099017));
#99488=DIRECTION('',(0.,-1.,0.));
#99489=DIRECTION('',(0.,-1.,0.));
#99490=DIRECTION('center_axis',(0.,-1.,0.));
#99491=DIRECTION('ref_axis',(0.,0.,-1.));
#99492=DIRECTION('',(-0.190809912898503,0.,0.981627005099017));
#99493=DIRECTION('',(-0.981627005099017,0.,-0.190809912898503));
#99494=DIRECTION('',(-0.981627005099017,0.,-0.190809912898503));
#99495=DIRECTION('center_axis',(-0.981627005099017,0.,-0.190809912898503));
#99496=DIRECTION('ref_axis',(-0.190809912898503,0.,0.981627005099017));
#99497=DIRECTION('',(0.,1.,0.));
#99498=DIRECTION('',(0.,1.,0.));
#99499=DIRECTION('center_axis',(0.,1.,0.));
#99500=DIRECTION('ref_axis',(1.,0.,0.));
#99501=DIRECTION('',(-0.190809912898503,0.,0.981627005099017));
#99502=DIRECTION('',(0.981627005099017,0.,0.190809912898503));
#99503=DIRECTION('',(-0.190809912898503,0.,0.981627005099017));
#99504=DIRECTION('',(0.981627005099017,0.,0.190809912898503));
#99505=DIRECTION('center_axis',(0.981627005099017,0.,0.190809912898503));
#99506=DIRECTION('ref_axis',(0.,-1.,0.));
#99507=DIRECTION('',(-0.190809912898503,0.,0.981627005099017));
#99508=DIRECTION('',(0.,-1.,0.));
#99509=DIRECTION('',(0.,-1.,0.));
#99510=DIRECTION('center_axis',(0.,-1.,0.));
#99511=DIRECTION('ref_axis',(0.,0.,-1.));
#99512=DIRECTION('',(-0.190809912898503,0.,0.981627005099017));
#99513=DIRECTION('',(-0.981627005099017,0.,-0.190809912898503));
#99514=DIRECTION('',(-0.981627005099017,0.,-0.190809912898503));
#99515=DIRECTION('center_axis',(-0.981627005099017,0.,-0.190809912898503));
#99516=DIRECTION('ref_axis',(-0.190809912898503,0.,0.981627005099017));
#99517=DIRECTION('',(0.,1.,0.));
#99518=DIRECTION('',(0.,1.,0.));
#99519=DIRECTION('center_axis',(0.,1.,0.));
#99520=DIRECTION('ref_axis',(1.,0.,0.));
#99521=DIRECTION('',(-0.190809912898503,0.,0.981627005099017));
#99522=DIRECTION('',(0.981627005099017,0.,0.190809912898503));
#99523=DIRECTION('',(-0.190809912898503,0.,0.981627005099017));
#99524=DIRECTION('',(0.981627005099017,0.,0.190809912898503));
#99525=DIRECTION('center_axis',(0.981627005099017,0.,0.190809912898503));
#99526=DIRECTION('ref_axis',(0.,-1.,0.));
#99527=DIRECTION('',(-0.190809912898503,0.,0.981627005099017));
#99528=DIRECTION('',(0.,-1.,0.));
#99529=DIRECTION('',(0.,-1.,0.));
#99530=DIRECTION('center_axis',(0.,-1.,0.));
#99531=DIRECTION('ref_axis',(0.,0.,-1.));
#99532=DIRECTION('',(-0.190809912898503,0.,0.981627005099017));
#99533=DIRECTION('',(-0.981627005099017,0.,-0.190809912898503));
#99534=DIRECTION('',(-0.981627005099017,0.,-0.190809912898503));
#99535=DIRECTION('center_axis',(-0.981627005099017,0.,-0.190809912898503));
#99536=DIRECTION('ref_axis',(-0.190809912898503,0.,0.981627005099017));
#99537=DIRECTION('',(0.,1.,0.));
#99538=DIRECTION('',(0.,1.,0.));
#99539=DIRECTION('center_axis',(0.,1.,0.));
#99540=DIRECTION('ref_axis',(1.,0.,0.));
#99541=DIRECTION('',(-0.190809912898503,0.,0.981627005099017));
#99542=DIRECTION('',(0.981627005099017,0.,0.190809912898503));
#99543=DIRECTION('',(-0.190809912898503,0.,0.981627005099017));
#99544=DIRECTION('',(0.981627005099017,0.,0.190809912898503));
#99545=DIRECTION('center_axis',(0.981627005099017,0.,0.190809912898503));
#99546=DIRECTION('ref_axis',(0.,-1.,0.));
#99547=DIRECTION('',(-0.190809912898503,0.,0.981627005099017));
#99548=DIRECTION('',(0.,-1.,0.));
#99549=DIRECTION('',(0.,-1.,0.));
#99550=DIRECTION('center_axis',(0.,-1.,0.));
#99551=DIRECTION('ref_axis',(0.,0.,-1.));
#99552=DIRECTION('',(-0.190809912898503,0.,0.981627005099017));
#99553=DIRECTION('',(-0.981627005099017,0.,-0.190809912898503));
#99554=DIRECTION('',(-0.981627005099017,0.,-0.190809912898503));
#99555=DIRECTION('center_axis',(-0.981627005099017,0.,-0.190809912898503));
#99556=DIRECTION('ref_axis',(-0.190809912898503,0.,0.981627005099017));
#99557=DIRECTION('',(0.,1.,0.));
#99558=DIRECTION('',(0.,1.,0.));
#99559=DIRECTION('center_axis',(0.,1.,0.));
#99560=DIRECTION('ref_axis',(1.,0.,0.));
#99561=DIRECTION('',(-0.190809912898503,0.,0.981627005099017));
#99562=DIRECTION('',(0.981627005099017,0.,0.190809912898503));
#99563=DIRECTION('',(-0.190809912898503,0.,0.981627005099017));
#99564=DIRECTION('',(0.981627005099017,0.,0.190809912898503));
#99565=DIRECTION('center_axis',(0.981627005099017,0.,0.190809912898503));
#99566=DIRECTION('ref_axis',(0.,-1.,0.));
#99567=DIRECTION('',(-0.190809912898503,0.,0.981627005099017));
#99568=DIRECTION('',(0.,-1.,0.));
#99569=DIRECTION('',(0.,-1.,0.));
#99570=DIRECTION('center_axis',(0.,-1.,0.));
#99571=DIRECTION('ref_axis',(0.,0.,-1.));
#99572=DIRECTION('',(-0.190809912898503,0.,0.981627005099017));
#99573=DIRECTION('',(-0.981627005099017,0.,-0.190809912898503));
#99574=DIRECTION('',(-0.981627005099017,0.,-0.190809912898503));
#99575=DIRECTION('center_axis',(-0.981627005099017,0.,-0.190809912898503));
#99576=DIRECTION('ref_axis',(-0.190809912898503,0.,0.981627005099017));
#99577=DIRECTION('',(0.,1.,0.));
#99578=DIRECTION('',(0.,1.,0.));
#99579=DIRECTION('center_axis',(0.,1.,0.));
#99580=DIRECTION('ref_axis',(1.,0.,0.));
#99581=DIRECTION('',(-0.190809912898503,0.,0.981627005099017));
#99582=DIRECTION('',(0.981627005099017,0.,0.190809912898503));
#99583=DIRECTION('',(-0.190809912898503,0.,0.981627005099017));
#99584=DIRECTION('',(0.981627005099017,0.,0.190809912898503));
#99585=DIRECTION('center_axis',(0.981627005099017,0.,0.190809912898503));
#99586=DIRECTION('ref_axis',(0.,-1.,0.));
#99587=DIRECTION('',(-0.190809912898503,0.,0.981627005099017));
#99588=DIRECTION('',(0.,-1.,0.));
#99589=DIRECTION('',(0.,-1.,0.));
#99590=DIRECTION('center_axis',(0.,-1.,0.));
#99591=DIRECTION('ref_axis',(0.,0.,-1.));
#99592=DIRECTION('',(-0.190809912898503,0.,0.981627005099017));
#99593=DIRECTION('',(-0.981627005099017,0.,-0.190809912898503));
#99594=DIRECTION('',(-0.981627005099017,0.,-0.190809912898503));
#99595=DIRECTION('center_axis',(-0.981627005099017,0.,-0.190809912898503));
#99596=DIRECTION('ref_axis',(-0.190809912898503,0.,0.981627005099017));
#99597=DIRECTION('',(0.,1.,0.));
#99598=DIRECTION('',(0.,1.,0.));
#99599=DIRECTION('center_axis',(0.,1.,0.));
#99600=DIRECTION('ref_axis',(1.,0.,0.));
#99601=DIRECTION('',(-0.190809912898503,0.,0.981627005099017));
#99602=DIRECTION('',(0.981627005099017,0.,0.190809912898503));
#99603=DIRECTION('',(-0.190809912898503,0.,0.981627005099017));
#99604=DIRECTION('',(0.981627005099017,0.,0.190809912898503));
#99605=DIRECTION('center_axis',(0.981627005099017,0.,0.190809912898503));
#99606=DIRECTION('ref_axis',(0.,-1.,0.));
#99607=DIRECTION('',(-0.190809912898503,0.,0.981627005099017));
#99608=DIRECTION('',(0.,-1.,0.));
#99609=DIRECTION('',(0.,-1.,0.));
#99610=DIRECTION('center_axis',(0.,-1.,0.));
#99611=DIRECTION('ref_axis',(0.,0.,-1.));
#99612=DIRECTION('',(-0.190809912898503,0.,0.981627005099017));
#99613=DIRECTION('',(-0.981627005099017,0.,-0.190809912898503));
#99614=DIRECTION('',(-0.981627005099017,0.,-0.190809912898503));
#99615=DIRECTION('center_axis',(-0.981627005099017,0.,-0.190809912898503));
#99616=DIRECTION('ref_axis',(-0.190809912898503,0.,0.981627005099017));
#99617=DIRECTION('',(0.,1.,0.));
#99618=DIRECTION('',(0.,1.,0.));
#99619=DIRECTION('center_axis',(0.,1.,0.));
#99620=DIRECTION('ref_axis',(1.,0.,0.));
#99621=DIRECTION('',(-0.190809912898503,0.,0.981627005099017));
#99622=DIRECTION('',(0.981627005099017,0.,0.190809912898503));
#99623=DIRECTION('',(-0.190809912898503,0.,0.981627005099017));
#99624=DIRECTION('',(0.981627005099017,0.,0.190809912898503));
#99625=DIRECTION('center_axis',(0.981627005099017,0.,0.190809912898503));
#99626=DIRECTION('ref_axis',(0.,-1.,0.));
#99627=DIRECTION('',(-0.190809912898503,0.,0.981627005099017));
#99628=DIRECTION('',(0.,-1.,0.));
#99629=DIRECTION('',(0.,-1.,0.));
#99630=DIRECTION('center_axis',(0.,-1.,0.));
#99631=DIRECTION('ref_axis',(0.,0.,-1.));
#99632=DIRECTION('',(-0.190809912898503,0.,0.981627005099017));
#99633=DIRECTION('',(-0.981627005099017,0.,-0.190809912898503));
#99634=DIRECTION('',(-0.981627005099017,0.,-0.190809912898503));
#99635=DIRECTION('center_axis',(-0.981627005099017,0.,-0.190809912898503));
#99636=DIRECTION('ref_axis',(-0.190809912898503,0.,0.981627005099017));
#99637=DIRECTION('',(0.,1.,0.));
#99638=DIRECTION('',(0.,1.,0.));
#99639=DIRECTION('center_axis',(0.,1.,0.));
#99640=DIRECTION('ref_axis',(1.,0.,0.));
#99641=DIRECTION('',(-0.190809912898503,0.,0.981627005099017));
#99642=DIRECTION('',(0.981627005099017,0.,0.190809912898503));
#99643=DIRECTION('',(-0.190809912898503,0.,0.981627005099017));
#99644=DIRECTION('',(0.981627005099017,0.,0.190809912898503));
#99645=DIRECTION('center_axis',(0.981627005099017,0.,0.190809912898503));
#99646=DIRECTION('ref_axis',(0.,-1.,0.));
#99647=DIRECTION('',(-0.190809912898503,0.,0.981627005099017));
#99648=DIRECTION('',(0.,-1.,0.));
#99649=DIRECTION('',(0.,-1.,0.));
#99650=DIRECTION('center_axis',(0.,-1.,0.));
#99651=DIRECTION('ref_axis',(0.,0.,-1.));
#99652=DIRECTION('',(-0.190809912898503,0.,0.981627005099017));
#99653=DIRECTION('',(-0.981627005099017,0.,-0.190809912898503));
#99654=DIRECTION('',(-0.981627005099017,0.,-0.190809912898503));
#99655=DIRECTION('center_axis',(-0.981627005099017,0.,-0.190809912898503));
#99656=DIRECTION('ref_axis',(-0.190809912898503,0.,0.981627005099017));
#99657=DIRECTION('',(0.,1.,0.));
#99658=DIRECTION('',(0.,1.,0.));
#99659=DIRECTION('center_axis',(0.,1.,0.));
#99660=DIRECTION('ref_axis',(1.,0.,0.));
#99661=DIRECTION('',(-0.190809912898503,0.,0.981627005099017));
#99662=DIRECTION('',(0.981627005099017,0.,0.190809912898503));
#99663=DIRECTION('',(-0.190809912898503,0.,0.981627005099017));
#99664=DIRECTION('',(0.981627005099017,0.,0.190809912898503));
#99665=DIRECTION('center_axis',(0.981627005099017,0.,0.190809912898503));
#99666=DIRECTION('ref_axis',(0.,-1.,0.));
#99667=DIRECTION('',(-0.190809912898503,0.,0.981627005099017));
#99668=DIRECTION('',(0.,-1.,0.));
#99669=DIRECTION('',(0.,-1.,0.));
#99670=DIRECTION('center_axis',(0.,-1.,0.));
#99671=DIRECTION('ref_axis',(0.,0.,-1.));
#99672=DIRECTION('',(-0.190809912898503,0.,0.981627005099017));
#99673=DIRECTION('',(-0.981627005099017,0.,-0.190809912898503));
#99674=DIRECTION('',(-0.981627005099017,0.,-0.190809912898503));
#99675=DIRECTION('center_axis',(-0.981627005099017,0.,-0.190809912898503));
#99676=DIRECTION('ref_axis',(-0.190809912898503,0.,0.981627005099017));
#99677=DIRECTION('',(0.,1.,0.));
#99678=DIRECTION('',(0.,1.,0.));
#99679=DIRECTION('center_axis',(0.,1.,0.));
#99680=DIRECTION('ref_axis',(1.,0.,0.));
#99681=DIRECTION('',(-0.190809912898503,0.,0.981627005099017));
#99682=DIRECTION('',(0.981627005099017,0.,0.190809912898503));
#99683=DIRECTION('',(-0.190809912898503,0.,0.981627005099017));
#99684=DIRECTION('',(0.981627005099017,0.,0.190809912898503));
#99685=DIRECTION('center_axis',(0.981627005099017,0.,0.190809912898503));
#99686=DIRECTION('ref_axis',(0.,-1.,0.));
#99687=DIRECTION('',(-0.190809912898503,0.,0.981627005099017));
#99688=DIRECTION('',(0.,-1.,0.));
#99689=DIRECTION('',(0.,-1.,0.));
#99690=DIRECTION('center_axis',(0.,-1.,0.));
#99691=DIRECTION('ref_axis',(0.,0.,-1.));
#99692=DIRECTION('',(-0.190809912898503,0.,0.981627005099017));
#99693=DIRECTION('',(-0.981627005099017,0.,-0.190809912898503));
#99694=DIRECTION('',(-0.981627005099017,0.,-0.190809912898503));
#99695=DIRECTION('center_axis',(-0.981627005099017,0.,-0.190809912898503));
#99696=DIRECTION('ref_axis',(-0.190809912898503,0.,0.981627005099017));
#99697=DIRECTION('',(0.,1.,0.));
#99698=DIRECTION('',(0.,1.,0.));
#99699=DIRECTION('center_axis',(0.,1.,0.));
#99700=DIRECTION('ref_axis',(1.,0.,0.));
#99701=DIRECTION('',(-0.190809912898503,0.,0.981627005099017));
#99702=DIRECTION('',(0.981627005099017,0.,0.190809912898503));
#99703=DIRECTION('',(-0.190809912898503,0.,0.981627005099017));
#99704=DIRECTION('',(0.981627005099017,0.,0.190809912898503));
#99705=DIRECTION('center_axis',(0.981627005099017,0.,0.190809912898503));
#99706=DIRECTION('ref_axis',(0.,-1.,0.));
#99707=DIRECTION('',(-0.190809912898503,0.,0.981627005099017));
#99708=DIRECTION('',(0.,-1.,0.));
#99709=DIRECTION('',(0.,-1.,0.));
#99710=DIRECTION('center_axis',(0.,-1.,0.));
#99711=DIRECTION('ref_axis',(0.,0.,-1.));
#99712=DIRECTION('',(-0.190809912898503,0.,0.981627005099017));
#99713=DIRECTION('',(-0.981627005099017,0.,-0.190809912898503));
#99714=DIRECTION('',(-0.981627005099017,0.,-0.190809912898503));
#99715=DIRECTION('center_axis',(-0.981627005099017,0.,-0.190809912898503));
#99716=DIRECTION('ref_axis',(-0.190809912898503,0.,0.981627005099017));
#99717=DIRECTION('',(0.,1.,0.));
#99718=DIRECTION('',(0.,1.,0.));
#99719=DIRECTION('center_axis',(0.,1.,0.));
#99720=DIRECTION('ref_axis',(1.,0.,0.));
#99721=DIRECTION('',(-0.190809912898503,0.,0.981627005099017));
#99722=DIRECTION('',(0.981627005099017,0.,0.190809912898503));
#99723=DIRECTION('',(-0.190809912898503,0.,0.981627005099017));
#99724=DIRECTION('',(0.981627005099017,0.,0.190809912898503));
#99725=DIRECTION('center_axis',(0.981627005099017,0.,0.190809912898503));
#99726=DIRECTION('ref_axis',(0.,-1.,0.));
#99727=DIRECTION('',(-0.190809912898503,0.,0.981627005099017));
#99728=DIRECTION('',(0.,-1.,0.));
#99729=DIRECTION('',(0.,-1.,0.));
#99730=DIRECTION('center_axis',(0.,-1.,0.));
#99731=DIRECTION('ref_axis',(0.,0.,-1.));
#99732=DIRECTION('',(-0.190809912898503,0.,0.981627005099017));
#99733=DIRECTION('',(-0.981627005099017,0.,-0.190809912898503));
#99734=DIRECTION('',(-0.981627005099017,0.,-0.190809912898503));
#99735=DIRECTION('center_axis',(-0.981627005099017,0.,-0.190809912898503));
#99736=DIRECTION('ref_axis',(-0.190809912898503,0.,0.981627005099017));
#99737=DIRECTION('',(0.,1.,0.));
#99738=DIRECTION('',(0.,1.,0.));
#99739=DIRECTION('center_axis',(0.,1.,0.));
#99740=DIRECTION('ref_axis',(1.,0.,0.));
#99741=DIRECTION('',(-0.190809912898503,0.,0.981627005099017));
#99742=DIRECTION('',(0.981627005099017,0.,0.190809912898503));
#99743=DIRECTION('',(-0.190809912898503,0.,0.981627005099017));
#99744=DIRECTION('',(0.981627005099017,0.,0.190809912898503));
#99745=DIRECTION('center_axis',(0.981627005099017,0.,0.190809912898503));
#99746=DIRECTION('ref_axis',(0.,-1.,0.));
#99747=DIRECTION('',(-0.190809912898503,0.,0.981627005099017));
#99748=DIRECTION('',(0.,-1.,0.));
#99749=DIRECTION('',(0.,-1.,0.));
#99750=DIRECTION('center_axis',(0.,-1.,0.));
#99751=DIRECTION('ref_axis',(0.,0.,-1.));
#99752=DIRECTION('',(-0.190809912898503,0.,0.981627005099017));
#99753=DIRECTION('',(-0.981627005099017,0.,-0.190809912898503));
#99754=DIRECTION('',(-0.981627005099017,0.,-0.190809912898503));
#99755=DIRECTION('center_axis',(-0.981627005099017,0.,-0.190809912898503));
#99756=DIRECTION('ref_axis',(-0.190809912898503,0.,0.981627005099017));
#99757=DIRECTION('',(0.,1.,0.));
#99758=DIRECTION('',(0.,1.,0.));
#99759=DIRECTION('center_axis',(0.,1.,0.));
#99760=DIRECTION('ref_axis',(1.,0.,0.));
#99761=DIRECTION('',(-0.190809912898503,0.,0.981627005099017));
#99762=DIRECTION('',(0.981627005099017,0.,0.190809912898503));
#99763=DIRECTION('',(-0.190809912898503,0.,0.981627005099017));
#99764=DIRECTION('',(0.981627005099017,0.,0.190809912898503));
#99765=DIRECTION('center_axis',(0.981627005099017,0.,0.190809912898503));
#99766=DIRECTION('ref_axis',(0.,-1.,0.));
#99767=DIRECTION('',(-0.190809912898503,0.,0.981627005099017));
#99768=DIRECTION('',(0.,-1.,0.));
#99769=DIRECTION('',(0.,-1.,0.));
#99770=DIRECTION('center_axis',(0.,-1.,0.));
#99771=DIRECTION('ref_axis',(0.,0.,-1.));
#99772=DIRECTION('',(-0.190809912898503,0.,0.981627005099017));
#99773=DIRECTION('',(-0.981627005099017,0.,-0.190809912898503));
#99774=DIRECTION('',(-0.981627005099017,0.,-0.190809912898503));
#99775=DIRECTION('center_axis',(-0.981627005099017,0.,-0.190809912898503));
#99776=DIRECTION('ref_axis',(-0.190809912898503,0.,0.981627005099017));
#99777=DIRECTION('',(0.,1.,0.));
#99778=DIRECTION('',(0.,1.,0.));
#99779=DIRECTION('center_axis',(0.,1.,0.));
#99780=DIRECTION('ref_axis',(1.,0.,0.));
#99781=DIRECTION('',(-0.190809912898503,0.,0.981627005099017));
#99782=DIRECTION('',(0.981627005099017,0.,0.190809912898503));
#99783=DIRECTION('',(-0.190809912898503,0.,0.981627005099017));
#99784=DIRECTION('',(0.981627005099017,0.,0.190809912898503));
#99785=DIRECTION('center_axis',(0.981627005099017,0.,0.190809912898503));
#99786=DIRECTION('ref_axis',(0.,-1.,0.));
#99787=DIRECTION('',(-0.190809912898503,0.,0.981627005099017));
#99788=DIRECTION('',(0.,-1.,0.));
#99789=DIRECTION('',(0.,-1.,0.));
#99790=DIRECTION('center_axis',(0.,-1.,0.));
#99791=DIRECTION('ref_axis',(0.,0.,-1.));
#99792=DIRECTION('',(-0.190809912898503,0.,0.981627005099017));
#99793=DIRECTION('',(-0.981627005099017,0.,-0.190809912898503));
#99794=DIRECTION('',(-0.981627005099017,0.,-0.190809912898503));
#99795=DIRECTION('center_axis',(-0.981627005099017,0.,-0.190809912898503));
#99796=DIRECTION('ref_axis',(-0.190809912898503,0.,0.981627005099017));
#99797=DIRECTION('',(0.,1.,0.));
#99798=DIRECTION('',(0.,1.,0.));
#99799=DIRECTION('center_axis',(0.,1.,0.));
#99800=DIRECTION('ref_axis',(1.,0.,0.));
#99801=DIRECTION('',(-0.190809912898503,0.,0.981627005099017));
#99802=DIRECTION('',(0.981627005099017,0.,0.190809912898503));
#99803=DIRECTION('',(-0.190809912898503,0.,0.981627005099017));
#99804=DIRECTION('',(0.981627005099017,0.,0.190809912898503));
#99805=DIRECTION('center_axis',(0.981627005099017,0.,0.190809912898503));
#99806=DIRECTION('ref_axis',(0.,-1.,0.));
#99807=DIRECTION('',(-0.190809912898503,0.,0.981627005099017));
#99808=DIRECTION('',(0.,-1.,0.));
#99809=DIRECTION('',(0.,-1.,0.));
#99810=DIRECTION('center_axis',(0.,-1.,0.));
#99811=DIRECTION('ref_axis',(0.,0.,-1.));
#99812=DIRECTION('',(-0.190809912898503,0.,0.981627005099017));
#99813=DIRECTION('',(-0.981627005099017,0.,-0.190809912898503));
#99814=DIRECTION('',(-0.981627005099017,0.,-0.190809912898503));
#99815=DIRECTION('center_axis',(-0.981627005099017,0.,-0.190809912898503));
#99816=DIRECTION('ref_axis',(-0.190809912898503,0.,0.981627005099017));
#99817=DIRECTION('',(0.,1.,0.));
#99818=DIRECTION('',(0.,1.,0.));
#99819=DIRECTION('center_axis',(0.,1.,0.));
#99820=DIRECTION('ref_axis',(1.,0.,0.));
#99821=DIRECTION('',(-0.190809912898503,0.,0.981627005099017));
#99822=DIRECTION('',(0.981627005099017,0.,0.190809912898503));
#99823=DIRECTION('',(-0.190809912898503,0.,0.981627005099017));
#99824=DIRECTION('',(0.981627005099017,0.,0.190809912898503));
#99825=DIRECTION('center_axis',(0.981627005099017,0.,0.190809912898503));
#99826=DIRECTION('ref_axis',(0.,-1.,0.));
#99827=DIRECTION('',(-0.190809912898503,0.,0.981627005099017));
#99828=DIRECTION('',(0.,-1.,0.));
#99829=DIRECTION('',(0.,-1.,0.));
#99830=DIRECTION('center_axis',(0.,-1.,0.));
#99831=DIRECTION('ref_axis',(0.,0.,-1.));
#99832=DIRECTION('',(-0.190809912898503,0.,0.981627005099017));
#99833=DIRECTION('',(-0.981627005099017,0.,-0.190809912898503));
#99834=DIRECTION('',(-0.981627005099017,0.,-0.190809912898503));
#99835=DIRECTION('center_axis',(-0.981627005099017,0.,-0.190809912898503));
#99836=DIRECTION('ref_axis',(-0.190809912898503,0.,0.981627005099017));
#99837=DIRECTION('',(0.,1.,0.));
#99838=DIRECTION('',(0.,1.,0.));
#99839=DIRECTION('center_axis',(0.,1.,0.));
#99840=DIRECTION('ref_axis',(1.,0.,0.));
#99841=DIRECTION('',(-0.190809912898503,0.,0.981627005099017));
#99842=DIRECTION('',(0.981627005099017,0.,0.190809912898503));
#99843=DIRECTION('',(-0.190809912898503,0.,0.981627005099017));
#99844=DIRECTION('',(0.981627005099017,0.,0.190809912898503));
#99845=DIRECTION('center_axis',(0.981627005099017,0.,0.190809912898503));
#99846=DIRECTION('ref_axis',(0.,-1.,0.));
#99847=DIRECTION('',(-0.190809912898503,0.,0.981627005099017));
#99848=DIRECTION('',(0.,-1.,0.));
#99849=DIRECTION('',(0.,-1.,0.));
#99850=DIRECTION('center_axis',(0.,-1.,0.));
#99851=DIRECTION('ref_axis',(0.,0.,-1.));
#99852=DIRECTION('',(-0.190809912898503,0.,0.981627005099017));
#99853=DIRECTION('',(-0.981627005099017,0.,-0.190809912898503));
#99854=DIRECTION('',(-0.981627005099017,0.,-0.190809912898503));
#99855=DIRECTION('center_axis',(-0.981627005099017,0.,-0.190809912898503));
#99856=DIRECTION('ref_axis',(-0.190809912898503,0.,0.981627005099017));
#99857=DIRECTION('',(0.,1.,0.));
#99858=DIRECTION('',(0.,1.,0.));
#99859=DIRECTION('center_axis',(0.,1.,0.));
#99860=DIRECTION('ref_axis',(1.,0.,0.));
#99861=DIRECTION('',(-0.190809912898503,0.,0.981627005099017));
#99862=DIRECTION('',(0.981627005099017,0.,0.190809912898503));
#99863=DIRECTION('',(-0.190809912898503,0.,0.981627005099017));
#99864=DIRECTION('',(0.981627005099017,0.,0.190809912898503));
#99865=DIRECTION('center_axis',(0.981627005099017,0.,0.190809912898503));
#99866=DIRECTION('ref_axis',(0.,-1.,0.));
#99867=DIRECTION('',(-0.190809912898503,0.,0.981627005099017));
#99868=DIRECTION('',(0.,-1.,0.));
#99869=DIRECTION('',(0.,-1.,0.));
#99870=DIRECTION('center_axis',(0.,-1.,0.));
#99871=DIRECTION('ref_axis',(0.,0.,-1.));
#99872=DIRECTION('',(-0.190809912898503,0.,0.981627005099017));
#99873=DIRECTION('',(-0.981627005099017,0.,-0.190809912898503));
#99874=DIRECTION('',(-0.981627005099017,0.,-0.190809912898503));
#99875=DIRECTION('center_axis',(-0.981627005099017,0.,-0.190809912898503));
#99876=DIRECTION('ref_axis',(-0.190809912898503,0.,0.981627005099017));
#99877=DIRECTION('',(0.,1.,0.));
#99878=DIRECTION('',(0.,1.,0.));
#99879=DIRECTION('center_axis',(0.,1.,0.));
#99880=DIRECTION('ref_axis',(1.,0.,0.));
#99881=DIRECTION('',(-0.190809912898503,0.,0.981627005099017));
#99882=DIRECTION('',(0.981627005099017,0.,0.190809912898503));
#99883=DIRECTION('',(-0.190809912898503,0.,0.981627005099017));
#99884=DIRECTION('',(0.981627005099017,0.,0.190809912898503));
#99885=DIRECTION('center_axis',(0.981627005099017,0.,0.190809912898503));
#99886=DIRECTION('ref_axis',(0.,-1.,0.));
#99887=DIRECTION('',(-0.190809912898503,0.,0.981627005099017));
#99888=DIRECTION('',(0.,-1.,0.));
#99889=DIRECTION('',(0.,-1.,0.));
#99890=DIRECTION('center_axis',(0.,-1.,0.));
#99891=DIRECTION('ref_axis',(0.,0.,-1.));
#99892=DIRECTION('',(-0.190809912898503,0.,0.981627005099017));
#99893=DIRECTION('',(-0.981627005099017,0.,-0.190809912898503));
#99894=DIRECTION('',(-0.981627005099017,0.,-0.190809912898503));
#99895=DIRECTION('center_axis',(-0.981627005099017,0.,-0.190809912898503));
#99896=DIRECTION('ref_axis',(-0.190809912898503,0.,0.981627005099017));
#99897=DIRECTION('',(0.,1.,0.));
#99898=DIRECTION('',(0.,1.,0.));
#99899=DIRECTION('center_axis',(0.,1.,0.));
#99900=DIRECTION('ref_axis',(1.,0.,0.));
#99901=DIRECTION('',(-0.190809912898503,0.,0.981627005099017));
#99902=DIRECTION('',(0.981627005099017,0.,0.190809912898503));
#99903=DIRECTION('',(-0.190809912898503,0.,0.981627005099017));
#99904=DIRECTION('',(0.981627005099017,0.,0.190809912898503));
#99905=DIRECTION('center_axis',(0.981627005099017,0.,0.190809912898503));
#99906=DIRECTION('ref_axis',(0.,-1.,0.));
#99907=DIRECTION('',(-0.190809912898503,0.,0.981627005099017));
#99908=DIRECTION('',(0.,-1.,0.));
#99909=DIRECTION('',(0.,-1.,0.));
#99910=DIRECTION('center_axis',(0.,-1.,0.));
#99911=DIRECTION('ref_axis',(0.,0.,-1.));
#99912=DIRECTION('',(-0.190809912898503,0.,0.981627005099017));
#99913=DIRECTION('',(-0.981627005099017,0.,-0.190809912898503));
#99914=DIRECTION('',(-0.981627005099017,0.,-0.190809912898503));
#99915=DIRECTION('center_axis',(-0.981627005099017,0.,-0.190809912898503));
#99916=DIRECTION('ref_axis',(-0.190809912898503,0.,0.981627005099017));
#99917=DIRECTION('',(0.,1.,0.));
#99918=DIRECTION('',(0.,1.,0.));
#99919=DIRECTION('center_axis',(0.,1.,0.));
#99920=DIRECTION('ref_axis',(1.,0.,0.));
#99921=DIRECTION('',(-0.190809912898503,0.,0.981627005099017));
#99922=DIRECTION('',(0.981627005099017,0.,0.190809912898503));
#99923=DIRECTION('',(-0.190809912898503,0.,0.981627005099017));
#99924=DIRECTION('',(0.981627005099017,0.,0.190809912898503));
#99925=DIRECTION('center_axis',(0.981627005099017,0.,0.190809912898503));
#99926=DIRECTION('ref_axis',(0.,-1.,0.));
#99927=DIRECTION('',(-0.190809912898503,0.,0.981627005099017));
#99928=DIRECTION('',(0.,-1.,0.));
#99929=DIRECTION('',(0.,-1.,0.));
#99930=DIRECTION('center_axis',(0.,-1.,0.));
#99931=DIRECTION('ref_axis',(0.,0.,-1.));
#99932=DIRECTION('',(-0.190809912898503,0.,0.981627005099017));
#99933=DIRECTION('',(-0.981627005099017,0.,-0.190809912898503));
#99934=DIRECTION('',(-0.981627005099017,0.,-0.190809912898503));
#99935=DIRECTION('center_axis',(-0.981627005099017,0.,-0.190809912898503));
#99936=DIRECTION('ref_axis',(-0.190809912898503,0.,0.981627005099017));
#99937=DIRECTION('',(0.,1.,0.));
#99938=DIRECTION('',(0.,1.,0.));
#99939=DIRECTION('center_axis',(0.,1.,0.));
#99940=DIRECTION('ref_axis',(1.,0.,0.));
#99941=DIRECTION('',(-0.190809912898503,0.,0.981627005099017));
#99942=DIRECTION('',(0.981627005099017,0.,0.190809912898503));
#99943=DIRECTION('',(-0.190809912898503,0.,0.981627005099017));
#99944=DIRECTION('',(0.981627005099017,0.,0.190809912898503));
#99945=DIRECTION('center_axis',(0.981627005099017,0.,0.190809912898503));
#99946=DIRECTION('ref_axis',(0.,-1.,0.));
#99947=DIRECTION('',(-0.190809912898503,0.,0.981627005099017));
#99948=DIRECTION('',(0.,-1.,0.));
#99949=DIRECTION('',(0.,-1.,0.));
#99950=DIRECTION('center_axis',(0.,-1.,0.));
#99951=DIRECTION('ref_axis',(0.,0.,-1.));
#99952=DIRECTION('',(-0.190809912898503,0.,0.981627005099017));
#99953=DIRECTION('',(-0.981627005099017,0.,-0.190809912898503));
#99954=DIRECTION('',(-0.981627005099017,0.,-0.190809912898503));
#99955=DIRECTION('center_axis',(-0.981627005099017,0.,-0.190809912898503));
#99956=DIRECTION('ref_axis',(-0.190809912898503,0.,0.981627005099017));
#99957=DIRECTION('',(0.,1.,0.));
#99958=DIRECTION('',(0.,1.,0.));
#99959=DIRECTION('center_axis',(0.,1.,0.));
#99960=DIRECTION('ref_axis',(1.,0.,0.));
#99961=DIRECTION('',(-0.190809912898503,0.,0.981627005099017));
#99962=DIRECTION('',(0.981627005099017,0.,0.190809912898503));
#99963=DIRECTION('',(-0.190809912898503,0.,0.981627005099017));
#99964=DIRECTION('',(0.981627005099017,0.,0.190809912898503));
#99965=DIRECTION('center_axis',(0.981627005099017,0.,0.190809912898503));
#99966=DIRECTION('ref_axis',(0.,-1.,0.));
#99967=DIRECTION('',(-0.190809912898503,0.,0.981627005099017));
#99968=DIRECTION('',(0.,-1.,0.));
#99969=DIRECTION('',(0.,-1.,0.));
#99970=DIRECTION('center_axis',(0.,-1.,0.));
#99971=DIRECTION('ref_axis',(0.,0.,-1.));
#99972=DIRECTION('',(-0.190809912898503,0.,0.981627005099017));
#99973=DIRECTION('',(-0.981627005099017,0.,-0.190809912898503));
#99974=DIRECTION('',(-0.981627005099017,0.,-0.190809912898503));
#99975=DIRECTION('center_axis',(-0.981627005099017,0.,-0.190809912898503));
#99976=DIRECTION('ref_axis',(-0.190809912898503,0.,0.981627005099017));
#99977=DIRECTION('',(0.,1.,0.));
#99978=DIRECTION('',(0.,1.,0.));
#99979=DIRECTION('center_axis',(0.,1.,0.));
#99980=DIRECTION('ref_axis',(1.,0.,0.));
#99981=DIRECTION('',(-0.190809912898503,0.,0.981627005099017));
#99982=DIRECTION('',(0.981627005099017,0.,0.190809912898503));
#99983=DIRECTION('',(-0.190809912898503,0.,0.981627005099017));
#99984=DIRECTION('',(0.981627005099017,0.,0.190809912898503));
#99985=DIRECTION('center_axis',(0.981627005099017,0.,0.190809912898503));
#99986=DIRECTION('ref_axis',(0.,-1.,0.));
#99987=DIRECTION('',(-0.190809912898503,0.,0.981627005099017));
#99988=DIRECTION('',(0.,-1.,0.));
#99989=DIRECTION('',(0.,-1.,0.));
#99990=DIRECTION('center_axis',(0.,-1.,0.));
#99991=DIRECTION('ref_axis',(0.,0.,-1.));
#99992=DIRECTION('',(-0.190809912898503,0.,0.981627005099017));
#99993=DIRECTION('',(-0.981627005099017,0.,-0.190809912898503));
#99994=DIRECTION('',(-0.981627005099017,0.,-0.190809912898503));
#99995=DIRECTION('center_axis',(-0.981627005099017,0.,-0.190809912898503));
#99996=DIRECTION('ref_axis',(-0.190809912898503,0.,0.981627005099017));
#99997=DIRECTION('',(0.,1.,0.));
#99998=DIRECTION('',(0.,1.,0.));
#99999=DIRECTION('center_axis',(0.,1.,0.));
#100000=DIRECTION('ref_axis',(1.,0.,0.));
#100001=DIRECTION('',(-0.190809912898503,0.,0.981627005099017));
#100002=DIRECTION('',(0.981627005099017,0.,0.190809912898503));
#100003=DIRECTION('',(-0.190809912898503,0.,0.981627005099017));
#100004=DIRECTION('',(0.981627005099017,0.,0.190809912898503));
#100005=DIRECTION('center_axis',(0.981627005099017,0.,0.190809912898503));
#100006=DIRECTION('ref_axis',(0.,-1.,0.));
#100007=DIRECTION('',(-0.190809912898503,0.,0.981627005099017));
#100008=DIRECTION('',(0.,-1.,0.));
#100009=DIRECTION('',(0.,-1.,0.));
#100010=DIRECTION('center_axis',(0.,-1.,0.));
#100011=DIRECTION('ref_axis',(0.,0.,-1.));
#100012=DIRECTION('',(-0.190809912898503,0.,0.981627005099017));
#100013=DIRECTION('',(-0.981627005099017,0.,-0.190809912898503));
#100014=DIRECTION('',(-0.981627005099017,0.,-0.190809912898503));
#100015=DIRECTION('center_axis',(-0.981627005099017,0.,-0.190809912898503));
#100016=DIRECTION('ref_axis',(-0.190809912898503,0.,0.981627005099017));
#100017=DIRECTION('',(0.,1.,0.));
#100018=DIRECTION('',(0.,1.,0.));
#100019=DIRECTION('center_axis',(0.,1.,0.));
#100020=DIRECTION('ref_axis',(1.,0.,0.));
#100021=DIRECTION('',(-0.190809912898503,0.,0.981627005099017));
#100022=DIRECTION('',(0.981627005099017,0.,0.190809912898503));
#100023=DIRECTION('',(-0.190809912898503,0.,0.981627005099017));
#100024=DIRECTION('',(0.981627005099017,0.,0.190809912898503));
#100025=DIRECTION('center_axis',(0.981627005099017,0.,0.190809912898503));
#100026=DIRECTION('ref_axis',(0.,-1.,0.));
#100027=DIRECTION('',(-0.190809912898503,0.,0.981627005099017));
#100028=DIRECTION('',(0.,-1.,0.));
#100029=DIRECTION('',(0.,-1.,0.));
#100030=DIRECTION('center_axis',(0.,-1.,0.));
#100031=DIRECTION('ref_axis',(0.,0.,-1.));
#100032=DIRECTION('',(-0.190809912898503,0.,0.981627005099017));
#100033=DIRECTION('',(-0.981627005099017,0.,-0.190809912898503));
#100034=DIRECTION('',(-0.981627005099017,0.,-0.190809912898503));
#100035=DIRECTION('center_axis',(-0.981627005099017,0.,-0.190809912898503));
#100036=DIRECTION('ref_axis',(-0.190809912898503,0.,0.981627005099017));
#100037=DIRECTION('',(0.,1.,0.));
#100038=DIRECTION('',(0.,1.,0.));
#100039=DIRECTION('center_axis',(0.,1.,0.));
#100040=DIRECTION('ref_axis',(1.,0.,0.));
#100041=DIRECTION('',(-0.190809912898503,0.,0.981627005099017));
#100042=DIRECTION('',(0.981627005099017,0.,0.190809912898503));
#100043=DIRECTION('',(-0.190809912898503,0.,0.981627005099017));
#100044=DIRECTION('',(0.981627005099017,0.,0.190809912898503));
#100045=DIRECTION('center_axis',(0.981627005099017,0.,0.190809912898503));
#100046=DIRECTION('ref_axis',(0.,-1.,0.));
#100047=DIRECTION('',(-0.190809912898503,0.,0.981627005099017));
#100048=DIRECTION('',(0.,-1.,0.));
#100049=DIRECTION('',(0.,-1.,0.));
#100050=DIRECTION('center_axis',(0.,-1.,0.));
#100051=DIRECTION('ref_axis',(0.,0.,-1.));
#100052=DIRECTION('',(-0.190809912898503,0.,0.981627005099017));
#100053=DIRECTION('',(-0.981627005099017,0.,-0.190809912898503));
#100054=DIRECTION('',(-0.981627005099017,0.,-0.190809912898503));
#100055=DIRECTION('center_axis',(-0.981627005099017,0.,-0.190809912898503));
#100056=DIRECTION('ref_axis',(-0.190809912898503,0.,0.981627005099017));
#100057=DIRECTION('',(0.,1.,0.));
#100058=DIRECTION('',(0.,1.,0.));
#100059=DIRECTION('center_axis',(0.,1.,0.));
#100060=DIRECTION('ref_axis',(1.,0.,0.));
#100061=DIRECTION('',(-0.190809912898503,0.,0.981627005099017));
#100062=DIRECTION('',(0.981627005099017,0.,0.190809912898503));
#100063=DIRECTION('',(-0.190809912898503,0.,0.981627005099017));
#100064=DIRECTION('',(0.981627005099017,0.,0.190809912898503));
#100065=DIRECTION('center_axis',(0.981627005099017,0.,0.190809912898503));
#100066=DIRECTION('ref_axis',(0.,-1.,0.));
#100067=DIRECTION('',(-0.190809912898503,0.,0.981627005099017));
#100068=DIRECTION('',(0.,-1.,0.));
#100069=DIRECTION('',(0.,-1.,0.));
#100070=DIRECTION('center_axis',(0.,-1.,0.));
#100071=DIRECTION('ref_axis',(0.,0.,-1.));
#100072=DIRECTION('',(-0.190809912898503,0.,0.981627005099017));
#100073=DIRECTION('',(-0.981627005099017,0.,-0.190809912898503));
#100074=DIRECTION('',(-0.981627005099017,0.,-0.190809912898503));
#100075=DIRECTION('center_axis',(-0.981627005099017,0.,-0.190809912898503));
#100076=DIRECTION('ref_axis',(-0.190809912898503,0.,0.981627005099017));
#100077=DIRECTION('',(0.,1.,0.));
#100078=DIRECTION('',(0.,1.,0.));
#100079=DIRECTION('center_axis',(0.,1.,0.));
#100080=DIRECTION('ref_axis',(1.,0.,0.));
#100081=DIRECTION('',(-0.190809912898503,0.,0.981627005099017));
#100082=DIRECTION('',(0.981627005099017,0.,0.190809912898503));
#100083=DIRECTION('',(-0.190809912898503,0.,0.981627005099017));
#100084=DIRECTION('',(0.981627005099017,0.,0.190809912898503));
#100085=DIRECTION('center_axis',(0.981627005099017,0.,0.190809912898503));
#100086=DIRECTION('ref_axis',(0.,-1.,0.));
#100087=DIRECTION('',(-0.190809912898503,0.,0.981627005099017));
#100088=DIRECTION('',(0.,-1.,0.));
#100089=DIRECTION('',(0.,-1.,0.));
#100090=DIRECTION('center_axis',(0.,-1.,0.));
#100091=DIRECTION('ref_axis',(0.,0.,-1.));
#100092=DIRECTION('',(-0.190809912898503,0.,0.981627005099017));
#100093=DIRECTION('',(-0.981627005099017,0.,-0.190809912898503));
#100094=DIRECTION('',(-0.981627005099017,0.,-0.190809912898503));
#100095=DIRECTION('center_axis',(-0.981627005099017,0.,-0.190809912898503));
#100096=DIRECTION('ref_axis',(-0.190809912898503,0.,0.981627005099017));
#100097=DIRECTION('',(0.,1.,0.));
#100098=DIRECTION('',(0.,1.,0.));
#100099=DIRECTION('center_axis',(0.,1.,0.));
#100100=DIRECTION('ref_axis',(1.,0.,0.));
#100101=DIRECTION('',(-0.190809912898503,0.,0.981627005099017));
#100102=DIRECTION('',(0.981627005099017,0.,0.190809912898503));
#100103=DIRECTION('',(-0.190809912898503,0.,0.981627005099017));
#100104=DIRECTION('',(0.981627005099017,0.,0.190809912898503));
#100105=DIRECTION('center_axis',(0.981627005099017,0.,0.190809912898503));
#100106=DIRECTION('ref_axis',(0.,-1.,0.));
#100107=DIRECTION('',(-0.190809912898503,0.,0.981627005099017));
#100108=DIRECTION('',(0.,-1.,0.));
#100109=DIRECTION('',(0.,-1.,0.));
#100110=DIRECTION('center_axis',(0.,-1.,0.));
#100111=DIRECTION('ref_axis',(0.,0.,-1.));
#100112=DIRECTION('',(-0.190809912898503,0.,0.981627005099017));
#100113=DIRECTION('',(-0.981627005099017,0.,-0.190809912898503));
#100114=DIRECTION('',(-0.981627005099017,0.,-0.190809912898503));
#100115=DIRECTION('center_axis',(-0.981627005099017,0.,-0.190809912898503));
#100116=DIRECTION('ref_axis',(-0.190809912898503,0.,0.981627005099017));
#100117=DIRECTION('',(0.,1.,0.));
#100118=DIRECTION('',(0.,1.,0.));
#100119=DIRECTION('center_axis',(0.,1.,0.));
#100120=DIRECTION('ref_axis',(1.,0.,0.));
#100121=DIRECTION('',(-0.190809912898503,0.,0.981627005099017));
#100122=DIRECTION('',(0.981627005099017,0.,0.190809912898503));
#100123=DIRECTION('',(-0.190809912898503,0.,0.981627005099017));
#100124=DIRECTION('',(0.981627005099017,0.,0.190809912898503));
#100125=DIRECTION('center_axis',(0.981627005099017,0.,0.190809912898503));
#100126=DIRECTION('ref_axis',(0.,-1.,0.));
#100127=DIRECTION('',(-0.190809912898503,0.,0.981627005099017));
#100128=DIRECTION('',(0.,-1.,0.));
#100129=DIRECTION('',(0.,-1.,0.));
#100130=DIRECTION('center_axis',(0.,-1.,0.));
#100131=DIRECTION('ref_axis',(0.,0.,-1.));
#100132=DIRECTION('',(-0.190809912898503,0.,0.981627005099017));
#100133=DIRECTION('',(-0.981627005099017,0.,-0.190809912898503));
#100134=DIRECTION('',(-0.981627005099017,0.,-0.190809912898503));
#100135=DIRECTION('center_axis',(-0.981627005099017,0.,-0.190809912898503));
#100136=DIRECTION('ref_axis',(-0.190809912898503,0.,0.981627005099017));
#100137=DIRECTION('',(0.,1.,0.));
#100138=DIRECTION('',(0.,1.,0.));
#100139=DIRECTION('center_axis',(0.,1.,0.));
#100140=DIRECTION('ref_axis',(1.,0.,0.));
#100141=DIRECTION('',(-0.190809912898503,0.,0.981627005099017));
#100142=DIRECTION('',(0.981627005099017,0.,0.190809912898503));
#100143=DIRECTION('',(-0.190809912898503,0.,0.981627005099017));
#100144=DIRECTION('',(0.981627005099017,0.,0.190809912898503));
#100145=DIRECTION('center_axis',(0.981627005099017,0.,0.190809912898503));
#100146=DIRECTION('ref_axis',(0.,-1.,0.));
#100147=DIRECTION('',(-0.190809912898503,0.,0.981627005099017));
#100148=DIRECTION('',(0.,-1.,0.));
#100149=DIRECTION('',(0.,-1.,0.));
#100150=DIRECTION('center_axis',(0.,-1.,0.));
#100151=DIRECTION('ref_axis',(0.,0.,-1.));
#100152=DIRECTION('',(-0.190809912898503,0.,0.981627005099017));
#100153=DIRECTION('',(-0.981627005099017,0.,-0.190809912898503));
#100154=DIRECTION('',(-0.981627005099017,0.,-0.190809912898503));
#100155=DIRECTION('center_axis',(-0.981627005099017,0.,-0.190809912898503));
#100156=DIRECTION('ref_axis',(-0.190809912898503,0.,0.981627005099017));
#100157=DIRECTION('',(0.,1.,0.));
#100158=DIRECTION('',(0.,1.,0.));
#100159=DIRECTION('center_axis',(0.,1.,0.));
#100160=DIRECTION('ref_axis',(1.,0.,0.));
#100161=DIRECTION('',(-0.190809912898503,0.,0.981627005099017));
#100162=DIRECTION('',(0.981627005099017,0.,0.190809912898503));
#100163=DIRECTION('',(-0.190809912898503,0.,0.981627005099017));
#100164=DIRECTION('',(0.981627005099017,0.,0.190809912898503));
#100165=DIRECTION('center_axis',(0.981627005099017,0.,0.190809912898503));
#100166=DIRECTION('ref_axis',(0.,-1.,0.));
#100167=DIRECTION('',(-0.190809912898503,0.,0.981627005099017));
#100168=DIRECTION('',(0.,-1.,0.));
#100169=DIRECTION('',(0.,-1.,0.));
#100170=DIRECTION('center_axis',(0.,-1.,0.));
#100171=DIRECTION('ref_axis',(0.,0.,-1.));
#100172=DIRECTION('',(-0.190809912898503,0.,0.981627005099017));
#100173=DIRECTION('',(-0.981627005099017,0.,-0.190809912898503));
#100174=DIRECTION('',(-0.981627005099017,0.,-0.190809912898503));
#100175=DIRECTION('center_axis',(-0.981627005099017,0.,-0.190809912898503));
#100176=DIRECTION('ref_axis',(-0.190809912898503,0.,0.981627005099017));
#100177=DIRECTION('',(0.,1.,0.));
#100178=DIRECTION('',(0.,1.,0.));
#100179=DIRECTION('center_axis',(0.,1.,0.));
#100180=DIRECTION('ref_axis',(1.,0.,0.));
#100181=DIRECTION('',(-0.190809912898503,0.,0.981627005099017));
#100182=DIRECTION('',(0.981627005099017,0.,0.190809912898503));
#100183=DIRECTION('',(-0.190809912898503,0.,0.981627005099017));
#100184=DIRECTION('',(0.981627005099017,0.,0.190809912898503));
#100185=DIRECTION('center_axis',(0.981627005099017,0.,0.190809912898503));
#100186=DIRECTION('ref_axis',(0.,-1.,0.));
#100187=DIRECTION('',(-0.190809912898503,0.,0.981627005099017));
#100188=DIRECTION('',(0.,-1.,0.));
#100189=DIRECTION('',(0.,-1.,0.));
#100190=DIRECTION('center_axis',(0.,-1.,0.));
#100191=DIRECTION('ref_axis',(0.,0.,-1.));
#100192=DIRECTION('',(-0.190809912898503,0.,0.981627005099017));
#100193=DIRECTION('',(-0.981627005099017,0.,-0.190809912898503));
#100194=DIRECTION('',(-0.981627005099017,0.,-0.190809912898503));
#100195=DIRECTION('center_axis',(-0.981627005099017,0.,-0.190809912898503));
#100196=DIRECTION('ref_axis',(-0.190809912898503,0.,0.981627005099017));
#100197=DIRECTION('',(0.,1.,0.));
#100198=DIRECTION('',(0.,1.,0.));
#100199=DIRECTION('center_axis',(0.,1.,0.));
#100200=DIRECTION('ref_axis',(1.,0.,0.));
#100201=DIRECTION('',(-0.190809912898503,0.,0.981627005099017));
#100202=DIRECTION('',(0.981627005099017,0.,0.190809912898503));
#100203=DIRECTION('',(-0.190809912898503,0.,0.981627005099017));
#100204=DIRECTION('',(0.981627005099017,0.,0.190809912898503));
#100205=DIRECTION('center_axis',(0.981627005099017,0.,0.190809912898503));
#100206=DIRECTION('ref_axis',(0.,-1.,0.));
#100207=DIRECTION('',(-0.190809912898503,0.,0.981627005099017));
#100208=DIRECTION('',(0.,-1.,0.));
#100209=DIRECTION('',(0.,-1.,0.));
#100210=DIRECTION('center_axis',(0.,-1.,0.));
#100211=DIRECTION('ref_axis',(0.,0.,-1.));
#100212=DIRECTION('',(-0.190809912898503,0.,0.981627005099017));
#100213=DIRECTION('',(-0.981627005099017,0.,-0.190809912898503));
#100214=DIRECTION('',(-0.981627005099017,0.,-0.190809912898503));
#100215=DIRECTION('center_axis',(-0.981627005099017,0.,-0.190809912898503));
#100216=DIRECTION('ref_axis',(-0.190809912898503,0.,0.981627005099017));
#100217=DIRECTION('',(0.,1.,0.));
#100218=DIRECTION('',(0.,1.,0.));
#100219=DIRECTION('center_axis',(0.,1.,0.));
#100220=DIRECTION('ref_axis',(1.,0.,0.));
#100221=DIRECTION('',(-0.190809912898503,0.,0.981627005099017));
#100222=DIRECTION('',(0.981627005099017,0.,0.190809912898503));
#100223=DIRECTION('',(-0.190809912898503,0.,0.981627005099017));
#100224=DIRECTION('',(0.981627005099017,0.,0.190809912898503));
#100225=DIRECTION('center_axis',(0.981627005099017,0.,0.190809912898503));
#100226=DIRECTION('ref_axis',(0.,-1.,0.));
#100227=DIRECTION('',(-0.190809912898503,0.,0.981627005099017));
#100228=DIRECTION('',(0.,-1.,0.));
#100229=DIRECTION('',(0.,-1.,0.));
#100230=DIRECTION('center_axis',(0.,-1.,0.));
#100231=DIRECTION('ref_axis',(0.,0.,-1.));
#100232=DIRECTION('',(-0.190809912898503,0.,0.981627005099017));
#100233=DIRECTION('',(-0.981627005099017,0.,-0.190809912898503));
#100234=DIRECTION('',(-0.981627005099017,0.,-0.190809912898503));
#100235=DIRECTION('center_axis',(-0.981627005099017,0.,-0.190809912898503));
#100236=DIRECTION('ref_axis',(-0.190809912898503,0.,0.981627005099017));
#100237=DIRECTION('',(0.,1.,0.));
#100238=DIRECTION('',(0.,1.,0.));
#100239=DIRECTION('center_axis',(0.,1.,0.));
#100240=DIRECTION('ref_axis',(1.,0.,0.));
#100241=DIRECTION('',(-0.190809912898503,0.,0.981627005099017));
#100242=DIRECTION('',(0.981627005099017,0.,0.190809912898503));
#100243=DIRECTION('',(-0.190809912898503,0.,0.981627005099017));
#100244=DIRECTION('',(0.981627005099017,0.,0.190809912898503));
#100245=DIRECTION('center_axis',(0.981627005099017,0.,0.190809912898503));
#100246=DIRECTION('ref_axis',(0.,-1.,0.));
#100247=DIRECTION('',(-0.190809912898503,0.,0.981627005099017));
#100248=DIRECTION('',(0.,-1.,0.));
#100249=DIRECTION('',(0.,-1.,0.));
#100250=DIRECTION('center_axis',(0.,-1.,0.));
#100251=DIRECTION('ref_axis',(0.,0.,-1.));
#100252=DIRECTION('',(-0.190809912898503,0.,0.981627005099017));
#100253=DIRECTION('',(-0.981627005099017,0.,-0.190809912898503));
#100254=DIRECTION('',(-0.981627005099017,0.,-0.190809912898503));
#100255=DIRECTION('center_axis',(-0.981627005099017,0.,-0.190809912898503));
#100256=DIRECTION('ref_axis',(-0.190809912898503,0.,0.981627005099017));
#100257=DIRECTION('',(0.,1.,0.));
#100258=DIRECTION('',(0.,1.,0.));
#100259=DIRECTION('center_axis',(0.,1.,0.));
#100260=DIRECTION('ref_axis',(1.,0.,0.));
#100261=DIRECTION('',(-0.190809912898503,0.,0.981627005099017));
#100262=DIRECTION('',(0.981627005099017,0.,0.190809912898503));
#100263=DIRECTION('',(-0.190809912898503,0.,0.981627005099017));
#100264=DIRECTION('',(0.981627005099017,0.,0.190809912898503));
#100265=DIRECTION('center_axis',(0.981627005099017,0.,0.190809912898503));
#100266=DIRECTION('ref_axis',(0.,-1.,0.));
#100267=DIRECTION('',(-0.190809912898503,0.,0.981627005099017));
#100268=DIRECTION('',(0.,-1.,0.));
#100269=DIRECTION('',(0.,-1.,0.));
#100270=DIRECTION('center_axis',(0.,-1.,0.));
#100271=DIRECTION('ref_axis',(0.,0.,-1.));
#100272=DIRECTION('',(-0.190809912898503,0.,0.981627005099017));
#100273=DIRECTION('',(-0.981627005099017,0.,-0.190809912898503));
#100274=DIRECTION('',(-0.981627005099017,0.,-0.190809912898503));
#100275=DIRECTION('center_axis',(-0.981627005099017,0.,-0.190809912898503));
#100276=DIRECTION('ref_axis',(-0.190809912898503,0.,0.981627005099017));
#100277=DIRECTION('',(0.,1.,0.));
#100278=DIRECTION('',(0.,1.,0.));
#100279=DIRECTION('center_axis',(0.,1.,0.));
#100280=DIRECTION('ref_axis',(1.,0.,0.));
#100281=DIRECTION('',(-0.190809912898503,0.,0.981627005099017));
#100282=DIRECTION('',(0.981627005099017,0.,0.190809912898503));
#100283=DIRECTION('',(-0.190809912898503,0.,0.981627005099017));
#100284=DIRECTION('',(0.981627005099017,0.,0.190809912898503));
#100285=DIRECTION('center_axis',(0.981627005099017,0.,0.190809912898503));
#100286=DIRECTION('ref_axis',(0.,-1.,0.));
#100287=DIRECTION('',(-0.190809912898503,0.,0.981627005099017));
#100288=DIRECTION('',(0.,-1.,0.));
#100289=DIRECTION('',(0.,-1.,0.));
#100290=DIRECTION('center_axis',(0.,-1.,0.));
#100291=DIRECTION('ref_axis',(0.,0.,-1.));
#100292=DIRECTION('',(-0.190809912898503,0.,0.981627005099017));
#100293=DIRECTION('',(-0.981627005099017,0.,-0.190809912898503));
#100294=DIRECTION('',(-0.981627005099017,0.,-0.190809912898503));
#100295=DIRECTION('center_axis',(-0.981627005099017,0.,-0.190809912898503));
#100296=DIRECTION('ref_axis',(-0.190809912898503,0.,0.981627005099017));
#100297=DIRECTION('',(0.,1.,0.));
#100298=DIRECTION('',(0.,1.,0.));
#100299=DIRECTION('center_axis',(0.,1.,0.));
#100300=DIRECTION('ref_axis',(1.,0.,0.));
#100301=DIRECTION('',(-0.190809912898503,0.,0.981627005099017));
#100302=DIRECTION('',(0.981627005099017,0.,0.190809912898503));
#100303=DIRECTION('',(-0.190809912898503,0.,0.981627005099017));
#100304=DIRECTION('',(0.981627005099017,0.,0.190809912898503));
#100305=DIRECTION('center_axis',(0.981627005099017,0.,0.190809912898503));
#100306=DIRECTION('ref_axis',(0.,-1.,0.));
#100307=DIRECTION('',(-0.190809912898503,0.,0.981627005099017));
#100308=DIRECTION('',(0.,-1.,0.));
#100309=DIRECTION('',(0.,-1.,0.));
#100310=DIRECTION('center_axis',(0.,-1.,0.));
#100311=DIRECTION('ref_axis',(0.,0.,-1.));
#100312=DIRECTION('',(-0.190809912898503,0.,0.981627005099017));
#100313=DIRECTION('',(-0.981627005099017,0.,-0.190809912898503));
#100314=DIRECTION('',(-0.981627005099017,0.,-0.190809912898503));
#100315=DIRECTION('center_axis',(-0.981627005099017,0.,-0.190809912898503));
#100316=DIRECTION('ref_axis',(-0.190809912898503,0.,0.981627005099017));
#100317=DIRECTION('',(0.,1.,0.));
#100318=DIRECTION('',(0.,1.,0.));
#100319=DIRECTION('center_axis',(0.,1.,0.));
#100320=DIRECTION('ref_axis',(1.,0.,0.));
#100321=DIRECTION('',(-0.190809912898503,0.,0.981627005099017));
#100322=DIRECTION('',(0.981627005099017,0.,0.190809912898503));
#100323=DIRECTION('',(-0.190809912898503,0.,0.981627005099017));
#100324=DIRECTION('',(0.981627005099017,0.,0.190809912898503));
#100325=DIRECTION('center_axis',(0.981627005099017,0.,0.190809912898503));
#100326=DIRECTION('ref_axis',(0.,-1.,0.));
#100327=DIRECTION('',(-0.190809912898503,0.,0.981627005099017));
#100328=DIRECTION('',(0.,-1.,0.));
#100329=DIRECTION('',(0.,-1.,0.));
#100330=DIRECTION('center_axis',(0.,-1.,0.));
#100331=DIRECTION('ref_axis',(0.,0.,-1.));
#100332=DIRECTION('',(-0.190809912898503,0.,0.981627005099017));
#100333=DIRECTION('',(-0.981627005099017,0.,-0.190809912898503));
#100334=DIRECTION('',(-0.981627005099017,0.,-0.190809912898503));
#100335=DIRECTION('center_axis',(-0.981627005099017,0.,-0.190809912898503));
#100336=DIRECTION('ref_axis',(-0.190809912898503,0.,0.981627005099017));
#100337=DIRECTION('',(0.,1.,0.));
#100338=DIRECTION('',(0.,1.,0.));
#100339=DIRECTION('center_axis',(0.,1.,0.));
#100340=DIRECTION('ref_axis',(1.,0.,0.));
#100341=DIRECTION('',(-0.190809912898503,0.,0.981627005099017));
#100342=DIRECTION('',(0.981627005099017,0.,0.190809912898503));
#100343=DIRECTION('',(-0.190809912898503,0.,0.981627005099017));
#100344=DIRECTION('',(0.981627005099017,0.,0.190809912898503));
#100345=DIRECTION('center_axis',(0.981627005099017,0.,0.190809912898503));
#100346=DIRECTION('ref_axis',(0.,-1.,0.));
#100347=DIRECTION('',(-0.190809912898503,0.,0.981627005099017));
#100348=DIRECTION('',(0.,-1.,0.));
#100349=DIRECTION('',(0.,-1.,0.));
#100350=DIRECTION('center_axis',(0.,-1.,0.));
#100351=DIRECTION('ref_axis',(0.,0.,-1.));
#100352=DIRECTION('',(-0.190809912898503,0.,0.981627005099017));
#100353=DIRECTION('',(-0.981627005099017,0.,-0.190809912898503));
#100354=DIRECTION('',(-0.981627005099017,0.,-0.190809912898503));
#100355=DIRECTION('center_axis',(-0.981627005099017,0.,-0.190809912898503));
#100356=DIRECTION('ref_axis',(-0.190809912898503,0.,0.981627005099017));
#100357=DIRECTION('',(0.,1.,0.));
#100358=DIRECTION('',(0.,1.,0.));
#100359=DIRECTION('center_axis',(0.,1.,0.));
#100360=DIRECTION('ref_axis',(1.,0.,0.));
#100361=DIRECTION('',(-0.190809912898503,0.,0.981627005099017));
#100362=DIRECTION('',(0.981627005099017,0.,0.190809912898503));
#100363=DIRECTION('',(-0.190809912898503,0.,0.981627005099017));
#100364=DIRECTION('',(0.981627005099017,0.,0.190809912898503));
#100365=DIRECTION('center_axis',(0.981627005099017,0.,0.190809912898503));
#100366=DIRECTION('ref_axis',(0.,-1.,0.));
#100367=DIRECTION('',(-0.190809912898503,0.,0.981627005099017));
#100368=DIRECTION('',(0.,-1.,0.));
#100369=DIRECTION('',(0.,-1.,0.));
#100370=DIRECTION('center_axis',(0.,-1.,0.));
#100371=DIRECTION('ref_axis',(0.,0.,-1.));
#100372=DIRECTION('',(-0.190809912898503,0.,0.981627005099017));
#100373=DIRECTION('',(-0.981627005099017,0.,-0.190809912898503));
#100374=DIRECTION('',(-0.981627005099017,0.,-0.190809912898503));
#100375=DIRECTION('center_axis',(-0.981627005099017,0.,-0.190809912898503));
#100376=DIRECTION('ref_axis',(-0.190809912898503,0.,0.981627005099017));
#100377=DIRECTION('',(0.,1.,0.));
#100378=DIRECTION('',(0.,1.,0.));
#100379=DIRECTION('center_axis',(0.,1.,0.));
#100380=DIRECTION('ref_axis',(1.,0.,0.));
#100381=DIRECTION('',(-0.190809912898503,0.,0.981627005099017));
#100382=DIRECTION('',(0.981627005099017,0.,0.190809912898503));
#100383=DIRECTION('',(-0.190809912898503,0.,0.981627005099017));
#100384=DIRECTION('',(0.981627005099017,0.,0.190809912898503));
#100385=DIRECTION('center_axis',(0.981627005099017,0.,0.190809912898503));
#100386=DIRECTION('ref_axis',(0.,-1.,0.));
#100387=DIRECTION('',(-0.190809912898503,0.,0.981627005099017));
#100388=DIRECTION('',(0.,-1.,0.));
#100389=DIRECTION('',(0.,-1.,0.));
#100390=DIRECTION('center_axis',(0.,-1.,0.));
#100391=DIRECTION('ref_axis',(0.,0.,-1.));
#100392=DIRECTION('',(-0.190809912898503,0.,0.981627005099017));
#100393=DIRECTION('',(-0.981627005099017,0.,-0.190809912898503));
#100394=DIRECTION('',(-0.981627005099017,0.,-0.190809912898503));
#100395=DIRECTION('center_axis',(-0.981627005099017,0.,-0.190809912898503));
#100396=DIRECTION('ref_axis',(-0.190809912898503,0.,0.981627005099017));
#100397=DIRECTION('',(0.,1.,0.));
#100398=DIRECTION('',(0.,1.,0.));
#100399=DIRECTION('center_axis',(0.,1.,0.));
#100400=DIRECTION('ref_axis',(1.,0.,0.));
#100401=DIRECTION('',(-0.190809912898503,0.,0.981627005099017));
#100402=DIRECTION('',(0.981627005099017,0.,0.190809912898503));
#100403=DIRECTION('',(-0.190809912898503,0.,0.981627005099017));
#100404=DIRECTION('',(0.981627005099017,0.,0.190809912898503));
#100405=DIRECTION('center_axis',(0.981627005099017,0.,0.190809912898503));
#100406=DIRECTION('ref_axis',(0.,-1.,0.));
#100407=DIRECTION('',(-0.190809912898503,0.,0.981627005099017));
#100408=DIRECTION('',(0.,-1.,0.));
#100409=DIRECTION('',(0.,-1.,0.));
#100410=DIRECTION('center_axis',(0.,-1.,0.));
#100411=DIRECTION('ref_axis',(0.,0.,-1.));
#100412=DIRECTION('',(-0.190809912898503,0.,0.981627005099017));
#100413=DIRECTION('',(-0.981627005099017,0.,-0.190809912898503));
#100414=DIRECTION('',(-0.981627005099017,0.,-0.190809912898503));
#100415=DIRECTION('center_axis',(-0.981627005099017,0.,-0.190809912898503));
#100416=DIRECTION('ref_axis',(-0.190809912898503,0.,0.981627005099017));
#100417=DIRECTION('',(0.,1.,0.));
#100418=DIRECTION('',(0.,1.,0.));
#100419=DIRECTION('center_axis',(0.,1.,0.));
#100420=DIRECTION('ref_axis',(1.,0.,0.));
#100421=DIRECTION('',(-0.190809912898503,0.,0.981627005099017));
#100422=DIRECTION('',(0.981627005099017,0.,0.190809912898503));
#100423=DIRECTION('',(-0.190809912898503,0.,0.981627005099017));
#100424=DIRECTION('',(0.981627005099017,0.,0.190809912898503));
#100425=DIRECTION('center_axis',(0.981627005099017,0.,0.190809912898503));
#100426=DIRECTION('ref_axis',(0.,-1.,0.));
#100427=DIRECTION('',(-0.190809912898503,0.,0.981627005099017));
#100428=DIRECTION('',(0.,-1.,0.));
#100429=DIRECTION('',(0.,-1.,0.));
#100430=DIRECTION('center_axis',(0.,-1.,0.));
#100431=DIRECTION('ref_axis',(0.,0.,-1.));
#100432=DIRECTION('',(-0.190809912898503,0.,0.981627005099017));
#100433=DIRECTION('',(-0.981627005099017,0.,-0.190809912898503));
#100434=DIRECTION('',(-0.981627005099017,0.,-0.190809912898503));
#100435=DIRECTION('center_axis',(-0.981627005099017,0.,-0.190809912898503));
#100436=DIRECTION('ref_axis',(-0.190809912898503,0.,0.981627005099017));
#100437=DIRECTION('',(0.,1.,0.));
#100438=DIRECTION('',(0.,1.,0.));
#100439=DIRECTION('center_axis',(0.,1.,0.));
#100440=DIRECTION('ref_axis',(1.,0.,0.));
#100441=DIRECTION('',(-0.190809912898503,0.,0.981627005099017));
#100442=DIRECTION('',(0.981627005099017,0.,0.190809912898503));
#100443=DIRECTION('',(-0.190809912898503,0.,0.981627005099017));
#100444=DIRECTION('',(0.981627005099017,0.,0.190809912898503));
#100445=DIRECTION('center_axis',(0.981627005099017,0.,0.190809912898503));
#100446=DIRECTION('ref_axis',(0.,-1.,0.));
#100447=DIRECTION('',(-0.190809912898503,0.,0.981627005099017));
#100448=DIRECTION('',(0.,-1.,0.));
#100449=DIRECTION('',(0.,-1.,0.));
#100450=DIRECTION('center_axis',(0.,-1.,0.));
#100451=DIRECTION('ref_axis',(0.,0.,-1.));
#100452=DIRECTION('',(-0.190809912898503,0.,0.981627005099017));
#100453=DIRECTION('',(-0.981627005099017,0.,-0.190809912898503));
#100454=DIRECTION('',(-0.981627005099017,0.,-0.190809912898503));
#100455=DIRECTION('center_axis',(-0.981627005099017,0.,-0.190809912898503));
#100456=DIRECTION('ref_axis',(-0.190809912898503,0.,0.981627005099017));
#100457=DIRECTION('',(0.,1.,0.));
#100458=DIRECTION('',(0.,1.,0.));
#100459=DIRECTION('center_axis',(0.,1.,0.));
#100460=DIRECTION('ref_axis',(1.,0.,0.));
#100461=DIRECTION('',(-0.190809912898503,0.,0.981627005099017));
#100462=DIRECTION('',(0.981627005099017,0.,0.190809912898503));
#100463=DIRECTION('',(-0.190809912898503,0.,0.981627005099017));
#100464=DIRECTION('',(0.981627005099017,0.,0.190809912898503));
#100465=DIRECTION('center_axis',(0.981627005099017,0.,0.190809912898503));
#100466=DIRECTION('ref_axis',(0.,-1.,0.));
#100467=DIRECTION('',(-0.190809912898503,0.,0.981627005099017));
#100468=DIRECTION('',(0.,-1.,0.));
#100469=DIRECTION('',(0.,-1.,0.));
#100470=DIRECTION('center_axis',(0.,-1.,0.));
#100471=DIRECTION('ref_axis',(0.,0.,-1.));
#100472=DIRECTION('',(-0.190809912898503,0.,0.981627005099017));
#100473=DIRECTION('',(-0.981627005099017,0.,-0.190809912898503));
#100474=DIRECTION('',(-0.981627005099017,0.,-0.190809912898503));
#100475=DIRECTION('center_axis',(-0.981627005099017,0.,-0.190809912898503));
#100476=DIRECTION('ref_axis',(-0.190809912898503,0.,0.981627005099017));
#100477=DIRECTION('',(0.,1.,0.));
#100478=DIRECTION('',(0.,1.,0.));
#100479=DIRECTION('center_axis',(0.,1.,0.));
#100480=DIRECTION('ref_axis',(1.,0.,0.));
#100481=DIRECTION('',(-0.190809912898503,0.,0.981627005099017));
#100482=DIRECTION('',(0.981627005099017,0.,0.190809912898503));
#100483=DIRECTION('',(-0.190809912898503,0.,0.981627005099017));
#100484=DIRECTION('',(0.981627005099017,0.,0.190809912898503));
#100485=DIRECTION('center_axis',(0.981627005099017,0.,0.190809912898503));
#100486=DIRECTION('ref_axis',(0.,-1.,0.));
#100487=DIRECTION('',(-0.190809912898503,0.,0.981627005099017));
#100488=DIRECTION('',(0.,-1.,0.));
#100489=DIRECTION('',(0.,-1.,0.));
#100490=DIRECTION('center_axis',(0.,-1.,0.));
#100491=DIRECTION('ref_axis',(0.,0.,-1.));
#100492=DIRECTION('',(-0.190809912898503,0.,0.981627005099017));
#100493=DIRECTION('',(-0.981627005099017,0.,-0.190809912898503));
#100494=DIRECTION('',(-0.981627005099017,0.,-0.190809912898503));
#100495=DIRECTION('center_axis',(-0.981627005099017,0.,-0.190809912898503));
#100496=DIRECTION('ref_axis',(-0.190809912898503,0.,0.981627005099017));
#100497=DIRECTION('',(0.,1.,0.));
#100498=DIRECTION('',(0.,1.,0.));
#100499=DIRECTION('center_axis',(0.,1.,0.));
#100500=DIRECTION('ref_axis',(1.,0.,0.));
#100501=DIRECTION('',(-0.190809912898503,0.,0.981627005099017));
#100502=DIRECTION('',(0.981627005099017,0.,0.190809912898503));
#100503=DIRECTION('',(-0.190809912898503,0.,0.981627005099017));
#100504=DIRECTION('',(0.981627005099017,0.,0.190809912898503));
#100505=DIRECTION('center_axis',(0.981627005099017,0.,0.190809912898503));
#100506=DIRECTION('ref_axis',(0.,-1.,0.));
#100507=DIRECTION('',(-0.190809912898503,0.,0.981627005099017));
#100508=DIRECTION('',(0.,-1.,0.));
#100509=DIRECTION('',(0.,-1.,0.));
#100510=DIRECTION('center_axis',(0.,-1.,0.));
#100511=DIRECTION('ref_axis',(0.,0.,-1.));
#100512=DIRECTION('',(-0.190809912898503,0.,0.981627005099017));
#100513=DIRECTION('',(-0.981627005099017,0.,-0.190809912898503));
#100514=DIRECTION('',(-0.981627005099017,0.,-0.190809912898503));
#100515=DIRECTION('center_axis',(-0.981627005099017,0.,-0.190809912898503));
#100516=DIRECTION('ref_axis',(-0.190809912898503,0.,0.981627005099017));
#100517=DIRECTION('',(0.,1.,0.));
#100518=DIRECTION('',(0.,1.,0.));
#100519=DIRECTION('center_axis',(0.,1.,0.));
#100520=DIRECTION('ref_axis',(1.,0.,0.));
#100521=DIRECTION('',(-0.190809912898503,0.,0.981627005099017));
#100522=DIRECTION('',(0.981627005099017,0.,0.190809912898503));
#100523=DIRECTION('',(-0.190809912898503,0.,0.981627005099017));
#100524=DIRECTION('',(0.981627005099017,0.,0.190809912898503));
#100525=DIRECTION('center_axis',(0.981627005099017,0.,0.190809912898503));
#100526=DIRECTION('ref_axis',(0.,-1.,0.));
#100527=DIRECTION('',(-0.190809912898503,0.,0.981627005099017));
#100528=DIRECTION('',(0.,-1.,0.));
#100529=DIRECTION('',(0.,-1.,0.));
#100530=DIRECTION('center_axis',(0.,-1.,0.));
#100531=DIRECTION('ref_axis',(0.,0.,-1.));
#100532=DIRECTION('',(-0.190809912898503,0.,0.981627005099017));
#100533=DIRECTION('',(-0.981627005099017,0.,-0.190809912898503));
#100534=DIRECTION('',(-0.981627005099017,0.,-0.190809912898503));
#100535=DIRECTION('center_axis',(-0.981627005099017,0.,-0.190809912898503));
#100536=DIRECTION('ref_axis',(-0.190809912898503,0.,0.981627005099017));
#100537=DIRECTION('',(0.,1.,0.));
#100538=DIRECTION('',(0.,1.,0.));
#100539=DIRECTION('center_axis',(0.,1.,0.));
#100540=DIRECTION('ref_axis',(1.,0.,0.));
#100541=DIRECTION('',(-0.190809912898503,0.,0.981627005099017));
#100542=DIRECTION('',(0.981627005099017,0.,0.190809912898503));
#100543=DIRECTION('',(-0.190809912898503,0.,0.981627005099017));
#100544=DIRECTION('',(0.981627005099017,0.,0.190809912898503));
#100545=DIRECTION('center_axis',(0.981627005099017,0.,0.190809912898503));
#100546=DIRECTION('ref_axis',(0.,-1.,0.));
#100547=DIRECTION('',(-0.190809912898503,0.,0.981627005099017));
#100548=DIRECTION('',(0.,-1.,0.));
#100549=DIRECTION('',(0.,-1.,0.));
#100550=DIRECTION('center_axis',(0.,-1.,0.));
#100551=DIRECTION('ref_axis',(0.,0.,-1.));
#100552=DIRECTION('',(-0.190809912898503,0.,0.981627005099017));
#100553=DIRECTION('',(-0.981627005099017,0.,-0.190809912898503));
#100554=DIRECTION('',(-0.981627005099017,0.,-0.190809912898503));
#100555=DIRECTION('center_axis',(-0.981627005099017,0.,-0.190809912898503));
#100556=DIRECTION('ref_axis',(-0.190809912898503,0.,0.981627005099017));
#100557=DIRECTION('',(0.,1.,0.));
#100558=DIRECTION('',(0.,1.,0.));
#100559=DIRECTION('center_axis',(0.,1.,0.));
#100560=DIRECTION('ref_axis',(1.,0.,0.));
#100561=DIRECTION('',(-0.190809912898503,0.,0.981627005099017));
#100562=DIRECTION('',(0.981627005099017,0.,0.190809912898503));
#100563=DIRECTION('',(-0.190809912898503,0.,0.981627005099017));
#100564=DIRECTION('',(0.981627005099017,0.,0.190809912898503));
#100565=DIRECTION('center_axis',(0.981627005099017,0.,0.190809912898503));
#100566=DIRECTION('ref_axis',(0.,-1.,0.));
#100567=DIRECTION('',(-0.190809912898503,0.,0.981627005099017));
#100568=DIRECTION('',(0.,-1.,0.));
#100569=DIRECTION('',(0.,-1.,0.));
#100570=DIRECTION('center_axis',(0.,-1.,0.));
#100571=DIRECTION('ref_axis',(0.,0.,-1.));
#100572=DIRECTION('',(-0.190809912898503,0.,0.981627005099017));
#100573=DIRECTION('',(-0.981627005099017,0.,-0.190809912898503));
#100574=DIRECTION('',(-0.981627005099017,0.,-0.190809912898503));
#100575=DIRECTION('center_axis',(-0.981627005099017,0.,-0.190809912898503));
#100576=DIRECTION('ref_axis',(-0.190809912898503,0.,0.981627005099017));
#100577=DIRECTION('',(0.,1.,0.));
#100578=DIRECTION('',(0.,1.,0.));
#100579=DIRECTION('center_axis',(0.,1.,0.));
#100580=DIRECTION('ref_axis',(1.,0.,0.));
#100581=DIRECTION('',(-0.190809912898503,0.,0.981627005099017));
#100582=DIRECTION('',(0.981627005099017,0.,0.190809912898503));
#100583=DIRECTION('',(-0.190809912898503,0.,0.981627005099017));
#100584=DIRECTION('',(0.981627005099017,0.,0.190809912898503));
#100585=DIRECTION('center_axis',(0.981627005099017,0.,0.190809912898503));
#100586=DIRECTION('ref_axis',(0.,-1.,0.));
#100587=DIRECTION('',(-0.190809912898503,0.,0.981627005099017));
#100588=DIRECTION('',(0.,-1.,0.));
#100589=DIRECTION('',(0.,-1.,0.));
#100590=DIRECTION('center_axis',(0.,-1.,0.));
#100591=DIRECTION('ref_axis',(0.,0.,-1.));
#100592=DIRECTION('',(-0.190809912898503,0.,0.981627005099017));
#100593=DIRECTION('',(-0.981627005099017,0.,-0.190809912898503));
#100594=DIRECTION('',(-0.981627005099017,0.,-0.190809912898503));
#100595=DIRECTION('center_axis',(-0.981627005099017,0.,-0.190809912898503));
#100596=DIRECTION('ref_axis',(-0.190809912898503,0.,0.981627005099017));
#100597=DIRECTION('',(0.,1.,0.));
#100598=DIRECTION('',(0.,1.,0.));
#100599=DIRECTION('center_axis',(0.,1.,0.));
#100600=DIRECTION('ref_axis',(1.,0.,0.));
#100601=DIRECTION('',(-0.190809912898503,0.,0.981627005099017));
#100602=DIRECTION('',(0.981627005099017,0.,0.190809912898503));
#100603=DIRECTION('',(-0.190809912898503,0.,0.981627005099017));
#100604=DIRECTION('',(0.981627005099017,0.,0.190809912898503));
#100605=DIRECTION('center_axis',(0.981627005099017,0.,0.190809912898503));
#100606=DIRECTION('ref_axis',(0.,-1.,0.));
#100607=DIRECTION('',(-0.190809912898503,0.,0.981627005099017));
#100608=DIRECTION('',(0.,-1.,0.));
#100609=DIRECTION('',(0.,-1.,0.));
#100610=DIRECTION('center_axis',(0.,-1.,0.));
#100611=DIRECTION('ref_axis',(0.,0.,-1.));
#100612=DIRECTION('',(-0.190809912898503,0.,0.981627005099017));
#100613=DIRECTION('',(-0.981627005099017,0.,-0.190809912898503));
#100614=DIRECTION('',(-0.981627005099017,0.,-0.190809912898503));
#100615=DIRECTION('center_axis',(-0.981627005099017,0.,-0.190809912898503));
#100616=DIRECTION('ref_axis',(-0.190809912898503,0.,0.981627005099017));
#100617=DIRECTION('',(0.,1.,0.));
#100618=DIRECTION('',(0.,1.,0.));
#100619=DIRECTION('center_axis',(0.,1.,0.));
#100620=DIRECTION('ref_axis',(1.,0.,0.));
#100621=DIRECTION('',(-0.190809912898503,0.,0.981627005099017));
#100622=DIRECTION('',(0.981627005099017,0.,0.190809912898503));
#100623=DIRECTION('',(-0.190809912898503,0.,0.981627005099017));
#100624=DIRECTION('',(0.981627005099017,0.,0.190809912898503));
#100625=DIRECTION('center_axis',(0.981627005099017,0.,0.190809912898503));
#100626=DIRECTION('ref_axis',(0.,-1.,0.));
#100627=DIRECTION('',(-0.190809912898503,0.,0.981627005099017));
#100628=DIRECTION('',(0.,-1.,0.));
#100629=DIRECTION('',(0.,-1.,0.));
#100630=DIRECTION('center_axis',(0.,-1.,0.));
#100631=DIRECTION('ref_axis',(0.,0.,-1.));
#100632=DIRECTION('',(-0.190809912898503,0.,0.981627005099017));
#100633=DIRECTION('',(-0.981627005099017,0.,-0.190809912898503));
#100634=DIRECTION('',(-0.981627005099017,0.,-0.190809912898503));
#100635=DIRECTION('center_axis',(-0.981627005099017,0.,-0.190809912898503));
#100636=DIRECTION('ref_axis',(-0.190809912898503,0.,0.981627005099017));
#100637=DIRECTION('',(0.,1.,0.));
#100638=DIRECTION('',(0.,1.,0.));
#100639=DIRECTION('center_axis',(0.,1.,0.));
#100640=DIRECTION('ref_axis',(1.,0.,0.));
#100641=DIRECTION('',(-0.190809912898503,0.,0.981627005099017));
#100642=DIRECTION('',(0.981627005099017,0.,0.190809912898503));
#100643=DIRECTION('',(-0.190809912898503,0.,0.981627005099017));
#100644=DIRECTION('',(0.981627005099017,0.,0.190809912898503));
#100645=DIRECTION('center_axis',(0.981627005099017,0.,0.190809912898503));
#100646=DIRECTION('ref_axis',(0.,-1.,0.));
#100647=DIRECTION('',(-0.190809912898503,0.,0.981627005099017));
#100648=DIRECTION('',(0.,-1.,0.));
#100649=DIRECTION('',(0.,-1.,0.));
#100650=DIRECTION('center_axis',(0.,-1.,0.));
#100651=DIRECTION('ref_axis',(0.,0.,-1.));
#100652=DIRECTION('',(-0.190809912898503,0.,0.981627005099017));
#100653=DIRECTION('',(-0.981627005099017,0.,-0.190809912898503));
#100654=DIRECTION('',(-0.981627005099017,0.,-0.190809912898503));
#100655=DIRECTION('center_axis',(-0.981627005099017,0.,-0.190809912898503));
#100656=DIRECTION('ref_axis',(-0.190809912898503,0.,0.981627005099017));
#100657=DIRECTION('',(0.,1.,0.));
#100658=DIRECTION('',(0.,1.,0.));
#100659=DIRECTION('center_axis',(0.,1.,0.));
#100660=DIRECTION('ref_axis',(1.,0.,0.));
#100661=DIRECTION('',(-0.190809912898503,0.,0.981627005099017));
#100662=DIRECTION('',(0.981627005099017,0.,0.190809912898503));
#100663=DIRECTION('',(-0.190809912898503,0.,0.981627005099017));
#100664=DIRECTION('',(0.981627005099017,0.,0.190809912898503));
#100665=DIRECTION('center_axis',(0.981627005099017,0.,0.190809912898503));
#100666=DIRECTION('ref_axis',(0.,-1.,0.));
#100667=DIRECTION('',(-0.190809912898503,0.,0.981627005099017));
#100668=DIRECTION('',(0.,-1.,0.));
#100669=DIRECTION('',(0.,-1.,0.));
#100670=DIRECTION('center_axis',(0.,-1.,0.));
#100671=DIRECTION('ref_axis',(0.,0.,-1.));
#100672=DIRECTION('',(-0.190809912898503,0.,0.981627005099017));
#100673=DIRECTION('',(-0.981627005099017,0.,-0.190809912898503));
#100674=DIRECTION('',(-0.981627005099017,0.,-0.190809912898503));
#100675=DIRECTION('center_axis',(-0.981627005099017,0.,-0.190809912898503));
#100676=DIRECTION('ref_axis',(-0.190809912898503,0.,0.981627005099017));
#100677=DIRECTION('',(0.,1.,0.));
#100678=DIRECTION('',(0.,1.,0.));
#100679=DIRECTION('center_axis',(0.,1.,0.));
#100680=DIRECTION('ref_axis',(1.,0.,0.));
#100681=DIRECTION('',(-0.190809912898503,0.,0.981627005099017));
#100682=DIRECTION('',(0.981627005099017,0.,0.190809912898503));
#100683=DIRECTION('',(-0.190809912898503,0.,0.981627005099017));
#100684=DIRECTION('',(0.981627005099017,0.,0.190809912898503));
#100685=DIRECTION('center_axis',(0.981627005099017,0.,0.190809912898503));
#100686=DIRECTION('ref_axis',(0.,-1.,0.));
#100687=DIRECTION('',(-0.190809912898503,0.,0.981627005099017));
#100688=DIRECTION('',(0.,-1.,0.));
#100689=DIRECTION('',(0.,-1.,0.));
#100690=DIRECTION('center_axis',(0.,-1.,0.));
#100691=DIRECTION('ref_axis',(0.,0.,-1.));
#100692=DIRECTION('',(-0.190809912898503,0.,0.981627005099017));
#100693=DIRECTION('',(-0.981627005099017,0.,-0.190809912898503));
#100694=DIRECTION('',(-0.981627005099017,0.,-0.190809912898503));
#100695=DIRECTION('center_axis',(-0.981627005099017,0.,-0.190809912898503));
#100696=DIRECTION('ref_axis',(-0.190809912898503,0.,0.981627005099017));
#100697=DIRECTION('',(0.,1.,0.));
#100698=DIRECTION('',(0.,1.,0.));
#100699=DIRECTION('center_axis',(0.,1.,0.));
#100700=DIRECTION('ref_axis',(1.,0.,0.));
#100701=DIRECTION('',(-0.190809912898503,0.,0.981627005099017));
#100702=DIRECTION('',(0.981627005099017,0.,0.190809912898503));
#100703=DIRECTION('',(-0.190809912898503,0.,0.981627005099017));
#100704=DIRECTION('',(0.981627005099017,0.,0.190809912898503));
#100705=DIRECTION('center_axis',(0.981627005099017,0.,0.190809912898503));
#100706=DIRECTION('ref_axis',(0.,-1.,0.));
#100707=DIRECTION('',(-0.190809912898503,0.,0.981627005099017));
#100708=DIRECTION('',(0.,-1.,0.));
#100709=DIRECTION('',(0.,-1.,0.));
#100710=DIRECTION('center_axis',(0.,-1.,0.));
#100711=DIRECTION('ref_axis',(0.,0.,-1.));
#100712=DIRECTION('',(-0.190809912898503,0.,0.981627005099017));
#100713=DIRECTION('',(-0.981627005099017,0.,-0.190809912898503));
#100714=DIRECTION('',(-0.981627005099017,0.,-0.190809912898503));
#100715=DIRECTION('center_axis',(-0.981627005099017,0.,-0.190809912898503));
#100716=DIRECTION('ref_axis',(-0.190809912898503,0.,0.981627005099017));
#100717=DIRECTION('',(0.,1.,0.));
#100718=DIRECTION('',(0.,1.,0.));
#100719=DIRECTION('center_axis',(0.,1.,0.));
#100720=DIRECTION('ref_axis',(1.,0.,0.));
#100721=DIRECTION('',(-0.190809912898503,0.,0.981627005099017));
#100722=DIRECTION('',(0.981627005099017,0.,0.190809912898503));
#100723=DIRECTION('',(-0.190809912898503,0.,0.981627005099017));
#100724=DIRECTION('',(0.981627005099017,0.,0.190809912898503));
#100725=DIRECTION('center_axis',(0.981627005099017,0.,0.190809912898503));
#100726=DIRECTION('ref_axis',(0.,-1.,0.));
#100727=DIRECTION('',(-0.190809912898503,0.,0.981627005099017));
#100728=DIRECTION('',(0.,-1.,0.));
#100729=DIRECTION('',(0.,-1.,0.));
#100730=DIRECTION('center_axis',(0.,-1.,0.));
#100731=DIRECTION('ref_axis',(0.,0.,-1.));
#100732=DIRECTION('',(-0.190809912898503,0.,0.981627005099017));
#100733=DIRECTION('',(-0.981627005099017,0.,-0.190809912898503));
#100734=DIRECTION('',(-0.981627005099017,0.,-0.190809912898503));
#100735=DIRECTION('center_axis',(-0.981627005099017,0.,-0.190809912898503));
#100736=DIRECTION('ref_axis',(-0.190809912898503,0.,0.981627005099017));
#100737=DIRECTION('',(0.,1.,0.));
#100738=DIRECTION('',(0.,1.,0.));
#100739=DIRECTION('center_axis',(0.,1.,0.));
#100740=DIRECTION('ref_axis',(1.,0.,0.));
#100741=DIRECTION('',(-0.190809912898503,0.,0.981627005099017));
#100742=DIRECTION('',(0.981627005099017,0.,0.190809912898503));
#100743=DIRECTION('',(-0.190809912898503,0.,0.981627005099017));
#100744=DIRECTION('',(0.981627005099017,0.,0.190809912898503));
#100745=DIRECTION('center_axis',(0.981627005099017,0.,0.190809912898503));
#100746=DIRECTION('ref_axis',(0.,-1.,0.));
#100747=DIRECTION('',(-0.190809912898503,0.,0.981627005099017));
#100748=DIRECTION('',(0.,-1.,0.));
#100749=DIRECTION('',(0.,-1.,0.));
#100750=DIRECTION('center_axis',(0.,-1.,0.));
#100751=DIRECTION('ref_axis',(0.,0.,-1.));
#100752=DIRECTION('',(-0.190809912898503,0.,0.981627005099017));
#100753=DIRECTION('',(-0.981627005099017,0.,-0.190809912898503));
#100754=DIRECTION('',(-0.981627005099017,0.,-0.190809912898503));
#100755=DIRECTION('center_axis',(-0.981627005099017,0.,-0.190809912898503));
#100756=DIRECTION('ref_axis',(-0.190809912898503,0.,0.981627005099017));
#100757=DIRECTION('',(0.,1.,0.));
#100758=DIRECTION('',(0.,1.,0.));
#100759=DIRECTION('center_axis',(0.,1.,0.));
#100760=DIRECTION('ref_axis',(1.,0.,0.));
#100761=DIRECTION('',(-0.190809912898503,0.,0.981627005099017));
#100762=DIRECTION('',(0.981627005099017,0.,0.190809912898503));
#100763=DIRECTION('',(-0.190809912898503,0.,0.981627005099017));
#100764=DIRECTION('',(0.981627005099017,0.,0.190809912898503));
#100765=DIRECTION('center_axis',(0.981627005099017,0.,0.190809912898503));
#100766=DIRECTION('ref_axis',(0.,-1.,0.));
#100767=DIRECTION('',(-0.190809912898503,0.,0.981627005099017));
#100768=DIRECTION('',(0.,-1.,0.));
#100769=DIRECTION('',(0.,-1.,0.));
#100770=DIRECTION('center_axis',(0.,-1.,0.));
#100771=DIRECTION('ref_axis',(0.,0.,-1.));
#100772=DIRECTION('',(-0.190809912898503,0.,0.981627005099017));
#100773=DIRECTION('',(-0.981627005099017,0.,-0.190809912898503));
#100774=DIRECTION('',(-0.981627005099017,0.,-0.190809912898503));
#100775=DIRECTION('center_axis',(-0.981627005099017,0.,-0.190809912898503));
#100776=DIRECTION('ref_axis',(-0.190809912898503,0.,0.981627005099017));
#100777=DIRECTION('',(0.,1.,0.));
#100778=DIRECTION('',(0.,1.,0.));
#100779=DIRECTION('center_axis',(0.,1.,0.));
#100780=DIRECTION('ref_axis',(1.,0.,0.));
#100781=DIRECTION('',(-0.190809912898503,0.,0.981627005099017));
#100782=DIRECTION('',(0.981627005099017,0.,0.190809912898503));
#100783=DIRECTION('',(-0.190809912898503,0.,0.981627005099017));
#100784=DIRECTION('',(0.981627005099017,0.,0.190809912898503));
#100785=DIRECTION('center_axis',(0.981627005099017,0.,0.190809912898503));
#100786=DIRECTION('ref_axis',(0.,-1.,0.));
#100787=DIRECTION('',(-0.190809912898503,0.,0.981627005099017));
#100788=DIRECTION('',(0.,-1.,0.));
#100789=DIRECTION('',(0.,-1.,0.));
#100790=DIRECTION('center_axis',(0.,-1.,0.));
#100791=DIRECTION('ref_axis',(0.,0.,-1.));
#100792=DIRECTION('',(-0.190809912898503,0.,0.981627005099017));
#100793=DIRECTION('',(-0.981627005099017,0.,-0.190809912898503));
#100794=DIRECTION('',(-0.981627005099017,0.,-0.190809912898503));
#100795=DIRECTION('center_axis',(-0.981627005099017,0.,-0.190809912898503));
#100796=DIRECTION('ref_axis',(-0.190809912898503,0.,0.981627005099017));
#100797=DIRECTION('',(0.,1.,0.));
#100798=DIRECTION('',(0.,1.,0.));
#100799=DIRECTION('center_axis',(0.,1.,0.));
#100800=DIRECTION('ref_axis',(1.,0.,0.));
#100801=DIRECTION('',(-0.190809912898503,0.,0.981627005099017));
#100802=DIRECTION('',(0.981627005099017,0.,0.190809912898503));
#100803=DIRECTION('',(-0.190809912898503,0.,0.981627005099017));
#100804=DIRECTION('',(0.981627005099017,0.,0.190809912898503));
#100805=DIRECTION('center_axis',(0.981627005099017,0.,0.190809912898503));
#100806=DIRECTION('ref_axis',(0.,-1.,0.));
#100807=DIRECTION('',(-0.190809912898503,0.,0.981627005099017));
#100808=DIRECTION('',(0.,-1.,0.));
#100809=DIRECTION('',(0.,-1.,0.));
#100810=DIRECTION('center_axis',(0.,-1.,0.));
#100811=DIRECTION('ref_axis',(0.,0.,-1.));
#100812=DIRECTION('',(-0.190809912898503,0.,0.981627005099017));
#100813=DIRECTION('',(-0.981627005099017,0.,-0.190809912898503));
#100814=DIRECTION('',(-0.981627005099017,0.,-0.190809912898503));
#100815=DIRECTION('center_axis',(-0.981627005099017,0.,-0.190809912898503));
#100816=DIRECTION('ref_axis',(-0.190809912898503,0.,0.981627005099017));
#100817=DIRECTION('',(0.,1.,0.));
#100818=DIRECTION('',(0.,1.,0.));
#100819=DIRECTION('center_axis',(0.,1.,0.));
#100820=DIRECTION('ref_axis',(1.,0.,0.));
#100821=DIRECTION('',(-0.190809912898503,0.,0.981627005099017));
#100822=DIRECTION('',(0.981627005099017,0.,0.190809912898503));
#100823=DIRECTION('',(-0.190809912898503,0.,0.981627005099017));
#100824=DIRECTION('',(0.981627005099017,0.,0.190809912898503));
#100825=DIRECTION('center_axis',(0.981627005099017,0.,0.190809912898503));
#100826=DIRECTION('ref_axis',(0.,-1.,0.));
#100827=DIRECTION('',(-0.190809912898503,0.,0.981627005099017));
#100828=DIRECTION('',(0.,-1.,0.));
#100829=DIRECTION('',(0.,-1.,0.));
#100830=DIRECTION('center_axis',(0.,-1.,0.));
#100831=DIRECTION('ref_axis',(0.,0.,-1.));
#100832=DIRECTION('',(-0.190809912898503,0.,0.981627005099017));
#100833=DIRECTION('',(-0.981627005099017,0.,-0.190809912898503));
#100834=DIRECTION('',(-0.981627005099017,0.,-0.190809912898503));
#100835=DIRECTION('center_axis',(-0.981627005099017,0.,-0.190809912898503));
#100836=DIRECTION('ref_axis',(-0.190809912898503,0.,0.981627005099017));
#100837=DIRECTION('',(0.,1.,0.));
#100838=DIRECTION('',(0.,1.,0.));
#100839=DIRECTION('center_axis',(0.,1.,0.));
#100840=DIRECTION('ref_axis',(1.,0.,0.));
#100841=DIRECTION('',(-0.190809912898503,0.,0.981627005099017));
#100842=DIRECTION('',(0.981627005099017,0.,0.190809912898503));
#100843=DIRECTION('',(-0.190809912898503,0.,0.981627005099017));
#100844=DIRECTION('',(0.981627005099017,0.,0.190809912898503));
#100845=DIRECTION('center_axis',(0.981627005099017,0.,0.190809912898503));
#100846=DIRECTION('ref_axis',(0.,-1.,0.));
#100847=DIRECTION('',(-0.190809912898503,0.,0.981627005099017));
#100848=DIRECTION('',(0.,-1.,0.));
#100849=DIRECTION('',(0.,-1.,0.));
#100850=DIRECTION('center_axis',(0.,-1.,0.));
#100851=DIRECTION('ref_axis',(0.,0.,-1.));
#100852=DIRECTION('',(-0.190809912898503,0.,0.981627005099017));
#100853=DIRECTION('',(-0.981627005099017,0.,-0.190809912898503));
#100854=DIRECTION('',(-0.981627005099017,0.,-0.190809912898503));
#100855=DIRECTION('center_axis',(-0.981627005099017,0.,-0.190809912898503));
#100856=DIRECTION('ref_axis',(-0.190809912898503,0.,0.981627005099017));
#100857=DIRECTION('',(0.,1.,0.));
#100858=DIRECTION('',(0.,1.,0.));
#100859=DIRECTION('center_axis',(0.,1.,0.));
#100860=DIRECTION('ref_axis',(1.,0.,0.));
#100861=DIRECTION('',(-0.190809912898503,0.,0.981627005099017));
#100862=DIRECTION('',(0.981627005099017,0.,0.190809912898503));
#100863=DIRECTION('',(-0.190809912898503,0.,0.981627005099017));
#100864=DIRECTION('',(0.981627005099017,0.,0.190809912898503));
#100865=DIRECTION('center_axis',(0.981627005099017,0.,0.190809912898503));
#100866=DIRECTION('ref_axis',(0.,-1.,0.));
#100867=DIRECTION('',(-0.190809912898503,0.,0.981627005099017));
#100868=DIRECTION('',(0.,-1.,0.));
#100869=DIRECTION('',(0.,-1.,0.));
#100870=DIRECTION('center_axis',(0.,-1.,0.));
#100871=DIRECTION('ref_axis',(0.,0.,-1.));
#100872=DIRECTION('',(-0.190809912898503,0.,0.981627005099017));
#100873=DIRECTION('',(-0.981627005099017,0.,-0.190809912898503));
#100874=DIRECTION('',(-0.981627005099017,0.,-0.190809912898503));
#100875=DIRECTION('center_axis',(-0.981627005099017,0.,-0.190809912898503));
#100876=DIRECTION('ref_axis',(-0.190809912898503,0.,0.981627005099017));
#100877=DIRECTION('',(0.,1.,0.));
#100878=DIRECTION('',(0.,1.,0.));
#100879=DIRECTION('center_axis',(0.,1.,0.));
#100880=DIRECTION('ref_axis',(1.,0.,0.));
#100881=DIRECTION('',(-0.190809912898503,0.,0.981627005099017));
#100882=DIRECTION('',(0.981627005099017,0.,0.190809912898503));
#100883=DIRECTION('',(-0.190809912898503,0.,0.981627005099017));
#100884=DIRECTION('',(0.981627005099017,0.,0.190809912898503));
#100885=DIRECTION('center_axis',(0.981627005099017,0.,0.190809912898503));
#100886=DIRECTION('ref_axis',(0.,-1.,0.));
#100887=DIRECTION('',(-0.190809912898503,0.,0.981627005099017));
#100888=DIRECTION('',(0.,-1.,0.));
#100889=DIRECTION('',(0.,-1.,0.));
#100890=DIRECTION('center_axis',(0.,-1.,0.));
#100891=DIRECTION('ref_axis',(0.,0.,-1.));
#100892=DIRECTION('',(-0.190809912898503,0.,0.981627005099017));
#100893=DIRECTION('',(-0.981627005099017,0.,-0.190809912898503));
#100894=DIRECTION('',(-0.981627005099017,0.,-0.190809912898503));
#100895=DIRECTION('center_axis',(-0.981627005099017,0.,-0.190809912898503));
#100896=DIRECTION('ref_axis',(-0.190809912898503,0.,0.981627005099017));
#100897=DIRECTION('',(0.,1.,0.));
#100898=DIRECTION('',(0.,1.,0.));
#100899=DIRECTION('center_axis',(0.,1.,0.));
#100900=DIRECTION('ref_axis',(1.,0.,0.));
#100901=DIRECTION('',(-0.190809912898503,0.,0.981627005099017));
#100902=DIRECTION('',(0.981627005099017,0.,0.190809912898503));
#100903=DIRECTION('',(-0.190809912898503,0.,0.981627005099017));
#100904=DIRECTION('',(0.981627005099017,0.,0.190809912898503));
#100905=DIRECTION('center_axis',(0.981627005099017,0.,0.190809912898503));
#100906=DIRECTION('ref_axis',(0.,-1.,0.));
#100907=DIRECTION('',(-0.190809912898503,0.,0.981627005099017));
#100908=DIRECTION('',(0.,-1.,0.));
#100909=DIRECTION('',(0.,-1.,0.));
#100910=DIRECTION('center_axis',(0.,-1.,0.));
#100911=DIRECTION('ref_axis',(0.,0.,-1.));
#100912=DIRECTION('',(-0.190809912898503,0.,0.981627005099017));
#100913=DIRECTION('',(-0.981627005099017,0.,-0.190809912898503));
#100914=DIRECTION('',(-0.981627005099017,0.,-0.190809912898503));
#100915=DIRECTION('center_axis',(-0.981627005099017,0.,-0.190809912898503));
#100916=DIRECTION('ref_axis',(-0.190809912898503,0.,0.981627005099017));
#100917=DIRECTION('',(0.,1.,0.));
#100918=DIRECTION('',(0.,1.,0.));
#100919=DIRECTION('center_axis',(0.,1.,0.));
#100920=DIRECTION('ref_axis',(1.,0.,0.));
#100921=DIRECTION('',(-0.190809912898503,0.,0.981627005099017));
#100922=DIRECTION('',(0.981627005099017,0.,0.190809912898503));
#100923=DIRECTION('',(-0.190809912898503,0.,0.981627005099017));
#100924=DIRECTION('',(0.981627005099017,0.,0.190809912898503));
#100925=DIRECTION('center_axis',(0.981627005099017,0.,0.190809912898503));
#100926=DIRECTION('ref_axis',(0.,-1.,0.));
#100927=DIRECTION('',(-0.190809912898503,0.,0.981627005099017));
#100928=DIRECTION('',(0.,-1.,0.));
#100929=DIRECTION('',(0.,-1.,0.));
#100930=DIRECTION('center_axis',(0.,-1.,0.));
#100931=DIRECTION('ref_axis',(0.,0.,-1.));
#100932=DIRECTION('',(-0.190809912898503,0.,0.981627005099017));
#100933=DIRECTION('',(-0.981627005099017,0.,-0.190809912898503));
#100934=DIRECTION('',(-0.981627005099017,0.,-0.190809912898503));
#100935=DIRECTION('center_axis',(-0.981627005099017,0.,-0.190809912898503));
#100936=DIRECTION('ref_axis',(-0.190809912898503,0.,0.981627005099017));
#100937=DIRECTION('',(0.,1.,0.));
#100938=DIRECTION('',(0.,1.,0.));
#100939=DIRECTION('center_axis',(0.,1.,0.));
#100940=DIRECTION('ref_axis',(1.,0.,0.));
#100941=DIRECTION('',(-0.190809912898503,0.,0.981627005099017));
#100942=DIRECTION('',(0.981627005099017,0.,0.190809912898503));
#100943=DIRECTION('',(-0.190809912898503,0.,0.981627005099017));
#100944=DIRECTION('',(0.981627005099017,0.,0.190809912898503));
#100945=DIRECTION('center_axis',(0.981627005099017,0.,0.190809912898503));
#100946=DIRECTION('ref_axis',(0.,-1.,0.));
#100947=DIRECTION('',(-0.190809912898503,0.,0.981627005099017));
#100948=DIRECTION('',(0.,-1.,0.));
#100949=DIRECTION('',(0.,-1.,0.));
#100950=DIRECTION('center_axis',(0.,-1.,0.));
#100951=DIRECTION('ref_axis',(0.,0.,-1.));
#100952=DIRECTION('',(-0.190809912898503,0.,0.981627005099017));
#100953=DIRECTION('',(-0.981627005099017,0.,-0.190809912898503));
#100954=DIRECTION('',(-0.981627005099017,0.,-0.190809912898503));
#100955=DIRECTION('center_axis',(-0.981627005099017,0.,-0.190809912898503));
#100956=DIRECTION('ref_axis',(-0.190809912898503,0.,0.981627005099017));
#100957=DIRECTION('',(0.,1.,0.));
#100958=DIRECTION('',(0.,1.,0.));
#100959=DIRECTION('center_axis',(0.,1.,0.));
#100960=DIRECTION('ref_axis',(1.,0.,0.));
#100961=DIRECTION('',(-0.190809912898503,0.,0.981627005099017));
#100962=DIRECTION('',(0.981627005099017,0.,0.190809912898503));
#100963=DIRECTION('',(-0.190809912898503,0.,0.981627005099017));
#100964=DIRECTION('',(0.981627005099017,0.,0.190809912898503));
#100965=DIRECTION('center_axis',(0.981627005099017,0.,0.190809912898503));
#100966=DIRECTION('ref_axis',(0.,-1.,0.));
#100967=DIRECTION('',(-0.190809912898503,0.,0.981627005099017));
#100968=DIRECTION('',(0.,-1.,0.));
#100969=DIRECTION('',(0.,-1.,0.));
#100970=DIRECTION('center_axis',(0.,-1.,0.));
#100971=DIRECTION('ref_axis',(0.,0.,-1.));
#100972=DIRECTION('',(-0.190809912898503,0.,0.981627005099017));
#100973=DIRECTION('',(-0.981627005099017,0.,-0.190809912898503));
#100974=DIRECTION('',(-0.981627005099017,0.,-0.190809912898503));
#100975=DIRECTION('center_axis',(-0.981627005099017,0.,-0.190809912898503));
#100976=DIRECTION('ref_axis',(-0.190809912898503,0.,0.981627005099017));
#100977=DIRECTION('',(0.,1.,0.));
#100978=DIRECTION('',(0.,1.,0.));
#100979=DIRECTION('center_axis',(0.,1.,0.));
#100980=DIRECTION('ref_axis',(1.,0.,0.));
#100981=DIRECTION('',(-0.190809912898503,0.,0.981627005099017));
#100982=DIRECTION('',(0.981627005099017,0.,0.190809912898503));
#100983=DIRECTION('',(-0.190809912898503,0.,0.981627005099017));
#100984=DIRECTION('',(0.981627005099017,0.,0.190809912898503));
#100985=DIRECTION('center_axis',(0.981627005099017,0.,0.190809912898503));
#100986=DIRECTION('ref_axis',(0.,-1.,0.));
#100987=DIRECTION('',(-0.190809912898503,0.,0.981627005099017));
#100988=DIRECTION('',(0.,-1.,0.));
#100989=DIRECTION('',(0.,-1.,0.));
#100990=DIRECTION('center_axis',(0.,-1.,0.));
#100991=DIRECTION('ref_axis',(0.,0.,-1.));
#100992=DIRECTION('',(-0.190809912898503,0.,0.981627005099017));
#100993=DIRECTION('',(-0.981627005099017,0.,-0.190809912898503));
#100994=DIRECTION('',(-0.981627005099017,0.,-0.190809912898503));
#100995=DIRECTION('center_axis',(-0.981627005099017,0.,-0.190809912898503));
#100996=DIRECTION('ref_axis',(-0.190809912898503,0.,0.981627005099017));
#100997=DIRECTION('',(0.,1.,0.));
#100998=DIRECTION('',(0.,1.,0.));
#100999=DIRECTION('center_axis',(0.,1.,0.));
#101000=DIRECTION('ref_axis',(1.,0.,0.));
#101001=DIRECTION('',(-0.190809912898503,0.,0.981627005099017));
#101002=DIRECTION('',(0.981627005099017,0.,0.190809912898503));
#101003=DIRECTION('',(-0.190809912898503,0.,0.981627005099017));
#101004=DIRECTION('',(0.981627005099017,0.,0.190809912898503));
#101005=DIRECTION('center_axis',(0.981627005099017,0.,0.190809912898503));
#101006=DIRECTION('ref_axis',(0.,-1.,0.));
#101007=DIRECTION('',(-0.190809912898503,0.,0.981627005099017));
#101008=DIRECTION('',(0.,-1.,0.));
#101009=DIRECTION('',(0.,-1.,0.));
#101010=DIRECTION('center_axis',(0.,-1.,0.));
#101011=DIRECTION('ref_axis',(0.,0.,-1.));
#101012=DIRECTION('',(-0.190809912898503,0.,0.981627005099017));
#101013=DIRECTION('',(-0.981627005099017,0.,-0.190809912898503));
#101014=DIRECTION('',(-0.981627005099017,0.,-0.190809912898503));
#101015=DIRECTION('center_axis',(-0.981627005099017,0.,-0.190809912898503));
#101016=DIRECTION('ref_axis',(-0.190809912898503,0.,0.981627005099017));
#101017=DIRECTION('',(0.,1.,0.));
#101018=DIRECTION('',(0.,1.,0.));
#101019=DIRECTION('center_axis',(0.,1.,0.));
#101020=DIRECTION('ref_axis',(1.,0.,0.));
#101021=DIRECTION('',(-0.190809912898503,0.,0.981627005099017));
#101022=DIRECTION('',(0.981627005099017,0.,0.190809912898503));
#101023=DIRECTION('',(-0.190809912898503,0.,0.981627005099017));
#101024=DIRECTION('',(0.981627005099017,0.,0.190809912898503));
#101025=DIRECTION('center_axis',(0.981627005099017,0.,0.190809912898503));
#101026=DIRECTION('ref_axis',(0.,-1.,0.));
#101027=DIRECTION('',(-0.190809912898503,0.,0.981627005099017));
#101028=DIRECTION('',(0.,-1.,0.));
#101029=DIRECTION('',(0.,-1.,0.));
#101030=DIRECTION('center_axis',(0.,-1.,0.));
#101031=DIRECTION('ref_axis',(0.,0.,-1.));
#101032=DIRECTION('',(-0.190809912898503,0.,0.981627005099017));
#101033=DIRECTION('',(-0.981627005099017,0.,-0.190809912898503));
#101034=DIRECTION('',(-0.981627005099017,0.,-0.190809912898503));
#101035=DIRECTION('center_axis',(-0.981627005099017,0.,-0.190809912898503));
#101036=DIRECTION('ref_axis',(-0.190809912898503,0.,0.981627005099017));
#101037=DIRECTION('',(0.,1.,0.));
#101038=DIRECTION('',(0.,1.,0.));
#101039=DIRECTION('center_axis',(0.,1.,0.));
#101040=DIRECTION('ref_axis',(1.,0.,0.));
#101041=DIRECTION('',(-0.190809912898503,0.,0.981627005099017));
#101042=DIRECTION('',(0.981627005099017,0.,0.190809912898503));
#101043=DIRECTION('',(-0.190809912898503,0.,0.981627005099017));
#101044=DIRECTION('',(0.981627005099017,0.,0.190809912898503));
#101045=DIRECTION('center_axis',(0.981627005099017,0.,0.190809912898503));
#101046=DIRECTION('ref_axis',(0.,-1.,0.));
#101047=DIRECTION('',(-0.190809912898503,0.,0.981627005099017));
#101048=DIRECTION('',(0.,-1.,0.));
#101049=DIRECTION('',(0.,-1.,0.));
#101050=DIRECTION('center_axis',(0.,-1.,0.));
#101051=DIRECTION('ref_axis',(0.,0.,-1.));
#101052=DIRECTION('',(-0.190809912898503,0.,0.981627005099017));
#101053=DIRECTION('',(-0.981627005099017,0.,-0.190809912898503));
#101054=DIRECTION('',(-0.981627005099017,0.,-0.190809912898503));
#101055=DIRECTION('center_axis',(-0.981627005099017,0.,-0.190809912898503));
#101056=DIRECTION('ref_axis',(-0.190809912898503,0.,0.981627005099017));
#101057=DIRECTION('',(0.,1.,0.));
#101058=DIRECTION('',(0.,1.,0.));
#101059=DIRECTION('center_axis',(0.,1.,0.));
#101060=DIRECTION('ref_axis',(1.,0.,0.));
#101061=DIRECTION('',(-0.190809912898503,0.,0.981627005099017));
#101062=DIRECTION('',(0.981627005099017,0.,0.190809912898503));
#101063=DIRECTION('',(-0.190809912898503,0.,0.981627005099017));
#101064=DIRECTION('',(0.981627005099017,0.,0.190809912898503));
#101065=DIRECTION('center_axis',(0.981627005099017,0.,0.190809912898503));
#101066=DIRECTION('ref_axis',(0.,-1.,0.));
#101067=DIRECTION('',(-0.190809912898503,0.,0.981627005099017));
#101068=DIRECTION('',(0.,-1.,0.));
#101069=DIRECTION('',(0.,-1.,0.));
#101070=DIRECTION('center_axis',(0.,-1.,0.));
#101071=DIRECTION('ref_axis',(0.,0.,-1.));
#101072=DIRECTION('',(-0.190809912898503,0.,0.981627005099017));
#101073=DIRECTION('',(-0.981627005099017,0.,-0.190809912898503));
#101074=DIRECTION('',(-0.981627005099017,0.,-0.190809912898503));
#101075=DIRECTION('center_axis',(-0.981627005099017,0.,-0.190809912898503));
#101076=DIRECTION('ref_axis',(-0.190809912898503,0.,0.981627005099017));
#101077=DIRECTION('',(0.,1.,0.));
#101078=DIRECTION('',(0.,1.,0.));
#101079=DIRECTION('center_axis',(0.,1.,0.));
#101080=DIRECTION('ref_axis',(1.,0.,0.));
#101081=DIRECTION('',(-0.190809912898503,0.,0.981627005099017));
#101082=DIRECTION('',(0.981627005099017,0.,0.190809912898503));
#101083=DIRECTION('',(-0.190809912898503,0.,0.981627005099017));
#101084=DIRECTION('',(0.981627005099017,0.,0.190809912898503));
#101085=DIRECTION('center_axis',(0.981627005099017,0.,0.190809912898503));
#101086=DIRECTION('ref_axis',(0.,-1.,0.));
#101087=DIRECTION('',(-0.190809912898503,0.,0.981627005099017));
#101088=DIRECTION('',(0.,-1.,0.));
#101089=DIRECTION('',(0.,-1.,0.));
#101090=DIRECTION('center_axis',(0.,-1.,0.));
#101091=DIRECTION('ref_axis',(0.,0.,-1.));
#101092=DIRECTION('',(-0.190809912898503,0.,0.981627005099017));
#101093=DIRECTION('',(-0.981627005099017,0.,-0.190809912898503));
#101094=DIRECTION('',(-0.981627005099017,0.,-0.190809912898503));
#101095=DIRECTION('center_axis',(-0.981627005099017,0.,-0.190809912898503));
#101096=DIRECTION('ref_axis',(-0.190809912898503,0.,0.981627005099017));
#101097=DIRECTION('',(0.,1.,0.));
#101098=DIRECTION('',(0.,1.,0.));
#101099=DIRECTION('center_axis',(0.,1.,0.));
#101100=DIRECTION('ref_axis',(1.,0.,0.));
#101101=DIRECTION('',(-0.190809912898503,0.,0.981627005099017));
#101102=DIRECTION('',(0.981627005099017,0.,0.190809912898503));
#101103=DIRECTION('',(-0.190809912898503,0.,0.981627005099017));
#101104=DIRECTION('',(0.981627005099017,0.,0.190809912898503));
#101105=DIRECTION('center_axis',(0.981627005099017,0.,0.190809912898503));
#101106=DIRECTION('ref_axis',(0.,-1.,0.));
#101107=DIRECTION('',(-0.190809912898503,0.,0.981627005099017));
#101108=DIRECTION('',(0.,-1.,0.));
#101109=DIRECTION('',(0.,-1.,0.));
#101110=DIRECTION('center_axis',(0.,-1.,0.));
#101111=DIRECTION('ref_axis',(0.,0.,-1.));
#101112=DIRECTION('',(-0.190809912898503,0.,0.981627005099017));
#101113=DIRECTION('',(-0.981627005099017,0.,-0.190809912898503));
#101114=DIRECTION('',(-0.981627005099017,0.,-0.190809912898503));
#101115=DIRECTION('center_axis',(-0.981627005099017,0.,-0.190809912898503));
#101116=DIRECTION('ref_axis',(-0.190809912898503,0.,0.981627005099017));
#101117=DIRECTION('',(0.,1.,0.));
#101118=DIRECTION('',(0.,1.,0.));
#101119=DIRECTION('center_axis',(0.,1.,0.));
#101120=DIRECTION('ref_axis',(1.,0.,0.));
#101121=DIRECTION('',(-0.190809912898503,0.,0.981627005099017));
#101122=DIRECTION('',(0.981627005099017,0.,0.190809912898503));
#101123=DIRECTION('',(-0.190809912898503,0.,0.981627005099017));
#101124=DIRECTION('',(0.981627005099017,0.,0.190809912898503));
#101125=DIRECTION('center_axis',(0.981627005099017,0.,0.190809912898503));
#101126=DIRECTION('ref_axis',(0.,-1.,0.));
#101127=DIRECTION('',(-0.190809912898503,0.,0.981627005099017));
#101128=DIRECTION('',(0.,-1.,0.));
#101129=DIRECTION('',(0.,-1.,0.));
#101130=DIRECTION('center_axis',(0.,-1.,0.));
#101131=DIRECTION('ref_axis',(0.,0.,-1.));
#101132=DIRECTION('',(-0.190809912898503,0.,0.981627005099017));
#101133=DIRECTION('',(-0.981627005099017,0.,-0.190809912898503));
#101134=DIRECTION('',(-0.981627005099017,0.,-0.190809912898503));
#101135=DIRECTION('center_axis',(-0.981627005099017,0.,-0.190809912898503));
#101136=DIRECTION('ref_axis',(-0.190809912898503,0.,0.981627005099017));
#101137=DIRECTION('',(0.,1.,0.));
#101138=DIRECTION('',(0.,1.,0.));
#101139=DIRECTION('center_axis',(0.,1.,0.));
#101140=DIRECTION('ref_axis',(1.,0.,0.));
#101141=DIRECTION('',(-0.190809912898503,0.,0.981627005099017));
#101142=DIRECTION('',(0.981627005099017,0.,0.190809912898503));
#101143=DIRECTION('',(-0.190809912898503,0.,0.981627005099017));
#101144=DIRECTION('',(0.981627005099017,0.,0.190809912898503));
#101145=DIRECTION('center_axis',(0.981627005099017,0.,0.190809912898503));
#101146=DIRECTION('ref_axis',(0.,-1.,0.));
#101147=DIRECTION('',(-0.190809912898503,0.,0.981627005099017));
#101148=DIRECTION('',(0.,-1.,0.));
#101149=DIRECTION('',(0.,-1.,0.));
#101150=DIRECTION('center_axis',(0.,-1.,0.));
#101151=DIRECTION('ref_axis',(0.,0.,-1.));
#101152=DIRECTION('',(-0.190809912898503,0.,0.981627005099017));
#101153=DIRECTION('',(-0.981627005099017,0.,-0.190809912898503));
#101154=DIRECTION('',(-0.981627005099017,0.,-0.190809912898503));
#101155=DIRECTION('center_axis',(-0.981627005099017,0.,-0.190809912898503));
#101156=DIRECTION('ref_axis',(-0.190809912898503,0.,0.981627005099017));
#101157=DIRECTION('',(0.,1.,0.));
#101158=DIRECTION('',(0.,1.,0.));
#101159=DIRECTION('center_axis',(0.,1.,0.));
#101160=DIRECTION('ref_axis',(1.,0.,0.));
#101161=DIRECTION('',(-0.190809912898503,0.,0.981627005099017));
#101162=DIRECTION('',(0.981627005099017,0.,0.190809912898503));
#101163=DIRECTION('',(-0.190809912898503,0.,0.981627005099017));
#101164=DIRECTION('',(0.981627005099017,0.,0.190809912898503));
#101165=DIRECTION('center_axis',(0.981627005099017,0.,0.190809912898503));
#101166=DIRECTION('ref_axis',(0.,-1.,0.));
#101167=DIRECTION('',(-0.190809912898503,0.,0.981627005099017));
#101168=DIRECTION('',(0.,-1.,0.));
#101169=DIRECTION('',(0.,-1.,0.));
#101170=DIRECTION('center_axis',(0.,-1.,0.));
#101171=DIRECTION('ref_axis',(0.,0.,-1.));
#101172=DIRECTION('',(-0.190809912898503,0.,0.981627005099017));
#101173=DIRECTION('',(-0.981627005099017,0.,-0.190809912898503));
#101174=DIRECTION('',(-0.981627005099017,0.,-0.190809912898503));
#101175=DIRECTION('center_axis',(-0.981627005099017,0.,-0.190809912898503));
#101176=DIRECTION('ref_axis',(-0.190809912898503,0.,0.981627005099017));
#101177=DIRECTION('',(0.,1.,0.));
#101178=DIRECTION('',(0.,1.,0.));
#101179=DIRECTION('center_axis',(0.,1.,0.));
#101180=DIRECTION('ref_axis',(1.,0.,0.));
#101181=DIRECTION('',(-0.190809912898503,0.,0.981627005099017));
#101182=DIRECTION('',(0.981627005099017,0.,0.190809912898503));
#101183=DIRECTION('',(-0.190809912898503,0.,0.981627005099017));
#101184=DIRECTION('',(0.981627005099017,0.,0.190809912898503));
#101185=DIRECTION('center_axis',(0.981627005099017,0.,0.190809912898503));
#101186=DIRECTION('ref_axis',(0.,-1.,0.));
#101187=DIRECTION('',(-0.190809912898503,0.,0.981627005099017));
#101188=DIRECTION('',(0.,-1.,0.));
#101189=DIRECTION('',(0.,-1.,0.));
#101190=DIRECTION('center_axis',(0.,-1.,0.));
#101191=DIRECTION('ref_axis',(0.,0.,-1.));
#101192=DIRECTION('',(-0.190809912898503,0.,0.981627005099017));
#101193=DIRECTION('',(-0.981627005099017,0.,-0.190809912898503));
#101194=DIRECTION('',(-0.981627005099017,0.,-0.190809912898503));
#101195=DIRECTION('center_axis',(-0.981627005099017,0.,-0.190809912898503));
#101196=DIRECTION('ref_axis',(-0.190809912898503,0.,0.981627005099017));
#101197=DIRECTION('',(0.,1.,0.));
#101198=DIRECTION('',(0.,1.,0.));
#101199=DIRECTION('center_axis',(0.,1.,0.));
#101200=DIRECTION('ref_axis',(1.,0.,0.));
#101201=DIRECTION('',(-0.190809912898503,0.,0.981627005099017));
#101202=DIRECTION('',(0.981627005099017,0.,0.190809912898503));
#101203=DIRECTION('',(-0.190809912898503,0.,0.981627005099017));
#101204=DIRECTION('',(0.981627005099017,0.,0.190809912898503));
#101205=DIRECTION('center_axis',(0.981627005099017,0.,0.190809912898503));
#101206=DIRECTION('ref_axis',(0.,-1.,0.));
#101207=DIRECTION('',(-0.190809912898503,0.,0.981627005099017));
#101208=DIRECTION('',(0.,-1.,0.));
#101209=DIRECTION('',(0.,-1.,0.));
#101210=DIRECTION('center_axis',(0.,-1.,0.));
#101211=DIRECTION('ref_axis',(0.,0.,-1.));
#101212=DIRECTION('',(-0.190809912898503,0.,0.981627005099017));
#101213=DIRECTION('',(-0.981627005099017,0.,-0.190809912898503));
#101214=DIRECTION('',(-0.981627005099017,0.,-0.190809912898503));
#101215=DIRECTION('center_axis',(-0.981627005099017,0.,-0.190809912898503));
#101216=DIRECTION('ref_axis',(-0.190809912898503,0.,0.981627005099017));
#101217=DIRECTION('',(0.,1.,0.));
#101218=DIRECTION('',(0.,1.,0.));
#101219=DIRECTION('center_axis',(0.,1.,0.));
#101220=DIRECTION('ref_axis',(1.,0.,0.));
#101221=DIRECTION('',(-0.190809912898503,0.,0.981627005099017));
#101222=DIRECTION('',(0.981627005099017,0.,0.190809912898503));
#101223=DIRECTION('',(-0.190809912898503,0.,0.981627005099017));
#101224=DIRECTION('',(0.981627005099017,0.,0.190809912898503));
#101225=DIRECTION('center_axis',(0.981627005099017,0.,0.190809912898503));
#101226=DIRECTION('ref_axis',(0.,-1.,0.));
#101227=DIRECTION('',(-0.190809912898503,0.,0.981627005099017));
#101228=DIRECTION('',(0.,-1.,0.));
#101229=DIRECTION('',(0.,-1.,0.));
#101230=DIRECTION('center_axis',(0.,-1.,0.));
#101231=DIRECTION('ref_axis',(0.,0.,-1.));
#101232=DIRECTION('',(-0.190809912898503,0.,0.981627005099017));
#101233=DIRECTION('',(-0.981627005099017,0.,-0.190809912898503));
#101234=DIRECTION('',(-0.981627005099017,0.,-0.190809912898503));
#101235=DIRECTION('center_axis',(-0.981627005099017,0.,-0.190809912898503));
#101236=DIRECTION('ref_axis',(-0.190809912898503,0.,0.981627005099017));
#101237=DIRECTION('',(0.,1.,0.));
#101238=DIRECTION('',(0.,1.,0.));
#101239=DIRECTION('center_axis',(0.,1.,0.));
#101240=DIRECTION('ref_axis',(1.,0.,0.));
#101241=DIRECTION('',(-0.190809912898503,0.,0.981627005099017));
#101242=DIRECTION('',(0.981627005099017,0.,0.190809912898503));
#101243=DIRECTION('',(-0.190809912898503,0.,0.981627005099017));
#101244=DIRECTION('',(0.981627005099017,0.,0.190809912898503));
#101245=DIRECTION('center_axis',(0.981627005099017,0.,0.190809912898503));
#101246=DIRECTION('ref_axis',(0.,-1.,0.));
#101247=DIRECTION('',(-0.190809912898503,0.,0.981627005099017));
#101248=DIRECTION('',(0.,-1.,0.));
#101249=DIRECTION('',(0.,-1.,0.));
#101250=DIRECTION('center_axis',(0.,-1.,0.));
#101251=DIRECTION('ref_axis',(0.,0.,-1.));
#101252=DIRECTION('',(-0.190809912898503,0.,0.981627005099017));
#101253=DIRECTION('',(-0.981627005099017,0.,-0.190809912898503));
#101254=DIRECTION('',(-0.981627005099017,0.,-0.190809912898503));
#101255=DIRECTION('center_axis',(-0.981627005099017,0.,-0.190809912898503));
#101256=DIRECTION('ref_axis',(-0.190809912898503,0.,0.981627005099017));
#101257=DIRECTION('',(0.,1.,0.));
#101258=DIRECTION('',(0.,1.,0.));
#101259=DIRECTION('center_axis',(0.,1.,0.));
#101260=DIRECTION('ref_axis',(1.,0.,0.));
#101261=DIRECTION('',(-0.190809912898503,0.,0.981627005099017));
#101262=DIRECTION('',(0.981627005099017,0.,0.190809912898503));
#101263=DIRECTION('',(-0.190809912898503,0.,0.981627005099017));
#101264=DIRECTION('',(0.981627005099017,0.,0.190809912898503));
#101265=DIRECTION('center_axis',(0.981627005099017,0.,0.190809912898503));
#101266=DIRECTION('ref_axis',(0.,-1.,0.));
#101267=DIRECTION('',(-0.190809912898503,0.,0.981627005099017));
#101268=DIRECTION('',(0.,-1.,0.));
#101269=DIRECTION('',(0.,-1.,0.));
#101270=DIRECTION('center_axis',(0.,-1.,0.));
#101271=DIRECTION('ref_axis',(0.,0.,-1.));
#101272=DIRECTION('',(-0.190809912898503,0.,0.981627005099017));
#101273=DIRECTION('',(-0.981627005099017,0.,-0.190809912898503));
#101274=DIRECTION('',(-0.981627005099017,0.,-0.190809912898503));
#101275=DIRECTION('center_axis',(-0.981627005099017,0.,-0.190809912898503));
#101276=DIRECTION('ref_axis',(-0.190809912898503,0.,0.981627005099017));
#101277=DIRECTION('',(0.,1.,0.));
#101278=DIRECTION('',(0.,1.,0.));
#101279=DIRECTION('center_axis',(0.,1.,0.));
#101280=DIRECTION('ref_axis',(1.,0.,0.));
#101281=DIRECTION('',(-0.190809912898503,0.,0.981627005099017));
#101282=DIRECTION('',(0.981627005099017,0.,0.190809912898503));
#101283=DIRECTION('',(-0.190809912898503,0.,0.981627005099017));
#101284=DIRECTION('',(0.981627005099017,0.,0.190809912898503));
#101285=DIRECTION('center_axis',(0.981627005099017,0.,0.190809912898503));
#101286=DIRECTION('ref_axis',(0.,-1.,0.));
#101287=DIRECTION('',(-0.190809912898503,0.,0.981627005099017));
#101288=DIRECTION('',(0.,-1.,0.));
#101289=DIRECTION('',(0.,-1.,0.));
#101290=DIRECTION('center_axis',(0.,-1.,0.));
#101291=DIRECTION('ref_axis',(0.,0.,-1.));
#101292=DIRECTION('',(-0.190809912898503,0.,0.981627005099017));
#101293=DIRECTION('',(-0.981627005099017,0.,-0.190809912898503));
#101294=DIRECTION('',(-0.981627005099017,0.,-0.190809912898503));
#101295=DIRECTION('center_axis',(-0.981627005099017,0.,-0.190809912898503));
#101296=DIRECTION('ref_axis',(-0.190809912898503,0.,0.981627005099017));
#101297=DIRECTION('',(0.,1.,0.));
#101298=DIRECTION('',(0.,1.,0.));
#101299=DIRECTION('center_axis',(0.,1.,0.));
#101300=DIRECTION('ref_axis',(1.,0.,0.));
#101301=DIRECTION('',(-0.190809912898503,0.,0.981627005099017));
#101302=DIRECTION('',(0.981627005099017,0.,0.190809912898503));
#101303=DIRECTION('',(-0.190809912898503,0.,0.981627005099017));
#101304=DIRECTION('',(0.981627005099017,0.,0.190809912898503));
#101305=DIRECTION('center_axis',(0.981627005099017,0.,0.190809912898503));
#101306=DIRECTION('ref_axis',(0.,-1.,0.));
#101307=DIRECTION('',(-0.190809912898503,0.,0.981627005099017));
#101308=DIRECTION('',(0.,-1.,0.));
#101309=DIRECTION('',(0.,-1.,0.));
#101310=DIRECTION('center_axis',(0.,-1.,0.));
#101311=DIRECTION('ref_axis',(0.,0.,-1.));
#101312=DIRECTION('',(-0.190809912898503,0.,0.981627005099017));
#101313=DIRECTION('',(-0.981627005099017,0.,-0.190809912898503));
#101314=DIRECTION('',(-0.981627005099017,0.,-0.190809912898503));
#101315=DIRECTION('center_axis',(-0.981627005099017,0.,-0.190809912898503));
#101316=DIRECTION('ref_axis',(-0.190809912898503,0.,0.981627005099017));
#101317=DIRECTION('',(0.,1.,0.));
#101318=DIRECTION('',(0.,1.,0.));
#101319=DIRECTION('center_axis',(0.,1.,0.));
#101320=DIRECTION('ref_axis',(1.,0.,0.));
#101321=DIRECTION('',(-0.190809912898503,0.,0.981627005099017));
#101322=DIRECTION('',(0.981627005099017,0.,0.190809912898503));
#101323=DIRECTION('',(-0.190809912898503,0.,0.981627005099017));
#101324=DIRECTION('',(0.981627005099017,0.,0.190809912898503));
#101325=DIRECTION('center_axis',(0.981627005099017,0.,0.190809912898503));
#101326=DIRECTION('ref_axis',(0.,-1.,0.));
#101327=DIRECTION('',(-0.190809912898503,0.,0.981627005099017));
#101328=DIRECTION('',(0.,-1.,0.));
#101329=DIRECTION('',(0.,-1.,0.));
#101330=DIRECTION('center_axis',(0.,-1.,0.));
#101331=DIRECTION('ref_axis',(0.,0.,-1.));
#101332=DIRECTION('',(-0.190809912898503,0.,0.981627005099017));
#101333=DIRECTION('',(-0.981627005099017,0.,-0.190809912898503));
#101334=DIRECTION('',(-0.981627005099017,0.,-0.190809912898503));
#101335=DIRECTION('center_axis',(-0.981627005099017,0.,-0.190809912898503));
#101336=DIRECTION('ref_axis',(-0.190809912898503,0.,0.981627005099017));
#101337=DIRECTION('',(0.,1.,0.));
#101338=DIRECTION('',(0.,1.,0.));
#101339=DIRECTION('center_axis',(0.,1.,0.));
#101340=DIRECTION('ref_axis',(1.,0.,0.));
#101341=DIRECTION('',(-0.190809912898503,0.,0.981627005099017));
#101342=DIRECTION('',(0.981627005099017,0.,0.190809912898503));
#101343=DIRECTION('',(-0.190809912898503,0.,0.981627005099017));
#101344=DIRECTION('',(0.981627005099017,0.,0.190809912898503));
#101345=DIRECTION('center_axis',(0.981627005099017,0.,0.190809912898503));
#101346=DIRECTION('ref_axis',(0.,-1.,0.));
#101347=DIRECTION('',(-0.190809912898503,0.,0.981627005099017));
#101348=DIRECTION('',(0.,-1.,0.));
#101349=DIRECTION('',(0.,-1.,0.));
#101350=DIRECTION('center_axis',(0.,-1.,0.));
#101351=DIRECTION('ref_axis',(0.,0.,-1.));
#101352=DIRECTION('',(-0.190809912898503,0.,0.981627005099017));
#101353=DIRECTION('',(-0.981627005099017,0.,-0.190809912898503));
#101354=DIRECTION('',(-0.981627005099017,0.,-0.190809912898503));
#101355=DIRECTION('center_axis',(-0.981627005099017,0.,-0.190809912898503));
#101356=DIRECTION('ref_axis',(-0.190809912898503,0.,0.981627005099017));
#101357=DIRECTION('',(0.,1.,0.));
#101358=DIRECTION('',(0.,1.,0.));
#101359=DIRECTION('center_axis',(0.,1.,0.));
#101360=DIRECTION('ref_axis',(1.,0.,0.));
#101361=DIRECTION('',(-0.190809912898503,0.,0.981627005099017));
#101362=DIRECTION('',(0.981627005099017,0.,0.190809912898503));
#101363=DIRECTION('',(-0.190809912898503,0.,0.981627005099017));
#101364=DIRECTION('',(0.981627005099017,0.,0.190809912898503));
#101365=DIRECTION('center_axis',(0.981627005099017,0.,0.190809912898503));
#101366=DIRECTION('ref_axis',(0.,-1.,0.));
#101367=DIRECTION('',(-0.190809912898503,0.,0.981627005099017));
#101368=DIRECTION('',(0.,-1.,0.));
#101369=DIRECTION('',(0.,-1.,0.));
#101370=DIRECTION('center_axis',(0.,-1.,0.));
#101371=DIRECTION('ref_axis',(0.,0.,-1.));
#101372=DIRECTION('',(-0.190809912898503,0.,0.981627005099017));
#101373=DIRECTION('',(-0.981627005099017,0.,-0.190809912898503));
#101374=DIRECTION('',(-0.981627005099017,0.,-0.190809912898503));
#101375=DIRECTION('center_axis',(-0.981627005099017,0.,-0.190809912898503));
#101376=DIRECTION('ref_axis',(-0.190809912898503,0.,0.981627005099017));
#101377=DIRECTION('',(0.,1.,0.));
#101378=DIRECTION('',(0.,1.,0.));
#101379=DIRECTION('center_axis',(0.,1.,0.));
#101380=DIRECTION('ref_axis',(1.,0.,0.));
#101381=DIRECTION('',(-0.190809912898503,0.,0.981627005099017));
#101382=DIRECTION('',(0.981627005099017,0.,0.190809912898503));
#101383=DIRECTION('',(-0.190809912898503,0.,0.981627005099017));
#101384=DIRECTION('',(0.981627005099017,0.,0.190809912898503));
#101385=DIRECTION('center_axis',(0.981627005099017,0.,0.190809912898503));
#101386=DIRECTION('ref_axis',(0.,-1.,0.));
#101387=DIRECTION('',(-0.190809912898503,0.,0.981627005099017));
#101388=DIRECTION('',(0.,-1.,0.));
#101389=DIRECTION('',(0.,-1.,0.));
#101390=DIRECTION('center_axis',(0.,-1.,0.));
#101391=DIRECTION('ref_axis',(0.,0.,-1.));
#101392=DIRECTION('',(-0.190809912898503,0.,0.981627005099017));
#101393=DIRECTION('',(-0.981627005099017,0.,-0.190809912898503));
#101394=DIRECTION('',(-0.981627005099017,0.,-0.190809912898503));
#101395=DIRECTION('center_axis',(-0.981627005099017,0.,-0.190809912898503));
#101396=DIRECTION('ref_axis',(-0.190809912898503,0.,0.981627005099017));
#101397=DIRECTION('',(0.,1.,0.));
#101398=DIRECTION('',(0.,1.,0.));
#101399=DIRECTION('center_axis',(0.,1.,0.));
#101400=DIRECTION('ref_axis',(1.,0.,0.));
#101401=DIRECTION('',(-0.190809912898503,0.,0.981627005099017));
#101402=DIRECTION('',(0.981627005099017,0.,0.190809912898503));
#101403=DIRECTION('',(-0.190809912898503,0.,0.981627005099017));
#101404=DIRECTION('',(0.981627005099017,0.,0.190809912898503));
#101405=DIRECTION('center_axis',(0.981627005099017,0.,0.190809912898503));
#101406=DIRECTION('ref_axis',(0.,-1.,0.));
#101407=DIRECTION('',(-0.190809912898503,0.,0.981627005099017));
#101408=DIRECTION('',(0.,-1.,0.));
#101409=DIRECTION('',(0.,-1.,0.));
#101410=DIRECTION('center_axis',(0.,-1.,0.));
#101411=DIRECTION('ref_axis',(0.,0.,-1.));
#101412=DIRECTION('',(-0.190809912898503,0.,0.981627005099017));
#101413=DIRECTION('',(-0.981627005099017,0.,-0.190809912898503));
#101414=DIRECTION('',(-0.981627005099017,0.,-0.190809912898503));
#101415=DIRECTION('center_axis',(-0.981627005099017,0.,-0.190809912898503));
#101416=DIRECTION('ref_axis',(-0.190809912898503,0.,0.981627005099017));
#101417=DIRECTION('',(0.,1.,0.));
#101418=DIRECTION('',(0.,1.,0.));
#101419=DIRECTION('center_axis',(0.,1.,0.));
#101420=DIRECTION('ref_axis',(1.,0.,0.));
#101421=DIRECTION('',(-0.190809912898503,0.,0.981627005099017));
#101422=DIRECTION('',(0.981627005099017,0.,0.190809912898503));
#101423=DIRECTION('',(-0.190809912898503,0.,0.981627005099017));
#101424=DIRECTION('',(0.981627005099017,0.,0.190809912898503));
#101425=DIRECTION('center_axis',(0.981627005099017,0.,0.190809912898503));
#101426=DIRECTION('ref_axis',(0.,-1.,0.));
#101427=DIRECTION('',(-0.190809912898503,0.,0.981627005099017));
#101428=DIRECTION('',(0.,-1.,0.));
#101429=DIRECTION('',(0.,-1.,0.));
#101430=DIRECTION('center_axis',(0.,-1.,0.));
#101431=DIRECTION('ref_axis',(0.,0.,-1.));
#101432=DIRECTION('',(-0.190809912898503,0.,0.981627005099017));
#101433=DIRECTION('',(-0.981627005099017,0.,-0.190809912898503));
#101434=DIRECTION('',(-0.981627005099017,0.,-0.190809912898503));
#101435=DIRECTION('center_axis',(-0.981627005099017,0.,-0.190809912898503));
#101436=DIRECTION('ref_axis',(-0.190809912898503,0.,0.981627005099017));
#101437=DIRECTION('',(0.,1.,0.));
#101438=DIRECTION('',(0.,1.,0.));
#101439=DIRECTION('center_axis',(0.,1.,0.));
#101440=DIRECTION('ref_axis',(1.,0.,0.));
#101441=DIRECTION('',(-0.190809912898503,0.,0.981627005099017));
#101442=DIRECTION('',(0.981627005099017,0.,0.190809912898503));
#101443=DIRECTION('',(-0.190809912898503,0.,0.981627005099017));
#101444=DIRECTION('',(0.981627005099017,0.,0.190809912898503));
#101445=DIRECTION('center_axis',(0.981627005099017,0.,0.190809912898503));
#101446=DIRECTION('ref_axis',(0.,-1.,0.));
#101447=DIRECTION('',(-0.190809912898503,0.,0.981627005099017));
#101448=DIRECTION('',(0.,-1.,0.));
#101449=DIRECTION('',(0.,-1.,0.));
#101450=DIRECTION('center_axis',(0.,-1.,0.));
#101451=DIRECTION('ref_axis',(0.,0.,-1.));
#101452=DIRECTION('',(-0.190809912898503,0.,0.981627005099017));
#101453=DIRECTION('',(-0.981627005099017,0.,-0.190809912898503));
#101454=DIRECTION('',(-0.981627005099017,0.,-0.190809912898503));
#101455=DIRECTION('center_axis',(-0.981627005099017,0.,-0.190809912898503));
#101456=DIRECTION('ref_axis',(-0.190809912898503,0.,0.981627005099017));
#101457=DIRECTION('',(0.,1.,0.));
#101458=DIRECTION('',(0.,1.,0.));
#101459=DIRECTION('center_axis',(0.,1.,0.));
#101460=DIRECTION('ref_axis',(1.,0.,0.));
#101461=DIRECTION('',(-0.190809912898503,0.,0.981627005099017));
#101462=DIRECTION('',(0.981627005099017,0.,0.190809912898503));
#101463=DIRECTION('',(-0.190809912898503,0.,0.981627005099017));
#101464=DIRECTION('',(0.981627005099017,0.,0.190809912898503));
#101465=DIRECTION('center_axis',(0.981627005099017,0.,0.190809912898503));
#101466=DIRECTION('ref_axis',(0.,-1.,0.));
#101467=DIRECTION('',(-0.190809912898503,0.,0.981627005099017));
#101468=DIRECTION('',(0.,-1.,0.));
#101469=DIRECTION('',(0.,-1.,0.));
#101470=DIRECTION('center_axis',(0.,-1.,0.));
#101471=DIRECTION('ref_axis',(0.,0.,-1.));
#101472=DIRECTION('',(-0.190809912898503,0.,0.981627005099017));
#101473=DIRECTION('',(-0.981627005099017,0.,-0.190809912898503));
#101474=DIRECTION('',(-0.981627005099017,0.,-0.190809912898503));
#101475=DIRECTION('center_axis',(-0.981627005099017,0.,-0.190809912898503));
#101476=DIRECTION('ref_axis',(-0.190809912898503,0.,0.981627005099017));
#101477=DIRECTION('',(0.,1.,0.));
#101478=DIRECTION('',(0.,1.,0.));
#101479=DIRECTION('center_axis',(0.,1.,0.));
#101480=DIRECTION('ref_axis',(1.,0.,0.));
#101481=DIRECTION('',(-0.190809912898503,0.,0.981627005099017));
#101482=DIRECTION('',(0.981627005099017,0.,0.190809912898503));
#101483=DIRECTION('',(-0.190809912898503,0.,0.981627005099017));
#101484=DIRECTION('',(0.981627005099017,0.,0.190809912898503));
#101485=DIRECTION('center_axis',(0.981627005099017,0.,0.190809912898503));
#101486=DIRECTION('ref_axis',(0.,-1.,0.));
#101487=DIRECTION('',(-0.190809912898503,0.,0.981627005099017));
#101488=DIRECTION('',(0.,-1.,0.));
#101489=DIRECTION('',(0.,-1.,0.));
#101490=DIRECTION('center_axis',(0.,-1.,0.));
#101491=DIRECTION('ref_axis',(0.,0.,-1.));
#101492=DIRECTION('',(-0.190809912898503,0.,0.981627005099017));
#101493=DIRECTION('',(-0.981627005099017,0.,-0.190809912898503));
#101494=DIRECTION('',(-0.981627005099017,0.,-0.190809912898503));
#101495=DIRECTION('center_axis',(-0.981627005099017,0.,-0.190809912898503));
#101496=DIRECTION('ref_axis',(-0.190809912898503,0.,0.981627005099017));
#101497=DIRECTION('',(0.,1.,0.));
#101498=DIRECTION('',(0.,1.,0.));
#101499=DIRECTION('center_axis',(0.,1.,0.));
#101500=DIRECTION('ref_axis',(1.,0.,0.));
#101501=DIRECTION('',(-0.190809912898503,0.,0.981627005099017));
#101502=DIRECTION('',(0.981627005099017,0.,0.190809912898503));
#101503=DIRECTION('',(-0.190809912898503,0.,0.981627005099017));
#101504=DIRECTION('',(0.981627005099017,0.,0.190809912898503));
#101505=DIRECTION('center_axis',(0.981627005099017,0.,0.190809912898503));
#101506=DIRECTION('ref_axis',(0.,-1.,0.));
#101507=DIRECTION('',(-0.190809912898503,0.,0.981627005099017));
#101508=DIRECTION('',(0.,-1.,0.));
#101509=DIRECTION('',(0.,-1.,0.));
#101510=DIRECTION('center_axis',(0.,-1.,0.));
#101511=DIRECTION('ref_axis',(0.,0.,-1.));
#101512=DIRECTION('',(-0.190809912898503,0.,0.981627005099017));
#101513=DIRECTION('',(-0.981627005099017,0.,-0.190809912898503));
#101514=DIRECTION('',(-0.981627005099017,0.,-0.190809912898503));
#101515=DIRECTION('center_axis',(-0.981627005099017,0.,-0.190809912898503));
#101516=DIRECTION('ref_axis',(-0.190809912898503,0.,0.981627005099017));
#101517=DIRECTION('',(0.,1.,0.));
#101518=DIRECTION('',(0.,1.,0.));
#101519=DIRECTION('center_axis',(0.,1.,0.));
#101520=DIRECTION('ref_axis',(1.,0.,0.));
#101521=DIRECTION('',(-0.190809912898503,0.,0.981627005099017));
#101522=DIRECTION('',(0.981627005099017,0.,0.190809912898503));
#101523=DIRECTION('',(-0.190809912898503,0.,0.981627005099017));
#101524=DIRECTION('',(0.981627005099017,0.,0.190809912898503));
#101525=DIRECTION('center_axis',(0.981627005099017,0.,0.190809912898503));
#101526=DIRECTION('ref_axis',(0.,-1.,0.));
#101527=DIRECTION('',(-0.190809912898503,0.,0.981627005099017));
#101528=DIRECTION('',(0.,-1.,0.));
#101529=DIRECTION('',(0.,-1.,0.));
#101530=DIRECTION('center_axis',(0.,-1.,0.));
#101531=DIRECTION('ref_axis',(0.,0.,-1.));
#101532=DIRECTION('',(-0.190809912898503,0.,0.981627005099017));
#101533=DIRECTION('',(-0.981627005099017,0.,-0.190809912898503));
#101534=DIRECTION('',(-0.981627005099017,0.,-0.190809912898503));
#101535=DIRECTION('center_axis',(-0.981627005099017,0.,-0.190809912898503));
#101536=DIRECTION('ref_axis',(-0.190809912898503,0.,0.981627005099017));
#101537=DIRECTION('',(0.,1.,0.));
#101538=DIRECTION('',(0.,1.,0.));
#101539=DIRECTION('center_axis',(0.,1.,0.));
#101540=DIRECTION('ref_axis',(1.,0.,0.));
#101541=DIRECTION('',(-0.190809912898503,0.,0.981627005099017));
#101542=DIRECTION('',(0.981627005099017,0.,0.190809912898503));
#101543=DIRECTION('',(-0.190809912898503,0.,0.981627005099017));
#101544=DIRECTION('',(0.981627005099017,0.,0.190809912898503));
#101545=DIRECTION('center_axis',(0.981627005099017,0.,0.190809912898503));
#101546=DIRECTION('ref_axis',(0.,-1.,0.));
#101547=DIRECTION('',(-0.190809912898503,0.,0.981627005099017));
#101548=DIRECTION('',(0.,-1.,0.));
#101549=DIRECTION('',(0.,-1.,0.));
#101550=DIRECTION('center_axis',(0.,-1.,0.));
#101551=DIRECTION('ref_axis',(0.,0.,-1.));
#101552=DIRECTION('',(-0.190809912898503,0.,0.981627005099017));
#101553=DIRECTION('',(-0.981627005099017,0.,-0.190809912898503));
#101554=DIRECTION('',(-0.981627005099017,0.,-0.190809912898503));
#101555=DIRECTION('center_axis',(-0.981627005099017,0.,-0.190809912898503));
#101556=DIRECTION('ref_axis',(-0.190809912898503,0.,0.981627005099017));
#101557=DIRECTION('',(0.,1.,0.));
#101558=DIRECTION('',(0.,1.,0.));
#101559=DIRECTION('center_axis',(0.,1.,0.));
#101560=DIRECTION('ref_axis',(1.,0.,0.));
#101561=DIRECTION('',(-0.190809912898503,0.,0.981627005099017));
#101562=DIRECTION('',(0.981627005099017,0.,0.190809912898503));
#101563=DIRECTION('',(-0.190809912898503,0.,0.981627005099017));
#101564=DIRECTION('',(0.981627005099017,0.,0.190809912898503));
#101565=DIRECTION('center_axis',(0.981627005099017,0.,0.190809912898503));
#101566=DIRECTION('ref_axis',(0.,-1.,0.));
#101567=DIRECTION('',(-0.190809912898503,0.,0.981627005099017));
#101568=DIRECTION('',(0.,-1.,0.));
#101569=DIRECTION('',(0.,-1.,0.));
#101570=DIRECTION('center_axis',(0.,-1.,0.));
#101571=DIRECTION('ref_axis',(0.,0.,-1.));
#101572=DIRECTION('',(-0.190809912898503,0.,0.981627005099017));
#101573=DIRECTION('',(-0.981627005099017,0.,-0.190809912898503));
#101574=DIRECTION('',(-0.981627005099017,0.,-0.190809912898503));
#101575=DIRECTION('center_axis',(-0.981627005099017,0.,-0.190809912898503));
#101576=DIRECTION('ref_axis',(-0.190809912898503,0.,0.981627005099017));
#101577=DIRECTION('',(0.,1.,0.));
#101578=DIRECTION('',(0.,1.,0.));
#101579=DIRECTION('center_axis',(0.,1.,0.));
#101580=DIRECTION('ref_axis',(1.,0.,0.));
#101581=DIRECTION('',(-0.190809912898503,0.,0.981627005099017));
#101582=DIRECTION('',(0.981627005099017,0.,0.190809912898503));
#101583=DIRECTION('',(-0.190809912898503,0.,0.981627005099017));
#101584=DIRECTION('',(0.981627005099017,0.,0.190809912898503));
#101585=DIRECTION('center_axis',(0.981627005099017,0.,0.190809912898503));
#101586=DIRECTION('ref_axis',(0.,-1.,0.));
#101587=DIRECTION('',(-0.190809912898503,0.,0.981627005099017));
#101588=DIRECTION('',(0.,-1.,0.));
#101589=DIRECTION('',(0.,-1.,0.));
#101590=DIRECTION('center_axis',(0.,-1.,0.));
#101591=DIRECTION('ref_axis',(0.,0.,-1.));
#101592=DIRECTION('',(-0.190809912898503,0.,0.981627005099017));
#101593=DIRECTION('',(-0.981627005099017,0.,-0.190809912898503));
#101594=DIRECTION('',(-0.981627005099017,0.,-0.190809912898503));
#101595=DIRECTION('center_axis',(-0.981627005099017,0.,-0.190809912898503));
#101596=DIRECTION('ref_axis',(-0.190809912898503,0.,0.981627005099017));
#101597=DIRECTION('',(0.,1.,0.));
#101598=DIRECTION('',(0.,1.,0.));
#101599=DIRECTION('center_axis',(0.,1.,0.));
#101600=DIRECTION('ref_axis',(1.,0.,0.));
#101601=DIRECTION('',(-0.190809912898503,0.,0.981627005099017));
#101602=DIRECTION('',(0.981627005099017,0.,0.190809912898503));
#101603=DIRECTION('',(-0.190809912898503,0.,0.981627005099017));
#101604=DIRECTION('',(0.981627005099017,0.,0.190809912898503));
#101605=DIRECTION('center_axis',(0.981627005099017,0.,0.190809912898503));
#101606=DIRECTION('ref_axis',(0.,-1.,0.));
#101607=DIRECTION('',(-0.190809912898503,0.,0.981627005099017));
#101608=DIRECTION('',(0.,-1.,0.));
#101609=DIRECTION('',(0.,-1.,0.));
#101610=DIRECTION('center_axis',(0.,-1.,0.));
#101611=DIRECTION('ref_axis',(0.,0.,-1.));
#101612=DIRECTION('',(-0.190809912898503,0.,0.981627005099017));
#101613=DIRECTION('',(-0.981627005099017,0.,-0.190809912898503));
#101614=DIRECTION('',(-0.981627005099017,0.,-0.190809912898503));
#101615=DIRECTION('center_axis',(-0.981627005099017,0.,-0.190809912898503));
#101616=DIRECTION('ref_axis',(-0.190809912898503,0.,0.981627005099017));
#101617=DIRECTION('',(0.,1.,0.));
#101618=DIRECTION('',(0.,1.,0.));
#101619=DIRECTION('center_axis',(0.,1.,0.));
#101620=DIRECTION('ref_axis',(1.,0.,0.));
#101621=DIRECTION('',(-0.190809912898503,0.,0.981627005099017));
#101622=DIRECTION('',(0.981627005099017,0.,0.190809912898503));
#101623=DIRECTION('',(-0.190809912898503,0.,0.981627005099017));
#101624=DIRECTION('',(0.981627005099017,0.,0.190809912898503));
#101625=DIRECTION('center_axis',(0.981627005099017,0.,0.190809912898503));
#101626=DIRECTION('ref_axis',(0.,-1.,0.));
#101627=DIRECTION('',(-0.190809912898503,0.,0.981627005099017));
#101628=DIRECTION('',(0.,-1.,0.));
#101629=DIRECTION('',(0.,-1.,0.));
#101630=DIRECTION('center_axis',(0.,-1.,0.));
#101631=DIRECTION('ref_axis',(0.,0.,-1.));
#101632=DIRECTION('',(-0.190809912898503,0.,0.981627005099017));
#101633=DIRECTION('',(-0.981627005099017,0.,-0.190809912898503));
#101634=DIRECTION('',(-0.981627005099017,0.,-0.190809912898503));
#101635=DIRECTION('center_axis',(-0.981627005099017,0.,-0.190809912898503));
#101636=DIRECTION('ref_axis',(-0.190809912898503,0.,0.981627005099017));
#101637=DIRECTION('',(0.,1.,0.));
#101638=DIRECTION('',(0.,1.,0.));
#101639=DIRECTION('center_axis',(0.,1.,0.));
#101640=DIRECTION('ref_axis',(1.,0.,0.));
#101641=DIRECTION('',(-0.190809912898503,0.,0.981627005099017));
#101642=DIRECTION('',(0.981627005099017,0.,0.190809912898503));
#101643=DIRECTION('',(-0.190809912898503,0.,0.981627005099017));
#101644=DIRECTION('',(0.981627005099017,0.,0.190809912898503));
#101645=DIRECTION('center_axis',(0.981627005099017,0.,0.190809912898503));
#101646=DIRECTION('ref_axis',(0.,-1.,0.));
#101647=DIRECTION('',(-0.190809912898503,0.,0.981627005099017));
#101648=DIRECTION('',(0.,-1.,0.));
#101649=DIRECTION('',(0.,-1.,0.));
#101650=DIRECTION('center_axis',(0.,-1.,0.));
#101651=DIRECTION('ref_axis',(0.,0.,-1.));
#101652=DIRECTION('',(-0.190809912898503,0.,0.981627005099017));
#101653=DIRECTION('',(-0.981627005099017,0.,-0.190809912898503));
#101654=DIRECTION('',(-0.981627005099017,0.,-0.190809912898503));
#101655=DIRECTION('center_axis',(-0.981627005099017,0.,-0.190809912898503));
#101656=DIRECTION('ref_axis',(-0.190809912898503,0.,0.981627005099017));
#101657=DIRECTION('',(0.,1.,0.));
#101658=DIRECTION('',(0.,1.,0.));
#101659=DIRECTION('center_axis',(0.,1.,0.));
#101660=DIRECTION('ref_axis',(1.,0.,0.));
#101661=DIRECTION('',(-0.190809912898503,0.,0.981627005099017));
#101662=DIRECTION('',(0.981627005099017,0.,0.190809912898503));
#101663=DIRECTION('',(-0.190809912898503,0.,0.981627005099017));
#101664=DIRECTION('',(0.981627005099017,0.,0.190809912898503));
#101665=DIRECTION('center_axis',(0.981627005099017,0.,0.190809912898503));
#101666=DIRECTION('ref_axis',(0.,-1.,0.));
#101667=DIRECTION('',(-0.190809912898503,0.,0.981627005099017));
#101668=DIRECTION('',(0.,-1.,0.));
#101669=DIRECTION('',(0.,-1.,0.));
#101670=DIRECTION('center_axis',(0.,-1.,0.));
#101671=DIRECTION('ref_axis',(0.,0.,-1.));
#101672=DIRECTION('',(-0.190809912898503,0.,0.981627005099017));
#101673=DIRECTION('',(-0.981627005099017,0.,-0.190809912898503));
#101674=DIRECTION('',(-0.981627005099017,0.,-0.190809912898503));
#101675=DIRECTION('center_axis',(-0.981627005099017,0.,-0.190809912898503));
#101676=DIRECTION('ref_axis',(-0.190809912898503,0.,0.981627005099017));
#101677=DIRECTION('',(0.,1.,0.));
#101678=DIRECTION('',(0.,1.,0.));
#101679=DIRECTION('center_axis',(0.,1.,0.));
#101680=DIRECTION('ref_axis',(1.,0.,0.));
#101681=DIRECTION('',(-0.190809912898503,0.,0.981627005099017));
#101682=DIRECTION('',(0.981627005099017,0.,0.190809912898503));
#101683=DIRECTION('',(-0.190809912898503,0.,0.981627005099017));
#101684=DIRECTION('',(0.981627005099017,0.,0.190809912898503));
#101685=DIRECTION('center_axis',(0.981627005099017,0.,0.190809912898503));
#101686=DIRECTION('ref_axis',(0.,-1.,0.));
#101687=DIRECTION('',(-0.190809912898503,0.,0.981627005099017));
#101688=DIRECTION('',(0.,-1.,0.));
#101689=DIRECTION('',(0.,-1.,0.));
#101690=DIRECTION('center_axis',(0.,-1.,0.));
#101691=DIRECTION('ref_axis',(0.,0.,-1.));
#101692=DIRECTION('',(-0.190809912898503,0.,0.981627005099017));
#101693=DIRECTION('',(-0.981627005099017,0.,-0.190809912898503));
#101694=DIRECTION('',(-0.981627005099017,0.,-0.190809912898503));
#101695=DIRECTION('center_axis',(-0.981627005099017,0.,-0.190809912898503));
#101696=DIRECTION('ref_axis',(-0.190809912898503,0.,0.981627005099017));
#101697=DIRECTION('',(0.,1.,0.));
#101698=DIRECTION('',(0.,1.,0.));
#101699=DIRECTION('center_axis',(0.,1.,0.));
#101700=DIRECTION('ref_axis',(1.,0.,0.));
#101701=DIRECTION('',(-0.190809912898503,0.,0.981627005099017));
#101702=DIRECTION('',(0.981627005099017,0.,0.190809912898503));
#101703=DIRECTION('',(-0.190809912898503,0.,0.981627005099017));
#101704=DIRECTION('',(0.981627005099017,0.,0.190809912898503));
#101705=DIRECTION('center_axis',(0.981627005099017,0.,0.190809912898503));
#101706=DIRECTION('ref_axis',(0.,-1.,0.));
#101707=DIRECTION('',(-0.190809912898503,0.,0.981627005099017));
#101708=DIRECTION('',(0.,-1.,0.));
#101709=DIRECTION('',(0.,-1.,0.));
#101710=DIRECTION('center_axis',(0.,-1.,0.));
#101711=DIRECTION('ref_axis',(0.,0.,-1.));
#101712=DIRECTION('',(-0.190809912898503,0.,0.981627005099017));
#101713=DIRECTION('',(-0.981627005099017,0.,-0.190809912898503));
#101714=DIRECTION('',(-0.981627005099017,0.,-0.190809912898503));
#101715=DIRECTION('center_axis',(-0.981627005099017,0.,-0.190809912898503));
#101716=DIRECTION('ref_axis',(-0.190809912898503,0.,0.981627005099017));
#101717=DIRECTION('',(0.,1.,0.));
#101718=DIRECTION('',(0.,1.,0.));
#101719=DIRECTION('center_axis',(0.,1.,0.));
#101720=DIRECTION('ref_axis',(1.,0.,0.));
#101721=DIRECTION('',(-0.190809912898503,0.,0.981627005099017));
#101722=DIRECTION('',(0.981627005099017,0.,0.190809912898503));
#101723=DIRECTION('',(-0.190809912898503,0.,0.981627005099017));
#101724=DIRECTION('',(0.981627005099017,0.,0.190809912898503));
#101725=DIRECTION('center_axis',(0.981627005099017,0.,0.190809912898503));
#101726=DIRECTION('ref_axis',(0.,-1.,0.));
#101727=DIRECTION('',(-0.190809912898503,0.,0.981627005099017));
#101728=DIRECTION('',(0.,-1.,0.));
#101729=DIRECTION('',(0.,-1.,0.));
#101730=DIRECTION('center_axis',(0.,-1.,0.));
#101731=DIRECTION('ref_axis',(0.,0.,-1.));
#101732=DIRECTION('',(-0.190809912898503,0.,0.981627005099017));
#101733=DIRECTION('',(-0.981627005099017,0.,-0.190809912898503));
#101734=DIRECTION('',(-0.981627005099017,0.,-0.190809912898503));
#101735=DIRECTION('center_axis',(-0.981627005099017,0.,-0.190809912898503));
#101736=DIRECTION('ref_axis',(-0.190809912898503,0.,0.981627005099017));
#101737=DIRECTION('',(0.,1.,0.));
#101738=DIRECTION('',(0.,1.,0.));
#101739=DIRECTION('center_axis',(0.,1.,0.));
#101740=DIRECTION('ref_axis',(1.,0.,0.));
#101741=DIRECTION('',(-0.190809912898503,0.,0.981627005099017));
#101742=DIRECTION('',(0.981627005099017,0.,0.190809912898503));
#101743=DIRECTION('',(-0.190809912898503,0.,0.981627005099017));
#101744=DIRECTION('',(0.981627005099017,0.,0.190809912898503));
#101745=DIRECTION('center_axis',(0.981627005099017,0.,0.190809912898503));
#101746=DIRECTION('ref_axis',(0.,-1.,0.));
#101747=DIRECTION('',(-0.190809912898503,0.,0.981627005099017));
#101748=DIRECTION('',(0.,-1.,0.));
#101749=DIRECTION('',(0.,-1.,0.));
#101750=DIRECTION('center_axis',(0.,-1.,0.));
#101751=DIRECTION('ref_axis',(0.,0.,-1.));
#101752=DIRECTION('',(-0.190809912898503,0.,0.981627005099017));
#101753=DIRECTION('',(-0.981627005099017,0.,-0.190809912898503));
#101754=DIRECTION('',(-0.981627005099017,0.,-0.190809912898503));
#101755=DIRECTION('center_axis',(-0.981627005099017,0.,-0.190809912898503));
#101756=DIRECTION('ref_axis',(-0.190809912898503,0.,0.981627005099017));
#101757=DIRECTION('',(0.,1.,0.));
#101758=DIRECTION('',(0.,1.,0.));
#101759=DIRECTION('center_axis',(0.,1.,0.));
#101760=DIRECTION('ref_axis',(1.,0.,0.));
#101761=DIRECTION('',(-0.190809912898503,0.,0.981627005099017));
#101762=DIRECTION('',(0.981627005099017,0.,0.190809912898503));
#101763=DIRECTION('',(-0.190809912898503,0.,0.981627005099017));
#101764=DIRECTION('',(0.981627005099017,0.,0.190809912898503));
#101765=DIRECTION('center_axis',(0.981627005099017,0.,0.190809912898503));
#101766=DIRECTION('ref_axis',(0.,-1.,0.));
#101767=DIRECTION('',(-0.190809912898503,0.,0.981627005099017));
#101768=DIRECTION('',(0.,-1.,0.));
#101769=DIRECTION('',(0.,-1.,0.));
#101770=DIRECTION('center_axis',(0.,-1.,0.));
#101771=DIRECTION('ref_axis',(0.,0.,-1.));
#101772=DIRECTION('',(-0.190809912898503,0.,0.981627005099017));
#101773=DIRECTION('',(-0.981627005099017,0.,-0.190809912898503));
#101774=DIRECTION('',(-0.981627005099017,0.,-0.190809912898503));
#101775=DIRECTION('center_axis',(-0.981627005099017,0.,-0.190809912898503));
#101776=DIRECTION('ref_axis',(-0.190809912898503,0.,0.981627005099017));
#101777=DIRECTION('',(0.,1.,0.));
#101778=DIRECTION('',(0.,1.,0.));
#101779=DIRECTION('center_axis',(0.,1.,0.));
#101780=DIRECTION('ref_axis',(1.,0.,0.));
#101781=DIRECTION('',(-0.190809912898503,0.,0.981627005099017));
#101782=DIRECTION('',(0.981627005099017,0.,0.190809912898503));
#101783=DIRECTION('',(-0.190809912898503,0.,0.981627005099017));
#101784=DIRECTION('',(0.981627005099017,0.,0.190809912898503));
#101785=DIRECTION('center_axis',(0.981627005099017,0.,0.190809912898503));
#101786=DIRECTION('ref_axis',(0.,-1.,0.));
#101787=DIRECTION('',(-0.190809912898503,0.,0.981627005099017));
#101788=DIRECTION('',(0.,-1.,0.));
#101789=DIRECTION('',(0.,-1.,0.));
#101790=DIRECTION('center_axis',(0.,-1.,0.));
#101791=DIRECTION('ref_axis',(0.,0.,-1.));
#101792=DIRECTION('',(-0.190809912898503,0.,0.981627005099017));
#101793=DIRECTION('',(-0.981627005099017,0.,-0.190809912898503));
#101794=DIRECTION('',(-0.981627005099017,0.,-0.190809912898503));
#101795=DIRECTION('center_axis',(-0.981627005099017,0.,-0.190809912898503));
#101796=DIRECTION('ref_axis',(-0.190809912898503,0.,0.981627005099017));
#101797=DIRECTION('',(0.,1.,0.));
#101798=DIRECTION('',(0.,1.,0.));
#101799=DIRECTION('center_axis',(0.,1.,0.));
#101800=DIRECTION('ref_axis',(1.,0.,0.));
#101801=DIRECTION('',(-0.190809912898503,0.,0.981627005099017));
#101802=DIRECTION('',(0.981627005099017,0.,0.190809912898503));
#101803=DIRECTION('',(-0.190809912898503,0.,0.981627005099017));
#101804=DIRECTION('',(0.981627005099017,0.,0.190809912898503));
#101805=DIRECTION('center_axis',(0.981627005099017,0.,0.190809912898503));
#101806=DIRECTION('ref_axis',(0.,-1.,0.));
#101807=DIRECTION('',(-0.190809912898503,0.,0.981627005099017));
#101808=DIRECTION('',(0.,-1.,0.));
#101809=DIRECTION('',(0.,-1.,0.));
#101810=DIRECTION('center_axis',(0.,-1.,0.));
#101811=DIRECTION('ref_axis',(0.,0.,-1.));
#101812=DIRECTION('',(-0.190809912898503,0.,0.981627005099017));
#101813=DIRECTION('',(-0.981627005099017,0.,-0.190809912898503));
#101814=DIRECTION('',(-0.981627005099017,0.,-0.190809912898503));
#101815=DIRECTION('center_axis',(-0.981627005099017,0.,-0.190809912898503));
#101816=DIRECTION('ref_axis',(-0.190809912898503,0.,0.981627005099017));
#101817=DIRECTION('',(0.,1.,0.));
#101818=DIRECTION('',(0.,1.,0.));
#101819=DIRECTION('center_axis',(0.,1.,0.));
#101820=DIRECTION('ref_axis',(1.,0.,0.));
#101821=DIRECTION('',(-0.190809912898503,0.,0.981627005099017));
#101822=DIRECTION('',(0.981627005099017,0.,0.190809912898503));
#101823=DIRECTION('',(-0.190809912898503,0.,0.981627005099017));
#101824=DIRECTION('',(0.981627005099017,0.,0.190809912898503));
#101825=DIRECTION('center_axis',(0.981627005099017,0.,0.190809912898503));
#101826=DIRECTION('ref_axis',(0.,-1.,0.));
#101827=DIRECTION('',(-0.190809912898503,0.,0.981627005099017));
#101828=DIRECTION('',(0.,-1.,0.));
#101829=DIRECTION('',(0.,-1.,0.));
#101830=DIRECTION('center_axis',(0.,-1.,0.));
#101831=DIRECTION('ref_axis',(0.,0.,-1.));
#101832=DIRECTION('',(-0.190809912898503,0.,0.981627005099017));
#101833=DIRECTION('',(-0.981627005099017,0.,-0.190809912898503));
#101834=DIRECTION('',(-0.981627005099017,0.,-0.190809912898503));
#101835=DIRECTION('center_axis',(-0.981627005099017,0.,-0.190809912898503));
#101836=DIRECTION('ref_axis',(-0.190809912898503,0.,0.981627005099017));
#101837=DIRECTION('',(0.,1.,0.));
#101838=DIRECTION('',(0.,1.,0.));
#101839=DIRECTION('center_axis',(0.,1.,0.));
#101840=DIRECTION('ref_axis',(1.,0.,0.));
#101841=DIRECTION('',(-0.190809912898503,0.,0.981627005099017));
#101842=DIRECTION('',(0.981627005099017,0.,0.190809912898503));
#101843=DIRECTION('',(-0.190809912898503,0.,0.981627005099017));
#101844=DIRECTION('',(0.981627005099017,0.,0.190809912898503));
#101845=DIRECTION('center_axis',(0.981627005099017,0.,0.190809912898503));
#101846=DIRECTION('ref_axis',(0.,-1.,0.));
#101847=DIRECTION('',(-0.190809912898503,0.,0.981627005099017));
#101848=DIRECTION('',(0.,-1.,0.));
#101849=DIRECTION('',(0.,-1.,0.));
#101850=DIRECTION('center_axis',(0.,-1.,0.));
#101851=DIRECTION('ref_axis',(0.,0.,-1.));
#101852=DIRECTION('',(-0.190809912898503,0.,0.981627005099017));
#101853=DIRECTION('',(-0.981627005099017,0.,-0.190809912898503));
#101854=DIRECTION('',(-0.981627005099017,0.,-0.190809912898503));
#101855=DIRECTION('center_axis',(-0.981627005099017,0.,-0.190809912898503));
#101856=DIRECTION('ref_axis',(-0.190809912898503,0.,0.981627005099017));
#101857=DIRECTION('',(0.,1.,0.));
#101858=DIRECTION('',(0.,1.,0.));
#101859=DIRECTION('center_axis',(0.,1.,0.));
#101860=DIRECTION('ref_axis',(1.,0.,0.));
#101861=DIRECTION('',(-0.190809912898503,0.,0.981627005099017));
#101862=DIRECTION('',(0.981627005099017,0.,0.190809912898503));
#101863=DIRECTION('',(-0.190809912898503,0.,0.981627005099017));
#101864=DIRECTION('',(0.981627005099017,0.,0.190809912898503));
#101865=DIRECTION('center_axis',(0.981627005099017,0.,0.190809912898503));
#101866=DIRECTION('ref_axis',(0.,-1.,0.));
#101867=DIRECTION('',(-0.190809912898503,0.,0.981627005099017));
#101868=DIRECTION('',(0.,-1.,0.));
#101869=DIRECTION('',(0.,-1.,0.));
#101870=DIRECTION('center_axis',(0.,-1.,0.));
#101871=DIRECTION('ref_axis',(0.,0.,-1.));
#101872=DIRECTION('',(-0.190809912898503,0.,0.981627005099017));
#101873=DIRECTION('',(-0.981627005099017,0.,-0.190809912898503));
#101874=DIRECTION('',(-0.981627005099017,0.,-0.190809912898503));
#101875=DIRECTION('center_axis',(-0.981627005099017,0.,-0.190809912898503));
#101876=DIRECTION('ref_axis',(-0.190809912898503,0.,0.981627005099017));
#101877=DIRECTION('',(0.,1.,0.));
#101878=DIRECTION('',(0.,1.,0.));
#101879=DIRECTION('center_axis',(0.,1.,0.));
#101880=DIRECTION('ref_axis',(1.,0.,0.));
#101881=DIRECTION('',(-0.190809912898503,0.,0.981627005099017));
#101882=DIRECTION('',(0.981627005099017,0.,0.190809912898503));
#101883=DIRECTION('',(-0.190809912898503,0.,0.981627005099017));
#101884=DIRECTION('',(0.981627005099017,0.,0.190809912898503));
#101885=DIRECTION('center_axis',(0.981627005099017,0.,0.190809912898503));
#101886=DIRECTION('ref_axis',(0.,-1.,0.));
#101887=DIRECTION('',(-0.190809912898503,0.,0.981627005099017));
#101888=DIRECTION('',(0.,-1.,0.));
#101889=DIRECTION('',(0.,-1.,0.));
#101890=DIRECTION('center_axis',(0.,-1.,0.));
#101891=DIRECTION('ref_axis',(0.,0.,-1.));
#101892=DIRECTION('',(-0.190809912898503,0.,0.981627005099017));
#101893=DIRECTION('',(-0.981627005099017,0.,-0.190809912898503));
#101894=DIRECTION('',(-0.981627005099017,0.,-0.190809912898503));
#101895=DIRECTION('center_axis',(-0.981627005099017,0.,-0.190809912898503));
#101896=DIRECTION('ref_axis',(-0.190809912898503,0.,0.981627005099017));
#101897=DIRECTION('',(0.,1.,0.));
#101898=DIRECTION('',(0.,1.,0.));
#101899=DIRECTION('center_axis',(0.,1.,0.));
#101900=DIRECTION('ref_axis',(1.,0.,0.));
#101901=DIRECTION('',(-0.190809912898503,0.,0.981627005099017));
#101902=DIRECTION('',(0.981627005099017,0.,0.190809912898503));
#101903=DIRECTION('',(-0.190809912898503,0.,0.981627005099017));
#101904=DIRECTION('',(0.981627005099017,0.,0.190809912898503));
#101905=DIRECTION('center_axis',(0.981627005099017,0.,0.190809912898503));
#101906=DIRECTION('ref_axis',(0.,-1.,0.));
#101907=DIRECTION('',(-0.190809912898503,0.,0.981627005099017));
#101908=DIRECTION('',(0.,-1.,0.));
#101909=DIRECTION('',(0.,-1.,0.));
#101910=DIRECTION('center_axis',(0.,-1.,0.));
#101911=DIRECTION('ref_axis',(0.,0.,-1.));
#101912=DIRECTION('',(-0.190809912898503,0.,0.981627005099017));
#101913=DIRECTION('',(-0.981627005099017,0.,-0.190809912898503));
#101914=DIRECTION('',(-0.981627005099017,0.,-0.190809912898503));
#101915=DIRECTION('center_axis',(-0.981627005099017,0.,-0.190809912898503));
#101916=DIRECTION('ref_axis',(-0.190809912898503,0.,0.981627005099017));
#101917=DIRECTION('',(0.,1.,0.));
#101918=DIRECTION('',(0.,1.,0.));
#101919=DIRECTION('center_axis',(0.,1.,0.));
#101920=DIRECTION('ref_axis',(1.,0.,0.));
#101921=DIRECTION('',(-0.190809912898503,0.,0.981627005099017));
#101922=DIRECTION('',(0.981627005099017,0.,0.190809912898503));
#101923=DIRECTION('',(-0.190809912898503,0.,0.981627005099017));
#101924=DIRECTION('',(0.981627005099017,0.,0.190809912898503));
#101925=DIRECTION('center_axis',(0.981627005099017,0.,0.190809912898503));
#101926=DIRECTION('ref_axis',(0.,-1.,0.));
#101927=DIRECTION('',(-0.190809912898503,0.,0.981627005099017));
#101928=DIRECTION('',(0.,-1.,0.));
#101929=DIRECTION('',(0.,-1.,0.));
#101930=DIRECTION('center_axis',(0.,-1.,0.));
#101931=DIRECTION('ref_axis',(0.,0.,-1.));
#101932=DIRECTION('',(-0.190809912898503,0.,0.981627005099017));
#101933=DIRECTION('',(-0.981627005099017,0.,-0.190809912898503));
#101934=DIRECTION('',(-0.981627005099017,0.,-0.190809912898503));
#101935=DIRECTION('center_axis',(-0.981627005099017,0.,-0.190809912898503));
#101936=DIRECTION('ref_axis',(-0.190809912898503,0.,0.981627005099017));
#101937=DIRECTION('',(0.,1.,0.));
#101938=DIRECTION('',(0.,1.,0.));
#101939=DIRECTION('center_axis',(0.,1.,0.));
#101940=DIRECTION('ref_axis',(1.,0.,0.));
#101941=DIRECTION('',(-0.190809912898503,0.,0.981627005099017));
#101942=DIRECTION('',(0.981627005099017,0.,0.190809912898503));
#101943=DIRECTION('',(-0.190809912898503,0.,0.981627005099017));
#101944=DIRECTION('',(0.981627005099017,0.,0.190809912898503));
#101945=DIRECTION('center_axis',(0.981627005099017,0.,0.190809912898503));
#101946=DIRECTION('ref_axis',(0.,-1.,0.));
#101947=DIRECTION('',(-0.190809912898503,0.,0.981627005099017));
#101948=DIRECTION('',(0.,-1.,0.));
#101949=DIRECTION('',(0.,-1.,0.));
#101950=DIRECTION('center_axis',(0.,-1.,0.));
#101951=DIRECTION('ref_axis',(0.,0.,-1.));
#101952=DIRECTION('',(-0.190809912898503,0.,0.981627005099017));
#101953=DIRECTION('',(-0.981627005099017,0.,-0.190809912898503));
#101954=DIRECTION('',(-0.981627005099017,0.,-0.190809912898503));
#101955=DIRECTION('center_axis',(-0.981627005099017,0.,-0.190809912898503));
#101956=DIRECTION('ref_axis',(-0.190809912898503,0.,0.981627005099017));
#101957=DIRECTION('',(0.,1.,0.));
#101958=DIRECTION('',(0.,1.,0.));
#101959=DIRECTION('center_axis',(0.,1.,0.));
#101960=DIRECTION('ref_axis',(1.,0.,0.));
#101961=DIRECTION('',(-0.190809912898503,0.,0.981627005099017));
#101962=DIRECTION('',(0.981627005099017,0.,0.190809912898503));
#101963=DIRECTION('',(-0.190809912898503,0.,0.981627005099017));
#101964=DIRECTION('',(0.981627005099017,0.,0.190809912898503));
#101965=DIRECTION('center_axis',(0.981627005099017,0.,0.190809912898503));
#101966=DIRECTION('ref_axis',(0.,-1.,0.));
#101967=DIRECTION('',(-0.190809912898503,0.,0.981627005099017));
#101968=DIRECTION('',(0.,-1.,0.));
#101969=DIRECTION('',(0.,-1.,0.));
#101970=DIRECTION('center_axis',(0.,-1.,0.));
#101971=DIRECTION('ref_axis',(0.,0.,-1.));
#101972=DIRECTION('',(-0.190809912898503,0.,0.981627005099017));
#101973=DIRECTION('',(-0.981627005099017,0.,-0.190809912898503));
#101974=DIRECTION('',(-0.981627005099017,0.,-0.190809912898503));
#101975=DIRECTION('center_axis',(-0.981627005099017,0.,-0.190809912898503));
#101976=DIRECTION('ref_axis',(-0.190809912898503,0.,0.981627005099017));
#101977=DIRECTION('',(0.,1.,0.));
#101978=DIRECTION('',(0.,1.,0.));
#101979=DIRECTION('center_axis',(0.,1.,0.));
#101980=DIRECTION('ref_axis',(1.,0.,0.));
#101981=DIRECTION('',(-0.190809912898503,0.,0.981627005099017));
#101982=DIRECTION('',(0.981627005099017,0.,0.190809912898503));
#101983=DIRECTION('',(-0.190809912898503,0.,0.981627005099017));
#101984=DIRECTION('',(0.981627005099017,0.,0.190809912898503));
#101985=DIRECTION('center_axis',(0.981627005099017,0.,0.190809912898503));
#101986=DIRECTION('ref_axis',(0.,-1.,0.));
#101987=DIRECTION('',(-0.190809912898503,0.,0.981627005099017));
#101988=DIRECTION('',(0.,-1.,0.));
#101989=DIRECTION('',(0.,-1.,0.));
#101990=DIRECTION('center_axis',(0.,-1.,0.));
#101991=DIRECTION('ref_axis',(0.,0.,-1.));
#101992=DIRECTION('',(-0.190809912898503,0.,0.981627005099017));
#101993=DIRECTION('',(-0.981627005099017,0.,-0.190809912898503));
#101994=DIRECTION('',(-0.981627005099017,0.,-0.190809912898503));
#101995=DIRECTION('center_axis',(-0.981627005099017,0.,-0.190809912898503));
#101996=DIRECTION('ref_axis',(-0.190809912898503,0.,0.981627005099017));
#101997=DIRECTION('',(0.,1.,0.));
#101998=DIRECTION('',(0.,1.,0.));
#101999=DIRECTION('center_axis',(0.,1.,0.));
#102000=DIRECTION('ref_axis',(1.,0.,0.));
#102001=DIRECTION('',(-0.190809912898503,0.,0.981627005099017));
#102002=DIRECTION('',(0.981627005099017,0.,0.190809912898503));
#102003=DIRECTION('',(-0.190809912898503,0.,0.981627005099017));
#102004=DIRECTION('',(0.981627005099017,0.,0.190809912898503));
#102005=DIRECTION('center_axis',(0.981627005099017,0.,0.190809912898503));
#102006=DIRECTION('ref_axis',(0.,-1.,0.));
#102007=DIRECTION('',(-0.190809912898503,0.,0.981627005099017));
#102008=DIRECTION('',(0.,-1.,0.));
#102009=DIRECTION('',(0.,-1.,0.));
#102010=DIRECTION('center_axis',(0.,-1.,0.));
#102011=DIRECTION('ref_axis',(0.,0.,-1.));
#102012=DIRECTION('',(-0.190809912898503,0.,0.981627005099017));
#102013=DIRECTION('',(-0.981627005099017,0.,-0.190809912898503));
#102014=DIRECTION('',(-0.981627005099017,0.,-0.190809912898503));
#102015=DIRECTION('center_axis',(-0.981627005099017,0.,-0.190809912898503));
#102016=DIRECTION('ref_axis',(-0.190809912898503,0.,0.981627005099017));
#102017=DIRECTION('',(0.,1.,0.));
#102018=DIRECTION('',(0.,1.,0.));
#102019=DIRECTION('center_axis',(0.,1.,0.));
#102020=DIRECTION('ref_axis',(1.,0.,0.));
#102021=DIRECTION('',(-0.190809912898503,0.,0.981627005099017));
#102022=DIRECTION('',(0.981627005099017,0.,0.190809912898503));
#102023=DIRECTION('',(-0.190809912898503,0.,0.981627005099017));
#102024=DIRECTION('',(0.981627005099017,0.,0.190809912898503));
#102025=DIRECTION('center_axis',(0.981627005099017,0.,0.190809912898503));
#102026=DIRECTION('ref_axis',(0.,-1.,0.));
#102027=DIRECTION('',(-0.190809912898503,0.,0.981627005099017));
#102028=DIRECTION('',(0.,-1.,0.));
#102029=DIRECTION('',(0.,-1.,0.));
#102030=DIRECTION('center_axis',(0.,-1.,0.));
#102031=DIRECTION('ref_axis',(0.,0.,-1.));
#102032=DIRECTION('',(-0.190809912898503,0.,0.981627005099017));
#102033=DIRECTION('',(-0.981627005099017,0.,-0.190809912898503));
#102034=DIRECTION('',(-0.981627005099017,0.,-0.190809912898503));
#102035=DIRECTION('center_axis',(-0.981627005099017,0.,-0.190809912898503));
#102036=DIRECTION('ref_axis',(-0.190809912898503,0.,0.981627005099017));
#102037=DIRECTION('',(0.,1.,0.));
#102038=DIRECTION('',(0.,1.,0.));
#102039=DIRECTION('center_axis',(0.,1.,0.));
#102040=DIRECTION('ref_axis',(1.,0.,0.));
#102041=DIRECTION('',(-0.190809912898503,0.,0.981627005099017));
#102042=DIRECTION('',(0.981627005099017,0.,0.190809912898503));
#102043=DIRECTION('',(-0.190809912898503,0.,0.981627005099017));
#102044=DIRECTION('',(0.981627005099017,0.,0.190809912898503));
#102045=DIRECTION('center_axis',(0.981627005099017,0.,0.190809912898503));
#102046=DIRECTION('ref_axis',(0.,-1.,0.));
#102047=DIRECTION('',(-0.190809912898503,0.,0.981627005099017));
#102048=DIRECTION('',(0.,-1.,0.));
#102049=DIRECTION('',(0.,-1.,0.));
#102050=DIRECTION('center_axis',(0.,-1.,0.));
#102051=DIRECTION('ref_axis',(0.,0.,-1.));
#102052=DIRECTION('',(-0.190809912898503,0.,0.981627005099017));
#102053=DIRECTION('',(-0.981627005099017,0.,-0.190809912898503));
#102054=DIRECTION('',(-0.981627005099017,0.,-0.190809912898503));
#102055=DIRECTION('center_axis',(-0.981627005099017,0.,-0.190809912898503));
#102056=DIRECTION('ref_axis',(-0.190809912898503,0.,0.981627005099017));
#102057=DIRECTION('',(0.,1.,0.));
#102058=DIRECTION('',(0.,1.,0.));
#102059=DIRECTION('center_axis',(0.,1.,0.));
#102060=DIRECTION('ref_axis',(1.,0.,0.));
#102061=DIRECTION('',(-0.190809912898503,0.,0.981627005099017));
#102062=DIRECTION('',(0.981627005099017,0.,0.190809912898503));
#102063=DIRECTION('',(-0.190809912898503,0.,0.981627005099017));
#102064=DIRECTION('',(0.981627005099017,0.,0.190809912898503));
#102065=DIRECTION('center_axis',(0.981627005099017,0.,0.190809912898503));
#102066=DIRECTION('ref_axis',(0.,-1.,0.));
#102067=DIRECTION('',(-0.190809912898503,0.,0.981627005099017));
#102068=DIRECTION('',(0.,-1.,0.));
#102069=DIRECTION('',(0.,-1.,0.));
#102070=DIRECTION('center_axis',(0.,-1.,0.));
#102071=DIRECTION('ref_axis',(0.,0.,-1.));
#102072=DIRECTION('',(-0.190809912898503,0.,0.981627005099017));
#102073=DIRECTION('',(-0.981627005099017,0.,-0.190809912898503));
#102074=DIRECTION('',(-0.981627005099017,0.,-0.190809912898503));
#102075=DIRECTION('center_axis',(-0.981627005099017,0.,-0.190809912898503));
#102076=DIRECTION('ref_axis',(-0.190809912898503,0.,0.981627005099017));
#102077=DIRECTION('',(0.,1.,0.));
#102078=DIRECTION('',(0.,1.,0.));
#102079=DIRECTION('center_axis',(0.,1.,0.));
#102080=DIRECTION('ref_axis',(1.,0.,0.));
#102081=DIRECTION('',(-0.190809912898503,0.,0.981627005099017));
#102082=DIRECTION('',(0.981627005099017,0.,0.190809912898503));
#102083=DIRECTION('',(-0.190809912898503,0.,0.981627005099017));
#102084=DIRECTION('',(0.981627005099017,0.,0.190809912898503));
#102085=DIRECTION('center_axis',(0.981627005099017,0.,0.190809912898503));
#102086=DIRECTION('ref_axis',(0.,-1.,0.));
#102087=DIRECTION('',(-0.190809912898503,0.,0.981627005099017));
#102088=DIRECTION('',(0.,-1.,0.));
#102089=DIRECTION('',(0.,-1.,0.));
#102090=DIRECTION('center_axis',(0.,-1.,0.));
#102091=DIRECTION('ref_axis',(0.,0.,-1.));
#102092=DIRECTION('',(-0.190809912898503,0.,0.981627005099017));
#102093=DIRECTION('',(-0.981627005099017,0.,-0.190809912898503));
#102094=DIRECTION('',(-0.981627005099017,0.,-0.190809912898503));
#102095=DIRECTION('center_axis',(-0.981627005099017,0.,-0.190809912898503));
#102096=DIRECTION('ref_axis',(-0.190809912898503,0.,0.981627005099017));
#102097=DIRECTION('',(0.,1.,0.));
#102098=DIRECTION('',(0.,1.,0.));
#102099=DIRECTION('center_axis',(0.,1.,0.));
#102100=DIRECTION('ref_axis',(1.,0.,0.));
#102101=DIRECTION('',(-0.190809912898503,0.,0.981627005099017));
#102102=DIRECTION('',(0.981627005099017,0.,0.190809912898503));
#102103=DIRECTION('',(-0.190809912898503,0.,0.981627005099017));
#102104=DIRECTION('',(0.981627005099017,0.,0.190809912898503));
#102105=DIRECTION('center_axis',(0.981627005099017,0.,0.190809912898503));
#102106=DIRECTION('ref_axis',(0.,-1.,0.));
#102107=DIRECTION('',(-0.190809912898503,0.,0.981627005099017));
#102108=DIRECTION('',(0.,-1.,0.));
#102109=DIRECTION('',(0.,-1.,0.));
#102110=DIRECTION('center_axis',(0.,-1.,0.));
#102111=DIRECTION('ref_axis',(0.,0.,-1.));
#102112=DIRECTION('',(-0.190809912898503,0.,0.981627005099017));
#102113=DIRECTION('',(-0.981627005099017,0.,-0.190809912898503));
#102114=DIRECTION('',(-0.981627005099017,0.,-0.190809912898503));
#102115=DIRECTION('center_axis',(-0.981627005099017,0.,-0.190809912898503));
#102116=DIRECTION('ref_axis',(-0.190809912898503,0.,0.981627005099017));
#102117=DIRECTION('',(0.,1.,0.));
#102118=DIRECTION('',(0.,1.,0.));
#102119=DIRECTION('center_axis',(0.,1.,0.));
#102120=DIRECTION('ref_axis',(1.,0.,0.));
#102121=DIRECTION('',(-0.190809912898503,0.,0.981627005099017));
#102122=DIRECTION('',(0.981627005099017,0.,0.190809912898503));
#102123=DIRECTION('',(-0.190809912898503,0.,0.981627005099017));
#102124=DIRECTION('',(0.981627005099017,0.,0.190809912898503));
#102125=DIRECTION('center_axis',(0.981627005099017,0.,0.190809912898503));
#102126=DIRECTION('ref_axis',(0.,-1.,0.));
#102127=DIRECTION('',(-0.190809912898503,0.,0.981627005099017));
#102128=DIRECTION('',(0.,-1.,0.));
#102129=DIRECTION('',(0.,-1.,0.));
#102130=DIRECTION('center_axis',(0.,-1.,0.));
#102131=DIRECTION('ref_axis',(0.,0.,-1.));
#102132=DIRECTION('',(-0.190809912898503,0.,0.981627005099017));
#102133=DIRECTION('',(-0.981627005099017,0.,-0.190809912898503));
#102134=DIRECTION('',(-0.981627005099017,0.,-0.190809912898503));
#102135=DIRECTION('center_axis',(-0.981627005099017,0.,-0.190809912898503));
#102136=DIRECTION('ref_axis',(-0.190809912898503,0.,0.981627005099017));
#102137=DIRECTION('',(0.,1.,0.));
#102138=DIRECTION('',(0.,1.,0.));
#102139=DIRECTION('center_axis',(0.,1.,0.));
#102140=DIRECTION('ref_axis',(1.,0.,0.));
#102141=DIRECTION('',(-0.190809912898503,0.,0.981627005099017));
#102142=DIRECTION('',(0.981627005099017,0.,0.190809912898503));
#102143=DIRECTION('',(-0.190809912898503,0.,0.981627005099017));
#102144=DIRECTION('',(0.981627005099017,0.,0.190809912898503));
#102145=DIRECTION('center_axis',(0.981627005099017,0.,0.190809912898503));
#102146=DIRECTION('ref_axis',(0.,-1.,0.));
#102147=DIRECTION('',(-0.190809912898503,0.,0.981627005099017));
#102148=DIRECTION('',(0.,-1.,0.));
#102149=DIRECTION('',(0.,-1.,0.));
#102150=DIRECTION('center_axis',(0.,-1.,0.));
#102151=DIRECTION('ref_axis',(0.,0.,-1.));
#102152=DIRECTION('',(-0.190809912898503,0.,0.981627005099017));
#102153=DIRECTION('',(-0.981627005099017,0.,-0.190809912898503));
#102154=DIRECTION('',(-0.981627005099017,0.,-0.190809912898503));
#102155=DIRECTION('center_axis',(-0.981627005099017,0.,-0.190809912898503));
#102156=DIRECTION('ref_axis',(-0.190809912898503,0.,0.981627005099017));
#102157=DIRECTION('',(0.,1.,0.));
#102158=DIRECTION('',(0.,1.,0.));
#102159=DIRECTION('center_axis',(0.,1.,0.));
#102160=DIRECTION('ref_axis',(1.,0.,0.));
#102161=DIRECTION('',(-0.190809912898503,0.,0.981627005099017));
#102162=DIRECTION('',(0.981627005099017,0.,0.190809912898503));
#102163=DIRECTION('',(-0.190809912898503,0.,0.981627005099017));
#102164=DIRECTION('',(0.981627005099017,0.,0.190809912898503));
#102165=DIRECTION('center_axis',(0.981627005099017,0.,0.190809912898503));
#102166=DIRECTION('ref_axis',(0.,-1.,0.));
#102167=DIRECTION('',(-0.190809912898503,0.,0.981627005099017));
#102168=DIRECTION('',(0.,-1.,0.));
#102169=DIRECTION('',(0.,-1.,0.));
#102170=DIRECTION('center_axis',(0.,-1.,0.));
#102171=DIRECTION('ref_axis',(0.,0.,-1.));
#102172=DIRECTION('',(-0.190809912898503,0.,0.981627005099017));
#102173=DIRECTION('',(-0.981627005099017,0.,-0.190809912898503));
#102174=DIRECTION('',(-0.981627005099017,0.,-0.190809912898503));
#102175=DIRECTION('center_axis',(-0.981627005099017,0.,-0.190809912898503));
#102176=DIRECTION('ref_axis',(-0.190809912898503,0.,0.981627005099017));
#102177=DIRECTION('',(0.,1.,0.));
#102178=DIRECTION('',(0.,1.,0.));
#102179=DIRECTION('center_axis',(0.,1.,0.));
#102180=DIRECTION('ref_axis',(1.,0.,0.));
#102181=DIRECTION('',(-0.190809912898503,0.,0.981627005099017));
#102182=DIRECTION('',(0.981627005099017,0.,0.190809912898503));
#102183=DIRECTION('',(-0.190809912898503,0.,0.981627005099017));
#102184=DIRECTION('',(0.981627005099017,0.,0.190809912898503));
#102185=DIRECTION('center_axis',(0.981627005099017,0.,0.190809912898503));
#102186=DIRECTION('ref_axis',(0.,-1.,0.));
#102187=DIRECTION('',(-0.190809912898503,0.,0.981627005099017));
#102188=DIRECTION('',(0.,-1.,0.));
#102189=DIRECTION('',(0.,-1.,0.));
#102190=DIRECTION('center_axis',(0.,-1.,0.));
#102191=DIRECTION('ref_axis',(0.,0.,-1.));
#102192=DIRECTION('',(-0.190809912898503,0.,0.981627005099017));
#102193=DIRECTION('',(-0.981627005099017,0.,-0.190809912898503));
#102194=DIRECTION('',(-0.981627005099017,0.,-0.190809912898503));
#102195=DIRECTION('center_axis',(-0.981627005099017,0.,-0.190809912898503));
#102196=DIRECTION('ref_axis',(-0.190809912898503,0.,0.981627005099017));
#102197=DIRECTION('',(0.,1.,0.));
#102198=DIRECTION('',(0.,1.,0.));
#102199=DIRECTION('center_axis',(0.,1.,0.));
#102200=DIRECTION('ref_axis',(1.,0.,0.));
#102201=DIRECTION('',(-0.190809912898503,0.,0.981627005099017));
#102202=DIRECTION('',(0.981627005099017,0.,0.190809912898503));
#102203=DIRECTION('',(-0.190809912898503,0.,0.981627005099017));
#102204=DIRECTION('',(0.981627005099017,0.,0.190809912898503));
#102205=DIRECTION('center_axis',(0.981627005099017,0.,0.190809912898503));
#102206=DIRECTION('ref_axis',(0.,-1.,0.));
#102207=DIRECTION('',(-0.190809912898503,0.,0.981627005099017));
#102208=DIRECTION('',(0.,-1.,0.));
#102209=DIRECTION('',(0.,-1.,0.));
#102210=DIRECTION('center_axis',(0.,-1.,0.));
#102211=DIRECTION('ref_axis',(0.,0.,-1.));
#102212=DIRECTION('',(-0.190809912898503,0.,0.981627005099017));
#102213=DIRECTION('',(-0.981627005099017,0.,-0.190809912898503));
#102214=DIRECTION('',(-0.981627005099017,0.,-0.190809912898503));
#102215=DIRECTION('center_axis',(-0.981627005099017,0.,-0.190809912898503));
#102216=DIRECTION('ref_axis',(-0.190809912898503,0.,0.981627005099017));
#102217=DIRECTION('',(0.,1.,0.));
#102218=DIRECTION('',(0.,1.,0.));
#102219=DIRECTION('center_axis',(0.,1.,0.));
#102220=DIRECTION('ref_axis',(1.,0.,0.));
#102221=DIRECTION('',(-0.190809912898503,0.,0.981627005099017));
#102222=DIRECTION('',(0.981627005099017,0.,0.190809912898503));
#102223=DIRECTION('',(-0.190809912898503,0.,0.981627005099017));
#102224=DIRECTION('',(0.981627005099017,0.,0.190809912898503));
#102225=DIRECTION('center_axis',(0.981627005099017,0.,0.190809912898503));
#102226=DIRECTION('ref_axis',(0.,-1.,0.));
#102227=DIRECTION('',(-0.190809912898503,0.,0.981627005099017));
#102228=DIRECTION('',(0.,-1.,0.));
#102229=DIRECTION('',(0.,-1.,0.));
#102230=DIRECTION('center_axis',(0.,-1.,0.));
#102231=DIRECTION('ref_axis',(0.,0.,-1.));
#102232=DIRECTION('',(-0.190809912898503,0.,0.981627005099017));
#102233=DIRECTION('',(-0.981627005099017,0.,-0.190809912898503));
#102234=DIRECTION('',(-0.981627005099017,0.,-0.190809912898503));
#102235=DIRECTION('center_axis',(-0.981627005099017,0.,-0.190809912898503));
#102236=DIRECTION('ref_axis',(-0.190809912898503,0.,0.981627005099017));
#102237=DIRECTION('',(0.,1.,0.));
#102238=DIRECTION('',(0.,1.,0.));
#102239=DIRECTION('center_axis',(0.,1.,0.));
#102240=DIRECTION('ref_axis',(1.,0.,0.));
#102241=DIRECTION('',(-0.190809912898503,0.,0.981627005099017));
#102242=DIRECTION('',(0.981627005099017,0.,0.190809912898503));
#102243=DIRECTION('',(-0.190809912898503,0.,0.981627005099017));
#102244=DIRECTION('',(0.981627005099017,0.,0.190809912898503));
#102245=DIRECTION('center_axis',(0.981627005099017,0.,0.190809912898503));
#102246=DIRECTION('ref_axis',(0.,-1.,0.));
#102247=DIRECTION('',(-0.190809912898503,0.,0.981627005099017));
#102248=DIRECTION('',(0.,-1.,0.));
#102249=DIRECTION('',(0.,-1.,0.));
#102250=DIRECTION('center_axis',(0.,-1.,0.));
#102251=DIRECTION('ref_axis',(0.,0.,-1.));
#102252=DIRECTION('',(-0.190809912898503,0.,0.981627005099017));
#102253=DIRECTION('',(-0.981627005099017,0.,-0.190809912898503));
#102254=DIRECTION('',(-0.981627005099017,0.,-0.190809912898503));
#102255=DIRECTION('center_axis',(-0.981627005099017,0.,-0.190809912898503));
#102256=DIRECTION('ref_axis',(-0.190809912898503,0.,0.981627005099017));
#102257=DIRECTION('',(0.,1.,0.));
#102258=DIRECTION('',(0.,1.,0.));
#102259=DIRECTION('center_axis',(0.,1.,0.));
#102260=DIRECTION('ref_axis',(1.,0.,0.));
#102261=DIRECTION('',(-0.190809912898503,0.,0.981627005099017));
#102262=DIRECTION('',(0.981627005099017,0.,0.190809912898503));
#102263=DIRECTION('',(-0.190809912898503,0.,0.981627005099017));
#102264=DIRECTION('',(0.981627005099017,0.,0.190809912898503));
#102265=DIRECTION('center_axis',(0.981627005099017,0.,0.190809912898503));
#102266=DIRECTION('ref_axis',(0.,-1.,0.));
#102267=DIRECTION('',(-0.190809912898503,0.,0.981627005099017));
#102268=DIRECTION('',(0.,-1.,0.));
#102269=DIRECTION('',(0.,-1.,0.));
#102270=DIRECTION('center_axis',(0.,-1.,0.));
#102271=DIRECTION('ref_axis',(0.,0.,-1.));
#102272=DIRECTION('',(-0.190809912898503,0.,0.981627005099017));
#102273=DIRECTION('',(-0.981627005099017,0.,-0.190809912898503));
#102274=DIRECTION('',(-0.981627005099017,0.,-0.190809912898503));
#102275=DIRECTION('center_axis',(-0.981627005099017,0.,-0.190809912898503));
#102276=DIRECTION('ref_axis',(-0.190809912898503,0.,0.981627005099017));
#102277=DIRECTION('',(0.,1.,0.));
#102278=DIRECTION('',(0.,1.,0.));
#102279=DIRECTION('center_axis',(0.,1.,0.));
#102280=DIRECTION('ref_axis',(1.,0.,0.));
#102281=DIRECTION('',(-0.190809912898503,0.,0.981627005099017));
#102282=DIRECTION('',(0.981627005099017,0.,0.190809912898503));
#102283=DIRECTION('',(-0.190809912898503,0.,0.981627005099017));
#102284=DIRECTION('',(0.981627005099017,0.,0.190809912898503));
#102285=DIRECTION('center_axis',(0.981627005099017,0.,0.190809912898503));
#102286=DIRECTION('ref_axis',(0.,-1.,0.));
#102287=DIRECTION('',(-0.190809912898503,0.,0.981627005099017));
#102288=DIRECTION('',(0.,-1.,0.));
#102289=DIRECTION('',(0.,-1.,0.));
#102290=DIRECTION('center_axis',(0.,-1.,0.));
#102291=DIRECTION('ref_axis',(0.,0.,-1.));
#102292=DIRECTION('',(-0.190809912898503,0.,0.981627005099017));
#102293=DIRECTION('',(-0.981627005099017,0.,-0.190809912898503));
#102294=DIRECTION('',(-0.981627005099017,0.,-0.190809912898503));
#102295=DIRECTION('center_axis',(-0.981627005099017,0.,-0.190809912898503));
#102296=DIRECTION('ref_axis',(-0.190809912898503,0.,0.981627005099017));
#102297=DIRECTION('',(0.,1.,0.));
#102298=DIRECTION('',(0.,1.,0.));
#102299=DIRECTION('center_axis',(0.,1.,0.));
#102300=DIRECTION('ref_axis',(1.,0.,0.));
#102301=DIRECTION('',(-0.190809912898503,0.,0.981627005099017));
#102302=DIRECTION('',(0.981627005099017,0.,0.190809912898503));
#102303=DIRECTION('',(-0.190809912898503,0.,0.981627005099017));
#102304=DIRECTION('',(0.981627005099017,0.,0.190809912898503));
#102305=DIRECTION('center_axis',(0.981627005099017,0.,0.190809912898503));
#102306=DIRECTION('ref_axis',(0.,-1.,0.));
#102307=DIRECTION('',(-0.190809912898503,0.,0.981627005099017));
#102308=DIRECTION('',(0.,-1.,0.));
#102309=DIRECTION('',(0.,-1.,0.));
#102310=DIRECTION('center_axis',(0.,-1.,0.));
#102311=DIRECTION('ref_axis',(0.,0.,-1.));
#102312=DIRECTION('',(-0.190809912898503,0.,0.981627005099017));
#102313=DIRECTION('',(-0.981627005099017,0.,-0.190809912898503));
#102314=DIRECTION('',(-0.981627005099017,0.,-0.190809912898503));
#102315=DIRECTION('center_axis',(-0.981627005099017,0.,-0.190809912898503));
#102316=DIRECTION('ref_axis',(-0.190809912898503,0.,0.981627005099017));
#102317=DIRECTION('',(0.,1.,0.));
#102318=DIRECTION('',(0.,1.,0.));
#102319=DIRECTION('center_axis',(0.,1.,0.));
#102320=DIRECTION('ref_axis',(1.,0.,0.));
#102321=DIRECTION('',(-0.190809912898503,0.,0.981627005099017));
#102322=DIRECTION('',(0.981627005099017,0.,0.190809912898503));
#102323=DIRECTION('',(-0.190809912898503,0.,0.981627005099017));
#102324=DIRECTION('',(0.981627005099017,0.,0.190809912898503));
#102325=DIRECTION('center_axis',(0.981627005099017,0.,0.190809912898503));
#102326=DIRECTION('ref_axis',(0.,-1.,0.));
#102327=DIRECTION('',(-0.190809912898503,0.,0.981627005099017));
#102328=DIRECTION('',(0.,-1.,0.));
#102329=DIRECTION('',(0.,-1.,0.));
#102330=DIRECTION('center_axis',(0.,-1.,0.));
#102331=DIRECTION('ref_axis',(0.,0.,-1.));
#102332=DIRECTION('',(-0.190809912898503,0.,0.981627005099017));
#102333=DIRECTION('',(-0.981627005099017,0.,-0.190809912898503));
#102334=DIRECTION('',(-0.981627005099017,0.,-0.190809912898503));
#102335=DIRECTION('center_axis',(-0.981627005099017,0.,-0.190809912898503));
#102336=DIRECTION('ref_axis',(-0.190809912898503,0.,0.981627005099017));
#102337=DIRECTION('',(0.,1.,0.));
#102338=DIRECTION('',(0.,1.,0.));
#102339=DIRECTION('center_axis',(0.,1.,0.));
#102340=DIRECTION('ref_axis',(1.,0.,0.));
#102341=DIRECTION('',(-0.190809912898503,0.,0.981627005099017));
#102342=DIRECTION('',(0.981627005099017,0.,0.190809912898503));
#102343=DIRECTION('',(-0.190809912898503,0.,0.981627005099017));
#102344=DIRECTION('',(0.981627005099017,0.,0.190809912898503));
#102345=DIRECTION('center_axis',(0.981627005099017,0.,0.190809912898503));
#102346=DIRECTION('ref_axis',(0.,-1.,0.));
#102347=DIRECTION('',(-0.190809912898503,0.,0.981627005099017));
#102348=DIRECTION('',(0.,-1.,0.));
#102349=DIRECTION('',(0.,-1.,0.));
#102350=DIRECTION('center_axis',(0.,-1.,0.));
#102351=DIRECTION('ref_axis',(0.,0.,-1.));
#102352=DIRECTION('',(-0.190809912898503,0.,0.981627005099017));
#102353=DIRECTION('',(-0.981627005099017,0.,-0.190809912898503));
#102354=DIRECTION('',(-0.981627005099017,0.,-0.190809912898503));
#102355=DIRECTION('center_axis',(-0.981627005099017,0.,-0.190809912898503));
#102356=DIRECTION('ref_axis',(-0.190809912898503,0.,0.981627005099017));
#102357=DIRECTION('',(0.,1.,0.));
#102358=DIRECTION('',(0.,1.,0.));
#102359=DIRECTION('center_axis',(0.,1.,0.));
#102360=DIRECTION('ref_axis',(1.,0.,0.));
#102361=DIRECTION('',(-0.190809912898503,0.,0.981627005099017));
#102362=DIRECTION('',(0.981627005099017,0.,0.190809912898503));
#102363=DIRECTION('',(-0.190809912898503,0.,0.981627005099017));
#102364=DIRECTION('',(0.981627005099017,0.,0.190809912898503));
#102365=DIRECTION('center_axis',(0.981627005099017,0.,0.190809912898503));
#102366=DIRECTION('ref_axis',(0.,-1.,0.));
#102367=DIRECTION('',(-0.190809912898503,0.,0.981627005099017));
#102368=DIRECTION('',(0.,-1.,0.));
#102369=DIRECTION('',(0.,-1.,0.));
#102370=DIRECTION('center_axis',(0.,-1.,0.));
#102371=DIRECTION('ref_axis',(0.,0.,-1.));
#102372=DIRECTION('',(-0.190809912898503,0.,0.981627005099017));
#102373=DIRECTION('',(-0.981627005099017,0.,-0.190809912898503));
#102374=DIRECTION('',(-0.981627005099017,0.,-0.190809912898503));
#102375=DIRECTION('center_axis',(-0.981627005099017,0.,-0.190809912898503));
#102376=DIRECTION('ref_axis',(-0.190809912898503,0.,0.981627005099017));
#102377=DIRECTION('',(0.,1.,0.));
#102378=DIRECTION('',(0.,1.,0.));
#102379=DIRECTION('center_axis',(0.,1.,0.));
#102380=DIRECTION('ref_axis',(1.,0.,0.));
#102381=DIRECTION('',(-0.190809912898503,0.,0.981627005099017));
#102382=DIRECTION('',(0.981627005099017,0.,0.190809912898503));
#102383=DIRECTION('',(-0.190809912898503,0.,0.981627005099017));
#102384=DIRECTION('',(0.981627005099017,0.,0.190809912898503));
#102385=DIRECTION('center_axis',(0.981627005099017,0.,0.190809912898503));
#102386=DIRECTION('ref_axis',(0.,-1.,0.));
#102387=DIRECTION('',(-0.190809912898503,0.,0.981627005099017));
#102388=DIRECTION('',(0.,-1.,0.));
#102389=DIRECTION('',(0.,-1.,0.));
#102390=DIRECTION('center_axis',(0.,-1.,0.));
#102391=DIRECTION('ref_axis',(0.,0.,-1.));
#102392=DIRECTION('',(-0.190809912898503,0.,0.981627005099017));
#102393=DIRECTION('',(-0.981627005099017,0.,-0.190809912898503));
#102394=DIRECTION('',(-0.981627005099017,0.,-0.190809912898503));
#102395=DIRECTION('center_axis',(-0.981627005099017,0.,-0.190809912898503));
#102396=DIRECTION('ref_axis',(-0.190809912898503,0.,0.981627005099017));
#102397=DIRECTION('',(0.,1.,0.));
#102398=DIRECTION('',(0.,1.,0.));
#102399=DIRECTION('center_axis',(0.,1.,0.));
#102400=DIRECTION('ref_axis',(1.,0.,0.));
#102401=DIRECTION('',(-0.190809912898503,0.,0.981627005099017));
#102402=DIRECTION('',(0.981627005099017,0.,0.190809912898503));
#102403=DIRECTION('',(-0.190809912898503,0.,0.981627005099017));
#102404=DIRECTION('',(0.981627005099017,0.,0.190809912898503));
#102405=DIRECTION('center_axis',(0.981627005099017,0.,0.190809912898503));
#102406=DIRECTION('ref_axis',(0.,-1.,0.));
#102407=DIRECTION('',(-0.190809912898503,0.,0.981627005099017));
#102408=DIRECTION('',(0.,-1.,0.));
#102409=DIRECTION('',(0.,-1.,0.));
#102410=DIRECTION('center_axis',(0.,-1.,0.));
#102411=DIRECTION('ref_axis',(0.,0.,-1.));
#102412=DIRECTION('',(-0.190809912898503,0.,0.981627005099017));
#102413=DIRECTION('',(-0.981627005099017,0.,-0.190809912898503));
#102414=DIRECTION('',(-0.981627005099017,0.,-0.190809912898503));
#102415=DIRECTION('center_axis',(-0.981627005099017,0.,-0.190809912898503));
#102416=DIRECTION('ref_axis',(-0.190809912898503,0.,0.981627005099017));
#102417=DIRECTION('',(0.,1.,0.));
#102418=DIRECTION('',(0.,1.,0.));
#102419=DIRECTION('center_axis',(0.,1.,0.));
#102420=DIRECTION('ref_axis',(1.,0.,0.));
#102421=DIRECTION('',(-0.190809912898503,0.,0.981627005099017));
#102422=DIRECTION('',(0.981627005099017,0.,0.190809912898503));
#102423=DIRECTION('',(-0.190809912898503,0.,0.981627005099017));
#102424=DIRECTION('',(0.981627005099017,0.,0.190809912898503));
#102425=DIRECTION('center_axis',(0.981627005099017,0.,0.190809912898503));
#102426=DIRECTION('ref_axis',(0.,-1.,0.));
#102427=DIRECTION('',(-0.190809912898503,0.,0.981627005099017));
#102428=DIRECTION('',(0.,-1.,0.));
#102429=DIRECTION('',(0.,-1.,0.));
#102430=DIRECTION('center_axis',(0.,-1.,0.));
#102431=DIRECTION('ref_axis',(0.,0.,-1.));
#102432=DIRECTION('',(-0.190809912898503,0.,0.981627005099017));
#102433=DIRECTION('',(-0.981627005099017,0.,-0.190809912898503));
#102434=DIRECTION('',(-0.981627005099017,0.,-0.190809912898503));
#102435=DIRECTION('center_axis',(-0.981627005099017,0.,-0.190809912898503));
#102436=DIRECTION('ref_axis',(-0.190809912898503,0.,0.981627005099017));
#102437=DIRECTION('',(0.,1.,0.));
#102438=DIRECTION('',(0.,1.,0.));
#102439=DIRECTION('center_axis',(0.,1.,0.));
#102440=DIRECTION('ref_axis',(1.,0.,0.));
#102441=DIRECTION('',(-0.190809912898503,0.,0.981627005099017));
#102442=DIRECTION('',(0.981627005099017,0.,0.190809912898503));
#102443=DIRECTION('',(-0.190809912898503,0.,0.981627005099017));
#102444=DIRECTION('',(0.981627005099017,0.,0.190809912898503));
#102445=DIRECTION('center_axis',(0.981627005099017,0.,0.190809912898503));
#102446=DIRECTION('ref_axis',(0.,-1.,0.));
#102447=DIRECTION('',(-0.190809912898503,0.,0.981627005099017));
#102448=DIRECTION('',(0.,-1.,0.));
#102449=DIRECTION('',(0.,-1.,0.));
#102450=DIRECTION('center_axis',(0.,-1.,0.));
#102451=DIRECTION('ref_axis',(0.,0.,-1.));
#102452=DIRECTION('',(-0.190809912898503,0.,0.981627005099017));
#102453=DIRECTION('',(-0.981627005099017,0.,-0.190809912898503));
#102454=DIRECTION('',(-0.981627005099017,0.,-0.190809912898503));
#102455=DIRECTION('center_axis',(-0.981627005099017,0.,-0.190809912898503));
#102456=DIRECTION('ref_axis',(-0.190809912898503,0.,0.981627005099017));
#102457=DIRECTION('',(0.,1.,0.));
#102458=DIRECTION('',(0.,1.,0.));
#102459=DIRECTION('center_axis',(0.,1.,0.));
#102460=DIRECTION('ref_axis',(1.,0.,0.));
#102461=DIRECTION('',(-0.190809912898503,0.,0.981627005099017));
#102462=DIRECTION('',(0.981627005099017,0.,0.190809912898503));
#102463=DIRECTION('',(-0.190809912898503,0.,0.981627005099017));
#102464=DIRECTION('',(0.981627005099017,0.,0.190809912898503));
#102465=DIRECTION('center_axis',(0.981627005099017,0.,0.190809912898503));
#102466=DIRECTION('ref_axis',(0.,-1.,0.));
#102467=DIRECTION('',(-0.190809912898503,0.,0.981627005099017));
#102468=DIRECTION('',(0.,-1.,0.));
#102469=DIRECTION('',(0.,-1.,0.));
#102470=DIRECTION('center_axis',(0.,-1.,0.));
#102471=DIRECTION('ref_axis',(0.,0.,-1.));
#102472=DIRECTION('',(-0.190809912898503,0.,0.981627005099017));
#102473=DIRECTION('',(-0.981627005099017,0.,-0.190809912898503));
#102474=DIRECTION('',(-0.981627005099017,0.,-0.190809912898503));
#102475=DIRECTION('center_axis',(-0.981627005099017,0.,-0.190809912898503));
#102476=DIRECTION('ref_axis',(-0.190809912898503,0.,0.981627005099017));
#102477=DIRECTION('',(0.,1.,0.));
#102478=DIRECTION('',(0.,1.,0.));
#102479=DIRECTION('center_axis',(0.,1.,0.));
#102480=DIRECTION('ref_axis',(1.,0.,0.));
#102481=DIRECTION('',(-0.190809912898503,0.,0.981627005099017));
#102482=DIRECTION('',(0.981627005099017,0.,0.190809912898503));
#102483=DIRECTION('',(-0.190809912898503,0.,0.981627005099017));
#102484=DIRECTION('',(0.981627005099017,0.,0.190809912898503));
#102485=DIRECTION('center_axis',(0.981627005099017,0.,0.190809912898503));
#102486=DIRECTION('ref_axis',(0.,-1.,0.));
#102487=DIRECTION('',(-0.190809912898503,0.,0.981627005099017));
#102488=DIRECTION('',(0.,-1.,0.));
#102489=DIRECTION('',(0.,-1.,0.));
#102490=DIRECTION('center_axis',(0.,-1.,0.));
#102491=DIRECTION('ref_axis',(0.,0.,-1.));
#102492=DIRECTION('',(-0.190809912898503,0.,0.981627005099017));
#102493=DIRECTION('',(-0.981627005099017,0.,-0.190809912898503));
#102494=DIRECTION('',(-0.981627005099017,0.,-0.190809912898503));
#102495=DIRECTION('center_axis',(-0.981627005099017,0.,-0.190809912898503));
#102496=DIRECTION('ref_axis',(-0.190809912898503,0.,0.981627005099017));
#102497=DIRECTION('',(0.,1.,0.));
#102498=DIRECTION('',(0.,1.,0.));
#102499=DIRECTION('center_axis',(0.,1.,0.));
#102500=DIRECTION('ref_axis',(1.,0.,0.));
#102501=DIRECTION('',(-0.190809912898503,0.,0.981627005099017));
#102502=DIRECTION('',(0.981627005099017,0.,0.190809912898503));
#102503=DIRECTION('',(-0.190809912898503,0.,0.981627005099017));
#102504=DIRECTION('',(0.981627005099017,0.,0.190809912898503));
#102505=DIRECTION('center_axis',(0.981627005099017,0.,0.190809912898503));
#102506=DIRECTION('ref_axis',(0.,-1.,0.));
#102507=DIRECTION('',(-0.190809912898503,0.,0.981627005099017));
#102508=DIRECTION('',(0.,-1.,0.));
#102509=DIRECTION('',(0.,-1.,0.));
#102510=DIRECTION('center_axis',(0.,-1.,0.));
#102511=DIRECTION('ref_axis',(0.,0.,-1.));
#102512=DIRECTION('',(-0.190809912898503,0.,0.981627005099017));
#102513=DIRECTION('',(-0.981627005099017,0.,-0.190809912898503));
#102514=DIRECTION('',(-0.981627005099017,0.,-0.190809912898503));
#102515=DIRECTION('center_axis',(-0.981627005099017,0.,-0.190809912898503));
#102516=DIRECTION('ref_axis',(-0.190809912898503,0.,0.981627005099017));
#102517=DIRECTION('',(0.,1.,0.));
#102518=DIRECTION('',(0.,1.,0.));
#102519=DIRECTION('center_axis',(0.,1.,0.));
#102520=DIRECTION('ref_axis',(1.,0.,0.));
#102521=DIRECTION('',(-0.190809912898503,0.,0.981627005099017));
#102522=DIRECTION('',(0.981627005099017,0.,0.190809912898503));
#102523=DIRECTION('',(-0.190809912898503,0.,0.981627005099017));
#102524=DIRECTION('',(0.981627005099017,0.,0.190809912898503));
#102525=DIRECTION('center_axis',(0.981627005099017,0.,0.190809912898503));
#102526=DIRECTION('ref_axis',(0.,-1.,0.));
#102527=DIRECTION('',(-0.190809912898503,0.,0.981627005099017));
#102528=DIRECTION('',(0.,-1.,0.));
#102529=DIRECTION('',(0.,-1.,0.));
#102530=DIRECTION('center_axis',(0.,-1.,0.));
#102531=DIRECTION('ref_axis',(0.,0.,-1.));
#102532=DIRECTION('',(-0.190809912898503,0.,0.981627005099017));
#102533=DIRECTION('',(-0.981627005099017,0.,-0.190809912898503));
#102534=DIRECTION('',(-0.981627005099017,0.,-0.190809912898503));
#102535=DIRECTION('center_axis',(-0.981627005099017,0.,-0.190809912898503));
#102536=DIRECTION('ref_axis',(-0.190809912898503,0.,0.981627005099017));
#102537=DIRECTION('',(0.,1.,0.));
#102538=DIRECTION('',(0.,1.,0.));
#102539=DIRECTION('center_axis',(0.,1.,0.));
#102540=DIRECTION('ref_axis',(1.,0.,0.));
#102541=DIRECTION('',(-0.190809912898503,0.,0.981627005099017));
#102542=DIRECTION('',(0.981627005099017,0.,0.190809912898503));
#102543=DIRECTION('',(-0.190809912898503,0.,0.981627005099017));
#102544=DIRECTION('',(0.981627005099017,0.,0.190809912898503));
#102545=DIRECTION('center_axis',(0.981627005099017,0.,0.190809912898503));
#102546=DIRECTION('ref_axis',(0.,-1.,0.));
#102547=DIRECTION('',(-0.190809912898503,0.,0.981627005099017));
#102548=DIRECTION('',(0.,-1.,0.));
#102549=DIRECTION('',(0.,-1.,0.));
#102550=DIRECTION('center_axis',(0.,-1.,0.));
#102551=DIRECTION('ref_axis',(0.,0.,-1.));
#102552=DIRECTION('',(-0.190809912898503,0.,0.981627005099017));
#102553=DIRECTION('',(-0.981627005099017,0.,-0.190809912898503));
#102554=DIRECTION('',(-0.981627005099017,0.,-0.190809912898503));
#102555=DIRECTION('center_axis',(-0.981627005099017,0.,-0.190809912898503));
#102556=DIRECTION('ref_axis',(-0.190809912898503,0.,0.981627005099017));
#102557=DIRECTION('',(0.,1.,0.));
#102558=DIRECTION('',(0.,1.,0.));
#102559=DIRECTION('center_axis',(0.,1.,0.));
#102560=DIRECTION('ref_axis',(1.,0.,0.));
#102561=DIRECTION('',(-0.190809912898503,0.,0.981627005099017));
#102562=DIRECTION('',(0.981627005099017,0.,0.190809912898503));
#102563=DIRECTION('',(-0.190809912898503,0.,0.981627005099017));
#102564=DIRECTION('',(0.981627005099017,0.,0.190809912898503));
#102565=DIRECTION('center_axis',(0.981627005099017,0.,0.190809912898503));
#102566=DIRECTION('ref_axis',(0.,-1.,0.));
#102567=DIRECTION('',(-0.190809912898503,0.,0.981627005099017));
#102568=DIRECTION('',(0.,-1.,0.));
#102569=DIRECTION('',(0.,-1.,0.));
#102570=DIRECTION('center_axis',(0.,-1.,0.));
#102571=DIRECTION('ref_axis',(0.,0.,-1.));
#102572=DIRECTION('',(-0.190809912898503,0.,0.981627005099017));
#102573=DIRECTION('',(-0.981627005099017,0.,-0.190809912898503));
#102574=DIRECTION('',(-0.981627005099017,0.,-0.190809912898503));
#102575=DIRECTION('center_axis',(-0.981627005099017,0.,-0.190809912898503));
#102576=DIRECTION('ref_axis',(-0.190809912898503,0.,0.981627005099017));
#102577=DIRECTION('',(0.,1.,0.));
#102578=DIRECTION('',(0.,1.,0.));
#102579=DIRECTION('center_axis',(0.,1.,0.));
#102580=DIRECTION('ref_axis',(1.,0.,0.));
#102581=DIRECTION('',(-0.190809912898503,0.,0.981627005099017));
#102582=DIRECTION('',(0.981627005099017,0.,0.190809912898503));
#102583=DIRECTION('',(-0.190809912898503,0.,0.981627005099017));
#102584=DIRECTION('',(0.981627005099017,0.,0.190809912898503));
#102585=DIRECTION('center_axis',(0.981627005099017,0.,0.190809912898503));
#102586=DIRECTION('ref_axis',(0.,-1.,0.));
#102587=DIRECTION('',(-0.190809912898503,0.,0.981627005099017));
#102588=DIRECTION('',(0.,-1.,0.));
#102589=DIRECTION('',(0.,-1.,0.));
#102590=DIRECTION('center_axis',(0.,-1.,0.));
#102591=DIRECTION('ref_axis',(0.,0.,-1.));
#102592=DIRECTION('',(-0.190809912898503,0.,0.981627005099017));
#102593=DIRECTION('',(-0.981627005099017,0.,-0.190809912898503));
#102594=DIRECTION('',(-0.981627005099017,0.,-0.190809912898503));
#102595=DIRECTION('center_axis',(-0.981627005099017,0.,-0.190809912898503));
#102596=DIRECTION('ref_axis',(-0.190809912898503,0.,0.981627005099017));
#102597=DIRECTION('',(0.,1.,0.));
#102598=DIRECTION('',(0.,1.,0.));
#102599=DIRECTION('center_axis',(0.,1.,0.));
#102600=DIRECTION('ref_axis',(1.,0.,0.));
#102601=DIRECTION('',(-0.190809912898503,0.,0.981627005099017));
#102602=DIRECTION('',(0.981627005099017,0.,0.190809912898503));
#102603=DIRECTION('',(-0.190809912898503,0.,0.981627005099017));
#102604=DIRECTION('',(0.981627005099017,0.,0.190809912898503));
#102605=DIRECTION('center_axis',(0.981627005099017,0.,0.190809912898503));
#102606=DIRECTION('ref_axis',(0.,-1.,0.));
#102607=DIRECTION('',(-0.190809912898503,0.,0.981627005099017));
#102608=DIRECTION('',(0.,-1.,0.));
#102609=DIRECTION('',(0.,-1.,0.));
#102610=DIRECTION('center_axis',(0.,-1.,0.));
#102611=DIRECTION('ref_axis',(0.,0.,-1.));
#102612=DIRECTION('',(-0.190809912898503,0.,0.981627005099017));
#102613=DIRECTION('',(-0.981627005099017,0.,-0.190809912898503));
#102614=DIRECTION('',(-0.981627005099017,0.,-0.190809912898503));
#102615=DIRECTION('center_axis',(-0.981627005099017,0.,-0.190809912898503));
#102616=DIRECTION('ref_axis',(-0.190809912898503,0.,0.981627005099017));
#102617=DIRECTION('',(0.,1.,0.));
#102618=DIRECTION('',(0.,1.,0.));
#102619=DIRECTION('center_axis',(0.,1.,0.));
#102620=DIRECTION('ref_axis',(1.,0.,0.));
#102621=DIRECTION('',(-0.190809912898503,0.,0.981627005099017));
#102622=DIRECTION('',(0.981627005099017,0.,0.190809912898503));
#102623=DIRECTION('',(-0.190809912898503,0.,0.981627005099017));
#102624=DIRECTION('',(0.981627005099017,0.,0.190809912898503));
#102625=DIRECTION('center_axis',(0.981627005099017,0.,0.190809912898503));
#102626=DIRECTION('ref_axis',(0.,-1.,0.));
#102627=DIRECTION('',(-0.190809912898503,0.,0.981627005099017));
#102628=DIRECTION('',(0.,-1.,0.));
#102629=DIRECTION('',(0.,-1.,0.));
#102630=DIRECTION('center_axis',(0.,-1.,0.));
#102631=DIRECTION('ref_axis',(0.,0.,-1.));
#102632=DIRECTION('',(-0.190809912898503,0.,0.981627005099017));
#102633=DIRECTION('',(-0.981627005099017,0.,-0.190809912898503));
#102634=DIRECTION('',(-0.981627005099017,0.,-0.190809912898503));
#102635=DIRECTION('center_axis',(-0.981627005099017,0.,-0.190809912898503));
#102636=DIRECTION('ref_axis',(-0.190809912898503,0.,0.981627005099017));
#102637=DIRECTION('',(0.,1.,0.));
#102638=DIRECTION('',(0.,1.,0.));
#102639=DIRECTION('center_axis',(0.,1.,0.));
#102640=DIRECTION('ref_axis',(1.,0.,0.));
#102641=DIRECTION('',(-0.190809912898503,0.,0.981627005099017));
#102642=DIRECTION('',(0.981627005099017,0.,0.190809912898503));
#102643=DIRECTION('',(-0.190809912898503,0.,0.981627005099017));
#102644=DIRECTION('',(0.981627005099017,0.,0.190809912898503));
#102645=DIRECTION('center_axis',(0.981627005099017,0.,0.190809912898503));
#102646=DIRECTION('ref_axis',(0.,-1.,0.));
#102647=DIRECTION('',(-0.190809912898503,0.,0.981627005099017));
#102648=DIRECTION('',(0.,-1.,0.));
#102649=DIRECTION('',(0.,-1.,0.));
#102650=DIRECTION('center_axis',(0.,-1.,0.));
#102651=DIRECTION('ref_axis',(0.,0.,-1.));
#102652=DIRECTION('',(-0.190809912898503,0.,0.981627005099017));
#102653=DIRECTION('',(-0.981627005099017,0.,-0.190809912898503));
#102654=DIRECTION('',(-0.981627005099017,0.,-0.190809912898503));
#102655=DIRECTION('center_axis',(-0.981627005099017,0.,-0.190809912898503));
#102656=DIRECTION('ref_axis',(-0.190809912898503,0.,0.981627005099017));
#102657=DIRECTION('',(0.,1.,0.));
#102658=DIRECTION('',(0.,1.,0.));
#102659=DIRECTION('center_axis',(0.,1.,0.));
#102660=DIRECTION('ref_axis',(1.,0.,0.));
#102661=DIRECTION('',(-0.190809912898503,0.,0.981627005099017));
#102662=DIRECTION('',(0.981627005099017,0.,0.190809912898503));
#102663=DIRECTION('',(-0.190809912898503,0.,0.981627005099017));
#102664=DIRECTION('',(0.981627005099017,0.,0.190809912898503));
#102665=DIRECTION('center_axis',(0.981627005099017,0.,0.190809912898503));
#102666=DIRECTION('ref_axis',(0.,-1.,0.));
#102667=DIRECTION('',(-0.190809912898503,0.,0.981627005099017));
#102668=DIRECTION('',(0.,-1.,0.));
#102669=DIRECTION('',(0.,-1.,0.));
#102670=DIRECTION('center_axis',(0.,-1.,0.));
#102671=DIRECTION('ref_axis',(0.,0.,-1.));
#102672=DIRECTION('',(-0.190809912898503,0.,0.981627005099017));
#102673=DIRECTION('',(-0.981627005099017,0.,-0.190809912898503));
#102674=DIRECTION('',(-0.981627005099017,0.,-0.190809912898503));
#102675=DIRECTION('center_axis',(-0.981627005099017,0.,-0.190809912898503));
#102676=DIRECTION('ref_axis',(-0.190809912898503,0.,0.981627005099017));
#102677=DIRECTION('',(0.,1.,0.));
#102678=DIRECTION('',(0.,1.,0.));
#102679=DIRECTION('center_axis',(0.,1.,0.));
#102680=DIRECTION('ref_axis',(1.,0.,0.));
#102681=DIRECTION('',(-0.190809912898503,0.,0.981627005099017));
#102682=DIRECTION('',(0.981627005099017,0.,0.190809912898503));
#102683=DIRECTION('',(-0.190809912898503,0.,0.981627005099017));
#102684=DIRECTION('',(0.981627005099017,0.,0.190809912898503));
#102685=DIRECTION('center_axis',(0.981627005099017,0.,0.190809912898503));
#102686=DIRECTION('ref_axis',(0.,-1.,0.));
#102687=DIRECTION('',(-0.190809912898503,0.,0.981627005099017));
#102688=DIRECTION('',(0.,-1.,0.));
#102689=DIRECTION('',(0.,-1.,0.));
#102690=DIRECTION('center_axis',(0.,-1.,0.));
#102691=DIRECTION('ref_axis',(0.,0.,-1.));
#102692=DIRECTION('',(-0.190809912898503,0.,0.981627005099017));
#102693=DIRECTION('',(-0.981627005099017,0.,-0.190809912898503));
#102694=DIRECTION('',(-0.981627005099017,0.,-0.190809912898503));
#102695=DIRECTION('center_axis',(-0.981627005099017,0.,-0.190809912898503));
#102696=DIRECTION('ref_axis',(-0.190809912898503,0.,0.981627005099017));
#102697=DIRECTION('',(0.,1.,0.));
#102698=DIRECTION('',(0.,1.,0.));
#102699=DIRECTION('center_axis',(0.,1.,0.));
#102700=DIRECTION('ref_axis',(1.,0.,0.));
#102701=DIRECTION('',(-0.190809912898503,0.,0.981627005099017));
#102702=DIRECTION('',(0.981627005099017,0.,0.190809912898503));
#102703=DIRECTION('',(-0.190809912898503,0.,0.981627005099017));
#102704=DIRECTION('',(0.981627005099017,0.,0.190809912898503));
#102705=DIRECTION('center_axis',(0.981627005099017,0.,0.190809912898503));
#102706=DIRECTION('ref_axis',(0.,-1.,0.));
#102707=DIRECTION('',(-0.190809912898503,0.,0.981627005099017));
#102708=DIRECTION('',(0.,-1.,0.));
#102709=DIRECTION('',(0.,-1.,0.));
#102710=DIRECTION('center_axis',(0.,-1.,0.));
#102711=DIRECTION('ref_axis',(0.,0.,-1.));
#102712=DIRECTION('',(-0.190809912898503,0.,0.981627005099017));
#102713=DIRECTION('',(-0.981627005099017,0.,-0.190809912898503));
#102714=DIRECTION('',(-0.981627005099017,0.,-0.190809912898503));
#102715=DIRECTION('center_axis',(-0.981627005099017,0.,-0.190809912898503));
#102716=DIRECTION('ref_axis',(-0.190809912898503,0.,0.981627005099017));
#102717=DIRECTION('',(0.,1.,0.));
#102718=DIRECTION('',(0.,1.,0.));
#102719=DIRECTION('center_axis',(0.,1.,0.));
#102720=DIRECTION('ref_axis',(1.,0.,0.));
#102721=DIRECTION('',(-0.190809912898503,0.,0.981627005099017));
#102722=DIRECTION('',(0.981627005099017,0.,0.190809912898503));
#102723=DIRECTION('',(-0.190809912898503,0.,0.981627005099017));
#102724=DIRECTION('',(0.981627005099017,0.,0.190809912898503));
#102725=DIRECTION('center_axis',(0.981627005099017,0.,0.190809912898503));
#102726=DIRECTION('ref_axis',(0.,-1.,0.));
#102727=DIRECTION('',(-0.190809912898503,0.,0.981627005099017));
#102728=DIRECTION('',(0.,-1.,0.));
#102729=DIRECTION('',(0.,-1.,0.));
#102730=DIRECTION('center_axis',(0.,-1.,0.));
#102731=DIRECTION('ref_axis',(0.,0.,-1.));
#102732=DIRECTION('',(-0.190809912898503,0.,0.981627005099017));
#102733=DIRECTION('',(-0.981627005099017,0.,-0.190809912898503));
#102734=DIRECTION('',(-0.981627005099017,0.,-0.190809912898503));
#102735=DIRECTION('center_axis',(-0.981627005099017,0.,-0.190809912898503));
#102736=DIRECTION('ref_axis',(-0.190809912898503,0.,0.981627005099017));
#102737=DIRECTION('',(0.,1.,0.));
#102738=DIRECTION('',(0.,1.,0.));
#102739=DIRECTION('center_axis',(0.,1.,0.));
#102740=DIRECTION('ref_axis',(1.,0.,0.));
#102741=DIRECTION('',(-0.190809912898503,0.,0.981627005099017));
#102742=DIRECTION('',(0.981627005099017,0.,0.190809912898503));
#102743=DIRECTION('',(-0.190809912898503,0.,0.981627005099017));
#102744=DIRECTION('',(0.981627005099017,0.,0.190809912898503));
#102745=DIRECTION('center_axis',(0.981627005099017,0.,0.190809912898503));
#102746=DIRECTION('ref_axis',(0.,-1.,0.));
#102747=DIRECTION('',(-0.190809912898503,0.,0.981627005099017));
#102748=DIRECTION('',(0.,-1.,0.));
#102749=DIRECTION('',(0.,-1.,0.));
#102750=DIRECTION('center_axis',(0.,-1.,0.));
#102751=DIRECTION('ref_axis',(0.,0.,-1.));
#102752=DIRECTION('',(-0.190809912898503,0.,0.981627005099017));
#102753=DIRECTION('',(-0.981627005099017,0.,-0.190809912898503));
#102754=DIRECTION('',(-0.981627005099017,0.,-0.190809912898503));
#102755=DIRECTION('center_axis',(-0.981627005099017,0.,-0.190809912898503));
#102756=DIRECTION('ref_axis',(-0.190809912898503,0.,0.981627005099017));
#102757=DIRECTION('',(0.,1.,0.));
#102758=DIRECTION('',(0.,1.,0.));
#102759=DIRECTION('center_axis',(0.,1.,0.));
#102760=DIRECTION('ref_axis',(1.,0.,0.));
#102761=DIRECTION('',(-0.190809912898503,0.,0.981627005099017));
#102762=DIRECTION('',(0.981627005099017,0.,0.190809912898503));
#102763=DIRECTION('',(-0.190809912898503,0.,0.981627005099017));
#102764=DIRECTION('',(0.981627005099017,0.,0.190809912898503));
#102765=DIRECTION('center_axis',(0.981627005099017,0.,0.190809912898503));
#102766=DIRECTION('ref_axis',(0.,-1.,0.));
#102767=DIRECTION('',(-0.190809912898503,0.,0.981627005099017));
#102768=DIRECTION('',(0.,-1.,0.));
#102769=DIRECTION('',(0.,-1.,0.));
#102770=DIRECTION('center_axis',(0.,-1.,0.));
#102771=DIRECTION('ref_axis',(0.,0.,-1.));
#102772=DIRECTION('',(-0.190809912898503,0.,0.981627005099017));
#102773=DIRECTION('',(-0.981627005099017,0.,-0.190809912898503));
#102774=DIRECTION('',(-0.981627005099017,0.,-0.190809912898503));
#102775=DIRECTION('center_axis',(-0.981627005099017,0.,-0.190809912898503));
#102776=DIRECTION('ref_axis',(-0.190809912898503,0.,0.981627005099017));
#102777=DIRECTION('',(0.,1.,0.));
#102778=DIRECTION('',(0.,1.,0.));
#102779=DIRECTION('center_axis',(0.,1.,0.));
#102780=DIRECTION('ref_axis',(1.,0.,0.));
#102781=DIRECTION('',(-0.190809912898503,0.,0.981627005099017));
#102782=DIRECTION('',(0.981627005099017,0.,0.190809912898503));
#102783=DIRECTION('',(-0.190809912898503,0.,0.981627005099017));
#102784=DIRECTION('',(0.981627005099017,0.,0.190809912898503));
#102785=DIRECTION('center_axis',(0.981627005099017,0.,0.190809912898503));
#102786=DIRECTION('ref_axis',(0.,-1.,0.));
#102787=DIRECTION('',(-0.190809912898503,0.,0.981627005099017));
#102788=DIRECTION('',(0.,-1.,0.));
#102789=DIRECTION('',(0.,-1.,0.));
#102790=DIRECTION('center_axis',(0.,-1.,0.));
#102791=DIRECTION('ref_axis',(0.,0.,-1.));
#102792=DIRECTION('',(-0.190809912898503,0.,0.981627005099017));
#102793=DIRECTION('',(-0.981627005099017,0.,-0.190809912898503));
#102794=DIRECTION('',(-0.981627005099017,0.,-0.190809912898503));
#102795=DIRECTION('center_axis',(-0.981627005099017,0.,-0.190809912898503));
#102796=DIRECTION('ref_axis',(-0.190809912898503,0.,0.981627005099017));
#102797=DIRECTION('',(0.,1.,0.));
#102798=DIRECTION('',(0.,1.,0.));
#102799=DIRECTION('center_axis',(0.,1.,0.));
#102800=DIRECTION('ref_axis',(1.,0.,0.));
#102801=DIRECTION('',(-0.190809912898503,0.,0.981627005099017));
#102802=DIRECTION('',(0.981627005099017,0.,0.190809912898503));
#102803=DIRECTION('',(-0.190809912898503,0.,0.981627005099017));
#102804=DIRECTION('',(0.981627005099017,0.,0.190809912898503));
#102805=DIRECTION('center_axis',(0.981627005099017,0.,0.190809912898503));
#102806=DIRECTION('ref_axis',(0.,-1.,0.));
#102807=DIRECTION('',(-0.190809912898503,0.,0.981627005099017));
#102808=DIRECTION('',(0.,-1.,0.));
#102809=DIRECTION('',(0.,-1.,0.));
#102810=DIRECTION('center_axis',(0.,-1.,0.));
#102811=DIRECTION('ref_axis',(0.,0.,-1.));
#102812=DIRECTION('',(-0.190809912898503,0.,0.981627005099017));
#102813=DIRECTION('',(-0.981627005099017,0.,-0.190809912898503));
#102814=DIRECTION('',(-0.981627005099017,0.,-0.190809912898503));
#102815=DIRECTION('center_axis',(-0.981627005099017,0.,-0.190809912898503));
#102816=DIRECTION('ref_axis',(-0.190809912898503,0.,0.981627005099017));
#102817=DIRECTION('',(0.,1.,0.));
#102818=DIRECTION('',(0.,1.,0.));
#102819=DIRECTION('center_axis',(0.,1.,0.));
#102820=DIRECTION('ref_axis',(1.,0.,0.));
#102821=DIRECTION('',(-0.190809912898503,0.,0.981627005099017));
#102822=DIRECTION('',(0.981627005099017,0.,0.190809912898503));
#102823=DIRECTION('',(-0.190809912898503,0.,0.981627005099017));
#102824=DIRECTION('',(0.981627005099017,0.,0.190809912898503));
#102825=DIRECTION('center_axis',(0.981627005099017,0.,0.190809912898503));
#102826=DIRECTION('ref_axis',(0.,-1.,0.));
#102827=DIRECTION('',(-0.190809912898503,0.,0.981627005099017));
#102828=DIRECTION('',(0.,-1.,0.));
#102829=DIRECTION('',(0.,-1.,0.));
#102830=DIRECTION('center_axis',(0.,-1.,0.));
#102831=DIRECTION('ref_axis',(0.,0.,-1.));
#102832=DIRECTION('',(-0.190809912898503,0.,0.981627005099017));
#102833=DIRECTION('',(-0.981627005099017,0.,-0.190809912898503));
#102834=DIRECTION('',(-0.981627005099017,0.,-0.190809912898503));
#102835=DIRECTION('center_axis',(-0.981627005099017,0.,-0.190809912898503));
#102836=DIRECTION('ref_axis',(-0.190809912898503,0.,0.981627005099017));
#102837=DIRECTION('',(0.,1.,0.));
#102838=DIRECTION('',(0.,1.,0.));
#102839=DIRECTION('center_axis',(0.,1.,0.));
#102840=DIRECTION('ref_axis',(1.,0.,0.));
#102841=DIRECTION('',(-0.190809912898503,0.,0.981627005099017));
#102842=DIRECTION('',(0.981627005099017,0.,0.190809912898503));
#102843=DIRECTION('',(-0.190809912898503,0.,0.981627005099017));
#102844=DIRECTION('',(0.981627005099017,0.,0.190809912898503));
#102845=DIRECTION('center_axis',(0.981627005099017,0.,0.190809912898503));
#102846=DIRECTION('ref_axis',(0.,-1.,0.));
#102847=DIRECTION('',(-0.190809912898503,0.,0.981627005099017));
#102848=DIRECTION('',(0.,-1.,0.));
#102849=DIRECTION('',(0.,-1.,0.));
#102850=DIRECTION('center_axis',(0.,-1.,0.));
#102851=DIRECTION('ref_axis',(0.,0.,-1.));
#102852=DIRECTION('',(-0.190809912898503,0.,0.981627005099017));
#102853=DIRECTION('',(-0.981627005099017,0.,-0.190809912898503));
#102854=DIRECTION('',(-0.981627005099017,0.,-0.190809912898503));
#102855=DIRECTION('center_axis',(-0.981627005099017,0.,-0.190809912898503));
#102856=DIRECTION('ref_axis',(-0.190809912898503,0.,0.981627005099017));
#102857=DIRECTION('',(0.,1.,0.));
#102858=DIRECTION('',(0.,1.,0.));
#102859=DIRECTION('center_axis',(0.,1.,0.));
#102860=DIRECTION('ref_axis',(1.,0.,0.));
#102861=DIRECTION('',(-0.190809912898503,0.,0.981627005099017));
#102862=DIRECTION('',(0.981627005099017,0.,0.190809912898503));
#102863=DIRECTION('',(-0.190809912898503,0.,0.981627005099017));
#102864=DIRECTION('',(0.981627005099017,0.,0.190809912898503));
#102865=DIRECTION('center_axis',(0.981627005099017,0.,0.190809912898503));
#102866=DIRECTION('ref_axis',(0.,-1.,0.));
#102867=DIRECTION('',(-0.190809912898503,0.,0.981627005099017));
#102868=DIRECTION('',(0.,-1.,0.));
#102869=DIRECTION('',(0.,-1.,0.));
#102870=DIRECTION('center_axis',(0.,-1.,0.));
#102871=DIRECTION('ref_axis',(0.,0.,-1.));
#102872=DIRECTION('',(-0.190809912898503,0.,0.981627005099017));
#102873=DIRECTION('',(-0.981627005099017,0.,-0.190809912898503));
#102874=DIRECTION('',(-0.981627005099017,0.,-0.190809912898503));
#102875=DIRECTION('center_axis',(-0.981627005099017,0.,-0.190809912898503));
#102876=DIRECTION('ref_axis',(-0.190809912898503,0.,0.981627005099017));
#102877=DIRECTION('',(0.,1.,0.));
#102878=DIRECTION('',(0.,1.,0.));
#102879=DIRECTION('center_axis',(0.,1.,0.));
#102880=DIRECTION('ref_axis',(1.,0.,0.));
#102881=DIRECTION('',(-0.190809912898503,0.,0.981627005099017));
#102882=DIRECTION('',(0.981627005099017,0.,0.190809912898503));
#102883=DIRECTION('',(-0.190809912898503,0.,0.981627005099017));
#102884=DIRECTION('',(0.981627005099017,0.,0.190809912898503));
#102885=DIRECTION('center_axis',(0.981627005099017,0.,0.190809912898503));
#102886=DIRECTION('ref_axis',(0.,-1.,0.));
#102887=DIRECTION('',(-0.190809912898503,0.,0.981627005099017));
#102888=DIRECTION('',(0.,-1.,0.));
#102889=DIRECTION('',(0.,-1.,0.));
#102890=DIRECTION('center_axis',(0.,-1.,0.));
#102891=DIRECTION('ref_axis',(0.,0.,-1.));
#102892=DIRECTION('',(-0.190809912898503,0.,0.981627005099017));
#102893=DIRECTION('',(-0.981627005099017,0.,-0.190809912898503));
#102894=DIRECTION('',(-0.981627005099017,0.,-0.190809912898503));
#102895=DIRECTION('center_axis',(-0.981627005099017,0.,-0.190809912898503));
#102896=DIRECTION('ref_axis',(-0.190809912898503,0.,0.981627005099017));
#102897=DIRECTION('',(0.,1.,0.));
#102898=DIRECTION('',(0.,1.,0.));
#102899=DIRECTION('center_axis',(0.,1.,0.));
#102900=DIRECTION('ref_axis',(1.,0.,0.));
#102901=DIRECTION('',(-0.190809912898503,0.,0.981627005099017));
#102902=DIRECTION('',(0.981627005099017,0.,0.190809912898503));
#102903=DIRECTION('',(-0.190809912898503,0.,0.981627005099017));
#102904=DIRECTION('',(0.981627005099017,0.,0.190809912898503));
#102905=DIRECTION('center_axis',(0.981627005099017,0.,0.190809912898503));
#102906=DIRECTION('ref_axis',(0.,-1.,0.));
#102907=DIRECTION('',(-0.190809912898503,0.,0.981627005099017));
#102908=DIRECTION('',(0.,-1.,0.));
#102909=DIRECTION('',(0.,-1.,0.));
#102910=DIRECTION('center_axis',(0.,-1.,0.));
#102911=DIRECTION('ref_axis',(0.,0.,-1.));
#102912=DIRECTION('',(-0.190809912898503,0.,0.981627005099017));
#102913=DIRECTION('',(-0.981627005099017,0.,-0.190809912898503));
#102914=DIRECTION('',(-0.981627005099017,0.,-0.190809912898503));
#102915=DIRECTION('center_axis',(-0.981627005099017,0.,-0.190809912898503));
#102916=DIRECTION('ref_axis',(-0.190809912898503,0.,0.981627005099017));
#102917=DIRECTION('',(0.,1.,0.));
#102918=DIRECTION('',(0.,1.,0.));
#102919=DIRECTION('center_axis',(0.,1.,0.));
#102920=DIRECTION('ref_axis',(1.,0.,0.));
#102921=DIRECTION('',(-0.190809912898503,0.,0.981627005099017));
#102922=DIRECTION('',(0.981627005099017,0.,0.190809912898503));
#102923=DIRECTION('',(-0.190809912898503,0.,0.981627005099017));
#102924=DIRECTION('',(0.981627005099017,0.,0.190809912898503));
#102925=DIRECTION('center_axis',(0.981627005099017,0.,0.190809912898503));
#102926=DIRECTION('ref_axis',(0.,-1.,0.));
#102927=DIRECTION('',(-0.190809912898503,0.,0.981627005099017));
#102928=DIRECTION('',(0.,-1.,0.));
#102929=DIRECTION('',(0.,-1.,0.));
#102930=DIRECTION('center_axis',(0.,-1.,0.));
#102931=DIRECTION('ref_axis',(0.,0.,-1.));
#102932=DIRECTION('',(-0.190809912898503,0.,0.981627005099017));
#102933=DIRECTION('',(-0.981627005099017,0.,-0.190809912898503));
#102934=DIRECTION('',(-0.981627005099017,0.,-0.190809912898503));
#102935=DIRECTION('center_axis',(-0.981627005099017,0.,-0.190809912898503));
#102936=DIRECTION('ref_axis',(-0.190809912898503,0.,0.981627005099017));
#102937=DIRECTION('',(0.,1.,0.));
#102938=DIRECTION('',(0.,1.,0.));
#102939=DIRECTION('center_axis',(0.,1.,0.));
#102940=DIRECTION('ref_axis',(1.,0.,0.));
#102941=DIRECTION('',(-0.190809912898503,0.,0.981627005099017));
#102942=DIRECTION('',(0.981627005099017,0.,0.190809912898503));
#102943=DIRECTION('',(-0.190809912898503,0.,0.981627005099017));
#102944=DIRECTION('',(0.981627005099017,0.,0.190809912898503));
#102945=DIRECTION('center_axis',(0.981627005099017,0.,0.190809912898503));
#102946=DIRECTION('ref_axis',(0.,-1.,0.));
#102947=DIRECTION('',(-0.190809912898503,0.,0.981627005099017));
#102948=DIRECTION('',(0.,-1.,0.));
#102949=DIRECTION('',(0.,-1.,0.));
#102950=DIRECTION('center_axis',(0.,-1.,0.));
#102951=DIRECTION('ref_axis',(0.,0.,-1.));
#102952=DIRECTION('',(-0.190809912898503,0.,0.981627005099017));
#102953=DIRECTION('',(-0.981627005099017,0.,-0.190809912898503));
#102954=DIRECTION('',(-0.981627005099017,0.,-0.190809912898503));
#102955=DIRECTION('center_axis',(-0.981627005099017,0.,-0.190809912898503));
#102956=DIRECTION('ref_axis',(-0.190809912898503,0.,0.981627005099017));
#102957=DIRECTION('',(0.,1.,0.));
#102958=DIRECTION('',(0.,1.,0.));
#102959=DIRECTION('center_axis',(0.,1.,0.));
#102960=DIRECTION('ref_axis',(1.,0.,0.));
#102961=DIRECTION('',(-0.190809912898503,0.,0.981627005099017));
#102962=DIRECTION('',(0.981627005099017,0.,0.190809912898503));
#102963=DIRECTION('',(-0.190809912898503,0.,0.981627005099017));
#102964=DIRECTION('',(0.981627005099017,0.,0.190809912898503));
#102965=DIRECTION('center_axis',(0.981627005099017,0.,0.190809912898503));
#102966=DIRECTION('ref_axis',(0.,-1.,0.));
#102967=DIRECTION('',(-0.190809912898503,0.,0.981627005099017));
#102968=DIRECTION('',(0.,-1.,0.));
#102969=DIRECTION('',(0.,-1.,0.));
#102970=DIRECTION('center_axis',(0.,-1.,0.));
#102971=DIRECTION('ref_axis',(0.,0.,-1.));
#102972=DIRECTION('',(-0.190809912898503,0.,0.981627005099017));
#102973=DIRECTION('',(-0.981627005099017,0.,-0.190809912898503));
#102974=DIRECTION('',(-0.981627005099017,0.,-0.190809912898503));
#102975=DIRECTION('center_axis',(-0.981627005099017,0.,-0.190809912898503));
#102976=DIRECTION('ref_axis',(-0.190809912898503,0.,0.981627005099017));
#102977=DIRECTION('',(0.,1.,0.));
#102978=DIRECTION('',(0.,1.,0.));
#102979=DIRECTION('center_axis',(0.,1.,0.));
#102980=DIRECTION('ref_axis',(1.,0.,0.));
#102981=DIRECTION('',(-0.190809912898503,0.,0.981627005099017));
#102982=DIRECTION('',(0.981627005099017,0.,0.190809912898503));
#102983=DIRECTION('',(-0.190809912898503,0.,0.981627005099017));
#102984=DIRECTION('',(0.981627005099017,0.,0.190809912898503));
#102985=DIRECTION('center_axis',(0.981627005099017,0.,0.190809912898503));
#102986=DIRECTION('ref_axis',(0.,-1.,0.));
#102987=DIRECTION('',(-0.190809912898503,0.,0.981627005099017));
#102988=DIRECTION('',(0.,-1.,0.));
#102989=DIRECTION('',(0.,-1.,0.));
#102990=DIRECTION('center_axis',(0.,-1.,0.));
#102991=DIRECTION('ref_axis',(0.,0.,-1.));
#102992=DIRECTION('',(-0.190809912898503,0.,0.981627005099017));
#102993=DIRECTION('',(-0.981627005099017,0.,-0.190809912898503));
#102994=DIRECTION('',(-0.981627005099017,0.,-0.190809912898503));
#102995=DIRECTION('center_axis',(-0.981627005099017,0.,-0.190809912898503));
#102996=DIRECTION('ref_axis',(-0.190809912898503,0.,0.981627005099017));
#102997=DIRECTION('',(0.,1.,0.));
#102998=DIRECTION('',(0.,1.,0.));
#102999=DIRECTION('center_axis',(0.,1.,0.));
#103000=DIRECTION('ref_axis',(1.,0.,0.));
#103001=DIRECTION('',(-0.190809912898503,0.,0.981627005099017));
#103002=DIRECTION('',(0.981627005099017,0.,0.190809912898503));
#103003=DIRECTION('',(-0.190809912898503,0.,0.981627005099017));
#103004=DIRECTION('',(0.981627005099017,0.,0.190809912898503));
#103005=DIRECTION('center_axis',(0.981627005099017,0.,0.190809912898503));
#103006=DIRECTION('ref_axis',(0.,-1.,0.));
#103007=DIRECTION('',(-0.190809912898503,0.,0.981627005099017));
#103008=DIRECTION('',(0.,-1.,0.));
#103009=DIRECTION('',(0.,-1.,0.));
#103010=DIRECTION('center_axis',(0.,-1.,0.));
#103011=DIRECTION('ref_axis',(0.,0.,-1.));
#103012=DIRECTION('',(-0.190809912898503,0.,0.981627005099017));
#103013=DIRECTION('',(-0.981627005099017,0.,-0.190809912898503));
#103014=DIRECTION('',(-0.981627005099017,0.,-0.190809912898503));
#103015=DIRECTION('center_axis',(-0.981627005099017,0.,-0.190809912898503));
#103016=DIRECTION('ref_axis',(-0.190809912898503,0.,0.981627005099017));
#103017=DIRECTION('',(0.,1.,0.));
#103018=DIRECTION('',(0.,1.,0.));
#103019=DIRECTION('center_axis',(0.,1.,0.));
#103020=DIRECTION('ref_axis',(1.,0.,0.));
#103021=DIRECTION('',(-0.190809912898503,0.,0.981627005099017));
#103022=DIRECTION('',(0.981627005099017,0.,0.190809912898503));
#103023=DIRECTION('',(-0.190809912898503,0.,0.981627005099017));
#103024=DIRECTION('',(0.981627005099017,0.,0.190809912898503));
#103025=DIRECTION('center_axis',(0.981627005099017,0.,0.190809912898503));
#103026=DIRECTION('ref_axis',(0.,-1.,0.));
#103027=DIRECTION('',(-0.190809912898503,0.,0.981627005099017));
#103028=DIRECTION('',(0.,-1.,0.));
#103029=DIRECTION('',(0.,-1.,0.));
#103030=DIRECTION('center_axis',(0.,-1.,0.));
#103031=DIRECTION('ref_axis',(0.,0.,-1.));
#103032=DIRECTION('',(-0.190809912898503,0.,0.981627005099017));
#103033=DIRECTION('',(-0.981627005099017,0.,-0.190809912898503));
#103034=DIRECTION('',(-0.981627005099017,0.,-0.190809912898503));
#103035=DIRECTION('center_axis',(-0.981627005099017,0.,-0.190809912898503));
#103036=DIRECTION('ref_axis',(-0.190809912898503,0.,0.981627005099017));
#103037=DIRECTION('',(0.,1.,0.));
#103038=DIRECTION('',(0.,1.,0.));
#103039=DIRECTION('center_axis',(0.,1.,0.));
#103040=DIRECTION('ref_axis',(1.,0.,0.));
#103041=DIRECTION('',(-0.190809912898503,0.,0.981627005099017));
#103042=DIRECTION('',(0.981627005099017,0.,0.190809912898503));
#103043=DIRECTION('',(-0.190809912898503,0.,0.981627005099017));
#103044=DIRECTION('',(0.981627005099017,0.,0.190809912898503));
#103045=DIRECTION('center_axis',(0.981627005099017,0.,0.190809912898503));
#103046=DIRECTION('ref_axis',(0.,-1.,0.));
#103047=DIRECTION('',(-0.190809912898503,0.,0.981627005099017));
#103048=DIRECTION('',(0.,-1.,0.));
#103049=DIRECTION('',(0.,-1.,0.));
#103050=DIRECTION('center_axis',(0.,-1.,0.));
#103051=DIRECTION('ref_axis',(0.,0.,-1.));
#103052=DIRECTION('',(-0.190809912898503,0.,0.981627005099017));
#103053=DIRECTION('',(-0.981627005099017,0.,-0.190809912898503));
#103054=DIRECTION('',(-0.981627005099017,0.,-0.190809912898503));
#103055=DIRECTION('center_axis',(-0.981627005099017,0.,-0.190809912898503));
#103056=DIRECTION('ref_axis',(-0.190809912898503,0.,0.981627005099017));
#103057=DIRECTION('',(0.,1.,0.));
#103058=DIRECTION('',(0.,1.,0.));
#103059=DIRECTION('center_axis',(0.,1.,0.));
#103060=DIRECTION('ref_axis',(1.,0.,0.));
#103061=DIRECTION('',(-0.190809912898503,0.,0.981627005099017));
#103062=DIRECTION('',(0.981627005099017,0.,0.190809912898503));
#103063=DIRECTION('',(-0.190809912898503,0.,0.981627005099017));
#103064=DIRECTION('',(0.981627005099017,0.,0.190809912898503));
#103065=DIRECTION('center_axis',(0.981627005099017,0.,0.190809912898503));
#103066=DIRECTION('ref_axis',(0.,-1.,0.));
#103067=DIRECTION('',(-0.190809912898503,0.,0.981627005099017));
#103068=DIRECTION('',(0.,-1.,0.));
#103069=DIRECTION('',(0.,-1.,0.));
#103070=DIRECTION('center_axis',(0.,-1.,0.));
#103071=DIRECTION('ref_axis',(0.,0.,-1.));
#103072=DIRECTION('',(-0.190809912898503,0.,0.981627005099017));
#103073=DIRECTION('',(-0.981627005099017,0.,-0.190809912898503));
#103074=DIRECTION('',(-0.981627005099017,0.,-0.190809912898503));
#103075=DIRECTION('center_axis',(-0.981627005099017,0.,-0.190809912898503));
#103076=DIRECTION('ref_axis',(-0.190809912898503,0.,0.981627005099017));
#103077=DIRECTION('',(0.,1.,0.));
#103078=DIRECTION('',(0.,1.,0.));
#103079=DIRECTION('center_axis',(0.,1.,0.));
#103080=DIRECTION('ref_axis',(1.,0.,0.));
#103081=DIRECTION('',(-0.190809912898503,0.,0.981627005099017));
#103082=DIRECTION('',(0.981627005099017,0.,0.190809912898503));
#103083=DIRECTION('',(-0.190809912898503,0.,0.981627005099017));
#103084=DIRECTION('',(0.981627005099017,0.,0.190809912898503));
#103085=DIRECTION('center_axis',(0.981627005099017,0.,0.190809912898503));
#103086=DIRECTION('ref_axis',(0.,-1.,0.));
#103087=DIRECTION('',(-0.190809912898503,0.,0.981627005099017));
#103088=DIRECTION('',(0.,-1.,0.));
#103089=DIRECTION('',(0.,-1.,0.));
#103090=DIRECTION('center_axis',(0.,-1.,0.));
#103091=DIRECTION('ref_axis',(0.,0.,-1.));
#103092=DIRECTION('',(-0.190809912898503,0.,0.981627005099017));
#103093=DIRECTION('',(-0.981627005099017,0.,-0.190809912898503));
#103094=DIRECTION('',(-0.981627005099017,0.,-0.190809912898503));
#103095=DIRECTION('center_axis',(-0.981627005099017,0.,-0.190809912898503));
#103096=DIRECTION('ref_axis',(-0.190809912898503,0.,0.981627005099017));
#103097=DIRECTION('',(0.,1.,0.));
#103098=DIRECTION('',(0.,1.,0.));
#103099=DIRECTION('center_axis',(0.,1.,0.));
#103100=DIRECTION('ref_axis',(1.,0.,0.));
#103101=DIRECTION('',(-0.190809912898503,0.,0.981627005099017));
#103102=DIRECTION('',(0.981627005099017,0.,0.190809912898503));
#103103=DIRECTION('',(-0.190809912898503,0.,0.981627005099017));
#103104=DIRECTION('',(0.981627005099017,0.,0.190809912898503));
#103105=DIRECTION('center_axis',(0.981627005099017,0.,0.190809912898503));
#103106=DIRECTION('ref_axis',(0.,-1.,0.));
#103107=DIRECTION('',(-0.190809912898503,0.,0.981627005099017));
#103108=DIRECTION('',(0.,-1.,0.));
#103109=DIRECTION('',(0.,-1.,0.));
#103110=DIRECTION('center_axis',(0.,-1.,0.));
#103111=DIRECTION('ref_axis',(0.,0.,-1.));
#103112=DIRECTION('',(-0.190809912898503,0.,0.981627005099017));
#103113=DIRECTION('',(-0.981627005099017,0.,-0.190809912898503));
#103114=DIRECTION('',(-0.981627005099017,0.,-0.190809912898503));
#103115=DIRECTION('center_axis',(-0.981627005099017,0.,-0.190809912898503));
#103116=DIRECTION('ref_axis',(-0.190809912898503,0.,0.981627005099017));
#103117=DIRECTION('',(0.,1.,0.));
#103118=DIRECTION('',(0.,1.,0.));
#103119=DIRECTION('center_axis',(0.,1.,0.));
#103120=DIRECTION('ref_axis',(1.,0.,0.));
#103121=DIRECTION('',(-0.190809912898503,0.,0.981627005099017));
#103122=DIRECTION('',(0.981627005099017,0.,0.190809912898503));
#103123=DIRECTION('',(-0.190809912898503,0.,0.981627005099017));
#103124=DIRECTION('',(0.981627005099017,0.,0.190809912898503));
#103125=DIRECTION('center_axis',(0.981627005099017,0.,0.190809912898503));
#103126=DIRECTION('ref_axis',(0.,-1.,0.));
#103127=DIRECTION('',(-0.190809912898503,0.,0.981627005099017));
#103128=DIRECTION('',(0.,-1.,0.));
#103129=DIRECTION('',(0.,-1.,0.));
#103130=DIRECTION('center_axis',(0.,-1.,0.));
#103131=DIRECTION('ref_axis',(0.,0.,-1.));
#103132=DIRECTION('',(-0.190809912898503,0.,0.981627005099017));
#103133=DIRECTION('',(-0.981627005099017,0.,-0.190809912898503));
#103134=DIRECTION('',(-0.981627005099017,0.,-0.190809912898503));
#103135=DIRECTION('center_axis',(-0.981627005099017,0.,-0.190809912898503));
#103136=DIRECTION('ref_axis',(-0.190809912898503,0.,0.981627005099017));
#103137=DIRECTION('',(0.,1.,0.));
#103138=DIRECTION('',(0.,1.,0.));
#103139=DIRECTION('center_axis',(0.,1.,0.));
#103140=DIRECTION('ref_axis',(1.,0.,0.));
#103141=DIRECTION('',(-0.190809912898503,0.,0.981627005099017));
#103142=DIRECTION('',(0.981627005099017,0.,0.190809912898503));
#103143=DIRECTION('',(-0.190809912898503,0.,0.981627005099017));
#103144=DIRECTION('',(0.981627005099017,0.,0.190809912898503));
#103145=DIRECTION('center_axis',(0.981627005099017,0.,0.190809912898503));
#103146=DIRECTION('ref_axis',(0.,-1.,0.));
#103147=DIRECTION('',(-0.190809912898503,0.,0.981627005099017));
#103148=DIRECTION('',(0.,-1.,0.));
#103149=DIRECTION('',(0.,-1.,0.));
#103150=DIRECTION('center_axis',(0.,-1.,0.));
#103151=DIRECTION('ref_axis',(0.,0.,-1.));
#103152=DIRECTION('',(-0.190809912898503,0.,0.981627005099017));
#103153=DIRECTION('',(-0.981627005099017,0.,-0.190809912898503));
#103154=DIRECTION('',(-0.981627005099017,0.,-0.190809912898503));
#103155=DIRECTION('center_axis',(-0.981627005099017,0.,-0.190809912898503));
#103156=DIRECTION('ref_axis',(-0.190809912898503,0.,0.981627005099017));
#103157=DIRECTION('',(0.,1.,0.));
#103158=DIRECTION('',(0.,1.,0.));
#103159=DIRECTION('center_axis',(0.,1.,0.));
#103160=DIRECTION('ref_axis',(1.,0.,0.));
#103161=DIRECTION('',(-0.190809912898503,0.,0.981627005099017));
#103162=DIRECTION('',(0.981627005099017,0.,0.190809912898503));
#103163=DIRECTION('',(-0.190809912898503,0.,0.981627005099017));
#103164=DIRECTION('',(0.981627005099017,0.,0.190809912898503));
#103165=DIRECTION('center_axis',(0.981627005099017,0.,0.190809912898503));
#103166=DIRECTION('ref_axis',(0.,-1.,0.));
#103167=DIRECTION('',(-0.190809912898503,0.,0.981627005099017));
#103168=DIRECTION('',(0.,-1.,0.));
#103169=DIRECTION('',(0.,-1.,0.));
#103170=DIRECTION('center_axis',(0.,-1.,0.));
#103171=DIRECTION('ref_axis',(0.,0.,-1.));
#103172=DIRECTION('',(-0.190809912898503,0.,0.981627005099017));
#103173=DIRECTION('',(-0.981627005099017,0.,-0.190809912898503));
#103174=DIRECTION('',(-0.981627005099017,0.,-0.190809912898503));
#103175=DIRECTION('center_axis',(-0.981627005099017,0.,-0.190809912898503));
#103176=DIRECTION('ref_axis',(-0.190809912898503,0.,0.981627005099017));
#103177=DIRECTION('',(0.,1.,0.));
#103178=DIRECTION('',(0.,1.,0.));
#103179=DIRECTION('center_axis',(0.,1.,0.));
#103180=DIRECTION('ref_axis',(1.,0.,0.));
#103181=DIRECTION('',(-0.190809912898503,0.,0.981627005099017));
#103182=DIRECTION('',(0.981627005099017,0.,0.190809912898503));
#103183=DIRECTION('',(-0.190809912898503,0.,0.981627005099017));
#103184=DIRECTION('',(0.981627005099017,0.,0.190809912898503));
#103185=DIRECTION('center_axis',(0.981627005099017,0.,0.190809912898503));
#103186=DIRECTION('ref_axis',(0.,-1.,0.));
#103187=DIRECTION('',(-0.190809912898503,0.,0.981627005099017));
#103188=DIRECTION('',(0.,-1.,0.));
#103189=DIRECTION('',(0.,-1.,0.));
#103190=DIRECTION('center_axis',(0.,-1.,0.));
#103191=DIRECTION('ref_axis',(0.,0.,-1.));
#103192=DIRECTION('',(-0.190809912898503,0.,0.981627005099017));
#103193=DIRECTION('',(-0.981627005099017,0.,-0.190809912898503));
#103194=DIRECTION('',(-0.981627005099017,0.,-0.190809912898503));
#103195=DIRECTION('center_axis',(-0.981627005099017,0.,-0.190809912898503));
#103196=DIRECTION('ref_axis',(-0.190809912898503,0.,0.981627005099017));
#103197=DIRECTION('',(0.,1.,0.));
#103198=DIRECTION('',(0.,1.,0.));
#103199=DIRECTION('center_axis',(0.,1.,0.));
#103200=DIRECTION('ref_axis',(1.,0.,0.));
#103201=DIRECTION('',(-0.190809912898503,0.,0.981627005099017));
#103202=DIRECTION('',(0.981627005099017,0.,0.190809912898503));
#103203=DIRECTION('',(-0.190809912898503,0.,0.981627005099017));
#103204=DIRECTION('',(0.981627005099017,0.,0.190809912898503));
#103205=DIRECTION('center_axis',(0.981627005099017,0.,0.190809912898503));
#103206=DIRECTION('ref_axis',(0.,-1.,0.));
#103207=DIRECTION('',(-0.190809912898503,0.,0.981627005099017));
#103208=DIRECTION('',(0.,-1.,0.));
#103209=DIRECTION('',(0.,-1.,0.));
#103210=DIRECTION('center_axis',(0.,-1.,0.));
#103211=DIRECTION('ref_axis',(0.,0.,-1.));
#103212=DIRECTION('',(-0.190809912898503,0.,0.981627005099017));
#103213=DIRECTION('',(-0.981627005099017,0.,-0.190809912898503));
#103214=DIRECTION('',(-0.981627005099017,0.,-0.190809912898503));
#103215=DIRECTION('center_axis',(-0.981627005099017,0.,-0.190809912898503));
#103216=DIRECTION('ref_axis',(-0.190809912898503,0.,0.981627005099017));
#103217=DIRECTION('',(0.,1.,0.));
#103218=DIRECTION('',(0.,1.,0.));
#103219=DIRECTION('center_axis',(0.,1.,0.));
#103220=DIRECTION('ref_axis',(1.,0.,0.));
#103221=DIRECTION('',(-0.190809912898503,0.,0.981627005099017));
#103222=DIRECTION('',(0.981627005099017,0.,0.190809912898503));
#103223=DIRECTION('',(-0.190809912898503,0.,0.981627005099017));
#103224=DIRECTION('',(0.981627005099017,0.,0.190809912898503));
#103225=DIRECTION('center_axis',(0.981627005099017,0.,0.190809912898503));
#103226=DIRECTION('ref_axis',(0.,-1.,0.));
#103227=DIRECTION('',(-0.190809912898503,0.,0.981627005099017));
#103228=DIRECTION('',(0.,-1.,0.));
#103229=DIRECTION('',(0.,-1.,0.));
#103230=DIRECTION('center_axis',(0.,-1.,0.));
#103231=DIRECTION('ref_axis',(0.,0.,-1.));
#103232=DIRECTION('',(-0.190809912898503,0.,0.981627005099017));
#103233=DIRECTION('',(-0.981627005099017,0.,-0.190809912898503));
#103234=DIRECTION('',(-0.981627005099017,0.,-0.190809912898503));
#103235=DIRECTION('center_axis',(-0.981627005099017,0.,-0.190809912898503));
#103236=DIRECTION('ref_axis',(-0.190809912898503,0.,0.981627005099017));
#103237=DIRECTION('',(0.,1.,0.));
#103238=DIRECTION('',(0.,1.,0.));
#103239=DIRECTION('center_axis',(0.,1.,0.));
#103240=DIRECTION('ref_axis',(1.,0.,0.));
#103241=DIRECTION('',(-0.190809912898503,0.,0.981627005099017));
#103242=DIRECTION('',(0.981627005099017,0.,0.190809912898503));
#103243=DIRECTION('',(-0.190809912898503,0.,0.981627005099017));
#103244=DIRECTION('',(0.981627005099017,0.,0.190809912898503));
#103245=DIRECTION('center_axis',(0.981627005099017,0.,0.190809912898503));
#103246=DIRECTION('ref_axis',(0.,-1.,0.));
#103247=DIRECTION('',(-0.190809912898503,0.,0.981627005099017));
#103248=DIRECTION('',(0.,-1.,0.));
#103249=DIRECTION('',(0.,-1.,0.));
#103250=DIRECTION('center_axis',(0.,-1.,0.));
#103251=DIRECTION('ref_axis',(0.,0.,-1.));
#103252=DIRECTION('',(-0.190809912898503,0.,0.981627005099017));
#103253=DIRECTION('',(-0.981627005099017,0.,-0.190809912898503));
#103254=DIRECTION('',(-0.981627005099017,0.,-0.190809912898503));
#103255=DIRECTION('center_axis',(-0.981627005099017,0.,-0.190809912898503));
#103256=DIRECTION('ref_axis',(-0.190809912898503,0.,0.981627005099017));
#103257=DIRECTION('',(0.,1.,0.));
#103258=DIRECTION('',(0.,1.,0.));
#103259=DIRECTION('center_axis',(0.,1.,0.));
#103260=DIRECTION('ref_axis',(1.,0.,0.));
#103261=DIRECTION('',(-0.190809912898503,0.,0.981627005099017));
#103262=DIRECTION('',(0.981627005099017,0.,0.190809912898503));
#103263=DIRECTION('',(-0.190809912898503,0.,0.981627005099017));
#103264=DIRECTION('',(0.981627005099017,0.,0.190809912898503));
#103265=DIRECTION('center_axis',(0.981627005099017,0.,0.190809912898503));
#103266=DIRECTION('ref_axis',(0.,-1.,0.));
#103267=DIRECTION('',(-0.190809912898503,0.,0.981627005099017));
#103268=DIRECTION('',(0.,-1.,0.));
#103269=DIRECTION('',(0.,-1.,0.));
#103270=DIRECTION('center_axis',(0.,-1.,0.));
#103271=DIRECTION('ref_axis',(0.,0.,-1.));
#103272=DIRECTION('',(-0.190809912898503,0.,0.981627005099017));
#103273=DIRECTION('',(-0.981627005099017,0.,-0.190809912898503));
#103274=DIRECTION('',(-0.981627005099017,0.,-0.190809912898503));
#103275=DIRECTION('center_axis',(-0.981627005099017,0.,-0.190809912898503));
#103276=DIRECTION('ref_axis',(-0.190809912898503,0.,0.981627005099017));
#103277=DIRECTION('',(0.,1.,0.));
#103278=DIRECTION('',(0.,1.,0.));
#103279=DIRECTION('center_axis',(0.,1.,0.));
#103280=DIRECTION('ref_axis',(1.,0.,0.));
#103281=DIRECTION('',(-0.190809912898503,0.,0.981627005099017));
#103282=DIRECTION('',(0.981627005099017,0.,0.190809912898503));
#103283=DIRECTION('',(-0.190809912898503,0.,0.981627005099017));
#103284=DIRECTION('',(0.981627005099017,0.,0.190809912898503));
#103285=DIRECTION('center_axis',(0.981627005099017,0.,0.190809912898503));
#103286=DIRECTION('ref_axis',(0.,-1.,0.));
#103287=DIRECTION('',(-0.190809912898503,0.,0.981627005099017));
#103288=DIRECTION('',(0.,-1.,0.));
#103289=DIRECTION('',(0.,-1.,0.));
#103290=DIRECTION('center_axis',(0.,-1.,0.));
#103291=DIRECTION('ref_axis',(0.,0.,-1.));
#103292=DIRECTION('',(-0.190809912898503,0.,0.981627005099017));
#103293=DIRECTION('',(-0.981627005099017,0.,-0.190809912898503));
#103294=DIRECTION('',(-0.981627005099017,0.,-0.190809912898503));
#103295=DIRECTION('center_axis',(-0.981627005099017,0.,-0.190809912898503));
#103296=DIRECTION('ref_axis',(-0.190809912898503,0.,0.981627005099017));
#103297=DIRECTION('',(0.,1.,0.));
#103298=DIRECTION('',(0.,1.,0.));
#103299=DIRECTION('center_axis',(0.,1.,0.));
#103300=DIRECTION('ref_axis',(1.,0.,0.));
#103301=DIRECTION('',(-0.190809912898503,0.,0.981627005099017));
#103302=DIRECTION('',(0.981627005099017,0.,0.190809912898503));
#103303=DIRECTION('',(-0.190809912898503,0.,0.981627005099017));
#103304=DIRECTION('',(0.981627005099017,0.,0.190809912898503));
#103305=DIRECTION('center_axis',(0.981627005099017,0.,0.190809912898503));
#103306=DIRECTION('ref_axis',(0.,-1.,0.));
#103307=DIRECTION('',(-0.190809912898503,0.,0.981627005099017));
#103308=DIRECTION('',(0.,-1.,0.));
#103309=DIRECTION('',(0.,-1.,0.));
#103310=DIRECTION('center_axis',(0.,-1.,0.));
#103311=DIRECTION('ref_axis',(0.,0.,-1.));
#103312=DIRECTION('',(-0.190809912898503,0.,0.981627005099017));
#103313=DIRECTION('',(-0.981627005099017,0.,-0.190809912898503));
#103314=DIRECTION('',(-0.981627005099017,0.,-0.190809912898503));
#103315=DIRECTION('center_axis',(-0.981627005099017,0.,-0.190809912898503));
#103316=DIRECTION('ref_axis',(-0.190809912898503,0.,0.981627005099017));
#103317=DIRECTION('',(0.,1.,0.));
#103318=DIRECTION('',(0.,1.,0.));
#103319=DIRECTION('center_axis',(0.,1.,0.));
#103320=DIRECTION('ref_axis',(1.,0.,0.));
#103321=DIRECTION('',(-0.190809912898503,0.,0.981627005099017));
#103322=DIRECTION('',(0.981627005099017,0.,0.190809912898503));
#103323=DIRECTION('',(-0.190809912898503,0.,0.981627005099017));
#103324=DIRECTION('',(0.981627005099017,0.,0.190809912898503));
#103325=DIRECTION('center_axis',(0.981627005099017,0.,0.190809912898503));
#103326=DIRECTION('ref_axis',(0.,-1.,0.));
#103327=DIRECTION('',(-0.190809912898503,0.,0.981627005099017));
#103328=DIRECTION('',(0.,-1.,0.));
#103329=DIRECTION('',(0.,-1.,0.));
#103330=DIRECTION('center_axis',(0.,-1.,0.));
#103331=DIRECTION('ref_axis',(0.,0.,-1.));
#103332=DIRECTION('',(-0.190809912898503,0.,0.981627005099017));
#103333=DIRECTION('',(-0.981627005099017,0.,-0.190809912898503));
#103334=DIRECTION('',(-0.981627005099017,0.,-0.190809912898503));
#103335=DIRECTION('center_axis',(-0.981627005099017,0.,-0.190809912898503));
#103336=DIRECTION('ref_axis',(-0.190809912898503,0.,0.981627005099017));
#103337=DIRECTION('',(0.,1.,0.));
#103338=DIRECTION('',(0.,1.,0.));
#103339=DIRECTION('center_axis',(0.,1.,0.));
#103340=DIRECTION('ref_axis',(1.,0.,0.));
#103341=DIRECTION('',(-0.190809912898503,0.,0.981627005099017));
#103342=DIRECTION('',(0.981627005099017,0.,0.190809912898503));
#103343=DIRECTION('',(-0.190809912898503,0.,0.981627005099017));
#103344=DIRECTION('',(0.981627005099017,0.,0.190809912898503));
#103345=DIRECTION('center_axis',(0.981627005099017,0.,0.190809912898503));
#103346=DIRECTION('ref_axis',(0.,-1.,0.));
#103347=DIRECTION('',(-0.190809912898503,0.,0.981627005099017));
#103348=DIRECTION('',(0.,-1.,0.));
#103349=DIRECTION('',(0.,-1.,0.));
#103350=DIRECTION('center_axis',(0.,-1.,0.));
#103351=DIRECTION('ref_axis',(0.,0.,-1.));
#103352=DIRECTION('',(-0.190809912898503,0.,0.981627005099017));
#103353=DIRECTION('',(-0.981627005099017,0.,-0.190809912898503));
#103354=DIRECTION('',(-0.981627005099017,0.,-0.190809912898503));
#103355=DIRECTION('center_axis',(-0.981627005099017,0.,-0.190809912898503));
#103356=DIRECTION('ref_axis',(-0.190809912898503,0.,0.981627005099017));
#103357=DIRECTION('',(0.,1.,0.));
#103358=DIRECTION('',(0.,1.,0.));
#103359=DIRECTION('center_axis',(0.,1.,0.));
#103360=DIRECTION('ref_axis',(1.,0.,0.));
#103361=DIRECTION('',(-0.190809912898503,0.,0.981627005099017));
#103362=DIRECTION('',(0.981627005099017,0.,0.190809912898503));
#103363=DIRECTION('',(-0.190809912898503,0.,0.981627005099017));
#103364=DIRECTION('',(0.981627005099017,0.,0.190809912898503));
#103365=DIRECTION('center_axis',(0.981627005099017,0.,0.190809912898503));
#103366=DIRECTION('ref_axis',(0.,-1.,0.));
#103367=DIRECTION('',(-0.190809912898503,0.,0.981627005099017));
#103368=DIRECTION('',(0.,-1.,0.));
#103369=DIRECTION('',(0.,-1.,0.));
#103370=DIRECTION('center_axis',(0.,-1.,0.));
#103371=DIRECTION('ref_axis',(0.,0.,-1.));
#103372=DIRECTION('',(-0.190809912898503,0.,0.981627005099017));
#103373=DIRECTION('',(-0.981627005099017,0.,-0.190809912898503));
#103374=DIRECTION('',(-0.981627005099017,0.,-0.190809912898503));
#103375=DIRECTION('center_axis',(-0.981627005099017,0.,-0.190809912898503));
#103376=DIRECTION('ref_axis',(-0.190809912898503,0.,0.981627005099017));
#103377=DIRECTION('',(0.,1.,0.));
#103378=DIRECTION('',(0.,1.,0.));
#103379=DIRECTION('center_axis',(0.,1.,0.));
#103380=DIRECTION('ref_axis',(1.,0.,0.));
#103381=DIRECTION('',(-0.190809912898503,0.,0.981627005099017));
#103382=DIRECTION('',(0.981627005099017,0.,0.190809912898503));
#103383=DIRECTION('',(-0.190809912898503,0.,0.981627005099017));
#103384=DIRECTION('',(0.981627005099017,0.,0.190809912898503));
#103385=DIRECTION('center_axis',(0.981627005099017,0.,0.190809912898503));
#103386=DIRECTION('ref_axis',(0.,-1.,0.));
#103387=DIRECTION('',(-0.190809912898503,0.,0.981627005099017));
#103388=DIRECTION('',(0.,-1.,0.));
#103389=DIRECTION('',(0.,-1.,0.));
#103390=DIRECTION('center_axis',(0.,-1.,0.));
#103391=DIRECTION('ref_axis',(0.,0.,-1.));
#103392=DIRECTION('',(-0.190809912898503,0.,0.981627005099017));
#103393=DIRECTION('',(-0.981627005099017,0.,-0.190809912898503));
#103394=DIRECTION('',(-0.981627005099017,0.,-0.190809912898503));
#103395=DIRECTION('center_axis',(-0.981627005099017,0.,-0.190809912898503));
#103396=DIRECTION('ref_axis',(-0.190809912898503,0.,0.981627005099017));
#103397=DIRECTION('',(0.,1.,0.));
#103398=DIRECTION('',(0.,1.,0.));
#103399=DIRECTION('center_axis',(0.,1.,0.));
#103400=DIRECTION('ref_axis',(1.,0.,0.));
#103401=DIRECTION('',(-0.190809912898503,0.,0.981627005099017));
#103402=DIRECTION('',(0.981627005099017,0.,0.190809912898503));
#103403=DIRECTION('',(-0.190809912898503,0.,0.981627005099017));
#103404=DIRECTION('',(0.981627005099017,0.,0.190809912898503));
#103405=DIRECTION('center_axis',(0.981627005099017,0.,0.190809912898503));
#103406=DIRECTION('ref_axis',(0.,-1.,0.));
#103407=DIRECTION('',(-0.190809912898503,0.,0.981627005099017));
#103408=DIRECTION('',(0.,-1.,0.));
#103409=DIRECTION('',(0.,-1.,0.));
#103410=DIRECTION('center_axis',(0.,-1.,0.));
#103411=DIRECTION('ref_axis',(0.,0.,-1.));
#103412=DIRECTION('',(-0.190809912898503,0.,0.981627005099017));
#103413=DIRECTION('',(-0.981627005099017,0.,-0.190809912898503));
#103414=DIRECTION('',(-0.981627005099017,0.,-0.190809912898503));
#103415=DIRECTION('center_axis',(-0.981627005099017,0.,-0.190809912898503));
#103416=DIRECTION('ref_axis',(-0.190809912898503,0.,0.981627005099017));
#103417=DIRECTION('',(0.,1.,0.));
#103418=DIRECTION('',(0.,1.,0.));
#103419=DIRECTION('center_axis',(0.,1.,0.));
#103420=DIRECTION('ref_axis',(1.,0.,0.));
#103421=DIRECTION('',(-0.190809912898503,0.,0.981627005099017));
#103422=DIRECTION('',(0.981627005099017,0.,0.190809912898503));
#103423=DIRECTION('',(-0.190809912898503,0.,0.981627005099017));
#103424=DIRECTION('',(0.981627005099017,0.,0.190809912898503));
#103425=DIRECTION('center_axis',(0.981627005099017,0.,0.190809912898503));
#103426=DIRECTION('ref_axis',(0.,-1.,0.));
#103427=DIRECTION('',(-0.190809912898503,0.,0.981627005099017));
#103428=DIRECTION('',(0.,-1.,0.));
#103429=DIRECTION('',(0.,-1.,0.));
#103430=DIRECTION('center_axis',(0.,-1.,0.));
#103431=DIRECTION('ref_axis',(0.,0.,-1.));
#103432=DIRECTION('',(-0.190809912898503,0.,0.981627005099017));
#103433=DIRECTION('',(-0.981627005099017,0.,-0.190809912898503));
#103434=DIRECTION('',(-0.981627005099017,0.,-0.190809912898503));
#103435=DIRECTION('center_axis',(-0.981627005099017,0.,-0.190809912898503));
#103436=DIRECTION('ref_axis',(-0.190809912898503,0.,0.981627005099017));
#103437=DIRECTION('',(0.,1.,0.));
#103438=DIRECTION('',(0.,1.,0.));
#103439=DIRECTION('center_axis',(0.,1.,0.));
#103440=DIRECTION('ref_axis',(1.,0.,0.));
#103441=DIRECTION('',(-0.190809912898503,0.,0.981627005099017));
#103442=DIRECTION('',(0.981627005099017,0.,0.190809912898503));
#103443=DIRECTION('',(-0.190809912898503,0.,0.981627005099017));
#103444=DIRECTION('',(0.981627005099017,0.,0.190809912898503));
#103445=DIRECTION('center_axis',(0.981627005099017,0.,0.190809912898503));
#103446=DIRECTION('ref_axis',(0.,-1.,0.));
#103447=DIRECTION('',(-0.190809912898503,0.,0.981627005099017));
#103448=DIRECTION('',(0.,-1.,0.));
#103449=DIRECTION('',(0.,-1.,0.));
#103450=DIRECTION('center_axis',(0.,-1.,0.));
#103451=DIRECTION('ref_axis',(0.,0.,-1.));
#103452=DIRECTION('',(-0.190809912898503,0.,0.981627005099017));
#103453=DIRECTION('',(-0.981627005099017,0.,-0.190809912898503));
#103454=DIRECTION('',(-0.981627005099017,0.,-0.190809912898503));
#103455=DIRECTION('center_axis',(-0.981627005099017,0.,-0.190809912898503));
#103456=DIRECTION('ref_axis',(-0.190809912898503,0.,0.981627005099017));
#103457=DIRECTION('',(0.,1.,0.));
#103458=DIRECTION('',(0.,1.,0.));
#103459=DIRECTION('center_axis',(0.,1.,0.));
#103460=DIRECTION('ref_axis',(1.,0.,0.));
#103461=DIRECTION('',(-0.190809912898503,0.,0.981627005099017));
#103462=DIRECTION('',(0.981627005099017,0.,0.190809912898503));
#103463=DIRECTION('',(-0.190809912898503,0.,0.981627005099017));
#103464=DIRECTION('',(0.981627005099017,0.,0.190809912898503));
#103465=DIRECTION('center_axis',(0.981627005099017,0.,0.190809912898503));
#103466=DIRECTION('ref_axis',(0.,-1.,0.));
#103467=DIRECTION('',(-0.190809912898503,0.,0.981627005099017));
#103468=DIRECTION('',(0.,-1.,0.));
#103469=DIRECTION('',(0.,-1.,0.));
#103470=DIRECTION('center_axis',(0.,-1.,0.));
#103471=DIRECTION('ref_axis',(0.,0.,-1.));
#103472=DIRECTION('',(-0.190809912898503,0.,0.981627005099017));
#103473=DIRECTION('',(-0.981627005099017,0.,-0.190809912898503));
#103474=DIRECTION('',(-0.981627005099017,0.,-0.190809912898503));
#103475=DIRECTION('center_axis',(-0.981627005099017,0.,-0.190809912898503));
#103476=DIRECTION('ref_axis',(-0.190809912898503,0.,0.981627005099017));
#103477=DIRECTION('',(0.,1.,0.));
#103478=DIRECTION('',(0.,1.,0.));
#103479=DIRECTION('center_axis',(0.,1.,0.));
#103480=DIRECTION('ref_axis',(1.,0.,0.));
#103481=DIRECTION('',(-0.190809912898503,0.,0.981627005099017));
#103482=DIRECTION('',(0.981627005099017,0.,0.190809912898503));
#103483=DIRECTION('',(-0.190809912898503,0.,0.981627005099017));
#103484=DIRECTION('',(0.981627005099017,0.,0.190809912898503));
#103485=DIRECTION('center_axis',(0.981627005099017,0.,0.190809912898503));
#103486=DIRECTION('ref_axis',(0.,-1.,0.));
#103487=DIRECTION('',(-0.190809912898503,0.,0.981627005099017));
#103488=DIRECTION('',(0.,-1.,0.));
#103489=DIRECTION('',(0.,-1.,0.));
#103490=DIRECTION('center_axis',(0.,-1.,0.));
#103491=DIRECTION('ref_axis',(0.,0.,-1.));
#103492=DIRECTION('',(-0.190809912898503,0.,0.981627005099017));
#103493=DIRECTION('',(-0.981627005099017,0.,-0.190809912898503));
#103494=DIRECTION('',(-0.981627005099017,0.,-0.190809912898503));
#103495=DIRECTION('center_axis',(-0.981627005099017,0.,-0.190809912898503));
#103496=DIRECTION('ref_axis',(-0.190809912898503,0.,0.981627005099017));
#103497=DIRECTION('',(0.,1.,0.));
#103498=DIRECTION('',(0.,1.,0.));
#103499=DIRECTION('center_axis',(0.,1.,0.));
#103500=DIRECTION('ref_axis',(1.,0.,0.));
#103501=DIRECTION('',(-0.190809912898503,0.,0.981627005099017));
#103502=DIRECTION('',(0.981627005099017,0.,0.190809912898503));
#103503=DIRECTION('',(-0.190809912898503,0.,0.981627005099017));
#103504=DIRECTION('',(0.981627005099017,0.,0.190809912898503));
#103505=DIRECTION('center_axis',(0.981627005099017,0.,0.190809912898503));
#103506=DIRECTION('ref_axis',(0.,-1.,0.));
#103507=DIRECTION('',(-0.190809912898503,0.,0.981627005099017));
#103508=DIRECTION('',(0.,-1.,0.));
#103509=DIRECTION('',(0.,-1.,0.));
#103510=DIRECTION('center_axis',(0.,-1.,0.));
#103511=DIRECTION('ref_axis',(0.,0.,-1.));
#103512=DIRECTION('',(-0.190809912898503,0.,0.981627005099017));
#103513=DIRECTION('',(-0.981627005099017,0.,-0.190809912898503));
#103514=DIRECTION('',(-0.981627005099017,0.,-0.190809912898503));
#103515=DIRECTION('center_axis',(-0.981627005099017,0.,-0.190809912898503));
#103516=DIRECTION('ref_axis',(-0.190809912898503,0.,0.981627005099017));
#103517=DIRECTION('',(0.,1.,0.));
#103518=DIRECTION('',(0.,1.,0.));
#103519=DIRECTION('center_axis',(0.,1.,0.));
#103520=DIRECTION('ref_axis',(1.,0.,0.));
#103521=DIRECTION('',(-0.190809912898503,0.,0.981627005099017));
#103522=DIRECTION('',(0.981627005099017,0.,0.190809912898503));
#103523=DIRECTION('',(-0.190809912898503,0.,0.981627005099017));
#103524=DIRECTION('',(0.981627005099017,0.,0.190809912898503));
#103525=DIRECTION('center_axis',(0.981627005099017,0.,0.190809912898503));
#103526=DIRECTION('ref_axis',(0.,-1.,0.));
#103527=DIRECTION('',(-0.190809912898503,0.,0.981627005099017));
#103528=DIRECTION('',(0.,-1.,0.));
#103529=DIRECTION('',(0.,-1.,0.));
#103530=DIRECTION('center_axis',(0.,-1.,0.));
#103531=DIRECTION('ref_axis',(0.,0.,-1.));
#103532=DIRECTION('',(-0.190809912898503,0.,0.981627005099017));
#103533=DIRECTION('',(-0.981627005099017,0.,-0.190809912898503));
#103534=DIRECTION('',(-0.981627005099017,0.,-0.190809912898503));
#103535=DIRECTION('center_axis',(-0.981627005099017,0.,-0.190809912898503));
#103536=DIRECTION('ref_axis',(-0.190809912898503,0.,0.981627005099017));
#103537=DIRECTION('',(0.,1.,0.));
#103538=DIRECTION('',(0.,1.,0.));
#103539=DIRECTION('center_axis',(0.,1.,0.));
#103540=DIRECTION('ref_axis',(1.,0.,0.));
#103541=DIRECTION('',(-0.190809912898503,0.,0.981627005099017));
#103542=DIRECTION('',(0.981627005099017,0.,0.190809912898503));
#103543=DIRECTION('',(-0.190809912898503,0.,0.981627005099017));
#103544=DIRECTION('',(0.981627005099017,0.,0.190809912898503));
#103545=DIRECTION('center_axis',(0.981627005099017,0.,0.190809912898503));
#103546=DIRECTION('ref_axis',(0.,-1.,0.));
#103547=DIRECTION('',(-0.190809912898503,0.,0.981627005099017));
#103548=DIRECTION('',(0.,-1.,0.));
#103549=DIRECTION('',(0.,-1.,0.));
#103550=DIRECTION('center_axis',(0.,-1.,0.));
#103551=DIRECTION('ref_axis',(0.,0.,-1.));
#103552=DIRECTION('',(-0.190809912898503,0.,0.981627005099017));
#103553=DIRECTION('',(-0.981627005099017,0.,-0.190809912898503));
#103554=DIRECTION('',(-0.981627005099017,0.,-0.190809912898503));
#103555=DIRECTION('center_axis',(-0.981627005099017,0.,-0.190809912898503));
#103556=DIRECTION('ref_axis',(-0.190809912898503,0.,0.981627005099017));
#103557=DIRECTION('',(0.,1.,0.));
#103558=DIRECTION('',(0.,1.,0.));
#103559=DIRECTION('center_axis',(0.,1.,0.));
#103560=DIRECTION('ref_axis',(1.,0.,0.));
#103561=DIRECTION('',(-0.190809912898503,0.,0.981627005099017));
#103562=DIRECTION('',(0.981627005099017,0.,0.190809912898503));
#103563=DIRECTION('',(-0.190809912898503,0.,0.981627005099017));
#103564=DIRECTION('',(0.981627005099017,0.,0.190809912898503));
#103565=DIRECTION('center_axis',(0.981627005099017,0.,0.190809912898503));
#103566=DIRECTION('ref_axis',(0.,-1.,0.));
#103567=DIRECTION('',(-0.190809912898503,0.,0.981627005099017));
#103568=DIRECTION('',(0.,-1.,0.));
#103569=DIRECTION('',(0.,-1.,0.));
#103570=DIRECTION('center_axis',(0.,-1.,0.));
#103571=DIRECTION('ref_axis',(0.,0.,-1.));
#103572=DIRECTION('',(-0.190809912898503,0.,0.981627005099017));
#103573=DIRECTION('',(-0.981627005099017,0.,-0.190809912898503));
#103574=DIRECTION('',(-0.981627005099017,0.,-0.190809912898503));
#103575=DIRECTION('center_axis',(-0.981627005099017,0.,-0.190809912898503));
#103576=DIRECTION('ref_axis',(-0.190809912898503,0.,0.981627005099017));
#103577=DIRECTION('',(0.,1.,0.));
#103578=DIRECTION('',(0.,1.,0.));
#103579=DIRECTION('center_axis',(0.,1.,0.));
#103580=DIRECTION('ref_axis',(1.,0.,0.));
#103581=DIRECTION('',(-0.190809912898503,0.,0.981627005099017));
#103582=DIRECTION('',(0.981627005099017,0.,0.190809912898503));
#103583=DIRECTION('',(-0.190809912898503,0.,0.981627005099017));
#103584=DIRECTION('',(0.981627005099017,0.,0.190809912898503));
#103585=DIRECTION('center_axis',(0.981627005099017,0.,0.190809912898503));
#103586=DIRECTION('ref_axis',(0.,-1.,0.));
#103587=DIRECTION('',(-0.190809912898503,0.,0.981627005099017));
#103588=DIRECTION('',(0.,-1.,0.));
#103589=DIRECTION('',(0.,-1.,0.));
#103590=DIRECTION('center_axis',(0.,-1.,0.));
#103591=DIRECTION('ref_axis',(0.,0.,-1.));
#103592=DIRECTION('',(-0.190809912898503,0.,0.981627005099017));
#103593=DIRECTION('',(-0.981627005099017,0.,-0.190809912898503));
#103594=DIRECTION('',(-0.981627005099017,0.,-0.190809912898503));
#103595=DIRECTION('center_axis',(-0.981627005099017,0.,-0.190809912898503));
#103596=DIRECTION('ref_axis',(-0.190809912898503,0.,0.981627005099017));
#103597=DIRECTION('',(0.,1.,0.));
#103598=DIRECTION('',(0.,1.,0.));
#103599=DIRECTION('center_axis',(0.,1.,0.));
#103600=DIRECTION('ref_axis',(1.,0.,0.));
#103601=DIRECTION('',(-0.190809912898503,0.,0.981627005099017));
#103602=DIRECTION('',(0.981627005099017,0.,0.190809912898503));
#103603=DIRECTION('',(-0.190809912898503,0.,0.981627005099017));
#103604=DIRECTION('',(0.981627005099017,0.,0.190809912898503));
#103605=DIRECTION('center_axis',(0.981627005099017,0.,0.190809912898503));
#103606=DIRECTION('ref_axis',(0.,-1.,0.));
#103607=DIRECTION('',(-0.190809912898503,0.,0.981627005099017));
#103608=DIRECTION('',(0.,-1.,0.));
#103609=DIRECTION('',(0.,-1.,0.));
#103610=DIRECTION('center_axis',(0.,-1.,0.));
#103611=DIRECTION('ref_axis',(0.,0.,-1.));
#103612=DIRECTION('',(-0.190809912898503,0.,0.981627005099017));
#103613=DIRECTION('',(-0.981627005099017,0.,-0.190809912898503));
#103614=DIRECTION('',(-0.981627005099017,0.,-0.190809912898503));
#103615=DIRECTION('center_axis',(-0.981627005099017,0.,-0.190809912898503));
#103616=DIRECTION('ref_axis',(-0.190809912898503,0.,0.981627005099017));
#103617=DIRECTION('',(0.,1.,0.));
#103618=DIRECTION('',(0.,1.,0.));
#103619=DIRECTION('center_axis',(0.,1.,0.));
#103620=DIRECTION('ref_axis',(1.,0.,0.));
#103621=DIRECTION('',(-0.190809912898503,0.,0.981627005099017));
#103622=DIRECTION('',(0.981627005099017,0.,0.190809912898503));
#103623=DIRECTION('',(-0.190809912898503,0.,0.981627005099017));
#103624=DIRECTION('',(0.981627005099017,0.,0.190809912898503));
#103625=DIRECTION('center_axis',(0.981627005099017,0.,0.190809912898503));
#103626=DIRECTION('ref_axis',(0.,-1.,0.));
#103627=DIRECTION('',(-0.190809912898503,0.,0.981627005099017));
#103628=DIRECTION('',(0.,-1.,0.));
#103629=DIRECTION('',(0.,-1.,0.));
#103630=DIRECTION('center_axis',(0.,-1.,0.));
#103631=DIRECTION('ref_axis',(0.,0.,-1.));
#103632=DIRECTION('',(-0.190809912898503,0.,0.981627005099017));
#103633=DIRECTION('',(-0.981627005099017,0.,-0.190809912898503));
#103634=DIRECTION('',(-0.981627005099017,0.,-0.190809912898503));
#103635=DIRECTION('center_axis',(-0.981627005099017,0.,-0.190809912898503));
#103636=DIRECTION('ref_axis',(-0.190809912898503,0.,0.981627005099017));
#103637=DIRECTION('',(0.,1.,0.));
#103638=DIRECTION('',(0.,1.,0.));
#103639=DIRECTION('center_axis',(0.,1.,0.));
#103640=DIRECTION('ref_axis',(1.,0.,0.));
#103641=DIRECTION('',(-0.190809912898503,0.,0.981627005099017));
#103642=DIRECTION('',(0.981627005099017,0.,0.190809912898503));
#103643=DIRECTION('',(-0.190809912898503,0.,0.981627005099017));
#103644=DIRECTION('',(0.981627005099017,0.,0.190809912898503));
#103645=DIRECTION('center_axis',(0.981627005099017,0.,0.190809912898503));
#103646=DIRECTION('ref_axis',(0.,-1.,0.));
#103647=DIRECTION('',(-0.190809912898503,0.,0.981627005099017));
#103648=DIRECTION('',(0.,-1.,0.));
#103649=DIRECTION('',(0.,-1.,0.));
#103650=DIRECTION('center_axis',(0.,-1.,0.));
#103651=DIRECTION('ref_axis',(0.,0.,-1.));
#103652=DIRECTION('',(-0.190809912898503,0.,0.981627005099017));
#103653=DIRECTION('',(-0.981627005099017,0.,-0.190809912898503));
#103654=DIRECTION('',(-0.981627005099017,0.,-0.190809912898503));
#103655=DIRECTION('center_axis',(-0.981627005099017,0.,-0.190809912898503));
#103656=DIRECTION('ref_axis',(-0.190809912898503,0.,0.981627005099017));
#103657=DIRECTION('',(0.,1.,0.));
#103658=DIRECTION('',(0.,1.,0.));
#103659=DIRECTION('center_axis',(0.,1.,0.));
#103660=DIRECTION('ref_axis',(1.,0.,0.));
#103661=DIRECTION('',(-0.190809912898503,0.,0.981627005099017));
#103662=DIRECTION('',(0.981627005099017,0.,0.190809912898503));
#103663=DIRECTION('',(-0.190809912898503,0.,0.981627005099017));
#103664=DIRECTION('',(0.981627005099017,0.,0.190809912898503));
#103665=DIRECTION('center_axis',(0.981627005099017,0.,0.190809912898503));
#103666=DIRECTION('ref_axis',(0.,-1.,0.));
#103667=DIRECTION('',(-0.190809912898503,0.,0.981627005099017));
#103668=DIRECTION('',(0.,-1.,0.));
#103669=DIRECTION('',(0.,-1.,0.));
#103670=DIRECTION('center_axis',(0.,-1.,0.));
#103671=DIRECTION('ref_axis',(0.,0.,-1.));
#103672=DIRECTION('',(-0.190809912898503,0.,0.981627005099017));
#103673=DIRECTION('',(-0.981627005099017,0.,-0.190809912898503));
#103674=DIRECTION('',(-0.981627005099017,0.,-0.190809912898503));
#103675=DIRECTION('center_axis',(-0.981627005099017,0.,-0.190809912898503));
#103676=DIRECTION('ref_axis',(-0.190809912898503,0.,0.981627005099017));
#103677=DIRECTION('',(0.,1.,0.));
#103678=DIRECTION('',(0.,1.,0.));
#103679=DIRECTION('center_axis',(0.,1.,0.));
#103680=DIRECTION('ref_axis',(1.,0.,0.));
#103681=DIRECTION('',(-0.190809912898503,0.,0.981627005099017));
#103682=DIRECTION('',(0.981627005099017,0.,0.190809912898503));
#103683=DIRECTION('',(-0.190809912898503,0.,0.981627005099017));
#103684=DIRECTION('',(0.981627005099017,0.,0.190809912898503));
#103685=DIRECTION('center_axis',(0.981627005099017,0.,0.190809912898503));
#103686=DIRECTION('ref_axis',(0.,-1.,0.));
#103687=DIRECTION('',(-0.190809912898503,0.,0.981627005099017));
#103688=DIRECTION('',(0.,-1.,0.));
#103689=DIRECTION('',(0.,-1.,0.));
#103690=DIRECTION('center_axis',(0.,-1.,0.));
#103691=DIRECTION('ref_axis',(0.,0.,-1.));
#103692=DIRECTION('',(-0.190809912898503,0.,0.981627005099017));
#103693=DIRECTION('',(-0.981627005099017,0.,-0.190809912898503));
#103694=DIRECTION('',(-0.981627005099017,0.,-0.190809912898503));
#103695=DIRECTION('center_axis',(-0.981627005099017,0.,-0.190809912898503));
#103696=DIRECTION('ref_axis',(-0.190809912898503,0.,0.981627005099017));
#103697=DIRECTION('',(0.,1.,0.));
#103698=DIRECTION('',(0.,1.,0.));
#103699=DIRECTION('center_axis',(0.,1.,0.));
#103700=DIRECTION('ref_axis',(1.,0.,0.));
#103701=DIRECTION('',(-0.190809912898503,0.,0.981627005099017));
#103702=DIRECTION('',(0.981627005099017,0.,0.190809912898503));
#103703=DIRECTION('',(-0.190809912898503,0.,0.981627005099017));
#103704=DIRECTION('',(0.981627005099017,0.,0.190809912898503));
#103705=DIRECTION('center_axis',(0.981627005099017,0.,0.190809912898503));
#103706=DIRECTION('ref_axis',(0.,-1.,0.));
#103707=DIRECTION('',(-0.190809912898503,0.,0.981627005099017));
#103708=DIRECTION('',(0.,-1.,0.));
#103709=DIRECTION('',(0.,-1.,0.));
#103710=DIRECTION('center_axis',(0.,-1.,0.));
#103711=DIRECTION('ref_axis',(0.,0.,-1.));
#103712=DIRECTION('',(-0.190809912898503,0.,0.981627005099017));
#103713=DIRECTION('',(-0.981627005099017,0.,-0.190809912898503));
#103714=DIRECTION('',(-0.981627005099017,0.,-0.190809912898503));
#103715=DIRECTION('center_axis',(-0.981627005099017,0.,-0.190809912898503));
#103716=DIRECTION('ref_axis',(-0.190809912898503,0.,0.981627005099017));
#103717=DIRECTION('',(0.,1.,0.));
#103718=DIRECTION('',(0.,1.,0.));
#103719=DIRECTION('center_axis',(0.,1.,0.));
#103720=DIRECTION('ref_axis',(1.,0.,0.));
#103721=DIRECTION('',(-0.190809912898503,0.,0.981627005099017));
#103722=DIRECTION('',(0.981627005099017,0.,0.190809912898503));
#103723=DIRECTION('',(-0.190809912898503,0.,0.981627005099017));
#103724=DIRECTION('',(0.981627005099017,0.,0.190809912898503));
#103725=DIRECTION('center_axis',(0.981627005099017,0.,0.190809912898503));
#103726=DIRECTION('ref_axis',(0.,-1.,0.));
#103727=DIRECTION('',(-0.190809912898503,0.,0.981627005099017));
#103728=DIRECTION('',(0.,-1.,0.));
#103729=DIRECTION('',(0.,-1.,0.));
#103730=DIRECTION('center_axis',(0.,-1.,0.));
#103731=DIRECTION('ref_axis',(0.,0.,-1.));
#103732=DIRECTION('',(-0.190809912898503,0.,0.981627005099017));
#103733=DIRECTION('',(-0.981627005099017,0.,-0.190809912898503));
#103734=DIRECTION('',(-0.981627005099017,0.,-0.190809912898503));
#103735=DIRECTION('center_axis',(-0.981627005099017,0.,-0.190809912898503));
#103736=DIRECTION('ref_axis',(-0.190809912898503,0.,0.981627005099017));
#103737=DIRECTION('',(0.,1.,0.));
#103738=DIRECTION('',(0.,1.,0.));
#103739=DIRECTION('center_axis',(0.,1.,0.));
#103740=DIRECTION('ref_axis',(1.,0.,0.));
#103741=DIRECTION('',(-0.190809912898503,0.,0.981627005099017));
#103742=DIRECTION('',(0.981627005099017,0.,0.190809912898503));
#103743=DIRECTION('',(-0.190809912898503,0.,0.981627005099017));
#103744=DIRECTION('',(0.981627005099017,0.,0.190809912898503));
#103745=DIRECTION('center_axis',(0.981627005099017,0.,0.190809912898503));
#103746=DIRECTION('ref_axis',(0.,-1.,0.));
#103747=DIRECTION('',(-0.190809912898503,0.,0.981627005099017));
#103748=DIRECTION('',(0.,-1.,0.));
#103749=DIRECTION('',(0.,-1.,0.));
#103750=DIRECTION('center_axis',(0.,-1.,0.));
#103751=DIRECTION('ref_axis',(0.,0.,-1.));
#103752=DIRECTION('',(-0.190809912898503,0.,0.981627005099017));
#103753=DIRECTION('',(-0.981627005099017,0.,-0.190809912898503));
#103754=DIRECTION('',(-0.981627005099017,0.,-0.190809912898503));
#103755=DIRECTION('center_axis',(-0.981627005099017,0.,-0.190809912898503));
#103756=DIRECTION('ref_axis',(-0.190809912898503,0.,0.981627005099017));
#103757=DIRECTION('',(0.,1.,0.));
#103758=DIRECTION('',(0.,1.,0.));
#103759=DIRECTION('center_axis',(0.,1.,0.));
#103760=DIRECTION('ref_axis',(1.,0.,0.));
#103761=DIRECTION('',(-0.190809912898503,0.,0.981627005099017));
#103762=DIRECTION('',(0.981627005099017,0.,0.190809912898503));
#103763=DIRECTION('',(-0.190809912898503,0.,0.981627005099017));
#103764=DIRECTION('',(0.981627005099017,0.,0.190809912898503));
#103765=DIRECTION('center_axis',(0.981627005099017,0.,0.190809912898503));
#103766=DIRECTION('ref_axis',(0.,-1.,0.));
#103767=DIRECTION('',(-0.190809912898503,0.,0.981627005099017));
#103768=DIRECTION('',(0.,-1.,0.));
#103769=DIRECTION('',(0.,-1.,0.));
#103770=DIRECTION('center_axis',(0.,-1.,0.));
#103771=DIRECTION('ref_axis',(0.,0.,-1.));
#103772=DIRECTION('',(-0.190809912898503,0.,0.981627005099017));
#103773=DIRECTION('',(-0.981627005099017,0.,-0.190809912898503));
#103774=DIRECTION('',(-0.981627005099017,0.,-0.190809912898503));
#103775=DIRECTION('center_axis',(-0.981627005099017,0.,-0.190809912898503));
#103776=DIRECTION('ref_axis',(-0.190809912898503,0.,0.981627005099017));
#103777=DIRECTION('',(0.,1.,0.));
#103778=DIRECTION('',(0.,1.,0.));
#103779=DIRECTION('center_axis',(0.,1.,0.));
#103780=DIRECTION('ref_axis',(1.,0.,0.));
#103781=DIRECTION('',(-0.190809912898503,0.,0.981627005099017));
#103782=DIRECTION('',(0.981627005099017,0.,0.190809912898503));
#103783=DIRECTION('',(-0.190809912898503,0.,0.981627005099017));
#103784=DIRECTION('',(0.981627005099017,0.,0.190809912898503));
#103785=DIRECTION('center_axis',(0.981627005099017,0.,0.190809912898503));
#103786=DIRECTION('ref_axis',(0.,-1.,0.));
#103787=DIRECTION('',(-0.190809912898503,0.,0.981627005099017));
#103788=DIRECTION('',(0.,-1.,0.));
#103789=DIRECTION('',(0.,-1.,0.));
#103790=DIRECTION('center_axis',(0.,-1.,0.));
#103791=DIRECTION('ref_axis',(0.,0.,-1.));
#103792=DIRECTION('',(-0.190809912898503,0.,0.981627005099017));
#103793=DIRECTION('',(-0.981627005099017,0.,-0.190809912898503));
#103794=DIRECTION('',(-0.981627005099017,0.,-0.190809912898503));
#103795=DIRECTION('center_axis',(-0.981627005099017,0.,-0.190809912898503));
#103796=DIRECTION('ref_axis',(-0.190809912898503,0.,0.981627005099017));
#103797=DIRECTION('',(0.,1.,0.));
#103798=DIRECTION('',(0.,1.,0.));
#103799=DIRECTION('center_axis',(0.,1.,0.));
#103800=DIRECTION('ref_axis',(1.,0.,0.));
#103801=DIRECTION('',(-0.190809912898503,0.,0.981627005099017));
#103802=DIRECTION('',(0.981627005099017,0.,0.190809912898503));
#103803=DIRECTION('',(-0.190809912898503,0.,0.981627005099017));
#103804=DIRECTION('',(0.981627005099017,0.,0.190809912898503));
#103805=DIRECTION('center_axis',(0.981627005099017,0.,0.190809912898503));
#103806=DIRECTION('ref_axis',(0.,-1.,0.));
#103807=DIRECTION('',(-0.190809912898503,0.,0.981627005099017));
#103808=DIRECTION('',(0.,-1.,0.));
#103809=DIRECTION('',(0.,-1.,0.));
#103810=DIRECTION('center_axis',(0.,-1.,0.));
#103811=DIRECTION('ref_axis',(0.,0.,-1.));
#103812=DIRECTION('',(-0.190809912898503,0.,0.981627005099017));
#103813=DIRECTION('',(-0.981627005099017,0.,-0.190809912898503));
#103814=DIRECTION('',(-0.981627005099017,0.,-0.190809912898503));
#103815=DIRECTION('center_axis',(-0.981627005099017,0.,-0.190809912898503));
#103816=DIRECTION('ref_axis',(-0.190809912898503,0.,0.981627005099017));
#103817=DIRECTION('',(0.,1.,0.));
#103818=DIRECTION('',(0.,1.,0.));
#103819=DIRECTION('center_axis',(0.,1.,0.));
#103820=DIRECTION('ref_axis',(1.,0.,0.));
#103821=DIRECTION('',(-0.190809912898503,0.,0.981627005099017));
#103822=DIRECTION('',(0.981627005099017,0.,0.190809912898503));
#103823=DIRECTION('',(-0.190809912898503,0.,0.981627005099017));
#103824=DIRECTION('',(0.981627005099017,0.,0.190809912898503));
#103825=DIRECTION('center_axis',(0.981627005099017,0.,0.190809912898503));
#103826=DIRECTION('ref_axis',(0.,-1.,0.));
#103827=DIRECTION('',(-0.190809912898503,0.,0.981627005099017));
#103828=DIRECTION('',(0.,-1.,0.));
#103829=DIRECTION('',(0.,-1.,0.));
#103830=DIRECTION('center_axis',(0.,-1.,0.));
#103831=DIRECTION('ref_axis',(0.,0.,-1.));
#103832=DIRECTION('',(-0.190809912898503,0.,0.981627005099017));
#103833=DIRECTION('',(-0.981627005099017,0.,-0.190809912898503));
#103834=DIRECTION('',(-0.981627005099017,0.,-0.190809912898503));
#103835=DIRECTION('center_axis',(-0.981627005099017,0.,-0.190809912898503));
#103836=DIRECTION('ref_axis',(-0.190809912898503,0.,0.981627005099017));
#103837=DIRECTION('',(0.,1.,0.));
#103838=DIRECTION('',(0.,1.,0.));
#103839=DIRECTION('center_axis',(0.,1.,0.));
#103840=DIRECTION('ref_axis',(1.,0.,0.));
#103841=DIRECTION('',(-0.190809912898503,0.,0.981627005099017));
#103842=DIRECTION('',(0.981627005099017,0.,0.190809912898503));
#103843=DIRECTION('',(-0.190809912898503,0.,0.981627005099017));
#103844=DIRECTION('',(0.981627005099017,0.,0.190809912898503));
#103845=DIRECTION('center_axis',(0.981627005099017,0.,0.190809912898503));
#103846=DIRECTION('ref_axis',(0.,-1.,0.));
#103847=DIRECTION('',(-0.190809912898503,0.,0.981627005099017));
#103848=DIRECTION('',(0.,-1.,0.));
#103849=DIRECTION('',(0.,-1.,0.));
#103850=DIRECTION('center_axis',(0.,-1.,0.));
#103851=DIRECTION('ref_axis',(0.,0.,-1.));
#103852=DIRECTION('',(-0.190809912898503,0.,0.981627005099017));
#103853=DIRECTION('',(-0.981627005099017,0.,-0.190809912898503));
#103854=DIRECTION('',(-0.981627005099017,0.,-0.190809912898503));
#103855=DIRECTION('center_axis',(-0.981627005099017,0.,-0.190809912898503));
#103856=DIRECTION('ref_axis',(-0.190809912898503,0.,0.981627005099017));
#103857=DIRECTION('',(0.,1.,0.));
#103858=DIRECTION('',(0.,1.,0.));
#103859=DIRECTION('center_axis',(0.,1.,0.));
#103860=DIRECTION('ref_axis',(1.,0.,0.));
#103861=DIRECTION('',(-0.190809912898503,0.,0.981627005099017));
#103862=DIRECTION('',(0.981627005099017,0.,0.190809912898503));
#103863=DIRECTION('',(-0.190809912898503,0.,0.981627005099017));
#103864=DIRECTION('',(0.981627005099017,0.,0.190809912898503));
#103865=DIRECTION('center_axis',(0.981627005099017,0.,0.190809912898503));
#103866=DIRECTION('ref_axis',(0.,-1.,0.));
#103867=DIRECTION('',(-0.190809912898503,0.,0.981627005099017));
#103868=DIRECTION('',(0.,-1.,0.));
#103869=DIRECTION('',(0.,-1.,0.));
#103870=DIRECTION('center_axis',(0.,-1.,0.));
#103871=DIRECTION('ref_axis',(0.,0.,-1.));
#103872=DIRECTION('',(-0.190809912898503,0.,0.981627005099017));
#103873=DIRECTION('',(-0.981627005099017,0.,-0.190809912898503));
#103874=DIRECTION('',(-0.981627005099017,0.,-0.190809912898503));
#103875=DIRECTION('center_axis',(-0.981627005099017,0.,-0.190809912898503));
#103876=DIRECTION('ref_axis',(-0.190809912898503,0.,0.981627005099017));
#103877=DIRECTION('',(0.,1.,0.));
#103878=DIRECTION('',(0.,1.,0.));
#103879=DIRECTION('center_axis',(0.,1.,0.));
#103880=DIRECTION('ref_axis',(1.,0.,0.));
#103881=DIRECTION('',(-0.190809912898503,0.,0.981627005099017));
#103882=DIRECTION('',(0.981627005099017,0.,0.190809912898503));
#103883=DIRECTION('',(-0.190809912898503,0.,0.981627005099017));
#103884=DIRECTION('',(0.981627005099017,0.,0.190809912898503));
#103885=DIRECTION('center_axis',(0.981627005099017,0.,0.190809912898503));
#103886=DIRECTION('ref_axis',(0.,-1.,0.));
#103887=DIRECTION('',(-0.190809912898503,0.,0.981627005099017));
#103888=DIRECTION('',(0.,-1.,0.));
#103889=DIRECTION('',(0.,-1.,0.));
#103890=DIRECTION('center_axis',(0.,-1.,0.));
#103891=DIRECTION('ref_axis',(0.,0.,-1.));
#103892=DIRECTION('',(-0.190809912898503,0.,0.981627005099017));
#103893=DIRECTION('',(-0.981627005099017,0.,-0.190809912898503));
#103894=DIRECTION('',(-0.981627005099017,0.,-0.190809912898503));
#103895=DIRECTION('center_axis',(-0.981627005099017,0.,-0.190809912898503));
#103896=DIRECTION('ref_axis',(-0.190809912898503,0.,0.981627005099017));
#103897=DIRECTION('',(0.,1.,0.));
#103898=DIRECTION('',(0.,1.,0.));
#103899=DIRECTION('center_axis',(0.,1.,0.));
#103900=DIRECTION('ref_axis',(1.,0.,0.));
#103901=DIRECTION('',(-0.190809912898503,0.,0.981627005099017));
#103902=DIRECTION('',(0.981627005099017,0.,0.190809912898503));
#103903=DIRECTION('',(-0.190809912898503,0.,0.981627005099017));
#103904=DIRECTION('',(0.981627005099017,0.,0.190809912898503));
#103905=DIRECTION('center_axis',(0.981627005099017,0.,0.190809912898503));
#103906=DIRECTION('ref_axis',(0.,-1.,0.));
#103907=DIRECTION('',(-0.190809912898503,0.,0.981627005099017));
#103908=DIRECTION('',(0.,-1.,0.));
#103909=DIRECTION('',(0.,-1.,0.));
#103910=DIRECTION('center_axis',(0.,-1.,0.));
#103911=DIRECTION('ref_axis',(0.,0.,-1.));
#103912=DIRECTION('',(-0.190809912898503,0.,0.981627005099017));
#103913=DIRECTION('',(-0.981627005099017,0.,-0.190809912898503));
#103914=DIRECTION('',(-0.981627005099017,0.,-0.190809912898503));
#103915=DIRECTION('center_axis',(-0.981627005099017,0.,-0.190809912898503));
#103916=DIRECTION('ref_axis',(-0.190809912898503,0.,0.981627005099017));
#103917=DIRECTION('',(0.,1.,0.));
#103918=DIRECTION('',(0.,1.,0.));
#103919=DIRECTION('center_axis',(0.,1.,0.));
#103920=DIRECTION('ref_axis',(1.,0.,0.));
#103921=DIRECTION('',(-0.190809912898503,0.,0.981627005099017));
#103922=DIRECTION('',(0.981627005099017,0.,0.190809912898503));
#103923=DIRECTION('',(-0.190809912898503,0.,0.981627005099017));
#103924=DIRECTION('',(0.981627005099017,0.,0.190809912898503));
#103925=DIRECTION('center_axis',(0.981627005099017,0.,0.190809912898503));
#103926=DIRECTION('ref_axis',(0.,-1.,0.));
#103927=DIRECTION('',(-0.190809912898503,0.,0.981627005099017));
#103928=DIRECTION('',(0.,-1.,0.));
#103929=DIRECTION('',(0.,-1.,0.));
#103930=DIRECTION('center_axis',(0.,-1.,0.));
#103931=DIRECTION('ref_axis',(0.,0.,-1.));
#103932=DIRECTION('',(-0.190809912898503,0.,0.981627005099017));
#103933=DIRECTION('',(-0.981627005099017,0.,-0.190809912898503));
#103934=DIRECTION('',(-0.981627005099017,0.,-0.190809912898503));
#103935=DIRECTION('center_axis',(-0.981627005099017,0.,-0.190809912898503));
#103936=DIRECTION('ref_axis',(-0.190809912898503,0.,0.981627005099017));
#103937=DIRECTION('',(0.,1.,0.));
#103938=DIRECTION('',(0.,1.,0.));
#103939=DIRECTION('center_axis',(0.,1.,0.));
#103940=DIRECTION('ref_axis',(1.,0.,0.));
#103941=DIRECTION('',(-0.190809912898503,0.,0.981627005099017));
#103942=DIRECTION('',(0.981627005099017,0.,0.190809912898503));
#103943=DIRECTION('',(-0.190809912898503,0.,0.981627005099017));
#103944=DIRECTION('',(0.981627005099017,0.,0.190809912898503));
#103945=DIRECTION('center_axis',(0.981627005099017,0.,0.190809912898503));
#103946=DIRECTION('ref_axis',(0.,-1.,0.));
#103947=DIRECTION('',(-0.190809912898503,0.,0.981627005099017));
#103948=DIRECTION('',(0.,-1.,0.));
#103949=DIRECTION('',(0.,-1.,0.));
#103950=DIRECTION('center_axis',(0.,-1.,0.));
#103951=DIRECTION('ref_axis',(0.,0.,-1.));
#103952=DIRECTION('',(-0.190809912898503,0.,0.981627005099017));
#103953=DIRECTION('',(-0.981627005099017,0.,-0.190809912898503));
#103954=DIRECTION('',(-0.981627005099017,0.,-0.190809912898503));
#103955=DIRECTION('center_axis',(-0.981627005099017,0.,-0.190809912898503));
#103956=DIRECTION('ref_axis',(-0.190809912898503,0.,0.981627005099017));
#103957=DIRECTION('',(0.,1.,0.));
#103958=DIRECTION('',(0.,1.,0.));
#103959=DIRECTION('center_axis',(0.,1.,0.));
#103960=DIRECTION('ref_axis',(1.,0.,0.));
#103961=DIRECTION('',(-0.190809912898503,0.,0.981627005099017));
#103962=DIRECTION('',(0.981627005099017,0.,0.190809912898503));
#103963=DIRECTION('',(-0.190809912898503,0.,0.981627005099017));
#103964=DIRECTION('',(0.981627005099017,0.,0.190809912898503));
#103965=DIRECTION('center_axis',(0.981627005099017,0.,0.190809912898503));
#103966=DIRECTION('ref_axis',(0.,-1.,0.));
#103967=DIRECTION('',(-0.190809912898503,0.,0.981627005099017));
#103968=DIRECTION('',(0.,-1.,0.));
#103969=DIRECTION('',(0.,-1.,0.));
#103970=DIRECTION('center_axis',(0.,-1.,0.));
#103971=DIRECTION('ref_axis',(0.,0.,-1.));
#103972=DIRECTION('',(-0.190809912898503,0.,0.981627005099017));
#103973=DIRECTION('',(-0.981627005099017,0.,-0.190809912898503));
#103974=DIRECTION('',(-0.981627005099017,0.,-0.190809912898503));
#103975=DIRECTION('center_axis',(-0.981627005099017,0.,-0.190809912898503));
#103976=DIRECTION('ref_axis',(-0.190809912898503,0.,0.981627005099017));
#103977=DIRECTION('',(0.,1.,0.));
#103978=DIRECTION('',(0.,1.,0.));
#103979=DIRECTION('center_axis',(0.,1.,0.));
#103980=DIRECTION('ref_axis',(1.,0.,0.));
#103981=DIRECTION('',(-0.190809912898503,0.,0.981627005099017));
#103982=DIRECTION('',(0.981627005099017,0.,0.190809912898503));
#103983=DIRECTION('',(-0.190809912898503,0.,0.981627005099017));
#103984=DIRECTION('',(0.981627005099017,0.,0.190809912898503));
#103985=DIRECTION('center_axis',(0.981627005099017,0.,0.190809912898503));
#103986=DIRECTION('ref_axis',(0.,-1.,0.));
#103987=DIRECTION('',(-0.190809912898503,0.,0.981627005099017));
#103988=DIRECTION('',(0.,-1.,0.));
#103989=DIRECTION('',(0.,-1.,0.));
#103990=DIRECTION('center_axis',(0.,-1.,0.));
#103991=DIRECTION('ref_axis',(0.,0.,-1.));
#103992=DIRECTION('',(-0.190809912898503,0.,0.981627005099017));
#103993=DIRECTION('',(-0.981627005099017,0.,-0.190809912898503));
#103994=DIRECTION('',(-0.981627005099017,0.,-0.190809912898503));
#103995=DIRECTION('center_axis',(-0.981627005099017,0.,-0.190809912898503));
#103996=DIRECTION('ref_axis',(-0.190809912898503,0.,0.981627005099017));
#103997=DIRECTION('',(0.,1.,0.));
#103998=DIRECTION('',(0.,1.,0.));
#103999=DIRECTION('center_axis',(0.,1.,0.));
#104000=DIRECTION('ref_axis',(1.,0.,0.));
#104001=DIRECTION('',(-0.190809912898503,0.,0.981627005099017));
#104002=DIRECTION('',(0.981627005099017,0.,0.190809912898503));
#104003=DIRECTION('',(-0.190809912898503,0.,0.981627005099017));
#104004=DIRECTION('',(0.981627005099017,0.,0.190809912898503));
#104005=DIRECTION('center_axis',(0.981627005099017,0.,0.190809912898503));
#104006=DIRECTION('ref_axis',(0.,-1.,0.));
#104007=DIRECTION('',(-0.190809912898503,0.,0.981627005099017));
#104008=DIRECTION('',(0.,-1.,0.));
#104009=DIRECTION('',(0.,-1.,0.));
#104010=DIRECTION('center_axis',(0.,-1.,0.));
#104011=DIRECTION('ref_axis',(0.,0.,-1.));
#104012=DIRECTION('',(-0.190809912898503,0.,0.981627005099017));
#104013=DIRECTION('',(-0.981627005099017,0.,-0.190809912898503));
#104014=DIRECTION('',(-0.981627005099017,0.,-0.190809912898503));
#104015=DIRECTION('center_axis',(-0.981627005099017,0.,-0.190809912898503));
#104016=DIRECTION('ref_axis',(-0.190809912898503,0.,0.981627005099017));
#104017=DIRECTION('',(0.,1.,0.));
#104018=DIRECTION('',(0.,1.,0.));
#104019=DIRECTION('center_axis',(0.,1.,0.));
#104020=DIRECTION('ref_axis',(1.,0.,0.));
#104021=DIRECTION('',(-0.190809912898503,0.,0.981627005099017));
#104022=DIRECTION('',(0.981627005099017,0.,0.190809912898503));
#104023=DIRECTION('',(-0.190809912898503,0.,0.981627005099017));
#104024=DIRECTION('',(0.981627005099017,0.,0.190809912898503));
#104025=DIRECTION('center_axis',(0.981627005099017,0.,0.190809912898503));
#104026=DIRECTION('ref_axis',(0.,-1.,0.));
#104027=DIRECTION('',(-0.190809912898503,0.,0.981627005099017));
#104028=DIRECTION('',(0.,-1.,0.));
#104029=DIRECTION('',(0.,-1.,0.));
#104030=DIRECTION('center_axis',(0.,-1.,0.));
#104031=DIRECTION('ref_axis',(0.,0.,-1.));
#104032=DIRECTION('',(-0.190809912898503,0.,0.981627005099017));
#104033=DIRECTION('',(-0.981627005099017,0.,-0.190809912898503));
#104034=DIRECTION('',(-0.981627005099017,0.,-0.190809912898503));
#104035=DIRECTION('center_axis',(-0.981627005099017,0.,-0.190809912898503));
#104036=DIRECTION('ref_axis',(-0.190809912898503,0.,0.981627005099017));
#104037=DIRECTION('',(0.,1.,0.));
#104038=DIRECTION('',(0.,1.,0.));
#104039=DIRECTION('center_axis',(0.,1.,0.));
#104040=DIRECTION('ref_axis',(1.,0.,0.));
#104041=DIRECTION('',(-0.190809912898503,0.,0.981627005099017));
#104042=DIRECTION('',(0.981627005099017,0.,0.190809912898503));
#104043=DIRECTION('',(-0.190809912898503,0.,0.981627005099017));
#104044=DIRECTION('',(0.981627005099017,0.,0.190809912898503));
#104045=DIRECTION('center_axis',(0.981627005099017,0.,0.190809912898503));
#104046=DIRECTION('ref_axis',(0.,-1.,0.));
#104047=DIRECTION('',(-0.190809912898503,0.,0.981627005099017));
#104048=DIRECTION('',(0.,-1.,0.));
#104049=DIRECTION('',(0.,-1.,0.));
#104050=DIRECTION('center_axis',(0.,-1.,0.));
#104051=DIRECTION('ref_axis',(0.,0.,-1.));
#104052=DIRECTION('',(-0.190809912898503,0.,0.981627005099017));
#104053=DIRECTION('',(-0.981627005099017,0.,-0.190809912898503));
#104054=DIRECTION('',(-0.981627005099017,0.,-0.190809912898503));
#104055=DIRECTION('center_axis',(-0.981627005099017,0.,-0.190809912898503));
#104056=DIRECTION('ref_axis',(-0.190809912898503,0.,0.981627005099017));
#104057=DIRECTION('',(0.,1.,0.));
#104058=DIRECTION('',(0.,1.,0.));
#104059=DIRECTION('center_axis',(0.,1.,0.));
#104060=DIRECTION('ref_axis',(1.,0.,0.));
#104061=DIRECTION('',(-0.190809912898503,0.,0.981627005099017));
#104062=DIRECTION('',(0.981627005099017,0.,0.190809912898503));
#104063=DIRECTION('',(-0.190809912898503,0.,0.981627005099017));
#104064=DIRECTION('',(0.981627005099017,0.,0.190809912898503));
#104065=DIRECTION('center_axis',(0.981627005099017,0.,0.190809912898503));
#104066=DIRECTION('ref_axis',(0.,-1.,0.));
#104067=DIRECTION('',(-0.190809912898503,0.,0.981627005099017));
#104068=DIRECTION('',(0.,-1.,0.));
#104069=DIRECTION('',(0.,-1.,0.));
#104070=DIRECTION('center_axis',(0.,-1.,0.));
#104071=DIRECTION('ref_axis',(0.,0.,-1.));
#104072=DIRECTION('',(-0.190809912898503,0.,0.981627005099017));
#104073=DIRECTION('',(-0.981627005099017,0.,-0.190809912898503));
#104074=DIRECTION('',(-0.981627005099017,0.,-0.190809912898503));
#104075=DIRECTION('center_axis',(-0.981627005099017,0.,-0.190809912898503));
#104076=DIRECTION('ref_axis',(-0.190809912898503,0.,0.981627005099017));
#104077=DIRECTION('',(0.,1.,0.));
#104078=DIRECTION('',(0.,1.,0.));
#104079=DIRECTION('center_axis',(0.,1.,0.));
#104080=DIRECTION('ref_axis',(1.,0.,0.));
#104081=DIRECTION('',(-0.190809912898503,0.,0.981627005099017));
#104082=DIRECTION('',(0.981627005099017,0.,0.190809912898503));
#104083=DIRECTION('',(-0.190809912898503,0.,0.981627005099017));
#104084=DIRECTION('',(0.981627005099017,0.,0.190809912898503));
#104085=DIRECTION('center_axis',(0.981627005099017,0.,0.190809912898503));
#104086=DIRECTION('ref_axis',(0.,-1.,0.));
#104087=DIRECTION('',(-0.190809912898503,0.,0.981627005099017));
#104088=DIRECTION('',(0.,-1.,0.));
#104089=DIRECTION('',(0.,-1.,0.));
#104090=DIRECTION('center_axis',(0.,-1.,0.));
#104091=DIRECTION('ref_axis',(0.,0.,-1.));
#104092=DIRECTION('',(-0.190809912898503,0.,0.981627005099017));
#104093=DIRECTION('',(-0.981627005099017,0.,-0.190809912898503));
#104094=DIRECTION('',(-0.981627005099017,0.,-0.190809912898503));
#104095=DIRECTION('center_axis',(-0.981627005099017,0.,-0.190809912898503));
#104096=DIRECTION('ref_axis',(-0.190809912898503,0.,0.981627005099017));
#104097=DIRECTION('',(0.,1.,0.));
#104098=DIRECTION('',(0.,1.,0.));
#104099=DIRECTION('center_axis',(0.,1.,0.));
#104100=DIRECTION('ref_axis',(1.,0.,0.));
#104101=DIRECTION('',(-0.190809912898503,0.,0.981627005099017));
#104102=DIRECTION('',(0.981627005099017,0.,0.190809912898503));
#104103=DIRECTION('',(-0.190809912898503,0.,0.981627005099017));
#104104=DIRECTION('',(0.981627005099017,0.,0.190809912898503));
#104105=DIRECTION('center_axis',(0.981627005099017,0.,0.190809912898503));
#104106=DIRECTION('ref_axis',(0.,-1.,0.));
#104107=DIRECTION('',(-0.190809912898503,0.,0.981627005099017));
#104108=DIRECTION('',(0.,-1.,0.));
#104109=DIRECTION('',(0.,-1.,0.));
#104110=DIRECTION('center_axis',(0.,-1.,0.));
#104111=DIRECTION('ref_axis',(0.,0.,-1.));
#104112=DIRECTION('',(-0.190809912898503,0.,0.981627005099017));
#104113=DIRECTION('',(-0.981627005099017,0.,-0.190809912898503));
#104114=DIRECTION('',(-0.981627005099017,0.,-0.190809912898503));
#104115=DIRECTION('center_axis',(-0.981627005099017,0.,-0.190809912898503));
#104116=DIRECTION('ref_axis',(-0.190809912898503,0.,0.981627005099017));
#104117=DIRECTION('',(0.,1.,0.));
#104118=DIRECTION('',(0.,1.,0.));
#104119=DIRECTION('center_axis',(0.,1.,0.));
#104120=DIRECTION('ref_axis',(1.,0.,0.));
#104121=DIRECTION('',(-0.190809912898503,0.,0.981627005099017));
#104122=DIRECTION('',(0.981627005099017,0.,0.190809912898503));
#104123=DIRECTION('',(-0.190809912898503,0.,0.981627005099017));
#104124=DIRECTION('',(0.981627005099017,0.,0.190809912898503));
#104125=DIRECTION('center_axis',(0.981627005099017,0.,0.190809912898503));
#104126=DIRECTION('ref_axis',(0.,-1.,0.));
#104127=DIRECTION('',(-0.190809912898503,0.,0.981627005099017));
#104128=DIRECTION('',(0.,-1.,0.));
#104129=DIRECTION('',(0.,-1.,0.));
#104130=DIRECTION('center_axis',(0.,-1.,0.));
#104131=DIRECTION('ref_axis',(0.,0.,-1.));
#104132=DIRECTION('',(-0.190809912898503,0.,0.981627005099017));
#104133=DIRECTION('',(-0.981627005099017,0.,-0.190809912898503));
#104134=DIRECTION('',(-0.981627005099017,0.,-0.190809912898503));
#104135=DIRECTION('center_axis',(-0.981627005099017,0.,-0.190809912898503));
#104136=DIRECTION('ref_axis',(-0.190809912898503,0.,0.981627005099017));
#104137=DIRECTION('',(0.,1.,0.));
#104138=DIRECTION('',(0.,1.,0.));
#104139=DIRECTION('center_axis',(0.,1.,0.));
#104140=DIRECTION('ref_axis',(1.,0.,0.));
#104141=DIRECTION('',(-0.190809912898503,0.,0.981627005099017));
#104142=DIRECTION('',(0.981627005099017,0.,0.190809912898503));
#104143=DIRECTION('',(-0.190809912898503,0.,0.981627005099017));
#104144=DIRECTION('',(0.981627005099017,0.,0.190809912898503));
#104145=DIRECTION('center_axis',(0.981627005099017,0.,0.190809912898503));
#104146=DIRECTION('ref_axis',(0.,-1.,0.));
#104147=DIRECTION('',(-0.190809912898503,0.,0.981627005099017));
#104148=DIRECTION('',(0.,-1.,0.));
#104149=DIRECTION('',(0.,-1.,0.));
#104150=DIRECTION('center_axis',(0.,-1.,0.));
#104151=DIRECTION('ref_axis',(0.,0.,-1.));
#104152=DIRECTION('',(-0.190809912898503,0.,0.981627005099017));
#104153=DIRECTION('',(-0.981627005099017,0.,-0.190809912898503));
#104154=DIRECTION('',(-0.981627005099017,0.,-0.190809912898503));
#104155=DIRECTION('center_axis',(-0.981627005099017,0.,-0.190809912898503));
#104156=DIRECTION('ref_axis',(-0.190809912898503,0.,0.981627005099017));
#104157=DIRECTION('',(0.,1.,0.));
#104158=DIRECTION('',(0.,1.,0.));
#104159=DIRECTION('center_axis',(0.,1.,0.));
#104160=DIRECTION('ref_axis',(1.,0.,0.));
#104161=DIRECTION('',(-0.190809912898503,0.,0.981627005099017));
#104162=DIRECTION('',(0.981627005099017,0.,0.190809912898503));
#104163=DIRECTION('',(-0.190809912898503,0.,0.981627005099017));
#104164=DIRECTION('',(0.981627005099017,0.,0.190809912898503));
#104165=DIRECTION('center_axis',(0.981627005099017,0.,0.190809912898503));
#104166=DIRECTION('ref_axis',(0.,-1.,0.));
#104167=DIRECTION('',(-0.190809912898503,0.,0.981627005099017));
#104168=DIRECTION('',(0.,-1.,0.));
#104169=DIRECTION('',(0.,-1.,0.));
#104170=DIRECTION('center_axis',(0.,-1.,0.));
#104171=DIRECTION('ref_axis',(0.,0.,-1.));
#104172=DIRECTION('',(-0.190809912898503,0.,0.981627005099017));
#104173=DIRECTION('',(-0.981627005099017,0.,-0.190809912898503));
#104174=DIRECTION('',(-0.981627005099017,0.,-0.190809912898503));
#104175=DIRECTION('center_axis',(-0.981627005099017,0.,-0.190809912898503));
#104176=DIRECTION('ref_axis',(-0.190809912898503,0.,0.981627005099017));
#104177=DIRECTION('',(0.,1.,0.));
#104178=DIRECTION('',(0.,1.,0.));
#104179=DIRECTION('center_axis',(0.,1.,0.));
#104180=DIRECTION('ref_axis',(1.,0.,0.));
#104181=DIRECTION('',(-0.190809912898503,0.,0.981627005099017));
#104182=DIRECTION('',(0.981627005099017,0.,0.190809912898503));
#104183=DIRECTION('',(-0.190809912898503,0.,0.981627005099017));
#104184=DIRECTION('',(0.981627005099017,0.,0.190809912898503));
#104185=DIRECTION('center_axis',(0.981627005099017,0.,0.190809912898503));
#104186=DIRECTION('ref_axis',(0.,-1.,0.));
#104187=DIRECTION('',(-0.190809912898503,0.,0.981627005099017));
#104188=DIRECTION('',(0.,-1.,0.));
#104189=DIRECTION('',(0.,-1.,0.));
#104190=DIRECTION('center_axis',(0.,-1.,0.));
#104191=DIRECTION('ref_axis',(0.,0.,-1.));
#104192=DIRECTION('',(-0.190809912898503,0.,0.981627005099017));
#104193=DIRECTION('',(-0.981627005099017,0.,-0.190809912898503));
#104194=DIRECTION('',(-0.981627005099017,0.,-0.190809912898503));
#104195=DIRECTION('center_axis',(-0.981627005099017,0.,-0.190809912898503));
#104196=DIRECTION('ref_axis',(-0.190809912898503,0.,0.981627005099017));
#104197=DIRECTION('',(0.,1.,0.));
#104198=DIRECTION('',(0.,1.,0.));
#104199=DIRECTION('center_axis',(0.,1.,0.));
#104200=DIRECTION('ref_axis',(1.,0.,0.));
#104201=DIRECTION('',(-0.190809912898503,0.,0.981627005099017));
#104202=DIRECTION('',(0.981627005099017,0.,0.190809912898503));
#104203=DIRECTION('',(-0.190809912898503,0.,0.981627005099017));
#104204=DIRECTION('',(0.981627005099017,0.,0.190809912898503));
#104205=DIRECTION('center_axis',(0.981627005099017,0.,0.190809912898503));
#104206=DIRECTION('ref_axis',(0.,-1.,0.));
#104207=DIRECTION('',(-0.190809912898503,0.,0.981627005099017));
#104208=DIRECTION('',(0.,-1.,0.));
#104209=DIRECTION('',(0.,-1.,0.));
#104210=DIRECTION('center_axis',(0.,-1.,0.));
#104211=DIRECTION('ref_axis',(0.,0.,-1.));
#104212=DIRECTION('',(-0.190809912898503,0.,0.981627005099017));
#104213=DIRECTION('',(-0.981627005099017,0.,-0.190809912898503));
#104214=DIRECTION('',(-0.981627005099017,0.,-0.190809912898503));
#104215=DIRECTION('center_axis',(-0.981627005099017,0.,-0.190809912898503));
#104216=DIRECTION('ref_axis',(-0.190809912898503,0.,0.981627005099017));
#104217=DIRECTION('',(0.,1.,0.));
#104218=DIRECTION('',(0.,1.,0.));
#104219=DIRECTION('center_axis',(0.,1.,0.));
#104220=DIRECTION('ref_axis',(1.,0.,0.));
#104221=DIRECTION('',(-0.190809912898503,0.,0.981627005099017));
#104222=DIRECTION('',(0.981627005099017,0.,0.190809912898503));
#104223=DIRECTION('',(-0.190809912898503,0.,0.981627005099017));
#104224=DIRECTION('',(0.981627005099017,0.,0.190809912898503));
#104225=DIRECTION('center_axis',(0.981627005099017,0.,0.190809912898503));
#104226=DIRECTION('ref_axis',(0.,-1.,0.));
#104227=DIRECTION('',(-0.190809912898503,0.,0.981627005099017));
#104228=DIRECTION('',(0.,-1.,0.));
#104229=DIRECTION('',(0.,-1.,0.));
#104230=DIRECTION('center_axis',(0.,-1.,0.));
#104231=DIRECTION('ref_axis',(0.,0.,-1.));
#104232=DIRECTION('',(-0.190809912898503,0.,0.981627005099017));
#104233=DIRECTION('',(-0.981627005099017,0.,-0.190809912898503));
#104234=DIRECTION('',(-0.981627005099017,0.,-0.190809912898503));
#104235=DIRECTION('center_axis',(-0.981627005099017,0.,-0.190809912898503));
#104236=DIRECTION('ref_axis',(-0.190809912898503,0.,0.981627005099017));
#104237=DIRECTION('',(0.,1.,0.));
#104238=DIRECTION('',(0.,1.,0.));
#104239=DIRECTION('center_axis',(0.,1.,0.));
#104240=DIRECTION('ref_axis',(1.,0.,0.));
#104241=DIRECTION('',(-0.190809912898503,0.,0.981627005099017));
#104242=DIRECTION('',(0.981627005099017,0.,0.190809912898503));
#104243=DIRECTION('',(-0.190809912898503,0.,0.981627005099017));
#104244=DIRECTION('',(0.981627005099017,0.,0.190809912898503));
#104245=DIRECTION('center_axis',(0.981627005099017,0.,0.190809912898503));
#104246=DIRECTION('ref_axis',(0.,-1.,0.));
#104247=DIRECTION('',(-0.190809912898503,0.,0.981627005099017));
#104248=DIRECTION('',(0.,-1.,0.));
#104249=DIRECTION('',(0.,-1.,0.));
#104250=DIRECTION('center_axis',(0.,-1.,0.));
#104251=DIRECTION('ref_axis',(0.,0.,-1.));
#104252=DIRECTION('',(-0.190809912898503,0.,0.981627005099017));
#104253=DIRECTION('',(-0.981627005099017,0.,-0.190809912898503));
#104254=DIRECTION('',(-0.981627005099017,0.,-0.190809912898503));
#104255=DIRECTION('center_axis',(-0.981627005099017,0.,-0.190809912898503));
#104256=DIRECTION('ref_axis',(-0.190809912898503,0.,0.981627005099017));
#104257=DIRECTION('',(0.,1.,0.));
#104258=DIRECTION('',(0.,1.,0.));
#104259=DIRECTION('center_axis',(0.,1.,0.));
#104260=DIRECTION('ref_axis',(1.,0.,0.));
#104261=DIRECTION('',(-0.190809912898503,0.,0.981627005099017));
#104262=DIRECTION('',(0.981627005099017,0.,0.190809912898503));
#104263=DIRECTION('',(-0.190809912898503,0.,0.981627005099017));
#104264=DIRECTION('',(0.981627005099017,0.,0.190809912898503));
#104265=DIRECTION('center_axis',(0.981627005099017,0.,0.190809912898503));
#104266=DIRECTION('ref_axis',(0.,-1.,0.));
#104267=DIRECTION('',(-0.190809912898503,0.,0.981627005099017));
#104268=DIRECTION('',(0.,-1.,0.));
#104269=DIRECTION('',(0.,-1.,0.));
#104270=DIRECTION('center_axis',(0.,-1.,0.));
#104271=DIRECTION('ref_axis',(0.,0.,-1.));
#104272=DIRECTION('',(-0.190809912898503,0.,0.981627005099017));
#104273=DIRECTION('',(-0.981627005099017,0.,-0.190809912898503));
#104274=DIRECTION('',(-0.981627005099017,0.,-0.190809912898503));
#104275=DIRECTION('center_axis',(-0.981627005099017,0.,-0.190809912898503));
#104276=DIRECTION('ref_axis',(-0.190809912898503,0.,0.981627005099017));
#104277=DIRECTION('',(0.,1.,0.));
#104278=DIRECTION('',(0.,1.,0.));
#104279=DIRECTION('center_axis',(0.,1.,0.));
#104280=DIRECTION('ref_axis',(1.,0.,0.));
#104281=DIRECTION('',(-0.190809912898503,0.,0.981627005099017));
#104282=DIRECTION('',(0.981627005099017,0.,0.190809912898503));
#104283=DIRECTION('',(-0.190809912898503,0.,0.981627005099017));
#104284=DIRECTION('',(0.981627005099017,0.,0.190809912898503));
#104285=DIRECTION('center_axis',(0.981627005099017,0.,0.190809912898503));
#104286=DIRECTION('ref_axis',(0.,-1.,0.));
#104287=DIRECTION('',(-0.190809912898503,0.,0.981627005099017));
#104288=DIRECTION('',(0.,-1.,0.));
#104289=DIRECTION('',(0.,-1.,0.));
#104290=DIRECTION('center_axis',(0.,-1.,0.));
#104291=DIRECTION('ref_axis',(0.,0.,-1.));
#104292=DIRECTION('',(-0.190809912898503,0.,0.981627005099017));
#104293=DIRECTION('',(-0.981627005099017,0.,-0.190809912898503));
#104294=DIRECTION('',(-0.981627005099017,0.,-0.190809912898503));
#104295=DIRECTION('center_axis',(-0.981627005099017,0.,-0.190809912898503));
#104296=DIRECTION('ref_axis',(-0.190809912898503,0.,0.981627005099017));
#104297=DIRECTION('',(0.,1.,0.));
#104298=DIRECTION('',(0.,1.,0.));
#104299=DIRECTION('center_axis',(0.,1.,0.));
#104300=DIRECTION('ref_axis',(1.,0.,0.));
#104301=DIRECTION('',(-0.190809912898503,0.,0.981627005099017));
#104302=DIRECTION('',(0.981627005099017,0.,0.190809912898503));
#104303=DIRECTION('',(-0.190809912898503,0.,0.981627005099017));
#104304=DIRECTION('',(0.981627005099017,0.,0.190809912898503));
#104305=DIRECTION('center_axis',(0.981627005099017,0.,0.190809912898503));
#104306=DIRECTION('ref_axis',(0.,-1.,0.));
#104307=DIRECTION('',(-0.190809912898503,0.,0.981627005099017));
#104308=DIRECTION('',(0.,-1.,0.));
#104309=DIRECTION('',(0.,-1.,0.));
#104310=DIRECTION('center_axis',(0.,-1.,0.));
#104311=DIRECTION('ref_axis',(0.,0.,-1.));
#104312=DIRECTION('',(-0.190809912898503,0.,0.981627005099017));
#104313=DIRECTION('',(-0.981627005099017,0.,-0.190809912898503));
#104314=DIRECTION('',(-0.981627005099017,0.,-0.190809912898503));
#104315=DIRECTION('center_axis',(-0.981627005099017,0.,-0.190809912898503));
#104316=DIRECTION('ref_axis',(-0.190809912898503,0.,0.981627005099017));
#104317=DIRECTION('',(0.,1.,0.));
#104318=DIRECTION('',(0.,1.,0.));
#104319=DIRECTION('center_axis',(0.,1.,0.));
#104320=DIRECTION('ref_axis',(1.,0.,0.));
#104321=DIRECTION('',(-0.190809912898503,0.,0.981627005099017));
#104322=DIRECTION('',(0.981627005099017,0.,0.190809912898503));
#104323=DIRECTION('',(-0.190809912898503,0.,0.981627005099017));
#104324=DIRECTION('',(0.981627005099017,0.,0.190809912898503));
#104325=DIRECTION('center_axis',(0.981627005099017,0.,0.190809912898503));
#104326=DIRECTION('ref_axis',(0.,-1.,0.));
#104327=DIRECTION('',(-0.190809912898503,0.,0.981627005099017));
#104328=DIRECTION('',(0.,-1.,0.));
#104329=DIRECTION('',(0.,-1.,0.));
#104330=DIRECTION('center_axis',(0.,-1.,0.));
#104331=DIRECTION('ref_axis',(0.,0.,-1.));
#104332=DIRECTION('',(-0.190809912898503,0.,0.981627005099017));
#104333=DIRECTION('',(-0.981627005099017,0.,-0.190809912898503));
#104334=DIRECTION('',(-0.981627005099017,0.,-0.190809912898503));
#104335=DIRECTION('center_axis',(-0.981627005099017,0.,-0.190809912898503));
#104336=DIRECTION('ref_axis',(-0.190809912898503,0.,0.981627005099017));
#104337=DIRECTION('',(0.,1.,0.));
#104338=DIRECTION('',(0.,1.,0.));
#104339=DIRECTION('center_axis',(0.,1.,0.));
#104340=DIRECTION('ref_axis',(1.,0.,0.));
#104341=DIRECTION('',(-0.190809912898503,0.,0.981627005099017));
#104342=DIRECTION('',(0.981627005099017,0.,0.190809912898503));
#104343=DIRECTION('',(-0.190809912898503,0.,0.981627005099017));
#104344=DIRECTION('',(0.981627005099017,0.,0.190809912898503));
#104345=DIRECTION('center_axis',(0.981627005099017,0.,0.190809912898503));
#104346=DIRECTION('ref_axis',(0.,-1.,0.));
#104347=DIRECTION('',(-0.190809912898503,0.,0.981627005099017));
#104348=DIRECTION('',(0.,-1.,0.));
#104349=DIRECTION('',(0.,-1.,0.));
#104350=DIRECTION('center_axis',(0.,-1.,0.));
#104351=DIRECTION('ref_axis',(0.,0.,-1.));
#104352=DIRECTION('',(-0.190809912898503,0.,0.981627005099017));
#104353=DIRECTION('',(-0.981627005099017,0.,-0.190809912898503));
#104354=DIRECTION('',(-0.981627005099017,0.,-0.190809912898503));
#104355=DIRECTION('center_axis',(-0.981627005099017,0.,-0.190809912898503));
#104356=DIRECTION('ref_axis',(-0.190809912898503,0.,0.981627005099017));
#104357=DIRECTION('',(0.,1.,0.));
#104358=DIRECTION('',(0.,1.,0.));
#104359=DIRECTION('center_axis',(0.,1.,0.));
#104360=DIRECTION('ref_axis',(1.,0.,0.));
#104361=DIRECTION('',(-0.190809912898503,0.,0.981627005099017));
#104362=DIRECTION('',(0.981627005099017,0.,0.190809912898503));
#104363=DIRECTION('',(-0.190809912898503,0.,0.981627005099017));
#104364=DIRECTION('',(0.981627005099017,0.,0.190809912898503));
#104365=DIRECTION('center_axis',(0.981627005099017,0.,0.190809912898503));
#104366=DIRECTION('ref_axis',(0.,-1.,0.));
#104367=DIRECTION('',(-0.190809912898503,0.,0.981627005099017));
#104368=DIRECTION('',(0.,-1.,0.));
#104369=DIRECTION('',(0.,-1.,0.));
#104370=DIRECTION('center_axis',(0.,-1.,0.));
#104371=DIRECTION('ref_axis',(0.,0.,-1.));
#104372=DIRECTION('',(-0.190809912898503,0.,0.981627005099017));
#104373=DIRECTION('',(-0.981627005099017,0.,-0.190809912898503));
#104374=DIRECTION('',(-0.981627005099017,0.,-0.190809912898503));
#104375=DIRECTION('center_axis',(-0.981627005099017,0.,-0.190809912898503));
#104376=DIRECTION('ref_axis',(-0.190809912898503,0.,0.981627005099017));
#104377=DIRECTION('',(0.,1.,0.));
#104378=DIRECTION('',(0.,1.,0.));
#104379=DIRECTION('center_axis',(0.,1.,0.));
#104380=DIRECTION('ref_axis',(1.,0.,0.));
#104381=DIRECTION('',(-0.190809912898503,0.,0.981627005099017));
#104382=DIRECTION('',(0.981627005099017,0.,0.190809912898503));
#104383=DIRECTION('',(-0.190809912898503,0.,0.981627005099017));
#104384=DIRECTION('',(0.981627005099017,0.,0.190809912898503));
#104385=DIRECTION('center_axis',(0.981627005099017,0.,0.190809912898503));
#104386=DIRECTION('ref_axis',(0.,-1.,0.));
#104387=DIRECTION('',(-0.190809912898503,0.,0.981627005099017));
#104388=DIRECTION('',(0.,-1.,0.));
#104389=DIRECTION('',(0.,-1.,0.));
#104390=DIRECTION('center_axis',(0.,-1.,0.));
#104391=DIRECTION('ref_axis',(0.,0.,-1.));
#104392=DIRECTION('',(-0.190809912898503,0.,0.981627005099017));
#104393=DIRECTION('',(-0.981627005099017,0.,-0.190809912898503));
#104394=DIRECTION('',(-0.981627005099017,0.,-0.190809912898503));
#104395=DIRECTION('center_axis',(-0.981627005099017,0.,-0.190809912898503));
#104396=DIRECTION('ref_axis',(-0.190809912898503,0.,0.981627005099017));
#104397=DIRECTION('',(0.,1.,0.));
#104398=DIRECTION('',(0.,1.,0.));
#104399=DIRECTION('center_axis',(0.,1.,0.));
#104400=DIRECTION('ref_axis',(1.,0.,0.));
#104401=DIRECTION('',(-0.190809912898503,0.,0.981627005099017));
#104402=DIRECTION('',(0.981627005099017,0.,0.190809912898503));
#104403=DIRECTION('',(-0.190809912898503,0.,0.981627005099017));
#104404=DIRECTION('',(0.981627005099017,0.,0.190809912898503));
#104405=DIRECTION('center_axis',(0.981627005099017,0.,0.190809912898503));
#104406=DIRECTION('ref_axis',(0.,-1.,0.));
#104407=DIRECTION('',(-0.190809912898503,0.,0.981627005099017));
#104408=DIRECTION('',(0.,-1.,0.));
#104409=DIRECTION('',(0.,-1.,0.));
#104410=DIRECTION('center_axis',(0.,-1.,0.));
#104411=DIRECTION('ref_axis',(0.,0.,-1.));
#104412=DIRECTION('',(-0.190809912898503,0.,0.981627005099017));
#104413=DIRECTION('',(-0.981627005099017,0.,-0.190809912898503));
#104414=DIRECTION('',(-0.981627005099017,0.,-0.190809912898503));
#104415=DIRECTION('center_axis',(-0.981627005099017,0.,-0.190809912898503));
#104416=DIRECTION('ref_axis',(-0.190809912898503,0.,0.981627005099017));
#104417=DIRECTION('',(0.,1.,0.));
#104418=DIRECTION('',(0.,1.,0.));
#104419=DIRECTION('center_axis',(0.,1.,0.));
#104420=DIRECTION('ref_axis',(1.,0.,0.));
#104421=DIRECTION('',(-0.190809912898503,0.,0.981627005099017));
#104422=DIRECTION('',(0.981627005099017,0.,0.190809912898503));
#104423=DIRECTION('',(-0.190809912898503,0.,0.981627005099017));
#104424=DIRECTION('',(0.981627005099017,0.,0.190809912898503));
#104425=DIRECTION('center_axis',(0.981627005099017,0.,0.190809912898503));
#104426=DIRECTION('ref_axis',(0.,-1.,0.));
#104427=DIRECTION('',(-0.190809912898503,0.,0.981627005099017));
#104428=DIRECTION('',(0.,-1.,0.));
#104429=DIRECTION('',(0.,-1.,0.));
#104430=DIRECTION('center_axis',(0.,-1.,0.));
#104431=DIRECTION('ref_axis',(0.,0.,-1.));
#104432=DIRECTION('',(-0.190809912898503,0.,0.981627005099017));
#104433=DIRECTION('',(-0.981627005099017,0.,-0.190809912898503));
#104434=DIRECTION('',(-0.981627005099017,0.,-0.190809912898503));
#104435=DIRECTION('center_axis',(-0.981627005099017,0.,-0.190809912898503));
#104436=DIRECTION('ref_axis',(-0.190809912898503,0.,0.981627005099017));
#104437=DIRECTION('',(0.,1.,0.));
#104438=DIRECTION('',(0.,1.,0.));
#104439=DIRECTION('center_axis',(0.,1.,0.));
#104440=DIRECTION('ref_axis',(1.,0.,0.));
#104441=DIRECTION('',(-0.190809912898503,0.,0.981627005099017));
#104442=DIRECTION('',(0.981627005099017,0.,0.190809912898503));
#104443=DIRECTION('',(-0.190809912898503,0.,0.981627005099017));
#104444=DIRECTION('',(0.981627005099017,0.,0.190809912898503));
#104445=DIRECTION('center_axis',(0.981627005099017,0.,0.190809912898503));
#104446=DIRECTION('ref_axis',(0.,-1.,0.));
#104447=DIRECTION('',(-0.190809912898503,0.,0.981627005099017));
#104448=DIRECTION('',(0.,-1.,0.));
#104449=DIRECTION('',(0.,-1.,0.));
#104450=DIRECTION('center_axis',(0.,-1.,0.));
#104451=DIRECTION('ref_axis',(0.,0.,-1.));
#104452=DIRECTION('',(-0.190809912898503,0.,0.981627005099017));
#104453=DIRECTION('',(-0.981627005099017,0.,-0.190809912898503));
#104454=DIRECTION('',(-0.981627005099017,0.,-0.190809912898503));
#104455=DIRECTION('center_axis',(-0.981627005099017,0.,-0.190809912898503));
#104456=DIRECTION('ref_axis',(-0.190809912898503,0.,0.981627005099017));
#104457=DIRECTION('',(0.,1.,0.));
#104458=DIRECTION('',(0.,1.,0.));
#104459=DIRECTION('center_axis',(0.,1.,0.));
#104460=DIRECTION('ref_axis',(1.,0.,0.));
#104461=DIRECTION('',(-0.190809912898503,0.,0.981627005099017));
#104462=DIRECTION('',(0.981627005099017,0.,0.190809912898503));
#104463=DIRECTION('',(-0.190809912898503,0.,0.981627005099017));
#104464=DIRECTION('',(0.981627005099017,0.,0.190809912898503));
#104465=DIRECTION('center_axis',(0.981627005099017,0.,0.190809912898503));
#104466=DIRECTION('ref_axis',(0.,-1.,0.));
#104467=DIRECTION('',(-0.190809912898503,0.,0.981627005099017));
#104468=DIRECTION('',(0.,-1.,0.));
#104469=DIRECTION('',(0.,-1.,0.));
#104470=DIRECTION('center_axis',(0.,-1.,0.));
#104471=DIRECTION('ref_axis',(0.,0.,-1.));
#104472=DIRECTION('',(-0.190809912898503,0.,0.981627005099017));
#104473=DIRECTION('',(-0.981627005099017,0.,-0.190809912898503));
#104474=DIRECTION('',(-0.981627005099017,0.,-0.190809912898503));
#104475=DIRECTION('center_axis',(-0.981627005099017,0.,-0.190809912898503));
#104476=DIRECTION('ref_axis',(-0.190809912898503,0.,0.981627005099017));
#104477=DIRECTION('',(0.,1.,0.));
#104478=DIRECTION('',(0.,1.,0.));
#104479=DIRECTION('center_axis',(0.,1.,0.));
#104480=DIRECTION('ref_axis',(1.,0.,0.));
#104481=DIRECTION('',(-0.190809912898503,0.,0.981627005099017));
#104482=DIRECTION('',(0.981627005099017,0.,0.190809912898503));
#104483=DIRECTION('',(-0.190809912898503,0.,0.981627005099017));
#104484=DIRECTION('',(0.981627005099017,0.,0.190809912898503));
#104485=DIRECTION('center_axis',(0.981627005099017,0.,0.190809912898503));
#104486=DIRECTION('ref_axis',(0.,-1.,0.));
#104487=DIRECTION('',(-0.190809912898503,0.,0.981627005099017));
#104488=DIRECTION('',(0.,-1.,0.));
#104489=DIRECTION('',(0.,-1.,0.));
#104490=DIRECTION('center_axis',(0.,-1.,0.));
#104491=DIRECTION('ref_axis',(0.,0.,-1.));
#104492=DIRECTION('',(-0.190809912898503,0.,0.981627005099017));
#104493=DIRECTION('',(-0.981627005099017,0.,-0.190809912898503));
#104494=DIRECTION('',(-0.981627005099017,0.,-0.190809912898503));
#104495=DIRECTION('center_axis',(-0.981627005099017,0.,-0.190809912898503));
#104496=DIRECTION('ref_axis',(-0.190809912898503,0.,0.981627005099017));
#104497=DIRECTION('',(0.,1.,0.));
#104498=DIRECTION('',(0.,1.,0.));
#104499=DIRECTION('center_axis',(0.,1.,0.));
#104500=DIRECTION('ref_axis',(1.,0.,0.));
#104501=DIRECTION('',(-0.190809912898503,0.,0.981627005099017));
#104502=DIRECTION('',(0.981627005099017,0.,0.190809912898503));
#104503=DIRECTION('',(-0.190809912898503,0.,0.981627005099017));
#104504=DIRECTION('',(0.981627005099017,0.,0.190809912898503));
#104505=DIRECTION('center_axis',(0.981627005099017,0.,0.190809912898503));
#104506=DIRECTION('ref_axis',(0.,-1.,0.));
#104507=DIRECTION('',(-0.190809912898503,0.,0.981627005099017));
#104508=DIRECTION('',(0.,-1.,0.));
#104509=DIRECTION('',(0.,-1.,0.));
#104510=DIRECTION('center_axis',(0.,-1.,0.));
#104511=DIRECTION('ref_axis',(0.,0.,-1.));
#104512=DIRECTION('',(-0.190809912898503,0.,0.981627005099017));
#104513=DIRECTION('',(-0.981627005099017,0.,-0.190809912898503));
#104514=DIRECTION('',(-0.981627005099017,0.,-0.190809912898503));
#104515=DIRECTION('center_axis',(-0.981627005099017,0.,-0.190809912898503));
#104516=DIRECTION('ref_axis',(-0.190809912898503,0.,0.981627005099017));
#104517=DIRECTION('',(0.,1.,0.));
#104518=DIRECTION('',(0.,1.,0.));
#104519=DIRECTION('center_axis',(0.,1.,0.));
#104520=DIRECTION('ref_axis',(1.,0.,0.));
#104521=DIRECTION('',(-0.190809912898503,0.,0.981627005099017));
#104522=DIRECTION('',(0.981627005099017,0.,0.190809912898503));
#104523=DIRECTION('',(-0.190809912898503,0.,0.981627005099017));
#104524=DIRECTION('',(0.981627005099017,0.,0.190809912898503));
#104525=DIRECTION('center_axis',(0.981627005099017,0.,0.190809912898503));
#104526=DIRECTION('ref_axis',(0.,-1.,0.));
#104527=DIRECTION('',(-0.190809912898503,0.,0.981627005099017));
#104528=DIRECTION('',(0.,-1.,0.));
#104529=DIRECTION('',(0.,-1.,0.));
#104530=DIRECTION('center_axis',(0.,-1.,0.));
#104531=DIRECTION('ref_axis',(0.,0.,-1.));
#104532=DIRECTION('',(-0.190809912898503,0.,0.981627005099017));
#104533=DIRECTION('',(-0.981627005099017,0.,-0.190809912898503));
#104534=DIRECTION('',(-0.981627005099017,0.,-0.190809912898503));
#104535=DIRECTION('center_axis',(-0.981627005099017,0.,-0.190809912898503));
#104536=DIRECTION('ref_axis',(-0.190809912898503,0.,0.981627005099017));
#104537=DIRECTION('',(0.,1.,0.));
#104538=DIRECTION('',(0.,1.,0.));
#104539=DIRECTION('center_axis',(0.,1.,0.));
#104540=DIRECTION('ref_axis',(1.,0.,0.));
#104541=DIRECTION('',(-0.190809912898503,0.,0.981627005099017));
#104542=DIRECTION('',(0.981627005099017,0.,0.190809912898503));
#104543=DIRECTION('',(-0.190809912898503,0.,0.981627005099017));
#104544=DIRECTION('',(0.981627005099017,0.,0.190809912898503));
#104545=DIRECTION('center_axis',(0.981627005099017,0.,0.190809912898503));
#104546=DIRECTION('ref_axis',(0.,-1.,0.));
#104547=DIRECTION('',(-0.190809912898503,0.,0.981627005099017));
#104548=DIRECTION('',(0.,-1.,0.));
#104549=DIRECTION('',(0.,-1.,0.));
#104550=DIRECTION('center_axis',(0.,-1.,0.));
#104551=DIRECTION('ref_axis',(0.,0.,-1.));
#104552=DIRECTION('',(-0.190809912898503,0.,0.981627005099017));
#104553=DIRECTION('',(-0.981627005099017,0.,-0.190809912898503));
#104554=DIRECTION('',(-0.981627005099017,0.,-0.190809912898503));
#104555=DIRECTION('center_axis',(-0.981627005099017,0.,-0.190809912898503));
#104556=DIRECTION('ref_axis',(-0.190809912898503,0.,0.981627005099017));
#104557=DIRECTION('',(0.,1.,0.));
#104558=DIRECTION('',(0.,1.,0.));
#104559=DIRECTION('center_axis',(0.,1.,0.));
#104560=DIRECTION('ref_axis',(1.,0.,0.));
#104561=DIRECTION('',(-0.190809912898503,0.,0.981627005099017));
#104562=DIRECTION('',(0.981627005099017,0.,0.190809912898503));
#104563=DIRECTION('',(-0.190809912898503,0.,0.981627005099017));
#104564=DIRECTION('',(0.981627005099017,0.,0.190809912898503));
#104565=DIRECTION('center_axis',(0.981627005099017,0.,0.190809912898503));
#104566=DIRECTION('ref_axis',(0.,-1.,0.));
#104567=DIRECTION('',(-0.190809912898503,0.,0.981627005099017));
#104568=DIRECTION('',(0.,-1.,0.));
#104569=DIRECTION('',(0.,-1.,0.));
#104570=DIRECTION('center_axis',(0.,-1.,0.));
#104571=DIRECTION('ref_axis',(0.,0.,-1.));
#104572=DIRECTION('',(-0.190809912898503,0.,0.981627005099017));
#104573=DIRECTION('',(-0.981627005099017,0.,-0.190809912898503));
#104574=DIRECTION('',(-0.981627005099017,0.,-0.190809912898503));
#104575=DIRECTION('center_axis',(-0.981627005099017,0.,-0.190809912898503));
#104576=DIRECTION('ref_axis',(-0.190809912898503,0.,0.981627005099017));
#104577=DIRECTION('',(0.,1.,0.));
#104578=DIRECTION('',(0.,1.,0.));
#104579=DIRECTION('center_axis',(0.,1.,0.));
#104580=DIRECTION('ref_axis',(1.,0.,0.));
#104581=DIRECTION('',(-0.190809912898503,0.,0.981627005099017));
#104582=DIRECTION('',(0.981627005099017,0.,0.190809912898503));
#104583=DIRECTION('',(-0.190809912898503,0.,0.981627005099017));
#104584=DIRECTION('',(0.981627005099017,0.,0.190809912898503));
#104585=DIRECTION('center_axis',(0.981627005099017,0.,0.190809912898503));
#104586=DIRECTION('ref_axis',(0.,-1.,0.));
#104587=DIRECTION('',(-0.190809912898503,0.,0.981627005099017));
#104588=DIRECTION('',(0.,-1.,0.));
#104589=DIRECTION('',(0.,-1.,0.));
#104590=DIRECTION('center_axis',(0.,-1.,0.));
#104591=DIRECTION('ref_axis',(0.,0.,-1.));
#104592=DIRECTION('',(-0.190809912898503,0.,0.981627005099017));
#104593=DIRECTION('',(-0.981627005099017,0.,-0.190809912898503));
#104594=DIRECTION('',(-0.981627005099017,0.,-0.190809912898503));
#104595=DIRECTION('center_axis',(-0.981627005099017,0.,-0.190809912898503));
#104596=DIRECTION('ref_axis',(-0.190809912898503,0.,0.981627005099017));
#104597=DIRECTION('',(0.,1.,0.));
#104598=DIRECTION('',(0.,1.,0.));
#104599=DIRECTION('center_axis',(0.,1.,0.));
#104600=DIRECTION('ref_axis',(1.,0.,0.));
#104601=DIRECTION('',(-0.190809912898503,0.,0.981627005099017));
#104602=DIRECTION('',(0.981627005099017,0.,0.190809912898503));
#104603=DIRECTION('',(-0.190809912898503,0.,0.981627005099017));
#104604=DIRECTION('',(0.981627005099017,0.,0.190809912898503));
#104605=DIRECTION('center_axis',(0.981627005099017,0.,0.190809912898503));
#104606=DIRECTION('ref_axis',(0.,-1.,0.));
#104607=DIRECTION('',(-0.190809912898503,0.,0.981627005099017));
#104608=DIRECTION('',(0.,-1.,0.));
#104609=DIRECTION('',(0.,-1.,0.));
#104610=DIRECTION('center_axis',(0.,-1.,0.));
#104611=DIRECTION('ref_axis',(0.,0.,-1.));
#104612=DIRECTION('',(-0.190809912898503,0.,0.981627005099017));
#104613=DIRECTION('',(-0.981627005099017,0.,-0.190809912898503));
#104614=DIRECTION('',(-0.981627005099017,0.,-0.190809912898503));
#104615=DIRECTION('center_axis',(-0.981627005099017,0.,-0.190809912898503));
#104616=DIRECTION('ref_axis',(-0.190809912898503,0.,0.981627005099017));
#104617=DIRECTION('',(0.,1.,0.));
#104618=DIRECTION('',(0.,1.,0.));
#104619=DIRECTION('center_axis',(0.,1.,0.));
#104620=DIRECTION('ref_axis',(1.,0.,0.));
#104621=DIRECTION('',(-0.190809912898503,0.,0.981627005099017));
#104622=DIRECTION('',(0.981627005099017,0.,0.190809912898503));
#104623=DIRECTION('',(-0.190809912898503,0.,0.981627005099017));
#104624=DIRECTION('',(0.981627005099017,0.,0.190809912898503));
#104625=DIRECTION('center_axis',(0.981627005099017,0.,0.190809912898503));
#104626=DIRECTION('ref_axis',(0.,-1.,0.));
#104627=DIRECTION('',(-0.190809912898503,0.,0.981627005099017));
#104628=DIRECTION('',(0.,-1.,0.));
#104629=DIRECTION('',(0.,-1.,0.));
#104630=DIRECTION('center_axis',(0.,-1.,0.));
#104631=DIRECTION('ref_axis',(0.,0.,-1.));
#104632=DIRECTION('',(-0.190809912898503,0.,0.981627005099017));
#104633=DIRECTION('',(-0.981627005099017,0.,-0.190809912898503));
#104634=DIRECTION('',(-0.981627005099017,0.,-0.190809912898503));
#104635=DIRECTION('center_axis',(-0.981627005099017,0.,-0.190809912898503));
#104636=DIRECTION('ref_axis',(-0.190809912898503,0.,0.981627005099017));
#104637=DIRECTION('',(0.,1.,0.));
#104638=DIRECTION('',(0.,1.,0.));
#104639=DIRECTION('center_axis',(0.,1.,0.));
#104640=DIRECTION('ref_axis',(1.,0.,0.));
#104641=DIRECTION('',(-0.190809912898503,0.,0.981627005099017));
#104642=DIRECTION('',(0.981627005099017,0.,0.190809912898503));
#104643=DIRECTION('',(-0.190809912898503,0.,0.981627005099017));
#104644=DIRECTION('',(0.981627005099017,0.,0.190809912898503));
#104645=DIRECTION('center_axis',(0.981627005099017,0.,0.190809912898503));
#104646=DIRECTION('ref_axis',(0.,-1.,0.));
#104647=DIRECTION('',(-0.190809912898503,0.,0.981627005099017));
#104648=DIRECTION('',(0.,-1.,0.));
#104649=DIRECTION('',(0.,-1.,0.));
#104650=DIRECTION('center_axis',(0.,-1.,0.));
#104651=DIRECTION('ref_axis',(0.,0.,-1.));
#104652=DIRECTION('',(-0.190809912898503,0.,0.981627005099017));
#104653=DIRECTION('',(-0.981627005099017,0.,-0.190809912898503));
#104654=DIRECTION('',(-0.981627005099017,0.,-0.190809912898503));
#104655=DIRECTION('center_axis',(-0.981627005099017,0.,-0.190809912898503));
#104656=DIRECTION('ref_axis',(-0.190809912898503,0.,0.981627005099017));
#104657=DIRECTION('',(0.,1.,0.));
#104658=DIRECTION('',(0.,1.,0.));
#104659=DIRECTION('center_axis',(0.,1.,0.));
#104660=DIRECTION('ref_axis',(1.,0.,0.));
#104661=DIRECTION('',(-0.190809912898503,0.,0.981627005099017));
#104662=DIRECTION('',(0.981627005099017,0.,0.190809912898503));
#104663=DIRECTION('',(-0.190809912898503,0.,0.981627005099017));
#104664=DIRECTION('',(0.981627005099017,0.,0.190809912898503));
#104665=DIRECTION('center_axis',(0.981627005099017,0.,0.190809912898503));
#104666=DIRECTION('ref_axis',(0.,-1.,0.));
#104667=DIRECTION('',(-0.190809912898503,0.,0.981627005099017));
#104668=DIRECTION('',(0.,-1.,0.));
#104669=DIRECTION('',(0.,-1.,0.));
#104670=DIRECTION('center_axis',(0.,-1.,0.));
#104671=DIRECTION('ref_axis',(0.,0.,-1.));
#104672=DIRECTION('',(-0.190809912898503,0.,0.981627005099017));
#104673=DIRECTION('',(-0.981627005099017,0.,-0.190809912898503));
#104674=DIRECTION('',(-0.981627005099017,0.,-0.190809912898503));
#104675=DIRECTION('center_axis',(-0.981627005099017,0.,-0.190809912898503));
#104676=DIRECTION('ref_axis',(-0.190809912898503,0.,0.981627005099017));
#104677=DIRECTION('',(0.,1.,0.));
#104678=DIRECTION('',(0.,1.,0.));
#104679=DIRECTION('center_axis',(0.,1.,0.));
#104680=DIRECTION('ref_axis',(1.,0.,0.));
#104681=DIRECTION('',(-0.190809912898503,0.,0.981627005099017));
#104682=DIRECTION('',(0.981627005099017,0.,0.190809912898503));
#104683=DIRECTION('',(-0.190809912898503,0.,0.981627005099017));
#104684=DIRECTION('',(0.981627005099017,0.,0.190809912898503));
#104685=DIRECTION('center_axis',(0.981627005099017,0.,0.190809912898503));
#104686=DIRECTION('ref_axis',(0.,-1.,0.));
#104687=DIRECTION('',(-0.190809912898503,0.,0.981627005099017));
#104688=DIRECTION('',(0.,-1.,0.));
#104689=DIRECTION('',(0.,-1.,0.));
#104690=DIRECTION('center_axis',(0.,-1.,0.));
#104691=DIRECTION('ref_axis',(0.,0.,-1.));
#104692=DIRECTION('',(-0.190809912898503,0.,0.981627005099017));
#104693=DIRECTION('',(-0.981627005099017,0.,-0.190809912898503));
#104694=DIRECTION('',(-0.981627005099017,0.,-0.190809912898503));
#104695=DIRECTION('center_axis',(-0.981627005099017,0.,-0.190809912898503));
#104696=DIRECTION('ref_axis',(-0.190809912898503,0.,0.981627005099017));
#104697=DIRECTION('',(0.,1.,0.));
#104698=DIRECTION('',(0.,1.,0.));
#104699=DIRECTION('center_axis',(0.,1.,0.));
#104700=DIRECTION('ref_axis',(1.,0.,0.));
#104701=DIRECTION('',(-0.190809912898503,0.,0.981627005099017));
#104702=DIRECTION('',(0.981627005099017,0.,0.190809912898503));
#104703=DIRECTION('',(-0.190809912898503,0.,0.981627005099017));
#104704=DIRECTION('',(0.981627005099017,0.,0.190809912898503));
#104705=DIRECTION('center_axis',(0.981627005099017,0.,0.190809912898503));
#104706=DIRECTION('ref_axis',(0.,-1.,0.));
#104707=DIRECTION('',(-0.190809912898503,0.,0.981627005099017));
#104708=DIRECTION('',(0.,-1.,0.));
#104709=DIRECTION('',(0.,-1.,0.));
#104710=DIRECTION('center_axis',(0.,-1.,0.));
#104711=DIRECTION('ref_axis',(0.,0.,-1.));
#104712=DIRECTION('',(-0.190809912898503,0.,0.981627005099017));
#104713=DIRECTION('',(-0.981627005099017,0.,-0.190809912898503));
#104714=DIRECTION('',(-0.981627005099017,0.,-0.190809912898503));
#104715=DIRECTION('center_axis',(-0.981627005099017,0.,-0.190809912898503));
#104716=DIRECTION('ref_axis',(-0.190809912898503,0.,0.981627005099017));
#104717=DIRECTION('',(0.,1.,0.));
#104718=DIRECTION('',(0.,1.,0.));
#104719=DIRECTION('center_axis',(0.,1.,0.));
#104720=DIRECTION('ref_axis',(1.,0.,0.));
#104721=DIRECTION('',(-0.190809912898503,0.,0.981627005099017));
#104722=DIRECTION('',(0.981627005099017,0.,0.190809912898503));
#104723=DIRECTION('',(-0.190809912898503,0.,0.981627005099017));
#104724=DIRECTION('',(0.981627005099017,0.,0.190809912898503));
#104725=DIRECTION('center_axis',(0.981627005099017,0.,0.190809912898503));
#104726=DIRECTION('ref_axis',(0.,-1.,0.));
#104727=DIRECTION('',(-0.190809912898503,0.,0.981627005099017));
#104728=DIRECTION('',(0.,-1.,0.));
#104729=DIRECTION('',(0.,-1.,0.));
#104730=DIRECTION('center_axis',(0.,-1.,0.));
#104731=DIRECTION('ref_axis',(0.,0.,-1.));
#104732=DIRECTION('',(-0.190809912898503,0.,0.981627005099017));
#104733=DIRECTION('',(-0.981627005099017,0.,-0.190809912898503));
#104734=DIRECTION('',(-0.981627005099017,0.,-0.190809912898503));
#104735=DIRECTION('center_axis',(-0.981627005099017,0.,-0.190809912898503));
#104736=DIRECTION('ref_axis',(-0.190809912898503,0.,0.981627005099017));
#104737=DIRECTION('',(0.,1.,0.));
#104738=DIRECTION('',(0.,1.,0.));
#104739=DIRECTION('center_axis',(0.,1.,0.));
#104740=DIRECTION('ref_axis',(1.,0.,0.));
#104741=DIRECTION('',(-0.190809912898503,0.,0.981627005099017));
#104742=DIRECTION('',(0.981627005099017,0.,0.190809912898503));
#104743=DIRECTION('',(-0.190809912898503,0.,0.981627005099017));
#104744=DIRECTION('',(0.981627005099017,0.,0.190809912898503));
#104745=DIRECTION('center_axis',(0.981627005099017,0.,0.190809912898503));
#104746=DIRECTION('ref_axis',(0.,-1.,0.));
#104747=DIRECTION('',(-0.190809912898503,0.,0.981627005099017));
#104748=DIRECTION('',(0.,-1.,0.));
#104749=DIRECTION('',(0.,-1.,0.));
#104750=DIRECTION('center_axis',(0.,-1.,0.));
#104751=DIRECTION('ref_axis',(0.,0.,-1.));
#104752=DIRECTION('',(-0.190809912898503,0.,0.981627005099017));
#104753=DIRECTION('',(-0.981627005099017,0.,-0.190809912898503));
#104754=DIRECTION('',(-0.981627005099017,0.,-0.190809912898503));
#104755=DIRECTION('center_axis',(-0.981627005099017,0.,-0.190809912898503));
#104756=DIRECTION('ref_axis',(-0.190809912898503,0.,0.981627005099017));
#104757=DIRECTION('',(0.,1.,0.));
#104758=DIRECTION('',(0.,1.,0.));
#104759=DIRECTION('center_axis',(0.,1.,0.));
#104760=DIRECTION('ref_axis',(1.,0.,0.));
#104761=DIRECTION('',(-0.190809912898503,0.,0.981627005099017));
#104762=DIRECTION('',(0.981627005099017,0.,0.190809912898503));
#104763=DIRECTION('',(-0.190809912898503,0.,0.981627005099017));
#104764=DIRECTION('',(0.981627005099017,0.,0.190809912898503));
#104765=DIRECTION('center_axis',(0.981627005099017,0.,0.190809912898503));
#104766=DIRECTION('ref_axis',(0.,-1.,0.));
#104767=DIRECTION('',(-0.190809912898503,0.,0.981627005099017));
#104768=DIRECTION('',(0.,-1.,0.));
#104769=DIRECTION('',(0.,-1.,0.));
#104770=DIRECTION('center_axis',(0.,-1.,0.));
#104771=DIRECTION('ref_axis',(0.,0.,-1.));
#104772=DIRECTION('',(-0.190809912898503,0.,0.981627005099017));
#104773=DIRECTION('',(-0.981627005099017,0.,-0.190809912898503));
#104774=DIRECTION('',(-0.981627005099017,0.,-0.190809912898503));
#104775=DIRECTION('center_axis',(-0.981627005099017,0.,-0.190809912898503));
#104776=DIRECTION('ref_axis',(-0.190809912898503,0.,0.981627005099017));
#104777=DIRECTION('',(0.,1.,0.));
#104778=DIRECTION('',(0.,1.,0.));
#104779=DIRECTION('center_axis',(0.,1.,0.));
#104780=DIRECTION('ref_axis',(1.,0.,0.));
#104781=DIRECTION('',(-0.190809912898503,0.,0.981627005099017));
#104782=DIRECTION('',(0.981627005099017,0.,0.190809912898503));
#104783=DIRECTION('',(-0.190809912898503,0.,0.981627005099017));
#104784=DIRECTION('',(0.981627005099017,0.,0.190809912898503));
#104785=DIRECTION('center_axis',(0.981627005099017,0.,0.190809912898503));
#104786=DIRECTION('ref_axis',(0.,-1.,0.));
#104787=DIRECTION('',(-0.190809912898503,0.,0.981627005099017));
#104788=DIRECTION('',(0.,-1.,0.));
#104789=DIRECTION('',(0.,-1.,0.));
#104790=DIRECTION('center_axis',(0.,-1.,0.));
#104791=DIRECTION('ref_axis',(0.,0.,-1.));
#104792=DIRECTION('',(-0.190809912898503,0.,0.981627005099017));
#104793=DIRECTION('',(-0.981627005099017,0.,-0.190809912898503));
#104794=DIRECTION('',(-0.981627005099017,0.,-0.190809912898503));
#104795=DIRECTION('center_axis',(-0.981627005099017,0.,-0.190809912898503));
#104796=DIRECTION('ref_axis',(-0.190809912898503,0.,0.981627005099017));
#104797=DIRECTION('',(0.,1.,0.));
#104798=DIRECTION('',(0.,1.,0.));
#104799=DIRECTION('center_axis',(0.,1.,0.));
#104800=DIRECTION('ref_axis',(1.,0.,0.));
#104801=DIRECTION('',(-0.190809912898503,0.,0.981627005099017));
#104802=DIRECTION('',(0.981627005099017,0.,0.190809912898503));
#104803=DIRECTION('',(-0.190809912898503,0.,0.981627005099017));
#104804=DIRECTION('',(0.981627005099017,0.,0.190809912898503));
#104805=DIRECTION('center_axis',(0.981627005099017,0.,0.190809912898503));
#104806=DIRECTION('ref_axis',(0.,-1.,0.));
#104807=DIRECTION('',(-0.190809912898503,0.,0.981627005099017));
#104808=DIRECTION('',(0.,-1.,0.));
#104809=DIRECTION('',(0.,-1.,0.));
#104810=DIRECTION('center_axis',(0.,-1.,0.));
#104811=DIRECTION('ref_axis',(0.,0.,-1.));
#104812=DIRECTION('',(-0.190809912898503,0.,0.981627005099017));
#104813=DIRECTION('',(-0.981627005099017,0.,-0.190809912898503));
#104814=DIRECTION('',(-0.981627005099017,0.,-0.190809912898503));
#104815=DIRECTION('center_axis',(-0.981627005099017,0.,-0.190809912898503));
#104816=DIRECTION('ref_axis',(-0.190809912898503,0.,0.981627005099017));
#104817=DIRECTION('',(0.,1.,0.));
#104818=DIRECTION('',(0.,1.,0.));
#104819=DIRECTION('center_axis',(0.,1.,0.));
#104820=DIRECTION('ref_axis',(1.,0.,0.));
#104821=DIRECTION('',(-0.190809912898503,0.,0.981627005099017));
#104822=DIRECTION('',(0.981627005099017,0.,0.190809912898503));
#104823=DIRECTION('',(-0.190809912898503,0.,0.981627005099017));
#104824=DIRECTION('',(0.981627005099017,0.,0.190809912898503));
#104825=DIRECTION('center_axis',(0.981627005099017,0.,0.190809912898503));
#104826=DIRECTION('ref_axis',(0.,-1.,0.));
#104827=DIRECTION('',(-0.190809912898503,0.,0.981627005099017));
#104828=DIRECTION('',(0.,-1.,0.));
#104829=DIRECTION('',(0.,-1.,0.));
#104830=DIRECTION('center_axis',(0.,-1.,0.));
#104831=DIRECTION('ref_axis',(0.,0.,-1.));
#104832=DIRECTION('',(-0.190809912898503,0.,0.981627005099017));
#104833=DIRECTION('',(-0.981627005099017,0.,-0.190809912898503));
#104834=DIRECTION('',(-0.981627005099017,0.,-0.190809912898503));
#104835=DIRECTION('center_axis',(-0.981627005099017,0.,-0.190809912898503));
#104836=DIRECTION('ref_axis',(-0.190809912898503,0.,0.981627005099017));
#104837=DIRECTION('',(0.,1.,0.));
#104838=DIRECTION('',(0.,1.,0.));
#104839=DIRECTION('center_axis',(0.,1.,0.));
#104840=DIRECTION('ref_axis',(1.,0.,0.));
#104841=DIRECTION('',(-0.190809912898503,0.,0.981627005099017));
#104842=DIRECTION('',(0.981627005099017,0.,0.190809912898503));
#104843=DIRECTION('',(-0.190809912898503,0.,0.981627005099017));
#104844=DIRECTION('',(0.981627005099017,0.,0.190809912898503));
#104845=DIRECTION('center_axis',(0.981627005099017,0.,0.190809912898503));
#104846=DIRECTION('ref_axis',(0.,-1.,0.));
#104847=DIRECTION('',(-0.190809912898503,0.,0.981627005099017));
#104848=DIRECTION('',(0.,-1.,0.));
#104849=DIRECTION('',(0.,-1.,0.));
#104850=DIRECTION('center_axis',(0.,-1.,0.));
#104851=DIRECTION('ref_axis',(0.,0.,-1.));
#104852=DIRECTION('',(-0.190809912898503,0.,0.981627005099017));
#104853=DIRECTION('',(-0.981627005099017,0.,-0.190809912898503));
#104854=DIRECTION('',(-0.981627005099017,0.,-0.190809912898503));
#104855=DIRECTION('center_axis',(-0.981627005099017,0.,-0.190809912898503));
#104856=DIRECTION('ref_axis',(-0.190809912898503,0.,0.981627005099017));
#104857=DIRECTION('',(0.,1.,0.));
#104858=DIRECTION('',(0.,1.,0.));
#104859=DIRECTION('center_axis',(0.,1.,0.));
#104860=DIRECTION('ref_axis',(1.,0.,0.));
#104861=DIRECTION('',(-0.190809912898503,0.,0.981627005099017));
#104862=DIRECTION('',(0.981627005099017,0.,0.190809912898503));
#104863=DIRECTION('',(-0.190809912898503,0.,0.981627005099017));
#104864=DIRECTION('',(0.981627005099017,0.,0.190809912898503));
#104865=DIRECTION('center_axis',(0.981627005099017,0.,0.190809912898503));
#104866=DIRECTION('ref_axis',(0.,-1.,0.));
#104867=DIRECTION('',(-0.190809912898503,0.,0.981627005099017));
#104868=DIRECTION('',(0.,-1.,0.));
#104869=DIRECTION('',(0.,-1.,0.));
#104870=DIRECTION('center_axis',(0.,-1.,0.));
#104871=DIRECTION('ref_axis',(0.,0.,-1.));
#104872=DIRECTION('',(-0.190809912898503,0.,0.981627005099017));
#104873=DIRECTION('',(-0.981627005099017,0.,-0.190809912898503));
#104874=DIRECTION('',(-0.981627005099017,0.,-0.190809912898503));
#104875=DIRECTION('center_axis',(-0.981627005099017,0.,-0.190809912898503));
#104876=DIRECTION('ref_axis',(-0.190809912898503,0.,0.981627005099017));
#104877=DIRECTION('',(0.,1.,0.));
#104878=DIRECTION('',(0.,1.,0.));
#104879=DIRECTION('center_axis',(0.,1.,0.));
#104880=DIRECTION('ref_axis',(1.,0.,0.));
#104881=DIRECTION('',(-0.190809912898503,0.,0.981627005099017));
#104882=DIRECTION('',(0.981627005099017,0.,0.190809912898503));
#104883=DIRECTION('',(-0.190809912898503,0.,0.981627005099017));
#104884=DIRECTION('',(0.981627005099017,0.,0.190809912898503));
#104885=DIRECTION('center_axis',(0.981627005099017,0.,0.190809912898503));
#104886=DIRECTION('ref_axis',(0.,-1.,0.));
#104887=DIRECTION('',(-0.190809912898503,0.,0.981627005099017));
#104888=DIRECTION('',(0.,-1.,0.));
#104889=DIRECTION('',(0.,-1.,0.));
#104890=DIRECTION('center_axis',(0.,-1.,0.));
#104891=DIRECTION('ref_axis',(0.,0.,-1.));
#104892=DIRECTION('',(-0.190809912898503,0.,0.981627005099017));
#104893=DIRECTION('',(-0.981627005099017,0.,-0.190809912898503));
#104894=DIRECTION('',(-0.981627005099017,0.,-0.190809912898503));
#104895=DIRECTION('center_axis',(-0.981627005099017,0.,-0.190809912898503));
#104896=DIRECTION('ref_axis',(-0.190809912898503,0.,0.981627005099017));
#104897=DIRECTION('',(0.,1.,0.));
#104898=DIRECTION('',(0.,1.,0.));
#104899=DIRECTION('center_axis',(0.,1.,0.));
#104900=DIRECTION('ref_axis',(1.,0.,0.));
#104901=DIRECTION('',(-0.190809912898503,0.,0.981627005099017));
#104902=DIRECTION('',(0.981627005099017,0.,0.190809912898503));
#104903=DIRECTION('',(-0.190809912898503,0.,0.981627005099017));
#104904=DIRECTION('',(0.981627005099017,0.,0.190809912898503));
#104905=DIRECTION('center_axis',(0.981627005099017,0.,0.190809912898503));
#104906=DIRECTION('ref_axis',(0.,-1.,0.));
#104907=DIRECTION('',(-0.190809912898503,0.,0.981627005099017));
#104908=DIRECTION('',(0.,-1.,0.));
#104909=DIRECTION('',(0.,-1.,0.));
#104910=DIRECTION('center_axis',(0.,-1.,0.));
#104911=DIRECTION('ref_axis',(0.,0.,-1.));
#104912=DIRECTION('',(-0.190809912898503,0.,0.981627005099017));
#104913=DIRECTION('',(-0.981627005099017,0.,-0.190809912898503));
#104914=DIRECTION('',(-0.981627005099017,0.,-0.190809912898503));
#104915=DIRECTION('center_axis',(-0.981627005099017,0.,-0.190809912898503));
#104916=DIRECTION('ref_axis',(-0.190809912898503,0.,0.981627005099017));
#104917=DIRECTION('',(0.,1.,0.));
#104918=DIRECTION('',(0.,1.,0.));
#104919=DIRECTION('center_axis',(0.,1.,0.));
#104920=DIRECTION('ref_axis',(1.,0.,0.));
#104921=DIRECTION('',(-0.190809912898503,0.,0.981627005099017));
#104922=DIRECTION('',(0.981627005099017,0.,0.190809912898503));
#104923=DIRECTION('',(-0.190809912898503,0.,0.981627005099017));
#104924=DIRECTION('',(0.981627005099017,0.,0.190809912898503));
#104925=DIRECTION('center_axis',(0.981627005099017,0.,0.190809912898503));
#104926=DIRECTION('ref_axis',(0.,-1.,0.));
#104927=DIRECTION('',(-0.190809912898503,0.,0.981627005099017));
#104928=DIRECTION('',(0.,-1.,0.));
#104929=DIRECTION('',(0.,-1.,0.));
#104930=DIRECTION('center_axis',(0.,-1.,0.));
#104931=DIRECTION('ref_axis',(0.,0.,-1.));
#104932=DIRECTION('',(-0.190809912898503,0.,0.981627005099017));
#104933=DIRECTION('',(-0.981627005099017,0.,-0.190809912898503));
#104934=DIRECTION('',(-0.981627005099017,0.,-0.190809912898503));
#104935=DIRECTION('center_axis',(-0.981627005099017,0.,-0.190809912898503));
#104936=DIRECTION('ref_axis',(-0.190809912898503,0.,0.981627005099017));
#104937=DIRECTION('',(0.,1.,0.));
#104938=DIRECTION('',(0.,1.,0.));
#104939=DIRECTION('center_axis',(0.,1.,0.));
#104940=DIRECTION('ref_axis',(1.,0.,0.));
#104941=DIRECTION('',(-0.190809912898503,0.,0.981627005099017));
#104942=DIRECTION('',(0.981627005099017,0.,0.190809912898503));
#104943=DIRECTION('',(-0.190809912898503,0.,0.981627005099017));
#104944=DIRECTION('',(0.981627005099017,0.,0.190809912898503));
#104945=DIRECTION('center_axis',(0.981627005099017,0.,0.190809912898503));
#104946=DIRECTION('ref_axis',(0.,-1.,0.));
#104947=DIRECTION('',(-0.190809912898503,0.,0.981627005099017));
#104948=DIRECTION('',(0.,-1.,0.));
#104949=DIRECTION('',(0.,-1.,0.));
#104950=DIRECTION('center_axis',(0.,-1.,0.));
#104951=DIRECTION('ref_axis',(0.,0.,-1.));
#104952=DIRECTION('',(-0.190809912898503,0.,0.981627005099017));
#104953=DIRECTION('',(-0.981627005099017,0.,-0.190809912898503));
#104954=DIRECTION('',(-0.981627005099017,0.,-0.190809912898503));
#104955=DIRECTION('center_axis',(-0.981627005099017,0.,-0.190809912898503));
#104956=DIRECTION('ref_axis',(-0.190809912898503,0.,0.981627005099017));
#104957=DIRECTION('',(0.,1.,0.));
#104958=DIRECTION('',(0.,1.,0.));
#104959=DIRECTION('center_axis',(0.,1.,0.));
#104960=DIRECTION('ref_axis',(1.,0.,0.));
#104961=DIRECTION('',(-0.190809912898503,0.,0.981627005099017));
#104962=DIRECTION('',(0.981627005099017,0.,0.190809912898503));
#104963=DIRECTION('',(-0.190809912898503,0.,0.981627005099017));
#104964=DIRECTION('',(0.981627005099017,0.,0.190809912898503));
#104965=DIRECTION('center_axis',(0.981627005099017,0.,0.190809912898503));
#104966=DIRECTION('ref_axis',(0.,-1.,0.));
#104967=DIRECTION('',(-0.190809912898503,0.,0.981627005099017));
#104968=DIRECTION('',(0.,-1.,0.));
#104969=DIRECTION('',(0.,-1.,0.));
#104970=DIRECTION('center_axis',(0.,-1.,0.));
#104971=DIRECTION('ref_axis',(0.,0.,-1.));
#104972=DIRECTION('',(-0.190809912898503,0.,0.981627005099017));
#104973=DIRECTION('',(-0.981627005099017,0.,-0.190809912898503));
#104974=DIRECTION('',(-0.981627005099017,0.,-0.190809912898503));
#104975=DIRECTION('center_axis',(-0.981627005099017,0.,-0.190809912898503));
#104976=DIRECTION('ref_axis',(-0.190809912898503,0.,0.981627005099017));
#104977=DIRECTION('',(0.,1.,0.));
#104978=DIRECTION('',(0.,1.,0.));
#104979=DIRECTION('center_axis',(0.,1.,0.));
#104980=DIRECTION('ref_axis',(1.,0.,0.));
#104981=DIRECTION('',(-0.190809912898503,0.,0.981627005099017));
#104982=DIRECTION('',(0.981627005099017,0.,0.190809912898503));
#104983=DIRECTION('',(-0.190809912898503,0.,0.981627005099017));
#104984=DIRECTION('',(0.981627005099017,0.,0.190809912898503));
#104985=DIRECTION('center_axis',(0.981627005099017,0.,0.190809912898503));
#104986=DIRECTION('ref_axis',(0.,-1.,0.));
#104987=DIRECTION('',(-0.190809912898503,0.,0.981627005099017));
#104988=DIRECTION('',(0.,-1.,0.));
#104989=DIRECTION('',(0.,-1.,0.));
#104990=DIRECTION('center_axis',(0.,-1.,0.));
#104991=DIRECTION('ref_axis',(0.,0.,-1.));
#104992=DIRECTION('',(-0.190809912898503,0.,0.981627005099017));
#104993=DIRECTION('',(-0.981627005099017,0.,-0.190809912898503));
#104994=DIRECTION('',(-0.981627005099017,0.,-0.190809912898503));
#104995=DIRECTION('center_axis',(-0.981627005099017,0.,-0.190809912898503));
#104996=DIRECTION('ref_axis',(-0.190809912898503,0.,0.981627005099017));
#104997=DIRECTION('',(0.,1.,0.));
#104998=DIRECTION('',(0.,1.,0.));
#104999=DIRECTION('center_axis',(0.,1.,0.));
#105000=DIRECTION('ref_axis',(1.,0.,0.));
#105001=DIRECTION('',(-0.190809912898503,0.,0.981627005099017));
#105002=DIRECTION('',(0.981627005099017,0.,0.190809912898503));
#105003=DIRECTION('',(-0.190809912898503,0.,0.981627005099017));
#105004=DIRECTION('',(0.981627005099017,0.,0.190809912898503));
#105005=DIRECTION('center_axis',(0.981627005099017,0.,0.190809912898503));
#105006=DIRECTION('ref_axis',(0.,-1.,0.));
#105007=DIRECTION('',(-0.190809912898503,0.,0.981627005099017));
#105008=DIRECTION('',(0.,-1.,0.));
#105009=DIRECTION('',(0.,-1.,0.));
#105010=DIRECTION('center_axis',(0.,-1.,0.));
#105011=DIRECTION('ref_axis',(0.,0.,-1.));
#105012=DIRECTION('',(-0.190809912898503,0.,0.981627005099017));
#105013=DIRECTION('',(-0.981627005099017,0.,-0.190809912898503));
#105014=DIRECTION('',(-0.981627005099017,0.,-0.190809912898503));
#105015=DIRECTION('center_axis',(-0.981627005099017,0.,-0.190809912898503));
#105016=DIRECTION('ref_axis',(-0.190809912898503,0.,0.981627005099017));
#105017=DIRECTION('',(0.,1.,0.));
#105018=DIRECTION('',(0.,1.,0.));
#105019=DIRECTION('center_axis',(0.,1.,0.));
#105020=DIRECTION('ref_axis',(1.,0.,0.));
#105021=DIRECTION('',(-0.190809912898503,0.,0.981627005099017));
#105022=DIRECTION('',(0.981627005099017,0.,0.190809912898503));
#105023=DIRECTION('',(-0.190809912898503,0.,0.981627005099017));
#105024=DIRECTION('',(0.981627005099017,0.,0.190809912898503));
#105025=DIRECTION('center_axis',(0.981627005099017,0.,0.190809912898503));
#105026=DIRECTION('ref_axis',(0.,-1.,0.));
#105027=DIRECTION('',(-0.190809912898503,0.,0.981627005099017));
#105028=DIRECTION('',(0.,-1.,0.));
#105029=DIRECTION('',(0.,-1.,0.));
#105030=DIRECTION('center_axis',(0.,-1.,0.));
#105031=DIRECTION('ref_axis',(0.,0.,-1.));
#105032=DIRECTION('',(-0.190809912898503,0.,0.981627005099017));
#105033=DIRECTION('',(-0.981627005099017,0.,-0.190809912898503));
#105034=DIRECTION('',(-0.981627005099017,0.,-0.190809912898503));
#105035=DIRECTION('center_axis',(-0.981627005099017,0.,-0.190809912898503));
#105036=DIRECTION('ref_axis',(-0.190809912898503,0.,0.981627005099017));
#105037=DIRECTION('',(0.,1.,0.));
#105038=DIRECTION('',(0.,1.,0.));
#105039=DIRECTION('center_axis',(0.,1.,0.));
#105040=DIRECTION('ref_axis',(1.,0.,0.));
#105041=DIRECTION('',(-0.190809912898503,0.,0.981627005099017));
#105042=DIRECTION('',(0.981627005099017,0.,0.190809912898503));
#105043=DIRECTION('',(-0.190809912898503,0.,0.981627005099017));
#105044=DIRECTION('',(0.981627005099017,0.,0.190809912898503));
#105045=DIRECTION('center_axis',(0.981627005099017,0.,0.190809912898503));
#105046=DIRECTION('ref_axis',(0.,-1.,0.));
#105047=DIRECTION('',(-0.190809912898503,0.,0.981627005099017));
#105048=DIRECTION('',(0.,-1.,0.));
#105049=DIRECTION('',(0.,-1.,0.));
#105050=DIRECTION('center_axis',(0.,-1.,0.));
#105051=DIRECTION('ref_axis',(0.,0.,-1.));
#105052=DIRECTION('',(-0.190809912898503,0.,0.981627005099017));
#105053=DIRECTION('',(-0.981627005099017,0.,-0.190809912898503));
#105054=DIRECTION('',(-0.981627005099017,0.,-0.190809912898503));
#105055=DIRECTION('center_axis',(-0.981627005099017,0.,-0.190809912898503));
#105056=DIRECTION('ref_axis',(-0.190809912898503,0.,0.981627005099017));
#105057=DIRECTION('',(0.,1.,0.));
#105058=DIRECTION('',(0.,1.,0.));
#105059=DIRECTION('center_axis',(0.,1.,0.));
#105060=DIRECTION('ref_axis',(1.,0.,0.));
#105061=DIRECTION('',(-0.190809912898503,0.,0.981627005099017));
#105062=DIRECTION('',(0.981627005099017,0.,0.190809912898503));
#105063=DIRECTION('',(-0.190809912898503,0.,0.981627005099017));
#105064=DIRECTION('',(0.981627005099017,0.,0.190809912898503));
#105065=DIRECTION('center_axis',(0.981627005099017,0.,0.190809912898503));
#105066=DIRECTION('ref_axis',(0.,-1.,0.));
#105067=DIRECTION('',(-0.190809912898503,0.,0.981627005099017));
#105068=DIRECTION('',(0.,-1.,0.));
#105069=DIRECTION('',(0.,-1.,0.));
#105070=DIRECTION('center_axis',(0.,-1.,0.));
#105071=DIRECTION('ref_axis',(0.,0.,-1.));
#105072=DIRECTION('',(-0.190809912898503,0.,0.981627005099017));
#105073=DIRECTION('',(-0.981627005099017,0.,-0.190809912898503));
#105074=DIRECTION('',(-0.981627005099017,0.,-0.190809912898503));
#105075=DIRECTION('center_axis',(-0.981627005099017,0.,-0.190809912898503));
#105076=DIRECTION('ref_axis',(-0.190809912898503,0.,0.981627005099017));
#105077=DIRECTION('',(0.,1.,0.));
#105078=DIRECTION('',(0.,1.,0.));
#105079=DIRECTION('center_axis',(0.,1.,0.));
#105080=DIRECTION('ref_axis',(1.,0.,0.));
#105081=DIRECTION('',(-0.190809912898503,0.,0.981627005099017));
#105082=DIRECTION('',(0.981627005099017,0.,0.190809912898503));
#105083=DIRECTION('',(-0.190809912898503,0.,0.981627005099017));
#105084=DIRECTION('',(0.981627005099017,0.,0.190809912898503));
#105085=DIRECTION('center_axis',(0.981627005099017,0.,0.190809912898503));
#105086=DIRECTION('ref_axis',(0.,-1.,0.));
#105087=DIRECTION('',(-0.190809912898503,0.,0.981627005099017));
#105088=DIRECTION('',(0.,-1.,0.));
#105089=DIRECTION('',(0.,-1.,0.));
#105090=DIRECTION('center_axis',(0.,-1.,0.));
#105091=DIRECTION('ref_axis',(0.,0.,-1.));
#105092=DIRECTION('',(-0.190809912898503,0.,0.981627005099017));
#105093=DIRECTION('',(-0.981627005099017,0.,-0.190809912898503));
#105094=DIRECTION('',(-0.981627005099017,0.,-0.190809912898503));
#105095=DIRECTION('center_axis',(-0.981627005099017,0.,-0.190809912898503));
#105096=DIRECTION('ref_axis',(-0.190809912898503,0.,0.981627005099017));
#105097=DIRECTION('',(0.,1.,0.));
#105098=DIRECTION('',(0.,1.,0.));
#105099=DIRECTION('center_axis',(0.,1.,0.));
#105100=DIRECTION('ref_axis',(1.,0.,0.));
#105101=DIRECTION('',(-0.190809912898503,0.,0.981627005099017));
#105102=DIRECTION('',(0.981627005099017,0.,0.190809912898503));
#105103=DIRECTION('',(-0.190809912898503,0.,0.981627005099017));
#105104=DIRECTION('',(0.981627005099017,0.,0.190809912898503));
#105105=DIRECTION('center_axis',(0.981627005099017,0.,0.190809912898503));
#105106=DIRECTION('ref_axis',(0.,-1.,0.));
#105107=DIRECTION('',(-0.190809912898503,0.,0.981627005099017));
#105108=DIRECTION('',(0.,-1.,0.));
#105109=DIRECTION('',(0.,-1.,0.));
#105110=DIRECTION('center_axis',(0.,-1.,0.));
#105111=DIRECTION('ref_axis',(0.,0.,-1.));
#105112=DIRECTION('',(-0.190809912898503,0.,0.981627005099017));
#105113=DIRECTION('',(-0.981627005099017,0.,-0.190809912898503));
#105114=DIRECTION('',(-0.981627005099017,0.,-0.190809912898503));
#105115=DIRECTION('center_axis',(-0.981627005099017,0.,-0.190809912898503));
#105116=DIRECTION('ref_axis',(-0.190809912898503,0.,0.981627005099017));
#105117=DIRECTION('',(0.,1.,0.));
#105118=DIRECTION('',(0.,1.,0.));
#105119=DIRECTION('center_axis',(0.,1.,0.));
#105120=DIRECTION('ref_axis',(1.,0.,0.));
#105121=DIRECTION('',(-0.190809912898503,0.,0.981627005099017));
#105122=DIRECTION('',(0.981627005099017,0.,0.190809912898503));
#105123=DIRECTION('',(-0.190809912898503,0.,0.981627005099017));
#105124=DIRECTION('',(0.981627005099017,0.,0.190809912898503));
#105125=DIRECTION('center_axis',(0.981627005099017,0.,0.190809912898503));
#105126=DIRECTION('ref_axis',(0.,-1.,0.));
#105127=DIRECTION('',(-0.190809912898503,0.,0.981627005099017));
#105128=DIRECTION('',(0.,-1.,0.));
#105129=DIRECTION('',(0.,-1.,0.));
#105130=DIRECTION('center_axis',(0.,-1.,0.));
#105131=DIRECTION('ref_axis',(0.,0.,-1.));
#105132=DIRECTION('',(-0.190809912898503,0.,0.981627005099017));
#105133=DIRECTION('',(-0.981627005099017,0.,-0.190809912898503));
#105134=DIRECTION('',(-0.981627005099017,0.,-0.190809912898503));
#105135=DIRECTION('center_axis',(-0.981627005099017,0.,-0.190809912898503));
#105136=DIRECTION('ref_axis',(-0.190809912898503,0.,0.981627005099017));
#105137=DIRECTION('',(0.,1.,0.));
#105138=DIRECTION('',(0.,1.,0.));
#105139=DIRECTION('center_axis',(0.,1.,0.));
#105140=DIRECTION('ref_axis',(1.,0.,0.));
#105141=DIRECTION('',(-0.190809912898503,0.,0.981627005099017));
#105142=DIRECTION('',(0.981627005099017,0.,0.190809912898503));
#105143=DIRECTION('',(-0.190809912898503,0.,0.981627005099017));
#105144=DIRECTION('',(0.981627005099017,0.,0.190809912898503));
#105145=DIRECTION('center_axis',(0.981627005099017,0.,0.190809912898503));
#105146=DIRECTION('ref_axis',(0.,-1.,0.));
#105147=DIRECTION('',(-0.190809912898503,0.,0.981627005099017));
#105148=DIRECTION('',(0.,-1.,0.));
#105149=DIRECTION('',(0.,-1.,0.));
#105150=DIRECTION('center_axis',(0.,-1.,0.));
#105151=DIRECTION('ref_axis',(0.,0.,-1.));
#105152=DIRECTION('',(-0.190809912898503,0.,0.981627005099017));
#105153=DIRECTION('',(-0.981627005099017,0.,-0.190809912898503));
#105154=DIRECTION('',(-0.981627005099017,0.,-0.190809912898503));
#105155=DIRECTION('center_axis',(-0.981627005099017,0.,-0.190809912898503));
#105156=DIRECTION('ref_axis',(-0.190809912898503,0.,0.981627005099017));
#105157=DIRECTION('',(0.,1.,0.));
#105158=DIRECTION('',(0.,1.,0.));
#105159=DIRECTION('center_axis',(0.,1.,0.));
#105160=DIRECTION('ref_axis',(1.,0.,0.));
#105161=DIRECTION('',(-0.190809912898503,0.,0.981627005099017));
#105162=DIRECTION('',(0.981627005099017,0.,0.190809912898503));
#105163=DIRECTION('',(-0.190809912898503,0.,0.981627005099017));
#105164=DIRECTION('',(0.981627005099017,0.,0.190809912898503));
#105165=DIRECTION('center_axis',(0.981627005099017,0.,0.190809912898503));
#105166=DIRECTION('ref_axis',(0.,-1.,0.));
#105167=DIRECTION('',(-0.190809912898503,0.,0.981627005099017));
#105168=DIRECTION('',(0.,-1.,0.));
#105169=DIRECTION('',(0.,-1.,0.));
#105170=DIRECTION('center_axis',(0.,-1.,0.));
#105171=DIRECTION('ref_axis',(0.,0.,-1.));
#105172=DIRECTION('',(-0.190809912898503,0.,0.981627005099017));
#105173=DIRECTION('',(-0.981627005099017,0.,-0.190809912898503));
#105174=DIRECTION('',(-0.981627005099017,0.,-0.190809912898503));
#105175=DIRECTION('center_axis',(-0.981627005099017,0.,-0.190809912898503));
#105176=DIRECTION('ref_axis',(-0.190809912898503,0.,0.981627005099017));
#105177=DIRECTION('',(0.,1.,0.));
#105178=DIRECTION('',(0.,1.,0.));
#105179=DIRECTION('center_axis',(0.,1.,0.));
#105180=DIRECTION('ref_axis',(1.,0.,0.));
#105181=DIRECTION('',(-0.190809912898503,0.,0.981627005099017));
#105182=DIRECTION('',(0.981627005099017,0.,0.190809912898503));
#105183=DIRECTION('',(-0.190809912898503,0.,0.981627005099017));
#105184=DIRECTION('',(0.981627005099017,0.,0.190809912898503));
#105185=DIRECTION('center_axis',(0.981627005099017,0.,0.190809912898503));
#105186=DIRECTION('ref_axis',(0.,-1.,0.));
#105187=DIRECTION('',(-0.190809912898503,0.,0.981627005099017));
#105188=DIRECTION('',(0.,-1.,0.));
#105189=DIRECTION('',(0.,-1.,0.));
#105190=DIRECTION('center_axis',(0.,-1.,0.));
#105191=DIRECTION('ref_axis',(0.,0.,-1.));
#105192=DIRECTION('',(-0.190809912898503,0.,0.981627005099017));
#105193=DIRECTION('',(-0.981627005099017,0.,-0.190809912898503));
#105194=DIRECTION('',(-0.981627005099017,0.,-0.190809912898503));
#105195=DIRECTION('center_axis',(-0.981627005099017,0.,-0.190809912898503));
#105196=DIRECTION('ref_axis',(-0.190809912898503,0.,0.981627005099017));
#105197=DIRECTION('',(0.,1.,0.));
#105198=DIRECTION('',(0.,1.,0.));
#105199=DIRECTION('center_axis',(0.,1.,0.));
#105200=DIRECTION('ref_axis',(1.,0.,0.));
#105201=DIRECTION('',(-0.190809912898503,0.,0.981627005099017));
#105202=DIRECTION('',(0.981627005099017,0.,0.190809912898503));
#105203=DIRECTION('',(-0.190809912898503,0.,0.981627005099017));
#105204=DIRECTION('',(0.981627005099017,0.,0.190809912898503));
#105205=DIRECTION('center_axis',(0.981627005099017,0.,0.190809912898503));
#105206=DIRECTION('ref_axis',(0.,-1.,0.));
#105207=DIRECTION('',(-0.190809912898503,0.,0.981627005099017));
#105208=DIRECTION('',(0.,-1.,0.));
#105209=DIRECTION('',(0.,-1.,0.));
#105210=DIRECTION('center_axis',(0.,-1.,0.));
#105211=DIRECTION('ref_axis',(0.,0.,-1.));
#105212=DIRECTION('',(-0.190809912898503,0.,0.981627005099017));
#105213=DIRECTION('',(-0.981627005099017,0.,-0.190809912898503));
#105214=DIRECTION('',(-0.981627005099017,0.,-0.190809912898503));
#105215=DIRECTION('center_axis',(-0.981627005099017,0.,-0.190809912898503));
#105216=DIRECTION('ref_axis',(-0.190809912898503,0.,0.981627005099017));
#105217=DIRECTION('',(0.,1.,0.));
#105218=DIRECTION('',(0.,1.,0.));
#105219=DIRECTION('center_axis',(0.,1.,0.));
#105220=DIRECTION('ref_axis',(1.,0.,0.));
#105221=DIRECTION('',(-0.190809912898503,0.,0.981627005099017));
#105222=DIRECTION('',(0.981627005099017,0.,0.190809912898503));
#105223=DIRECTION('',(-0.190809912898503,0.,0.981627005099017));
#105224=DIRECTION('',(0.981627005099017,0.,0.190809912898503));
#105225=DIRECTION('center_axis',(0.981627005099017,0.,0.190809912898503));
#105226=DIRECTION('ref_axis',(0.,-1.,0.));
#105227=DIRECTION('',(-0.190809912898503,0.,0.981627005099017));
#105228=DIRECTION('',(0.,-1.,0.));
#105229=DIRECTION('',(0.,-1.,0.));
#105230=DIRECTION('center_axis',(0.,-1.,0.));
#105231=DIRECTION('ref_axis',(0.,0.,-1.));
#105232=DIRECTION('',(-0.190809912898503,0.,0.981627005099017));
#105233=DIRECTION('',(-0.981627005099017,0.,-0.190809912898503));
#105234=DIRECTION('',(-0.981627005099017,0.,-0.190809912898503));
#105235=DIRECTION('center_axis',(-0.981627005099017,0.,-0.190809912898503));
#105236=DIRECTION('ref_axis',(-0.190809912898503,0.,0.981627005099017));
#105237=DIRECTION('',(0.,1.,0.));
#105238=DIRECTION('',(0.,1.,0.));
#105239=DIRECTION('center_axis',(0.,1.,0.));
#105240=DIRECTION('ref_axis',(1.,0.,0.));
#105241=DIRECTION('',(-0.190809912898503,0.,0.981627005099017));
#105242=DIRECTION('',(0.981627005099017,0.,0.190809912898503));
#105243=DIRECTION('',(-0.190809912898503,0.,0.981627005099017));
#105244=DIRECTION('',(0.981627005099017,0.,0.190809912898503));
#105245=DIRECTION('center_axis',(0.981627005099017,0.,0.190809912898503));
#105246=DIRECTION('ref_axis',(0.,-1.,0.));
#105247=DIRECTION('',(-0.190809912898503,0.,0.981627005099017));
#105248=DIRECTION('',(0.,-1.,0.));
#105249=DIRECTION('',(0.,-1.,0.));
#105250=DIRECTION('center_axis',(0.,-1.,0.));
#105251=DIRECTION('ref_axis',(0.,0.,-1.));
#105252=DIRECTION('',(-0.190809912898503,0.,0.981627005099017));
#105253=DIRECTION('',(-0.981627005099017,0.,-0.190809912898503));
#105254=DIRECTION('',(-0.981627005099017,0.,-0.190809912898503));
#105255=DIRECTION('center_axis',(-0.981627005099017,0.,-0.190809912898503));
#105256=DIRECTION('ref_axis',(-0.190809912898503,0.,0.981627005099017));
#105257=DIRECTION('',(0.,1.,0.));
#105258=DIRECTION('',(0.,1.,0.));
#105259=DIRECTION('center_axis',(0.,1.,0.));
#105260=DIRECTION('ref_axis',(1.,0.,0.));
#105261=DIRECTION('',(-0.190809912898503,0.,0.981627005099017));
#105262=DIRECTION('',(0.981627005099017,0.,0.190809912898503));
#105263=DIRECTION('',(-0.190809912898503,0.,0.981627005099017));
#105264=DIRECTION('',(0.981627005099017,0.,0.190809912898503));
#105265=DIRECTION('center_axis',(0.981627005099017,0.,0.190809912898503));
#105266=DIRECTION('ref_axis',(0.,-1.,0.));
#105267=DIRECTION('',(-0.190809912898503,0.,0.981627005099017));
#105268=DIRECTION('',(0.,-1.,0.));
#105269=DIRECTION('',(0.,-1.,0.));
#105270=DIRECTION('center_axis',(0.,-1.,0.));
#105271=DIRECTION('ref_axis',(0.,0.,-1.));
#105272=DIRECTION('',(-0.190809912898503,0.,0.981627005099017));
#105273=DIRECTION('',(-0.981627005099017,0.,-0.190809912898503));
#105274=DIRECTION('',(-0.981627005099017,0.,-0.190809912898503));
#105275=DIRECTION('center_axis',(-0.981627005099017,0.,-0.190809912898503));
#105276=DIRECTION('ref_axis',(-0.190809912898503,0.,0.981627005099017));
#105277=DIRECTION('',(0.,1.,0.));
#105278=DIRECTION('',(0.,1.,0.));
#105279=DIRECTION('center_axis',(0.,1.,0.));
#105280=DIRECTION('ref_axis',(1.,0.,0.));
#105281=DIRECTION('',(-0.190809912898503,0.,0.981627005099017));
#105282=DIRECTION('',(0.981627005099017,0.,0.190809912898503));
#105283=DIRECTION('',(-0.190809912898503,0.,0.981627005099017));
#105284=DIRECTION('',(0.981627005099017,0.,0.190809912898503));
#105285=DIRECTION('center_axis',(0.981627005099017,0.,0.190809912898503));
#105286=DIRECTION('ref_axis',(0.,-1.,0.));
#105287=DIRECTION('',(-0.190809912898503,0.,0.981627005099017));
#105288=DIRECTION('',(0.,-1.,0.));
#105289=DIRECTION('',(0.,-1.,0.));
#105290=DIRECTION('center_axis',(0.,-1.,0.));
#105291=DIRECTION('ref_axis',(0.,0.,-1.));
#105292=DIRECTION('',(-0.190809912898503,0.,0.981627005099017));
#105293=DIRECTION('',(-0.981627005099017,0.,-0.190809912898503));
#105294=DIRECTION('',(-0.981627005099017,0.,-0.190809912898503));
#105295=DIRECTION('center_axis',(-0.981627005099017,0.,-0.190809912898503));
#105296=DIRECTION('ref_axis',(-0.190809912898503,0.,0.981627005099017));
#105297=DIRECTION('',(0.,1.,0.));
#105298=DIRECTION('',(0.,1.,0.));
#105299=DIRECTION('center_axis',(0.,1.,0.));
#105300=DIRECTION('ref_axis',(1.,0.,0.));
#105301=DIRECTION('',(-0.190809912898503,0.,0.981627005099017));
#105302=DIRECTION('',(0.981627005099017,0.,0.190809912898503));
#105303=DIRECTION('',(-0.190809912898503,0.,0.981627005099017));
#105304=DIRECTION('',(0.981627005099017,0.,0.190809912898503));
#105305=DIRECTION('center_axis',(0.981627005099017,0.,0.190809912898503));
#105306=DIRECTION('ref_axis',(0.,-1.,0.));
#105307=DIRECTION('',(-0.190809912898503,0.,0.981627005099017));
#105308=DIRECTION('',(0.,-1.,0.));
#105309=DIRECTION('',(0.,-1.,0.));
#105310=DIRECTION('center_axis',(0.,-1.,0.));
#105311=DIRECTION('ref_axis',(0.,0.,-1.));
#105312=DIRECTION('',(-0.190809912898503,0.,0.981627005099017));
#105313=DIRECTION('',(-0.981627005099017,0.,-0.190809912898503));
#105314=DIRECTION('',(-0.981627005099017,0.,-0.190809912898503));
#105315=DIRECTION('center_axis',(-0.981627005099017,0.,-0.190809912898503));
#105316=DIRECTION('ref_axis',(-0.190809912898503,0.,0.981627005099017));
#105317=DIRECTION('',(0.,1.,0.));
#105318=DIRECTION('',(0.,1.,0.));
#105319=DIRECTION('center_axis',(0.,1.,0.));
#105320=DIRECTION('ref_axis',(1.,0.,0.));
#105321=DIRECTION('',(-0.190809912898503,0.,0.981627005099017));
#105322=DIRECTION('',(0.981627005099017,0.,0.190809912898503));
#105323=DIRECTION('',(-0.190809912898503,0.,0.981627005099017));
#105324=DIRECTION('',(0.981627005099017,0.,0.190809912898503));
#105325=DIRECTION('center_axis',(0.981627005099017,0.,0.190809912898503));
#105326=DIRECTION('ref_axis',(0.,-1.,0.));
#105327=DIRECTION('',(-0.190809912898503,0.,0.981627005099017));
#105328=DIRECTION('',(0.,-1.,0.));
#105329=DIRECTION('',(0.,-1.,0.));
#105330=DIRECTION('center_axis',(0.,-1.,0.));
#105331=DIRECTION('ref_axis',(0.,0.,-1.));
#105332=DIRECTION('',(-0.190809912898503,0.,0.981627005099017));
#105333=DIRECTION('',(-0.981627005099017,0.,-0.190809912898503));
#105334=DIRECTION('',(-0.981627005099017,0.,-0.190809912898503));
#105335=DIRECTION('center_axis',(-0.981627005099017,0.,-0.190809912898503));
#105336=DIRECTION('ref_axis',(-0.190809912898503,0.,0.981627005099017));
#105337=DIRECTION('',(0.,1.,0.));
#105338=DIRECTION('',(0.,1.,0.));
#105339=DIRECTION('center_axis',(0.,1.,0.));
#105340=DIRECTION('ref_axis',(1.,0.,0.));
#105341=DIRECTION('',(-0.190809912898503,0.,0.981627005099017));
#105342=DIRECTION('',(0.981627005099017,0.,0.190809912898503));
#105343=DIRECTION('',(-0.190809912898503,0.,0.981627005099017));
#105344=DIRECTION('',(0.981627005099017,0.,0.190809912898503));
#105345=DIRECTION('center_axis',(0.981627005099017,0.,0.190809912898503));
#105346=DIRECTION('ref_axis',(0.,-1.,0.));
#105347=DIRECTION('',(-0.190809912898503,0.,0.981627005099017));
#105348=DIRECTION('',(0.,-1.,0.));
#105349=DIRECTION('',(0.,-1.,0.));
#105350=DIRECTION('center_axis',(0.,-1.,0.));
#105351=DIRECTION('ref_axis',(0.,0.,-1.));
#105352=DIRECTION('',(-0.190809912898503,0.,0.981627005099017));
#105353=DIRECTION('',(-0.981627005099017,0.,-0.190809912898503));
#105354=DIRECTION('',(-0.981627005099017,0.,-0.190809912898503));
#105355=DIRECTION('center_axis',(-0.981627005099017,0.,-0.190809912898503));
#105356=DIRECTION('ref_axis',(-0.190809912898503,0.,0.981627005099017));
#105357=DIRECTION('',(0.,1.,0.));
#105358=DIRECTION('',(0.,1.,0.));
#105359=DIRECTION('center_axis',(0.,1.,0.));
#105360=DIRECTION('ref_axis',(1.,0.,0.));
#105361=DIRECTION('',(-0.190809912898503,0.,0.981627005099017));
#105362=DIRECTION('',(0.981627005099017,0.,0.190809912898503));
#105363=DIRECTION('',(-0.190809912898503,0.,0.981627005099017));
#105364=DIRECTION('',(0.981627005099017,0.,0.190809912898503));
#105365=DIRECTION('center_axis',(0.981627005099017,0.,0.190809912898503));
#105366=DIRECTION('ref_axis',(0.,-1.,0.));
#105367=DIRECTION('',(-0.190809912898503,0.,0.981627005099017));
#105368=DIRECTION('',(0.,-1.,0.));
#105369=DIRECTION('',(0.,-1.,0.));
#105370=DIRECTION('center_axis',(0.,-1.,0.));
#105371=DIRECTION('ref_axis',(0.,0.,-1.));
#105372=DIRECTION('',(-0.190809912898503,0.,0.981627005099017));
#105373=DIRECTION('',(-0.981627005099017,0.,-0.190809912898503));
#105374=DIRECTION('',(-0.981627005099017,0.,-0.190809912898503));
#105375=DIRECTION('center_axis',(-0.981627005099017,0.,-0.190809912898503));
#105376=DIRECTION('ref_axis',(-0.190809912898503,0.,0.981627005099017));
#105377=DIRECTION('',(0.,1.,0.));
#105378=DIRECTION('',(0.,1.,0.));
#105379=DIRECTION('center_axis',(0.,1.,0.));
#105380=DIRECTION('ref_axis',(1.,0.,0.));
#105381=DIRECTION('',(-0.190809912898503,0.,0.981627005099017));
#105382=DIRECTION('',(0.981627005099017,0.,0.190809912898503));
#105383=DIRECTION('',(-0.190809912898503,0.,0.981627005099017));
#105384=DIRECTION('',(0.981627005099017,0.,0.190809912898503));
#105385=DIRECTION('center_axis',(0.981627005099017,0.,0.190809912898503));
#105386=DIRECTION('ref_axis',(0.,-1.,0.));
#105387=DIRECTION('',(-0.190809912898503,0.,0.981627005099017));
#105388=DIRECTION('',(0.,-1.,0.));
#105389=DIRECTION('',(0.,-1.,0.));
#105390=DIRECTION('center_axis',(0.,-1.,0.));
#105391=DIRECTION('ref_axis',(0.,0.,-1.));
#105392=DIRECTION('',(-0.190809912898503,0.,0.981627005099017));
#105393=DIRECTION('',(-0.981627005099017,0.,-0.190809912898503));
#105394=DIRECTION('',(-0.981627005099017,0.,-0.190809912898503));
#105395=DIRECTION('center_axis',(-0.981627005099017,0.,-0.190809912898503));
#105396=DIRECTION('ref_axis',(-0.190809912898503,0.,0.981627005099017));
#105397=DIRECTION('',(0.,1.,0.));
#105398=DIRECTION('',(0.,1.,0.));
#105399=DIRECTION('center_axis',(0.,1.,0.));
#105400=DIRECTION('ref_axis',(1.,0.,0.));
#105401=DIRECTION('',(-0.190809912898503,0.,0.981627005099017));
#105402=DIRECTION('',(0.981627005099017,0.,0.190809912898503));
#105403=DIRECTION('',(-0.190809912898503,0.,0.981627005099017));
#105404=DIRECTION('',(0.981627005099017,0.,0.190809912898503));
#105405=DIRECTION('center_axis',(0.981627005099017,0.,0.190809912898503));
#105406=DIRECTION('ref_axis',(0.,-1.,0.));
#105407=DIRECTION('',(-0.190809912898503,0.,0.981627005099017));
#105408=DIRECTION('',(0.,-1.,0.));
#105409=DIRECTION('',(0.,-1.,0.));
#105410=DIRECTION('center_axis',(0.,-1.,0.));
#105411=DIRECTION('ref_axis',(0.,0.,-1.));
#105412=DIRECTION('',(-0.190809912898503,0.,0.981627005099017));
#105413=DIRECTION('',(-0.981627005099017,0.,-0.190809912898503));
#105414=DIRECTION('',(-0.981627005099017,0.,-0.190809912898503));
#105415=DIRECTION('center_axis',(-0.981627005099017,0.,-0.190809912898503));
#105416=DIRECTION('ref_axis',(-0.190809912898503,0.,0.981627005099017));
#105417=DIRECTION('',(0.,1.,0.));
#105418=DIRECTION('',(0.,1.,0.));
#105419=DIRECTION('center_axis',(0.,1.,0.));
#105420=DIRECTION('ref_axis',(1.,0.,0.));
#105421=DIRECTION('',(-0.190809912898503,0.,0.981627005099017));
#105422=DIRECTION('',(0.981627005099017,0.,0.190809912898503));
#105423=DIRECTION('',(-0.190809912898503,0.,0.981627005099017));
#105424=DIRECTION('',(0.981627005099017,0.,0.190809912898503));
#105425=DIRECTION('center_axis',(0.981627005099017,0.,0.190809912898503));
#105426=DIRECTION('ref_axis',(0.,-1.,0.));
#105427=DIRECTION('',(-0.190809912898503,0.,0.981627005099017));
#105428=DIRECTION('',(0.,-1.,0.));
#105429=DIRECTION('',(0.,-1.,0.));
#105430=DIRECTION('center_axis',(0.,-1.,0.));
#105431=DIRECTION('ref_axis',(0.,0.,-1.));
#105432=DIRECTION('',(-0.190809912898503,0.,0.981627005099017));
#105433=DIRECTION('',(-0.981627005099017,0.,-0.190809912898503));
#105434=DIRECTION('',(-0.981627005099017,0.,-0.190809912898503));
#105435=DIRECTION('center_axis',(-0.981627005099017,0.,-0.190809912898503));
#105436=DIRECTION('ref_axis',(-0.190809912898503,0.,0.981627005099017));
#105437=DIRECTION('',(0.,1.,0.));
#105438=DIRECTION('',(0.,1.,0.));
#105439=DIRECTION('center_axis',(0.,1.,0.));
#105440=DIRECTION('ref_axis',(1.,0.,0.));
#105441=DIRECTION('',(-0.190809912898503,0.,0.981627005099017));
#105442=DIRECTION('',(0.981627005099017,0.,0.190809912898503));
#105443=DIRECTION('',(-0.190809912898503,0.,0.981627005099017));
#105444=DIRECTION('',(0.981627005099017,0.,0.190809912898503));
#105445=DIRECTION('center_axis',(0.981627005099017,0.,0.190809912898503));
#105446=DIRECTION('ref_axis',(0.,-1.,0.));
#105447=DIRECTION('',(-0.190809912898503,0.,0.981627005099017));
#105448=DIRECTION('',(0.,-1.,0.));
#105449=DIRECTION('',(0.,-1.,0.));
#105450=DIRECTION('center_axis',(0.,-1.,0.));
#105451=DIRECTION('ref_axis',(0.,0.,-1.));
#105452=DIRECTION('',(-0.190809912898503,0.,0.981627005099017));
#105453=DIRECTION('',(-0.981627005099017,0.,-0.190809912898503));
#105454=DIRECTION('',(-0.981627005099017,0.,-0.190809912898503));
#105455=DIRECTION('center_axis',(-0.981627005099017,0.,-0.190809912898503));
#105456=DIRECTION('ref_axis',(-0.190809912898503,0.,0.981627005099017));
#105457=DIRECTION('',(0.,1.,0.));
#105458=DIRECTION('',(0.,1.,0.));
#105459=DIRECTION('center_axis',(0.,1.,0.));
#105460=DIRECTION('ref_axis',(1.,0.,0.));
#105461=DIRECTION('',(-0.190809912898503,0.,0.981627005099017));
#105462=DIRECTION('',(0.981627005099017,0.,0.190809912898503));
#105463=DIRECTION('',(-0.190809912898503,0.,0.981627005099017));
#105464=DIRECTION('',(0.981627005099017,0.,0.190809912898503));
#105465=DIRECTION('center_axis',(0.981627005099017,0.,0.190809912898503));
#105466=DIRECTION('ref_axis',(0.,-1.,0.));
#105467=DIRECTION('',(-0.190809912898503,0.,0.981627005099017));
#105468=DIRECTION('',(0.,-1.,0.));
#105469=DIRECTION('',(0.,-1.,0.));
#105470=DIRECTION('center_axis',(0.,-1.,0.));
#105471=DIRECTION('ref_axis',(0.,0.,-1.));
#105472=DIRECTION('',(-0.190809912898503,0.,0.981627005099017));
#105473=DIRECTION('',(-0.981627005099017,0.,-0.190809912898503));
#105474=DIRECTION('',(-0.981627005099017,0.,-0.190809912898503));
#105475=DIRECTION('center_axis',(-0.981627005099017,0.,-0.190809912898503));
#105476=DIRECTION('ref_axis',(-0.190809912898503,0.,0.981627005099017));
#105477=DIRECTION('',(0.,1.,0.));
#105478=DIRECTION('',(0.,1.,0.));
#105479=DIRECTION('center_axis',(0.,1.,0.));
#105480=DIRECTION('ref_axis',(1.,0.,0.));
#105481=DIRECTION('',(-0.190809912898503,0.,0.981627005099017));
#105482=DIRECTION('',(0.981627005099017,0.,0.190809912898503));
#105483=DIRECTION('',(-0.190809912898503,0.,0.981627005099017));
#105484=DIRECTION('',(0.981627005099017,0.,0.190809912898503));
#105485=DIRECTION('center_axis',(0.981627005099017,0.,0.190809912898503));
#105486=DIRECTION('ref_axis',(0.,-1.,0.));
#105487=DIRECTION('',(-0.190809912898503,0.,0.981627005099017));
#105488=DIRECTION('',(0.,-1.,0.));
#105489=DIRECTION('',(0.,-1.,0.));
#105490=DIRECTION('center_axis',(0.,-1.,0.));
#105491=DIRECTION('ref_axis',(0.,0.,-1.));
#105492=DIRECTION('',(-0.190809912898503,0.,0.981627005099017));
#105493=DIRECTION('',(-0.981627005099017,0.,-0.190809912898503));
#105494=DIRECTION('',(-0.981627005099017,0.,-0.190809912898503));
#105495=DIRECTION('center_axis',(-0.981627005099017,0.,-0.190809912898503));
#105496=DIRECTION('ref_axis',(-0.190809912898503,0.,0.981627005099017));
#105497=DIRECTION('',(0.,1.,0.));
#105498=DIRECTION('',(0.,1.,0.));
#105499=DIRECTION('center_axis',(0.,1.,0.));
#105500=DIRECTION('ref_axis',(1.,0.,0.));
#105501=DIRECTION('',(-0.190809912898503,0.,0.981627005099017));
#105502=DIRECTION('',(0.981627005099017,0.,0.190809912898503));
#105503=DIRECTION('',(-0.190809912898503,0.,0.981627005099017));
#105504=DIRECTION('',(0.981627005099017,0.,0.190809912898503));
#105505=DIRECTION('center_axis',(0.981627005099017,0.,0.190809912898503));
#105506=DIRECTION('ref_axis',(0.,-1.,0.));
#105507=DIRECTION('',(-0.190809912898503,0.,0.981627005099017));
#105508=DIRECTION('',(0.,-1.,0.));
#105509=DIRECTION('',(0.,-1.,0.));
#105510=DIRECTION('center_axis',(0.,-1.,0.));
#105511=DIRECTION('ref_axis',(0.,0.,-1.));
#105512=DIRECTION('',(-0.190809912898503,0.,0.981627005099017));
#105513=DIRECTION('',(-0.981627005099017,0.,-0.190809912898503));
#105514=DIRECTION('',(-0.981627005099017,0.,-0.190809912898503));
#105515=DIRECTION('center_axis',(-0.981627005099017,0.,-0.190809912898503));
#105516=DIRECTION('ref_axis',(-0.190809912898503,0.,0.981627005099017));
#105517=DIRECTION('',(0.,1.,0.));
#105518=DIRECTION('',(0.,1.,0.));
#105519=DIRECTION('center_axis',(0.,1.,0.));
#105520=DIRECTION('ref_axis',(1.,0.,0.));
#105521=DIRECTION('',(-0.190809912898503,0.,0.981627005099017));
#105522=DIRECTION('',(0.981627005099017,0.,0.190809912898503));
#105523=DIRECTION('',(-0.190809912898503,0.,0.981627005099017));
#105524=DIRECTION('',(0.981627005099017,0.,0.190809912898503));
#105525=DIRECTION('center_axis',(0.981627005099017,0.,0.190809912898503));
#105526=DIRECTION('ref_axis',(0.,-1.,0.));
#105527=DIRECTION('',(-0.190809912898503,0.,0.981627005099017));
#105528=DIRECTION('',(0.,-1.,0.));
#105529=DIRECTION('',(0.,-1.,0.));
#105530=DIRECTION('center_axis',(0.,-1.,0.));
#105531=DIRECTION('ref_axis',(0.,0.,-1.));
#105532=DIRECTION('',(-0.190809912898503,0.,0.981627005099017));
#105533=DIRECTION('',(-0.981627005099017,0.,-0.190809912898503));
#105534=DIRECTION('',(-0.981627005099017,0.,-0.190809912898503));
#105535=DIRECTION('center_axis',(-0.981627005099017,0.,-0.190809912898503));
#105536=DIRECTION('ref_axis',(-0.190809912898503,0.,0.981627005099017));
#105537=DIRECTION('',(0.,1.,0.));
#105538=DIRECTION('',(0.,1.,0.));
#105539=DIRECTION('center_axis',(0.,1.,0.));
#105540=DIRECTION('ref_axis',(1.,0.,0.));
#105541=DIRECTION('',(-0.190809912898503,0.,0.981627005099017));
#105542=DIRECTION('',(0.981627005099017,0.,0.190809912898503));
#105543=DIRECTION('',(-0.190809912898503,0.,0.981627005099017));
#105544=DIRECTION('',(0.981627005099017,0.,0.190809912898503));
#105545=DIRECTION('center_axis',(0.981627005099017,0.,0.190809912898503));
#105546=DIRECTION('ref_axis',(0.,-1.,0.));
#105547=DIRECTION('',(-0.190809912898503,0.,0.981627005099017));
#105548=DIRECTION('',(0.,-1.,0.));
#105549=DIRECTION('',(0.,-1.,0.));
#105550=DIRECTION('center_axis',(0.,-1.,0.));
#105551=DIRECTION('ref_axis',(0.,0.,-1.));
#105552=DIRECTION('',(-0.190809912898503,0.,0.981627005099017));
#105553=DIRECTION('',(-0.981627005099017,0.,-0.190809912898503));
#105554=DIRECTION('',(-0.981627005099017,0.,-0.190809912898503));
#105555=DIRECTION('center_axis',(-0.981627005099017,0.,-0.190809912898503));
#105556=DIRECTION('ref_axis',(-0.190809912898503,0.,0.981627005099017));
#105557=DIRECTION('',(0.,1.,0.));
#105558=DIRECTION('',(0.,1.,0.));
#105559=DIRECTION('center_axis',(0.,1.,0.));
#105560=DIRECTION('ref_axis',(1.,0.,0.));
#105561=DIRECTION('',(-0.190809912898503,0.,0.981627005099017));
#105562=DIRECTION('',(0.981627005099017,0.,0.190809912898503));
#105563=DIRECTION('',(-0.190809912898503,0.,0.981627005099017));
#105564=DIRECTION('',(0.981627005099017,0.,0.190809912898503));
#105565=DIRECTION('center_axis',(0.981627005099017,0.,0.190809912898503));
#105566=DIRECTION('ref_axis',(0.,-1.,0.));
#105567=DIRECTION('',(-0.190809912898503,0.,0.981627005099017));
#105568=DIRECTION('',(0.,-1.,0.));
#105569=DIRECTION('',(0.,-1.,0.));
#105570=DIRECTION('center_axis',(0.,-1.,0.));
#105571=DIRECTION('ref_axis',(0.,0.,-1.));
#105572=DIRECTION('',(-0.190809912898503,0.,0.981627005099017));
#105573=DIRECTION('',(-0.981627005099017,0.,-0.190809912898503));
#105574=DIRECTION('',(-0.981627005099017,0.,-0.190809912898503));
#105575=DIRECTION('center_axis',(-0.981627005099017,0.,-0.190809912898503));
#105576=DIRECTION('ref_axis',(-0.190809912898503,0.,0.981627005099017));
#105577=DIRECTION('',(0.,1.,0.));
#105578=DIRECTION('',(0.,1.,0.));
#105579=DIRECTION('center_axis',(0.,1.,0.));
#105580=DIRECTION('ref_axis',(1.,0.,0.));
#105581=DIRECTION('',(-0.190809912898503,0.,0.981627005099017));
#105582=DIRECTION('',(0.981627005099017,0.,0.190809912898503));
#105583=DIRECTION('',(-0.190809912898503,0.,0.981627005099017));
#105584=DIRECTION('',(0.981627005099017,0.,0.190809912898503));
#105585=DIRECTION('center_axis',(0.981627005099017,0.,0.190809912898503));
#105586=DIRECTION('ref_axis',(0.,-1.,0.));
#105587=DIRECTION('',(-0.190809912898503,0.,0.981627005099017));
#105588=DIRECTION('',(0.,-1.,0.));
#105589=DIRECTION('',(0.,-1.,0.));
#105590=DIRECTION('center_axis',(0.,-1.,0.));
#105591=DIRECTION('ref_axis',(0.,0.,-1.));
#105592=DIRECTION('',(-0.190809912898503,0.,0.981627005099017));
#105593=DIRECTION('',(-0.981627005099017,0.,-0.190809912898503));
#105594=DIRECTION('',(-0.981627005099017,0.,-0.190809912898503));
#105595=DIRECTION('center_axis',(-0.981627005099017,0.,-0.190809912898503));
#105596=DIRECTION('ref_axis',(-0.190809912898503,0.,0.981627005099017));
#105597=DIRECTION('',(0.,1.,0.));
#105598=DIRECTION('',(0.,1.,0.));
#105599=DIRECTION('center_axis',(0.,1.,0.));
#105600=DIRECTION('ref_axis',(1.,0.,0.));
#105601=DIRECTION('',(-0.190809912898503,0.,0.981627005099017));
#105602=DIRECTION('',(0.981627005099017,0.,0.190809912898503));
#105603=DIRECTION('',(-0.190809912898503,0.,0.981627005099017));
#105604=DIRECTION('',(0.981627005099017,0.,0.190809912898503));
#105605=DIRECTION('center_axis',(0.981627005099017,0.,0.190809912898503));
#105606=DIRECTION('ref_axis',(0.,-1.,0.));
#105607=DIRECTION('',(-0.190809912898503,0.,0.981627005099017));
#105608=DIRECTION('',(0.,-1.,0.));
#105609=DIRECTION('',(0.,-1.,0.));
#105610=DIRECTION('center_axis',(0.,-1.,0.));
#105611=DIRECTION('ref_axis',(0.,0.,-1.));
#105612=DIRECTION('',(-0.190809912898503,0.,0.981627005099017));
#105613=DIRECTION('',(-0.981627005099017,0.,-0.190809912898503));
#105614=DIRECTION('',(-0.981627005099017,0.,-0.190809912898503));
#105615=DIRECTION('center_axis',(-0.981627005099017,0.,-0.190809912898503));
#105616=DIRECTION('ref_axis',(-0.190809912898503,0.,0.981627005099017));
#105617=DIRECTION('',(0.,1.,0.));
#105618=DIRECTION('',(0.,1.,0.));
#105619=DIRECTION('center_axis',(0.,1.,0.));
#105620=DIRECTION('ref_axis',(1.,0.,0.));
#105621=DIRECTION('',(-0.190809912898503,0.,0.981627005099017));
#105622=DIRECTION('',(0.981627005099017,0.,0.190809912898503));
#105623=DIRECTION('',(-0.190809912898503,0.,0.981627005099017));
#105624=DIRECTION('',(0.981627005099017,0.,0.190809912898503));
#105625=DIRECTION('center_axis',(0.981627005099017,0.,0.190809912898503));
#105626=DIRECTION('ref_axis',(0.,-1.,0.));
#105627=DIRECTION('',(-0.190809912898503,0.,0.981627005099017));
#105628=DIRECTION('',(0.,-1.,0.));
#105629=DIRECTION('',(0.,-1.,0.));
#105630=DIRECTION('center_axis',(0.,-1.,0.));
#105631=DIRECTION('ref_axis',(0.,0.,-1.));
#105632=DIRECTION('',(-0.190809912898503,0.,0.981627005099017));
#105633=DIRECTION('',(-0.981627005099017,0.,-0.190809912898503));
#105634=DIRECTION('',(-0.981627005099017,0.,-0.190809912898503));
#105635=DIRECTION('center_axis',(-0.981627005099017,0.,-0.190809912898503));
#105636=DIRECTION('ref_axis',(-0.190809912898503,0.,0.981627005099017));
#105637=DIRECTION('',(0.,1.,0.));
#105638=DIRECTION('',(0.,1.,0.));
#105639=DIRECTION('center_axis',(0.,1.,0.));
#105640=DIRECTION('ref_axis',(1.,0.,0.));
#105641=DIRECTION('',(-0.190809912898503,0.,0.981627005099017));
#105642=DIRECTION('',(0.981627005099017,0.,0.190809912898503));
#105643=DIRECTION('',(-0.190809912898503,0.,0.981627005099017));
#105644=DIRECTION('',(0.981627005099017,0.,0.190809912898503));
#105645=DIRECTION('center_axis',(0.981627005099017,0.,0.190809912898503));
#105646=DIRECTION('ref_axis',(0.,-1.,0.));
#105647=DIRECTION('',(-0.190809912898503,0.,0.981627005099017));
#105648=DIRECTION('',(0.,-1.,0.));
#105649=DIRECTION('',(0.,-1.,0.));
#105650=DIRECTION('center_axis',(0.,-1.,0.));
#105651=DIRECTION('ref_axis',(0.,0.,-1.));
#105652=DIRECTION('',(-0.190809912898503,0.,0.981627005099017));
#105653=DIRECTION('',(-0.981627005099017,0.,-0.190809912898503));
#105654=DIRECTION('',(-0.981627005099017,0.,-0.190809912898503));
#105655=DIRECTION('center_axis',(-0.981627005099017,0.,-0.190809912898503));
#105656=DIRECTION('ref_axis',(-0.190809912898503,0.,0.981627005099017));
#105657=DIRECTION('',(0.,1.,0.));
#105658=DIRECTION('',(0.,1.,0.));
#105659=DIRECTION('center_axis',(0.,1.,0.));
#105660=DIRECTION('ref_axis',(1.,0.,0.));
#105661=DIRECTION('',(-0.190809912898503,0.,0.981627005099017));
#105662=DIRECTION('',(0.981627005099017,0.,0.190809912898503));
#105663=DIRECTION('',(-0.190809912898503,0.,0.981627005099017));
#105664=DIRECTION('',(0.981627005099017,0.,0.190809912898503));
#105665=DIRECTION('center_axis',(0.981627005099017,0.,0.190809912898503));
#105666=DIRECTION('ref_axis',(0.,-1.,0.));
#105667=DIRECTION('',(-0.190809912898503,0.,0.981627005099017));
#105668=DIRECTION('',(0.,-1.,0.));
#105669=DIRECTION('',(0.,-1.,0.));
#105670=DIRECTION('center_axis',(0.,-1.,0.));
#105671=DIRECTION('ref_axis',(0.,0.,-1.));
#105672=DIRECTION('',(-0.190809912898503,0.,0.981627005099017));
#105673=DIRECTION('',(-0.981627005099017,0.,-0.190809912898503));
#105674=DIRECTION('',(-0.981627005099017,0.,-0.190809912898503));
#105675=DIRECTION('center_axis',(-0.981627005099017,0.,-0.190809912898503));
#105676=DIRECTION('ref_axis',(-0.190809912898503,0.,0.981627005099017));
#105677=DIRECTION('',(0.,1.,0.));
#105678=DIRECTION('',(0.,1.,0.));
#105679=DIRECTION('center_axis',(0.,1.,0.));
#105680=DIRECTION('ref_axis',(1.,0.,0.));
#105681=DIRECTION('',(-0.190809912898503,0.,0.981627005099017));
#105682=DIRECTION('',(0.981627005099017,0.,0.190809912898503));
#105683=DIRECTION('',(-0.190809912898503,0.,0.981627005099017));
#105684=DIRECTION('',(0.981627005099017,0.,0.190809912898503));
#105685=DIRECTION('center_axis',(0.981627005099017,0.,0.190809912898503));
#105686=DIRECTION('ref_axis',(0.,-1.,0.));
#105687=DIRECTION('',(-0.190809912898503,0.,0.981627005099017));
#105688=DIRECTION('',(0.,-1.,0.));
#105689=DIRECTION('',(0.,-1.,0.));
#105690=DIRECTION('center_axis',(0.,-1.,0.));
#105691=DIRECTION('ref_axis',(0.,0.,-1.));
#105692=DIRECTION('',(-0.190809912898503,0.,0.981627005099017));
#105693=DIRECTION('',(-0.981627005099017,0.,-0.190809912898503));
#105694=DIRECTION('',(-0.981627005099017,0.,-0.190809912898503));
#105695=DIRECTION('center_axis',(-0.981627005099017,0.,-0.190809912898503));
#105696=DIRECTION('ref_axis',(-0.190809912898503,0.,0.981627005099017));
#105697=DIRECTION('',(0.,1.,0.));
#105698=DIRECTION('',(0.,1.,0.));
#105699=DIRECTION('center_axis',(0.,1.,0.));
#105700=DIRECTION('ref_axis',(1.,0.,0.));
#105701=DIRECTION('',(-0.190809912898503,0.,0.981627005099017));
#105702=DIRECTION('',(0.981627005099017,0.,0.190809912898503));
#105703=DIRECTION('',(-0.190809912898503,0.,0.981627005099017));
#105704=DIRECTION('',(0.981627005099017,0.,0.190809912898503));
#105705=DIRECTION('center_axis',(0.981627005099017,0.,0.190809912898503));
#105706=DIRECTION('ref_axis',(0.,-1.,0.));
#105707=DIRECTION('',(-0.190809912898503,0.,0.981627005099017));
#105708=DIRECTION('',(0.,-1.,0.));
#105709=DIRECTION('',(0.,-1.,0.));
#105710=DIRECTION('center_axis',(0.,-1.,0.));
#105711=DIRECTION('ref_axis',(0.,0.,-1.));
#105712=DIRECTION('',(-0.190809912898503,0.,0.981627005099017));
#105713=DIRECTION('',(-0.981627005099017,0.,-0.190809912898503));
#105714=DIRECTION('',(-0.981627005099017,0.,-0.190809912898503));
#105715=DIRECTION('center_axis',(-0.981627005099017,0.,-0.190809912898503));
#105716=DIRECTION('ref_axis',(-0.190809912898503,0.,0.981627005099017));
#105717=DIRECTION('',(0.,1.,0.));
#105718=DIRECTION('',(0.,1.,0.));
#105719=DIRECTION('center_axis',(0.,1.,0.));
#105720=DIRECTION('ref_axis',(1.,0.,0.));
#105721=DIRECTION('',(-0.190809912898503,0.,0.981627005099017));
#105722=DIRECTION('',(0.981627005099017,0.,0.190809912898503));
#105723=DIRECTION('',(-0.190809912898503,0.,0.981627005099017));
#105724=DIRECTION('',(0.981627005099017,0.,0.190809912898503));
#105725=DIRECTION('center_axis',(0.981627005099017,0.,0.190809912898503));
#105726=DIRECTION('ref_axis',(0.,-1.,0.));
#105727=DIRECTION('',(-0.190809912898503,0.,0.981627005099017));
#105728=DIRECTION('',(0.,-1.,0.));
#105729=DIRECTION('',(0.,-1.,0.));
#105730=DIRECTION('center_axis',(0.,-1.,0.));
#105731=DIRECTION('ref_axis',(0.,0.,-1.));
#105732=DIRECTION('',(-0.190809912898503,0.,0.981627005099017));
#105733=DIRECTION('',(-0.981627005099017,0.,-0.190809912898503));
#105734=DIRECTION('',(-0.981627005099017,0.,-0.190809912898503));
#105735=DIRECTION('center_axis',(-0.981627005099017,0.,-0.190809912898503));
#105736=DIRECTION('ref_axis',(-0.190809912898503,0.,0.981627005099017));
#105737=DIRECTION('',(0.,1.,0.));
#105738=DIRECTION('',(0.,1.,0.));
#105739=DIRECTION('center_axis',(0.,1.,0.));
#105740=DIRECTION('ref_axis',(1.,0.,0.));
#105741=DIRECTION('',(-0.190809912898503,0.,0.981627005099017));
#105742=DIRECTION('',(0.981627005099017,0.,0.190809912898503));
#105743=DIRECTION('',(-0.190809912898503,0.,0.981627005099017));
#105744=DIRECTION('',(0.981627005099017,0.,0.190809912898503));
#105745=DIRECTION('center_axis',(0.981627005099017,0.,0.190809912898503));
#105746=DIRECTION('ref_axis',(0.,-1.,0.));
#105747=DIRECTION('',(-0.190809912898503,0.,0.981627005099017));
#105748=DIRECTION('',(0.,-1.,0.));
#105749=DIRECTION('',(0.,-1.,0.));
#105750=DIRECTION('center_axis',(0.,-1.,0.));
#105751=DIRECTION('ref_axis',(0.,0.,-1.));
#105752=DIRECTION('',(-0.190809912898503,0.,0.981627005099017));
#105753=DIRECTION('',(-0.981627005099017,0.,-0.190809912898503));
#105754=DIRECTION('',(-0.981627005099017,0.,-0.190809912898503));
#105755=DIRECTION('center_axis',(-0.981627005099017,0.,-0.190809912898503));
#105756=DIRECTION('ref_axis',(-0.190809912898503,0.,0.981627005099017));
#105757=DIRECTION('',(0.,1.,0.));
#105758=DIRECTION('',(0.,1.,0.));
#105759=DIRECTION('center_axis',(0.,1.,0.));
#105760=DIRECTION('ref_axis',(1.,0.,0.));
#105761=DIRECTION('',(-0.190809912898503,0.,0.981627005099017));
#105762=DIRECTION('',(0.981627005099017,0.,0.190809912898503));
#105763=DIRECTION('',(-0.190809912898503,0.,0.981627005099017));
#105764=DIRECTION('',(0.981627005099017,0.,0.190809912898503));
#105765=DIRECTION('center_axis',(0.981627005099017,0.,0.190809912898503));
#105766=DIRECTION('ref_axis',(0.,-1.,0.));
#105767=DIRECTION('',(-0.190809912898503,0.,0.981627005099017));
#105768=DIRECTION('',(0.,-1.,0.));
#105769=DIRECTION('',(0.,-1.,0.));
#105770=DIRECTION('center_axis',(0.,-1.,0.));
#105771=DIRECTION('ref_axis',(0.,0.,-1.));
#105772=DIRECTION('',(-0.190809912898503,0.,0.981627005099017));
#105773=DIRECTION('',(-0.981627005099017,0.,-0.190809912898503));
#105774=DIRECTION('',(-0.981627005099017,0.,-0.190809912898503));
#105775=DIRECTION('center_axis',(-0.981627005099017,0.,-0.190809912898503));
#105776=DIRECTION('ref_axis',(-0.190809912898503,0.,0.981627005099017));
#105777=DIRECTION('',(0.,1.,0.));
#105778=DIRECTION('',(0.,1.,0.));
#105779=DIRECTION('center_axis',(0.,1.,0.));
#105780=DIRECTION('ref_axis',(1.,0.,0.));
#105781=DIRECTION('',(-0.190809912898503,0.,0.981627005099017));
#105782=DIRECTION('',(0.981627005099017,0.,0.190809912898503));
#105783=DIRECTION('',(-0.190809912898503,0.,0.981627005099017));
#105784=DIRECTION('',(0.981627005099017,0.,0.190809912898503));
#105785=DIRECTION('center_axis',(0.981627005099017,0.,0.190809912898503));
#105786=DIRECTION('ref_axis',(0.,-1.,0.));
#105787=DIRECTION('',(-0.190809912898503,0.,0.981627005099017));
#105788=DIRECTION('',(0.,-1.,0.));
#105789=DIRECTION('',(0.,-1.,0.));
#105790=DIRECTION('center_axis',(0.,-1.,0.));
#105791=DIRECTION('ref_axis',(0.,0.,-1.));
#105792=DIRECTION('',(-0.190809912898503,0.,0.981627005099017));
#105793=DIRECTION('',(-0.981627005099017,0.,-0.190809912898503));
#105794=DIRECTION('',(-0.981627005099017,0.,-0.190809912898503));
#105795=DIRECTION('center_axis',(-0.981627005099017,0.,-0.190809912898503));
#105796=DIRECTION('ref_axis',(-0.190809912898503,0.,0.981627005099017));
#105797=DIRECTION('',(0.,1.,0.));
#105798=DIRECTION('',(0.,1.,0.));
#105799=DIRECTION('center_axis',(0.,1.,0.));
#105800=DIRECTION('ref_axis',(1.,0.,0.));
#105801=DIRECTION('',(-0.190809912898503,0.,0.981627005099017));
#105802=DIRECTION('',(0.981627005099017,0.,0.190809912898503));
#105803=DIRECTION('',(-0.190809912898503,0.,0.981627005099017));
#105804=DIRECTION('',(0.981627005099017,0.,0.190809912898503));
#105805=DIRECTION('center_axis',(0.981627005099017,0.,0.190809912898503));
#105806=DIRECTION('ref_axis',(0.,-1.,0.));
#105807=DIRECTION('',(-0.190809912898503,0.,0.981627005099017));
#105808=DIRECTION('',(0.,-1.,0.));
#105809=DIRECTION('',(0.,-1.,0.));
#105810=DIRECTION('center_axis',(0.,-1.,0.));
#105811=DIRECTION('ref_axis',(0.,0.,-1.));
#105812=DIRECTION('',(-0.190809912898503,0.,0.981627005099017));
#105813=DIRECTION('',(-0.981627005099017,0.,-0.190809912898503));
#105814=DIRECTION('',(-0.981627005099017,0.,-0.190809912898503));
#105815=DIRECTION('center_axis',(-0.981627005099017,0.,-0.190809912898503));
#105816=DIRECTION('ref_axis',(-0.190809912898503,0.,0.981627005099017));
#105817=DIRECTION('',(0.,1.,0.));
#105818=DIRECTION('',(0.,1.,0.));
#105819=DIRECTION('center_axis',(0.,1.,0.));
#105820=DIRECTION('ref_axis',(1.,0.,0.));
#105821=DIRECTION('',(-0.190809912898503,0.,0.981627005099017));
#105822=DIRECTION('',(0.981627005099017,0.,0.190809912898503));
#105823=DIRECTION('',(-0.190809912898503,0.,0.981627005099017));
#105824=DIRECTION('',(0.981627005099017,0.,0.190809912898503));
#105825=DIRECTION('center_axis',(0.981627005099017,0.,0.190809912898503));
#105826=DIRECTION('ref_axis',(0.,-1.,0.));
#105827=DIRECTION('',(-0.190809912898503,0.,0.981627005099017));
#105828=DIRECTION('',(0.,-1.,0.));
#105829=DIRECTION('',(0.,-1.,0.));
#105830=DIRECTION('center_axis',(0.,-1.,0.));
#105831=DIRECTION('ref_axis',(0.,0.,-1.));
#105832=DIRECTION('',(-0.190809912898503,0.,0.981627005099017));
#105833=DIRECTION('',(-0.981627005099017,0.,-0.190809912898503));
#105834=DIRECTION('',(-0.981627005099017,0.,-0.190809912898503));
#105835=DIRECTION('center_axis',(-0.981627005099017,0.,-0.190809912898503));
#105836=DIRECTION('ref_axis',(-0.190809912898503,0.,0.981627005099017));
#105837=DIRECTION('',(0.,1.,0.));
#105838=DIRECTION('',(0.,1.,0.));
#105839=DIRECTION('center_axis',(0.,1.,0.));
#105840=DIRECTION('ref_axis',(1.,0.,0.));
#105841=DIRECTION('',(-0.190809912898503,0.,0.981627005099017));
#105842=DIRECTION('',(0.981627005099017,0.,0.190809912898503));
#105843=DIRECTION('',(-0.190809912898503,0.,0.981627005099017));
#105844=DIRECTION('',(0.981627005099017,0.,0.190809912898503));
#105845=DIRECTION('center_axis',(0.981627005099017,0.,0.190809912898503));
#105846=DIRECTION('ref_axis',(0.,-1.,0.));
#105847=DIRECTION('',(-0.190809912898503,0.,0.981627005099017));
#105848=DIRECTION('',(0.,-1.,0.));
#105849=DIRECTION('',(0.,-1.,0.));
#105850=DIRECTION('center_axis',(0.,-1.,0.));
#105851=DIRECTION('ref_axis',(0.,0.,-1.));
#105852=DIRECTION('',(-0.190809912898503,0.,0.981627005099017));
#105853=DIRECTION('',(-0.981627005099017,0.,-0.190809912898503));
#105854=DIRECTION('',(-0.981627005099017,0.,-0.190809912898503));
#105855=DIRECTION('center_axis',(-0.981627005099017,0.,-0.190809912898503));
#105856=DIRECTION('ref_axis',(-0.190809912898503,0.,0.981627005099017));
#105857=DIRECTION('',(0.,1.,0.));
#105858=DIRECTION('',(0.,1.,0.));
#105859=DIRECTION('center_axis',(0.,1.,0.));
#105860=DIRECTION('ref_axis',(1.,0.,0.));
#105861=DIRECTION('',(-0.190809912898503,0.,0.981627005099017));
#105862=DIRECTION('',(0.981627005099017,0.,0.190809912898503));
#105863=DIRECTION('',(-0.190809912898503,0.,0.981627005099017));
#105864=DIRECTION('',(0.981627005099017,0.,0.190809912898503));
#105865=DIRECTION('center_axis',(0.981627005099017,0.,0.190809912898503));
#105866=DIRECTION('ref_axis',(0.,-1.,0.));
#105867=DIRECTION('',(-0.190809912898503,0.,0.981627005099017));
#105868=DIRECTION('',(0.,-1.,0.));
#105869=DIRECTION('',(0.,-1.,0.));
#105870=DIRECTION('center_axis',(0.,-1.,0.));
#105871=DIRECTION('ref_axis',(0.,0.,-1.));
#105872=DIRECTION('',(-0.190809912898503,0.,0.981627005099017));
#105873=DIRECTION('',(-0.981627005099017,0.,-0.190809912898503));
#105874=DIRECTION('',(-0.981627005099017,0.,-0.190809912898503));
#105875=DIRECTION('center_axis',(-0.981627005099017,0.,-0.190809912898503));
#105876=DIRECTION('ref_axis',(-0.190809912898503,0.,0.981627005099017));
#105877=DIRECTION('',(0.,1.,0.));
#105878=DIRECTION('',(0.,1.,0.));
#105879=DIRECTION('center_axis',(0.,1.,0.));
#105880=DIRECTION('ref_axis',(1.,0.,0.));
#105881=DIRECTION('',(-0.190809912898503,0.,0.981627005099017));
#105882=DIRECTION('',(0.981627005099017,0.,0.190809912898503));
#105883=DIRECTION('',(-0.190809912898503,0.,0.981627005099017));
#105884=DIRECTION('',(0.981627005099017,0.,0.190809912898503));
#105885=DIRECTION('center_axis',(0.981627005099017,0.,0.190809912898503));
#105886=DIRECTION('ref_axis',(0.,-1.,0.));
#105887=DIRECTION('',(-0.190809912898503,0.,0.981627005099017));
#105888=DIRECTION('',(0.,-1.,0.));
#105889=DIRECTION('',(0.,-1.,0.));
#105890=DIRECTION('center_axis',(0.,-1.,0.));
#105891=DIRECTION('ref_axis',(0.,0.,-1.));
#105892=DIRECTION('',(-0.190809912898503,0.,0.981627005099017));
#105893=DIRECTION('',(-0.981627005099017,0.,-0.190809912898503));
#105894=DIRECTION('',(-0.981627005099017,0.,-0.190809912898503));
#105895=DIRECTION('center_axis',(-0.981627005099017,0.,-0.190809912898503));
#105896=DIRECTION('ref_axis',(-0.190809912898503,0.,0.981627005099017));
#105897=DIRECTION('',(0.,1.,0.));
#105898=DIRECTION('',(0.,1.,0.));
#105899=DIRECTION('center_axis',(0.,1.,0.));
#105900=DIRECTION('ref_axis',(1.,0.,0.));
#105901=DIRECTION('',(-0.190809912898503,0.,0.981627005099017));
#105902=DIRECTION('',(0.981627005099017,0.,0.190809912898503));
#105903=DIRECTION('',(-0.190809912898503,0.,0.981627005099017));
#105904=DIRECTION('',(0.981627005099017,0.,0.190809912898503));
#105905=DIRECTION('center_axis',(0.981627005099017,0.,0.190809912898503));
#105906=DIRECTION('ref_axis',(0.,-1.,0.));
#105907=DIRECTION('',(-0.190809912898503,0.,0.981627005099017));
#105908=DIRECTION('',(0.,-1.,0.));
#105909=DIRECTION('',(0.,-1.,0.));
#105910=DIRECTION('center_axis',(0.,-1.,0.));
#105911=DIRECTION('ref_axis',(0.,0.,-1.));
#105912=DIRECTION('',(-0.190809912898503,0.,0.981627005099017));
#105913=DIRECTION('',(-0.981627005099017,0.,-0.190809912898503));
#105914=DIRECTION('',(-0.981627005099017,0.,-0.190809912898503));
#105915=DIRECTION('center_axis',(-0.981627005099017,0.,-0.190809912898503));
#105916=DIRECTION('ref_axis',(-0.190809912898503,0.,0.981627005099017));
#105917=DIRECTION('',(0.,1.,0.));
#105918=DIRECTION('',(0.,1.,0.));
#105919=DIRECTION('center_axis',(0.,1.,0.));
#105920=DIRECTION('ref_axis',(1.,0.,0.));
#105921=DIRECTION('',(-0.190809912898503,0.,0.981627005099017));
#105922=DIRECTION('',(0.981627005099017,0.,0.190809912898503));
#105923=DIRECTION('',(-0.190809912898503,0.,0.981627005099017));
#105924=DIRECTION('',(0.981627005099017,0.,0.190809912898503));
#105925=DIRECTION('center_axis',(0.981627005099017,0.,0.190809912898503));
#105926=DIRECTION('ref_axis',(0.,-1.,0.));
#105927=DIRECTION('',(-0.190809912898503,0.,0.981627005099017));
#105928=DIRECTION('',(0.,-1.,0.));
#105929=DIRECTION('',(0.,-1.,0.));
#105930=DIRECTION('center_axis',(0.,-1.,0.));
#105931=DIRECTION('ref_axis',(0.,0.,-1.));
#105932=DIRECTION('',(-0.190809912898503,0.,0.981627005099017));
#105933=DIRECTION('',(-0.981627005099017,0.,-0.190809912898503));
#105934=DIRECTION('',(-0.981627005099017,0.,-0.190809912898503));
#105935=DIRECTION('center_axis',(-0.981627005099017,0.,-0.190809912898503));
#105936=DIRECTION('ref_axis',(-0.190809912898503,0.,0.981627005099017));
#105937=DIRECTION('',(0.,1.,0.));
#105938=DIRECTION('',(0.,1.,0.));
#105939=DIRECTION('center_axis',(0.,1.,0.));
#105940=DIRECTION('ref_axis',(1.,0.,0.));
#105941=DIRECTION('',(-0.190809912898503,0.,0.981627005099017));
#105942=DIRECTION('',(0.981627005099017,0.,0.190809912898503));
#105943=DIRECTION('',(-0.190809912898503,0.,0.981627005099017));
#105944=DIRECTION('',(0.981627005099017,0.,0.190809912898503));
#105945=DIRECTION('center_axis',(0.981627005099017,0.,0.190809912898503));
#105946=DIRECTION('ref_axis',(0.,-1.,0.));
#105947=DIRECTION('',(-0.190809912898503,0.,0.981627005099017));
#105948=DIRECTION('',(0.,-1.,0.));
#105949=DIRECTION('',(0.,-1.,0.));
#105950=DIRECTION('center_axis',(0.,-1.,0.));
#105951=DIRECTION('ref_axis',(0.,0.,-1.));
#105952=DIRECTION('',(-0.190809912898503,0.,0.981627005099017));
#105953=DIRECTION('',(-0.981627005099017,0.,-0.190809912898503));
#105954=DIRECTION('',(-0.981627005099017,0.,-0.190809912898503));
#105955=DIRECTION('center_axis',(-0.981627005099017,0.,-0.190809912898503));
#105956=DIRECTION('ref_axis',(-0.190809912898503,0.,0.981627005099017));
#105957=DIRECTION('',(0.,1.,0.));
#105958=DIRECTION('',(0.,1.,0.));
#105959=DIRECTION('center_axis',(0.,1.,0.));
#105960=DIRECTION('ref_axis',(1.,0.,0.));
#105961=DIRECTION('',(-0.190809912898503,0.,0.981627005099017));
#105962=DIRECTION('',(0.981627005099017,0.,0.190809912898503));
#105963=DIRECTION('',(-0.190809912898503,0.,0.981627005099017));
#105964=DIRECTION('',(0.981627005099017,0.,0.190809912898503));
#105965=DIRECTION('center_axis',(0.981627005099017,0.,0.190809912898503));
#105966=DIRECTION('ref_axis',(0.,-1.,0.));
#105967=DIRECTION('',(-0.190809912898503,0.,0.981627005099017));
#105968=DIRECTION('',(0.,-1.,0.));
#105969=DIRECTION('',(0.,-1.,0.));
#105970=DIRECTION('center_axis',(0.,-1.,0.));
#105971=DIRECTION('ref_axis',(0.,0.,-1.));
#105972=DIRECTION('',(-0.190809912898503,0.,0.981627005099017));
#105973=DIRECTION('',(-0.981627005099017,0.,-0.190809912898503));
#105974=DIRECTION('',(-0.981627005099017,0.,-0.190809912898503));
#105975=DIRECTION('center_axis',(-0.981627005099017,0.,-0.190809912898503));
#105976=DIRECTION('ref_axis',(-0.190809912898503,0.,0.981627005099017));
#105977=DIRECTION('',(0.,1.,0.));
#105978=DIRECTION('',(0.,1.,0.));
#105979=DIRECTION('center_axis',(0.190809912898503,0.,-0.981627005099017));
#105980=DIRECTION('ref_axis',(0.,-1.,0.));
#105981=DIRECTION('center_axis',(0.190809912898503,0.,-0.981627005099017));
#105982=DIRECTION('ref_axis',(0.,-1.,0.));
#105983=DIRECTION('',(0.981627005099017,0.,0.190809912898503));
#105984=DIRECTION('',(0.,-1.,0.));
#105985=DIRECTION('',(-0.981627005099017,0.,-0.190809912898503));
#105986=DIRECTION('',(0.,1.,0.));
#105987=DIRECTION('center_axis',(0.,1.,0.));
#105988=DIRECTION('ref_axis',(1.,0.,0.));
#105989=DIRECTION('',(-0.190809912898503,0.,0.981627005099017));
#105990=DIRECTION('',(-0.190809912898503,0.,0.981627005099017));
#105991=DIRECTION('',(0.981627005099017,0.,0.190809912898503));
#105992=DIRECTION('center_axis',(0.981627005099017,0.,0.190809912898503));
#105993=DIRECTION('ref_axis',(0.,-1.,0.));
#105994=DIRECTION('',(-0.190809912898503,0.,0.981627005099017));
#105995=DIRECTION('',(0.,-1.,0.));
#105996=DIRECTION('center_axis',(0.,-1.,0.));
#105997=DIRECTION('ref_axis',(0.,0.,-1.));
#105998=DIRECTION('',(-0.190809912898503,0.,0.981627005099017));
#105999=DIRECTION('',(-0.981627005099017,0.,-0.190809912898503));
#106000=DIRECTION('center_axis',(-0.981627005099017,0.,-0.190809912898503));
#106001=DIRECTION('ref_axis',(-0.190809912898503,0.,0.981627005099017));
#106002=DIRECTION('',(0.,1.,0.));
#106003=DIRECTION('center_axis',(0.190809912898503,0.,-0.981627005099017));
#106004=DIRECTION('ref_axis',(0.,-1.,0.));
#106005=DIRECTION('center_axis',(0.190809912898503,0.,-0.981627005099017));
#106006=DIRECTION('ref_axis',(0.,-1.,0.));
#106007=DIRECTION('center_axis',(0.190809912898503,0.,-0.981627005099017));
#106008=DIRECTION('ref_axis',(0.,-1.,0.));
#106009=DIRECTION('',(-0.981627005099017,0.,-0.190809912898503));
#106010=DIRECTION('center_axis',(0.190809912898503,0.,-0.981627005099017));
#106011=DIRECTION('ref_axis',(0.,-1.,0.));
#106012=DIRECTION('',(-0.981627005099017,-1.340542928837E-14,-0.190809912898503));
#106013=DIRECTION('center_axis',(-0.190809912898503,0.,0.981627005099017));
#106014=DIRECTION('ref_axis',(0.,1.,0.));
#106015=DIRECTION('',(-0.981627005099017,0.,-0.190809912898503));
#106016=DIRECTION('center_axis',(-0.190809912898503,0.,0.981627005099017));
#106017=DIRECTION('ref_axis',(0.,1.,0.));
#106018=DIRECTION('',(-0.981627005099017,1.608651514604E-14,-0.190809912898503));
#106019=DIRECTION('center_axis',(-0.981627005099017,0.,-0.190809912898503));
#106020=DIRECTION('ref_axis',(-1.19712313814501E-14,1.,6.15863391467038E-14));
#106021=DIRECTION('center_axis',(-0.981627005099017,0.,-0.190809912898503));
#106022=DIRECTION('ref_axis',(4.2134636976251E-15,1.,-2.16762834161202E-14));
#106023=DIRECTION('center_axis',(-0.190809912898503,0.,0.981627005099017));
#106024=DIRECTION('ref_axis',(0.,1.,0.));
#106025=DIRECTION('',(0.,-1.,0.));
#106026=DIRECTION('center_axis',(-0.190809912898503,0.,0.981627005099017));
#106027=DIRECTION('ref_axis',(0.,1.,0.));
#106028=DIRECTION('',(0.,-1.,0.));
#106029=DIRECTION('center_axis',(0.190809912898503,0.,-0.981627005099017));
#106030=DIRECTION('ref_axis',(0.,-1.,0.));
#106031=DIRECTION('',(0.,-1.,0.));
#106032=DIRECTION('center_axis',(0.190809912898503,0.,-0.981627005099017));
#106033=DIRECTION('ref_axis',(0.,-1.,0.));
#106034=DIRECTION('',(0.,-1.,0.));
#106035=DIRECTION('center_axis',(0.,-1.,0.));
#106036=DIRECTION('ref_axis',(-0.981627005099094,0.,-0.190809912898106));
#106037=DIRECTION('center_axis',(0.,-1.,0.));
#106038=DIRECTION('ref_axis',(-0.981627005099092,0.,-0.190809912898117));
#106039=DIRECTION('center_axis',(0.190809912898503,0.,-0.981627005099017));
#106040=DIRECTION('ref_axis',(0.,-1.,0.));
#106041=DIRECTION('center_axis',(-0.190809912898503,0.,0.981627005099017));
#106042=DIRECTION('ref_axis',(0.981627005099017,0.,0.190809912898503));
#106043=DIRECTION('center_axis',(1.,-6.12323399573677E-17,0.));
#106044=DIRECTION('ref_axis',(0.,-1.,0.));
#106045=DIRECTION('center_axis',(0.,-1.,0.));
#106046=DIRECTION('ref_axis',(-0.146165436076237,0.,0.989260160572861));
#106047=DIRECTION('center_axis',(0.981627005099017,2.42026211186394E-17,
0.190809912898504));
#106048=DIRECTION('ref_axis',(-0.190613830300973,0.0453233971548897,0.980618252618384));
#106049=DIRECTION('center_axis',(0.,1.,0.));
#106050=DIRECTION('ref_axis',(-0.17808229353532,0.,0.98401559780788));
#106051=DIRECTION('center_axis',(-0.981627005099017,-1.25430828081473E-17,
-0.190809912898504));
#106052=DIRECTION('ref_axis',(-0.190793943836834,0.0129373445166805,0.981544851808639));
#106053=DIRECTION('center_axis',(0.,-1.,0.));
#106054=DIRECTION('ref_axis',(0.,0.,-1.));
#106055=DIRECTION('',(-0.190809912898503,0.,0.981627005099017));
#106056=DIRECTION('',(-0.190809912898503,0.,0.981627005099017));
#106057=DIRECTION('center_axis',(0.,-1.,0.));
#106058=DIRECTION('ref_axis',(-0.147019041943122,0.,0.989133662002323));
#106059=DIRECTION('center_axis',(0.981627005099017,0.,0.190809912898503));
#106060=DIRECTION('ref_axis',(0.,-1.,0.));
#106061=DIRECTION('',(-0.190809912898503,0.,0.981627005099017));
#106062=DIRECTION('center_axis',(0.981627005099017,1.7913993378229E-18,
0.190809912898503));
#106063=DIRECTION('ref_axis',(-0.190621242411065,0.0444589430893387,0.980656384428838));
#106064=DIRECTION('center_axis',(0.,1.,0.));
#106065=DIRECTION('ref_axis',(1.,0.,0.));
#106066=DIRECTION('',(-0.190809912898503,0.,0.981627005099017));
#106067=DIRECTION('center_axis',(0.,1.,0.));
#106068=DIRECTION('ref_axis',(-0.178325347032483,0.,0.98397158018194));
#106069=DIRECTION('center_axis',(-0.981627005099017,0.,-0.190809912898503));
#106070=DIRECTION('ref_axis',(-0.190809912898503,0.,0.981627005099017));
#106071=DIRECTION('center_axis',(-0.981627005099017,8.94076702692101E-19,
-0.190809912898503));
#106072=DIRECTION('ref_axis',(-0.190794546115091,0.0126910417304199,0.981547950246208));
#106073=DIRECTION('center_axis',(1.,-6.12323399573677E-17,0.));
#106074=DIRECTION('ref_axis',(0.,-1.,0.));
#106075=DIRECTION('center_axis',(-0.190809912898504,0.,0.981627005099017));
#106076=DIRECTION('ref_axis',(0.981627005099017,0.,0.190809912898504));
#106077=DIRECTION('center_axis',(0.190809912898503,0.,-0.981627005099017));
#106078=DIRECTION('ref_axis',(0.,-1.,0.));
#183807=CARTESIAN_POINT('',(0.,0.,0.));
#183808=CARTESIAN_POINT('Origin',(114.28108174878,1.45439216225896E-14,
64.7979697995068));
#183809=CARTESIAN_POINT('',(114.543318806555,-13.8999677591299,63.4488784306985));
#183810=CARTESIAN_POINT('',(114.524364138745,-13.9,63.5463966488937));
#183811=CARTESIAN_POINT('',(114.28108174878,-13.9,64.7979697995068));
#183812=CARTESIAN_POINT('',(122.504911944309,-11.2745028192005,65.0976651712153));
#183813=CARTESIAN_POINT('Ctrl Pts',(114.543277020905,-13.8999999999995,
63.4490800523684));
#183814=CARTESIAN_POINT('Ctrl Pts',(115.963658533117,-13.9000003730414,
63.7423954021979));
#183815=CARTESIAN_POINT('Ctrl Pts',(117.375536377089,-13.6730345732275,
64.0328163031302));
#183816=CARTESIAN_POINT('Ctrl Pts',(119.398830937964,-13.005804924131,64.4519447188775));
#183817=CARTESIAN_POINT('Ctrl Pts',(120.052705348276,-12.7312234003918,
64.5876385202321));
#183818=CARTESIAN_POINT('Ctrl Pts',(121.318245112142,-12.0781519615802,
64.8504007864608));
#183819=CARTESIAN_POINT('Ctrl Pts',(121.927541701631,-11.6997943110756,
64.9769801574177));
#183820=CARTESIAN_POINT('Ctrl Pts',(122.504912016709,-11.2745030813742,
65.0976657537235));
#183821=CARTESIAN_POINT('Origin',(114.524364387726,1.45439216225896E-14,
63.5463953680056));
#183822=CARTESIAN_POINT('Origin',(114.28108174878,1.45439216225896E-14,
64.7979697995068));
#183823=CARTESIAN_POINT('',(114.734115976417,-13.9,62.4673223247922));
#183824=CARTESIAN_POINT('',(114.700601321121,-13.899802441188,62.6397761140198));
#183825=CARTESIAN_POINT('',(114.28108174878,-13.9,64.7979697995068));
#183826=CARTESIAN_POINT('Ctrl Pts',(114.543319397432,-13.8999999999999,
63.4488737117307));
#183827=CARTESIAN_POINT('Ctrl Pts',(114.095666858061,-13.8999999556334,
63.3565847360325));
#183828=CARTESIAN_POINT('Ctrl Pts',(113.648290388235,-13.8774585757879,
63.26433528182));
#183829=CARTESIAN_POINT('Ctrl Pts',(112.763519724712,-13.7880783064319,
63.0817266868347));
#183830=CARTESIAN_POINT('Ctrl Pts',(112.326596578786,-13.7219076525622,
62.991467458277));
#183831=CARTESIAN_POINT('Ctrl Pts',(111.04717373429,-13.4626911120813,62.7271043930887));
#183832=CARTESIAN_POINT('Ctrl Pts',(110.218606810636,-13.2094152370216,
62.5560384754181));
#183833=CARTESIAN_POINT('Ctrl Pts',(108.807977651217,-12.6241766275,62.2636692196187));
#183834=CARTESIAN_POINT('Ctrl Pts',(108.215659315782,-12.3255326627123,
62.1405161583243));
#183835=CARTESIAN_POINT('Ctrl Pts',(107.153869499696,-11.6883047558964,
61.9194894819314));
#183836=CARTESIAN_POINT('Ctrl Pts',(106.679601671333,-11.3609608995555,
61.8206212074063));
#183837=CARTESIAN_POINT('Ctrl Pts',(105.514845982761,-10.4426739187582,
61.5767317628101));
#183838=CARTESIAN_POINT('Ctrl Pts',(104.859172139605,-9.81046764030742,
61.4383282488724));
#183839=CARTESIAN_POINT('Ctrl Pts',(103.886795108932,-8.66655667634508,
61.2317970762891));
#183840=CARTESIAN_POINT('Ctrl Pts',(103.532920024943,-8.19162093957372,
61.1561537548604));
#183841=CARTESIAN_POINT('Ctrl Pts',(102.722495520566,-6.94462140645532,
60.981105216045));
#183842=CARTESIAN_POINT('Ctrl Pts',(102.307663196382,-6.14760569873943,
60.8898131920288));
#183843=CARTESIAN_POINT('Ctrl Pts',(101.515929828871,-4.18733815719314,
60.7114347669576));
#183844=CARTESIAN_POINT('Ctrl Pts',(101.208308156127,-3.00297326747312,
60.6371461238094));
#183845=CARTESIAN_POINT('Ctrl Pts',(100.965362890981,-1.06678823885153,
60.5673269685623));
#183846=CARTESIAN_POINT('Ctrl Pts',(100.930699011687,-0.334633476992079,
60.5521801336653));
#183847=CARTESIAN_POINT('Ctrl Pts',(100.972382330946,1.04335826550525,60.5440932546729));
#183848=CARTESIAN_POINT('Ctrl Pts',(101.036197286776,1.6876291483366,60.5488319398315));
#183849=CARTESIAN_POINT('Ctrl Pts',(101.263726472942,3.035974669637,60.5772361096543));
#183850=CARTESIAN_POINT('Ctrl Pts',(101.437780966737,3.73635802861391,60.6027837747792));
#183851=CARTESIAN_POINT('Ctrl Pts',(101.869716219272,5.03914724483873,60.6706094706755));
#183852=CARTESIAN_POINT('Ctrl Pts',(102.117613064756,5.6429504599671,60.7110521206048));
#183853=CARTESIAN_POINT('Ctrl Pts',(102.661437777928,6.74317933045791,60.8025239489437));
#183854=CARTESIAN_POINT('Ctrl Pts',(102.947976024289,7.24287385664565,60.8515898869089));
#183855=CARTESIAN_POINT('Ctrl Pts',(103.643933464606,8.299582680346,60.9720271090248));
#183856=CARTESIAN_POINT('Ctrl Pts',(104.065499529978,8.84648795263345,61.0457170265283));
#183857=CARTESIAN_POINT('Ctrl Pts',(104.911710572345,9.78996260364795,61.1953631768537));
#183858=CARTESIAN_POINT('Ctrl Pts',(105.324276576804,10.1956581742615,61.2688935280097));
#183859=CARTESIAN_POINT('Ctrl Pts',(106.448827986222,11.1703231066037,61.4700161663888));
#183860=CARTESIAN_POINT('Ctrl Pts',(107.19343788303,11.6960002788795,61.603803779604));
#183861=CARTESIAN_POINT('Ctrl Pts',(108.505403938263,12.438609519224,61.8411856915302));
#183862=CARTESIAN_POINT('Ctrl Pts',(109.045785726917,12.6989811367864,61.9392443328906));
#183863=CARTESIAN_POINT('Ctrl Pts',(110.15911199204,13.147279214675,62.1414081656069));
#183864=CARTESIAN_POINT('Ctrl Pts',(110.730986829252,13.3343797093401,62.2453201503661));
#183865=CARTESIAN_POINT('Ctrl Pts',(111.877370220333,13.6265072769908,62.454157501314));
#183866=CARTESIAN_POINT('Ctrl Pts',(112.450103197555,13.7335642527326,62.5587283502245));
#183867=CARTESIAN_POINT('Ctrl Pts',(113.925491520917,13.9114597597983,62.8279600194855));
#183868=CARTESIAN_POINT('Ctrl Pts',(114.831555553521,13.928957848391,62.9931269391823));
#183869=CARTESIAN_POINT('Ctrl Pts',(116.30312027824,13.8089226881333,63.2618155048913));
#183870=CARTESIAN_POINT('Ctrl Pts',(116.870184897286,13.7260270358041,63.3653591437266));
#183871=CARTESIAN_POINT('Ctrl Pts',(118.301747125635,13.4225894299414,63.6262596268049));
#183872=CARTESIAN_POINT('Ctrl Pts',(119.153252298888,13.1519152204113,63.7810545565729));
#183873=CARTESIAN_POINT('Ctrl Pts',(121.10410515881,12.312096190463,64.1354159651481));
#183874=CARTESIAN_POINT('Ctrl Pts',(122.165901283655,11.672408931806,64.3269975888839));
#183875=CARTESIAN_POINT('Ctrl Pts',(123.690027133608,10.446406698609,64.6004070749153));
#183876=CARTESIAN_POINT('Ctrl Pts',(124.215010895498,9.95156385919201,64.6941085162938));
#183877=CARTESIAN_POINT('Ctrl Pts',(125.133313068973,8.93931931230886,64.8564485403229));
#183878=CARTESIAN_POINT('Ctrl Pts',(125.533534293469,8.43101852891742,64.9265388233358));
#183879=CARTESIAN_POINT('Ctrl Pts',(126.300234608229,7.30386579935176,65.0597252056201));
#183880=CARTESIAN_POINT('Ctrl Pts',(126.657350831049,6.68070642598612,65.1208713547891));
#183881=CARTESIAN_POINT('Ctrl Pts',(127.245535158981,5.44319417078767,65.2190752083594));
#183882=CARTESIAN_POINT('Ctrl Pts',(127.484400106291,4.83478584246649,65.2577526502302));
#183883=CARTESIAN_POINT('Ctrl Pts',(127.853344441209,3.66119464150078,65.3152211153698));
#183884=CARTESIAN_POINT('Ctrl Pts',(127.992529580459,3.10039807508109,65.3356435666504));
#183885=CARTESIAN_POINT('Ctrl Pts',(128.222566968736,1.85097788176063,65.3655174364438));
#183886=CARTESIAN_POINT('Ctrl Pts',(128.297861298161,1.16097522242937,65.3719024044926));
#183887=CARTESIAN_POINT('Ctrl Pts',(128.342829339017,-0.114099057704563,
65.3658051851043));
#183888=CARTESIAN_POINT('Ctrl Pts',(128.327381754698,-0.697112821076571,
65.3561374270146));
#183889=CARTESIAN_POINT('Ctrl Pts',(128.195199470171,-2.1923670140522,65.3129742889966));
#183890=CARTESIAN_POINT('Ctrl Pts',(128.025491438625,-3.09677295482776,
65.2690355788747));
#183891=CARTESIAN_POINT('Ctrl Pts',(127.600229675744,-4.55878546281939,
65.1687354873144));
#183892=CARTESIAN_POINT('Ctrl Pts',(127.393875146453,-5.12829977345572,
65.1216451956539));
#183893=CARTESIAN_POINT('Ctrl Pts',(126.908088047125,-6.23919834028285,
65.0129688012945));
#183894=CARTESIAN_POINT('Ctrl Pts',(126.628771211294,-6.77919527132568,
64.9514195832402));
#183895=CARTESIAN_POINT('Ctrl Pts',(126.01203208648,-7.80184336414442,64.8175344690342));
#183896=CARTESIAN_POINT('Ctrl Pts',(125.677332042665,-8.28471927884472,
64.7457179487588));
#183897=CARTESIAN_POINT('Ctrl Pts',(124.748081073692,-9.45857911508621,
64.5475333442691));
#183898=CARTESIAN_POINT('Ctrl Pts',(124.11459511956,-10.1137542204333,64.413440583838));
#183899=CARTESIAN_POINT('Ctrl Pts',(122.98384959728,-11.0716104050755,64.1762880080513));
#183900=CARTESIAN_POINT('Ctrl Pts',(122.522981749875,-11.4144946474593,
64.0800199875524));
#183901=CARTESIAN_POINT('Ctrl Pts',(121.295261360778,-12.2125098687246,
63.8240049791676));
#183902=CARTESIAN_POINT('Ctrl Pts',(120.503393423168,-12.6225011135906,
63.6593592767822));
#183903=CARTESIAN_POINT('Ctrl Pts',(118.538928359555,-13.4043707646203,
63.2526584710292));
#183904=CARTESIAN_POINT('Ctrl Pts',(117.345142289443,-13.6989780332306,
63.0057991772094));
#183905=CARTESIAN_POINT('Ctrl Pts',(115.665401057228,-13.8755975852762,
62.6593395765601));
#183906=CARTESIAN_POINT('Ctrl Pts',(115.199873509996,-13.9000000006544,
62.5633870594715));
#183907=CARTESIAN_POINT('Ctrl Pts',(114.734115967029,-13.9,62.4673223229672));
#183908=CARTESIAN_POINT('',(108.175215076124,-12.3034455984317,62.3120820166501));
#183909=CARTESIAN_POINT('Origin',(114.524364387726,1.45439216225896E-14,
63.5463953680056));
#183910=CARTESIAN_POINT('Ctrl Pts',(108.175253011541,-12.3034472057424,
62.311902880219));
#183911=CARTESIAN_POINT('Ctrl Pts',(107.829254740664,-12.1176623915642,
62.2397973760768));
#183912=CARTESIAN_POINT('Ctrl Pts',(107.491277563595,-11.9167369790387,
62.1692332067497));
#183913=CARTESIAN_POINT('Ctrl Pts',(106.831310016517,-11.4844746236066,
62.0313407147435));
#183914=CARTESIAN_POINT('Ctrl Pts',(106.509733403427,-11.2531712530537,
61.9640985330967));
#183915=CARTESIAN_POINT('Ctrl Pts',(105.602344025973,-10.5384778680501,
61.7742112359076));
#183916=CARTESIAN_POINT('Ctrl Pts',(105.04545782268,-10.0192730233713,61.6575406729719));
#183917=CARTESIAN_POINT('Ctrl Pts',(103.760334761446,-8.60418667222819,
61.3859000074079));
#183918=CARTESIAN_POINT('Ctrl Pts',(103.095170897116,-7.65697825411397,
61.2419655442359));
#183919=CARTESIAN_POINT('Ctrl Pts',(102.124067674928,-5.82764326895935,
61.028631765501));
#183920=CARTESIAN_POINT('Ctrl Pts',(101.774591739413,-4.9774463721549,60.9505465000764));
#183921=CARTESIAN_POINT('Ctrl Pts',(101.16866552192,-2.96220367212895,60.8090494773863));
#183922=CARTESIAN_POINT('Ctrl Pts',(100.971876285014,-1.78602280028819,
60.7559125155545));
#183923=CARTESIAN_POINT('Ctrl Pts',(100.882216640194,0.451211526356952,
60.7119554141485));
#183924=CARTESIAN_POINT('Ctrl Pts',(100.956917923202,1.50253571188173,60.7150089831391));
#183925=CARTESIAN_POINT('Ctrl Pts',(101.356286852974,3.66982229471046,60.7676413643215));
#183926=CARTESIAN_POINT('Ctrl Pts',(101.703424332697,4.77356625794603,60.8205557150018));
#183927=CARTESIAN_POINT('Ctrl Pts',(102.539106412512,6.60966146675549,60.9591717826443));
#183928=CARTESIAN_POINT('Ctrl Pts',(102.969573248346,7.36229662531501,61.0332292093258));
#183929=CARTESIAN_POINT('Ctrl Pts',(104.508490782369,9.55311376250124,61.3021821784205));
#183930=CARTESIAN_POINT('Ctrl Pts',(105.827682525528,10.81452146383,61.5354704994559));
#183931=CARTESIAN_POINT('Ctrl Pts',(107.865340341772,12.1108218284781,61.9041305156421));
#183932=CARTESIAN_POINT('Ctrl Pts',(108.403950897371,12.4045022658587,62.0020176235738));
#183933=CARTESIAN_POINT('Ctrl Pts',(110.007432795916,13.1429611170253,62.2928996629309));
#183934=CARTESIAN_POINT('Ctrl Pts',(111.110541210227,13.4891653894966,62.4925723628407));
#183935=CARTESIAN_POINT('Ctrl Pts',(112.965752884932,13.8198863955061,62.8310419799776));
#183936=CARTESIAN_POINT('Ctrl Pts',(113.697498351287,13.8893915556794,62.9650733315565));
#183937=CARTESIAN_POINT('Ctrl Pts',(115.59178945293,13.9138787699293,63.3115985440927));
#183938=CARTESIAN_POINT('Ctrl Pts',(116.749786876645,13.7786142098174,63.5218867436072));
#183939=CARTESIAN_POINT('Ctrl Pts',(119.049155845185,13.2027979487908,63.9403577904306));
#183940=CARTESIAN_POINT('Ctrl Pts',(120.177786278009,12.7527836771607,64.1467207138746));
#183941=CARTESIAN_POINT('Ctrl Pts',(121.753889642778,11.8653084912738,64.4316950775613));
#183942=CARTESIAN_POINT('Ctrl Pts',(122.254588513511,11.5384354163202,64.5215824075115));
#183943=CARTESIAN_POINT('Ctrl Pts',(124.180794774509,10.0927655755584,64.866524455924));
#183944=CARTESIAN_POINT('Ctrl Pts',(125.40356229856,8.72635832711256,65.085168210104));
#183945=CARTESIAN_POINT('Ctrl Pts',(126.770953942903,6.41826960404145,65.3183833253468));
#183946=CARTESIAN_POINT('Ctrl Pts',(127.140959249248,5.63790441019896,65.3797443818023));
#183947=CARTESIAN_POINT('Ctrl Pts',(127.83023994192,3.75404615250889,65.4904859045506));
#183948=CARTESIAN_POINT('Ctrl Pts',(128.0911700665,2.63526781093659,65.5290708030479));
#183949=CARTESIAN_POINT('Ctrl Pts',(128.315084764473,0.5730578530517,65.5478115641301));
#183950=CARTESIAN_POINT('Ctrl Pts',(128.324290676776,-0.358476281530813,
65.5380796946296));
#183951=CARTESIAN_POINT('Ctrl Pts',(128.141415510887,-2.41660215404027,
65.4784331948131));
#183952=CARTESIAN_POINT('Ctrl Pts',(127.904389136551,-3.53226331065458,
65.4203161659102));
#183953=CARTESIAN_POINT('Ctrl Pts',(127.306122110614,-5.27960018632084,
65.282161846537));
#183954=CARTESIAN_POINT('Ctrl Pts',(127.024821956496,-5.93425990435274,
65.2186308296363));
#183955=CARTESIAN_POINT('Ctrl Pts',(125.99183594923,-7.90815734164247,64.9909955785248));
#183956=CARTESIAN_POINT('Ctrl Pts',(125.07553331115,-9.12479661675895,64.7969688624804));
#183957=CARTESIAN_POINT('Ctrl Pts',(123.303414517789,-10.8138306825123,
64.4228647444522));
#183958=CARTESIAN_POINT('Ctrl Pts',(122.559121563029,-11.3895644829671,
64.2663923791376));
#183959=CARTESIAN_POINT('Ctrl Pts',(120.823677322221,-12.4652132965739,
63.9049518929865));
#183960=CARTESIAN_POINT('Ctrl Pts',(119.818584531465,-12.9290262905671,
63.6977086298234));
#183961=CARTESIAN_POINT('Ctrl Pts',(117.453078853571,-13.68568167006,63.2079891353038));
#183962=CARTESIAN_POINT('Ctrl Pts',(116.081021780324,-13.8999991869096,
62.9238711704367));
#183963=CARTESIAN_POINT('Ctrl Pts',(114.700619831036,-13.8999999999977,
62.6396862741661));
#183964=CARTESIAN_POINT('Origin',(114.28108174878,1.45439216225896E-14,
64.7979697995068));
#183965=CARTESIAN_POINT('',(114.924931416105,-13.9,61.4856668343432));
#183966=CARTESIAN_POINT('',(114.891525389284,-13.9,61.6575251889163));
#183967=CARTESIAN_POINT('',(114.28108174878,-13.9,64.7979697995068));
#183968=CARTESIAN_POINT('Ctrl Pts',(114.734115967029,-13.9,62.4673223229672));
#183969=CARTESIAN_POINT('Ctrl Pts',(114.635896167658,-13.899999999862,62.4470640162828));
#183970=CARTESIAN_POINT('Ctrl Pts',(114.537666032757,-13.8989147967141,
62.4268012395597));
#183971=CARTESIAN_POINT('Ctrl Pts',(113.752677260478,-13.8815634299461,
62.264853343907));
#183972=CARTESIAN_POINT('Ctrl Pts',(113.068056815718,-13.8133361697656,
62.123426082441));
#183973=CARTESIAN_POINT('Ctrl Pts',(111.829864962314,-13.5924920938731,
61.8678210539804));
#183974=CARTESIAN_POINT('Ctrl Pts',(111.275045072243,-13.4564272681486,
61.7533165731196));
#183975=CARTESIAN_POINT('Ctrl Pts',(109.870150650892,-13.0150078958601,
61.4627690581557));
#183976=CARTESIAN_POINT('Ctrl Pts',(109.038517459101,-12.6583388104979,
61.2901654699463));
#183977=CARTESIAN_POINT('Ctrl Pts',(107.718273635188,-11.9275483923215,
61.0158078887912));
#183978=CARTESIAN_POINT('Ctrl Pts',(107.208712096802,-11.5990803884342,
60.9096883303051));
#183979=CARTESIAN_POINT('Ctrl Pts',(106.131717685568,-10.798078129996,60.6844050688731));
#183980=CARTESIAN_POINT('Ctrl Pts',(105.576928927187,-10.3110560287063,
60.5677004564676));
#183981=CARTESIAN_POINT('Ctrl Pts',(104.657889985637,-9.36269681458055,
60.373623394926));
#183982=CARTESIAN_POINT('Ctrl Pts',(104.279094634271,-8.91861240693393,
60.2932285124025));
#183983=CARTESIAN_POINT('Ctrl Pts',(103.540356978776,-7.93230470128705,
60.1351062031801));
#183984=CARTESIAN_POINT('Ctrl Pts',(103.188067335821,-7.38588896166875,
60.0588505195161));
#183985=CARTESIAN_POINT('Ctrl Pts',(102.593852577201,-6.30515520550776,
59.9289116231603));
#183986=CARTESIAN_POINT('Ctrl Pts',(102.344893342825,-5.77648160515211,
59.8738146532213));
#183987=CARTESIAN_POINT('Ctrl Pts',(101.791855358639,-4.38196891390696,
59.7488082625675));
#183988=CARTESIAN_POINT('Ctrl Pts',(101.537992795468,-3.4984291459401,59.6885085713535));
#183989=CARTESIAN_POINT('Ctrl Pts',(101.26454815401,-2.01541232078002,59.6179020922508));
#183990=CARTESIAN_POINT('Ctrl Pts',(101.193967076518,-1.42873676667916,
59.5973940526453));
#183991=CARTESIAN_POINT('Ctrl Pts',(101.108757269638,0.0615188109527515,
59.5633717388363));
#183992=CARTESIAN_POINT('Ctrl Pts',(101.143503601298,0.965396462221698,
59.5594450102026));
#183993=CARTESIAN_POINT('Ctrl Pts',(101.428127128293,3.07839382916166,59.5901666994286));
#183994=CARTESIAN_POINT('Ctrl Pts',(101.750431932911,4.26993893037958,59.6382183554188));
#183995=CARTESIAN_POINT('Ctrl Pts',(102.443128861265,5.93313458782272,59.7519764190383));
#183996=CARTESIAN_POINT('Ctrl Pts',(102.695991991924,6.44883437696944,59.7945232341841));
#183997=CARTESIAN_POINT('Ctrl Pts',(103.326935038705,7.55777733348192,59.9022182410436));
#183998=CARTESIAN_POINT('Ctrl Pts',(103.719479497111,8.14070209233188,59.9701279554908));
#183999=CARTESIAN_POINT('Ctrl Pts',(104.512005893588,9.14488540591357,60.109218648897));
#184000=CARTESIAN_POINT('Ctrl Pts',(104.897914135787,9.57560031567484,60.1775771644449));
#184001=CARTESIAN_POINT('Ctrl Pts',(105.958829077431,10.6200285364352,60.3663401625124));
#184002=CARTESIAN_POINT('Ctrl Pts',(106.66916132764,11.1925712253983,60.4934665576179));
#184003=CARTESIAN_POINT('Ctrl Pts',(107.945900174839,12.0271566367378,60.7238116492156));
#184004=CARTESIAN_POINT('Ctrl Pts',(108.483813730122,12.3289135698586,60.8211984225643));
#184005=CARTESIAN_POINT('Ctrl Pts',(109.556520553774,12.8383026118733,61.0156177886013));
#184006=CARTESIAN_POINT('Ctrl Pts',(110.087792735784,13.0505821597941,61.1120025791216));
#184007=CARTESIAN_POINT('Ctrl Pts',(111.172997793677,13.4064287005963,61.3094289387588));
#184008=CARTESIAN_POINT('Ctrl Pts',(111.725862323305,13.5496736965118,61.4102746261987));
#184009=CARTESIAN_POINT('Ctrl Pts',(112.886581533898,13.773013657989,61.6219503369437));
#184010=CARTESIAN_POINT('Ctrl Pts',(113.494209256948,13.8475220551837,61.7327298295075));
#184011=CARTESIAN_POINT('Ctrl Pts',(115.007418048799,13.9291643173604,62.0087394679497));
#184012=CARTESIAN_POINT('Ctrl Pts',(115.91260292229,13.8867665782517,62.1742559777357));
#184013=CARTESIAN_POINT('Ctrl Pts',(117.373453579555,13.6697583322359,62.4406714400258));
#184014=CARTESIAN_POINT('Ctrl Pts',(117.934073416039,13.5495724553436,62.5427423827476));
#184015=CARTESIAN_POINT('Ctrl Pts',(119.153592051578,13.2056843393237,62.764742210071));
#184016=CARTESIAN_POINT('Ctrl Pts',(119.806488951848,12.9659861092103,62.8836291520487));
#184017=CARTESIAN_POINT('Ctrl Pts',(120.955170085647,12.441007372748,63.091997273171));
#184018=CARTESIAN_POINT('Ctrl Pts',(121.456708344703,12.1726380502158,63.1826825581831));
#184019=CARTESIAN_POINT('Ctrl Pts',(122.97630808687,11.232849257144,63.4568125567142));
#184020=CARTESIAN_POINT('Ctrl Pts',(123.923874073463,10.4551372939055,63.6270106756665));
#184021=CARTESIAN_POINT('Ctrl Pts',(125.369961924471,8.90556080816441,63.8829353842257));
#184022=CARTESIAN_POINT('Ctrl Pts',(125.917271364093,8.19140609685299,63.9789988095767));
#184023=CARTESIAN_POINT('Ctrl Pts',(126.703248248531,6.93030851442651,64.1144186025104));
#184024=CARTESIAN_POINT('Ctrl Pts',(126.982319565787,6.41264139321977,64.1617037292598));
#184025=CARTESIAN_POINT('Ctrl Pts',(127.541630646307,5.19825218776111,64.2546543347858));
#184026=CARTESIAN_POINT('Ctrl Pts',(127.800300720684,4.49331540503752,64.2963683058652));
#184027=CARTESIAN_POINT('Ctrl Pts',(128.166003036208,3.1821969109469,64.3516255255006));
#184028=CARTESIAN_POINT('Ctrl Pts',(128.291875485707,2.58340175081135,64.3688768980793));
#184029=CARTESIAN_POINT('Ctrl Pts',(128.509038325966,1.06866058858028,64.3930768310356));
#184030=CARTESIAN_POINT('Ctrl Pts',(128.550514139004,0.148384806139156,
64.3907044141276));
#184031=CARTESIAN_POINT('Ctrl Pts',(128.4722674771,-1.35045934555967,64.357941167705));
#184032=CARTESIAN_POINT('Ctrl Pts',(128.406112151684,-1.92921059428031,
64.3381726626449));
#184033=CARTESIAN_POINT('Ctrl Pts',(128.1826243107,-3.18904527889961,64.2797455896531));
#184034=CARTESIAN_POINT('Ctrl Pts',(128.010029513088,-3.86569409566474,
64.2382398556052));
#184035=CARTESIAN_POINT('Ctrl Pts',(127.605269446791,-5.07121511591131,
64.1447082622545));
#184036=CARTESIAN_POINT('Ctrl Pts',(127.38916685262,-5.6040859641453,64.095885838586));
#184037=CARTESIAN_POINT('Ctrl Pts',(126.865819217611,-6.69649725754257,
63.9798490677641));
#184038=CARTESIAN_POINT('Ctrl Pts',(126.551735609575,-7.25116162208593,
63.9114670898447));
#184039=CARTESIAN_POINT('Ctrl Pts',(125.794462386711,-8.39749772082035,
63.7482436542481));
#184040=CARTESIAN_POINT('Ctrl Pts',(125.339869226604,-8.97894230383076,
63.6511060823714));
#184041=CARTESIAN_POINT('Ctrl Pts',(124.226088892404,-10.1899136983897,
63.4150725084999));
#184042=CARTESIAN_POINT('Ctrl Pts',(123.546627179499,-10.7953448027287,
63.2725735105477));
#184043=CARTESIAN_POINT('Ctrl Pts',(122.331099553002,-11.6783291334865,
63.0184528822517));
#184044=CARTESIAN_POINT('Ctrl Pts',(121.826691068776,-11.9962788257679,
62.9132163000579));
#184045=CARTESIAN_POINT('Ctrl Pts',(120.82300537439,-12.5399590865741,62.7046068003729));
#184046=CARTESIAN_POINT('Ctrl Pts',(120.327563078071,-12.7706032396118,
62.6019474893253));
#184047=CARTESIAN_POINT('Ctrl Pts',(119.249420650729,-13.1948381797639,
62.3786746269096));
#184048=CARTESIAN_POINT('Ctrl Pts',(118.664740636947,-13.3798201465247,
62.2576574802116));
#184049=CARTESIAN_POINT('Ctrl Pts',(117.19430633689,-13.7362978133568,61.9536683022571));
#184050=CARTESIAN_POINT('Ctrl Pts',(116.300198006568,-13.8593883826947,
61.769436047561));
#184051=CARTESIAN_POINT('Ctrl Pts',(115.242206907773,-13.8971693108471,
61.5511440092589));
#184052=CARTESIAN_POINT('Ctrl Pts',(115.08355907857,-13.9000000002285,61.5184055635395));
#184053=CARTESIAN_POINT('Ctrl Pts',(114.924931416059,-13.9,61.4856668345648));
#184054=CARTESIAN_POINT('Ctrl Pts',(114.891525389284,-13.9,61.6575251889163));
#184055=CARTESIAN_POINT('Ctrl Pts',(115.021517509571,-13.9,61.6843424943502));
#184056=CARTESIAN_POINT('Ctrl Pts',(115.15154264268,-13.898099124399,61.71117858686));
#184057=CARTESIAN_POINT('Ctrl Pts',(115.785600842462,-13.8795440287187,
61.8421018209282));
#184058=CARTESIAN_POINT('Ctrl Pts',(116.28840999186,-13.8362123171273,61.9461231274097));
#184059=CARTESIAN_POINT('Ctrl Pts',(117.268922403503,-13.6953797895739,
62.1490977346866));
#184060=CARTESIAN_POINT('Ctrl Pts',(117.746179025309,-13.599993637292,62.2479495590594));
#184061=CARTESIAN_POINT('Ctrl Pts',(118.738264858113,-13.3447687463504,
62.4529212773574));
#184062=CARTESIAN_POINT('Ctrl Pts',(119.250894910031,-13.179435075753,62.558577125659));
#184063=CARTESIAN_POINT('Ctrl Pts',(120.325277327308,-12.7600767453057,
62.7804514601469));
#184064=CARTESIAN_POINT('Ctrl Pts',(120.882475216428,-12.497292281585,62.8958055946432));
#184065=CARTESIAN_POINT('Ctrl Pts',(121.84406935716,-11.9605109365751,63.0958726894617));
#184066=CARTESIAN_POINT('Ctrl Pts',(122.255123020173,-11.7011005126847,
63.1817430709072));
#184067=CARTESIAN_POINT('Ctrl Pts',(123.136431562167,-11.0763349546819,
63.366455028576));
#184068=CARTESIAN_POINT('Ctrl Pts',(123.598645354841,-10.7009020034612,
63.4637544100384));
#184069=CARTESIAN_POINT('Ctrl Pts',(124.234286386822,-10.1118424866292,
63.5974713979145));
#184070=CARTESIAN_POINT('Ctrl Pts',(124.427635187138,-9.92171607736547,
63.6381411877191));
#184071=CARTESIAN_POINT('Ctrl Pts',(125.277745172076,-9.03476459572254,
63.8172342067226));
#184072=CARTESIAN_POINT('Ctrl Pts',(125.867547960082,-8.2748881592662,63.9424827405772));
#184073=CARTESIAN_POINT('Ctrl Pts',(126.645136494603,-7.02388795670556,
64.1111991518969));
#184074=CARTESIAN_POINT('Ctrl Pts',(126.891368446709,-6.57415787600783,
64.1653507515486));
#184075=CARTESIAN_POINT('Ctrl Pts',(127.325060840968,-5.66681791284177,
64.2620232394482));
#184076=CARTESIAN_POINT('Ctrl Pts',(127.514129745694,-5.21083948500054,
64.3048420588134));
#184077=CARTESIAN_POINT('Ctrl Pts',(127.861323649825,-4.23072694869992,
64.3844376577583));
#184078=CARTESIAN_POINT('Ctrl Pts',(128.01371730787,-3.70535502299583,64.4200630029777));
#184079=CARTESIAN_POINT('Ctrl Pts',(128.274360541119,-2.56195304650751,
64.483761209423));
#184080=CARTESIAN_POINT('Ctrl Pts',(128.372764495814,-1.94280823956164,
64.5099416324965));
#184081=CARTESIAN_POINT('Ctrl Pts',(128.474610308618,-0.827970181223037,
64.5428973473318));
#184082=CARTESIAN_POINT('Ctrl Pts',(128.493747115742,-0.334873068718832,
64.5525859719842));
#184083=CARTESIAN_POINT('Ctrl Pts',(128.478985407369,0.761119158531955,
64.5631206489104));
#184084=CARTESIAN_POINT('Ctrl Pts',(128.432356989912,1.36288458641404,64.5615132169177));
#184085=CARTESIAN_POINT('Ctrl Pts',(128.30907551438,2.23113739090421,64.5477121398652));
#184086=CARTESIAN_POINT('Ctrl Pts',(128.262687436482,2.50131657915118,64.5417815305607));
#184087=CARTESIAN_POINT('Ctrl Pts',(128.017240688512,3.71790181147584,64.5079189575195));
#184088=CARTESIAN_POINT('Ctrl Pts',(127.729400730189,4.64315108149147,64.4625703173702));
#184089=CARTESIAN_POINT('Ctrl Pts',(127.147070503319,6.00326429112005,64.3669441910773));
#184090=CARTESIAN_POINT('Ctrl Pts',(126.919053240595,6.46411574179415,64.328910658348));
#184091=CARTESIAN_POINT('Ctrl Pts',(126.423685186711,7.34061665366765,64.2449910986012));
#184092=CARTESIAN_POINT('Ctrl Pts',(126.158564659135,7.75670657393927,64.1995238686699));
#184093=CARTESIAN_POINT('Ctrl Pts',(125.555578569915,8.60099508833629,64.0944220572823));
#184094=CARTESIAN_POINT('Ctrl Pts',(125.213496478063,9.025047166611,64.0339304875756));
#184095=CARTESIAN_POINT('Ctrl Pts',(124.42917356429,9.88804004712674,63.8945068210594));
#184096=CARTESIAN_POINT('Ctrl Pts',(123.980503315742,10.3193027551998,63.8143463347171));
#184097=CARTESIAN_POINT('Ctrl Pts',(123.13034835435,11.0323519590428,63.6622509853));
#184098=CARTESIAN_POINT('Ctrl Pts',(122.739785572062,11.3259013103544,63.5923016600345));
#184099=CARTESIAN_POINT('Ctrl Pts',(121.839552196591,11.930058660532,63.4307172654153));
#184100=CARTESIAN_POINT('Ctrl Pts',(121.323660417594,12.2292977528083,63.3378938876921));
#184101=CARTESIAN_POINT('Ctrl Pts',(120.547959842612,12.6137155897992,63.1972748218409));
#184102=CARTESIAN_POINT('Ctrl Pts',(120.302087869348,12.7265544829315,63.1525682883864));
#184103=CARTESIAN_POINT('Ctrl Pts',(119.17445997396,13.2038002162657,62.9472262321971));
#184104=CARTESIAN_POINT('Ctrl Pts',(118.260137061622,13.4814294916997,62.780101043474));
#184105=CARTESIAN_POINT('Ctrl Pts',(116.826657287953,13.7555605107813,62.5190274253581));
#184106=CARTESIAN_POINT('Ctrl Pts',(116.323702084606,13.8225979074876,62.4275511452423));
#184107=CARTESIAN_POINT('Ctrl Pts',(115.332506604706,13.8981158963788,62.2472519725531));
#184108=CARTESIAN_POINT('Ctrl Pts',(114.845160031885,13.9087234874643,62.1585880743205));
#184109=CARTESIAN_POINT('Ctrl Pts',(113.819835237767,13.8753613438994,61.9713914397251));
#184110=CARTESIAN_POINT('Ctrl Pts',(113.282866416028,13.8255034635852,61.8730175292959));
#184111=CARTESIAN_POINT('Ctrl Pts',(112.140587816258,13.6498105473389,61.664013944062));
#184112=CARTESIAN_POINT('Ctrl Pts',(111.537912411116,13.5142507755298,61.5539177122545));
#184113=CARTESIAN_POINT('Ctrl Pts',(110.480592181834,13.1989780922456,61.3615532677561));
#184114=CARTESIAN_POINT('Ctrl Pts',(110.022521143674,13.035051444953,61.2784815831576));
#184115=CARTESIAN_POINT('Ctrl Pts',(109.025614601247,12.6165234382339,61.0981056687943));
#184116=CARTESIAN_POINT('Ctrl Pts',(108.492530134448,12.3503037033032,61.0019403084735));
#184117=CARTESIAN_POINT('Ctrl Pts',(107.744331939226,11.9131177471869,60.8666669881906));
#184118=CARTESIAN_POINT('Ctrl Pts',(107.514517861371,11.7694762972824,60.8250816542274));
#184119=CARTESIAN_POINT('Ctrl Pts',(106.49321331107,11.0880370533729,60.6404070889773));
#184120=CARTESIAN_POINT('Ctrl Pts',(105.754016041265,10.4740821218333,60.5073233445586));
#184121=CARTESIAN_POINT('Ctrl Pts',(104.72604115033,9.42135323739642,60.3250723201675));
#184122=CARTESIAN_POINT('Ctrl Pts',(104.389062285477,9.03569380088552,60.2658583482805));
#184123=CARTESIAN_POINT('Ctrl Pts',(103.770875999386,8.2438164311981,60.1580662167428));
#184124=CARTESIAN_POINT('Ctrl Pts',(103.488453887321,7.8395331923433,60.1092372159773));
#184125=CARTESIAN_POINT('Ctrl Pts',(102.939377720663,6.95727124887921,60.0146220051358));
#184126=CARTESIAN_POINT('Ctrl Pts',(102.678123595837,6.47681012098997,59.9698476723705));
#184127=CARTESIAN_POINT('Ctrl Pts',(102.17950710498,5.41662042944942,59.8859619836853));
#184128=CARTESIAN_POINT('Ctrl Pts',(101.951417578421,4.83371858962455,59.8486741937301));
#184129=CARTESIAN_POINT('Ctrl Pts',(101.613901059843,3.76731863456407,59.7962242624089));
#184130=CARTESIAN_POINT('Ctrl Pts',(101.489806550648,3.28973362356727,59.7780742275802));
#184131=CARTESIAN_POINT('Ctrl Pts',(101.270167196467,2.2167708119723,59.7487779054115));
#184132=CARTESIAN_POINT('Ctrl Pts',(101.187172359889,1.61975726573154,59.7400916512792));
#184133=CARTESIAN_POINT('Ctrl Pts',(101.122228509132,0.74626456947289,59.7376166869233));
#184134=CARTESIAN_POINT('Ctrl Pts',(101.109868852085,0.472759272948751,
59.7382958864607));
#184135=CARTESIAN_POINT('Ctrl Pts',(101.08981902723,-0.768734755580033,
59.7482469682073));
#184136=CARTESIAN_POINT('Ctrl Pts',(101.173492250125,-1.73534846174754,
59.775116930826));
#184137=CARTESIAN_POINT('Ctrl Pts',(101.451206389597,-3.18937214438392,
59.8466594858126));
#184138=CARTESIAN_POINT('Ctrl Pts',(101.574883950745,-3.68780863158581,
59.8769745944806));
#184139=CARTESIAN_POINT('Ctrl Pts',(101.871213089228,-4.6531841180264,59.9469716119864));
#184140=CARTESIAN_POINT('Ctrl Pts',(102.042026207939,-5.11992789505063,
59.9862814979261));
#184141=CARTESIAN_POINT('Ctrl Pts',(102.342523343261,-5.82278618631986,
60.0536013283003));
#184142=CARTESIAN_POINT('Ctrl Pts',(102.454944775281,-6.06612496004753,
60.0784902116731));
#184143=CARTESIAN_POINT('Ctrl Pts',(103.01347300846,-7.18909438449888,60.2011326425552));
#184144=CARTESIAN_POINT('Ctrl Pts',(103.544191229289,-8.0216124532401,60.3151449486792));
#184145=CARTESIAN_POINT('Ctrl Pts',(104.481086804791,-9.19514871257436,
60.5152325808007));
#184146=CARTESIAN_POINT('Ctrl Pts',(104.827298019057,-9.58191908442061,
60.5889330427703));
#184147=CARTESIAN_POINT('Ctrl Pts',(105.537693130351,-10.2905018848784,
60.7394373549886));
#184148=CARTESIAN_POINT('Ctrl Pts',(105.898861062892,-10.6143841362858,
60.8156374241978));
#184149=CARTESIAN_POINT('Ctrl Pts',(106.488905730394,-11.0893326319013,
60.9392043510138));
#184150=CARTESIAN_POINT('Ctrl Pts',(106.706657769267,-11.2540641417708,
60.984640004462));
#184151=CARTESIAN_POINT('Ctrl Pts',(107.688853630776,-11.9516505663239,
61.1891647643256));
#184152=CARTESIAN_POINT('Ctrl Pts',(108.500681383012,-12.4107006906213,
61.3573224772473));
#184153=CARTESIAN_POINT('Ctrl Pts',(109.801882807888,-12.9784814785239,
61.6273485841689));
#184154=CARTESIAN_POINT('Ctrl Pts',(110.26203464034,-13.1499501636883,61.7228850392036));
#184155=CARTESIAN_POINT('Ctrl Pts',(111.032303895836,-13.389784861275,61.8826911150567));
#184156=CARTESIAN_POINT('Ctrl Pts',(111.337488778907,-13.4730735079182,
61.9459739257766));
#184157=CARTESIAN_POINT('Ctrl Pts',(111.967082523259,-13.6211283345275,
62.0763086497608));
#184158=CARTESIAN_POINT('Ctrl Pts',(112.291527670746,-13.6848247953573,
62.1433284130294));
#184159=CARTESIAN_POINT('Ctrl Pts',(113.307033292684,-13.845309617044,62.3526423976342));
#184160=CARTESIAN_POINT('Ctrl Pts',(114.003376205078,-13.9000006098779,
62.4957211308413));
#184161=CARTESIAN_POINT('Ctrl Pts',(114.700691784751,-13.8999999999949,
62.6393364838496));
#184162=CARTESIAN_POINT('Origin',(114.28108174878,1.45439216225896E-14,
64.7979697995068));
#184163=CARTESIAN_POINT('',(115.096794126421,-13.9,60.6015143527077));
#184164=CARTESIAN_POINT('',(115.082307292334,-13.9,60.6760422812756));
#184165=CARTESIAN_POINT('',(114.28108174878,-13.9,64.7979697995068));
#184166=CARTESIAN_POINT('',(123.077303486518,-11.2745052982129,62.1528545153591));
#184167=CARTESIAN_POINT('Origin',(115.096794126421,1.45439216225896E-14,
60.6015143527085));
#184168=CARTESIAN_POINT('Ctrl Pts',(114.924931416059,-13.9,61.4856668345648));
#184169=CARTESIAN_POINT('Ctrl Pts',(114.514032905067,-13.8999999994081,
61.4008626158395));
#184170=CARTESIAN_POINT('Ctrl Pts',(114.103271002266,-13.8810065652294,
61.3160502304064));
#184171=CARTESIAN_POINT('Ctrl Pts',(113.006182867517,-13.7793020447828,
61.0896353703607));
#184172=CARTESIAN_POINT('Ctrl Pts',(112.32419036809,-13.6622179299309,60.9490390673702));
#184173=CARTESIAN_POINT('Ctrl Pts',(111.106950010177,-13.3545824949699,
60.6975111533049));
#184174=CARTESIAN_POINT('Ctrl Pts',(110.568961845001,-13.1818078541457,
60.586132889826));
#184175=CARTESIAN_POINT('Ctrl Pts',(108.91912136123,-12.5345900895855,60.2442150329164));
#184176=CARTESIAN_POINT('Ctrl Pts',(107.857503443739,-11.9433566579271,
60.0238958361878));
#184177=CARTESIAN_POINT('Ctrl Pts',(106.173466873143,-10.6844216139425,
59.6714179578747));
#184178=CARTESIAN_POINT('Ctrl Pts',(105.513242632352,-10.081920690969,59.5327614426922));
#184179=CARTESIAN_POINT('Ctrl Pts',(104.523379834472,-8.98380083103208,
59.3229804851965));
#184180=CARTESIAN_POINT('Ctrl Pts',(104.15931632535,-8.52420686601659,59.2452356543091));
#184181=CARTESIAN_POINT('Ctrl Pts',(103.30517093681,-7.2928162897431,59.0614402579498));
#184182=CARTESIAN_POINT('Ctrl Pts',(102.859450925484,-6.49242222282162,
58.964368624448));
#184183=CARTESIAN_POINT('Ctrl Pts',(102.261852437951,-5.11731025732404,
58.8305990211956));
#184184=CARTESIAN_POINT('Ctrl Pts',(102.062610649424,-4.56717406095993,
58.7849104071466));
#184185=CARTESIAN_POINT('Ctrl Pts',(101.71435217156,-3.37913966085079,58.7027126279407));
#184186=CARTESIAN_POINT('Ctrl Pts',(101.574294195277,-2.73995530396663,
58.6680256235161));
#184187=CARTESIAN_POINT('Ctrl Pts',(101.393312344925,-1.5113723845637,58.618385959947));
#184188=CARTESIAN_POINT('Ctrl Pts',(101.343988993651,-0.924703340505352,
58.6018489958612));
#184189=CARTESIAN_POINT('Ctrl Pts',(101.315244654731,0.407964465518804,
58.5805764040955));
#184190=CARTESIAN_POINT('Ctrl Pts',(101.357898658598,1.15271149000324,58.5803684918613));
#184191=CARTESIAN_POINT('Ctrl Pts',(101.542502280734,2.50059787146857,58.600446000922));
#184192=CARTESIAN_POINT('Ctrl Pts',(101.665786419606,3.10444337802267,58.617143174642));
#184193=CARTESIAN_POINT('Ctrl Pts',(102.069967945765,4.58382249217927,58.6776442243802));
#184194=CARTESIAN_POINT('Ctrl Pts',(102.397525016489,5.4431673293882,58.7308805870588));
#184195=CARTESIAN_POINT('Ctrl Pts',(103.064680271925,6.7830002870378,58.8430135639024));
#184196=CARTESIAN_POINT('Ctrl Pts',(103.35516433932,7.28554395667475,58.8925726843135));
#184197=CARTESIAN_POINT('Ctrl Pts',(104.062374500383,8.35032525702672,59.0150167603172));
#184198=CARTESIAN_POINT('Ctrl Pts',(104.491755830537,8.90195101712393,59.0904842415158));
#184199=CARTESIAN_POINT('Ctrl Pts',(105.344507528353,9.84178792739701,59.2413541929351));
#184200=CARTESIAN_POINT('Ctrl Pts',(105.754255712011,10.2406402662997,59.3141925519481));
#184201=CARTESIAN_POINT('Ctrl Pts',(107.122754069782,11.4164295324604,59.5587960795008));
#184202=CARTESIAN_POINT('Ctrl Pts',(108.160106711424,12.0890355007076,59.7462993795098));
#184203=CARTESIAN_POINT('Ctrl Pts',(110.078924821598,12.9923761103421,60.0939475105977));
#184204=CARTESIAN_POINT('Ctrl Pts',(110.920715000775,13.2915055588507,60.2472450692554));
#184205=CARTESIAN_POINT('Ctrl Pts',(112.342677018892,13.6434122958441,60.5063323924851));
#184206=CARTESIAN_POINT('Ctrl Pts',(112.908261903787,13.7455949846953,60.6093794931222));
#184207=CARTESIAN_POINT('Ctrl Pts',(114.172016931903,13.8913552454079,60.8398216962434));
#184208=CARTESIAN_POINT('Ctrl Pts',(114.87051676782,13.9172606779213,60.9674917987822));
#184209=CARTESIAN_POINT('Ctrl Pts',(116.203888882048,13.8629451010672,61.2109335502684));
#184210=CARTESIAN_POINT('Ctrl Pts',(116.837324029176,13.791939857829,61.3264299018168));
#184211=CARTESIAN_POINT('Ctrl Pts',(118.353143398592,13.5121776196015,61.6026464272976));
#184212=CARTESIAN_POINT('Ctrl Pts',(119.224454202326,13.2587478523551,61.7615785305218));
#184213=CARTESIAN_POINT('Ctrl Pts',(120.59777205431,12.7048673823582,62.0109666833633));
#184214=CARTESIAN_POINT('Ctrl Pts',(121.116878562841,12.4561119004247,62.1049571011554));
#184215=CARTESIAN_POINT('Ctrl Pts',(122.217063387199,11.8402934230996,62.3038804658098));
#184216=CARTESIAN_POINT('Ctrl Pts',(122.789544908906,11.4605812750697,62.4072577213345));
#184217=CARTESIAN_POINT('Ctrl Pts',(123.783277266587,10.6881250419808,62.5856140216536));
#184218=CARTESIAN_POINT('Ctrl Pts',(124.21282752135,10.3089754707472,62.6622838804847));
#184219=CARTESIAN_POINT('Ctrl Pts',(125.075773853561,9.44596303813536,62.815560484972));
#184220=CARTESIAN_POINT('Ctrl Pts',(125.501319723255,8.95596589329347,62.8908115068038));
#184221=CARTESIAN_POINT('Ctrl Pts',(126.323317115303,7.86364683973198,63.0346672225302));
#184222=CARTESIAN_POINT('Ctrl Pts',(126.710597312391,7.25657985429476,63.1014266317697));
#184223=CARTESIAN_POINT('Ctrl Pts',(127.352388534624,6.05554858354794,63.2101158813461));
#184224=CARTESIAN_POINT('Ctrl Pts',(127.615921914817,5.46871259357983,63.2539703214335));
#184225=CARTESIAN_POINT('Ctrl Pts',(128.093264497884,4.17553995924312,63.3307657133324));
#184226=CARTESIAN_POINT('Ctrl Pts',(128.293738852582,3.46619690256007,63.3610404174184));
#184227=CARTESIAN_POINT('Ctrl Pts',(128.673000277598,1.56923636877742,63.4120136903323));
#184228=CARTESIAN_POINT('Ctrl Pts',(128.757672525873,0.36863099498387,63.4148707438064));
#184229=CARTESIAN_POINT('Ctrl Pts',(128.639806890499,-1.72310636947871,
63.367256121098));
#184230=CARTESIAN_POINT('Ctrl Pts',(128.504352669513,-2.61119350013773,
63.3306392426059));
#184231=CARTESIAN_POINT('Ctrl Pts',(128.136508695066,-4.07342267385892,
63.2415897240375));
#184232=CARTESIAN_POINT('Ctrl Pts',(127.948721632206,-4.65644810255506,
63.1978490645046));
#184233=CARTESIAN_POINT('Ctrl Pts',(127.485560144224,-5.82663164171815,
63.0929549316484));
#184234=CARTESIAN_POINT('Ctrl Pts',(127.206225739339,-6.41058075592392,
63.0312083948543));
#184235=CARTESIAN_POINT('Ctrl Pts',(126.410934235089,-7.81401565086172,
62.8578407190614));
#184236=CARTESIAN_POINT('Ctrl Pts',(125.848656697341,-8.60208290761153,
62.7369504890977));
#184237=CARTESIAN_POINT('Ctrl Pts',(124.892306848933,-9.68288574856614,
62.5341475014423));
#184238=CARTESIAN_POINT('Ctrl Pts',(124.556191186077,-10.0249117786789,
62.4632588863853));
#184239=CARTESIAN_POINT('Ctrl Pts',(123.844304826822,-10.6772111200816,
62.3135416149205));
#184240=CARTESIAN_POINT('Ctrl Pts',(123.468460925162,-10.9863827970222,
62.2347035333859));
#184241=CARTESIAN_POINT('Ctrl Pts',(123.077309244396,-11.2745153368956,
62.1528629199185));
#184242=CARTESIAN_POINT('Ctrl Pts',(115.082307292334,-13.9,60.6760422812756));
#184243=CARTESIAN_POINT('Ctrl Pts',(115.616042419255,-13.9,60.7863377957508));
#184244=CARTESIAN_POINT('Ctrl Pts',(116.149634438892,-13.8679498804623,
60.8967905452979));
#184245=CARTESIAN_POINT('Ctrl Pts',(116.946936389828,-13.7717115486751,
61.061755407262));
#184246=CARTESIAN_POINT('Ctrl Pts',(117.212533291068,-13.7314886459556,
61.1166912867009));
#184247=CARTESIAN_POINT('Ctrl Pts',(118.058063530176,-13.5772256862302,
61.2913498752852));
#184248=CARTESIAN_POINT('Ctrl Pts',(118.63202293339,-13.4326778464348,61.4095142855781));
#184249=CARTESIAN_POINT('Ctrl Pts',(119.65540216623,-13.1015576008644,61.6206050814545));
#184250=CARTESIAN_POINT('Ctrl Pts',(120.107752768997,-12.9276543277861,
61.7140590829468));
#184251=CARTESIAN_POINT('Ctrl Pts',(121.112079230007,-12.4778568600849,
61.922240800819));
#184252=CARTESIAN_POINT('Ctrl Pts',(121.656709267083,-12.1876122794215,
62.0356533688479));
#184253=CARTESIAN_POINT('Ctrl Pts',(122.637702808448,-11.5752608259786,
62.2407023161625));
#184254=CARTESIAN_POINT('Ctrl Pts',(123.078203837442,-11.2623240489777,
62.3330930100192));
#184255=CARTESIAN_POINT('Ctrl Pts',(123.880316903993,-10.6175110244167,
62.5012349232633));
#184256=CARTESIAN_POINT('Ctrl Pts',(124.244876846336,-10.2908004521861,
62.5775759420006));
#184257=CARTESIAN_POINT('Ctrl Pts',(124.952272283699,-9.58500997890699,
62.7262780048108));
#184258=CARTESIAN_POINT('Ctrl Pts',(125.293078977684,-9.20488912953273,
62.7982419353592));
#184259=CARTESIAN_POINT('Ctrl Pts',(126.211888674503,-8.05785265431681,
62.9938494152688));
#184260=CARTESIAN_POINT('Ctrl Pts',(126.732937187918,-7.24745216020387,
63.1070284739973));
#184261=CARTESIAN_POINT('Ctrl Pts',(127.290192843733,-6.14485975785458,
63.2304683910818));
#184262=CARTESIAN_POINT('Ctrl Pts',(127.406144983826,-5.89773198881215,
63.2563162977466));
#184263=CARTESIAN_POINT('Ctrl Pts',(127.753979347159,-5.09636088709482,
63.3342323360609));
#184264=CARTESIAN_POINT('Ctrl Pts',(127.957747600777,-4.53011485428487,
63.3804385621099));
#184265=CARTESIAN_POINT('Ctrl Pts',(128.261382968012,-3.47927944773119,
63.4516246852519));
#184266=CARTESIAN_POINT('Ctrl Pts',(128.373194866698,-2.99932782019874,
63.4788843546972));
#184267=CARTESIAN_POINT('Ctrl Pts',(128.569617455717,-1.89790121626044,
63.5300247297703));
#184268=CARTESIAN_POINT('Ctrl Pts',(128.638435764157,-1.27455906081511,
63.55094843465));
#184269=CARTESIAN_POINT('Ctrl Pts',(128.689531621346,-0.101454672421391,
63.5752427187126));
#184270=CARTESIAN_POINT('Ctrl Pts',(128.68158699367,0.446648417759629,63.5804639802709));
#184271=CARTESIAN_POINT('Ctrl Pts',(128.606179419164,1.48672707588937,63.5780323923241));
#184272=CARTESIAN_POINT('Ctrl Pts',(128.544566093058,1.97829567180721,63.5715333723782));
#184273=CARTESIAN_POINT('Ctrl Pts',(128.366572414747,2.97249783873833,63.5481323985874));
#184274=CARTESIAN_POINT('Ctrl Pts',(128.24820971207,3.47400340878646,63.5308423597815));
#184275=CARTESIAN_POINT('Ctrl Pts',(127.829616911276,4.89484609785691,63.4664837943271));
#184276=CARTESIAN_POINT('Ctrl Pts',(127.462058360269,5.79061623110116,63.4069342778574));
#184277=CARTESIAN_POINT('Ctrl Pts',(126.877033908554,6.88125971934158,63.3083363147176));
#184278=CARTESIAN_POINT('Ctrl Pts',(126.740900778362,7.11814862389404,63.2851835530943));
#184279=CARTESIAN_POINT('Ctrl Pts',(126.283699321691,7.86248825818054,63.2066156482955));
#184280=CARTESIAN_POINT('Ctrl Pts',(125.937145253471,8.3528907924079,63.1458494828957));
#184281=CARTESIAN_POINT('Ctrl Pts',(125.252238119632,9.20011035830848,63.0248814256844));
#184282=CARTESIAN_POINT('Ctrl Pts',(124.924354826569,9.56439601985719,62.9666725938142));
#184283=CARTESIAN_POINT('Ctrl Pts',(124.138148244168,10.3496691989574,62.826808246281));
#184284=CARTESIAN_POINT('Ctrl Pts',(123.669443924711,10.7584001750359,62.7432475923838));
#184285=CARTESIAN_POINT('Ctrl Pts',(122.743379339098,11.4614950219372,62.5776001878554));
#184286=CARTESIAN_POINT('Ctrl Pts',(122.29285359685,11.7631683164195,62.4967919984508));
#184287=CARTESIAN_POINT('Ctrl Pts',(121.404162725771,12.2846322865785,62.3362733997077));
#184288=CARTESIAN_POINT('Ctrl Pts',(120.96960683995,12.5091320194283,62.2572813338858));
#184289=CARTESIAN_POINT('Ctrl Pts',(120.060775742327,12.9181750767093,62.0918192503852));
#184290=CARTESIAN_POINT('Ctrl Pts',(119.586306221414,13.1004134272832,62.0053087095122));
#184291=CARTESIAN_POINT('Ctrl Pts',(118.195315425746,13.5466241728586,61.7519341860998));
#184292=CARTESIAN_POINT('Ctrl Pts',(117.260151082802,13.7406847319864,61.5820527436966));
#184293=CARTESIAN_POINT('Ctrl Pts',(116.04439728924,13.861072793064,61.3608528118971));
#184294=CARTESIAN_POINT('Ctrl Pts',(115.775250170044,13.8795782638137,61.3118446162619));
#184295=CARTESIAN_POINT('Ctrl Pts',(114.913034024137,13.9128676342894,61.1545495648881));
#184296=CARTESIAN_POINT('Ctrl Pts',(114.319565819352,13.8965307205244,61.0457880281624));
#184297=CARTESIAN_POINT('Ctrl Pts',(113.245906885706,13.7957133502246,60.8492540105891));
#184298=CARTESIAN_POINT('Ctrl Pts',(112.765518849037,13.7242469493173,60.7614011010939));
#184299=CARTESIAN_POINT('Ctrl Pts',(111.685322670308,13.503367218759,60.5643911481585));
#184300=CARTESIAN_POINT('Ctrl Pts',(111.089648626595,13.3383375189148,60.4561504802148));
#184301=CARTESIAN_POINT('Ctrl Pts',(109.99776166544,12.9536271210321,60.2582703242228));
#184302=CARTESIAN_POINT('Ctrl Pts',(109.499440057304,12.7438116788286,60.1681709780323));
#184303=CARTESIAN_POINT('Ctrl Pts',(108.576410199111,12.2885127699548,60.0009762219196));
#184304=CARTESIAN_POINT('Ctrl Pts',(108.149895260732,12.0487187087438,59.9235464531746));
#184305=CARTESIAN_POINT('Ctrl Pts',(107.306974834155,11.5132291035049,59.770895615366));
#184306=CARTESIAN_POINT('Ctrl Pts',(106.892338827584,11.2160690548295,59.6960157522552));
#184307=CARTESIAN_POINT('Ctrl Pts',(105.748255525778,10.2955095149837,59.490636811986));
#184308=CARTESIAN_POINT('Ctrl Pts',(105.065145034467,9.61726589596268,59.3697513499223));
#184309=CARTESIAN_POINT('Ctrl Pts',(104.284373986162,8.66154336740987,59.2331048386539));
#184310=CARTESIAN_POINT('Ctrl Pts',(104.118177886365,8.44542689187018,59.2041080132545));
#184311=CARTESIAN_POINT('Ctrl Pts',(103.606088880832,7.7373363137978,59.1148865726734));
#184312=CARTESIAN_POINT('Ctrl Pts',(103.285444400724,7.22741273759473,59.0591706368313));
#184313=CARTESIAN_POINT('Ctrl Pts',(102.764153800281,6.26596019965551,58.9700200913392));
#184314=CARTESIAN_POINT('Ctrl Pts',(102.552653497572,5.8216494695253,58.9344326041966));
#184315=CARTESIAN_POINT('Ctrl Pts',(102.123916224237,4.78411018662792,58.8641116583317));
#184316=CARTESIAN_POINT('Ctrl Pts',(101.922322452508,4.18538019375447,58.8325372374376));
#184317=CARTESIAN_POINT('Ctrl Pts',(101.623149665034,3.05050736773772,58.7887482353137));
#184318=CARTESIAN_POINT('Ctrl Pts',(101.515164850384,2.51842728831526,58.7744579515986));
#184319=CARTESIAN_POINT('Ctrl Pts',(101.368885248289,1.49967186218422,58.7580890921657));
#184320=CARTESIAN_POINT('Ctrl Pts',(101.324659557079,1.01467517101568,58.7548810859808));
#184321=CARTESIAN_POINT('Ctrl Pts',(101.285112281498,0.0114122663443761,
58.7583228663086));
#184322=CARTESIAN_POINT('Ctrl Pts',(101.293079029211,-0.506241660897844,
58.7656095365548));
#184323=CARTESIAN_POINT('Ctrl Pts',(101.398004428674,-2.00028658790661,
58.8031822068209));
#184324=CARTESIAN_POINT('Ctrl Pts',(101.567963780223,-2.96801928523241,
58.8482895099458));
#184325=CARTESIAN_POINT('Ctrl Pts',(101.910574633612,-4.16888091616166,
58.9301184296819));
#184326=CARTESIAN_POINT('Ctrl Pts',(101.992103359967,-4.42630460544285,
58.9492298026959));
#184327=CARTESIAN_POINT('Ctrl Pts',(102.255238441565,-5.18079723970398,
59.0097829781108));
#184328=CARTESIAN_POINT('Ctrl Pts',(102.457520147463,-5.66982859382182,
59.0549538480031));
#184329=CARTESIAN_POINT('Ctrl Pts',(102.90556751856,-6.6002090175857,59.1535439611523));
#184330=CARTESIAN_POINT('Ctrl Pts',(103.148609140187,-7.04201895481002,
59.2064251158288));
#184331=CARTESIAN_POINT('Ctrl Pts',(103.887615213688,-8.22840482019988,
59.3662531375783));
#184332=CARTESIAN_POINT('Ctrl Pts',(104.431623533809,-8.93876189614676,
59.483025537428));
#184333=CARTESIAN_POINT('Ctrl Pts',(105.237619187511,-9.80311033484269,
59.6542754953128));
#184334=CARTESIAN_POINT('Ctrl Pts',(105.442623035857,-10.0094114411752,
59.6976895506399));
#184335=CARTESIAN_POINT('Ctrl Pts',(106.117163864108,-10.6463276054636,
59.8398879420105));
#184336=CARTESIAN_POINT('Ctrl Pts',(106.609823911186,-11.0502853987451,
59.9426924543749));
#184337=CARTESIAN_POINT('Ctrl Pts',(107.523221854039,-11.6979896699392,
60.1328517011599));
#184338=CARTESIAN_POINT('Ctrl Pts',(107.932543165812,-11.9565322526303,
60.2179289757807));
#184339=CARTESIAN_POINT('Ctrl Pts',(108.967397295296,-12.5351469137784,
60.4330520455173));
#184340=CARTESIAN_POINT('Ctrl Pts',(109.605317936245,-12.8291602920116,
60.5657223077177));
#184341=CARTESIAN_POINT('Ctrl Pts',(110.724017809939,-13.2422308406029,
60.7980531082487));
#184342=CARTESIAN_POINT('Ctrl Pts',(111.194200639975,-13.3870156589866,
60.8955857317533));
#184343=CARTESIAN_POINT('Ctrl Pts',(111.932428159116,-13.570514401821,61.0480714609832));
#184344=CARTESIAN_POINT('Ctrl Pts',(112.195614063017,-13.6275518090732,
61.1023215125712));
#184345=CARTESIAN_POINT('Ctrl Pts',(113.26277014282,-13.8252777392009,61.3221063681588));
#184346=CARTESIAN_POINT('Ctrl Pts',(114.076510955031,-13.9,61.4893881436234));
#184347=CARTESIAN_POINT('Ctrl Pts',(114.891525389284,-13.9,61.6575251889163));
#184348=CARTESIAN_POINT('Origin',(114.885904346743,1.45439216225896E-14,
61.6864428015861));
#184349=CARTESIAN_POINT('',(115.190201331893,-11.58843628952,60.1209783366866));
#184350=CARTESIAN_POINT('',(115.190201331893,11.5884362895886,60.1209783366842));
#184351=CARTESIAN_POINT('Origin',(115.190201331893,1.45439216225896E-14,
60.1209783366866));
#184352=CARTESIAN_POINT('',(114.581607361595,11.6998171366511,63.251907266478));
#184353=CARTESIAN_POINT('',(114.885904346743,11.64412671312,61.6864428015861));
#184354=CARTESIAN_POINT('Origin',(114.581607361595,1.45439216225896E-14,
63.2519072664759));
#184355=CARTESIAN_POINT('Origin',(115.190201331893,1.45439216225896E-14,
60.1209783366866));
#184356=CARTESIAN_POINT('Origin',(115.185539912945,1.45439216225896E-14,
60.1449591385841));
#184357=CARTESIAN_POINT('',(115.27674466279,-11.40026076189,59.6757537179573));
#184358=CARTESIAN_POINT('Origin',(115.185539912945,-10.88886271061,60.1449591385841));
#184359=CARTESIAN_POINT('Origin',(115.27674466279,1.45439216225896E-14,
59.6757537179573));
#184360=CARTESIAN_POINT('Origin',(115.446124912502,1.45439216225896E-14,
58.8043722225089));
#184361=CARTESIAN_POINT('',(115.446124912502,-11.05,58.8043722225089));
#184362=CARTESIAN_POINT('Origin',(115.446124912502,-12.35,58.8043722225089));
#184363=CARTESIAN_POINT('Origin',(115.446124912502,1.45439216225896E-14,
58.8043722225089));
#184364=CARTESIAN_POINT('Origin',(120.341492634982,15.3,58.5138990734244));
#184365=CARTESIAN_POINT('',(120.484600069656,-9.97697348898956,57.7776788196001));
#184366=CARTESIAN_POINT('',(120.198385200308,-9.97697348898956,59.2501193272487));
#184367=CARTESIAN_POINT('Ctrl Pts',(120.198385200308,-9.97697348898973,
59.2501193272487));
#184368=CARTESIAN_POINT('Ctrl Pts',(120.292749480214,-9.93120612242623,
59.2684619766829));
#184369=CARTESIAN_POINT('Ctrl Pts',(120.396910139201,-9.88061692723551,
59.268852030833));
#184370=CARTESIAN_POINT('Ctrl Pts',(120.597619254378,-9.7837357700295,59.2262362233364));
#184371=CARTESIAN_POINT('Ctrl Pts',(120.694200988075,-9.73750614463925,
59.1832454067965));
#184372=CARTESIAN_POINT('Ctrl Pts',(120.847180488313,-9.66686754951251,
59.0747124853458));
#184373=CARTESIAN_POINT('Ctrl Pts',(120.916107916634,-9.63634449458131,
59.0055914641224));
#184374=CARTESIAN_POINT('Ctrl Pts',(121.022448949448,-9.59481532313076,
58.842901490205));
#184375=CARTESIAN_POINT('Ctrl Pts',(121.059784384477,-9.58397099327854,
58.7492402067744));
#184376=CARTESIAN_POINT('Ctrl Pts',(121.095641393136,-9.58397099327854,
58.5647728094222));
#184377=CARTESIAN_POINT('Ctrl Pts',(121.09611090338,-9.59481532313077,58.4639454803748));
#184378=CARTESIAN_POINT('Ctrl Pts',(121.058458308044,-9.63634449458134,
58.2732658408284));
#184379=CARTESIAN_POINT('Ctrl Pts',(121.020443267736,-9.6668675495125,58.1833572057576));
#184380=CARTESIAN_POINT('Ctrl Pts',(120.91926058826,-9.73750614463925,58.0254199147028));
#184381=CARTESIAN_POINT('Ctrl Pts',(120.845816349612,-9.78373577002951,
57.9493792321698));
#184382=CARTESIAN_POINT('Ctrl Pts',(120.675686475446,-9.88061692723553,
57.8346792675662));
#184383=CARTESIAN_POINT('Ctrl Pts',(120.578964349562,-9.93120612242623,
57.7960214690343));
#184384=CARTESIAN_POINT('Ctrl Pts',(120.484600069656,-9.97697348898973,
57.7776788196001));
#184385=CARTESIAN_POINT('',(120.484600069656,-10.3082491238812,57.7776788196002));
#184386=CARTESIAN_POINT('',(120.484600069656,-9.97697348898999,57.7776788196002));
#184387=CARTESIAN_POINT('',(120.198385200308,-10.3082491238812,59.2501193272487));
#184388=CARTESIAN_POINT('Ctrl Pts',(120.484600069656,-10.3082491238815,
57.7776788196001));
#184389=CARTESIAN_POINT('Ctrl Pts',(120.578839835416,-10.2640110301723,
57.7959972658154));
#184390=CARTESIAN_POINT('Ctrl Pts',(120.675458711172,-10.2151256546928,
57.8345897929314));
#184391=CARTESIAN_POINT('Ctrl Pts',(120.845400127855,-10.1215699520295,
57.9490347799076));
#184392=CARTESIAN_POINT('Ctrl Pts',(120.918755915055,-10.076961159343,58.0248881638909));
#184393=CARTESIAN_POINT('Ctrl Pts',(121.020177899851,-10.008616368515,58.1827179406788));
#184394=CARTESIAN_POINT('Ctrl Pts',(121.058344974172,-9.97903582116519,
58.2728599212221));
#184395=CARTESIAN_POINT('Ctrl Pts',(121.096127121178,-9.93883620340095,
58.4638600184146));
#184396=CARTESIAN_POINT('Ctrl Pts',(121.095641986383,-9.92836844602397,
58.5647697574433));
#184397=CARTESIAN_POINT('Ctrl Pts',(121.059783791229,-9.92836844602397,
58.7492432587533));
#184398=CARTESIAN_POINT('Ctrl Pts',(121.022431971555,-9.93883620340095,
58.8429868044173));
#184399=CARTESIAN_POINT('Ctrl Pts',(120.915850774513,-9.97903582116519,
59.0059253701314));
#184400=CARTESIAN_POINT('Ctrl Pts',(120.846694969659,-10.008616368515,59.0752057921387));
#184401=CARTESIAN_POINT('Ctrl Pts',(120.6935338653,-10.076961159343,59.1835493824068));
#184402=CARTESIAN_POINT('Ctrl Pts',(120.597104305892,-10.1215699520295,
59.2263996735356));
#184403=CARTESIAN_POINT('Ctrl Pts',(120.39666544206,-10.2151256546928,59.2688496678139));
#184404=CARTESIAN_POINT('Ctrl Pts',(120.292624966069,-10.2640110301723,
59.2684377734639));
#184405=CARTESIAN_POINT('Ctrl Pts',(120.198385200308,-10.3082491238815,
59.2501193272487));
#184406=CARTESIAN_POINT('',(120.198385200308,-9.97697348898999,59.2501193272487));
#184407=CARTESIAN_POINT('Origin',(120.341492634982,15.3,58.5138990734244));
#184408=CARTESIAN_POINT('',(120.484600069656,10.3082491238813,57.7776788196002));
#184409=CARTESIAN_POINT('',(120.198385200308,10.3082491238812,59.2501193272487));
#184410=CARTESIAN_POINT('Ctrl Pts',(120.198385200308,10.3082491238815,59.2501193272487));
#184411=CARTESIAN_POINT('Ctrl Pts',(120.292624966069,10.2640110301723,59.2684377734639));
#184412=CARTESIAN_POINT('Ctrl Pts',(120.39666544206,10.2151256546929,59.2688496678139));
#184413=CARTESIAN_POINT('Ctrl Pts',(120.597104305892,10.1215699520295,59.2263996735356));
#184414=CARTESIAN_POINT('Ctrl Pts',(120.6935338653,10.076961159343,59.1835493824068));
#184415=CARTESIAN_POINT('Ctrl Pts',(120.846694969659,10.008616368515,59.0752057921387));
#184416=CARTESIAN_POINT('Ctrl Pts',(120.915850774513,9.97903582116521,59.0059253701314));
#184417=CARTESIAN_POINT('Ctrl Pts',(121.022431971555,9.93883620340097,58.8429868044173));
#184418=CARTESIAN_POINT('Ctrl Pts',(121.059783791229,9.928368446024,58.7492432587533));
#184419=CARTESIAN_POINT('Ctrl Pts',(121.095641986383,9.928368446024,58.5647697574433));
#184420=CARTESIAN_POINT('Ctrl Pts',(121.096127121178,9.93883620340099,58.4638600184146));
#184421=CARTESIAN_POINT('Ctrl Pts',(121.058344974172,9.97903582116522,58.2728599212221));
#184422=CARTESIAN_POINT('Ctrl Pts',(121.020177899851,10.008616368515,58.1827179406788));
#184423=CARTESIAN_POINT('Ctrl Pts',(120.918755915055,10.076961159343,58.0248881638909));
#184424=CARTESIAN_POINT('Ctrl Pts',(120.845400127855,10.1215699520295,57.9490347799076));
#184425=CARTESIAN_POINT('Ctrl Pts',(120.675458711172,10.2151256546929,57.8345897929314));
#184426=CARTESIAN_POINT('Ctrl Pts',(120.578839835416,10.2640110301723,57.7959972658154));
#184427=CARTESIAN_POINT('Ctrl Pts',(120.484600069656,10.3082491238815,57.7776788196001));
#184428=CARTESIAN_POINT('',(120.484600069656,9.97697348898955,57.7776788196002));
#184429=CARTESIAN_POINT('',(120.484600069656,10.30824912388,57.7776788196002));
#184430=CARTESIAN_POINT('',(120.198385200308,9.97697348898959,59.2501193272487));
#184431=CARTESIAN_POINT('Ctrl Pts',(120.484600069656,9.97697348898976,57.7776788196002));
#184432=CARTESIAN_POINT('Ctrl Pts',(120.576159926688,9.93256628805063,57.7954763417287));
#184433=CARTESIAN_POINT('Ctrl Pts',(120.670285760103,9.88345309913906,57.8324795460311));
#184434=CARTESIAN_POINT('Ctrl Pts',(120.836868483474,9.78905064146605,57.9420247394531));
#184435=CARTESIAN_POINT('Ctrl Pts',(120.909354963944,9.74381820661306,58.01457069919));
#184436=CARTESIAN_POINT('Ctrl Pts',(121.013972591701,9.67185393609447,58.1696730234398));
#184437=CARTESIAN_POINT('Ctrl Pts',(121.054855180413,9.63958427480582,58.2616338615531));
#184438=CARTESIAN_POINT('Ctrl Pts',(121.096047489807,9.59555522790789,58.4575893251544));
#184439=CARTESIAN_POINT('Ctrl Pts',(121.096249195621,9.58397099327857,58.5616459523084));
#184440=CARTESIAN_POINT('Ctrl Pts',(121.059784384477,9.58397099327857,58.7492402067744));
#184441=CARTESIAN_POINT('Ctrl Pts',(121.022448949448,9.59481532313079,58.842901490205));
#184442=CARTESIAN_POINT('Ctrl Pts',(120.916107916634,9.63634449458134,59.0055914641224));
#184443=CARTESIAN_POINT('Ctrl Pts',(120.847180488313,9.66686754951253,59.0747124853458));
#184444=CARTESIAN_POINT('Ctrl Pts',(120.694200988075,9.73750614463928,59.1832454067965));
#184445=CARTESIAN_POINT('Ctrl Pts',(120.597619254378,9.78373577002953,59.2262362233364));
#184446=CARTESIAN_POINT('Ctrl Pts',(120.396910139201,9.88061692723554,59.268852030833));
#184447=CARTESIAN_POINT('Ctrl Pts',(120.292749480214,9.93120612242626,59.2684619766829));
#184448=CARTESIAN_POINT('Ctrl Pts',(120.198385200308,9.97697348898976,59.2501193272487));
#184449=CARTESIAN_POINT('',(120.198385200308,10.30824912388,59.2501193272487));
#184450=CARTESIAN_POINT('Origin',(113.780205727422,1.45439216225896E-14,
67.3747406878918));
#184451=CARTESIAN_POINT('',(115.535656926088,-11.05,58.3437722409808));
#184452=CARTESIAN_POINT('',(113.780205727422,-11.05,67.3747406878918));
#184453=CARTESIAN_POINT('',(110.872928651868,-9.97697348898956,57.4374251547129));
#184454=CARTESIAN_POINT('Origin',(115.535656926088,1.45439216225896E-14,
58.3437722409808));
#184455=CARTESIAN_POINT('',(111.159143521215,-9.97697348898956,55.9649846470644));
#184456=CARTESIAN_POINT('Ctrl Pts',(110.872928651867,-9.97697348898916,
57.4374251547129));
#184457=CARTESIAN_POINT('Ctrl Pts',(110.778564371961,-9.93120612242566,
57.4190825052788));
#184458=CARTESIAN_POINT('Ctrl Pts',(110.681842246077,-9.88061692723491,
57.3804247067468));
#184459=CARTESIAN_POINT('Ctrl Pts',(110.511712371911,-9.78373577002886,
57.2657247421432));
#184460=CARTESIAN_POINT('Ctrl Pts',(110.438268133263,-9.7375061446386,57.1896840596102));
#184461=CARTESIAN_POINT('Ctrl Pts',(110.337085453787,-9.66686754951184,
57.0317467685554));
#184462=CARTESIAN_POINT('Ctrl Pts',(110.299070413479,-9.63634449458064,
56.9418381334846));
#184463=CARTESIAN_POINT('Ctrl Pts',(110.261417818143,-9.59481532313007,
56.7511584939382));
#184464=CARTESIAN_POINT('Ctrl Pts',(110.261887328387,-9.58397099327785,
56.6503311648909));
#184465=CARTESIAN_POINT('Ctrl Pts',(110.279815832717,-9.58397099327785,
56.5580974662147));
#184466=CARTESIAN_POINT('Ctrl Pts',(110.297744337046,-9.58397099327785,
56.4658637675386));
#184467=CARTESIAN_POINT('Ctrl Pts',(110.335079772075,-9.59481532313008,
56.372202484108));
#184468=CARTESIAN_POINT('Ctrl Pts',(110.441420804889,-9.63634449458065,
56.2095125101906));
#184469=CARTESIAN_POINT('Ctrl Pts',(110.51034823321,-9.66686754951184,56.1403914889672));
#184470=CARTESIAN_POINT('Ctrl Pts',(110.663327733448,-9.7375061446386,56.0318585675165));
#184471=CARTESIAN_POINT('Ctrl Pts',(110.759909467145,-9.78373577002887,
55.9888677509767));
#184472=CARTESIAN_POINT('Ctrl Pts',(110.960618582322,-9.88061692723491,
55.94625194348));
#184473=CARTESIAN_POINT('Ctrl Pts',(111.064779241308,-9.93120612242564,
55.9466419976302));
#184474=CARTESIAN_POINT('Ctrl Pts',(111.159143521215,-9.97697348898915,
55.9649846470643));
#184475=CARTESIAN_POINT('',(115.821871795436,-11.05,56.8713317333323));
#184476=CARTESIAN_POINT('Origin',(115.821871795436,1.45439216225896E-14,
56.8713317333323));
#184477=CARTESIAN_POINT('',(117.329270107334,-11.05,49.11647839305));
#184478=CARTESIAN_POINT('',(113.780205727422,-11.05,67.3747406878918));
#184479=CARTESIAN_POINT('Origin',(117.329270107334,1.45439216225896E-14,
49.11647839305));
#184480=CARTESIAN_POINT('Origin',(115.821871795436,1.45439216225896E-14,
56.8713317333323));
#184481=CARTESIAN_POINT('Origin',(115.535656926088,1.45439216225896E-14,
58.3437722409808));
#184482=CARTESIAN_POINT('',(106.028205189487,-4.7499999999999,54.9676262909075));
#184483=CARTESIAN_POINT('',(106.028205189487,4.74999999999992,54.9676262909075));
#184484=CARTESIAN_POINT('Origin',(115.821871795436,1.45439216225896E-14,
56.8713317333323));
#184485=CARTESIAN_POINT('',(105.741990320139,-4.7499999999999,56.440066798556));
#184486=CARTESIAN_POINT('Ctrl Pts',(106.028205189487,-4.75,54.9676262909075));
#184487=CARTESIAN_POINT('Ctrl Pts',(106.073131672458,-4.84613048481368,
54.9763591581351));
#184488=CARTESIAN_POINT('Ctrl Pts',(106.119072126072,-4.94845182674208,
55.0051459502539));
#184489=CARTESIAN_POINT('Ctrl Pts',(106.198883665765,-5.13734179585313,
55.102289721472));
#184490=CARTESIAN_POINT('Ctrl Pts',(106.232695166959,-5.22394595989023,
55.1706265418024));
#184491=CARTESIAN_POINT('Ctrl Pts',(106.276137509157,-5.35340561126171,
55.3173401922386));
#184492=CARTESIAN_POINT('Ctrl Pts',(106.290643570149,-5.40787766025428,
55.4026791218385));
#184493=CARTESIAN_POINT('Ctrl Pts',(106.297065507605,-5.48122203006144,
55.5872881061577));
#184494=CARTESIAN_POINT('Ctrl Pts',(106.288808122004,-5.5,55.6866016180312));
#184495=CARTESIAN_POINT('Ctrl Pts',(106.25234331086,-5.5,55.8741958724972));
#184496=CARTESIAN_POINT('Ctrl Pts',(106.221489017615,-5.47994696416173,
55.972215794829));
#184497=CARTESIAN_POINT('Ctrl Pts',(106.143065389029,-5.4021212359169,56.144920159399));
#184498=CARTESIAN_POINT('Ctrl Pts',(106.095652440797,-5.34444274328869,
56.219717998098));
#184499=CARTESIAN_POINT('Ctrl Pts',(105.999768021207,-5.21215219369169,
56.3358464779124));
#184500=CARTESIAN_POINT('Ctrl Pts',(105.94441759979,-5.12715501869964,56.383543337138));
#184501=CARTESIAN_POINT('Ctrl Pts',(105.837296341422,-4.94273061003997,
56.4398856004814));
#184502=CARTESIAN_POINT('Ctrl Pts',(105.785581627802,-4.84327357189262,
56.4485401326993));
#184503=CARTESIAN_POINT('Ctrl Pts',(105.741990320139,-4.75,56.440066798556));
#184504=CARTESIAN_POINT('',(105.741990320139,4.74999999999992,56.440066798556));
#184505=CARTESIAN_POINT('Origin',(115.535656926088,1.45439216225896E-14,
58.3437722409808));
#184506=CARTESIAN_POINT('Ctrl Pts',(105.741990320139,4.75,56.440066798556));
#184507=CARTESIAN_POINT('Ctrl Pts',(105.78691680311,4.84613048481368,56.4487996657836));
#184508=CARTESIAN_POINT('Ctrl Pts',(105.840295789827,4.94845182674209,56.4393187135207));
#184509=CARTESIAN_POINT('Ctrl Pts',(105.950686570531,5.13734179585313,56.3791467126385));
#184510=CARTESIAN_POINT('Ctrl Pts',(106.007635566774,5.22394595989023,56.3284520338962));
#184511=CARTESIAN_POINT('Ctrl Pts',(106.102874729734,5.35340561126171,56.2086954718268));
#184512=CARTESIAN_POINT('Ctrl Pts',(106.148293178739,5.40787766025429,56.1350047451325));
#184513=CARTESIAN_POINT('Ctrl Pts',(106.223403553673,5.48122203006144,55.9662441159878));
#184514=CARTESIAN_POINT('Ctrl Pts',(106.252951113345,5.5,55.8710690153834));
#184515=CARTESIAN_POINT('Ctrl Pts',(106.270879617674,5.5,55.7788353167073));
#184516=CARTESIAN_POINT('Ctrl Pts',(106.288808122004,5.5,55.6866016180312));
#184517=CARTESIAN_POINT('Ctrl Pts',(106.297065507605,5.48122203006144,55.5872881061577));
#184518=CARTESIAN_POINT('Ctrl Pts',(106.290643570149,5.40787766025429,55.4026791218385));
#184519=CARTESIAN_POINT('Ctrl Pts',(106.276137509157,5.35340561126171,55.3173401922386));
#184520=CARTESIAN_POINT('Ctrl Pts',(106.232695166959,5.22394595989023,55.1706265418024));
#184521=CARTESIAN_POINT('Ctrl Pts',(106.198883665765,5.13734179585313,55.102289721472));
#184522=CARTESIAN_POINT('Ctrl Pts',(106.119072126072,4.94845182674209,55.0051459502538));
#184523=CARTESIAN_POINT('Ctrl Pts',(106.073131672458,4.84613048481368,54.9763591581351));
#184524=CARTESIAN_POINT('Ctrl Pts',(106.028205189487,4.75,54.9676262909075));
#184525=CARTESIAN_POINT('',(125.329323532037,4.74999999999993,60.2474776834056));
#184526=CARTESIAN_POINT('',(125.329323532037,-4.7499999999999,60.2474776834056));
#184527=CARTESIAN_POINT('Origin',(115.535656926088,1.45439216225896E-14,
58.3437722409808));
#184528=CARTESIAN_POINT('',(125.615538401385,-4.7499999999999,58.775037175757));
#184529=CARTESIAN_POINT('Ctrl Pts',(125.329323532037,-4.75,60.2474776834055));
#184530=CARTESIAN_POINT('Ctrl Pts',(125.285732224375,-4.84327357189262,
60.2390043492623));
#184531=CARTESIAN_POINT('Ctrl Pts',(125.24102527291,-4.94273061003997,60.2116072504476));
#184532=CARTESIAN_POINT('Ctrl Pts',(125.162810527679,-5.12715501869964,
60.1192391376523));
#184533=CARTESIAN_POINT('Ctrl Pts',(125.129358189981,-5.21215219369169,
60.0542806845177));
#184534=CARTESIAN_POINT('Ctrl Pts',(125.083958466883,-5.34444274328869,
59.9106892123244));
#184535=CARTESIAN_POINT('Ctrl Pts',(125.068017873183,-5.4021212359169,59.8235766311058));
#184536=CARTESIAN_POINT('Ctrl Pts',(125.060001298882,-5.47994696416173,
59.6340699093286));
#184537=CARTESIAN_POINT('Ctrl Pts',(125.068112797035,-5.5,59.5316292133956));
#184538=CARTESIAN_POINT('Ctrl Pts',(125.104577608179,-5.5,59.3440349589296));
#184539=CARTESIAN_POINT('Ctrl Pts',(125.134125167851,-5.48122203006144,
59.2488598583252));
#184540=CARTESIAN_POINT('Ctrl Pts',(125.209235542785,-5.40787766025429,
59.0800992291805));
#184541=CARTESIAN_POINT('Ctrl Pts',(125.25465399179,-5.35340561126171,59.0064085024862));
#184542=CARTESIAN_POINT('Ctrl Pts',(125.34989315475,-5.22394595989023,58.8866519404169));
#184543=CARTESIAN_POINT('Ctrl Pts',(125.406842150993,-5.13734179585313,
58.8359572616745));
#184544=CARTESIAN_POINT('Ctrl Pts',(125.517232931697,-4.94845182674209,
58.7757852607923));
#184545=CARTESIAN_POINT('Ctrl Pts',(125.570611918414,-4.84613048481368,
58.7663043085294));
#184546=CARTESIAN_POINT('Ctrl Pts',(125.615538401385,-4.75,58.775037175757));
#184547=CARTESIAN_POINT('',(125.615538401385,4.74999999999992,58.775037175757));
#184548=CARTESIAN_POINT('Origin',(115.821871795436,1.45439216225896E-14,
56.8713317333323));
#184549=CARTESIAN_POINT('Ctrl Pts',(125.615538401385,4.75,58.775037175757));
#184550=CARTESIAN_POINT('Ctrl Pts',(125.570611918414,4.84613048481368,58.7663043085294));
#184551=CARTESIAN_POINT('Ctrl Pts',(125.517232931697,4.94845182674209,58.7757852607923));
#184552=CARTESIAN_POINT('Ctrl Pts',(125.406842150993,5.13734179585314,58.8359572616745));
#184553=CARTESIAN_POINT('Ctrl Pts',(125.34989315475,5.22394595989023,58.8866519404169));
#184554=CARTESIAN_POINT('Ctrl Pts',(125.25465399179,5.35340561126171,59.0064085024862));
#184555=CARTESIAN_POINT('Ctrl Pts',(125.209235542785,5.40787766025429,59.0800992291805));
#184556=CARTESIAN_POINT('Ctrl Pts',(125.134125167851,5.48122203006144,59.2488598583252));
#184557=CARTESIAN_POINT('Ctrl Pts',(125.104577608179,5.5,59.3440349589296));
#184558=CARTESIAN_POINT('Ctrl Pts',(125.08664910385,5.5,59.4362686576057));
#184559=CARTESIAN_POINT('Ctrl Pts',(125.06872059952,5.5,59.5285023562819));
#184560=CARTESIAN_POINT('Ctrl Pts',(125.060463213919,5.48122203006144,59.6278158681553));
#184561=CARTESIAN_POINT('Ctrl Pts',(125.066885151375,5.40787766025429,59.8124248524745));
#184562=CARTESIAN_POINT('Ctrl Pts',(125.081391212367,5.35340561126171,59.8977637820744));
#184563=CARTESIAN_POINT('Ctrl Pts',(125.124833554565,5.22394595989023,60.0444774325106));
#184564=CARTESIAN_POINT('Ctrl Pts',(125.158645055759,5.13734179585314,60.112814252841));
#184565=CARTESIAN_POINT('Ctrl Pts',(125.238456595452,4.94845182674209,60.2099580240592));
#184566=CARTESIAN_POINT('Ctrl Pts',(125.284397049066,4.84613048481368,60.238744816178));
#184567=CARTESIAN_POINT('Ctrl Pts',(125.329323532037,4.75,60.2474776834055));
#184568=CARTESIAN_POINT('',(111.159143521215,9.97697348898959,55.9649846470644));
#184569=CARTESIAN_POINT('Origin',(115.821871795436,1.45439216225896E-14,
56.8713317333323));
#184570=CARTESIAN_POINT('',(110.872928651868,9.97697348898959,57.4374251547129));
#184571=CARTESIAN_POINT('Ctrl Pts',(111.159143521215,9.97697348898918,55.9649846470643));
#184572=CARTESIAN_POINT('Ctrl Pts',(111.064779241308,9.93120612242567,55.9466419976301));
#184573=CARTESIAN_POINT('Ctrl Pts',(110.960618582322,9.88061692723494,55.94625194348));
#184574=CARTESIAN_POINT('Ctrl Pts',(110.759909467145,9.7837357700289,55.9888677509767));
#184575=CARTESIAN_POINT('Ctrl Pts',(110.663327733448,9.73750614463863,56.0318585675165));
#184576=CARTESIAN_POINT('Ctrl Pts',(110.51034823321,9.66686754951186,56.1403914889672));
#184577=CARTESIAN_POINT('Ctrl Pts',(110.441420804889,9.63634449458068,56.2095125101906));
#184578=CARTESIAN_POINT('Ctrl Pts',(110.335079772075,9.59481532313011,56.372202484108));
#184579=CARTESIAN_POINT('Ctrl Pts',(110.297744337046,9.58397099327788,56.4658637675386));
#184580=CARTESIAN_POINT('Ctrl Pts',(110.279815832717,9.58397099327788,56.5580974662147));
#184581=CARTESIAN_POINT('Ctrl Pts',(110.261887328387,9.58397099327788,56.6503311648909));
#184582=CARTESIAN_POINT('Ctrl Pts',(110.261417818143,9.5948153231301,56.7511584939382));
#184583=CARTESIAN_POINT('Ctrl Pts',(110.299070413479,9.63634449458067,56.9418381334846));
#184584=CARTESIAN_POINT('Ctrl Pts',(110.337085453787,9.66686754951186,57.0317467685554));
#184585=CARTESIAN_POINT('Ctrl Pts',(110.438268133263,9.73750614463863,57.1896840596102));
#184586=CARTESIAN_POINT('Ctrl Pts',(110.511712371911,9.78373577002889,57.2657247421432));
#184587=CARTESIAN_POINT('Ctrl Pts',(110.681842246077,9.88061692723494,57.3804247067468));
#184588=CARTESIAN_POINT('Ctrl Pts',(110.778564371961,9.93120612242567,57.4190825052787));
#184589=CARTESIAN_POINT('Ctrl Pts',(110.872928651867,9.97697348898919,57.4374251547129));
#184590=CARTESIAN_POINT('Origin',(115.535656926088,1.45439216225896E-14,
58.3437722409808));
#184591=CARTESIAN_POINT('Origin',(130.697657538777,-4.75,60.5269436545036));
#184592=CARTESIAN_POINT('',(125.940727510726,-4.75000000000024,58.8382478507961));
#184593=CARTESIAN_POINT('',(125.654512641378,-4.75000000000024,60.3106883584446));
#184594=CARTESIAN_POINT('Ctrl Pts',(125.654512641378,-4.75,60.3106883584446));
#184595=CARTESIAN_POINT('Ctrl Pts',(125.61230630101,-4.84330877665233,60.3024842360155));
#184596=CARTESIAN_POINT('Ctrl Pts',(125.569148299058,-4.94281444512932,
60.2753683060694));
#184597=CARTESIAN_POINT('Ctrl Pts',(125.493987021831,-5.12726283579728,
60.1835533615843));
#184598=CARTESIAN_POINT('Ctrl Pts',(125.462039039804,-5.21223335422367,
60.1188649340508));
#184599=CARTESIAN_POINT('Ctrl Pts',(125.419010017904,-5.34458926875733,
59.9756676934244));
#184600=CARTESIAN_POINT('Ctrl Pts',(125.404170373857,-5.40227743227456,
59.8886474008104));
#184601=CARTESIAN_POINT('Ctrl Pts',(125.397688170697,-5.4800270257108,59.6994100150999));
#184602=CARTESIAN_POINT('Ctrl Pts',(125.406220154262,-5.5,59.597150653446));
#184603=CARTESIAN_POINT('Ctrl Pts',(125.442648041529,-5.5,59.4097463549116));
#184604=CARTESIAN_POINT('Ctrl Pts',(125.471841952088,-5.4812216429014,59.3144170644385));
#184605=CARTESIAN_POINT('Ctrl Pts',(125.545702507498,-5.40768895518066,
59.1451182185494));
#184606=CARTESIAN_POINT('Ctrl Pts',(125.590233936868,-5.35302314086569,
59.0710512789374));
#184607=CARTESIAN_POINT('Ctrl Pts',(125.683192588985,-5.22334909571738,
58.9510054589944));
#184608=CARTESIAN_POINT('Ctrl Pts',(125.738518670655,-5.13686749643077,
58.9001654212853));
#184609=CARTESIAN_POINT('Ctrl Pts',(125.845604198444,-4.94821117453347,
58.8395692861344));
#184610=CARTESIAN_POINT('Ctrl Pts',(125.897302203287,-4.84600364015159,
58.8298067839887));
#184611=CARTESIAN_POINT('Ctrl Pts',(125.940727510726,-4.75,58.8382478507961));
#184612=CARTESIAN_POINT('',(125.940727510725,-4.75,58.8382478507959));
#184613=CARTESIAN_POINT('',(125.654512641377,-4.75,60.3106883584444));
#184614=CARTESIAN_POINT('Origin',(130.697657538777,-4.75,60.5269436545036));
#184615=CARTESIAN_POINT('',(105.703016080146,-4.75000000000024,54.9044156158684));
#184616=CARTESIAN_POINT('',(106.028205189486,-4.75,54.9676262909074));
#184617=CARTESIAN_POINT('',(105.416801210798,-4.75000000000024,56.376856123517));
#184618=CARTESIAN_POINT('Ctrl Pts',(105.703016080146,-4.75,54.9044156158684));
#184619=CARTESIAN_POINT('Ctrl Pts',(105.746441387585,-4.84600364015159,
54.9128566826758));
#184620=CARTESIAN_POINT('Ctrl Pts',(105.790717792192,-4.94821117453345,
54.9412748132961));
#184621=CARTESIAN_POINT('Ctrl Pts',(105.867305872833,-5.13686749643076,
55.0375736593997));
#184622=CARTESIAN_POINT('Ctrl Pts',(105.899558182295,-5.22334909571738,
55.1054372968028));
#184623=CARTESIAN_POINT('Ctrl Pts',(105.940777714848,-5.35302314086569,
55.2515648439157));
#184624=CARTESIAN_POINT('Ctrl Pts',(105.954320413686,-5.40768895518066,
55.3369203068544));
#184625=CARTESIAN_POINT('Ctrl Pts',(105.95938191906,-5.4812216429014,55.5215601238718));
#184626=CARTESIAN_POINT('Ctrl Pts',(105.950738875149,-5.5,55.6208841180915));
#184627=CARTESIAN_POINT('Ctrl Pts',(105.914310987882,-5.5,55.8082884166259));
#184628=CARTESIAN_POINT('Ctrl Pts',(105.883914490959,-5.4800270257108,55.9062977262052));
#184629=CARTESIAN_POINT('Ctrl Pts',(105.807014400979,-5.40227743227456,
56.0793271551169));
#184630=CARTESIAN_POINT('Ctrl Pts',(105.7606568068,-5.34458926875733,56.1544518502842));
#184631=CARTESIAN_POINT('Ctrl Pts',(105.667118143852,-5.21223335422367,
56.2711028896394));
#184632=CARTESIAN_POINT('Ctrl Pts',(105.613263689509,-5.12726283579729,
56.3191129298369));
#184633=CARTESIAN_POINT('Ctrl Pts',(105.509180776692,-4.94281444512933,
56.3760861593815));
#184634=CARTESIAN_POINT('Ctrl Pts',(105.459007551167,-4.84330877665234,
56.385060245946));
#184635=CARTESIAN_POINT('Ctrl Pts',(105.416801210798,-4.75,56.3768561235169));
#184636=CARTESIAN_POINT('',(105.741990320138,-4.75,56.4400667985559));
#184637=CARTESIAN_POINT('Origin',(113.780205727422,1.45439216225896E-14,
67.3747406878918));
#184638=CARTESIAN_POINT('',(117.291108124754,-11.35,49.3128037940699));
#184639=CARTESIAN_POINT('Origin',(117.291108124754,1.45439216225896E-14,
49.3128037940698));
#184640=CARTESIAN_POINT('',(115.821871795436,-11.35,56.8713317333323));
#184641=CARTESIAN_POINT('',(113.780205727422,-11.35,67.3747406878918));
#184642=CARTESIAN_POINT('',(111.159143521215,-10.3082491238812,55.9649846470643));
#184643=CARTESIAN_POINT('Origin',(115.821871795436,1.45439216225896E-14,
56.8713317333323));
#184644=CARTESIAN_POINT('',(110.872928651867,-10.3082491238812,57.4374251547129));
#184645=CARTESIAN_POINT('Ctrl Pts',(111.159143521215,-10.3082491238809,
55.9649846470643));
#184646=CARTESIAN_POINT('Ctrl Pts',(111.064903755454,-10.2640110301717,
55.9466662008491));
#184647=CARTESIAN_POINT('Ctrl Pts',(110.960863279463,-10.2151256546922,
55.9462543064991));
#184648=CARTESIAN_POINT('Ctrl Pts',(110.760424415631,-10.1215699520289,
55.9887043007774));
#184649=CARTESIAN_POINT('Ctrl Pts',(110.663994856223,-10.0769611593424,
56.0315545919063));
#184650=CARTESIAN_POINT('Ctrl Pts',(110.510833751864,-10.0086163685144,
56.1398981821743));
#184651=CARTESIAN_POINT('Ctrl Pts',(110.44167794701,-9.97903582116453,56.2091786041817));
#184652=CARTESIAN_POINT('Ctrl Pts',(110.335096749968,-9.93883620340028,
56.3721171698957));
#184653=CARTESIAN_POINT('Ctrl Pts',(110.297744930294,-9.92836844602331,
56.4658607155597));
#184654=CARTESIAN_POINT('Ctrl Pts',(110.279815832717,-9.92836844602331,
56.5580974662147));
#184655=CARTESIAN_POINT('Ctrl Pts',(110.26188673514,-9.92836844602331,56.6503342168697));
#184656=CARTESIAN_POINT('Ctrl Pts',(110.261401600345,-9.93883620340028,
56.7512439558984));
#184657=CARTESIAN_POINT('Ctrl Pts',(110.299183747351,-9.97903582116453,
56.9422440530909));
#184658=CARTESIAN_POINT('Ctrl Pts',(110.337350821672,-10.0086163685144,
57.0323860336342));
#184659=CARTESIAN_POINT('Ctrl Pts',(110.438772806468,-10.0769611593424,
57.1902158104221));
#184660=CARTESIAN_POINT('Ctrl Pts',(110.512128593668,-10.1215699520289,
57.2660691944054));
#184661=CARTESIAN_POINT('Ctrl Pts',(110.682070010351,-10.2151256546922,
57.3805141813816));
#184662=CARTESIAN_POINT('Ctrl Pts',(110.778688886107,-10.2640110301717,
57.4191067084976));
#184663=CARTESIAN_POINT('Ctrl Pts',(110.872928651867,-10.308249123881,57.4374251547129));
#184664=CARTESIAN_POINT('',(115.535656926088,-11.35,58.3437722409808));
#184665=CARTESIAN_POINT('Origin',(115.535656926088,1.45439216225896E-14,
58.3437722409808));
#184666=CARTESIAN_POINT('',(115.446124912503,-11.35,58.804372222509));
#184667=CARTESIAN_POINT('',(113.780205727422,-11.35,67.3747406878918));
#184668=CARTESIAN_POINT('Origin',(115.446124912502,1.45439216225896E-14,
58.8043722225089));
#184669=CARTESIAN_POINT('Origin',(115.535656926088,1.45439216225896E-14,
58.3437722409808));
#184670=CARTESIAN_POINT('Origin',(115.821871795436,1.45439216225896E-14,
56.8713317333323));
#184671=CARTESIAN_POINT('',(125.940727510726,4.75000000000027,58.8382478507961));
#184672=CARTESIAN_POINT('Origin',(115.821871795436,1.45439216225896E-14,
56.8713317333323));
#184673=CARTESIAN_POINT('',(125.654512641378,4.75000000000027,60.3106883584446));
#184674=CARTESIAN_POINT('Origin',(115.535656926088,1.45439216225896E-14,
58.3437722409808));
#184675=CARTESIAN_POINT('Ctrl Pts',(125.654512641378,4.75,60.3106883584447));
#184676=CARTESIAN_POINT('Ctrl Pts',(125.61230630101,4.84330877665233,60.3024842360155));
#184677=CARTESIAN_POINT('Ctrl Pts',(125.569148299058,4.94281444512933,60.2753683060694));
#184678=CARTESIAN_POINT('Ctrl Pts',(125.493987021832,5.12726283579729,60.1835533615843));
#184679=CARTESIAN_POINT('Ctrl Pts',(125.462039039804,5.21223335422367,60.1188649340508));
#184680=CARTESIAN_POINT('Ctrl Pts',(125.419010017904,5.34458926875732,59.9756676934244));
#184681=CARTESIAN_POINT('Ctrl Pts',(125.404170373857,5.40227743227456,59.8886474008104));
#184682=CARTESIAN_POINT('Ctrl Pts',(125.397688170697,5.4800270257108,59.6994100150999));
#184683=CARTESIAN_POINT('Ctrl Pts',(125.406220154262,5.5,59.597150653446));
#184684=CARTESIAN_POINT('Ctrl Pts',(125.424718943952,5.5,59.5019831055666));
#184685=CARTESIAN_POINT('Ctrl Pts',(125.442648041529,5.5,59.4097463549116));
#184686=CARTESIAN_POINT('Ctrl Pts',(125.471841952088,5.4812216429014,59.3144170644385));
#184687=CARTESIAN_POINT('Ctrl Pts',(125.545702507498,5.40768895518066,59.1451182185494));
#184688=CARTESIAN_POINT('Ctrl Pts',(125.590233936868,5.35302314086569,59.0710512789374));
#184689=CARTESIAN_POINT('Ctrl Pts',(125.683192588985,5.22334909571738,58.9510054589944));
#184690=CARTESIAN_POINT('Ctrl Pts',(125.738518670655,5.13686749643077,58.9001654212853));
#184691=CARTESIAN_POINT('Ctrl Pts',(125.845604198444,4.94821117453347,58.8395692861344));
#184692=CARTESIAN_POINT('Ctrl Pts',(125.897302203287,4.84600364015159,58.8298067839887));
#184693=CARTESIAN_POINT('Ctrl Pts',(125.940727510726,4.75,58.8382478507961));
#184694=CARTESIAN_POINT('',(105.416801210798,4.75000000000027,56.376856123517));
#184695=CARTESIAN_POINT('Origin',(115.535656926088,1.45439216225896E-14,
58.3437722409808));
#184696=CARTESIAN_POINT('',(105.703016080146,4.75000000000027,54.9044156158684));
#184697=CARTESIAN_POINT('Origin',(115.821871795436,1.45439216225896E-14,
56.8713317333323));
#184698=CARTESIAN_POINT('Ctrl Pts',(105.703016080146,4.75,54.9044156158684));
#184699=CARTESIAN_POINT('Ctrl Pts',(105.746441387585,4.84600364015159,54.9128566826759));
#184700=CARTESIAN_POINT('Ctrl Pts',(105.790717792192,4.94821117453345,54.9412748132961));
#184701=CARTESIAN_POINT('Ctrl Pts',(105.867305872833,5.13686749643076,55.0375736593997));
#184702=CARTESIAN_POINT('Ctrl Pts',(105.899558182295,5.22334909571738,55.1054372968028));
#184703=CARTESIAN_POINT('Ctrl Pts',(105.940777714848,5.35302314086569,55.2515648439157));
#184704=CARTESIAN_POINT('Ctrl Pts',(105.954320413686,5.40768895518066,55.3369203068544));
#184705=CARTESIAN_POINT('Ctrl Pts',(105.95938191906,5.4812216429014,55.5215601238718));
#184706=CARTESIAN_POINT('Ctrl Pts',(105.950738875149,5.5,55.6208841180915));
#184707=CARTESIAN_POINT('Ctrl Pts',(105.932809777572,5.5,55.7131208687465));
#184708=CARTESIAN_POINT('Ctrl Pts',(105.914310987882,5.5,55.8082884166259));
#184709=CARTESIAN_POINT('Ctrl Pts',(105.883914490959,5.4800270257108,55.9062977262052));
#184710=CARTESIAN_POINT('Ctrl Pts',(105.807014400979,5.40227743227456,56.0793271551169));
#184711=CARTESIAN_POINT('Ctrl Pts',(105.7606568068,5.34458926875732,56.1544518502842));
#184712=CARTESIAN_POINT('Ctrl Pts',(105.667118143852,5.21223335422367,56.2711028896394));
#184713=CARTESIAN_POINT('Ctrl Pts',(105.613263689509,5.12726283579728,56.3191129298369));
#184714=CARTESIAN_POINT('Ctrl Pts',(105.509180776692,4.94281444512933,56.3760861593815));
#184715=CARTESIAN_POINT('Ctrl Pts',(105.459007551167,4.84330877665233,56.385060245946));
#184716=CARTESIAN_POINT('Ctrl Pts',(105.416801210798,4.75,56.3768561235169));
#184717=CARTESIAN_POINT('',(111.159143521215,10.3082491238812,55.9649846470643));
#184718=CARTESIAN_POINT('Origin',(115.821871795436,1.45439216225896E-14,
56.8713317333323));
#184719=CARTESIAN_POINT('',(110.872928651867,10.3082491238812,57.4374251547129));
#184720=CARTESIAN_POINT('Origin',(115.535656926088,1.45439216225896E-14,
58.3437722409808));
#184721=CARTESIAN_POINT('Ctrl Pts',(110.872928651867,10.308249123881,57.4374251547129));
#184722=CARTESIAN_POINT('Ctrl Pts',(110.778688886107,10.2640110301718,57.4191067084976));
#184723=CARTESIAN_POINT('Ctrl Pts',(110.682070010351,10.2151256546923,57.3805141813816));
#184724=CARTESIAN_POINT('Ctrl Pts',(110.512128593668,10.1215699520289,57.2660691944054));
#184725=CARTESIAN_POINT('Ctrl Pts',(110.438772806468,10.0769611593424,57.1902158104221));
#184726=CARTESIAN_POINT('Ctrl Pts',(110.337350821672,10.0086163685144,57.0323860336342));
#184727=CARTESIAN_POINT('Ctrl Pts',(110.299183747351,9.97903582116456,56.9422440530909));
#184728=CARTESIAN_POINT('Ctrl Pts',(110.261401600345,9.93883620340031,56.7512439558984));
#184729=CARTESIAN_POINT('Ctrl Pts',(110.26188673514,9.92836844602334,56.6503342168697));
#184730=CARTESIAN_POINT('Ctrl Pts',(110.279815832717,9.92836844602334,56.5580974662147));
#184731=CARTESIAN_POINT('Ctrl Pts',(110.297744930294,9.92836844602334,56.4658607155597));
#184732=CARTESIAN_POINT('Ctrl Pts',(110.335096749968,9.93883620340031,56.3721171698957));
#184733=CARTESIAN_POINT('Ctrl Pts',(110.44167794701,9.97903582116456,56.2091786041817));
#184734=CARTESIAN_POINT('Ctrl Pts',(110.510833751864,10.0086163685144,56.1398981821743));
#184735=CARTESIAN_POINT('Ctrl Pts',(110.663994856223,10.0769611593424,56.0315545919063));
#184736=CARTESIAN_POINT('Ctrl Pts',(110.760424415631,10.1215699520289,55.9887043007774));
#184737=CARTESIAN_POINT('Ctrl Pts',(110.960863279463,10.2151256546923,55.9462543064991));
#184738=CARTESIAN_POINT('Ctrl Pts',(111.064903755454,10.2640110301718,55.9466662008491));
#184739=CARTESIAN_POINT('Ctrl Pts',(111.159143521215,10.308249123881,55.9649846470643));
#184740=CARTESIAN_POINT('Origin',(117.291108124754,1.45439216225896E-14,
49.3128037940698));
#184741=CARTESIAN_POINT('',(117.386513081203,-10.84999988564,48.8219902915204));
#184742=CARTESIAN_POINT('Origin',(117.386513081203,1.45439216225896E-14,
48.8219902915203));
#184743=CARTESIAN_POINT('Origin',(117.291108124754,-10.85,49.3128037940698));
#184744=CARTESIAN_POINT('Origin',(113.780205727422,1.45439216225896E-14,
67.3747406878918));
#184745=CARTESIAN_POINT('',(117.291108124754,-9.84999999999999,49.3128037940699));
#184746=CARTESIAN_POINT('Origin',(117.291108124754,1.45439216225896E-14,
49.3128037940698));
#184747=CARTESIAN_POINT('',(117.386513081204,-9.84999999999999,48.8219902915204));
#184748=CARTESIAN_POINT('',(113.780205727422,-9.84999999999999,67.3747406878918));
#184749=CARTESIAN_POINT('Origin',(117.386513081203,1.45439216225896E-14,
48.8219902915203));
#184750=CARTESIAN_POINT('Origin',(113.780205727422,1.45439216225896E-14,
67.3747406878918));
#184751=CARTESIAN_POINT('',(117.329270107334,-10.15,49.11647839305));
#184752=CARTESIAN_POINT('Origin',(117.329270107334,1.45439216225896E-14,
49.11647839305));
#184753=CARTESIAN_POINT('',(117.233865150885,-10.15,49.6072918955995));
#184754=CARTESIAN_POINT('',(113.780205727422,-10.15,67.3747406878918));
#184755=CARTESIAN_POINT('Origin',(117.233865150885,1.45439216225896E-14,
49.6072918955995));
#184756=CARTESIAN_POINT('Origin',(115.446124912502,1.45439216225896E-14,
58.8043722225089));
#184757=CARTESIAN_POINT('',(115.315832412722,-11.6194313553,59.4746656805513));
#184758=CARTESIAN_POINT('Origin',(115.446124912502,-12.35,58.8043722225089));
#184759=CARTESIAN_POINT('Origin',(115.315832412723,1.45439216225896E-14,
59.4746656805514));
#184760=CARTESIAN_POINT('Origin',(115.185539912945,1.45439216225896E-14,
60.1449591385841));
#184761=CARTESIAN_POINT('',(115.192199082871,-11.88825353763,60.1107008501589));
#184762=CARTESIAN_POINT('Origin',(115.185539912945,-10.88886271061,60.1449591385841));
#184763=CARTESIAN_POINT('',(115.192199082871,11.888253537687,60.1107008501569));
#184764=CARTESIAN_POINT('Origin',(115.192199082871,1.45439216225896E-14,
60.110700850159));
#184765=CARTESIAN_POINT('Origin',(115.192199082871,1.45439216225896E-14,
60.110700850159));
#184766=CARTESIAN_POINT('Origin',(114.886903222233,1.45439216225896E-14,
61.6813040583175));
#184767=CARTESIAN_POINT('',(114.581607361595,11.999999999933,63.2519072664783));
#184768=CARTESIAN_POINT('Origin',(114.581607361595,1.45439216225896E-14,
63.2519072664759));
#184769=CARTESIAN_POINT('',(114.886903222233,11.94412676881,61.6813040583175));
#184770=CARTESIAN_POINT('Origin',(114.28108174878,1.45439216225896E-14,
64.7979697995068));
#184771=CARTESIAN_POINT('',(114.772417274494,-12.25,62.2702802613768));
#184772=CARTESIAN_POINT('Origin',(114.772417274494,1.45439216225896E-14,
62.2702802613769));
#184773=CARTESIAN_POINT('',(117.386513081203,-12.25,48.8219902915203));
#184774=CARTESIAN_POINT('',(114.28108174878,-12.25,64.7979697995068));
#184775=CARTESIAN_POINT('Origin',(117.386513081203,1.45439216225896E-14,
48.8219902915203));
#184776=CARTESIAN_POINT('Origin',(114.28108174878,1.45439216225896E-14,
64.7979697995068));
#184777=CARTESIAN_POINT('',(114.581607361595,-12.75,63.2519072664759));
#184778=CARTESIAN_POINT('Origin',(114.581607361595,1.45439216225896E-14,
63.2519072664759));
#184779=CARTESIAN_POINT('',(114.772417274494,-12.75,62.2702802613768));
#184780=CARTESIAN_POINT('',(114.28108174878,-12.75,64.7979697995068));
#184781=CARTESIAN_POINT('Origin',(114.772417274494,1.45439216225896E-14,
62.2702802613769));
#184782=CARTESIAN_POINT('Origin',(114.28108174878,1.45439216225896E-14,
64.7979697995068));
#184783=CARTESIAN_POINT('',(115.383008995769,-13.1,59.12907384506));
#184784=CARTESIAN_POINT('Origin',(115.383008995769,1.45439216225896E-14,
59.12907384506));
#184785=CARTESIAN_POINT('',(115.096794126421,-13.1,60.6015143527085));
#184786=CARTESIAN_POINT('',(114.28108174878,-13.1,64.7979697995068));
#184787=CARTESIAN_POINT('Origin',(115.096794126421,1.45439216225896E-14,
60.6015143527085));
#184788=CARTESIAN_POINT('Origin',(114.28108174878,1.45439216225896E-14,
64.7979697995068));
#184789=CARTESIAN_POINT('',(121.534871381197,-13.,50.1377119242634));
#184790=CARTESIAN_POINT('',(121.534871381197,13.,50.1377119242634));
#184791=CARTESIAN_POINT('Origin',(117.291108124754,1.45439216225896E-14,
49.3128037940698));
#184792=CARTESIAN_POINT('',(121.057846598951,13.,52.591779437011));
#184793=CARTESIAN_POINT('',(121.057846598951,13.,52.591779437011));
#184794=CARTESIAN_POINT('',(112.570320086065,13.,50.9419631766238));
#184795=CARTESIAN_POINT('Origin',(116.814083342508,1.45439216225896E-14,
51.7668713068174));
#184796=CARTESIAN_POINT('',(113.047344868311,13.,48.4878956638762));
#184797=CARTESIAN_POINT('',(112.570320086065,13.,50.9419631766238));
#184798=CARTESIAN_POINT('',(113.047344868311,-13.,48.4878956638762));
#184799=CARTESIAN_POINT('Origin',(117.291108124754,1.45439216225896E-14,
49.3128037940698));
#184800=CARTESIAN_POINT('',(112.570320086065,-13.,50.9419631766238));
#184801=CARTESIAN_POINT('',(112.570320086065,-13.,50.9419631766238));
#184802=CARTESIAN_POINT('',(116.814083342508,-13.7,51.7668713068173));
#184803=CARTESIAN_POINT('Origin',(116.814083342508,1.45439216225896E-14,
51.7668713068174));
#184804=CARTESIAN_POINT('',(115.383008995769,-13.7,59.12907384506));
#184805=CARTESIAN_POINT('',(114.28108174878,-13.7,64.7979697995068));
#184806=CARTESIAN_POINT('Origin',(115.383008995769,1.45439216225896E-14,
59.12907384506));
#184807=CARTESIAN_POINT('',(121.057846598951,-13.,52.591779437011));
#184808=CARTESIAN_POINT('Origin',(116.814083342508,1.45439216225896E-14,
51.7668713068174));
#184809=CARTESIAN_POINT('',(121.057846598951,-13.,52.591779437011));
#184810=CARTESIAN_POINT('Origin',(114.476661909501,1.45439216225896E-14,
63.7918021192803));
#184811=CARTESIAN_POINT('',(105.907189290968,-10.2076212837564,62.3807362902962));
#184812=CARTESIAN_POINT('Ctrl Pts',(122.504911634294,-11.2745024089981,
65.0976651926838));
#184813=CARTESIAN_POINT('Ctrl Pts',(123.229846581212,-10.7328655109838,
65.2453382804213));
#184814=CARTESIAN_POINT('Ctrl Pts',(123.900533178686,-10.1186901216539,
65.3827789616297));
#184815=CARTESIAN_POINT('Ctrl Pts',(125.097983067777,-8.78240845240083,
65.6289243192982));
#184816=CARTESIAN_POINT('Ctrl Pts',(125.626442830263,-8.06472399520229,
65.7379736981974));
#184817=CARTESIAN_POINT('Ctrl Pts',(126.393898186431,-6.77838906626577,
65.8984097879606));
#184818=CARTESIAN_POINT('Ctrl Pts',(126.670869901367,-6.23612244254981,
65.9569283595829));
#184819=CARTESIAN_POINT('Ctrl Pts',(127.225281497024,-4.94994463554516,
66.0752469001846));
#184820=CARTESIAN_POINT('Ctrl Pts',(127.477101999605,-4.19597408503903,
66.1299606016456));
#184821=CARTESIAN_POINT('Ctrl Pts',(127.87399481505,-2.556029182679,66.2194221298755));
#184822=CARTESIAN_POINT('Ctrl Pts',(128.000343146586,-1.66956325408612,
66.2508298482742));
#184823=CARTESIAN_POINT('Ctrl Pts',(128.083737879612,0.118285322566095,
66.2805335003563));
#184824=CARTESIAN_POINT('Ctrl Pts',(128.040024208525,1.01687449567218,66.2785232628767));
#184825=CARTESIAN_POINT('Ctrl Pts',(127.78178873694,2.79232894127849,66.2414913384502));
#184826=CARTESIAN_POINT('Ctrl Pts',(127.567388976971,3.66503480243605,66.2067639194195));
#184827=CARTESIAN_POINT('Ctrl Pts',(126.979550286204,5.34528302425291,66.1059142543956));
#184828=CARTESIAN_POINT('Ctrl Pts',(126.608529648767,6.1512620066344,66.0401808204024));
#184829=CARTESIAN_POINT('Ctrl Pts',(125.713026001603,7.68934214784707,65.8793328936045));
#184830=CARTESIAN_POINT('Ctrl Pts',(125.187964517677,8.416928907309,65.7842870607944));
#184831=CARTESIAN_POINT('Ctrl Pts',(124.022781859346,9.73914833353154,65.5711253909796));
#184832=CARTESIAN_POINT('Ctrl Pts',(123.38722814423,10.3351025591763,65.4538764821083));
#184833=CARTESIAN_POINT('Ctrl Pts',(121.994162172805,11.4094174928648,65.1963808819556));
#184834=CARTESIAN_POINT('Ctrl Pts',(121.235991649557,11.8820277086889,65.0560519275869));
#184835=CARTESIAN_POINT('Ctrl Pts',(119.670104692157,12.6544884296133,64.7649352454329));
#184836=CARTESIAN_POINT('Ctrl Pts',(118.866867650534,12.9590403586294,64.6150367011459));
#184837=CARTESIAN_POINT('Ctrl Pts',(117.183754765794,13.4163303616198,64.3012694177438));
#184838=CARTESIAN_POINT('Ctrl Pts',(116.305307807354,13.5622060315306,64.1375519447353));
#184839=CARTESIAN_POINT('Ctrl Pts',(114.554928431228,13.6746520928841,63.8106529013362));
#184840=CARTESIAN_POINT('Ctrl Pts',(113.685441741559,13.6450888740068,63.6479984642041));
#184841=CARTESIAN_POINT('Ctrl Pts',(111.968639264187,13.4149320799642,63.3277473758802));
#184842=CARTESIAN_POINT('Ctrl Pts',(111.124955522097,13.2160582326946,63.1705638324682));
#184843=CARTESIAN_POINT('Ctrl Pts',(109.483290565272,12.6550171724688,62.8646119243846));
#184844=CARTESIAN_POINT('Ctrl Pts',(108.687973652607,12.2926589715997,62.7164434632677));
#184845=CARTESIAN_POINT('Ctrl Pts',(107.187366760791,11.4204732223485,62.4382823800872));
#184846=CARTESIAN_POINT('Ctrl Pts',(106.484490876799,10.9150751365952,62.3083969275442));
#184847=CARTESIAN_POINT('Ctrl Pts',(105.174918063374,9.76687727465901,62.0669615265641));
#184848=CARTESIAN_POINT('Ctrl Pts',(104.57216745938,9.12421627830972,61.9563161154106));
#184849=CARTESIAN_POINT('Ctrl Pts',(103.509288763409,7.74134958430475,61.7632882078509));
#184850=CARTESIAN_POINT('Ctrl Pts',(103.048965082131,7.0071913416104,61.6804785057821));
#184851=CARTESIAN_POINT('Ctrl Pts',(102.464674510065,5.84285378745556,61.5766532538355));
#184852=CARTESIAN_POINT('Ctrl Pts',(102.287086002315,5.44206810749397,61.5453754575537));
#184853=CARTESIAN_POINT('Ctrl Pts',(101.808535655182,4.20443804160805,61.4623588099708));
#184854=CARTESIAN_POINT('Ctrl Pts',(101.569522799854,3.34540366653471,61.4229519012272));
#184855=CARTESIAN_POINT('Ctrl Pts',(101.264583014311,1.61740419385571,61.3770688000621));
#184856=CARTESIAN_POINT('Ctrl Pts',(101.194723999211,0.751309308118347,
61.3698094353778));
#184857=CARTESIAN_POINT('Ctrl Pts',(101.219594865846,-0.992579368004674,
61.3879182276713));
#184858=CARTESIAN_POINT('Ctrl Pts',(101.316557330348,-1.8675772424215,61.4137312965633));
#184859=CARTESIAN_POINT('Ctrl Pts',(101.646121445148,-3.44371817065294,
61.4900696530388));
#184860=CARTESIAN_POINT('Ctrl Pts',(101.8536256679,-4.14832309282748,61.5358101090581));
#184861=CARTESIAN_POINT('Ctrl Pts',(102.518194464448,-5.87573706785547,
61.6790675863199));
#184862=CARTESIAN_POINT('Ctrl Pts',(103.04740164905,-6.8647922843056,61.7908934513442));
#184863=CARTESIAN_POINT('Ctrl Pts',(104.003808267056,-8.21865358302084,
61.9894116642463));
#184864=CARTESIAN_POINT('Ctrl Pts',(104.344782045948,-8.6437972103183,62.0597593868494));
#184865=CARTESIAN_POINT('Ctrl Pts',(105.085067467861,-9.45883829531425,
62.2121067994063));
#184866=CARTESIAN_POINT('Ctrl Pts',(105.484930025179,-9.8467254250202,62.2942672565808));
#184867=CARTESIAN_POINT('Ctrl Pts',(105.907189290968,-10.2076212837564,
62.3807362902962));
#184868=CARTESIAN_POINT('',(124.256736260291,-8.90570865984179,65.9470463235759));
#184869=CARTESIAN_POINT('Origin',(114.428959431277,1.45439216225896E-14,
64.0372088705551));
#184870=CARTESIAN_POINT('',(114.489783311165,-13.7191326559559,63.7243240965168));
#184871=CARTESIAN_POINT('Ctrl Pts',(124.256949391325,-8.90590330286328,
65.9470620427268));
#184872=CARTESIAN_POINT('Ctrl Pts',(123.99775328236,-9.224088446109,65.8841924187124));
#184873=CARTESIAN_POINT('Ctrl Pts',(123.723345529523,-9.53003896735735,
65.8186626717206));
#184874=CARTESIAN_POINT('Ctrl Pts',(123.435091579848,-9.82251828793179,
65.750626757231));
#184875=CARTESIAN_POINT('Ctrl Pts',(123.146396551434,-10.1154451527995,
65.6824867359444));
#184876=CARTESIAN_POINT('Ctrl Pts',(122.843813501118,-10.3948605139533,
65.6118329845868));
#184877=CARTESIAN_POINT('Ctrl Pts',(122.528671502062,-10.6595503748197,
65.5388118757864));
#184878=CARTESIAN_POINT('Ctrl Pts',(122.443732266683,-10.7308914035053,
65.5191307251729));
#184879=CARTESIAN_POINT('Ctrl Pts',(122.357880424489,-10.8011628143638,
65.4992775469335));
#184880=CARTESIAN_POINT('Ctrl Pts',(122.271141391864,-10.8703410420963,
65.479255089113));
#184881=CARTESIAN_POINT('Ctrl Pts',(121.891332759646,-11.1732552810398,
65.3915817304382));
#184882=CARTESIAN_POINT('Ctrl Pts',(121.494697233621,-11.455394761453,65.3005532770298));
#184883=CARTESIAN_POINT('Ctrl Pts',(121.083308218077,-11.7144688895035,
65.2065620719827));
#184884=CARTESIAN_POINT('Ctrl Pts',(120.704121940928,-11.9532631946719,
65.1199283171187));
#184885=CARTESIAN_POINT('Ctrl Pts',(120.312402038618,-12.1724609188301,
65.0307775938138));
#184886=CARTESIAN_POINT('Ctrl Pts',(119.910345037359,-12.3712103911295,
64.9395284962991));
#184887=CARTESIAN_POINT('Ctrl Pts',(119.491215508411,-12.5783993529999,
64.8444046926132));
#184888=CARTESIAN_POINT('Ctrl Pts',(119.060715016913,-12.7631480604679,
64.7471209483971));
#184889=CARTESIAN_POINT('Ctrl Pts',(118.621220734337,-12.9244627256754,
64.6481704279395));
#184890=CARTESIAN_POINT('Ctrl Pts',(118.18172645176,-13.0857773908829,64.5492199074818));
#184891=CARTESIAN_POINT('Ctrl Pts',(117.733237756405,-13.2236578222968,
64.4486024899362));
#184892=CARTESIAN_POINT('Ctrl Pts',(117.278172251404,-13.3370690493505,
64.3468191987493));
#184893=CARTESIAN_POINT('Ctrl Pts',(116.848023284575,-13.4442705876078,
64.2506089233859));
#184894=CARTESIAN_POINT('Ctrl Pts',(116.411989460296,-13.5297146283601,
64.1532941007664));
#184895=CARTESIAN_POINT('Ctrl Pts',(115.972297165646,-13.5927197612154,
64.0551965812453));
#184896=CARTESIAN_POINT('Ctrl Pts',(115.745509457432,-13.6252170095407,
64.0045991250144));
#184897=CARTESIAN_POINT('Ctrl Pts',(115.517747807483,-13.651745239074,63.9537933154996));
#184898=CARTESIAN_POINT('Ctrl Pts',(115.28931310856,-13.6722136550253,63.9028224206965));
#184899=CARTESIAN_POINT('Ctrl Pts',(115.023553746488,-13.6960264697663,
63.8435232312522));
#184900=CARTESIAN_POINT('Ctrl Pts',(114.7568835816,-13.7116373409563,63.7840006322766));
#184901=CARTESIAN_POINT('Ctrl Pts',(114.489783311165,-13.7191326559559,
63.7243240965168));
#184902=CARTESIAN_POINT('Ctrl Pts',(114.489803604467,-13.7190747033231,
63.7242257846487));
#184903=CARTESIAN_POINT('Ctrl Pts',(113.409266451882,-13.7491677927584,
63.4832965023283));
#184904=CARTESIAN_POINT('Ctrl Pts',(112.321523697456,-13.6449312950591,
63.2409659995486));
#184905=CARTESIAN_POINT('Ctrl Pts',(110.195514536491,-13.1698942968648,
62.7659222693647));
#184906=CARTESIAN_POINT('Ctrl Pts',(109.157373226761,-12.7991074634966,
62.5332333584385));
#184907=CARTESIAN_POINT('Ctrl Pts',(108.175183023666,-12.30344424038,62.3122333729097));
#184908=CARTESIAN_POINT('Origin',(114.28108174878,1.45439216225896E-14,
64.7979697995068));
#184909=CARTESIAN_POINT('',(114.428959431276,-12.75,64.037208870555));
#184910=CARTESIAN_POINT('Origin',(114.428959431277,1.45439216225896E-14,
64.0372088705551));
#184911=CARTESIAN_POINT('',(114.524364387726,-12.75,63.5463953680055));
#184912=CARTESIAN_POINT('',(114.28108174878,-12.75,64.7979697995068));
#184913=CARTESIAN_POINT('Origin',(114.524364387726,1.45439216225896E-14,
63.5463953680056));
#184914=CARTESIAN_POINT('Ctrl Pts',(118.491253192553,-12.7183023352,63.7707658968246));
#184915=CARTESIAN_POINT('Ctrl Pts',(116.466184337262,-13.35843074567,63.3507673831021));
#184916=CARTESIAN_POINT('Ctrl Pts',(112.105678659218,-13.60903770072,62.4504406331449));
#184917=CARTESIAN_POINT('Ctrl Pts',(106.15470984369,-10.81093357074,61.2145945848077));
#184918=CARTESIAN_POINT('Ctrl Pts',(102.187393024908,-5.49082338424599,
60.3643333489951));
#184919=CARTESIAN_POINT('Ctrl Pts',(101.132039193786,1.11008681820601,60.0801032035486));
#184920=CARTESIAN_POINT('Ctrl Pts',(103.238445493676,7.45205865399302,60.4104600367413));
#184921=CARTESIAN_POINT('Ctrl Pts',(108.018664973673,12.05569208811,61.2605560960788));
#184922=CARTESIAN_POINT('Ctrl Pts',(114.361086873968,13.84710498951,62.4143150601738));
#184923=CARTESIAN_POINT('Ctrl Pts',(120.789672201652,12.40841498499,63.5848225814906));
#184924=CARTESIAN_POINT('Ctrl Pts',(125.808286596475,8.07522435927901,64.4812581493247));
#184925=CARTESIAN_POINT('Ctrl Pts',(128.249697402688,1.85833282744001,64.8767335869671));
#184926=CARTESIAN_POINT('Ctrl Pts',(127.547854389266,-4.79205045842999,
64.6612193264683));
#184927=CARTESIAN_POINT('Ctrl Pts',(123.869931462632,-10.32459610784,63.8672108455791));
#184928=CARTESIAN_POINT('Ctrl Pts',(118.077330243317,-13.44873178266,62.66214849318));
#184929=CARTESIAN_POINT('Ctrl Pts',(111.524741598597,-13.43569294448,61.309358812883));
#184930=CARTESIAN_POINT('Ctrl Pts',(105.744138033829,-10.28852115219,60.1066285799213));
#184931=CARTESIAN_POINT('Ctrl Pts',(102.087411734415,-4.74135456058899,
59.3167403265448));
#184932=CARTESIAN_POINT('Ctrl Pts',(101.411019797005,1.91182387847601,59.1061732787571));
#184933=CARTESIAN_POINT('Ctrl Pts',(103.876199192475,8.11903274642801,59.5062688851827));
#184934=CARTESIAN_POINT('Ctrl Pts',(108.911355151527,12.43232157685,60.4059198234309));
#184935=CARTESIAN_POINT('Ctrl Pts',(115.345396602207,13.84553306015,61.5774879129147));
#184936=CARTESIAN_POINT('Ctrl Pts',(121.68091561507,12.02900852572,62.729905084921));
#184937=CARTESIAN_POINT('Ctrl Pts',(126.443486502869,7.40648714394101,63.576570588332));
#184938=CARTESIAN_POINT('Ctrl Pts',(128.525603902826,1.05626065173001,63.9022061140864));
#184939=CARTESIAN_POINT('Ctrl Pts',(127.445029542533,-5.54035890633199,
63.6130735699189));
#184940=CARTESIAN_POINT('Ctrl Pts',(123.457283904857,-10.84458346349,62.7588413541581));
#184941=CARTESIAN_POINT('Ctrl Pts',(117.496039897072,-13.61910129622,61.5209980008064));
#184942=CARTESIAN_POINT('Ctrl Pts',(110.95533052156,-13.21670165587,60.1705174280637));
#184943=CARTESIAN_POINT('Ctrl Pts',(105.364346129962,-9.73125672786299,
59.0046456125342));
#184944=CARTESIAN_POINT('Ctrl Pts',(102.030787974481,-3.97579561520298,
58.2775751963556));
#184945=CARTESIAN_POINT('Ctrl Pts',(101.735573576727,2.70704381218202,58.141101926309));
#184946=CARTESIAN_POINT('Ctrl Pts',(104.551599204905,8.75860830718901,58.6093954722332));
#184947=CARTESIAN_POINT('Ctrl Pts',(108.066051618942,11.43042410411,59.2398131494504));
#184948=CARTESIAN_POINT('Ctrl Pts',(110.029513630199,12.2704525675,59.5951103675036));
#184949=CARTESIAN_POINT('Ctrl Pts',(118.575698917339,-12.91976003203,63.6631452639466));
#184950=CARTESIAN_POINT('Ctrl Pts',(116.518474788798,-13.57002806584,63.2368963670782));
#184951=CARTESIAN_POINT('Ctrl Pts',(112.088742340823,-13.82460463088,62.3231132290306));
#184952=CARTESIAN_POINT('Ctrl Pts',(106.043275629434,-10.98217857815,61.0688985588191));
#184953=CARTESIAN_POINT('Ctrl Pts',(102.012881929328,-5.57779793505799,
60.2063763581299));
#184954=CARTESIAN_POINT('Ctrl Pts',(100.940576662033,1.12767057488801,59.9188511708367));
#184955=CARTESIAN_POINT('Ctrl Pts',(103.080113753482,7.57009913876102,60.2556480096718));
#184956=CARTESIAN_POINT('Ctrl Pts',(107.935817181206,12.24665404968,61.1204167353237));
#184957=CARTESIAN_POINT('Ctrl Pts',(114.378468289507,14.06644290155,62.2936583810791));
#184958=CARTESIAN_POINT('Ctrl Pts',(120.90864765245,12.60496407136,63.4839138809234));
#184959=CARTESIAN_POINT('Ctrl Pts',(126.006522166478,8.20313577842201,64.3957561321142));
#184960=CARTESIAN_POINT('Ctrl Pts',(128.486370230037,1.88776878842501,64.7987030530064));
#184961=CARTESIAN_POINT('Ctrl Pts',(127.773175385898,-4.86795645775498,
64.5809822091322));
#184962=CARTESIAN_POINT('Ctrl Pts',(124.03675957236,-10.48813753796,63.7756038060656));
#184963=CARTESIAN_POINT('Ctrl Pts',(118.152168997266,-13.66175946975,62.5526604450219));
#184964=CARTESIAN_POINT('Ctrl Pts',(111.495552808624,-13.6485140966,61.1796497576808));
#184965=CARTESIAN_POINT('Ctrl Pts',(105.623149930727,-10.45149115561,59.959075456798));
#184966=CARTESIAN_POINT('Ctrl Pts',(101.908266498638,-4.81645753773299,
59.1578825455907));
#184967=CARTESIAN_POINT('Ctrl Pts',(101.220925875135,1.94210713682301,58.9451872781849));
#184968=CARTESIAN_POINT('Ctrl Pts',(103.724919022004,8.24763808969801,59.3528275512662));
#184969=CARTESIAN_POINT('Ctrl Pts',(108.839597118367,12.62924934324,60.2679361042754));
#184970=CARTESIAN_POINT('Ctrl Pts',(115.375319029201,14.06484607286,61.4592689716785));
#184971=CARTESIAN_POINT('Ctrl Pts',(121.81095790845,12.21954782011,62.6311475713711));
#184972=CARTESIAN_POINT('Ctrl Pts',(126.648733190572,7.52380577674502,63.4924314011583));
#184973=CARTESIAN_POINT('Ctrl Pts',(128.763596646313,1.07299180282801,63.8244321471129));
#184974=CARTESIAN_POINT('Ctrl Pts',(127.665671357083,-5.62811809899199,
63.5319269071945));
#184975=CARTESIAN_POINT('Ctrl Pts',(123.614525245928,-11.01636148465,62.6653708262899));
#184976=CARTESIAN_POINT('Ctrl Pts',(117.558620583404,-13.83482763357,61.4091272137953));
#184977=CARTESIAN_POINT('Ctrl Pts',(110.9140718314,-13.42605398962,60.0384622102139));
#184978=CARTESIAN_POINT('Ctrl Pts',(105.234291691218,-9.88539967209599,
58.8553301634914));
#184979=CARTESIAN_POINT('Ctrl Pts',(101.847695381066,-4.03877215141899,
58.1179501229642));
#184980=CARTESIAN_POINT('Ctrl Pts',(101.547570143079,2.74992334101601,57.9805222775116));
#184981=CARTESIAN_POINT('Ctrl Pts',(104.407966921148,8.89734451667401,58.4574407443087));
#184982=CARTESIAN_POINT('Ctrl Pts',(107.977931770066,11.61148183125,59.0986489996371));
#184983=CARTESIAN_POINT('Ctrl Pts',(109.972416770466,12.46481633148,59.4599765059926));
#184984=CARTESIAN_POINT('Ctrl Pts',(118.660144642124,-13.12121772886,63.5555246310785));
#184985=CARTESIAN_POINT('Ctrl Pts',(116.570765240331,-13.78162538602,63.123025351064));
#184986=CARTESIAN_POINT('Ctrl Pts',(112.071806022429,-14.04017156104,62.1957858249163));
#184987=CARTESIAN_POINT('Ctrl Pts',(105.931841415176,-11.15342358557,60.9232025328403));
#184988=CARTESIAN_POINT('Ctrl Pts',(101.838370833747,-5.66477248586999,
60.0484193672646));
#184989=CARTESIAN_POINT('Ctrl Pts',(100.749114130278,1.14525433156901,59.7575991381346));
#184990=CARTESIAN_POINT('Ctrl Pts',(102.921782013287,7.68813962352701,60.1008359826022));
#184991=CARTESIAN_POINT('Ctrl Pts',(107.852969388734,12.43761601124,60.9802773745779));
#184992=CARTESIAN_POINT('Ctrl Pts',(114.39584970504,14.28578081359,62.1730017019832));
#184993=CARTESIAN_POINT('Ctrl Pts',(121.027623103238,12.80151315773,63.3830051803645));
#184994=CARTESIAN_POINT('Ctrl Pts',(126.204757736472,8.33104719757401,64.3102541149019));
#184995=CARTESIAN_POINT('Ctrl Pts',(128.723043057384,1.91720474942301,64.7206725190554));
#184996=CARTESIAN_POINT('Ctrl Pts',(127.99849638253,-4.94386245706599,64.5007450917961));
#184997=CARTESIAN_POINT('Ctrl Pts',(124.203587682101,-10.65167896807,63.6839967665646));
#184998=CARTESIAN_POINT('Ctrl Pts',(118.227007751235,-13.87478715684,62.4431723968677));
#184999=CARTESIAN_POINT('Ctrl Pts',(111.466364018676,-13.86133524872,61.0499407024733));
#185000=CARTESIAN_POINT('Ctrl Pts',(105.502161827646,-10.61446115905,59.8115223336785));
#185001=CARTESIAN_POINT('Ctrl Pts',(101.729121262874,-4.89156051490299,
58.9990247646287));
#185002=CARTESIAN_POINT('Ctrl Pts',(101.030831953255,1.97239039513901,58.7842012776108));
#185003=CARTESIAN_POINT('Ctrl Pts',(103.573638851525,8.37624343293902,59.199386217338));
#185004=CARTESIAN_POINT('Ctrl Pts',(108.767839085174,12.82617710962,60.1299523851135));
#185005=CARTESIAN_POINT('Ctrl Pts',(115.405241456157,14.28415908557,61.341050030425));
#185006=CARTESIAN_POINT('Ctrl Pts',(121.941000201793,12.41008711451,62.532390057814));
#185007=CARTESIAN_POINT('Ctrl Pts',(126.853979878247,7.64112440958602,63.408292213969));
#185008=CARTESIAN_POINT('Ctrl Pts',(129.001589389788,1.08972295397001,63.7466581801474));
#185009=CARTESIAN_POINT('Ctrl Pts',(127.886313171645,-5.71587729160999,
63.4507802444622));
#185010=CARTESIAN_POINT('Ctrl Pts',(123.771766587033,-11.18813950578,62.5719002984386));
#185011=CARTESIAN_POINT('Ctrl Pts',(117.621201269786,-14.05055397091,61.2972564267837));
#185012=CARTESIAN_POINT('Ctrl Pts',(110.872813141286,-13.63540632339,59.9064069923831));
#185013=CARTESIAN_POINT('Ctrl Pts',(105.104237252503,-10.03954261636,58.7060147144545));
#185014=CARTESIAN_POINT('Ctrl Pts',(101.664602787659,-4.10174868768399,
57.9583250495846));
#185015=CARTESIAN_POINT('Ctrl Pts',(101.359566709432,2.79280286980002,57.8199426287141));
#185016=CARTESIAN_POINT('Ctrl Pts',(104.264334637359,9.03608072612001,58.3054860163884));
#185017=CARTESIAN_POINT('Ctrl Pts',(107.889811921153,11.79253955836,58.9574848498063));
#185018=CARTESIAN_POINT('Ctrl Pts',(109.91531991069,12.65918009544,59.3248426444734));
#185019=CARTESIAN_POINT('Ctrl Pts',(118.74459036691,-13.32267542569,63.4479039982005));
#185020=CARTESIAN_POINT('Ctrl Pts',(116.623055691866,-13.99322270619,63.0091543350402));
#185021=CARTESIAN_POINT('Ctrl Pts',(112.054869704034,-14.2557384912,62.068458420802));
#185022=CARTESIAN_POINT('Ctrl Pts',(105.820407200921,-11.32466859299,60.7775065068516));
#185023=CARTESIAN_POINT('Ctrl Pts',(101.663859738167,-5.75174703668099,
59.8904623763993));
#185024=CARTESIAN_POINT('Ctrl Pts',(100.557651598525,1.16283808825201,59.5963471054226));
#185025=CARTESIAN_POINT('Ctrl Pts',(102.763450273093,7.80618010829502,59.9460239555327));
#185026=CARTESIAN_POINT('Ctrl Pts',(107.770121596268,12.62857797281,60.840138013823));
#185027=CARTESIAN_POINT('Ctrl Pts',(114.413231120579,14.50511872564,62.0523450228885));
#185028=CARTESIAN_POINT('Ctrl Pts',(121.146598554036,12.9980622441,63.2820964797973));
#185029=CARTESIAN_POINT('Ctrl Pts',(126.402993306465,8.45895861671701,64.2247520976895));
#185030=CARTESIAN_POINT('Ctrl Pts',(128.959715884732,1.94664071040801,64.6426419850946));
#185031=CARTESIAN_POINT('Ctrl Pts',(128.223817379161,-5.01976845639098,
64.4205079744699));
#185032=CARTESIAN_POINT('Ctrl Pts',(124.37041579183,-10.81522039819,63.5923897270511));
#185033=CARTESIAN_POINT('Ctrl Pts',(118.301846505182,-14.08781484393,62.3336843487194));
#185034=CARTESIAN_POINT('Ctrl Pts',(111.437175228705,-14.07415640083,60.9202316472613));
#185035=CARTESIAN_POINT('Ctrl Pts',(105.381173724543,-10.77743116247,59.6639692105651));
#185036=CARTESIAN_POINT('Ctrl Pts',(101.549976027089,-4.96666349204699,
58.8401669836628));
#185037=CARTESIAN_POINT('Ctrl Pts',(100.840738031383,2.00267365348601,58.6232152770484));
#185038=CARTESIAN_POINT('Ctrl Pts',(103.422358681056,8.50484877620901,59.0459448834116));
#185039=CARTESIAN_POINT('Ctrl Pts',(108.696081052011,13.02310487601,59.9919686659676));
#185040=CARTESIAN_POINT('Ctrl Pts',(115.435163883153,14.50347209828,61.222831089179));
#185041=CARTESIAN_POINT('Ctrl Pts',(122.07104249517,12.60062640889,62.4336325442737));
#185042=CARTESIAN_POINT('Ctrl Pts',(127.059226565942,7.75844304239001,63.3241530267836));
#185043=CARTESIAN_POINT('Ctrl Pts',(129.239582133274,1.10645410506801,63.6688842131738));
#185044=CARTESIAN_POINT('Ctrl Pts',(128.106954986187,-5.80363648426999,
63.369633581726));
#185045=CARTESIAN_POINT('Ctrl Pts',(123.929007928104,-11.35991752694,62.4784297705705));
#185046=CARTESIAN_POINT('Ctrl Pts',(117.683781956121,-14.26628030825,61.1853856397628));
#185047=CARTESIAN_POINT('Ctrl Pts',(110.831554451127,-13.84475865714,59.7743517745333));
#185048=CARTESIAN_POINT('Ctrl Pts',(104.97418281375,-10.1936855606,58.5566992654099));
#185049=CARTESIAN_POINT('Ctrl Pts',(101.481510194244,-4.16472522390098,
57.7986999761932));
#185050=CARTESIAN_POINT('Ctrl Pts',(101.171563275794,2.83568239863401,57.6593629799186));
#185051=CARTESIAN_POINT('Ctrl Pts',(104.120702353602,9.17481693560401,58.1535312884639));
#185052=CARTESIAN_POINT('Ctrl Pts',(107.801692072279,11.97359728549,58.8163206999831));
#185053=CARTESIAN_POINT('Ctrl Pts',(109.858223050957,12.85354385943,59.1897087829625));
#185054=CARTESIAN_POINT('',(114.640971711999,-13.3588720674388,62.9464971841653));
#185055=CARTESIAN_POINT('',(106.597794810055,10.1748376800446,58.9494679941055));
#185056=CARTESIAN_POINT('Ctrl Pts',(114.640904788072,-13.357524695892,62.9468179160091));
#185057=CARTESIAN_POINT('Ctrl Pts',(114.13304666145,-13.3578942130633,62.8417580704295));
#185058=CARTESIAN_POINT('Ctrl Pts',(113.625151177201,-13.3283693476066,
62.7366625756605));
#185059=CARTESIAN_POINT('Ctrl Pts',(112.651945528154,-13.2132690486779,
62.5351724262472));
#185060=CARTESIAN_POINT('Ctrl Pts',(112.185897821086,-13.131779068876,62.438598105965));
#185061=CARTESIAN_POINT('Ctrl Pts',(110.86466155124,-12.8224878570432,62.1648732340489));
#185062=CARTESIAN_POINT('Ctrl Pts',(110.025581150313,-12.5309381011058,
61.9911471537562));
#185063=CARTESIAN_POINT('Ctrl Pts',(108.546930020057,-11.842867295222,61.6840357448642));
#185064=CARTESIAN_POINT('Ctrl Pts',(107.896456525995,-11.4698948337182,
61.548539340477));
#185065=CARTESIAN_POINT('Ctrl Pts',(106.939222074391,-10.8062052962347,
61.347910397855));
#185066=CARTESIAN_POINT('Ctrl Pts',(106.607799893718,-10.5521992865497,
61.2781728990859));
#185067=CARTESIAN_POINT('Ctrl Pts',(106.121768221915,-10.1408419147875,
61.1754516486887));
#185068=CARTESIAN_POINT('Ctrl Pts',(105.957880515477,-9.99482870805906,
61.140751262454));
#185069=CARTESIAN_POINT('Ctrl Pts',(105.612695754859,-9.67101177218622,
61.0676578688006));
#185070=CARTESIAN_POINT('Ctrl Pts',(105.432895117018,-9.49210227679692,
61.0295659988766));
#185071=CARTESIAN_POINT('Ctrl Pts',(104.832010780966,-8.85843031270054,
60.9021190377937));
#185072=CARTESIAN_POINT('Ctrl Pts',(104.436926515002,-8.37796342960463,
60.8180630804526));
#185073=CARTESIAN_POINT('Ctrl Pts',(103.741955795032,-7.40238028037761,
60.6689588910643));
#185074=CARTESIAN_POINT('Ctrl Pts',(103.437181924747,-6.91072317790111,
60.6029579528933));
#185075=CARTESIAN_POINT('Ctrl Pts',(103.043287231502,-6.17374123906158,
60.5162504514931));
#185076=CARTESIAN_POINT('Ctrl Pts',(102.928200845802,-5.9427688350452,60.4907002080805));
#185077=CARTESIAN_POINT('Ctrl Pts',(102.699405821129,-5.44847187495716,
60.439368713644));
#185078=CARTESIAN_POINT('Ctrl Pts',(102.587263172405,-5.18439711493227,
60.4138551208945));
#185079=CARTESIAN_POINT('Ctrl Pts',(102.397216298565,-4.69348794710408,
60.3700056759946));
#185080=CARTESIAN_POINT('Ctrl Pts',(102.316716708879,-4.46771302769359,
60.3511964766176));
#185081=CARTESIAN_POINT('Ctrl Pts',(102.185025218202,-4.06408315937053,
60.3201206455682));
#185082=CARTESIAN_POINT('Ctrl Pts',(102.131448804967,-3.88739373852614,
60.3073740468952));
#185083=CARTESIAN_POINT('Ctrl Pts',(102.029090310271,-3.52270003785181,
60.2827933355699));
#185084=CARTESIAN_POINT('Ctrl Pts',(101.980712552168,-3.3346608650091,60.2710403841923));
#185085=CARTESIAN_POINT('Ctrl Pts',(101.798178471838,-2.55578924910197,
60.2260349284972));
#185086=CARTESIAN_POINT('Ctrl Pts',(101.699610622787,-1.95619866277338,
60.2000300640393));
#185087=CARTESIAN_POINT('Ctrl Pts',(101.610625441262,-1.03983478435559,
60.172252824418));
#185088=CARTESIAN_POINT('Ctrl Pts',(101.590977191464,-0.726006611478508,
60.1648406494029));
#185089=CARTESIAN_POINT('Ctrl Pts',(101.57531060063,-0.172071079279196,
60.1553272403031));
#185090=CARTESIAN_POINT('Ctrl Pts',(101.574798965633,0.0679138644798712,
60.1523838865166));
#185091=CARTESIAN_POINT('Ctrl Pts',(101.584821993279,0.483796087568609,
60.1492814152502));
#185092=CARTESIAN_POINT('Ctrl Pts',(101.592454895292,0.659766305083154,
60.1485899668375));
#185093=CARTESIAN_POINT('Ctrl Pts',(101.621674565384,1.12527544274108,60.1483860600609));
#185094=CARTESIAN_POINT('Ctrl Pts',(101.649105093071,1.41444195504571,60.1499043701699));
#185095=CARTESIAN_POINT('Ctrl Pts',(101.72091325271,1.97807314072567,60.1563133725514));
#185096=CARTESIAN_POINT('Ctrl Pts',(101.764513908999,2.25262977683502,60.1610657767085));
#185097=CARTESIAN_POINT('Ctrl Pts',(101.84054682363,2.65099254421983,60.1705467407519));
#185098=CARTESIAN_POINT('Ctrl Pts',(101.866287086771,2.77610820298583,60.173901059286));
#185099=CARTESIAN_POINT('Ctrl Pts',(101.923255407581,3.03413364715345,60.181627688659));
#185100=CARTESIAN_POINT('Ctrl Pts',(101.954735519064,3.16697189908343,60.1860533901494));
#185101=CARTESIAN_POINT('Ctrl Pts',(102.029106806634,3.46071636523449,60.1968163652399));
#185102=CARTESIAN_POINT('Ctrl Pts',(102.072983375827,3.62136124193086,60.2033598051749));
#185103=CARTESIAN_POINT('Ctrl Pts',(102.255161442947,4.24285204003838,60.2311772757719));
#185104=CARTESIAN_POINT('Ctrl Pts',(102.415166968247,4.69712640278496,60.2569152596301));
#185105=CARTESIAN_POINT('Ctrl Pts',(102.771763089177,5.5610456371751,60.3157856608415));
#185106=CARTESIAN_POINT('Ctrl Pts',(102.965847169219,5.97181244352332,60.3484295301969));
#185107=CARTESIAN_POINT('Ctrl Pts',(103.258015477615,6.51787531835683,60.3979413406901));
#185108=CARTESIAN_POINT('Ctrl Pts',(103.338934764958,6.66268499607493,60.4116872955399));
#185109=CARTESIAN_POINT('Ctrl Pts',(103.491557146343,6.92442733874645,60.4376497680994));
#185110=CARTESIAN_POINT('Ctrl Pts',(103.562438951009,7.04185656772653,60.4497205345221));
#185111=CARTESIAN_POINT('Ctrl Pts',(103.884876156801,7.55811042508076,60.5046572184889));
#185112=CARTESIAN_POINT('Ctrl Pts',(104.155453484377,7.94472372294211,60.5508111381471));
#185113=CARTESIAN_POINT('Ctrl Pts',(104.626711861602,8.54730141158604,60.6321141893237));
#185114=CARTESIAN_POINT('Ctrl Pts',(104.815519761776,8.7728585396044,60.6648944677146));
#185115=CARTESIAN_POINT('Ctrl Pts',(105.089172256251,9.07824165106905,60.7128567585429));
#185116=CARTESIAN_POINT('Ctrl Pts',(105.167794290818,9.16365274147528,60.7266871712758));
#185117=CARTESIAN_POINT('Ctrl Pts',(105.338775798923,9.34450156421968,60.7568670518337));
#185118=CARTESIAN_POINT('Ctrl Pts',(105.431442676693,9.43957023304213,60.7732841223262));
#185119=CARTESIAN_POINT('Ctrl Pts',(105.719210938087,9.72598188051344,60.8244230471412));
#185120=CARTESIAN_POINT('Ctrl Pts',(105.918820637734,9.91261159695927,60.860110349335));
#185121=CARTESIAN_POINT('Ctrl Pts',(106.45767539947,10.3860623669133,60.9568062099594));
#185122=CARTESIAN_POINT('Ctrl Pts',(106.805938440753,10.6622590205496,61.0196502005837));
#185123=CARTESIAN_POINT('Ctrl Pts',(107.37130808444,11.0663362138372,61.1216993410473));
#185124=CARTESIAN_POINT('Ctrl Pts',(107.579862313223,11.2066305252831,61.1593489157711));
#185125=CARTESIAN_POINT('Ctrl Pts',(107.900203246337,11.4091694152764,61.2171031647627));
#185126=CARTESIAN_POINT('Ctrl Pts',(108.009233602305,11.4759194192547,61.2367474916503));
#185127=CARTESIAN_POINT('Ctrl Pts',(108.223838497537,11.6030718995451,61.2753750687715));
#185128=CARTESIAN_POINT('Ctrl Pts',(108.329326260351,11.6636251040241,61.2943427192708));
#185129=CARTESIAN_POINT('Ctrl Pts',(108.71838722681,11.8798753972669,61.3642350011784));
#185130=CARTESIAN_POINT('Ctrl Pts',(109.006819513345,12.0266019269427,61.4159368321564));
#185131=CARTESIAN_POINT('Ctrl Pts',(109.589614463954,12.2964189745832,61.5204772214287));
#185132=CARTESIAN_POINT('Ctrl Pts',(109.883857650602,12.4197975079218,61.5732939196274));
#185133=CARTESIAN_POINT('Ctrl Pts',(110.366124575335,12.6013301593778,61.6601501351901));
#185134=CARTESIAN_POINT('Ctrl Pts',(110.551650540504,12.6663619514185,61.6936304822));
#185135=CARTESIAN_POINT('Ctrl Pts',(110.837901980005,12.7593314357167,61.7454400582351));
#185136=CARTESIAN_POINT('Ctrl Pts',(110.937582650568,12.7903554986743,61.763510348273));
#185137=CARTESIAN_POINT('Ctrl Pts',(111.157239307974,12.8557592462737,61.8033958907701));
#185138=CARTESIAN_POINT('Ctrl Pts',(111.277248983378,12.8895799988415,61.8252280723137));
#185139=CARTESIAN_POINT('Ctrl Pts',(111.731759509055,13.0105293791575,61.9080350703606));
#185140=CARTESIAN_POINT('Ctrl Pts',(112.069249071377,13.0858417092473,61.9697709998442));
#185141=CARTESIAN_POINT('Ctrl Pts',(112.748917318068,13.2092406064118,62.094238900772));
#185142=CARTESIAN_POINT('Ctrl Pts',(113.091094796768,13.2573335129592,62.1569699886093));
#185143=CARTESIAN_POINT('Ctrl Pts',(113.646626204469,13.3130789845115,62.2586363878786));
#185144=CARTESIAN_POINT('Ctrl Pts',(113.859163680795,13.3291654628939,62.2974904189975));
#185145=CARTESIAN_POINT('Ctrl Pts',(114.183570544218,13.3457674206309,62.3566696298158));
#185146=CARTESIAN_POINT('Ctrl Pts',(114.2952469085,13.3500498490439,62.3770192560691));
#185147=CARTESIAN_POINT('Ctrl Pts',(114.531678159406,13.3560865719153,62.420042125316));
#185148=CARTESIAN_POINT('Ctrl Pts',(114.656443115949,13.3574887819261,62.4427111977239));
#185149=CARTESIAN_POINT('Ctrl Pts',(115.114235986337,13.3560888231383,62.52579022643));
#185150=CARTESIAN_POINT('Ctrl Pts',(115.447276730587,13.3423610169083,62.5860363662682));
#185151=CARTESIAN_POINT('Ctrl Pts',(116.122663385045,13.2885137617653,62.7081014206246));
#185152=CARTESIAN_POINT('Ctrl Pts',(116.464959387862,13.2475121823014,62.7699081560095));
#185153=CARTESIAN_POINT('Ctrl Pts',(117.014012552028,13.1592593830363,62.8692040249979));
#185154=CARTESIAN_POINT('Ctrl Pts',(117.222101108764,13.120524924425,62.906873359065));
#185155=CARTESIAN_POINT('Ctrl Pts',(117.536777166574,13.0537945091799,62.9639462656728));
#185156=CARTESIAN_POINT('Ctrl Pts',(117.644142120415,13.0295682205426,62.9834384668156));
#185157=CARTESIAN_POINT('Ctrl Pts',(117.862349572319,12.977330759556,63.0231033782953));
#185158=CARTESIAN_POINT('Ctrl Pts',(117.973119772814,12.9492193191486,63.0432657062975));
#185159=CARTESIAN_POINT('Ctrl Pts',(118.321955664972,12.8556772957132,63.1068242587273));
#185160=CARTESIAN_POINT('Ctrl Pts',(118.55861118124,12.7847812121831,63.1500375013425));
#185161=CARTESIAN_POINT('Ctrl Pts',(119.158344923045,12.5861951733289,63.2596032859501));
#185162=CARTESIAN_POINT('Ctrl Pts',(119.518326470209,12.4488839811277,63.3254202861066));
#185163=CARTESIAN_POINT('Ctrl Pts',(120.014884681342,12.2340275500708,63.4158869726836));
#185164=CARTESIAN_POINT('Ctrl Pts',(120.156909005605,12.1695513992125,63.4417238991393));
#185165=CARTESIAN_POINT('Ctrl Pts',(120.414002169005,12.0472973300729,63.4883905620043));
#185166=CARTESIAN_POINT('Ctrl Pts',(120.529438477687,11.9903221868223,63.5093047926723));
#185167=CARTESIAN_POINT('Ctrl Pts',(120.74971540413,11.8775798137548,63.5491210550845));
#185168=CARTESIAN_POINT('Ctrl Pts',(120.854678807306,11.8220657143635,63.5680542592931));
#185169=CARTESIAN_POINT('Ctrl Pts',(121.139737692372,11.66636932674,63.6193774817783));
#185170=CARTESIAN_POINT('Ctrl Pts',(121.318348492923,11.5633469345845,63.6514294780892));
#185171=CARTESIAN_POINT('Ctrl Pts',(121.936950761117,11.1870749230793,63.7621547519484));
#185172=CARTESIAN_POINT('Ctrl Pts',(122.364104677741,10.8918150597322,63.8380952042949));
#185173=CARTESIAN_POINT('Ctrl Pts',(122.982618292788,10.4079138296809,63.9478893155293));
#185174=CARTESIAN_POINT('Ctrl Pts',(123.187627201529,10.2372507000208,63.9842507749081));
#185175=CARTESIAN_POINT('Ctrl Pts',(123.482893485197,9.97569886736661,64.0366568474352));
#185176=CARTESIAN_POINT('Ctrl Pts',(123.577259438626,9.88960137156063,64.0534113238723));
#185177=CARTESIAN_POINT('Ctrl Pts',(123.75454575661,9.72297861908504,64.0849101284806));
#185178=CARTESIAN_POINT('Ctrl Pts',(123.837624325387,9.6427765129703,64.099681658678));
#185179=CARTESIAN_POINT('Ctrl Pts',(124.24254908312,9.24124425607086,64.1717294617124));
#185180=CARTESIAN_POINT('Ctrl Pts',(124.548743051469,8.90393366013752,64.2263481457952));
#185181=CARTESIAN_POINT('Ctrl Pts',(125.036109703474,8.30848060673347,64.3126758184803));
#185182=CARTESIAN_POINT('Ctrl Pts',(125.22659224287,8.0582513325356,64.3462334918513));
#185183=CARTESIAN_POINT('Ctrl Pts',(125.484113128596,7.69433067021073,64.3910974689351));
#185184=CARTESIAN_POINT('Ctrl Pts',(125.558442486502,7.58598438779627,64.4039811197604));
#185185=CARTESIAN_POINT('Ctrl Pts',(125.717542070755,7.34670631634288,64.4314222542772));
#185186=CARTESIAN_POINT('Ctrl Pts',(125.801673439851,7.21533075686617,64.4458436783326));
#185187=CARTESIAN_POINT('Ctrl Pts',(126.171376844117,6.61557940636577,64.5088411145553));
#185188=CARTESIAN_POINT('Ctrl Pts',(126.431326233362,6.13076090329836,64.5520786961174));
#185189=CARTESIAN_POINT('Ctrl Pts',(126.780279820338,5.37293252424908,64.6089238011067));
#185190=CARTESIAN_POINT('Ctrl Pts',(126.89133380384,5.11032410667716,64.6267754663688));
#185191=CARTESIAN_POINT('Ctrl Pts',(127.069193557119,4.64946524302802,64.6550099767178));
#185192=CARTESIAN_POINT('Ctrl Pts',(127.139894121765,4.45276366113968,64.6661139986393));
#185193=CARTESIAN_POINT('Ctrl Pts',(127.249195142221,4.12464289832333,64.6831011863358));
#185194=CARTESIAN_POINT('Ctrl Pts',(127.290449168039,3.99413725472788,64.6894630103175));
#185195=CARTESIAN_POINT('Ctrl Pts',(127.375043346053,3.71135019989342,64.7024063481235));
#185196=CARTESIAN_POINT('Ctrl Pts',(127.417619770423,3.55911024014224,64.7088585538984));
#185197=CARTESIAN_POINT('Ctrl Pts',(127.557327739738,3.02279510302719,64.7297541786284));
#185198=CARTESIAN_POINT('Ctrl Pts',(127.640055702074,2.63503439590416,64.7415833085844));
#185199=CARTESIAN_POINT('Ctrl Pts',(127.732353209115,2.08601699603026,64.7533664684811));
#185200=CARTESIAN_POINT('Ctrl Pts',(127.75616800248,1.92723139664744,64.7561986023379));
#185201=CARTESIAN_POINT('Ctrl Pts',(127.799126716805,1.60195605970232,64.7607857850457));
#185202=CARTESIAN_POINT('Ctrl Pts',(127.818021103159,1.43543230925132,64.7624898441099));
#185203=CARTESIAN_POINT('Ctrl Pts',(127.851832881245,1.07953660699374,64.7647801264296));
#185204=CARTESIAN_POINT('Ctrl Pts',(127.86588332986,0.890077168074348,64.7651868304453));
#185205=CARTESIAN_POINT('Ctrl Pts',(127.906290085679,0.133790222627718,
64.7636271346906));
#185206=CARTESIAN_POINT('Ctrl Pts',(127.901608590714,-0.434766238665586,
64.7553360502631));
#185207=CARTESIAN_POINT('Ctrl Pts',(127.839502281003,-1.31798964527625,
64.7318073303138));
#185208=CARTESIAN_POINT('Ctrl Pts',(127.80613617809,-1.63455218091816,64.7212178660795));
#185209=CARTESIAN_POINT('Ctrl Pts',(127.728443943764,-2.18501095480177,
64.6990792097848));
#185210=CARTESIAN_POINT('Ctrl Pts',(127.68899934161,-2.41963383820523,64.688444509012));
#185211=CARTESIAN_POINT('Ctrl Pts',(127.610990645598,-2.81833512942862,
64.6683297623307));
#185212=CARTESIAN_POINT('Ctrl Pts',(127.575520933379,-2.98304090406737,
64.6594166434494));
#185213=CARTESIAN_POINT('Ctrl Pts',(127.463920336948,-3.45712537536408,
64.6320123940435));
#185214=CARTESIAN_POINT('Ctrl Pts',(127.379834488355,-3.76392998567303,
64.6121221090456));
#185215=CARTESIAN_POINT('Ctrl Pts',(127.185593936981,-4.38521353303955,
64.5670997996144));
#185216=CARTESIAN_POINT('Ctrl Pts',(127.074289841842,-4.69952565835987,
64.5417087831309));
#185217=CARTESIAN_POINT('Ctrl Pts',(126.864801569003,-5.22840183646511,
64.4942934614358));
#185218=CARTESIAN_POINT('Ctrl Pts',(126.772266854945,-5.44530138853266,
64.473468394417));
#185219=CARTESIAN_POINT('Ctrl Pts',(126.354258986003,-6.35860802414336,
64.3799200115085));
#185220=CARTESIAN_POINT('Ctrl Pts',(125.975394107594,-7.02968604150785,
64.2963647961218));
#185221=CARTESIAN_POINT('Ctrl Pts',(125.357727517744,-7.934022287407,64.1623214125837));
#185222=CARTESIAN_POINT('Ctrl Pts',(125.162470146833,-8.19848977855258,
64.1201938050918));
#185223=CARTESIAN_POINT('Ctrl Pts',(124.79007615719,-8.66546649467137,64.0403457523059));
#185224=CARTESIAN_POINT('Ctrl Pts',(124.616034928297,-8.87053820418804,
64.0032033395742));
#185225=CARTESIAN_POINT('Ctrl Pts',(124.256206717355,-9.26882654474569,
63.9267898520112));
#185226=CARTESIAN_POINT('Ctrl Pts',(124.070968901256,-9.46148931235269,
63.8876533053748));
#185227=CARTESIAN_POINT('Ctrl Pts',(123.639997309396,-9.88272035615241,
63.7969049457651));
#185228=CARTESIAN_POINT('Ctrl Pts',(123.391662550018,-10.1073027448131,
63.7447495300018));
#185229=CARTESIAN_POINT('Ctrl Pts',(122.806595195361,-10.5971434142374,
63.6219157172491));
#185230=CARTESIAN_POINT('Ctrl Pts',(122.464700240288,-10.8559748928838,
63.5502163113335));
#185231=CARTESIAN_POINT('Ctrl Pts',(121.621751717589,-11.4319571617041,
63.3736837492754));
#185232=CARTESIAN_POINT('Ctrl Pts',(121.110087858341,-11.7331363248134,
63.2667199064968));
#185233=CARTESIAN_POINT('Ctrl Pts',(119.932002719735,-12.3232369511335,
63.0210355140993));
#185234=CARTESIAN_POINT('Ctrl Pts',(119.256658901038,-12.5939329065661,
62.8805888329962));
#185235=CARTESIAN_POINT('Ctrl Pts',(118.209943403202,-12.9126257556509,
62.6637175782328));
#185236=CARTESIAN_POINT('Ctrl Pts',(117.852842553851,-13.0043295678821,
62.589882982709));
#185237=CARTESIAN_POINT('Ctrl Pts',(115.837578810976,-13.4295284185426,
62.1731546981305));
#185238=CARTESIAN_POINT('Ctrl Pts',(114.114959940367,-13.4482587470028,
61.8173097145917));
#185239=CARTESIAN_POINT('Ctrl Pts',(112.03054112538,-13.0573242410817,61.3854465567167));
#185240=CARTESIAN_POINT('Ctrl Pts',(111.611477861188,-12.9566211394342,
61.2985227316503));
#185241=CARTESIAN_POINT('Ctrl Pts',(110.397387606598,-12.5975714198071,
61.0467081907155));
#185242=CARTESIAN_POINT('Ctrl Pts',(109.620181202009,-12.2815155199788,
60.8855747287923));
#185243=CARTESIAN_POINT('Ctrl Pts',(108.189127318744,-11.5333105127569,
60.5879512297827));
#185244=CARTESIAN_POINT('Ctrl Pts',(107.530223181635,-11.1105921007965,
60.4504708231738));
#185245=CARTESIAN_POINT('Ctrl Pts',(106.565391608009,-10.3626609457922,
60.2477237874993));
#185246=CARTESIAN_POINT('Ctrl Pts',(106.230927857509,-10.0754372090119,
60.1771151717748));
#185247=CARTESIAN_POINT('Ctrl Pts',(105.755854574157,-9.62344263598964,
60.0762812382923));
#185248=CARTESIAN_POINT('Ctrl Pts',(105.603627976406,-9.47124093647704,
60.0438999584807));
#185249=CARTESIAN_POINT('Ctrl Pts',(105.28542516852,-9.1367100684019,59.9761891014369));
#185250=CARTESIAN_POINT('Ctrl Pts',(105.12078442685,-8.95342524094493,59.9411296926167));
#185251=CARTESIAN_POINT('Ctrl Pts',(104.484015436306,-8.20311836289615,
59.8053438764008));
#185252=CARTESIAN_POINT('Ctrl Pts',(104.053206909363,-7.59951364863668,
59.7130424172221));
#185253=CARTESIAN_POINT('Ctrl Pts',(103.493058578304,-6.6606480910518,59.5913850382532));
#185254=CARTESIAN_POINT('Ctrl Pts',(103.323834555591,-6.35003030243997,
59.5543429022173));
#185255=CARTESIAN_POINT('Ctrl Pts',(103.040169531912,-5.77712997366257,
59.4915643561494));
#185256=CARTESIAN_POINT('Ctrl Pts',(102.9214432161,-5.51702662733298,59.465021842453));
#185257=CARTESIAN_POINT('Ctrl Pts',(102.71687156982,-5.02842043346527,59.4186921025178));
#185258=CARTESIAN_POINT('Ctrl Pts',(102.628756185847,-4.80089832486037,
59.398485087806));
#185259=CARTESIAN_POINT('Ctrl Pts',(102.466176581298,-4.34458733978355,
59.3606248610168));
#185260=CARTESIAN_POINT('Ctrl Pts',(102.391532211094,-4.11586718307708,
59.3429390963345));
#185261=CARTESIAN_POINT('Ctrl Pts',(102.247983228326,-3.63207010985547,
59.308411029996));
#185262=CARTESIAN_POINT('Ctrl Pts',(102.180341702018,-3.37658064438319,
59.2918239647526));
#185263=CARTESIAN_POINT('Ctrl Pts',(102.081029130435,-2.95018503945331,
59.2670271651299));
#185264=CARTESIAN_POINT('Ctrl Pts',(102.045067128554,-2.78091983344021,
59.2579110564241));
#185265=CARTESIAN_POINT('Ctrl Pts',(101.962162099715,-2.34991924665055,
59.2364929455991));
#185266=CARTESIAN_POINT('Ctrl Pts',(101.919676027197,-2.08728907043755,
59.2251050769411));
#185267=CARTESIAN_POINT('Ctrl Pts',(101.834493987048,-1.44103113278861,
59.2009941404104));
#185268=CARTESIAN_POINT('Ctrl Pts',(101.800331278556,-1.05620878670474,
59.1899818655806));
#185269=CARTESIAN_POINT('Ctrl Pts',(101.761585684893,-0.222212896363878,
59.1729668446853));
#185270=CARTESIAN_POINT('Ctrl Pts',(101.762717532769,0.227301074504134,
59.1680686407415));
#185271=CARTESIAN_POINT('Ctrl Pts',(101.796075427552,0.87503831262595,59.1668789481708));
#185272=CARTESIAN_POINT('Ctrl Pts',(101.81068659318,1.07420437693522,59.1673186852143));
#185273=CARTESIAN_POINT('Ctrl Pts',(101.846198155655,1.44654474799569,59.1696260495175));
#185274=CARTESIAN_POINT('Ctrl Pts',(101.866069156421,1.6198226259679,59.1713059851813));
#185275=CARTESIAN_POINT('Ctrl Pts',(101.911383702352,1.95758477126266,59.1757530132773));
#185276=CARTESIAN_POINT('Ctrl Pts',(101.936531992671,2.12210891398788,59.1784643348455));
#185277=CARTESIAN_POINT('Ctrl Pts',(102.031055909962,2.6725213419252,59.1894571603034));
#185278=CARTESIAN_POINT('Ctrl Pts',(102.114153895364,3.0559900424101,59.2003078888467));
#185279=CARTESIAN_POINT('Ctrl Pts',(102.253498585011,3.5853398825905,59.2203022328071));
#185280=CARTESIAN_POINT('Ctrl Pts',(102.295647488564,3.73478678808129,59.2265221875798));
#185281=CARTESIAN_POINT('Ctrl Pts',(102.381229485447,4.01907104596501,59.2394736579373));
#185282=CARTESIAN_POINT('Ctrl Pts',(102.424134919428,4.15379101364896,59.2460946161624));
#185283=CARTESIAN_POINT('Ctrl Pts',(102.542551928911,4.50624815897289,59.2646659863145));
#185284=CARTESIAN_POINT('Ctrl Pts',(102.621562993342,4.72276527838593,59.2773442539343));
#185285=CARTESIAN_POINT('Ctrl Pts',(102.964754595082,5.59347480677453,59.3333488940382));
#185286=CARTESIAN_POINT('Ctrl Pts',(103.274674513585,6.22910346089313,59.385943733931));
#185287=CARTESIAN_POINT('Ctrl Pts',(103.732364324106,7.00825960094132,59.4644574231797));
#185288=CARTESIAN_POINT('Ctrl Pts',(103.837151023302,7.17797672653731,59.4824788168627));
#185289=CARTESIAN_POINT('Ctrl Pts',(104.020560831428,7.4608774878375,59.5140596166069));
#185290=CARTESIAN_POINT('Ctrl Pts',(104.097275873635,7.57534131046127,59.527279257401));
#185291=CARTESIAN_POINT('Ctrl Pts',(104.273213723829,7.82935854437856,59.5576041448866));
#185292=CARTESIAN_POINT('Ctrl Pts',(104.373373062807,7.96824228242872,59.57486702255));
#185293=CARTESIAN_POINT('Ctrl Pts',(104.711478063147,8.41867106841112,59.6331863903608));
#185294=CARTESIAN_POINT('Ctrl Pts',(104.960416178103,8.72171765659465,59.6762105652636));
#185295=CARTESIAN_POINT('Ctrl Pts',(105.38747103816,9.19694853716043,59.7506355611185));
#185296=CARTESIAN_POINT('Ctrl Pts',(105.557930481459,9.37624280645495,59.7804861710088));
#185297=CARTESIAN_POINT('Ctrl Pts',(105.816303686599,9.63297574535571,59.8260468283476));
#185298=CARTESIAN_POINT('Ctrl Pts',(105.900332501203,9.71424556620526,59.840912503126));
#185299=CARTESIAN_POINT('Ctrl Pts',(106.079180881687,9.88261487660262,59.8726521429693));
#185300=CARTESIAN_POINT('Ctrl Pts',(106.174146425296,9.96939657171607,59.8895602644886));
#185301=CARTESIAN_POINT('Ctrl Pts',(106.470262730222,10.2320900527407,59.9424259455987));
#185302=CARTESIAN_POINT('Ctrl Pts',(106.675495992491,10.4032103926802,59.9792654642311));
#185303=CARTESIAN_POINT('Ctrl Pts',(107.292909532275,10.8870065603853,60.0904594425795));
#185304=CARTESIAN_POINT('Ctrl Pts',(107.718584203814,11.1818520194149,60.1675803068146));
#185305=CARTESIAN_POINT('Ctrl Pts',(108.340583859555,11.5610238326694,60.2801760033078));
#185306=CARTESIAN_POINT('Ctrl Pts',(108.524180022238,11.6669882992912,60.3134002252302));
#185307=CARTESIAN_POINT('Ctrl Pts',(108.81701691476,11.8267595165838,60.3663234140233));
#185308=CARTESIAN_POINT('Ctrl Pts',(108.924666048635,11.883579416695,60.3857640028567));
#185309=CARTESIAN_POINT('Ctrl Pts',(109.147469865246,11.9972733932899,60.425958637828));
#185310=CARTESIAN_POINT('Ctrl Pts',(109.262709192914,12.0539752970978,60.4467233268338));
#185311=CARTESIAN_POINT('Ctrl Pts',(109.51836357355,12.1751596859855,60.4927474071913));
#185312=CARTESIAN_POINT('Ctrl Pts',(109.659131381816,12.2388786151289,60.5180632099643));
#185313=CARTESIAN_POINT('Ctrl Pts',(110.152966684795,12.4519996258401,60.6068411387627));
#185314=CARTESIAN_POINT('Ctrl Pts',(110.511477807722,12.5884291439847,60.6712321388829));
#185315=CARTESIAN_POINT('Ctrl Pts',(111.110761189675,12.7865223416564,60.7791792956319));
#185316=CARTESIAN_POINT('Ctrl Pts',(111.348534779621,12.8575951696771,60.8220871967081));
#185317=CARTESIAN_POINT('Ctrl Pts',(111.696982298278,12.9507766116275,60.8851758595882));
#185318=CARTESIAN_POINT('Ctrl Pts',(111.806257456764,12.9784523627262,60.9049904016825));
#185319=CARTESIAN_POINT('Ctrl Pts',(112.024768640315,13.030698595976,60.9446820508834));
#185320=CARTESIAN_POINT('Ctrl Pts',(112.133934046305,13.0552773269553,60.9645446522991));
#185321=CARTESIAN_POINT('Ctrl Pts',(112.460585923521,13.1243201292389,61.0240600354854));
#185322=CARTESIAN_POINT('Ctrl Pts',(112.678919291209,13.1645424546652,61.0639469246329));
#185323=CARTESIAN_POINT('Ctrl Pts',(113.27156198627,13.2579522062865,61.1723764068122));
#185324=CARTESIAN_POINT('Ctrl Pts',(113.647491875916,13.3003406800254,61.2413280404868));
#185325=CARTESIAN_POINT('Ctrl Pts',(114.323869233451,13.3469353335515,61.3652690251981));
#185326=CARTESIAN_POINT('Ctrl Pts',(114.623923271277,13.3572098583343,61.4202100941643));
#185327=CARTESIAN_POINT('Ctrl Pts',(115.046956661045,13.3571445088591,61.4974474842622));
#185328=CARTESIAN_POINT('Ctrl Pts',(115.169925101734,13.3553924193983,61.5198727043834));
#185329=CARTESIAN_POINT('Ctrl Pts',(115.405198708932,13.348725025691,61.5627134105093));
#185330=CARTESIAN_POINT('Ctrl Pts',(115.517510728658,13.3440949431127,61.5831347218507));
#185331=CARTESIAN_POINT('Ctrl Pts',(115.85758979214,13.3256873097016,61.644894804552));
#185332=CARTESIAN_POINT('Ctrl Pts',(116.085139378964,13.3073995152239,61.6861169571957));
#185333=CARTESIAN_POINT('Ctrl Pts',(116.713262388815,13.2403213543822,61.7997441406783));
#185334=CARTESIAN_POINT('Ctrl Pts',(117.112572439651,13.1788886262657,61.871796494688));
#185335=CARTESIAN_POINT('Ctrl Pts',(117.769680192754,13.0460469723418,61.9904708841293));
#185336=CARTESIAN_POINT('Ctrl Pts',(118.029533828077,12.9850907459908,62.0374286321465));
#185337=CARTESIAN_POINT('Ctrl Pts',(118.404079829578,12.8847539166844,62.1052535833919));
#185338=CARTESIAN_POINT('Ctrl Pts',(118.520445138148,12.8518033841174,62.1263457761989));
#185339=CARTESIAN_POINT('Ctrl Pts',(118.737422001928,12.7869995035274,62.1657239844516));
#185340=CARTESIAN_POINT('Ctrl Pts',(118.838040288695,12.7555738559908,62.1840062924034));
#185341=CARTESIAN_POINT('Ctrl Pts',(119.137574327383,12.6579173529554,62.2384868131258));
#185342=CARTESIAN_POINT('Ctrl Pts',(119.335274950334,12.5880145499723,62.2745161405742));
#185343=CARTESIAN_POINT('Ctrl Pts',(119.869220579337,12.3844301842922,62.3718950442556));
#185344=CARTESIAN_POINT('Ctrl Pts',(120.201944627898,12.2412666976497,62.4326547766958));
#185345=CARTESIAN_POINT('Ctrl Pts',(120.773855900682,11.9666068003245,62.5368216568667));
#185346=CARTESIAN_POINT('Ctrl Pts',(121.01578349039,11.8410179525605,62.5807963174894));
#185347=CARTESIAN_POINT('Ctrl Pts',(121.358280630884,11.6495832185981,62.6427789639281));
#185348=CARTESIAN_POINT('Ctrl Pts',(121.462064458879,11.5897146565807,62.661522730782));
#185349=CARTESIAN_POINT('Ctrl Pts',(121.673215832394,11.4640744742082,62.6995707144856));
#185350=CARTESIAN_POINT('Ctrl Pts',(121.780499512891,11.3981577294354,62.7188574787436));
#185351=CARTESIAN_POINT('Ctrl Pts',(122.101041998008,11.1948906646997,62.7763631439923));
#185352=CARTESIAN_POINT('Ctrl Pts',(122.311464895034,11.0528735255313,62.8139510442209));
#185353=CARTESIAN_POINT('Ctrl Pts',(122.893478721781,10.635360077766,62.9175878177493));
#185354=CARTESIAN_POINT('Ctrl Pts',(123.255529262677,10.3460087821746,62.9816631022324));
#185355=CARTESIAN_POINT('Ctrl Pts',(123.794068310345,9.86709086608706,63.0768008267119));
#185356=CARTESIAN_POINT('Ctrl Pts',(123.981558507471,9.69027869162565,63.10988691107));
#185357=CARTESIAN_POINT('Ctrl Pts',(124.253864150465,9.41782771610808,63.1579586157631));
#185358=CARTESIAN_POINT('Ctrl Pts',(124.342683808822,9.32632345901294,63.1736415257899));
#185359=CARTESIAN_POINT('Ctrl Pts',(124.510575252109,9.14818441900784,63.203302918294));
#185360=CARTESIAN_POINT('Ctrl Pts',(124.589777868112,9.06183428159915,63.2173044726143));
#185361=CARTESIAN_POINT('Ctrl Pts',(124.902783268493,8.71115180496017,63.2726704095001));
#185362=CARTESIAN_POINT('Ctrl Pts',(125.127074376163,8.438311997959,63.3124029319295));
#185363=CARTESIAN_POINT('Ctrl Pts',(125.570375822247,7.85306020050244,63.3905698715235));
#185364=CARTESIAN_POINT('Ctrl Pts',(125.787562475328,7.5392381035402,63.4286513981591));
#185365=CARTESIAN_POINT('Ctrl Pts',(126.06390060534,7.10159865812917,63.4763939227996));
#185366=CARTESIAN_POINT('Ctrl Pts',(126.134809761169,6.98547006954439,63.4885714921778));
#185367=CARTESIAN_POINT('Ctrl Pts',(126.279413224307,6.74047198977275,63.5132546095883));
#185368=CARTESIAN_POINT('Ctrl Pts',(126.35277927908,6.61139884496046,63.5256909653223));
#185369=CARTESIAN_POINT('Ctrl Pts',(126.57029275137,6.21376842058214,63.5623112512778));
#185370=CARTESIAN_POINT('Ctrl Pts',(126.707677361444,5.94136527396956,63.5850848026988));
#185371=CARTESIAN_POINT('Ctrl Pts',(127.097179258571,5.10017515670289,63.6486932939701));
#185372=CARTESIAN_POINT('Ctrl Pts',(127.320241730258,4.51740472396742,63.6837194836451));
#185373=CARTESIAN_POINT('Ctrl Pts',(127.55469395533,3.74917435090967,63.7190974658576));
#185374=CARTESIAN_POINT('Ctrl Pts',(127.603887272878,3.57555523236867,63.7264056878772));
#185375=CARTESIAN_POINT('Ctrl Pts',(127.6837414034,3.27024422545214,63.7380736540996));
#185376=CARTESIAN_POINT('Ctrl Pts',(127.715953475882,3.13897282342005,63.742712872544));
#185377=CARTESIAN_POINT('Ctrl Pts',(127.791469551845,2.8095227410864,63.7534204685536));
#185378=CARTESIAN_POINT('Ctrl Pts',(127.832183153652,2.61100261092291,63.7590386510351));
#185379=CARTESIAN_POINT('Ctrl Pts',(127.93608630686,2.03862105746458,63.7727656608263));
#185380=CARTESIAN_POINT('Ctrl Pts',(127.987954637871,1.66259288423845,63.778773729528));
#185381=CARTESIAN_POINT('Ctrl Pts',(128.042889127933,1.08870161315972,63.7830043603928));
#185382=CARTESIAN_POINT('Ctrl Pts',(128.057430979649,0.891963419645197,
63.7835724840572));
#185383=CARTESIAN_POINT('Ctrl Pts',(128.076766242742,0.52236522668691,63.7829731526187));
#185384=CARTESIAN_POINT('Ctrl Pts',(128.082540766683,0.349555808739192,
63.7820159683859));
#185385=CARTESIAN_POINT('Ctrl Pts',(128.089034112713,-0.0953612492450678,
63.7778356498596));
#185386=CARTESIAN_POINT('Ctrl Pts',(128.08494830738,-0.36754022781548,63.7736269984285));
#185387=CARTESIAN_POINT('Ctrl Pts',(128.054662620318,-1.04635916252852,
63.7590930615933));
#185388=CARTESIAN_POINT('Ctrl Pts',(128.018466256329,-1.45254861838066,
63.7467650667485));
#185389=CARTESIAN_POINT('Ctrl Pts',(127.905720865122,-2.29229219647711,
63.7138979305539));
#185390=CARTESIAN_POINT('Ctrl Pts',(127.826149809687,-2.72545598915823,
63.6927765111203));
#185391=CARTESIAN_POINT('Ctrl Pts',(127.682735756832,-3.33597312199448,
63.6571198256226));
#185392=CARTESIAN_POINT('Ctrl Pts',(127.636052598337,-3.51753650449608,
63.6457562053938));
#185393=CARTESIAN_POINT('Ctrl Pts',(127.537139474974,-3.87104890404324,
63.6221392418014));
#185394=CARTESIAN_POINT('Ctrl Pts',(127.48522892673,-4.04303671301638,63.609947395542));
#185395=CARTESIAN_POINT('Ctrl Pts',(127.35983215172,-4.42966896154413,63.5809245515613));
#185396=CARTESIAN_POINT('Ctrl Pts',(127.284403776974,-4.64333557414903,
63.5637370540283));
#185397=CARTESIAN_POINT('Ctrl Pts',(127.08810201439,-5.15742758929339,63.5194228349989));
#185398=CARTESIAN_POINT('Ctrl Pts',(126.961651796966,-5.45561033970457,
63.4911754126882));
#185399=CARTESIAN_POINT('Ctrl Pts',(126.721950285634,-5.96885125057334,
63.437899210874));
#185400=CARTESIAN_POINT('Ctrl Pts',(126.613244129366,-6.18612506944329,
63.4138376499016));
#185401=CARTESIAN_POINT('Ctrl Pts',(126.228806746939,-6.90557805916941,
63.3291014925126));
#185402=CARTESIAN_POINT('Ctrl Pts',(125.926999873965,-7.39329765439399,
63.2631398864311));
#185403=CARTESIAN_POINT('Ctrl Pts',(125.242339179045,-8.35710750634763,
63.1149355030169));
#185404=CARTESIAN_POINT('Ctrl Pts',(124.855268790752,-8.83025003519495,
63.0318724215669));
#185405=CARTESIAN_POINT('Ctrl Pts',(124.268174871789,-9.45390692713134,
62.9071577054099));
#185406=CARTESIAN_POINT('Ctrl Pts',(124.093503188441,-9.62922064665647,
62.8701909474783));
#185407=CARTESIAN_POINT('Ctrl Pts',(123.761317826565,-9.94398538855665,
62.8001646453368));
#185408=CARTESIAN_POINT('Ctrl Pts',(123.605431083467,-10.0845840004652,
62.76741912026));
#185409=CARTESIAN_POINT('Ctrl Pts',(123.117910263833,-10.5032208846779,
62.6651988756454));
#185410=CARTESIAN_POINT('Ctrl Pts',(122.775801999737,-10.7683585796145,
62.5936132799717));
#185411=CARTESIAN_POINT('Ctrl Pts',(121.942386100403,-11.3508099273098,
62.4193000587018));
#185412=CARTESIAN_POINT('Ctrl Pts',(121.441114511936,-11.6533540788972,
62.3145802764286));
#185413=CARTESIAN_POINT('Ctrl Pts',(119.91297790932,-12.4422557176493,61.995879137436));
#185414=CARTESIAN_POINT('Ctrl Pts',(118.837482177309,-12.8315201955363,
61.772265222769));
#185415=CARTESIAN_POINT('Ctrl Pts',(117.35376376487,-13.1521509064902,61.4653674022185));
#185416=CARTESIAN_POINT('Ctrl Pts',(116.97387542283,-13.2160641974833,61.3868775472256));
#185417=CARTESIAN_POINT('Ctrl Pts',(114.895288982598,-13.4699600416556,
60.9573247662507));
#185418=CARTESIAN_POINT('Ctrl Pts',(113.157173146467,-13.3361685680301,
60.5982366964183));
#185419=CARTESIAN_POINT('Ctrl Pts',(111.165941872547,-12.7716038830549,
60.1850714064443));
#185420=CARTESIAN_POINT('Ctrl Pts',(110.825714924704,-12.6593948278489,
60.1143910742432));
#185421=CARTESIAN_POINT('Ctrl Pts',(110.081186138087,-12.3780218950513,
59.9597634374073));
#185422=CARTESIAN_POINT('Ctrl Pts',(109.680637189306,-12.2025850285081,
59.8765714240575));
#185423=CARTESIAN_POINT('Ctrl Pts',(108.46463464669,-11.5951576663429,59.6237514982524));
#185424=CARTESIAN_POINT('Ctrl Pts',(107.681880334891,-11.0944295597603,
59.460619994412));
#185425=CARTESIAN_POINT('Ctrl Pts',(106.623565344028,-10.2492312356769,
59.2383053753914));
#185426=CARTESIAN_POINT('Ctrl Pts',(106.301217433876,-9.96510114004388,
59.1703134723297));
#185427=CARTESIAN_POINT('Ctrl Pts',(105.739246669316,-9.41843069592504,
59.0511155093957));
#185428=CARTESIAN_POINT('Ctrl Pts',(105.495040866814,-9.16082429711028,
58.9990100524303));
#185429=CARTESIAN_POINT('Ctrl Pts',(105.103487043763,-8.71224724580841,
58.9152489820056));
#185430=CARTESIAN_POINT('Ctrl Pts',(104.950598413732,-8.52690380625557,
58.8825085712831));
#185431=CARTESIAN_POINT('Ctrl Pts',(104.604870287619,-8.08352746608162,
58.8083691573518));
#185432=CARTESIAN_POINT('Ctrl Pts',(104.41606482338,-7.82212053329414,58.7677928385312));
#185433=CARTESIAN_POINT('Ctrl Pts',(103.981472604273,-7.17204939697519,
58.6740466758329));
#185434=CARTESIAN_POINT('Ctrl Pts',(103.745546727541,-6.77649136647243,
58.6228481668308));
#185435=CARTESIAN_POINT('Ctrl Pts',(103.303452588012,-5.94142311213269,
58.52590543329));
#185436=CARTESIAN_POINT('Ctrl Pts',(103.099458028566,-5.50062150387374,
58.4805791170773));
#185437=CARTESIAN_POINT('Ctrl Pts',(102.825741709879,-4.81516588624815,
58.4184742886835));
#185438=CARTESIAN_POINT('Ctrl Pts',(102.738518068587,-4.57774036248472,
58.3984238208679));
#185439=CARTESIAN_POINT('Ctrl Pts',(102.56938333461,-4.07420572585244,58.3589035424022));
#185440=CARTESIAN_POINT('Ctrl Pts',(102.488880017043,-3.80760221179232,
58.3396796064654));
#185441=CARTESIAN_POINT('Ctrl Pts',(102.306178391686,-3.12675766107656,
58.2949371640255));
#185442=CARTESIAN_POINT('Ctrl Pts',(102.215099288727,-2.70906488331788,
58.2715529161298));
#185443=CARTESIAN_POINT('Ctrl Pts',(102.115375507199,-2.11463595783645,
58.2446403449956));
#185444=CARTESIAN_POINT('Ctrl Pts',(102.089899349981,-1.94213566451076,
58.2375558423345));
#185445=CARTESIAN_POINT('Ctrl Pts',(102.031527226192,-1.48574817323299,
58.2206749328734));
#185446=CARTESIAN_POINT('Ctrl Pts',(102.004287148895,-1.20110288736358,
58.2120371922918));
#185447=CARTESIAN_POINT('Ctrl Pts',(101.957204748187,-0.465989413848542,
58.1943975671659));
#185448=CARTESIAN_POINT('Ctrl Pts',(101.950697245743,-0.0145871090450379,
58.1880603225808));
#185449=CARTESIAN_POINT('Ctrl Pts',(101.979497898391,0.81521207874154,58.1842042345649));
#185450=CARTESIAN_POINT('Ctrl Pts',(102.008341185183,1.19388032184666,58.1854458145418));
#185451=CARTESIAN_POINT('Ctrl Pts',(102.074590931882,1.75552159806408,58.1915920056869));
#185452=CARTESIAN_POINT('Ctrl Pts',(102.100154072651,1.93994144346426,58.1943089792539));
#185453=CARTESIAN_POINT('Ctrl Pts',(102.157017519422,2.29653190820955,58.200900148097));
#185454=CARTESIAN_POINT('Ctrl Pts',(102.187882370866,2.4687774732748,58.2046951060956));
#185455=CARTESIAN_POINT('Ctrl Pts',(102.290119650855,2.98212696715096,58.2178187143168));
#185456=CARTESIAN_POINT('Ctrl Pts',(102.371301149614,3.32123500972588,58.2289098849127));
#185457=CARTESIAN_POINT('Ctrl Pts',(102.530608203569,3.88849320977765,58.2520241834284));
#185458=CARTESIAN_POINT('Ctrl Pts',(102.601948116002,4.11859234001682,58.2627041296762));
#185459=CARTESIAN_POINT('Ctrl Pts',(102.723885069958,4.47716221201858,58.2815531894713));
#185460=CARTESIAN_POINT('Ctrl Pts',(102.770284317948,4.60692406344235,58.288842812769));
#185461=CARTESIAN_POINT('Ctrl Pts',(102.8705386318,4.8741570529312,58.3048171564709));
#185462=CARTESIAN_POINT('Ctrl Pts',(102.924685302567,5.01150270663102,58.3135625388303));
#185463=CARTESIAN_POINT('Ctrl Pts',(103.092914039189,5.41840244215338,58.3410419072278));
#185464=CARTESIAN_POINT('Ctrl Pts',(103.213569054479,5.68513865651778,58.3611408147348));
#185465=CARTESIAN_POINT('Ctrl Pts',(103.590998532217,6.45227214745571,58.4248524127774));
#185466=CARTESIAN_POINT('Ctrl Pts',(103.870623444065,6.9410893339289,58.4730448124913));
#185467=CARTESIAN_POINT('Ctrl Pts',(104.299957315108,7.59415472485762,58.5475262349333));
#185468=CARTESIAN_POINT('Ctrl Pts',(104.425277670601,7.77503149492879,58.5693158241309));
#185469=CARTESIAN_POINT('Ctrl Pts',(104.635865489267,8.06367459540217,58.6059582701477));
#185470=CARTESIAN_POINT('Ctrl Pts',(104.718521290145,8.17341224649394,58.6203468117229));
#185471=CARTESIAN_POINT('Ctrl Pts',(104.89667119073,8.40255547130351,58.6513570157837));
#185472=CARTESIAN_POINT('Ctrl Pts',(104.99255859074,8.52164582674666,58.6680434143177));
#185473=CARTESIAN_POINT('Ctrl Pts',(105.467611677194,9.09143480230328,58.7507175916747));
#185474=CARTESIAN_POINT('Ctrl Pts',(105.874241507033,9.51855185457868,58.8215420309538));
#185475=CARTESIAN_POINT('Ctrl Pts',(106.373042354692,9.97642146938205,58.9096250944761));
#185476=CARTESIAN_POINT('Ctrl Pts',(106.439498159346,10.0361782021163,58.9213831907577));
#185477=CARTESIAN_POINT('Ctrl Pts',(106.536842319661,10.121909575254,58.9386440145915));
#185478=CARTESIAN_POINT('Ctrl Pts',(106.56725522764,10.1484435821163,58.9440419953321));
#185479=CARTESIAN_POINT('Ctrl Pts',(106.597794810055,10.1748376800446,58.9494679941055));
#185480=CARTESIAN_POINT('',(108.748391092788,-12.3027435596069,59.3669505783331));
#185481=CARTESIAN_POINT('Ctrl Pts',(108.748724298952,-12.3019154543241,
59.3675684195169));
#185482=CARTESIAN_POINT('Ctrl Pts',(107.602691759852,-11.657374533869,59.14480114862));
#185483=CARTESIAN_POINT('Ctrl Pts',(106.54648133059,-10.8459005742635,58.9394936143287));
#185484=CARTESIAN_POINT('Ctrl Pts',(104.710420613127,-8.94979049702961,
58.5825977834728));
#185485=CARTESIAN_POINT('Ctrl Pts',(103.934314629432,-7.86845478333372,
58.4317373096063));
#185486=CARTESIAN_POINT('Ctrl Pts',(102.494214638211,-5.1163968120187,58.1518088312101));
#185487=CARTESIAN_POINT('Ctrl Pts',(101.978499526416,-3.38953146267605,
58.051563468104));
#185488=CARTESIAN_POINT('Ctrl Pts',(101.694535872802,-0.397371037757389,
57.9963662498825));
#185489=CARTESIAN_POINT('Ctrl Pts',(101.662183633473,1.4774576465605,57.9900775802182));
#185490=CARTESIAN_POINT('Ctrl Pts',(102.704999893562,4.95633168042048,58.1927815387717));
#185491=CARTESIAN_POINT('Ctrl Pts',(103.278228008759,6.181755194884,58.304206353048));
#185492=CARTESIAN_POINT('Ctrl Pts',(104.735425788297,8.38385488749155,58.5874583214079));
#185493=CARTESIAN_POINT('Ctrl Pts',(105.604862919118,9.35048684197738,58.7564606230372));
#185494=CARTESIAN_POINT('Ctrl Pts',(106.597794810055,10.1748376800446,58.9494679941055));
#185495=CARTESIAN_POINT('',(108.827755276219,-12.3460198217725,59.3829305619696));
#185496=CARTESIAN_POINT('Ctrl Pts',(108.827755276219,-12.3460198217725,
59.3829305619696));
#185497=CARTESIAN_POINT('Ctrl Pts',(108.801111662428,-12.3319613983389,
59.3775671848589));
#185498=CARTESIAN_POINT('Ctrl Pts',(108.774513616443,-12.3178132353077,
59.3722126652767));
#185499=CARTESIAN_POINT('Ctrl Pts',(108.747961719012,-12.3035756411923,
59.3668671161093));
#185500=CARTESIAN_POINT('Ctrl Pts',(108.827755276219,-12.3460198217725,
59.3829305619696));
#185501=CARTESIAN_POINT('Ctrl Pts',(109.261234383337,-12.5750413194122,
59.4732046875812));
#185502=CARTESIAN_POINT('Ctrl Pts',(109.706466269681,-12.7800813106308,
59.5658999124667));
#185503=CARTESIAN_POINT('Ctrl Pts',(110.41126587268,-13.0591110129488,59.7123004931389));
#185504=CARTESIAN_POINT('Ctrl Pts',(110.663792636116,-13.1504229782856,
59.7646880006138));
#185505=CARTESIAN_POINT('Ctrl Pts',(111.388554457391,-13.3881353111418,
59.9146985118048));
#185506=CARTESIAN_POINT('Ctrl Pts',(111.866231409931,-13.5160120037384,
60.0131245420342));
#185507=CARTESIAN_POINT('Ctrl Pts',(112.843955012572,-13.7205230380231,
60.2144696807969));
#185508=CARTESIAN_POINT('Ctrl Pts',(113.343506898725,-13.7957831208322,
60.3172903773583));
#185509=CARTESIAN_POINT('Ctrl Pts',(114.257307723694,-13.8808602579056,
60.5056637641811));
#185510=CARTESIAN_POINT('Ctrl Pts',(114.669849720597,-13.9,60.5908085805516));
#185511=CARTESIAN_POINT('Ctrl Pts',(115.082307292334,-13.9,60.6760422812756));
#185512=CARTESIAN_POINT('',(114.641143207841,-13.3595548147716,62.9456702505604));
#185513=CARTESIAN_POINT('Ctrl Pts',(124.127322289755,-8.93395457648499,
66.2032737914971));
#185514=CARTESIAN_POINT('Ctrl Pts',(122.805272603048,-10.43663118481,65.9217654640849));
#185515=CARTESIAN_POINT('Ctrl Pts',(119.481298892218,-12.81680175343,65.226593965893));
#185516=CARTESIAN_POINT('Ctrl Pts',(113.463801884159,-13.79335473887,63.9833253455664));
#185517=CARTESIAN_POINT('Ctrl Pts',(107.636855155043,-11.97726991923,62.7770961322029));
#185518=CARTESIAN_POINT('Ctrl Pts',(103.182583853411,-7.73653374972899,
61.8376893242906));
#185519=CARTESIAN_POINT('Ctrl Pts',(101.00559514138,-1.92956717280499,61.3409436191289));
#185520=CARTESIAN_POINT('Ctrl Pts',(101.549375432396,4.26802286533402,61.3730644730488));
#185521=CARTESIAN_POINT('Ctrl Pts',(104.706635557586,9.60158040629401,61.9131968801661));
#185522=CARTESIAN_POINT('Ctrl Pts',(109.840997033316,12.99135922774,62.8376407768088));
#185523=CARTESIAN_POINT('Ctrl Pts',(115.915831602521,13.75112083595,63.9448950363666));
#185524=CARTESIAN_POINT('Ctrl Pts',(121.704118510716,11.72705615912,64.9964497950401));
#185525=CARTESIAN_POINT('Ctrl Pts',(126.036844041747,7.32892445847002,65.7650706713404));
#185526=CARTESIAN_POINT('Ctrl Pts',(128.039674084356,1.44709807664901,66.0808034823172));
#185527=CARTESIAN_POINT('Ctrl Pts',(127.309907448893,-4.72768050995399,
65.8653706556117));
#185528=CARTESIAN_POINT('Ctrl Pts',(123.998186958828,-9.94538363148499,
65.1480543359445));
#185529=CARTESIAN_POINT('Ctrl Pts',(118.777305515395,-13.14965866642,64.0596328680601));
#185530=CARTESIAN_POINT('Ctrl Pts',(114.731505652229,-13.51125452112,63.2241518790638));
#185531=CARTESIAN_POINT('Ctrl Pts',(112.771522436493,-13.22996072786,62.818641216267));
#185532=CARTESIAN_POINT('Ctrl Pts',(124.14684851148,-8.93395457648499,66.102820590392));
#185533=CARTESIAN_POINT('Ctrl Pts',(122.824798824771,-10.43663118481,65.8213122629897));
#185534=CARTESIAN_POINT('Ctrl Pts',(119.500825113942,-12.81680175343,65.1261407647978));
#185535=CARTESIAN_POINT('Ctrl Pts',(113.483328105883,-13.79335473887,63.8828721444713));
#185536=CARTESIAN_POINT('Ctrl Pts',(107.656381376766,-11.97726991923,62.6766429311077));
#185537=CARTESIAN_POINT('Ctrl Pts',(103.202110075135,-7.73653374972899,
61.7372361231954));
#185538=CARTESIAN_POINT('Ctrl Pts',(101.025121363104,-1.92956717280499,
61.2404904180337));
#185539=CARTESIAN_POINT('Ctrl Pts',(101.568901654119,4.26802286533402,61.2726112719536));
#185540=CARTESIAN_POINT('Ctrl Pts',(104.72616177931,9.60158040629401,61.8127436790709));
#185541=CARTESIAN_POINT('Ctrl Pts',(109.860523255039,12.99135922774,62.7371875757135));
#185542=CARTESIAN_POINT('Ctrl Pts',(115.935357824245,13.75112083595,63.8444418352714));
#185543=CARTESIAN_POINT('Ctrl Pts',(121.72364473244,11.72705615912,64.8959965939449));
#185544=CARTESIAN_POINT('Ctrl Pts',(126.056370263471,7.32892445847002,65.6646174702451));
#185545=CARTESIAN_POINT('Ctrl Pts',(128.05920030608,1.44709807664901,65.980350281222));
#185546=CARTESIAN_POINT('Ctrl Pts',(127.329433670617,-4.72768050995399,
65.7649174545165));
#185547=CARTESIAN_POINT('Ctrl Pts',(124.017713180552,-9.94538363148499,
65.0476011348493));
#185548=CARTESIAN_POINT('Ctrl Pts',(118.796831737119,-13.14965866642,63.9591796669649));
#185549=CARTESIAN_POINT('Ctrl Pts',(114.751031873954,-13.51125452112,63.1236986779588));
#185550=CARTESIAN_POINT('Ctrl Pts',(112.791048658217,-13.22996072786,62.7181880151718));
#185551=CARTESIAN_POINT('Ctrl Pts',(124.166374733204,-8.93395457648499,
66.0023673892968));
#185552=CARTESIAN_POINT('Ctrl Pts',(122.844325046497,-10.43663118481,65.7208590618847));
#185553=CARTESIAN_POINT('Ctrl Pts',(119.520351335665,-12.81680175343,65.0256875637026));
#185554=CARTESIAN_POINT('Ctrl Pts',(113.502854327606,-13.79335473887,63.782418943376));
#185555=CARTESIAN_POINT('Ctrl Pts',(107.67590759849,-11.97726991923,62.5761897300125));
#185556=CARTESIAN_POINT('Ctrl Pts',(103.221636296858,-7.73653374972899,
61.6367829221002));
#185557=CARTESIAN_POINT('Ctrl Pts',(101.044647584827,-1.92956717280499,
61.1400372169385));
#185558=CARTESIAN_POINT('Ctrl Pts',(101.588427875843,4.26802286533402,61.1721580708584));
#185559=CARTESIAN_POINT('Ctrl Pts',(104.745688001033,9.60158040629401,61.7122904779757));
#185560=CARTESIAN_POINT('Ctrl Pts',(109.880049476763,12.99135922774,62.6367343746183));
#185561=CARTESIAN_POINT('Ctrl Pts',(115.954884045968,13.75112083595,63.7439886341762));
#185562=CARTESIAN_POINT('Ctrl Pts',(121.743170954163,11.72705615912,64.7955433928497));
#185563=CARTESIAN_POINT('Ctrl Pts',(126.075896485195,7.32892445847002,65.5641642691499));
#185564=CARTESIAN_POINT('Ctrl Pts',(128.078726527803,1.44709807664901,65.8798970801268));
#185565=CARTESIAN_POINT('Ctrl Pts',(127.34895989234,-4.72768050995399,65.6644642534212));
#185566=CARTESIAN_POINT('Ctrl Pts',(124.037239402277,-9.94538363148499,
64.9471479337443));
#185567=CARTESIAN_POINT('Ctrl Pts',(118.816357958844,-13.14965866642,63.8587264658599));
#185568=CARTESIAN_POINT('Ctrl Pts',(114.770558095677,-13.51125452112,63.0232454768636));
#185569=CARTESIAN_POINT('Ctrl Pts',(112.810574879942,-13.22996072786,62.6177348140668));
#185570=CARTESIAN_POINT('Ctrl Pts',(124.185900954927,-8.93395457648499,
65.9019141882016));
#185571=CARTESIAN_POINT('Ctrl Pts',(122.86385126822,-10.43663118481,65.6204058607894));
#185572=CARTESIAN_POINT('Ctrl Pts',(119.539877557389,-12.81680175343,64.9252343626074));
#185573=CARTESIAN_POINT('Ctrl Pts',(113.52238054933,-13.79335473887,63.6819657422808));
#185574=CARTESIAN_POINT('Ctrl Pts',(107.695433820213,-11.97726991923,62.4757365289173));
#185575=CARTESIAN_POINT('Ctrl Pts',(103.241162518582,-7.73653374972899,
61.536329721005));
#185576=CARTESIAN_POINT('Ctrl Pts',(101.064173806551,-1.92956717280499,
61.0395840158433));
#185577=CARTESIAN_POINT('Ctrl Pts',(101.607954097566,4.26802286533402,61.0717048697632));
#185578=CARTESIAN_POINT('Ctrl Pts',(104.765214222759,9.60158040629401,61.6118372768707));
#185579=CARTESIAN_POINT('Ctrl Pts',(109.899575698488,12.99135922774,62.5362811735133));
#185580=CARTESIAN_POINT('Ctrl Pts',(115.974410267694,13.75112083595,63.6435354330712));
#185581=CARTESIAN_POINT('Ctrl Pts',(121.762697175889,11.72705615912,64.6950901917447));
#185582=CARTESIAN_POINT('Ctrl Pts',(126.09542270692,7.32892445847002,65.4637110680449));
#185583=CARTESIAN_POINT('Ctrl Pts',(128.098252749529,1.44709807664901,65.7794438790217));
#185584=CARTESIAN_POINT('Ctrl Pts',(127.368486114066,-4.72768050995399,
65.5640110523162));
#185585=CARTESIAN_POINT('Ctrl Pts',(124.056765624,-9.94538363148499,64.8466947326491));
#185586=CARTESIAN_POINT('Ctrl Pts',(118.835884180567,-13.14965866642,63.7582732647647));
#185587=CARTESIAN_POINT('Ctrl Pts',(114.790084317401,-13.51125452112,62.9227922757684));
#185588=CARTESIAN_POINT('Ctrl Pts',(112.830101101666,-13.22996072786,62.5172816129716));
#185589=CARTESIAN_POINT('',(114.602947212677,-13.3588269031369,63.1421432529824));
#185590=CARTESIAN_POINT('',(114.602824644425,-13.358908889387,63.1427506256491));
#185591=CARTESIAN_POINT('',(122.863635671064,-10.2286061806799,65.6766524048838));
#185592=CARTESIAN_POINT('Ctrl Pts',(122.863760060438,-10.2287368491257,
65.6765769614792));
#185593=CARTESIAN_POINT('Ctrl Pts',(122.240146213124,-10.7632276682405,
65.5458260535504));
#185594=CARTESIAN_POINT('Ctrl Pts',(121.567667527631,-11.2386000580356,
65.4056673900111));
#185595=CARTESIAN_POINT('Ctrl Pts',(120.422256010174,-11.8971524039626,
65.1659826384782));
#185596=CARTESIAN_POINT('Ctrl Pts',(119.972280261939,-12.1223443916377,
65.0716961849902));
#185597=CARTESIAN_POINT('Ctrl Pts',(119.154752940445,-12.4727659840031,
64.90127152028));
#185598=CARTESIAN_POINT('Ctrl Pts',(118.792474245388,-12.6087267809308,
64.8260808448027));
#185599=CARTESIAN_POINT('Ctrl Pts',(117.712268209454,-12.9595326876314,
64.602483820945));
#185600=CARTESIAN_POINT('Ctrl Pts',(116.979574018507,-13.1284662514209,
64.4515484121121));
#185601=CARTESIAN_POINT('Ctrl Pts',(115.382030528533,-13.3538641526337,
64.1216421923012));
#185602=CARTESIAN_POINT('Ctrl Pts',(114.514268176837,-13.3888157087188,
63.94123680514));
#185603=CARTESIAN_POINT('Ctrl Pts',(112.882163285328,-13.2871455157589,
63.6027834419524));
#185604=CARTESIAN_POINT('Ctrl Pts',(112.117935990712,-13.168500674772,63.4451730291947));
#185605=CARTESIAN_POINT('Ctrl Pts',(110.576772771736,-12.7865358856342,
63.1269643432183));
#185606=CARTESIAN_POINT('Ctrl Pts',(109.800877120059,-12.5144474866061,
62.9664816746769));
#185607=CARTESIAN_POINT('Ctrl Pts',(108.744124181976,-12.0270341854416,
62.7459016018925));
#185608=CARTESIAN_POINT('Ctrl Pts',(108.437034204304,-11.8702494054068,
62.6816086394531));
#185609=CARTESIAN_POINT('Ctrl Pts',(107.367383543376,-11.2685768566542,
62.4577116956883));
#185610=CARTESIAN_POINT('Ctrl Pts',(106.644130952332,-10.7566383761923,
62.3068071526653));
#185611=CARTESIAN_POINT('Ctrl Pts',(105.39940592417,-9.6747655290772,62.0455752822621));
#185612=CARTESIAN_POINT('Ctrl Pts',(104.862872271295,-9.12003284756065,
61.9322384738739));
#185613=CARTESIAN_POINT('Ctrl Pts',(104.013688156968,-8.07338890431674,
61.7498632067556));
#185614=CARTESIAN_POINT('Ctrl Pts',(103.678542159989,-7.60034210331702,
61.6770036424679));
#185615=CARTESIAN_POINT('Ctrl Pts',(102.965863098996,-6.43776000726343,
61.5216204731177));
#185616=CARTESIAN_POINT('Ctrl Pts',(102.615546714304,-5.73384448039941,
61.4445272154993));
#185617=CARTESIAN_POINT('Ctrl Pts',(102.124533339922,-4.48787726460851,
61.3334637104734));
#185618=CARTESIAN_POINT('Ctrl Pts',(101.952461547406,-3.95857885737421,
61.2934636788593));
#185619=CARTESIAN_POINT('Ctrl Pts',(101.596124566779,-2.57950115143769,
61.2064914408388));
#185620=CARTESIAN_POINT('Ctrl Pts',(101.460405992341,-1.72069010498245,
61.1685699439471));
#185621=CARTESIAN_POINT('Ctrl Pts',(101.364478811265,-0.109464886862312,
61.1305919156548));
#185622=CARTESIAN_POINT('Ctrl Pts',(101.38098315129,0.634328801104304,61.1253212132384));
#185623=CARTESIAN_POINT('Ctrl Pts',(101.63922130165,3.13169786388764,61.1460319840433));
#185624=CARTESIAN_POINT('Ctrl Pts',(102.159133504572,4.82979500457738,61.2240371490054));
#185625=CARTESIAN_POINT('Ctrl Pts',(103.322134470119,6.99422477083511,61.4213202159224));
#185626=CARTESIAN_POINT('Ctrl Pts',(103.694429784937,7.57614415877838,61.485614547929));
#185627=CARTESIAN_POINT('Ctrl Pts',(104.504460129801,8.6506071400515,61.6264142201267));
#185628=CARTESIAN_POINT('Ctrl Pts',(104.938756384371,9.14611593047081,61.7021075136189));
#185629=CARTESIAN_POINT('Ctrl Pts',(106.013631261799,10.1996857606197,61.8923389269699));
#185630=CARTESIAN_POINT('Ctrl Pts',(106.673833749292,10.7324870133182,62.0107815663951));
#185631=CARTESIAN_POINT('Ctrl Pts',(107.929893822727,11.5626987947379,62.2370448228732));
#185632=CARTESIAN_POINT('Ctrl Pts',(108.509340409586,11.8861695854614,62.3417170605054));
#185633=CARTESIAN_POINT('Ctrl Pts',(109.416432484761,12.3056267423368,62.5053407714911));
#185634=CARTESIAN_POINT('Ctrl Pts',(109.728875559953,12.4355663395387,62.5616480894726));
#185635=CARTESIAN_POINT('Ctrl Pts',(110.70474560647,12.7968216736441,62.7380392767041));
#185636=CARTESIAN_POINT('Ctrl Pts',(111.382980529343,12.9861920178074,62.8613660333791));
#185637=CARTESIAN_POINT('Ctrl Pts',(112.897689287169,13.2803590562696,63.1372980237683));
#185638=CARTESIAN_POINT('Ctrl Pts',(113.73892015981,13.3607725717846,63.2908580231773));
#185639=CARTESIAN_POINT('Ctrl Pts',(115.336533881722,13.3577945987543,63.5814699441069));
#185640=CARTESIAN_POINT('Ctrl Pts',(116.089542267633,13.2900526257154,63.7178997427436));
#185641=CARTESIAN_POINT('Ctrl Pts',(117.93552764734,12.9565936607203,64.0535767474533));
#185642=CARTESIAN_POINT('Ctrl Pts',(119.009875870491,12.6151247506599,64.249334419709));
#185643=CARTESIAN_POINT('Ctrl Pts',(120.81305748656,11.7764189739414,64.5754658880205));
#185644=CARTESIAN_POINT('Ctrl Pts',(121.563089340139,11.3323021474241,64.7099299890663));
#185645=CARTESIAN_POINT('Ctrl Pts',(122.967289886509,10.2955208016799,64.961412049232));
#185646=CARTESIAN_POINT('Ctrl Pts',(123.616910763818,9.70826883189277,65.0773620752841));
#185647=CARTESIAN_POINT('Ctrl Pts',(125.379639856623,7.77153764746681,65.3885685191679));
#185648=CARTESIAN_POINT('Ctrl Pts',(126.286223890547,6.26842056998774,65.5428342292009));
#185649=CARTESIAN_POINT('Ctrl Pts',(127.183326724953,3.80455012558783,65.6859140196455));
#185650=CARTESIAN_POINT('Ctrl Pts',(127.403096581131,2.95846085195509,65.7182734354822));
#185651=CARTESIAN_POINT('Ctrl Pts',(127.637259599455,1.48709831544551,65.7454000803788));
#185652=CARTESIAN_POINT('Ctrl Pts',(127.691878872173,0.871913947897259,
65.7482971122607));
#185653=CARTESIAN_POINT('Ctrl Pts',(127.721704073428,-0.606022111551587,
65.7361311720197));
#185654=CARTESIAN_POINT('Ctrl Pts',(127.65734862261,-1.46774389326394,65.7133866238823));
#185655=CARTESIAN_POINT('Ctrl Pts',(127.218712115104,-4.04807163087889,
65.5966903809948));
#185656=CARTESIAN_POINT('Ctrl Pts',(126.594225323066,-5.69141216598206,
65.453722271121));
#185657=CARTESIAN_POINT('Ctrl Pts',(125.215914647381,-7.9075058974082,65.1542271548029));
#185658=CARTESIAN_POINT('Ctrl Pts',(124.6871438061,-8.59902863606933,65.040956822351));
#185659=CARTESIAN_POINT('Ctrl Pts',(123.809248021861,-9.53891006775381,
64.8544140425203));
#185660=CARTESIAN_POINT('Ctrl Pts',(123.508026186193,-9.83152877276116,
64.7906250911458));
#185661=CARTESIAN_POINT('Ctrl Pts',(122.019233236213,-11.144075489692,64.4766947679153));
#185662=CARTESIAN_POINT('Ctrl Pts',(120.663321346316,-11.9644757376867,
64.1941836778649));
#185663=CARTESIAN_POINT('Ctrl Pts',(118.479168800975,-12.7973455816125,
63.7406749481653));
#185664=CARTESIAN_POINT('Ctrl Pts',(117.727272371115,-13.006653057488,63.5848280374823));
#185665=CARTESIAN_POINT('Ctrl Pts',(116.19741872317,-13.287327677289,63.2681653310725));
#185666=CARTESIAN_POINT('Ctrl Pts',(115.419179639328,-13.3583908138007,
63.1072579646956));
#185667=CARTESIAN_POINT('Ctrl Pts',(114.640998168921,-13.3589088887046,
62.9463713323102));
#185668=CARTESIAN_POINT('',(107.485627742127,-11.3335893001804,62.6876626706917));
#185669=CARTESIAN_POINT('Ctrl Pts',(107.485561672623,-11.3337498925587,
62.6875423325866));
#185670=CARTESIAN_POINT('Ctrl Pts',(107.614804142611,-11.4160091339019,
62.7126646492232));
#185671=CARTESIAN_POINT('Ctrl Pts',(107.745249943893,-11.4958117911507,
62.7380208709361));
#185672=CARTESIAN_POINT('Ctrl Pts',(107.876899835385,-11.5731613609192,
62.763611145244));
#185673=CARTESIAN_POINT('Ctrl Pts',(108.061365151314,-11.6815421021619,
62.7994677493131));
#185674=CARTESIAN_POINT('Ctrl Pts',(108.24819346307,-11.78510864237,62.8357836755335));
#185675=CARTESIAN_POINT('Ctrl Pts',(108.437354282934,-11.8839349705715,
62.8725529976636));
#185676=CARTESIAN_POINT('Ctrl Pts',(108.6328913266,-11.9860925318822,62.9105617383324));
#185677=CARTESIAN_POINT('Ctrl Pts',(108.83092107342,-12.083185339433,62.9490550138287));
#185678=CARTESIAN_POINT('Ctrl Pts',(109.031436582887,-12.1752440931379,
62.9880314750483));
#185679=CARTESIAN_POINT('Ctrl Pts',(109.22430368395,-12.263791383079,63.0255212288587));
#185680=CARTESIAN_POINT('Ctrl Pts',(109.419468438602,-12.3476802430602,
63.0634576035127));
#185681=CARTESIAN_POINT('Ctrl Pts',(109.61695720614,-12.4268962909364,63.1018457227644));
#185682=CARTESIAN_POINT('Ctrl Pts',(109.771926507834,-12.4890570698777,
63.1319688538566));
#185683=CARTESIAN_POINT('Ctrl Pts',(109.928326637475,-12.5483393104261,
63.1623701111152));
#185684=CARTESIAN_POINT('Ctrl Pts',(110.086172426641,-12.6047129308209,
63.1930523775215));
#185685=CARTESIAN_POINT('Ctrl Pts',(110.130137395395,-12.6204147399875,
63.2015983443858));
#185686=CARTESIAN_POINT('Ctrl Pts',(110.174214539726,-12.635890784121,63.2101661160821));
#185687=CARTESIAN_POINT('Ctrl Pts',(110.218404225387,-12.6511401433646,
63.218755763706));
#185688=CARTESIAN_POINT('Ctrl Pts',(110.254123274814,-12.6634663821332,
63.2256988782237));
#185689=CARTESIAN_POINT('Ctrl Pts',(110.289911272532,-12.6756430115032,
63.2326553949984));
#185690=CARTESIAN_POINT('Ctrl Pts',(110.32579415179,-12.6876780033411,63.2396303549681));
#185691=CARTESIAN_POINT('Ctrl Pts',(110.473374762606,-12.7371760225445,
63.268317262876));
#185692=CARTESIAN_POINT('Ctrl Pts',(110.622478207417,-12.7842446063055,
63.2973001812039));
#185693=CARTESIAN_POINT('Ctrl Pts',(110.772679057295,-12.8286913645498,
63.3264964145326));
#185694=CARTESIAN_POINT('Ctrl Pts',(110.885625137274,-12.8621138592661,
63.3484510180337));
#185695=CARTESIAN_POINT('Ctrl Pts',(110.999191292185,-12.8940547885104,
63.3705261524935));
#185696=CARTESIAN_POINT('Ctrl Pts',(111.113190270013,-12.9244506654267,
63.3926854196253));
#185697=CARTESIAN_POINT('Ctrl Pts',(111.154854057468,-12.9355596014846,
63.400784079925));
#185698=CARTESIAN_POINT('Ctrl Pts',(111.196575611453,-12.9464623161029,
63.4088939689567));
#185699=CARTESIAN_POINT('Ctrl Pts',(111.238345640527,-12.9571562472333,
63.4170132806382));
#185700=CARTESIAN_POINT('Ctrl Pts',(111.266446655741,-12.9643506478132,
63.4224755919209));
#185701=CARTESIAN_POINT('Ctrl Pts',(111.294573102417,-12.9714513970515,
63.4279428466037));
#185702=CARTESIAN_POINT('Ctrl Pts',(111.322698384524,-12.9784519718767,
63.4334098749161));
#185703=CARTESIAN_POINT('Ctrl Pts',(111.536825921765,-13.0317497784859,
63.475032259506));
#185704=CARTESIAN_POINT('Ctrl Pts',(111.751164558969,-13.0793184605927,
63.5166956779769));
#185705=CARTESIAN_POINT('Ctrl Pts',(111.965659100288,-13.1212776219255,
63.5583894012888));
#185706=CARTESIAN_POINT('Ctrl Pts',(112.181521726303,-13.163504406323,63.6003490546542));
#185707=CARTESIAN_POINT('Ctrl Pts',(112.397542665596,-13.2000500000777,
63.642339481157));
#185708=CARTESIAN_POINT('Ctrl Pts',(112.613688198126,-13.2309885564611,
63.6843541262526));
#185709=CARTESIAN_POINT('Ctrl Pts',(112.830693324041,-13.2620501529929,
63.7265358602099));
#185710=CARTESIAN_POINT('Ctrl Pts',(113.047824453117,-13.2874601398532,
63.7687420868227));
#185711=CARTESIAN_POINT('Ctrl Pts',(113.265063829592,-13.3072438790148,
63.8109693547035));
#185712=CARTESIAN_POINT('Ctrl Pts',(113.350228480118,-13.3149997253955,
63.827523768411));
#185713=CARTESIAN_POINT('Ctrl Pts',(113.435409910131,-13.3218903354083,
63.8440814437367));
#185714=CARTESIAN_POINT('Ctrl Pts',(113.520607519528,-13.327915104691,63.8606422640318));
#185715=CARTESIAN_POINT('Ctrl Pts',(113.736958181362,-13.343214393379,63.9026967824238));
#185716=CARTESIAN_POINT('Ctrl Pts',(113.953412858971,-13.3529339642487,
63.9447715195353));
#185717=CARTESIAN_POINT('Ctrl Pts',(114.169957504393,-13.3571513294797,
63.9868637447053));
#185718=CARTESIAN_POINT('Ctrl Pts',(114.390268030086,-13.3614420379812,
64.0296879864995));
#185719=CARTESIAN_POINT('Ctrl Pts',(114.61067211477,-13.3600375840576,64.0725304144101));
#185720=CARTESIAN_POINT('Ctrl Pts',(114.831156415951,-13.3529648919269,
64.1153884349059));
#185721=CARTESIAN_POINT('Ctrl Pts',(114.927618297717,-13.3498705891197,
64.1341388188728));
#185722=CARTESIAN_POINT('Ctrl Pts',(115.024095512377,-13.345690645084,64.1528921832671));
#185723=CARTESIAN_POINT('Ctrl Pts',(115.120586694554,-13.3404240435081,
64.1716482626854));
#185724=CARTESIAN_POINT('Ctrl Pts',(115.172274692604,-13.337602852122,64.181695441863));
#185725=CARTESIAN_POINT('Ctrl Pts',(115.223966694672,-13.3344698120586,
64.1917433993467));
#185726=CARTESIAN_POINT('Ctrl Pts',(115.275662457027,-13.331024533966,64.2017920877599));
#185727=CARTESIAN_POINT('Ctrl Pts',(115.300632026009,-13.329360430274,64.2066457045184));
#185728=CARTESIAN_POINT('Ctrl Pts',(115.32560247186,-13.3276234794556,64.2114994917237));
#185729=CARTESIAN_POINT('Ctrl Pts',(115.350573764693,-13.3258136240892,
64.2163534435667));
#185730=CARTESIAN_POINT('Ctrl Pts',(115.369789998032,-13.3244208806993,
64.2200887195836));
#185731=CARTESIAN_POINT('Ctrl Pts',(115.389005122721,-13.3229850672834,
64.2238237800996));
#185732=CARTESIAN_POINT('Ctrl Pts',(115.408209864803,-13.3215069300936,
64.2275568224313));
#185733=CARTESIAN_POINT('Ctrl Pts',(115.620264914641,-13.3051856249646,
64.2687763542688));
#185734=CARTESIAN_POINT('Ctrl Pts',(115.831369254668,-13.2836859243608,
64.3098110859172));
#185735=CARTESIAN_POINT('Ctrl Pts',(116.041541009532,-13.2570867575058,
64.3506645404687));
#185736=CARTESIAN_POINT('Ctrl Pts',(116.252521508358,-13.2303852366707,
64.3916751997061));
#185737=CARTESIAN_POINT('Ctrl Pts',(116.462562646362,-13.1985448687571,
64.4325032647852));
#185738=CARTESIAN_POINT('Ctrl Pts',(116.671680915997,-13.1615929593013,
64.4731519415302));
#185739=CARTESIAN_POINT('Ctrl Pts',(116.880751147312,-13.1246495383798,
64.5137912805254));
#185740=CARTESIAN_POINT('Ctrl Pts',(117.088899348997,-13.0825968505039,
64.5542513942214));
#185741=CARTESIAN_POINT('Ctrl Pts',(117.296133937521,-13.0354108225876,
64.5945339186226));
#185742=CARTESIAN_POINT('Ctrl Pts',(117.501753324005,-12.9885925661379,
64.6345024779852));
#185743=CARTESIAN_POINT('Ctrl Pts',(117.70647367483,-12.9367205635069,64.6742962816465));
#185744=CARTESIAN_POINT('Ctrl Pts',(117.91028928519,-12.8797222224478,64.7139142206988));
#185745=CARTESIAN_POINT('Ctrl Pts',(118.031475045392,-12.8458318483036,
64.7374704637815));
#185746=CARTESIAN_POINT('Ctrl Pts',(118.152340658396,-12.8101282247323,
64.7609644762425));
#185747=CARTESIAN_POINT('Ctrl Pts',(118.272881693326,-12.7725879900098,
64.7843953968021));
#185748=CARTESIAN_POINT('Ctrl Pts',(118.303191203236,-12.7631486640822,
64.7902869981089));
#185749=CARTESIAN_POINT('Ctrl Pts',(118.33348017807,-12.7535931889409,64.7961746077812));
#185750=CARTESIAN_POINT('Ctrl Pts',(118.363748518854,-12.7439211333848,
64.8020582065804));
#185751=CARTESIAN_POINT('Ctrl Pts',(118.395124158262,-12.7338952476039,
64.8081570435028));
#185752=CARTESIAN_POINT('Ctrl Pts',(118.426470549753,-12.7237463489279,
64.8142501951775));
#185753=CARTESIAN_POINT('Ctrl Pts',(118.457784720862,-12.7134750686029,
64.8203370838131));
#185754=CARTESIAN_POINT('Ctrl Pts',(118.598547337112,-12.6673038866874,
64.8476987012161));
#185755=CARTESIAN_POINT('Ctrl Pts',(118.738697794193,-12.6186516797937,
64.874941326337));
#185756=CARTESIAN_POINT('Ctrl Pts',(118.878489383028,-12.5673757495857,
64.9021141941889));
#185757=CARTESIAN_POINT('Ctrl Pts',(118.956946557128,-12.5385974474216,
64.917364800049));
#185758=CARTESIAN_POINT('Ctrl Pts',(119.035290365746,-12.508991816977,64.9325933697815));
#185759=CARTESIAN_POINT('Ctrl Pts',(119.113562750043,-12.478526951352,64.9478080559632));
#185760=CARTESIAN_POINT('Ctrl Pts',(119.152698942191,-12.4632945185395,
64.955415399054));
#185761=CARTESIAN_POINT('Ctrl Pts',(119.191817243841,-12.4478472018354,
64.963019264567));
#185762=CARTESIAN_POINT('Ctrl Pts',(119.230922679739,-12.4321805612555,
64.9706206292184));
#185763=CARTESIAN_POINT('Ctrl Pts',(119.251451510466,-12.4239561851514,
64.9746110495946));
#185764=CARTESIAN_POINT('Ctrl Pts',(119.271976793086,-12.4156713618556,
64.9786007802852));
#185765=CARTESIAN_POINT('Ctrl Pts',(119.292499237416,-12.4073254157032,
64.9825899592652));
#185766=CARTESIAN_POINT('Ctrl Pts',(119.306734613276,-12.4015362573318,
64.9853570498342));
#185767=CARTESIAN_POINT('Ctrl Pts',(119.320968623249,-12.3957176892737,
64.9881238749001));
#185768=CARTESIAN_POINT('Ctrl Pts',(119.335201500787,-12.3898694795256,
64.9908904798418));
#185769=CARTESIAN_POINT('Ctrl Pts',(119.339536190148,-12.3880883799194,
64.9917330623046));
#185770=CARTESIAN_POINT('Ctrl Pts',(119.343870997956,-12.3863044387621,
64.9925756677911));
#185771=CARTESIAN_POINT('Ctrl Pts',(119.348205220554,-12.384517942185,64.9934181595239));
#185772=CARTESIAN_POINT('Ctrl Pts',(119.544789338538,-12.3034891426856,
65.031630431838));
#185773=CARTESIAN_POINT('Ctrl Pts',(119.738478069006,-12.2179058838895,
65.0692798950231));
#185774=CARTESIAN_POINT('Ctrl Pts',(119.929341495406,-12.1279359966252,
65.1063801719896));
#185775=CARTESIAN_POINT('Ctrl Pts',(120.122558815125,-12.0368565226763,
65.1439380017504));
#185776=CARTESIAN_POINT('Ctrl Pts',(120.31288104309,-11.9412813697266,65.1809330798728));
#185777=CARTESIAN_POINT('Ctrl Pts',(120.50036917076,-11.841332181931,65.2173772619545));
#185778=CARTESIAN_POINT('Ctrl Pts',(120.689606070474,-11.7404507305963,
65.2541613725831));
#185779=CARTESIAN_POINT('Ctrl Pts',(120.875956098769,-11.6351130659804,
65.2903843294525));
#185780=CARTESIAN_POINT('Ctrl Pts',(121.059464992335,-11.5253941026604,
65.3260550229191));
#185781=CARTESIAN_POINT('Ctrl Pts',(121.244274503297,-11.4148975073162,
65.3619785320589));
#185782=CARTESIAN_POINT('Ctrl Pts',(121.426202823407,-11.2999570785843,
65.3973419916353));
#185783=CARTESIAN_POINT('Ctrl Pts',(121.605274210285,-11.180601831691,65.4321501168758));
#185784=CARTESIAN_POINT('Ctrl Pts',(121.784368612727,-11.061231244389,65.4669627159108));
#185785=CARTESIAN_POINT('Ctrl Pts',(121.960605693043,-10.9374444567741,
65.5012199050162));
#185786=CARTESIAN_POINT('Ctrl Pts',(122.133982072171,-10.8092266649049,
65.5349210273653));
#185787=CARTESIAN_POINT('Ctrl Pts',(122.306425892347,-10.6816985324356,
65.5684408777125));
#185788=CARTESIAN_POINT('Ctrl Pts',(122.476040026031,-10.5497866711897,
65.6014106899798));
#185789=CARTESIAN_POINT('Ctrl Pts',(122.642788850821,-10.4134370267834,
65.6338235398391));
#185790=CARTESIAN_POINT('Ctrl Pts',(122.717000904232,-10.3527542177382,
65.6482489737095));
#185791=CARTESIAN_POINT('Ctrl Pts',(122.79064496167,-10.2911919068618,65.6625639997959));
#185792=CARTESIAN_POINT('Ctrl Pts',(122.863715547138,-10.2287429973371,
65.6767675536675));
#185793=CARTESIAN_POINT('',(107.470912577424,-11.3244123346074,62.6846948227235));
#185794=CARTESIAN_POINT('Ctrl Pts',(107.485627742145,-11.3335893001918,
62.6876626706956));
#185795=CARTESIAN_POINT('Ctrl Pts',(107.480720751801,-11.3305336178283,
62.6866730118255));
#185796=CARTESIAN_POINT('Ctrl Pts',(107.47581569552,-11.3274746283431,62.6856837289009));
#185797=CARTESIAN_POINT('Ctrl Pts',(107.470912577424,-11.3244123346074,
62.6846948227235));
#185798=CARTESIAN_POINT('Ctrl Pts',(107.470912577424,-11.3244123346074,
62.6846948227235));
#185799=CARTESIAN_POINT('Ctrl Pts',(106.274400038169,-10.558499336519,62.4344828152312));
#185800=CARTESIAN_POINT('Ctrl Pts',(105.20088303681,-9.59249959662681,62.2069325119651));
#185801=CARTESIAN_POINT('Ctrl Pts',(103.95853529321,-8.04858401858125,61.9426111970985));
#185802=CARTESIAN_POINT('Ctrl Pts',(103.639020846898,-7.5965992708658,61.8741089306158));
#185803=CARTESIAN_POINT('Ctrl Pts',(103.005157994299,-6.5665024217714,61.7357740944669));
#185804=CARTESIAN_POINT('Ctrl Pts',(102.70329262004,-5.98313165971164,61.6684239476137));
#185805=CARTESIAN_POINT('Ctrl Pts',(102.13470301904,-4.65742573741101,61.5397236763161));
#185806=CARTESIAN_POINT('Ctrl Pts',(101.886849244608,-3.90643332928001,
61.4825608413799));
#185807=CARTESIAN_POINT('Ctrl Pts',(101.606380445827,-2.71745730486092,
61.4139284022522));
#185808=CARTESIAN_POINT('Ctrl Pts',(101.527103418739,-2.29091550080621,
61.3934507827151));
#185809=CARTESIAN_POINT('Ctrl Pts',(101.369437898936,-1.12967719105034,
61.3483570289574));
#185810=CARTESIAN_POINT('Ctrl Pts',(101.330879433115,-0.389445079030975,
61.3310502435924));
#185811=CARTESIAN_POINT('Ctrl Pts',(101.381383843657,1.38471795578357,61.3191228559119));
#185812=CARTESIAN_POINT('Ctrl Pts',(101.528098343796,2.41736244468448,61.335856812152));
#185813=CARTESIAN_POINT('Ctrl Pts',(102.006775533799,4.24789039142094,61.4062133868773));
#185814=CARTESIAN_POINT('Ctrl Pts',(102.301591504679,5.04970934213961,61.4526635038114));
#185815=CARTESIAN_POINT('Ctrl Pts',(103.04391014446,6.60201841175238,61.5757503765786));
#185816=CARTESIAN_POINT('Ctrl Pts',(103.494532433191,7.35019918636513,61.6528035402932));
#185817=CARTESIAN_POINT('Ctrl Pts',(104.264830156951,8.38776329761607,61.7870168561449));
#185818=CARTESIAN_POINT('Ctrl Pts',(104.533803506792,8.71628340900593,61.8342336481498));
#185819=CARTESIAN_POINT('Ctrl Pts',(105.391433894827,9.66631592104284,61.9856619875418));
#185820=CARTESIAN_POINT('Ctrl Pts',(106.024476706078,10.2417873164856,62.0979956492993));
#185821=CARTESIAN_POINT('Ctrl Pts',(107.325363196647,11.2154249903307,62.3303691611087));
#185822=CARTESIAN_POINT('Ctrl Pts',(107.986739416363,11.6254157423024,62.4491993210171));
#185823=CARTESIAN_POINT('Ctrl Pts',(109.30206962946,12.288064782333,62.6875058937065));
#185824=CARTESIAN_POINT('Ctrl Pts',(109.94976826693,12.5517322071569,62.805433842119));
#185825=CARTESIAN_POINT('Ctrl Pts',(111.024128414873,12.8891408930617,63.0000736376732));
#185826=CARTESIAN_POINT('Ctrl Pts',(111.436116267895,12.9964564726427,63.0746275600137));
#185827=CARTESIAN_POINT('Ctrl Pts',(112.387345784475,13.1951971218302,63.2469597722259));
#185828=CARTESIAN_POINT('Ctrl Pts',(112.929322628392,13.2733025335376,63.3453035071527));
#185829=CARTESIAN_POINT('Ctrl Pts',(113.998736369994,13.3594764034328,63.5402847871116));
#185830=CARTESIAN_POINT('Ctrl Pts',(114.526067620634,13.3699725817027,63.636788996925));
#185831=CARTESIAN_POINT('Ctrl Pts',(115.589865537427,13.3258847307165,63.8310683835618));
#185832=CARTESIAN_POINT('Ctrl Pts',(116.123598056301,13.26996623454,63.9281991926313));
#185833=CARTESIAN_POINT('Ctrl Pts',(117.14090877311,13.0980526102477,64.1125799098966));
#185834=CARTESIAN_POINT('Ctrl Pts',(117.622521233663,12.9879604505935,64.1996577800957));
#185835=CARTESIAN_POINT('Ctrl Pts',(118.581644607567,12.7108171472874,64.3734971949168));
#185836=CARTESIAN_POINT('Ctrl Pts',(119.05885117347,12.5424808386177,64.4602302397172));
#185837=CARTESIAN_POINT('Ctrl Pts',(120.269595561566,12.0350375352245,64.6801119316231));
#185838=CARTESIAN_POINT('Ctrl Pts',(120.987439448018,11.653405886996,64.8102647342016));
#185839=CARTESIAN_POINT('Ctrl Pts',(122.178969727996,10.8671355693131,65.023761533422));
#185840=CARTESIAN_POINT('Ctrl Pts',(122.668385475051,10.4918447060699,65.1109046216195));
#185841=CARTESIAN_POINT('Ctrl Pts',(123.982720490917,9.33072838523825,65.3447478333531));
#185842=CARTESIAN_POINT('Ctrl Pts',(124.740910296221,8.46625703112186,65.4788130603719));
#185843=CARTESIAN_POINT('Ctrl Pts',(126.455173626972,5.91411760544508,65.774825677581));
#185844=CARTESIAN_POINT('Ctrl Pts',(127.079976237841,4.23004003854899,65.8738275446836));
#185845=CARTESIAN_POINT('Ctrl Pts',(127.521918605851,2.06461609064611,65.9335986559922));
#185846=CARTESIAN_POINT('Ctrl Pts',(127.604696841238,1.44096751722637,65.9425181099599));
#185847=CARTESIAN_POINT('Ctrl Pts',(127.69157796131,0.0271249438644891,
65.9420409839444));
#185848=CARTESIAN_POINT('Ctrl Pts',(127.671382588491,-0.761203590754172,
65.9279951415855));
#185849=CARTESIAN_POINT('Ctrl Pts',(127.536960431653,-1.96405359133338,
65.8868217647676));
#185850=CARTESIAN_POINT('Ctrl Pts',(127.470080944866,-2.38431013298785,
65.8686512888352));
#185851=CARTESIAN_POINT('Ctrl Pts',(127.250851352109,-3.44076794102639,
65.8134560522557));
#185852=CARTESIAN_POINT('Ctrl Pts',(127.071723489756,-4.07190745080252,
65.7713949622881));
#185853=CARTESIAN_POINT('Ctrl Pts',(126.695431475237,-5.10151277065501,
65.6849024742793));
#185854=CARTESIAN_POINT('Ctrl Pts',(126.523343650202,-5.50839992739275,
65.6457971789059));
#185855=CARTESIAN_POINT('Ctrl Pts',(125.975698112604,-6.64449929089201,
65.5231111714808));
#185856=CARTESIAN_POINT('Ctrl Pts',(125.552386113774,-7.34984794587801,
65.4305106531452));
#185857=CARTESIAN_POINT('Ctrl Pts',(124.692802634908,-8.5243484946755,65.2464636238839));
#185858=CARTESIAN_POINT('Ctrl Pts',(124.279879019018,-9.01139391102258,
65.158963056486));
#185859=CARTESIAN_POINT('Ctrl Pts',(123.504906080448,-9.80077588539326,
64.9947841549065));
#185860=CARTESIAN_POINT('Ctrl Pts',(123.158325467745,-10.1173084808118,
64.921297478286));
#185861=CARTESIAN_POINT('Ctrl Pts',(121.653507750894,-11.3509702814949,
64.6035100892289));
#185862=CARTESIAN_POINT('Ctrl Pts',(120.354661175151,-12.0919359407802,
64.3343530005754));
#185863=CARTESIAN_POINT('Ctrl Pts',(118.275599042184,-12.8452877574834,
63.9028610817256));
#185864=CARTESIAN_POINT('Ctrl Pts',(117.559956039398,-13.0353633222222,
63.7541248279207));
#185865=CARTESIAN_POINT('Ctrl Pts',(116.098077005825,-13.2928123808805,
63.4513742094034));
#185866=CARTESIAN_POINT('Ctrl Pts',(115.350465393516,-13.3584111921057,
63.2968556267763));
#185867=CARTESIAN_POINT('Ctrl Pts',(114.602892108729,-13.3589088885551,
63.1424102408455));
#185868=CARTESIAN_POINT('Ctrl Pts',(118.780288836585,-12.65925539485,64.0299347534317));
#185869=CARTESIAN_POINT('Ctrl Pts',(116.595886786058,-13.41168843809,63.5767576294984));
#185870=CARTESIAN_POINT('Ctrl Pts',(111.830850147376,-13.70841130529,62.5933831941367));
#185871=CARTESIAN_POINT('Ctrl Pts',(105.43801356551,-10.41179638488,61.2650246644536));
#185872=CARTESIAN_POINT('Ctrl Pts',(101.552926167766,-4.27236878269199,
60.4241256289558));
#185873=CARTESIAN_POINT('Ctrl Pts',(101.239769506549,3.03341342218001,60.277543059066));
#185874=CARTESIAN_POINT('Ctrl Pts',(104.588660551712,9.51104676477801,60.8427940066454));
#185875=CARTESIAN_POINT('Ctrl Pts',(110.689622481059,13.39202095622,61.9429960129963));
#185876=CARTESIAN_POINT('Ctrl Pts',(117.881403714159,13.61677928444,63.2552328709365));
#185877=CARTESIAN_POINT('Ctrl Pts',(124.204921450959,10.12395787573,64.3986955598227));
#185878=CARTESIAN_POINT('Ctrl Pts',(127.938147290484,3.86714835369002,65.0386539963514));
#185879=CARTESIAN_POINT('Ctrl Pts',(128.066238757101,-3.44544911201899,
64.977841801965));
#185880=CARTESIAN_POINT('Ctrl Pts',(124.558608071853,-9.81738869681499,
64.2103132850727));
#185881=CARTESIAN_POINT('Ctrl Pts',(118.37727253464,-13.50903793953,62.9230665989836));
#185882=CARTESIAN_POINT('Ctrl Pts',(111.214209907503,-13.51252273589,61.4449905453842));
#185883=CARTESIAN_POINT('Ctrl Pts',(105.029423762811,-9.82689168621099,
60.1570731257995));
#185884=CARTESIAN_POINT('Ctrl Pts',(101.515833922933,-3.45837583796399,
59.3883862608075));
#185885=CARTESIAN_POINT('Ctrl Pts',(101.637084647361,3.85432706958101,59.3262443542041));
#185886=CARTESIAN_POINT('Ctrl Pts',(105.364455691648,10.11474245491,59.9650647281479));
#185887=CARTESIAN_POINT('Ctrl Pts',(111.684703352911,13.6136855823,61.1078917755655));
#185888=CARTESIAN_POINT('Ctrl Pts',(118.876690783495,13.39589393048,62.4201687144387));
#185889=CARTESIAN_POINT('Ctrl Pts',(124.981283460208,9.52082779822401,63.5210764701047));
#185890=CARTESIAN_POINT('Ctrl Pts',(128.336221493489,3.04643677302001,64.0875028389717));
#185891=CARTESIAN_POINT('Ctrl Pts',(128.029940821833,-4.25967593268699,
63.9422568327185));
#185892=CARTESIAN_POINT('Ctrl Pts',(124.150443525087,-10.40283497821,63.102444408213));
#185893=CARTESIAN_POINT('Ctrl Pts',(117.761271878036,-13.70586824618,61.7747982732376));
#185894=CARTESIAN_POINT('Ctrl Pts',(110.611146146451,-13.266999738,60.2992369099465));
#185895=CARTESIAN_POINT('Ctrl Pts',(104.656537122664,-9.20604594134699,
59.0560616135515));
#185896=CARTESIAN_POINT('Ctrl Pts',(101.527525978629,-2.63171028823999,
58.3621296473937));
#185897=CARTESIAN_POINT('Ctrl Pts',(102.082749950975,4.66113184975601,58.3843440158345));
#185898=CARTESIAN_POINT('Ctrl Pts',(106.175050417972,10.68137526099,59.0940998377636));
#185899=CARTESIAN_POINT('Ctrl Pts',(112.691393445214,13.78560312531,60.275044153263));
#185900=CARTESIAN_POINT('Ctrl Pts',(119.857699338531,13.12557900619,61.5823290820643));
#185901=CARTESIAN_POINT('Ctrl Pts',(123.765651770777,10.29802594745,62.2848213563563));
#185902=CARTESIAN_POINT('Ctrl Pts',(125.237609274392,8.47864527230601,62.5423720795936));
#185903=CARTESIAN_POINT('Ctrl Pts',(118.79600886555,-12.65925539485,63.9490626188614));
#185904=CARTESIAN_POINT('Ctrl Pts',(116.611606815023,-13.41168843809,63.4958854949296));
#185905=CARTESIAN_POINT('Ctrl Pts',(111.846570176341,-13.70841130529,62.5125110595679));
#185906=CARTESIAN_POINT('Ctrl Pts',(105.453733594475,-10.41179638488,61.1841525298833));
#185907=CARTESIAN_POINT('Ctrl Pts',(101.568646196731,-4.27236878269199,
60.343253494387));
#185908=CARTESIAN_POINT('Ctrl Pts',(101.255489535514,3.03341342218001,60.1966709244958));
#185909=CARTESIAN_POINT('Ctrl Pts',(104.604380580679,9.51104676477801,60.7619218720702));
#185910=CARTESIAN_POINT('Ctrl Pts',(110.705342510024,13.39202095622,61.862123878426));
#185911=CARTESIAN_POINT('Ctrl Pts',(117.897123743125,13.61677928444,63.1743607363613));
#185912=CARTESIAN_POINT('Ctrl Pts',(124.220641479924,10.12395787573,64.3178234252538));
#185913=CARTESIAN_POINT('Ctrl Pts',(127.953867319451,3.86714835369002,64.9577818617762));
#185914=CARTESIAN_POINT('Ctrl Pts',(128.081958786066,-3.44544911201899,
64.8969696673961));
#185915=CARTESIAN_POINT('Ctrl Pts',(124.574328100819,-9.81738869681499,
64.1294411504975));
#185916=CARTESIAN_POINT('Ctrl Pts',(118.392992563605,-13.50903793953,62.8421944644147));
#185917=CARTESIAN_POINT('Ctrl Pts',(111.229929936469,-13.51252273589,61.364118410809));
#185918=CARTESIAN_POINT('Ctrl Pts',(105.045143791776,-9.82689168621099,
60.0762009912307));
#185919=CARTESIAN_POINT('Ctrl Pts',(101.531553951899,-3.45837583796399,
59.3075141262323));
#185920=CARTESIAN_POINT('Ctrl Pts',(101.652804676326,3.85432706958101,59.2453722196352));
#185921=CARTESIAN_POINT('Ctrl Pts',(105.380175720614,10.11474245491,59.8841925935776));
#185922=CARTESIAN_POINT('Ctrl Pts',(111.700423381876,13.6136855823,61.0270196409966));
#185923=CARTESIAN_POINT('Ctrl Pts',(118.89241081246,13.39589393048,62.3392965798684));
#185924=CARTESIAN_POINT('Ctrl Pts',(124.997003489173,9.52082779822401,63.4402043355359));
#185925=CARTESIAN_POINT('Ctrl Pts',(128.351941522455,3.04643677302001,64.0066307044015));
#185926=CARTESIAN_POINT('Ctrl Pts',(128.045660850798,-4.25967593268699,
63.8613846981497));
#185927=CARTESIAN_POINT('Ctrl Pts',(124.166163554053,-10.40283497821,63.0215722736427));
#185928=CARTESIAN_POINT('Ctrl Pts',(117.776991907001,-13.70586824618,61.6939261386688));
#185929=CARTESIAN_POINT('Ctrl Pts',(110.626866175417,-13.266999738,60.2183647753762));
#185930=CARTESIAN_POINT('Ctrl Pts',(104.672257151629,-9.20604594134699,
58.9751894789827));
#185931=CARTESIAN_POINT('Ctrl Pts',(101.543246007595,-2.63171028823999,
58.2812575128234));
#185932=CARTESIAN_POINT('Ctrl Pts',(102.09846997994,4.66113184975601,58.3034718812657));
#185933=CARTESIAN_POINT('Ctrl Pts',(106.190770446937,10.68137526099,59.0132277031934));
#185934=CARTESIAN_POINT('Ctrl Pts',(112.70711347418,13.78560312531,60.1941720186878));
#185935=CARTESIAN_POINT('Ctrl Pts',(119.873419367496,13.12557900619,61.501456947494));
#185936=CARTESIAN_POINT('Ctrl Pts',(123.781371799742,10.29802594745,62.203949221786));
#185937=CARTESIAN_POINT('Ctrl Pts',(125.253329303358,8.47864527230601,62.4614999450184));
#185938=CARTESIAN_POINT('Ctrl Pts',(118.811728894516,-12.65925539485,63.8681904842861));
#185939=CARTESIAN_POINT('Ctrl Pts',(116.627326843988,-13.41168843809,63.4150133603608));
#185940=CARTESIAN_POINT('Ctrl Pts',(111.862290205306,-13.70841130529,62.4316389249991));
#185941=CARTESIAN_POINT('Ctrl Pts',(105.469453623441,-10.41179638488,61.103280395308));
#185942=CARTESIAN_POINT('Ctrl Pts',(101.584366225696,-4.27236878269199,
60.2623813598182));
#185943=CARTESIAN_POINT('Ctrl Pts',(101.271209564481,3.03341342218001,60.1157987899205));
#185944=CARTESIAN_POINT('Ctrl Pts',(104.620100609644,9.51104676477801,60.6810497375008));
#185945=CARTESIAN_POINT('Ctrl Pts',(110.72106253899,13.39202095622,61.7812517438507));
#185946=CARTESIAN_POINT('Ctrl Pts',(117.91284377209,13.61677928444,63.0934886017919));
#185947=CARTESIAN_POINT('Ctrl Pts',(124.236361508889,10.12395787573,64.2369512906843));
#185948=CARTESIAN_POINT('Ctrl Pts',(127.969587348416,3.86714835369002,64.8769097272067));
#185949=CARTESIAN_POINT('Ctrl Pts',(128.097678815032,-3.44544911201899,
64.8160975328265));
#185950=CARTESIAN_POINT('Ctrl Pts',(124.590048129785,-9.81738869681499,
64.048569015928));
#185951=CARTESIAN_POINT('Ctrl Pts',(118.40871259257,-13.50903793953,62.7613223298451));
#185952=CARTESIAN_POINT('Ctrl Pts',(111.245649965435,-13.51252273589,61.2832462762396));
#185953=CARTESIAN_POINT('Ctrl Pts',(105.060863820742,-9.82689168621099,
59.9953288566611));
#185954=CARTESIAN_POINT('Ctrl Pts',(101.547273980864,-3.45837583796399,
59.2266419916628));
#185955=CARTESIAN_POINT('Ctrl Pts',(101.668524705291,3.85432706958101,59.1645000850656));
#185956=CARTESIAN_POINT('Ctrl Pts',(105.39589574958,10.11474245491,59.8033204590023));
#185957=CARTESIAN_POINT('Ctrl Pts',(111.716143410841,13.6136855823,60.9461475064271));
#185958=CARTESIAN_POINT('Ctrl Pts',(118.908130841426,13.39589393048,62.2584244452931));
#185959=CARTESIAN_POINT('Ctrl Pts',(125.012723518138,9.52082779822401,63.3593322009671));
#185960=CARTESIAN_POINT('Ctrl Pts',(128.367661551421,3.04643677302001,63.9257585698262));
#185961=CARTESIAN_POINT('Ctrl Pts',(128.061380879763,-4.25967593268699,
63.7805125635808));
#185962=CARTESIAN_POINT('Ctrl Pts',(124.181883583019,-10.40283497821,62.9407001390674));
#185963=CARTESIAN_POINT('Ctrl Pts',(117.792711935966,-13.70586824618,61.6130540041));
#185964=CARTESIAN_POINT('Ctrl Pts',(110.642586204383,-13.266999738,60.1374926408009));
#185965=CARTESIAN_POINT('Ctrl Pts',(104.687977180594,-9.20604594134699,
58.8943173444139));
#185966=CARTESIAN_POINT('Ctrl Pts',(101.558966036561,-2.63171028823999,
58.2003853782481));
#185967=CARTESIAN_POINT('Ctrl Pts',(102.114190008905,4.66113184975601,58.2225997466969));
#185968=CARTESIAN_POINT('Ctrl Pts',(106.206490475903,10.68137526099,58.9323555686181));
#185969=CARTESIAN_POINT('Ctrl Pts',(112.722833503145,13.78560312531,60.1132998841184));
#185970=CARTESIAN_POINT('Ctrl Pts',(119.889139396462,13.12557900619,61.4205848129187));
#185971=CARTESIAN_POINT('Ctrl Pts',(123.797091828709,10.29802594745,62.1230770872107));
#185972=CARTESIAN_POINT('Ctrl Pts',(125.269049332323,8.47864527230601,62.3806278104489));
#185973=CARTESIAN_POINT('Ctrl Pts',(118.827448923481,-12.65925539485,63.787318349716));
#185974=CARTESIAN_POINT('Ctrl Pts',(116.643046872953,-13.41168843809,63.334141225792));
#185975=CARTESIAN_POINT('Ctrl Pts',(111.878010234271,-13.70841130529,62.3507667904303));
#185976=CARTESIAN_POINT('Ctrl Pts',(105.485173652407,-10.41179638488,61.0224082607378));
#185977=CARTESIAN_POINT('Ctrl Pts',(101.600086254661,-4.27236878269199,
60.1815092252494));
#185978=CARTESIAN_POINT('Ctrl Pts',(101.286929593446,3.03341342218001,60.0349266553503));
#185979=CARTESIAN_POINT('Ctrl Pts',(104.635820638609,9.51104676477801,60.6001776029319));
#185980=CARTESIAN_POINT('Ctrl Pts',(110.736782567956,13.39202095622,61.7003796092806));
#185981=CARTESIAN_POINT('Ctrl Pts',(117.928563801055,13.61677928444,63.012616467223));
#185982=CARTESIAN_POINT('Ctrl Pts',(124.252081537856,10.12395787573,64.1560791561089));
#185983=CARTESIAN_POINT('Ctrl Pts',(127.985307377381,3.86714835369002,64.7960375926378));
#185984=CARTESIAN_POINT('Ctrl Pts',(128.113398843998,-3.44544911201899,
64.7352253982512));
#185985=CARTESIAN_POINT('Ctrl Pts',(124.60576815875,-9.81738869681499,63.9676968813591));
#185986=CARTESIAN_POINT('Ctrl Pts',(118.424432621537,-13.50903793953,62.6804501952698));
#185987=CARTESIAN_POINT('Ctrl Pts',(111.2613699944,-13.51252273589,61.2023741416707));
#185988=CARTESIAN_POINT('Ctrl Pts',(105.076583849708,-9.82689168621099,
59.9144567220858));
#185989=CARTESIAN_POINT('Ctrl Pts',(101.562994009829,-3.45837583796399,
59.145769857094));
#185990=CARTESIAN_POINT('Ctrl Pts',(101.684244734257,3.85432706958101,59.0836279504903));
#185991=CARTESIAN_POINT('Ctrl Pts',(105.411615778545,10.11474245491,59.7224483244321));
#185992=CARTESIAN_POINT('Ctrl Pts',(111.731863439807,13.6136855823,60.8652753718517));
#185993=CARTESIAN_POINT('Ctrl Pts',(118.923850870392,13.39589393048,62.177552310723));
#185994=CARTESIAN_POINT('Ctrl Pts',(125.028443547103,9.52082779822401,63.2784600663983));
#185995=CARTESIAN_POINT('Ctrl Pts',(128.383381580386,3.04643677302001,63.844886435256));
#185996=CARTESIAN_POINT('Ctrl Pts',(128.077100908728,-4.25967593268699,
63.699640429012));
#185997=CARTESIAN_POINT('Ctrl Pts',(124.197603611984,-10.40283497821,62.8598280044972));
#185998=CARTESIAN_POINT('Ctrl Pts',(117.808431964931,-13.70586824618,61.5321818695312));
#185999=CARTESIAN_POINT('Ctrl Pts',(110.658306233348,-13.266999738,60.0566205062307));
#186000=CARTESIAN_POINT('Ctrl Pts',(104.703697209559,-9.20604594134699,
58.8134452098451));
#186001=CARTESIAN_POINT('Ctrl Pts',(101.574686065526,-2.63171028823999,
58.119513243678));
#186002=CARTESIAN_POINT('Ctrl Pts',(102.12991003787,4.66113184975601,58.1417276121281));
#186003=CARTESIAN_POINT('Ctrl Pts',(106.222210504869,10.68137526099,58.8514834340479));
#186004=CARTESIAN_POINT('Ctrl Pts',(112.73855353211,13.78560312531,60.0324277495495));
#186005=CARTESIAN_POINT('Ctrl Pts',(119.904859425427,13.12557900619,61.3397126783486));
#186006=CARTESIAN_POINT('Ctrl Pts',(123.812811857674,10.29802594745,62.0422049526405));
#186007=CARTESIAN_POINT('Ctrl Pts',(125.284769361288,8.47864527230601,62.29975567588));
#186008=CARTESIAN_POINT('',(121.944453055693,11.3913829322761,61.9325710545576));
#186009=CARTESIAN_POINT('Ctrl Pts',(114.603093529674,-13.3575246836283,
63.1414291237798));
#186010=CARTESIAN_POINT('Ctrl Pts',(113.990399128991,-13.3579712225348,
63.0150807040448));
#186011=CARTESIAN_POINT('Ctrl Pts',(113.377598459867,-13.3149179937247,
62.8889596251551));
#186012=CARTESIAN_POINT('Ctrl Pts',(112.541949711885,-13.1951183779221,
62.7164706356709));
#186013=CARTESIAN_POINT('Ctrl Pts',(112.313896472985,-13.156046153819,62.6693449757331));
#186014=CARTESIAN_POINT('Ctrl Pts',(111.83368261156,-13.0600519108201,62.5699333560895));
#186015=CARTESIAN_POINT('Ctrl Pts',(111.582250764064,-13.0016394937268,
62.5177690092337));
#186016=CARTESIAN_POINT('Ctrl Pts',(110.736367646641,-12.7777826485591,
62.3420902766842));
#186017=CARTESIAN_POINT('Ctrl Pts',(110.150989524571,-12.5763566939195,
62.2201551227424));
#186018=CARTESIAN_POINT('Ctrl Pts',(109.257110310978,-12.1959211403354,
62.0338541239351));
#186019=CARTESIAN_POINT('Ctrl Pts',(108.9373775311,-12.0442498276864,61.9671938147611));
#186020=CARTESIAN_POINT('Ctrl Pts',(108.437323988917,-11.7818132071309,
61.8629873299671));
#186021=CARTESIAN_POINT('Ctrl Pts',(108.252845595734,-11.6792645761009,
61.8245546881921));
#186022=CARTESIAN_POINT('Ctrl Pts',(107.722356500847,-11.3674350300325,
61.7140987949494));
#186023=CARTESIAN_POINT('Ctrl Pts',(107.382965637735,-11.1463339682985,
61.643515121726));
#186024=CARTESIAN_POINT('Ctrl Pts',(106.761349151428,-10.6989278292122,
61.5139348992215));
#186025=CARTESIAN_POINT('Ctrl Pts',(106.476918491919,-10.4758011555531,
61.4545116996931));
#186026=CARTESIAN_POINT('Ctrl Pts',(106.087648063399,-10.1430954036906,
61.3727449161145));
#186027=CARTESIAN_POINT('Ctrl Pts',(105.974841627675,-10.0432137601379,
61.3489939526357));
#186028=CARTESIAN_POINT('Ctrl Pts',(105.72663775211,-9.81551201509332,61.2965812295366));
#186029=CARTESIAN_POINT('Ctrl Pts',(105.592182627668,-9.68665969691926,
61.2680810899966));
#186030=CARTESIAN_POINT('Ctrl Pts',(105.164012850198,-9.25828802477612,
61.1770676842786));
#186031=CARTESIAN_POINT('Ctrl Pts',(104.881607468134,-8.94702551784144,
61.1166754190157));
#186032=CARTESIAN_POINT('Ctrl Pts',(104.451172343227,-8.42494967512794,
61.0243126220469));
#186033=CARTESIAN_POINT('Ctrl Pts',(104.293679228789,-8.22228192446864,
60.9904257600904));
#186034=CARTESIAN_POINT('Ctrl Pts',(103.899979252224,-7.6845451033037,60.905480482773));
#186035=CARTESIAN_POINT('Ctrl Pts',(103.672797452591,-7.3425411504999,60.8562241236915));
#186036=CARTESIAN_POINT('Ctrl Pts',(103.288487906928,-6.70271984641751,
60.7724586431333));
#186037=CARTESIAN_POINT('Ctrl Pts',(103.126113862337,-6.40813787795307,
60.7368922019998));
#186038=CARTESIAN_POINT('Ctrl Pts',(102.736314164748,-5.63405145937279,
60.6510334912565));
#186039=CARTESIAN_POINT('Ctrl Pts',(102.525359677965,-5.1458644023358,60.604152712784));
#186040=CARTESIAN_POINT('Ctrl Pts',(102.284288680491,-4.48130736408789,
60.5491035341268));
#186041=CARTESIAN_POINT('Ctrl Pts',(102.227659467904,-4.31500044297743,
60.5360292504741));
#186042=CARTESIAN_POINT('Ctrl Pts',(102.133336072709,-4.0187047394526,60.5139403222276));
#186043=CARTESIAN_POINT('Ctrl Pts',(102.094324477853,-3.8892840859754,60.5046909968951));
#186044=CARTESIAN_POINT('Ctrl Pts',(101.940901963849,-3.35065271176429,
60.4678551803245));
#186045=CARTESIAN_POINT('Ctrl Pts',(101.844081773649,-2.93620937072642,
60.4434556038056));
#186046=CARTESIAN_POINT('Ctrl Pts',(101.714392725028,-2.23381695610262,
60.408965602747));
#186047=CARTESIAN_POINT('Ctrl Pts',(101.67096999485,-1.94792448789282,60.3968094589545));
#186048=CARTESIAN_POINT('Ctrl Pts',(101.598473111033,-1.34246095847658,
60.375049049133));
#186049=CARTESIAN_POINT('Ctrl Pts',(101.571488054667,-1.02260856995072,
60.3658534673498));
#186050=CARTESIAN_POINT('Ctrl Pts',(101.532822286821,-0.238679710083945,
60.3488377832787));
#186051=CARTESIAN_POINT('Ctrl Pts',(101.533348262028,0.226107876286849,
60.3434631935411));
#186052=CARTESIAN_POINT('Ctrl Pts',(101.581616641272,1.15641839581304,60.3420158780094));
#186053=CARTESIAN_POINT('Ctrl Pts',(101.629688549945,1.62196856350683,60.346019299718));
#186054=CARTESIAN_POINT('Ctrl Pts',(101.730287773067,2.26629813330814,60.3581004771507));
#186055=CARTESIAN_POINT('Ctrl Pts',(101.76255554724,2.44830131570257,60.3622439241077));
#186056=CARTESIAN_POINT('Ctrl Pts',(101.827890671572,2.77686456409949,60.3710068909742));
#186057=CARTESIAN_POINT('Ctrl Pts',(101.859650753442,2.92354205228318,60.3753860595442));
#186058=CARTESIAN_POINT('Ctrl Pts',(101.938522433542,3.25999282947182,60.3864959044332));
#186059=CARTESIAN_POINT('Ctrl Pts',(101.98728453623,3.44911749528315,60.3935302965536));
#186060=CARTESIAN_POINT('Ctrl Pts',(102.169929054132,4.09851524021271,60.4204630601464));
#186061=CARTESIAN_POINT('Ctrl Pts',(102.324406955099,4.55282166789539,60.4441827223226));
#186062=CARTESIAN_POINT('Ctrl Pts',(102.576490407172,5.18328923546371,60.4844168993197));
#186063=CARTESIAN_POINT('Ctrl Pts',(102.654850537588,5.36740702646428,60.4970871990457));
#186064=CARTESIAN_POINT('Ctrl Pts',(102.822598854042,5.73874769461095,60.5245706972002));
#186065=CARTESIAN_POINT('Ctrl Pts',(102.912291951358,5.92583453852271,60.5394502848693));
#186066=CARTESIAN_POINT('Ctrl Pts',(103.157878185703,6.40955926284171,60.5806142866393));
#186067=CARTESIAN_POINT('Ctrl Pts',(103.320515703495,6.70267873209368,60.6082769725156));
#186068=CARTESIAN_POINT('Ctrl Pts',(103.782695926849,7.46762915852709,60.6877061879545));
#186069=CARTESIAN_POINT('Ctrl Pts',(104.101032348795,7.92777487488369,60.7432166644688));
#186070=CARTESIAN_POINT('Ctrl Pts',(104.643581968534,8.61506328198171,60.838455772304));
#186071=CARTESIAN_POINT('Ctrl Pts',(104.849376098324,8.85730205307405,60.8747076682046));
#186072=CARTESIAN_POINT('Ctrl Pts',(105.211916819241,9.25360446151154,60.9386398140822));
#186073=CARTESIAN_POINT('Ctrl Pts',(105.364160067242,9.41176931881221,60.9654981659304));
#186074=CARTESIAN_POINT('Ctrl Pts',(105.914805879218,9.95582270744608,61.062741440476));
#186075=CARTESIAN_POINT('Ctrl Pts',(106.33373432711,10.3202241310802,61.1368991003599));
#186076=CARTESIAN_POINT('Ctrl Pts',(107.046553904861,10.8662092021664,61.2638464902885));
#186077=CARTESIAN_POINT('Ctrl Pts',(107.327877569277,11.0648492747695,61.3141227043485));
#186078=CARTESIAN_POINT('Ctrl Pts',(107.771210615629,11.3528471796474,61.393726947745));
#186079=CARTESIAN_POINT('Ctrl Pts',(107.928209517917,11.4502500553402,61.421988950572));
#186080=CARTESIAN_POINT('Ctrl Pts',(108.474337294025,11.7735030045097,61.5205427731455));
#186081=CARTESIAN_POINT('Ctrl Pts',(108.872912821115,11.9828420737496,61.5928613985386));
#186082=CARTESIAN_POINT('Ctrl Pts',(109.663541350441,12.3475323162289,61.7365354725881));
#186083=CARTESIAN_POINT('Ctrl Pts',(110.054473613383,12.5054328828345,61.8076726200996));
#186084=CARTESIAN_POINT('Ctrl Pts',(110.609223455065,12.6982886925242,61.9084425988955));
#186085=CARTESIAN_POINT('Ctrl Pts',(110.767469955839,12.7498663302499,61.9371682360402));
#186086=CARTESIAN_POINT('Ctrl Pts',(111.363249485869,12.9311309394018,62.04519857268));
#186087=CARTESIAN_POINT('Ctrl Pts',(111.806667237708,13.0403185425305,62.1254509820834));
#186088=CARTESIAN_POINT('Ctrl Pts',(112.862110238992,13.2418699389597,62.316686915616));
#186089=CARTESIAN_POINT('Ctrl Pts',(113.477839764735,13.3143197715914,62.4283409326716));
#186090=CARTESIAN_POINT('Ctrl Pts',(114.365275936587,13.3555827718125,62.5896880030508));
#186091=CARTESIAN_POINT('Ctrl Pts',(114.635529499474,13.3597800420865,62.6388792844762));
#186092=CARTESIAN_POINT('Ctrl Pts',(115.186965896953,13.3512644341853,62.7393961135737));
#186093=CARTESIAN_POINT('Ctrl Pts',(115.468148714922,13.337841615018,62.7907406314709));
#186094=CARTESIAN_POINT('Ctrl Pts',(116.121802857897,13.2853458171502,62.9102231332582));
#186095=CARTESIAN_POINT('Ctrl Pts',(116.493733483146,13.2392582619345,62.9782804683887));
#186096=CARTESIAN_POINT('Ctrl Pts',(117.082406931017,13.1400188510727,63.0857750469098));
#186097=CARTESIAN_POINT('Ctrl Pts',(117.300830280039,13.0973365343111,63.1256103648593));
#186098=CARTESIAN_POINT('Ctrl Pts',(117.647318249538,13.0201361057555,63.1886519774697));
#186099=CARTESIAN_POINT('Ctrl Pts',(117.776029707718,12.9893386278848,63.2120349993459));
#186100=CARTESIAN_POINT('Ctrl Pts',(118.260920770969,12.8652535870903,63.2999850507719));
#186101=CARTESIAN_POINT('Ctrl Pts',(118.613584209923,12.7585192387634,63.3636844776029));
#186102=CARTESIAN_POINT('Ctrl Pts',(119.474635456428,12.4573514852675,63.5190997726643));
#186103=CARTESIAN_POINT('Ctrl Pts',(119.977084610835,12.2453701443103,63.6097570810696));
#186104=CARTESIAN_POINT('Ctrl Pts',(120.806472734739,11.8333804996213,63.7593664832312));
#186105=CARTESIAN_POINT('Ctrl Pts',(121.140919423904,11.6488090164101,63.8196801823219));
#186106=CARTESIAN_POINT('Ctrl Pts',(121.838290784598,11.2236733904382,63.9453837087774));
#186107=CARTESIAN_POINT('Ctrl Pts',(122.198770165219,10.9788615259388,64.010324535685));
#186108=CARTESIAN_POINT('Ctrl Pts',(122.802348646447,10.5237137485963,64.1189457270106));
#186109=CARTESIAN_POINT('Ctrl Pts',(123.051293885605,10.3213649095711,64.163709649583));
#186110=CARTESIAN_POINT('Ctrl Pts',(123.439276718796,9.98155152818562,64.2331514937779));
#186111=CARTESIAN_POINT('Ctrl Pts',(123.583108545896,9.84978394265308,64.2588181818252));
#186112=CARTESIAN_POINT('Ctrl Pts',(123.821575857368,9.6212240690469,64.3011787757565));
#186113=CARTESIAN_POINT('Ctrl Pts',(123.917666763204,9.52619733132495,64.3181895209984));
#186114=CARTESIAN_POINT('Ctrl Pts',(124.324516419101,9.11117979478066,64.3899863887137));
#186115=CARTESIAN_POINT('Ctrl Pts',(124.620735406745,8.77640159922797,64.4416812578214));
#186116=CARTESIAN_POINT('Ctrl Pts',(125.129629014704,8.13966932052117,64.5299469177379));
#186117=CARTESIAN_POINT('Ctrl Pts',(125.347834048512,7.8422862133304,64.5676025306936));
#186118=CARTESIAN_POINT('Ctrl Pts',(125.713892906783,7.29809807681613,64.6305708973747));
#186119=CARTESIAN_POINT('Ctrl Pts',(125.866638509675,7.05465995084478,64.6567534501411));
#186120=CARTESIAN_POINT('Ctrl Pts',(126.269425035444,6.36511094393209,64.7254520590792));
#186121=CARTESIAN_POINT('Ctrl Pts',(126.502612962555,5.90876842958892,64.7648118599198));
#186122=CARTESIAN_POINT('Ctrl Pts',(126.884997982173,5.04273407190103,64.8281914697899));
#186123=CARTESIAN_POINT('Ctrl Pts',(127.041565807407,4.63636429983549,64.8536389038463));
#186124=CARTESIAN_POINT('Ctrl Pts',(127.226180793314,4.07732050402872,64.8826839013661));
#186125=CARTESIAN_POINT('Ctrl Pts',(127.27182798204,3.93066265157856,64.8897586781975));
#186126=CARTESIAN_POINT('Ctrl Pts',(127.358921359513,3.63274878555362,64.9029866170164));
#186127=CARTESIAN_POINT('Ctrl Pts',(127.400206249997,3.48163242963907,64.9091052687959));
#186128=CARTESIAN_POINT('Ctrl Pts',(127.586855709503,2.74799610622354,64.9360194697212));
#186129=CARTESIAN_POINT('Ctrl Pts',(127.69576976199,2.1559534205035,64.9493034547574));
#186130=CARTESIAN_POINT('Ctrl Pts',(127.802864054099,1.23846863873338,64.9582071320374));
#186131=CARTESIAN_POINT('Ctrl Pts',(127.828961547112,0.916315746228356,
64.9591552854305));
#186132=CARTESIAN_POINT('Ctrl Pts',(127.852757527575,0.394883279898758,
64.9573298409709));
#186133=CARTESIAN_POINT('Ctrl Pts',(127.85751236588,0.195904482082526,64.9558467078465));
#186134=CARTESIAN_POINT('Ctrl Pts',(127.859073009378,-0.513478792821087,
64.9477028540574));
#186135=CARTESIAN_POINT('Ctrl Pts',(127.831788820181,-1.02393759294173,
64.9365714982727));
#186136=CARTESIAN_POINT('Ctrl Pts',(127.725292970965,-1.99321268054657,
64.9047196082197));
#186137=CARTESIAN_POINT('Ctrl Pts',(127.650897750762,-2.45261458369212,
64.8849346109271));
#186138=CARTESIAN_POINT('Ctrl Pts',(127.506858377997,-3.11974815108727,
64.8488157552804));
#186139=CARTESIAN_POINT('Ctrl Pts',(127.455719142738,-3.331326615975,64.8362361394663));
#186140=CARTESIAN_POINT('Ctrl Pts',(127.230599950141,-4.17144759019554,
64.7817289946605));
#186141=CARTESIAN_POINT('Ctrl Pts',(127.015836385385,-4.7879106457032,64.7315324928152));
#186142=CARTESIAN_POINT('Ctrl Pts',(126.593301402418,-5.76812496720764,
64.635693285313));
#186143=CARTESIAN_POINT('Ctrl Pts',(126.410655559543,-6.14321701101547,
64.594877149254));
#186144=CARTESIAN_POINT('Ctrl Pts',(126.116202692636,-6.68329148997502,
64.5300454745718));
#186145=CARTESIAN_POINT('Ctrl Pts',(126.017270402795,-6.8556181497677,64.508400080519));
#186146=CARTESIAN_POINT('Ctrl Pts',(125.650352077731,-7.46331190321983,
64.4286298455308));
#186147=CARTESIAN_POINT('Ctrl Pts',(125.361457757297,-7.88560860618325,
64.3667151681209));
#186148=CARTESIAN_POINT('Ctrl Pts',(124.836072736936,-8.56612860916472,
64.2547677919321));
#186149=CARTESIAN_POINT('Ctrl Pts',(124.611730848969,-8.83414045673399,
64.2071328096745));
#186150=CARTESIAN_POINT('Ctrl Pts',(124.27609758154,-9.20389656957432,64.1358983363456));
#186151=CARTESIAN_POINT('Ctrl Pts',(124.173072262069,-9.31351948663113,
64.1140357286447));
#186152=CARTESIAN_POINT('Ctrl Pts',(123.78437624167,-9.71287015076297,64.0315317062448));
#186153=CARTESIAN_POINT('Ctrl Pts',(123.48720079234,-9.99065485180476,63.9684561583088));
#186154=CARTESIAN_POINT('Ctrl Pts',(122.675414468006,-10.6816878256984,
63.7968605506766));
#186155=CARTESIAN_POINT('Ctrl Pts',(122.141137842134,-11.0709225469987,
63.6844921281256));
#186156=CARTESIAN_POINT('Ctrl Pts',(121.31913387786,-11.5804619472397,63.5126042031283));
#186157=CARTESIAN_POINT('Ctrl Pts',(121.051033409447,-11.7338699920835,
63.4566841379968));
#186158=CARTESIAN_POINT('Ctrl Pts',(120.48833618688,-12.0300134240572,63.3396299291538));
#186159=CARTESIAN_POINT('Ctrl Pts',(120.193096662126,-12.171537845633,63.2783952214694));
#186160=CARTESIAN_POINT('Ctrl Pts',(119.588988333214,-12.4335413509648,
63.1533780556106));
#186161=CARTESIAN_POINT('Ctrl Pts',(119.279988086963,-12.5537086435395,
63.089547306203));
#186162=CARTESIAN_POINT('Ctrl Pts',(118.773320790979,-12.728412563179,62.9848087207607));
#186163=CARTESIAN_POINT('Ctrl Pts',(118.57815607602,-12.7904962382517,62.9444465084282));
#186164=CARTESIAN_POINT('Ctrl Pts',(118.257514733425,-12.8839711460315,
62.8780449302931));
#186165=CARTESIAN_POINT('Ctrl Pts',(118.133022492874,-12.9181922210399,
62.852239704963));
#186166=CARTESIAN_POINT('Ctrl Pts',(117.607496050715,-13.0539948854129,
62.7432115424693));
#186167=CARTESIAN_POINT('Ctrl Pts',(117.202250300468,-13.1377049950957,
62.6589251792515));
#186168=CARTESIAN_POINT('Ctrl Pts',(116.461094617542,-13.2538240182983,
62.5049356440482));
#186169=CARTESIAN_POINT('Ctrl Pts',(116.126187755109,-13.292848399882,62.4354379192552));
#186170=CARTESIAN_POINT('Ctrl Pts',(115.43101844711,-13.3464515712576,62.2913908971411));
#186171=CARTESIAN_POINT('Ctrl Pts',(115.07058717598,-13.3591407803865,62.2168100328529));
#186172=CARTESIAN_POINT('Ctrl Pts',(114.253503630022,-13.3538765372014,
62.0479170822489));
#186173=CARTESIAN_POINT('Ctrl Pts',(113.796836931941,-13.3268147639553,
61.9536501983375));
#186174=CARTESIAN_POINT('Ctrl Pts',(112.964062028573,-13.2329114512214,
61.7818653406047));
#186175=CARTESIAN_POINT('Ctrl Pts',(112.587127111227,-13.1734090120992,
61.7041812070377));
#186176=CARTESIAN_POINT('Ctrl Pts',(112.036675326882,-13.0609800384358,
61.5906465634742));
#186177=CARTESIAN_POINT('Ctrl Pts',(111.860603977884,-13.0211014353704,
61.5543083486569));
#186178=CARTESIAN_POINT('Ctrl Pts',(111.545434807673,-12.9425739328143,
61.4891650733484));
#186179=CARTESIAN_POINT('Ctrl Pts',(111.406031208211,-12.9052902859207,
61.4603151595134));
#186180=CARTESIAN_POINT('Ctrl Pts',(111.102252667029,-12.8183942533883,
61.3973426970148));
#186181=CARTESIAN_POINT('Ctrl Pts',(110.938332612829,-12.7678588459617,
61.3632998685479));
#186182=CARTESIAN_POINT('Ctrl Pts',(110.347535637555,-12.5725450063597,
61.240432705736));
#186183=CARTESIAN_POINT('Ctrl Pts',(109.926918022354,-12.4082541610369,
61.1526297606735));
#186184=CARTESIAN_POINT('Ctrl Pts',(109.329464262365,-12.138287729035,61.0278643889183));
#186185=CARTESIAN_POINT('Ctrl Pts',(109.145197258408,-12.0497436547561,
60.9893774315288));
#186186=CARTESIAN_POINT('Ctrl Pts',(108.759968061027,-11.8534066209237,
60.908960060838));
#186187=CARTESIAN_POINT('Ctrl Pts',(108.559508436871,-11.7445672318688,
60.8671377064275));
#186188=CARTESIAN_POINT('Ctrl Pts',(108.055610129353,-11.4537736453416,
60.7620247599346));
#186189=CARTESIAN_POINT('Ctrl Pts',(107.756174536728,-11.2645262356543,
60.699578638175));
#186190=CARTESIAN_POINT('Ctrl Pts',(106.954972154193,-10.7117862354286,
60.5323380063867));
#186191=CARTESIAN_POINT('Ctrl Pts',(106.469346848412,-10.3238003590776,
60.430794959707));
#186192=CARTESIAN_POINT('Ctrl Pts',(105.870541743564,-9.77082063875566,
60.3048069856716));
#186193=CARTESIAN_POINT('Ctrl Pts',(105.730755572468,-9.63581577841111,
60.2753387427463));
#186194=CARTESIAN_POINT('Ctrl Pts',(105.472453944849,-9.37481351423717,
60.2207164513879));
#186195=CARTESIAN_POINT('Ctrl Pts',(105.353510507324,-9.24968093933481,
60.1954818877547));
#186196=CARTESIAN_POINT('Ctrl Pts',(104.81733432664,-8.6625411529408,60.08134731658));
#186197=CARTESIAN_POINT('Ctrl Pts',(104.43019108471,-8.17220202521634,59.9978719182808));
#186198=CARTESIAN_POINT('Ctrl Pts',(103.885593824562,-7.3738994096418,59.8794922208696));
#186199=CARTESIAN_POINT('Ctrl Pts',(103.703348083998,-7.08354261682428,
59.839674168317));
#186200=CARTESIAN_POINT('Ctrl Pts',(103.439669756716,-6.62581518192857,
59.7818667741538));
#186201=CARTESIAN_POINT('Ctrl Pts',(103.35035870522,-6.46316754664296,59.7622509382567));
#186202=CARTESIAN_POINT('Ctrl Pts',(103.033510526149,-5.85706529756014,
59.692494099151));
#186203=CARTESIAN_POINT('Ctrl Pts',(102.826653077162,-5.40225905357714,
59.6466007045469));
#186204=CARTESIAN_POINT('Ctrl Pts',(102.487068323946,-4.53055175746746,
59.5699066853281));
#186205=CARTESIAN_POINT('Ctrl Pts',(102.348276674649,-4.11609423383822,
59.5379299371577));
#186206=CARTESIAN_POINT('Ctrl Pts',(102.180257084585,-3.51796211383271,
59.4978670558067));
#186207=CARTESIAN_POINT('Ctrl Pts',(102.134062417779,-3.33931372374463,
59.4866507402423));
#186208=CARTESIAN_POINT('Ctrl Pts',(101.971958078993,-2.65323768786973,
59.4464249527177));
#186209=CARTESIAN_POINT('Ctrl Pts',(101.882101016615,-2.13973237506003,
59.422296002869));
#186210=CARTESIAN_POINT('Ctrl Pts',(101.757857086493,-1.07291576295581,
59.3844126710314));
#186211=CARTESIAN_POINT('Ctrl Pts',(101.727303810479,-0.519109698192167,
59.371394102765));
#186212=CARTESIAN_POINT('Ctrl Pts',(101.731271809209,0.274346340597185,
59.3623652755867));
#186213=CARTESIAN_POINT('Ctrl Pts',(101.738722628582,0.514141584924893,
59.3608965589136));
#186214=CARTESIAN_POINT('Ctrl Pts',(101.768809432482,1.04017549387642,59.3604753263735));
#186215=CARTESIAN_POINT('Ctrl Pts',(101.794145457511,1.32626989230036,59.3620899828508));
#186216=CARTESIAN_POINT('Ctrl Pts',(101.874479959946,1.99401728511432,59.370063845904));
#186217=CARTESIAN_POINT('Ctrl Pts',(101.936676246456,2.37479690063633,59.377850930817));
#186218=CARTESIAN_POINT('Ctrl Pts',(102.050301619527,2.92186233280537,59.3935397502688));
#186219=CARTESIAN_POINT('Ctrl Pts',(102.088826290953,3.09089056309865,59.399021021663));
#186220=CARTESIAN_POINT('Ctrl Pts',(102.166564929235,3.40370280264371,59.4103262432364));
#186221=CARTESIAN_POINT('Ctrl Pts',(102.204929901869,3.54772295953015,59.4159951034999));
#186222=CARTESIAN_POINT('Ctrl Pts',(102.30030540256,3.88284706408452,59.4302602563008));
#186223=CARTESIAN_POINT('Ctrl Pts',(102.359217431612,4.07335890134234,59.4391968220913));
#186224=CARTESIAN_POINT('Ctrl Pts',(102.534693125102,4.59887196798283,59.4662316344382));
#186225=CARTESIAN_POINT('Ctrl Pts',(102.660388063998,4.93071944386864,59.4860603876968));
#186226=CARTESIAN_POINT('Ctrl Pts',(103.0150981765,5.76676162757953,59.5433859493828));
#186227=CARTESIAN_POINT('Ctrl Pts',(103.262488366159,6.26295389947851,59.5844864238727));
#186228=CARTESIAN_POINT('Ctrl Pts',(103.71339776416,7.04464691947722,59.6610255955423));
#186229=CARTESIAN_POINT('Ctrl Pts',(103.899616607257,7.34056394672016,59.692991585322));
#186230=CARTESIAN_POINT('Ctrl Pts',(104.339338176009,7.98291811571845,59.7692257793045));
#186231=CARTESIAN_POINT('Ctrl Pts',(104.598490075028,8.32538958658205,59.8146705297761));
#186232=CARTESIAN_POINT('Ctrl Pts',(105.105329222861,8.93206696220115,59.9042118354609));
#186233=CARTESIAN_POINT('Ctrl Pts',(105.348527623573,9.2001531104887,59.9473810850936));
#186234=CARTESIAN_POINT('Ctrl Pts',(105.694706448755,9.55122332925254,60.0088055477242));
#186235=CARTESIAN_POINT('Ctrl Pts',(105.788489308381,9.64348721462895,60.0254426646478));
#186236=CARTESIAN_POINT('Ctrl Pts',(106.015931419453,9.86050293142528,60.0657680598013));
#186237=CARTESIAN_POINT('Ctrl Pts',(106.150731784925,9.98377978897873,60.089654911538));
#186238=CARTESIAN_POINT('Ctrl Pts',(106.486688665688,10.2783280034598,60.1492089906058));
#186239=CARTESIAN_POINT('Ctrl Pts',(106.690552131011,10.4464005601864,60.1853657100624));
#186240=CARTESIAN_POINT('Ctrl Pts',(107.210323154609,10.849351275424,60.2777666053788));
#186241=CARTESIAN_POINT('Ctrl Pts',(107.532048619494,11.0764650379316,60.3351836812339));
#186242=CARTESIAN_POINT('Ctrl Pts',(108.13145529298,11.4609626719913,60.4427131326062));
#186243=CARTESIAN_POINT('Ctrl Pts',(108.406027674603,11.6234316216101,60.4921430409791));
#186244=CARTESIAN_POINT('Ctrl Pts',(109.181586494496,12.0454063103798,60.6321540848603));
#186245=CARTESIAN_POINT('Ctrl Pts',(109.694045300436,12.2832223442261,60.7251031530113));
#186246=CARTESIAN_POINT('Ctrl Pts',(110.656858173676,12.6565525849736,60.9001867589728));
#186247=CARTESIAN_POINT('Ctrl Pts',(111.103320675212,12.8025175224817,60.9816012342247));
#186248=CARTESIAN_POINT('Ctrl Pts',(111.702412603349,12.9624121663959,61.0906657332844));
#186249=CARTESIAN_POINT('Ctrl Pts',(111.849070138252,12.9987659994906,61.1173423283447));
#186250=CARTESIAN_POINT('Ctrl Pts',(112.182266698995,13.0750468217819,61.1778755177285));
#186251=CARTESIAN_POINT('Ctrl Pts',(112.368911696764,13.1133759068098,61.2117386811187));
#186252=CARTESIAN_POINT('Ctrl Pts',(113.270743147748,13.2777166253032,61.3752322029498));
#186253=CARTESIAN_POINT('Ctrl Pts',(113.995967849278,13.3471278131987,61.5063279130925));
#186254=CARTESIAN_POINT('Ctrl Pts',(114.931297617332,13.3587583818418,61.6763206603305));
#186255=CARTESIAN_POINT('Ctrl Pts',(115.140952460877,13.3563277685502,61.7144808472429));
#186256=CARTESIAN_POINT('Ctrl Pts',(115.865296282167,13.3305319188046,61.8464562028411));
#186257=CARTESIAN_POINT('Ctrl Pts',(116.379135200741,13.2818084306026,61.9403139337308));
#186258=CARTESIAN_POINT('Ctrl Pts',(117.438215883638,13.1174641702283,62.1336861666048));
#186259=CARTESIAN_POINT('Ctrl Pts',(117.982728905425,12.9968181043918,62.2330586948186));
#186260=CARTESIAN_POINT('Ctrl Pts',(118.711899683826,12.7842611624471,62.3655861347268));
#186261=CARTESIAN_POINT('Ctrl Pts',(118.904663692281,12.7230242617307,62.4005577440117));
#186262=CARTESIAN_POINT('Ctrl Pts',(119.490819433883,12.5213878339624,62.5066990972885));
#186263=CARTESIAN_POINT('Ctrl Pts',(119.879181565658,12.3661949774273,62.5767623580464));
#186264=CARTESIAN_POINT('Ctrl Pts',(120.689759635771,11.9963169906521,62.7227149854452));
#186265=CARTESIAN_POINT('Ctrl Pts',(121.109729522615,11.7764848283689,62.7981634508621));
#186266=CARTESIAN_POINT('Ctrl Pts',(121.693251830559,11.430033722902,62.9030226659486));
#186267=CARTESIAN_POINT('Ctrl Pts',(121.867128623607,11.3212721891398,62.9342721120155));
#186268=CARTESIAN_POINT('Ctrl Pts',(122.240682633842,11.0753959751299,63.0014485617585));
#186269=CARTESIAN_POINT('Ctrl Pts',(122.43936170471,10.9367007592207,63.0372046986133));
#186270=CARTESIAN_POINT('Ctrl Pts',(122.935071864527,10.5700890771558,63.1263830059613));
#186271=CARTESIAN_POINT('Ctrl Pts',(123.226772673359,10.334696351177,63.178827132535));
#186272=CARTESIAN_POINT('Ctrl Pts',(123.7207520185,9.90013447494156,63.2672995646437));
#186273=CARTESIAN_POINT('Ctrl Pts',(123.927459598736,9.70617552676832,63.3042067513528));
#186274=CARTESIAN_POINT('Ctrl Pts',(124.254676364109,9.37854786336352,63.3623258709278));
#186275=CARTESIAN_POINT('Ctrl Pts',(124.379001624991,9.2488473685348,63.3843308828263));
#186276=CARTESIAN_POINT('Ctrl Pts',(124.699904082089,8.89988778401403,63.4408761111308));
#186277=CARTESIAN_POINT('Ctrl Pts',(124.891816860741,8.67643052291237,63.4744247705943));
#186278=CARTESIAN_POINT('Ctrl Pts',(125.541904278356,7.8663041210362,63.5875186164069));
#186279=CARTESIAN_POINT('Ctrl Pts',(125.95941217609,7.24570641563249,63.6590240656914));
#186280=CARTESIAN_POINT('Ctrl Pts',(126.472481886112,6.32860285449774,63.7456313903176));
#186281=CARTESIAN_POINT('Ctrl Pts',(126.612395247932,6.05754829899803,63.7690772116149));
#186282=CARTESIAN_POINT('Ctrl Pts',(126.852014643002,5.55245517862468,63.8089334125459));
#186283=CARTESIAN_POINT('Ctrl Pts',(126.954540209441,5.31977410356813,63.8258684256751));
#186284=CARTESIAN_POINT('Ctrl Pts',(127.164228419731,4.80526949483151,63.8602328269393));
#186285=CARTESIAN_POINT('Ctrl Pts',(127.26873559346,4.5223202814057,63.8771599645833));
#186286=CARTESIAN_POINT('Ctrl Pts',(127.462351927687,3.93882141893424,63.9078548047792));
#186287=CARTESIAN_POINT('Ctrl Pts',(127.550706990229,3.63801922852502,63.9214742870542));
#186288=CARTESIAN_POINT('Ctrl Pts',(127.664862727722,3.19205124165761,63.9382519208259));
#186289=CARTESIAN_POINT('Ctrl Pts',(127.69896186235,3.04908434874342,63.9431242382031));
#186290=CARTESIAN_POINT('Ctrl Pts',(127.767163462692,2.74056520066485,63.9525216878805));
#186291=CARTESIAN_POINT('Ctrl Pts',(127.800499166874,2.57484993737074,63.9568853802017));
#186292=CARTESIAN_POINT('Ctrl Pts',(127.964565906962,1.67129687725773,63.9771156891775));
#186293=CARTESIAN_POINT('Ctrl Pts',(128.036688072689,0.922605975005862,
63.9812836524761));
#186294=CARTESIAN_POINT('Ctrl Pts',(128.053091050656,-0.218177777081743,
63.9702774680057));
#186295=CARTESIAN_POINT('Ctrl Pts',(128.041997650652,-0.609788606400816,
63.9633379770788));
#186296=CARTESIAN_POINT('Ctrl Pts',(127.983621303946,-1.43100647438174,
63.9421188950817));
#186297=CARTESIAN_POINT('Ctrl Pts',(127.932691422753,-1.86039262337457,
63.9271497778164));
#186298=CARTESIAN_POINT('Ctrl Pts',(127.782740837144,-2.75777645693293,
63.8875453859669));
#186299=CARTESIAN_POINT('Ctrl Pts',(127.679129178069,-3.22497637434037,
63.862097099584));
#186300=CARTESIAN_POINT('Ctrl Pts',(127.51060112987,-3.82953454489757,63.8220021106787));
#186301=CARTESIAN_POINT('Ctrl Pts',(127.467871035817,-3.97339419455098,
63.8119133852327));
#186302=CARTESIAN_POINT('Ctrl Pts',(127.37534701678,-4.26651999497137,63.7901883057961));
#186303=CARTESIAN_POINT('Ctrl Pts',(127.325352687751,-4.41560557477619,
63.7785128416517));
#186304=CARTESIAN_POINT('Ctrl Pts',(127.207009551048,-4.74884976880704,
63.7510372798475));
#186305=CARTESIAN_POINT('Ctrl Pts',(127.137197990067,-4.93245846603757,
63.7349359962479));
#186306=CARTESIAN_POINT('Ctrl Pts',(126.845763014017,-5.6510844006793,63.6682125453016));
#186307=CARTESIAN_POINT('Ctrl Pts',(126.593564354546,-6.1731528873397,63.6115520130025));
#186308=CARTESIAN_POINT('Ctrl Pts',(126.167987863232,-6.92690905571856,
63.5180417570039));
#186309=CARTESIAN_POINT('Ctrl Pts',(126.01864264227,-7.17275495149999,63.4855035475113));
#186310=CARTESIAN_POINT('Ctrl Pts',(125.514303532643,-7.94627078660459,
63.3763704607782));
#186311=CARTESIAN_POINT('Ctrl Pts',(125.129643765918,-8.45393733842158,
63.2942226989373));
#186312=CARTESIAN_POINT('Ctrl Pts',(124.41935384716,-9.26357998023273,63.1436351485535));
#186313=CARTESIAN_POINT('Ctrl Pts',(124.110988560638,-9.58136061805701,
63.078597795913));
#186314=CARTESIAN_POINT('Ctrl Pts',(123.67262068835,-9.98900230521898,62.9861548190844));
#186315=CARTESIAN_POINT('Ctrl Pts',(123.555961958387,-10.0935683813924,
62.9615455628932));
#186316=CARTESIAN_POINT('Ctrl Pts',(123.155247880156,-10.4398460019076,
62.8770102525141));
#186317=CARTESIAN_POINT('Ctrl Pts',(122.862685236626,-10.671328784282,62.8152862900541));
#186318=CARTESIAN_POINT('Ctrl Pts',(122.159797824742,-11.180264880214,62.6672746406744));
#186319=CARTESIAN_POINT('Ctrl Pts',(121.742468657624,-11.4476761776246,
62.5796037064665));
#186320=CARTESIAN_POINT('Ctrl Pts',(121.148562699661,-11.7826136804606,
62.4555314190495));
#186321=CARTESIAN_POINT('Ctrl Pts',(120.983377506188,-11.8711632738061,
62.4210970945461));
#186322=CARTESIAN_POINT('Ctrl Pts',(120.508991344542,-12.1125350242583,
62.3223919198141));
#186323=CARTESIAN_POINT('Ctrl Pts',(120.195543029721,-12.2567548452443,
62.2573852988289));
#186324=CARTESIAN_POINT('Ctrl Pts',(119.354447999188,-12.6040699377361,
62.0832447920378));
#186325=CARTESIAN_POINT('Ctrl Pts',(118.818218563734,-12.7856804477348,
61.972519341747));
#186326=CARTESIAN_POINT('Ctrl Pts',(118.052684370993,-12.9894033090308,
61.8142392204107));
#186327=CARTESIAN_POINT('Ctrl Pts',(117.831096009594,-13.0420435768363,
61.7684005408198));
#186328=CARTESIAN_POINT('Ctrl Pts',(117.309005986134,-13.1511373540155,
61.6602808060396));
#186329=CARTESIAN_POINT('Ctrl Pts',(117.007659058018,-13.2026988463473,
61.5978008101505));
#186330=CARTESIAN_POINT('Ctrl Pts',(116.214693322051,-13.3091861549093,
61.4333122961321));
#186331=CARTESIAN_POINT('Ctrl Pts',(115.720822048658,-13.3464251704356,
61.3307864325695));
#186332=CARTESIAN_POINT('Ctrl Pts',(114.888702387365,-13.361368067599,61.1582188651562));
#186333=CARTESIAN_POINT('Ctrl Pts',(114.550685094673,-13.3541943840866,
61.0881692756249));
#186334=CARTESIAN_POINT('Ctrl Pts',(114.016990026164,-13.3219977754822,
60.9777369926673));
#186335=CARTESIAN_POINT('Ctrl Pts',(113.820801172636,-13.3056779377818,
60.9371780810214));
#186336=CARTESIAN_POINT('Ctrl Pts',(113.44540351328,-13.2658306572991,60.8596592629578));
#186337=CARTESIAN_POINT('Ctrl Pts',(113.266119931918,-13.243005196364,60.8226742777998));
#186338=CARTESIAN_POINT('Ctrl Pts',(112.685274192186,-13.1566587477565,
60.7029039921763));
#186339=CARTESIAN_POINT('Ctrl Pts',(112.285854357962,-13.0779213233347,
60.6206285512193));
#186340=CARTESIAN_POINT('Ctrl Pts',(111.641850478772,-12.9187461343833,
60.4877295429215));
#186341=CARTESIAN_POINT('Ctrl Pts',(111.394559370389,-12.8496737090834,
60.4366376755461));
#186342=CARTESIAN_POINT('Ctrl Pts',(111.009641701352,-12.7294158528691,
60.3569250514861));
#186343=CARTESIAN_POINT('Ctrl Pts',(110.870468796284,-12.6832664974673,
60.3280639465654));
#186344=CARTESIAN_POINT('Ctrl Pts',(110.477781840778,-12.5453673215558,
60.2464941364024));
#186345=CARTESIAN_POINT('Ctrl Pts',(110.226382355776,-12.4479236444354,
60.1941216196114));
#186346=CARTESIAN_POINT('Ctrl Pts',(109.250792830405,-12.0339139003957,
59.9906797226233));
#186347=CARTESIAN_POINT('Ctrl Pts',(108.550967101069,-11.6575470229572,
59.8443399405338));
#186348=CARTESIAN_POINT('Ctrl Pts',(107.628519625626,-11.048776635446,59.6512194976542));
#186349=CARTESIAN_POINT('Ctrl Pts',(107.373529672581,-10.8671978593662,
59.5978079690161));
#186350=CARTESIAN_POINT('Ctrl Pts',(106.850294642191,-10.4658965124238,
59.4881725473388));
#186351=CARTESIAN_POINT('Ctrl Pts',(106.583500592508,-10.2441546883599,
59.4322671054812));
#186352=CARTESIAN_POINT('Ctrl Pts',(105.966221290747,-9.68851907553079,
59.3027759329984));
#186353=CARTESIAN_POINT('Ctrl Pts',(105.624189772017,-9.34486134790611,
59.2308502016745));
#186354=CARTESIAN_POINT('Ctrl Pts',(105.21524486331,-8.88506388942526,59.143984133459));
#186355=CARTESIAN_POINT('Ctrl Pts',(105.129875396587,-8.78610309430652,
59.1257962386369));
#186356=CARTESIAN_POINT('Ctrl Pts',(104.911838299881,-8.52544257103956,
59.0791880659478));
#186357=CARTESIAN_POINT('Ctrl Pts',(104.781603815473,-8.36186613787664,
59.0512003770977));
#186358=CARTESIAN_POINT('Ctrl Pts',(104.436161232675,-7.90606134668474,
58.9766487802347));
#186359=CARTESIAN_POINT('Ctrl Pts',(104.228840159586,-7.60763160336805,
58.9315488782535));
#186360=CARTESIAN_POINT('Ctrl Pts',(103.83041101936,-6.98127575743222,58.8445096536074));
#186361=CARTESIAN_POINT('Ctrl Pts',(103.640375514436,-6.65262136003278,
58.8027776458652));
#186362=CARTESIAN_POINT('Ctrl Pts',(103.287879427994,-5.97939108095663,
58.7248534295313));
#186363=CARTESIAN_POINT('Ctrl Pts',(103.125455760468,-5.63474501456723,
58.6886681631905));
#186364=CARTESIAN_POINT('Ctrl Pts',(102.754489486424,-4.75364716805687,
58.6051776592044));
#186365=CARTESIAN_POINT('Ctrl Pts',(102.564614963436,-4.20889762287071,
58.5616052014557));
#186366=CARTESIAN_POINT('Ctrl Pts',(102.317229074917,-3.31966234096533,
58.5029892298193));
#186367=CARTESIAN_POINT('Ctrl Pts',(102.237119228676,-2.98175700208736,
58.4834744150268));
#186368=CARTESIAN_POINT('Ctrl Pts',(102.143823970434,-2.50557116089143,
58.4595633350259));
#186369=CARTESIAN_POINT('Ctrl Pts',(102.119427593877,-2.36980130658472,
58.4531465691196));
#186370=CARTESIAN_POINT('Ctrl Pts',(102.057617438939,-1.99210732526352,
58.4364040758067));
#186371=CARTESIAN_POINT('Ctrl Pts',(102.024755348943,-1.74946093646282,
58.4269048771876));
#186372=CARTESIAN_POINT('Ctrl Pts',(101.951565432986,-1.07054042208053,
58.4038874117156));
#186373=CARTESIAN_POINT('Ctrl Pts',(101.92581646583,-0.632606724627165,
58.3931148720186));
#186374=CARTESIAN_POINT('Ctrl Pts',(101.918350216145,0.0517733804404306,
58.382898292293));
#186375=CARTESIAN_POINT('Ctrl Pts',(101.922279839217,0.298038649552079,
58.3805672237773));
#186376=CARTESIAN_POINT('Ctrl Pts',(101.944293541922,0.813131802559715,
58.378508659593));
#186377=CARTESIAN_POINT('Ctrl Pts',(101.963675680976,1.08191790442571,58.3790382325729));
#186378=CARTESIAN_POINT('Ctrl Pts',(102.024269068008,1.67818784857894,58.3837204401154));
#186379=CARTESIAN_POINT('Ctrl Pts',(102.06941541431,2.00528819897112,58.3886621852478));
#186380=CARTESIAN_POINT('Ctrl Pts',(102.252549109192,3.05167094571696,58.4119970789988));
#186381=CARTESIAN_POINT('Ctrl Pts',(102.436612856431,3.76271670958568,58.4395009374162));
#186382=CARTESIAN_POINT('Ctrl Pts',(102.740773885875,4.63307852635012,58.4875084157057));
#186383=CARTESIAN_POINT('Ctrl Pts',(102.807447662412,4.81138131478656,58.4981222182692));
#186384=CARTESIAN_POINT('Ctrl Pts',(102.962955648451,5.20157270975982,58.5230916109307));
#186385=CARTESIAN_POINT('Ctrl Pts',(103.053513781866,5.41274488839898,58.5377660429203));
#186386=CARTESIAN_POINT('Ctrl Pts',(103.372229421647,6.10639564721346,58.589905492546));
#186387=CARTESIAN_POINT('Ctrl Pts',(103.623788036266,6.57780657297239,58.6318163633313));
#186388=CARTESIAN_POINT('Ctrl Pts',(104.01468572894,7.21706777752638,58.6983130368445));
#186389=CARTESIAN_POINT('Ctrl Pts',(104.131951611141,7.39894151672453,58.7184069722934));
#186390=CARTESIAN_POINT('Ctrl Pts',(104.375829286261,7.75808924965383,58.7605178909363));
#186391=CARTESIAN_POINT('Ctrl Pts',(104.502509670978,7.93532551059293,58.7825480811276));
#186392=CARTESIAN_POINT('Ctrl Pts',(104.806069119068,8.33909106701811,58.8356272618875));
#186393=CARTESIAN_POINT('Ctrl Pts',(104.986036476691,8.56323146678516,58.8673059483869));
#186394=CARTESIAN_POINT('Ctrl Pts',(105.524614237572,9.19157060047395,58.9625122021844));
#186395=CARTESIAN_POINT('Ctrl Pts',(105.900780706283,9.58020194423673,59.0294844967148));
#186396=CARTESIAN_POINT('Ctrl Pts',(106.432416330796,10.0652659689011,59.1241819595329));
#186397=CARTESIAN_POINT('Ctrl Pts',(106.568062064155,10.1839519667814,59.1483446829909));
#186398=CARTESIAN_POINT('Ctrl Pts',(107.11332517056,10.6411825880818,59.2454578434561));
#186399=CARTESIAN_POINT('Ctrl Pts',(107.540906406993,10.9570240383061,59.3217094916449));
#186400=CARTESIAN_POINT('Ctrl Pts',(108.449380222038,11.5470377948677,59.4843150452172));
#186401=CARTESIAN_POINT('Ctrl Pts',(108.931802983704,11.8188256777415,59.570955894139));
#186402=CARTESIAN_POINT('Ctrl Pts',(109.640610281318,12.1617693850152,59.6989191194564));
#186403=CARTESIAN_POINT('Ctrl Pts',(109.855119747486,12.2585817559649,59.7377272239079));
#186404=CARTESIAN_POINT('Ctrl Pts',(110.401281311468,12.487708913009,59.8367735521387));
#186405=CARTESIAN_POINT('Ctrl Pts',(110.736014572361,12.6124110844187,59.8977177565918));
#186406=CARTESIAN_POINT('Ctrl Pts',(111.511137194225,12.8655114715568,60.0390407043567));
#186407=CARTESIAN_POINT('Ctrl Pts',(111.954399339892,12.9847903415047,60.119988526134));
#186408=CARTESIAN_POINT('Ctrl Pts',(112.542832544102,13.1095830730738,60.2271441174067));
#186409=CARTESIAN_POINT('Ctrl Pts',(112.683481461978,13.1369421209752,60.2527344594261));
#186410=CARTESIAN_POINT('Ctrl Pts',(113.020421265411,13.1965521251643,60.3139608042953));
#186411=CARTESIAN_POINT('Ctrl Pts',(113.21704746674,13.2265732737833,60.3496295521908));
#186412=CARTESIAN_POINT('Ctrl Pts',(113.770245336926,13.2978721680189,60.4499160475966));
#186413=CARTESIAN_POINT('Ctrl Pts',(114.128105727272,13.328749185719,60.5147370715045));
#186414=CARTESIAN_POINT('Ctrl Pts',(115.009487793307,13.3680815138604,60.6745963157342));
#186415=CARTESIAN_POINT('Ctrl Pts',(115.533764431818,13.3597628890784,60.7698056127025));
#186416=CARTESIAN_POINT('Ctrl Pts',(116.396792464626,13.2942870369107,60.9267630984186));
#186417=CARTESIAN_POINT('Ctrl Pts',(116.736951665917,13.2550401511003,60.988686797659));
#186418=CARTESIAN_POINT('Ctrl Pts',(117.530664211689,13.1317629284829,61.1333196159765));
#186419=CARTESIAN_POINT('Ctrl Pts',(117.982615037574,13.0369043089246,61.2158285959178));
#186420=CARTESIAN_POINT('Ctrl Pts',(118.753447251637,12.8315730227818,61.3565373467627));
#186421=CARTESIAN_POINT('Ctrl Pts',(119.075219000797,12.7322883896691,61.4152341570359));
#186422=CARTESIAN_POINT('Ctrl Pts',(119.517472589056,12.576433390397,61.4955966707724));
#186423=CARTESIAN_POINT('Ctrl Pts',(119.641491808641,12.5305504516168,61.5180962721938));
#186424=CARTESIAN_POINT('Ctrl Pts',(119.933687864695,12.4172323908981,61.5710059976784));
#186425=CARTESIAN_POINT('Ctrl Pts',(120.101077122722,12.3481859799875,61.6012415758661));
#186426=CARTESIAN_POINT('Ctrl Pts',(120.846030158616,12.0223757780061,61.735561964536));
#186427=CARTESIAN_POINT('Ctrl Pts',(121.406999501065,11.7263298088096,61.8361064899413));
#186428=CARTESIAN_POINT('Ctrl Pts',(121.944453055693,11.3913829322761,61.9325710545576));
#186429=CARTESIAN_POINT('',(106.661976927588,10.2288565995845,58.9614167108613));
#186430=CARTESIAN_POINT('Ctrl Pts',(106.661350930769,10.2295773178667,58.9618221141476));
#186431=CARTESIAN_POINT('Ctrl Pts',(106.825922779295,10.3703884207358,58.993811800576));
#186432=CARTESIAN_POINT('Ctrl Pts',(106.993951579293,10.506970800954,59.0264734536535));
#186433=CARTESIAN_POINT('Ctrl Pts',(107.16541057696,10.6393620137197,59.0598018729417));
#186434=CARTESIAN_POINT('Ctrl Pts',(107.336748834558,10.7716599976416,59.0931068226209));
#186435=CARTESIAN_POINT('Ctrl Pts',(107.51151194005,10.8997723090449,59.1270774986143));
#186436=CARTESIAN_POINT('Ctrl Pts',(107.689704886371,11.0236957681757,59.1617148714556));
#186437=CARTESIAN_POINT('Ctrl Pts',(107.732786344196,11.0536565684669,59.1700891003352));
#186438=CARTESIAN_POINT('Ctrl Pts',(107.776068430774,11.0833723346163,59.1785023276886));
#186439=CARTESIAN_POINT('Ctrl Pts',(107.819551448625,11.1128426273365,59.1869546123197));
#186440=CARTESIAN_POINT('Ctrl Pts',(107.837833222047,11.1252329636295,59.1905082468226));
#186441=CARTESIAN_POINT('Ctrl Pts',(107.856150514099,11.137579906738,59.1940687854823));
#186442=CARTESIAN_POINT('Ctrl Pts',(107.87450335123,11.1498834153761,59.1976362334398));
#186443=CARTESIAN_POINT('Ctrl Pts',(107.891038087995,11.1609680926477,59.2008502767225));
#186444=CARTESIAN_POINT('Ctrl Pts',(107.907599232881,11.17201591509,59.2040694532496));
#186445=CARTESIAN_POINT('Ctrl Pts',(107.924204326524,11.1830384116525,59.2072971725923));
#186446=CARTESIAN_POINT('Ctrl Pts',(108.004056796198,11.2360446512704,59.2228189977908));
#186447=CARTESIAN_POINT('Ctrl Pts',(108.084832644889,11.2883974214026,59.2385203105836));
#186448=CARTESIAN_POINT('Ctrl Pts',(108.166019887746,11.3397585101557,59.2543015907009));
#186449=CARTESIAN_POINT('Ctrl Pts',(108.210746221189,11.3680535119403,59.2629955526071));
#186450=CARTESIAN_POINT('Ctrl Pts',(108.255596909759,11.3960483115572,59.2717136868221));
#186451=CARTESIAN_POINT('Ctrl Pts',(108.30048285165,11.4236920848158,59.2804386736227));
#186452=CARTESIAN_POINT('Ctrl Pts',(108.312416977699,11.4310419199901,59.2827584443096));
#186453=CARTESIAN_POINT('Ctrl Pts',(108.324353582836,11.4383669634109,59.2850786968848));
#186454=CARTESIAN_POINT('Ctrl Pts',(108.336290964591,11.4456663086518,59.28739910042));
#186455=CARTESIAN_POINT('Ctrl Pts',(108.348094863653,11.4528840332931,59.2896935574187));
#186456=CARTESIAN_POINT('Ctrl Pts',(108.359907957709,11.4600817926637,59.291989801752));
#186457=CARTESIAN_POINT('Ctrl Pts',(108.371730890304,11.4672600077199,59.2942879585132));
#186458=CARTESIAN_POINT('Ctrl Pts',(108.544485776277,11.572146990161,59.3278682742278));
#186459=CARTESIAN_POINT('Ctrl Pts',(108.719293829397,11.6728372308274,59.3618476871988));
#186460=CARTESIAN_POINT('Ctrl Pts',(108.896190732468,11.769405294605,59.3962331334954));
#186461=CARTESIAN_POINT('Ctrl Pts',(109.073164318318,11.8660152195306,59.4306334854885));
#186462=CARTESIAN_POINT('Ctrl Pts',(109.252228929304,11.9584995635849,59.4654402936222));
#186463=CARTESIAN_POINT('Ctrl Pts',(109.43344545626,12.0468875256908,59.5006653939349));
#186464=CARTESIAN_POINT('Ctrl Pts',(109.567751674034,12.112395087758,59.5267720083435));
#186465=CARTESIAN_POINT('Ctrl Pts',(109.703240449451,12.1756516537283,59.5531084898193));
#186466=CARTESIAN_POINT('Ctrl Pts',(109.839943719786,12.2366521263733,59.579681046371));
#186467=CARTESIAN_POINT('Ctrl Pts',(109.913322473696,12.26939559081,59.5939445024184));
#186468=CARTESIAN_POINT('Ctrl Pts',(109.987051250195,12.3014887635243,59.6082759963045));
#186469=CARTESIAN_POINT('Ctrl Pts',(110.061135575156,12.3329290625992,59.6226766021551));
#186470=CARTESIAN_POINT('Ctrl Pts',(110.090300640985,12.3453062880477,59.6283457449576));
#186471=CARTESIAN_POINT('Ctrl Pts',(110.119520813447,12.3575823177664,59.6340255994577));
#186472=CARTESIAN_POINT('Ctrl Pts',(110.148796444678,12.3697569395208,59.6397162341043));
#186473=CARTESIAN_POINT('Ctrl Pts',(110.172247679429,12.3795094162652,59.6442747151128));
#186474=CARTESIAN_POINT('Ctrl Pts',(110.19573662675,12.3891976567719,59.6488405267389));
#186475=CARTESIAN_POINT('Ctrl Pts',(110.219242226367,12.3988129478252,59.6534095752596));
#186476=CARTESIAN_POINT('Ctrl Pts',(110.450827955009,12.4935462973671,59.6984255054258));
#186477=CARTESIAN_POINT('Ctrl Pts',(110.684462240573,12.5813844818697,59.7438396367068));
#186478=CARTESIAN_POINT('Ctrl Pts',(110.919958817175,12.6623105107267,59.7896157625019));
#186479=CARTESIAN_POINT('Ctrl Pts',(111.155664087698,12.7433082551496,59.8354324544883));
#186480=CARTESIAN_POINT('Ctrl Pts',(111.39323540817,12.8173817852037,59.8816118716509));
#186481=CARTESIAN_POINT('Ctrl Pts',(111.63250912853,12.8844674464811,59.9281222034812));
#186482=CARTESIAN_POINT('Ctrl Pts',(111.752135698328,12.9180073919844,59.9513753691388));
#186483=CARTESIAN_POINT('Ctrl Pts',(111.872188112893,12.9497999244005,59.9747113110469));
#186484=CARTESIAN_POINT('Ctrl Pts',(111.992647543251,12.9798324840516,59.9981263692054));
#186485=CARTESIAN_POINT('Ctrl Pts',(112.084399238805,13.0027077231394,60.0159611811513));
#186486=CARTESIAN_POINT('Ctrl Pts',(112.176392155673,13.0245628749281,60.0338428820048));
#186487=CARTESIAN_POINT('Ctrl Pts',(112.268589488635,13.045384961734,60.05176431752));
#186488=CARTESIAN_POINT('Ctrl Pts',(112.453592664605,13.0871665628464,60.0877254715117));
#186489=CARTESIAN_POINT('Ctrl Pts',(112.639442277684,13.1247970806182,60.1238511570314));
#186490=CARTESIAN_POINT('Ctrl Pts',(112.826148207148,13.1582277947365,60.1601432944253));
#186491=CARTESIAN_POINT('Ctrl Pts',(112.967943093299,13.1836169418084,60.1877055657722));
#186492=CARTESIAN_POINT('Ctrl Pts',(113.110232052057,13.2065831118267,60.2153638755844));
#186493=CARTESIAN_POINT('Ctrl Pts',(113.253013755355,13.2271344963784,60.2431179657105));
#186494=CARTESIAN_POINT('Ctrl Pts',(113.386871602196,13.2464014193957,60.2691374252037));
#186495=CARTESIAN_POINT('Ctrl Pts',(113.521162574455,13.2635458793658,60.2952410761696));
#186496=CARTESIAN_POINT('Ctrl Pts',(113.65588596443,13.2785663779232,60.3214287810442));
#186497=CARTESIAN_POINT('Ctrl Pts',(113.671894084392,13.2803511455337,60.3245404598793));
#186498=CARTESIAN_POINT('Ctrl Pts',(113.687917524092,13.2821069432664,60.3276551165844));
#186499=CARTESIAN_POINT('Ctrl Pts',(113.703955974844,13.2838336233231,60.3307726911571));
#186500=CARTESIAN_POINT('Ctrl Pts',(113.797462937436,13.2939004689287,60.3489486941553));
#186501=CARTESIAN_POINT('Ctrl Pts',(113.891450114483,13.3029699738907,60.3672180418533));
#186502=CARTESIAN_POINT('Ctrl Pts',(113.985307606065,13.3109824254935,60.3854621811247));
#186503=CARTESIAN_POINT('Ctrl Pts',(114.04762458284,13.3163023179392,60.3975754347829));
#186504=CARTESIAN_POINT('Ctrl Pts',(114.109884258143,13.3211573008145,60.4096775501077));
#186505=CARTESIAN_POINT('Ctrl Pts',(114.171907118068,13.3255425067845,60.4217336329563));
#186506=CARTESIAN_POINT('Ctrl Pts',(114.18402496701,13.3263992757821,60.4240891159344));
#186507=CARTESIAN_POINT('Ctrl Pts',(114.196142823531,13.32723878514,60.4264446003854));
#186508=CARTESIAN_POINT('Ctrl Pts',(114.20826199609,13.3280611378834,60.4288003406496));
#186509=CARTESIAN_POINT('Ctrl Pts',(114.445669580006,13.3441705526948,60.4749479304909));
#186510=CARTESIAN_POINT('Ctrl Pts',(114.683414492677,13.353688708566,60.5211610907271));
#186511=CARTESIAN_POINT('Ctrl Pts',(114.921378109398,13.3566581767227,60.5674167629362));
#186512=CARTESIAN_POINT('Ctrl Pts',(115.159173594614,13.3596255468228,60.6136397535285));
#186513=CARTESIAN_POINT('Ctrl Pts',(115.397187946768,13.3560534382267,60.6599052877561));
#186514=CARTESIAN_POINT('Ctrl Pts',(115.635301434022,13.3459323690487,60.7061900919911));
#186515=CARTESIAN_POINT('Ctrl Pts',(115.806511310614,13.3386550534085,60.739470086806));
#186516=CARTESIAN_POINT('Ctrl Pts',(115.977772432714,13.3279908526501,60.7727600427885));
#186517=CARTESIAN_POINT('Ctrl Pts',(116.149037779096,13.3139197681031,60.806050819892));
#186518=CARTESIAN_POINT('Ctrl Pts',(116.172635983815,13.3119809501182,60.810637869111));
#186519=CARTESIAN_POINT('Ctrl Pts',(116.196234263956,13.3099774298684,60.8152249329905));
#186520=CARTESIAN_POINT('Ctrl Pts',(116.219832491622,13.307909134588,60.8198119866698));
#186521=CARTESIAN_POINT('Ctrl Pts',(116.240170921855,13.3061265482066,60.8237653967545));
#186522=CARTESIAN_POINT('Ctrl Pts',(116.26050592698,13.3042961307879,60.8277181410621));
#186523=CARTESIAN_POINT('Ctrl Pts',(116.28082958516,13.3024186422104,60.8316686797361));
#186524=CARTESIAN_POINT('Ctrl Pts',(116.495305897586,13.282605436185,60.8733588596927));
#186525=CARTESIAN_POINT('Ctrl Pts',(116.708780448291,13.2575315963514,60.9148543159246));
#186526=CARTESIAN_POINT('Ctrl Pts',(116.921258479399,13.2272498512068,60.9561560674024));
#186527=CARTESIAN_POINT('Ctrl Pts',(116.979436757235,13.2189584538647,60.9674648354668));
#186528=CARTESIAN_POINT('Ctrl Pts',(117.037540322311,13.2102763125356,60.9787590807694));
#186529=CARTESIAN_POINT('Ctrl Pts',(117.095569257697,13.2012038297673,60.9900388194574));
#186530=CARTESIAN_POINT('Ctrl Pts',(117.137732860675,13.1946117984137,60.9982346345379));
#186531=CARTESIAN_POINT('Ctrl Pts',(117.179857063159,13.1878136833666,61.0064227908998));
#186532=CARTESIAN_POINT('Ctrl Pts',(117.221941887973,13.1808095430678,61.0146032929798));
#186533=CARTESIAN_POINT('Ctrl Pts',(117.250681779517,13.1760263882504,61.0201897898609));
#186534=CARTESIAN_POINT('Ctrl Pts',(117.279403577157,13.1711470762405,61.0257727696255));
#186535=CARTESIAN_POINT('Ctrl Pts',(117.308094681736,13.1661738703345,61.0313497832339));
#186536=CARTESIAN_POINT('Ctrl Pts',(117.448904624499,13.1417664155069,61.0587206000251));
#186537=CARTESIAN_POINT('Ctrl Pts',(117.58906394148,13.1150870864737,61.0859649473445));
#186538=CARTESIAN_POINT('Ctrl Pts',(117.728884739466,13.0860754292987,61.1131434929087));
#186539=CARTESIAN_POINT('Ctrl Pts',(117.868152999214,13.0571784192304,61.1402146353833));
#186540=CARTESIAN_POINT('Ctrl Pts',(118.007085685501,13.0259674344299,61.1672205486595));
#186541=CARTESIAN_POINT('Ctrl Pts',(118.14598009617,12.992332384803,61.1942190218719));
#186542=CARTESIAN_POINT('Ctrl Pts',(118.171469405761,12.9861598240143,61.1991736664749));
#186543=CARTESIAN_POINT('Ctrl Pts',(118.196957389447,12.9799054892575,61.2041280533467));
#186544=CARTESIAN_POINT('Ctrl Pts',(118.222445832201,12.9735685161642,61.2090825294528));
#186545=CARTESIAN_POINT('Ctrl Pts',(118.23754875077,12.9698136069482,61.212018254083));
#186546=CARTESIAN_POINT('Ctrl Pts',(118.252654100341,12.9660291080705,61.2149544512547));
#186547=CARTESIAN_POINT('Ctrl Pts',(118.267754790522,12.9622167157772,61.2178897427281));
#186548=CARTESIAN_POINT('Ctrl Pts',(118.477140301939,12.9093542505205,61.2585903662726));
#186549=CARTESIAN_POINT('Ctrl Pts',(118.684730096326,12.8513622271013,61.2989419360439));
#186550=CARTESIAN_POINT('Ctrl Pts',(118.890527441424,12.7882501539497,61.3389450872296));
#186551=CARTESIAN_POINT('Ctrl Pts',(118.954537756875,12.7686200478895,61.3513874942257));
#186552=CARTESIAN_POINT('Ctrl Pts',(119.018374602236,12.7484942377947,61.3637961818838));
#186553=CARTESIAN_POINT('Ctrl Pts',(119.082037874589,12.7278720011977,61.3761711301986));
#186554=CARTESIAN_POINT('Ctrl Pts',(119.128757185184,12.7127383669824,61.385252489553));
#186555=CARTESIAN_POINT('Ctrl Pts',(119.175383018273,12.6973373792244,61.3943156786303));
#186556=CARTESIAN_POINT('Ctrl Pts',(119.221915290494,12.6816685898537,61.4033606812262));
#186557=CARTESIAN_POINT('Ctrl Pts',(119.250628234944,12.6720000940479,61.4089419400966));
#186558=CARTESIAN_POINT('Ctrl Pts',(119.279305788299,12.6622295793524,61.4145163196007));
#186559=CARTESIAN_POINT('Ctrl Pts',(119.307959019654,12.6523529953859,61.4200859713631));
#186560=CARTESIAN_POINT('Ctrl Pts',(119.422699883056,12.6128025601217,61.442389447162));
#186561=CARTESIAN_POINT('Ctrl Pts',(119.536995525351,12.5715684555563,61.4646063803124));
#186562=CARTESIAN_POINT('Ctrl Pts',(119.650676763164,12.5286947613551,61.4867038847336));
#186563=CARTESIAN_POINT('Ctrl Pts',(119.750603748029,12.4910083403235,61.5061278198734));
#186564=CARTESIAN_POINT('Ctrl Pts',(119.850056043861,12.452055293347,61.5254594843514));
#186565=CARTESIAN_POINT('Ctrl Pts',(119.94892798088,12.4118901617296,61.5446783379412));
#186566=CARTESIAN_POINT('Ctrl Pts',(120.037512300966,12.3759042087613,61.561897471392));
#186567=CARTESIAN_POINT('Ctrl Pts',(120.125630778712,12.3389454038338,61.5790260538131));
#186568=CARTESIAN_POINT('Ctrl Pts',(120.213209775707,12.3010583961822,61.5960497712754));
#186569=CARTESIAN_POINT('Ctrl Pts',(120.237949446469,12.2903559203873,61.6008587001239));
#186570=CARTESIAN_POINT('Ctrl Pts',(120.262654935792,12.2795755831455,61.6056609847406));
#186571=CARTESIAN_POINT('Ctrl Pts',(120.287326902652,12.2687172406279,61.610456753218));
#186572=CARTESIAN_POINT('Ctrl Pts',(120.486416639678,12.1810961535618,61.6491560709665));
#186573=CARTESIAN_POINT('Ctrl Pts',(120.683311997193,12.0884052960903,61.6874288424188));
#186574=CARTESIAN_POINT('Ctrl Pts',(120.878023145789,11.9906823843153,61.7252770445476));
#186575=CARTESIAN_POINT('Ctrl Pts',(121.072799870817,11.89292656061,61.7631379935069));
#186576=CARTESIAN_POINT('Ctrl Pts',(121.265391273193,11.7901350574577,61.800574156654));
#186577=CARTESIAN_POINT('Ctrl Pts',(121.455782450768,11.6823003088381,61.8375826372896));
#186578=CARTESIAN_POINT('Ctrl Pts',(121.620325552598,11.5891055282344,61.8695667358985));
#186579=CARTESIAN_POINT('Ctrl Pts',(121.783225041274,11.4921431217687,61.9012313468801));
#186580=CARTESIAN_POINT('Ctrl Pts',(121.944453055693,11.3913829322761,61.9325710545575));
#186581=CARTESIAN_POINT('Ctrl Pts',(106.597794809764,10.1748376799211,58.949467993991));
#186582=CARTESIAN_POINT('Ctrl Pts',(106.619133959162,10.1929126322122,58.9534397950288));
#186583=CARTESIAN_POINT('Ctrl Pts',(106.640528384642,10.2109188565186,58.9574223407024));
#186584=CARTESIAN_POINT('Ctrl Pts',(106.661977627748,10.2288560234639,58.961415541896));
#186585=CARTESIAN_POINT('Origin',(121.630276337646,13.,49.6468984217139));
#186586=CARTESIAN_POINT('',(115.139466160418,13.,48.3852064367498));
#186587=CARTESIAN_POINT('Ctrl Pts',(113.04734486836,13.,48.4878956643013));
#186588=CARTESIAN_POINT('Ctrl Pts',(114.126636691851,13.,48.364665625098));
#186589=CARTESIAN_POINT('Ctrl Pts',(115.139466160442,13.,48.3852064363081));
#186590=CARTESIAN_POINT('',(121.057846598951,13.,52.591779437011));
#186591=CARTESIAN_POINT('',(119.633560001989,13.,49.2587741462908));
#186592=CARTESIAN_POINT('Ctrl Pts',(119.633560002146,13.,49.2587741458773));
#186593=CARTESIAN_POINT('Ctrl Pts',(120.58033318249,13.,49.6191434041911));
#186594=CARTESIAN_POINT('Ctrl Pts',(121.534871380993,13.,50.1377119246391));
#186595=CARTESIAN_POINT('',(119.633560001989,13.,49.2587741462908));
#186596=CARTESIAN_POINT('Origin',(117.338810602979,1.45439216225896E-14,
49.0673970427951));
#186597=CARTESIAN_POINT('',(115.139466160418,-13.,48.3852064367498));
#186598=CARTESIAN_POINT('Ctrl Pts',(115.139466160442,-13.,48.3852064363082));
#186599=CARTESIAN_POINT('Ctrl Pts',(114.126636691851,-13.,48.364665625098));
#186600=CARTESIAN_POINT('Ctrl Pts',(113.04734486836,-13.,48.4878956643013));
#186601=CARTESIAN_POINT('Origin',(117.386513081203,1.45439216225896E-14,
48.8219902915203));
#186602=CARTESIAN_POINT('Origin',(117.338810602979,1.45439216225896E-14,
49.0673970427951));
#186603=CARTESIAN_POINT('',(119.633560001989,-13.,49.2587741462908));
#186604=CARTESIAN_POINT('Ctrl Pts',(121.534871380993,-13.,50.1377119246392));
#186605=CARTESIAN_POINT('Ctrl Pts',(120.58033318249,-13.,49.6191434041912));
#186606=CARTESIAN_POINT('Ctrl Pts',(119.633560002146,-13.,49.2587741458774));
#186607=CARTESIAN_POINT('Origin',(117.386513081203,1.45439216225896E-14,
48.8219902915203));
#186608=CARTESIAN_POINT('Origin',(113.14274982476,-13.,47.9970821613267));
#186609=CARTESIAN_POINT('',(112.570320086065,-13.,50.9419631766238));
#186610=CARTESIAN_POINT('',(115.139466160418,-13.,48.3852064367498));
#186611=CARTESIAN_POINT('Origin',(116.814083342508,1.45439216225896E-14,
51.7668713068174));
#186612=CARTESIAN_POINT('Origin',(116.814083342508,1.45439216225896E-14,
51.7668713068174));
#186613=CARTESIAN_POINT('Origin',(115.383008995769,1.45439216225896E-14,
59.12907384506));
#186614=CARTESIAN_POINT('Origin',(115.096794126421,1.45439216225896E-14,
60.6015143527085));
#186615=CARTESIAN_POINT('',(122.039447043815,11.3329480580267,61.950331991012));
#186616=CARTESIAN_POINT('Ctrl Pts',(121.944453055789,11.3913829318325,61.9325710578547));
#186617=CARTESIAN_POINT('Ctrl Pts',(121.975991009671,11.3717006163854,61.9384667390898));
#186618=CARTESIAN_POINT('Ctrl Pts',(122.007448447719,11.3518837406497,61.9443467695542));
#186619=CARTESIAN_POINT('Ctrl Pts',(122.038824288318,11.3319330864622,61.9502109390019));
#186620=CARTESIAN_POINT('Ctrl Pts',(122.039928552843,11.333968991207,61.9511297038209));
#186621=CARTESIAN_POINT('Ctrl Pts',(123.16620920987,10.6501122569522,62.1700575786149));
#186622=CARTESIAN_POINT('Ctrl Pts',(124.187604468863,9.79818933144462,62.3685976955743));
#186623=CARTESIAN_POINT('Ctrl Pts',(125.955460550856,7.80211216460018,62.7122358221437));
#186624=CARTESIAN_POINT('Ctrl Pts',(126.689541950163,6.67413921942583,62.85492750354));
#186625=CARTESIAN_POINT('Ctrl Pts',(127.936628835462,3.93791384118314,63.0973378475144));
#186626=CARTESIAN_POINT('Ctrl Pts',(128.393441930735,2.20871226321621,63.1861337613069));
#186627=CARTESIAN_POINT('Ctrl Pts',(128.552284670311,-1.46551021789508,
63.2170098162093));
#186628=CARTESIAN_POINT('Ctrl Pts',(128.281605122352,-3.25174142720192,
63.164394779438));
#186629=CARTESIAN_POINT('Ctrl Pts',(127.241550546623,-6.18489950503424,
62.9622276406228));
#186630=CARTESIAN_POINT('Ctrl Pts',(126.617322374644,-7.36740292814777,
62.8408893700727));
#186631=CARTESIAN_POINT('Ctrl Pts',(125.059576412758,-9.51520023323271,
62.5380927174118));
#186632=CARTESIAN_POINT('Ctrl Pts',(124.124637298172,-10.4720112212054,
62.3563580563915));
#186633=CARTESIAN_POINT('Ctrl Pts',(123.077241409441,-11.2743970687384,
62.1527639037644));
#186634=CARTESIAN_POINT('Origin',(115.096794126421,1.45439216225896E-14,
60.6015143527085));
#186635=CARTESIAN_POINT('Ctrl Pts',(119.407391898135,-13.0301062068,64.4806209347011));
#186636=CARTESIAN_POINT('Ctrl Pts',(118.147720209373,-13.52088854622,64.2197588532859));
#186637=CARTESIAN_POINT('Ctrl Pts',(115.484843558882,-14.11864469328,63.6701345092559));
#186638=CARTESIAN_POINT('Ctrl Pts',(111.407779104958,-13.78606076252,62.8296130437921));
#186639=CARTESIAN_POINT('Ctrl Pts',(107.603918121139,-12.25314221515,62.042197218315));
#186640=CARTESIAN_POINT('Ctrl Pts',(104.405185821524,-9.65337632876199,
61.3724070805235));
#186641=CARTESIAN_POINT('Ctrl Pts',(102.090884786275,-6.21311314882798,
60.8745338232188));
#186642=CARTESIAN_POINT('Ctrl Pts',(100.863295028327,-2.23188950467599,
60.587896894062));
#186643=CARTESIAN_POINT('Ctrl Pts',(100.830083860925,1.94365945142001,60.5334248031237));
#186644=CARTESIAN_POINT('Ctrl Pts',(101.994925696463,5.94997864935902,60.7118317873852));
#186645=CARTESIAN_POINT('Ctrl Pts',(104.257183696659,9.43824757472701,61.1035559294922));
#186646=CARTESIAN_POINT('Ctrl Pts',(107.420671557756,12.10475106522,61.6704622847683));
#186647=CARTESIAN_POINT('Ctrl Pts',(111.210735091372,13.71732310055,62.3591632207526));
#186648=CARTESIAN_POINT('Ctrl Pts',(115.298165671407,14.13556092567,63.1056667435966));
#186649=CARTESIAN_POINT('Ctrl Pts',(119.327863642558,13.32304958287,63.8409481280871));
#186650=CARTESIAN_POINT('Ctrl Pts',(122.949755987961,11.35053247341,64.4969597333906));
#186651=CARTESIAN_POINT('Ctrl Pts',(125.849276342301,8.38975190055401,65.0125557470494));
#186652=CARTESIAN_POINT('Ctrl Pts',(127.774753525765,4.69849588175201,65.338816003207));
#186653=CARTESIAN_POINT('Ctrl Pts',(128.559323946183,0.598153168230215,
65.4433053433738));
#186654=CARTESIAN_POINT('Ctrl Pts',(128.135460009217,-3.55426929776699,
65.3128976673845));
#186655=CARTESIAN_POINT('Ctrl Pts',(126.540849582971,-7.39723011566199,
64.9549187912497));
#186656=CARTESIAN_POINT('Ctrl Pts',(123.915114606311,-10.59613196357,64.396508606043));
#186657=CARTESIAN_POINT('Ctrl Pts',(120.48765454368,-12.87245417943,63.6822580730997));
#186658=CARTESIAN_POINT('Ctrl Pts',(116.557673127465,-14.02800288271,62.8703267966466));
#186659=CARTESIAN_POINT('Ctrl Pts',(112.468127411276,-13.96216723722,62.0273792074582));
#186660=CARTESIAN_POINT('Ctrl Pts',(108.575867327145,-12.68067939367,61.2227802517869));
#186661=CARTESIAN_POINT('Ctrl Pts',(105.220565623354,-10.29511540522,60.5225559529361));
#186662=CARTESIAN_POINT('Ctrl Pts',(102.695143378168,-7.01318056982799,
59.9836446847886));
#186663=CARTESIAN_POINT('Ctrl Pts',(101.22026606865,-3.12062503134899,59.6489396850396));
#186664=CARTESIAN_POINT('Ctrl Pts',(100.925130760206,1.04363579573001,59.5435544445256));
#186665=CARTESIAN_POINT('Ctrl Pts',(101.836217230004,5.11702977330802,59.6726361362038));
#186666=CARTESIAN_POINT('Ctrl Pts',(103.874982436677,8.74489632052901,60.0209174632251));
#186667=CARTESIAN_POINT('Ctrl Pts',(106.864699073354,11.61136585444,60.5540459456192));
#186668=CARTESIAN_POINT('Ctrl Pts',(110.545842787632,13.46686179209,61.2215749077958));
#186669=CARTESIAN_POINT('Ctrl Pts',(114.598688340515,14.14983058118,61.9613557488326));
#186670=CARTESIAN_POINT('Ctrl Pts',(118.671147311171,13.60080777785,62.7049490710946));
#186671=CARTESIAN_POINT('Ctrl Pts',(122.409423585822,11.86759547232,63.3835835334376));
#186672=CARTESIAN_POINT('Ctrl Pts',(125.488817531349,9.10110027621301,63.9341436058365));
#186673=CARTESIAN_POINT('Ctrl Pts',(127.641996808559,5.54219424821201,64.3046648862414));
#186674=CARTESIAN_POINT('Ctrl Pts',(128.682272353622,1.50074274532801,64.4588585156218));
#186675=CARTESIAN_POINT('Ctrl Pts',(128.519852944246,-2.67137480574699,
64.3792707613319));
#186676=CARTESIAN_POINT('Ctrl Pts',(127.16966310462,-6.61090220091999,64.0688026714746));
#186677=CARTESIAN_POINT('Ctrl Pts',(124.750043663147,-9.97483429952299,
63.5504574876502));
#186678=CARTESIAN_POINT('Ctrl Pts',(121.472448102156,-12.47028165393,62.8653378082347));
#186679=CARTESIAN_POINT('Ctrl Pts',(117.623031813639,-13.87997168676,62.0690668843584));
#186680=CARTESIAN_POINT('Ctrl Pts',(113.537737240012,-14.0811660897,61.226945637699));
#186681=CARTESIAN_POINT('Ctrl Pts',(109.573044176586,-13.05634735175,60.4082670668599));
#186682=CARTESIAN_POINT('Ctrl Pts',(106.074931936307,-10.89474396662,59.6802830732504));
#186683=CARTESIAN_POINT('Ctrl Pts',(103.348755766122,-7.78456152314698,
59.1023490003672));
#186684=CARTESIAN_POINT('Ctrl Pts',(101.632660302733,-3.99659609901699,
58.720755707315));
#186685=CARTESIAN_POINT('Ctrl Pts',(101.076844893947,0.139343300067115,
58.5646991354477));
#186686=CARTESIAN_POINT('Ctrl Pts',(101.730486103999,4.26315041437501,58.6437382882256));
#186687=CARTESIAN_POINT('Ctrl Pts',(103.537456028837,8.01577531292601,58.946962951863));
#186688=CARTESIAN_POINT('Ctrl Pts',(106.34120921727,11.07048600428,59.4439436213124));
#186689=CARTESIAN_POINT('Ctrl Pts',(109.898412705345,13.16131620227,60.0873809237817));
#186690=CARTESIAN_POINT('Ctrl Pts',(113.900132430754,14.10622236873,60.8172238610665));
#186691=CARTESIAN_POINT('Ctrl Pts',(117.998731373649,13.82293380427,61.5658983045794));
#186692=CARTESIAN_POINT('Ctrl Pts',(121.838137481187,12.33611576178,62.2641905131989));
#186693=CARTESIAN_POINT('Ctrl Pts',(125.084845970359,9.77522189391502,62.847273400612));
#186694=CARTESIAN_POINT('Ctrl Pts',(127.456956901142,6.36322306770402,63.2603508958846));
#186695=CARTESIAN_POINT('Ctrl Pts',(128.748719088097,2.39719371119201,63.4634288204047));
#186696=CARTESIAN_POINT('Ctrl Pts',(128.848445985611,-1.77755329875599,
63.4347974005724));
#186697=CARTESIAN_POINT('Ctrl Pts',(127.748233896623,-5.79753384146799,
63.172920305643));
#186698=CARTESIAN_POINT('Ctrl Pts',(125.544672779088,-9.31273409308899,
62.6965728151966));
#186699=CARTESIAN_POINT('Ctrl Pts',(122.430351858199,-12.01710831635,62.0431906691766));
#186700=CARTESIAN_POINT('Ctrl Pts',(119.928388506017,-13.12246273504,61.524844857904));
#186701=CARTESIAN_POINT('Ctrl Pts',(118.625437907371,-13.47672248693,61.2555701666254));
#186702=CARTESIAN_POINT('Ctrl Pts',(119.35682826831,-12.83307257039,64.3467570107765));
#186703=CARTESIAN_POINT('Ctrl Pts',(118.11624992964,-13.31643358665,64.0896063191756));
#186704=CARTESIAN_POINT('Ctrl Pts',(115.493730405444,-13.90515081526,63.5478266449777));
#186705=CARTESIAN_POINT('Ctrl Pts',(111.47845293012,-13.57759602396,62.7193154114488));
#186706=CARTESIAN_POINT('Ctrl Pts',(107.732247701997,-12.06785737328,61.9431067855144));
#186707=CARTESIAN_POINT('Ctrl Pts',(104.582020756437,-9.50740362435499,
61.2827451804895));
#186708=CARTESIAN_POINT('Ctrl Pts',(102.302851223542,-6.11916208981799,
60.7917008295511));
#186709=CARTESIAN_POINT('Ctrl Pts',(101.093960356319,-2.19814017844699,
60.5086986147019));
#186710=CARTESIAN_POINT('Ctrl Pts',(101.061387385959,1.91426857128501,60.4543505773211));
#186711=CARTESIAN_POINT('Ctrl Pts',(102.208751162539,5.86000655617201,60.6293601541255));
#186712=CARTESIAN_POINT('Ctrl Pts',(104.436936619098,9.29552792137202,61.0144612316163));
#186713=CARTESIAN_POINT('Ctrl Pts',(107.552724066323,11.92171010742,61.5720955194281));
#186714=CARTESIAN_POINT('Ctrl Pts',(111.285612475627,13.50989777266,62.2496826816131));
#186715=CARTESIAN_POINT('Ctrl Pts',(115.311371320996,13.92181125028,62.9841983737852));
#186716=CARTESIAN_POINT('Ctrl Pts',(119.280270556188,13.12158622825,63.7076616221994));
#186717=CARTESIAN_POINT('Ctrl Pts',(122.847530763518,11.17889636753,64.3530537626213));
#186718=CARTESIAN_POINT('Ctrl Pts',(125.703342266057,8.26288698484901,64.8601535937572));
#186719=CARTESIAN_POINT('Ctrl Pts',(127.599839508207,4.62744797818601,65.1807806918523));
#186720=CARTESIAN_POINT('Ctrl Pts',(128.372682111344,0.589108246264615,
65.2829903638944));
#186721=CARTESIAN_POINT('Ctrl Pts',(127.955363593847,-3.50052371860999,
65.1538549949141));
#186722=CARTESIAN_POINT('Ctrl Pts',(126.385001929965,-7.28537353322399,
64.8005896242253));
#186723=CARTESIAN_POINT('Ctrl Pts',(123.799107777366,-10.43590346047,64.2499237493622));
#186724=CARTESIAN_POINT('Ctrl Pts',(120.423611756099,-12.67780446466,63.5457740532488));
#186725=CARTESIAN_POINT('Ctrl Pts',(116.553193214911,-13.81587963708,62.7454206846333));
#186726=CARTESIAN_POINT('Ctrl Pts',(112.525623211661,-13.75103951966,61.9145200138023));
#186727=CARTESIAN_POINT('Ctrl Pts',(108.692355602661,-12.48892958492,61.121388090907));
#186728=CARTESIAN_POINT('Ctrl Pts',(105.387926803782,-10.13943869826,60.4310525323871));
#186729=CARTESIAN_POINT('Ctrl Pts',(102.900828512264,-6.90713135975199,
59.8995907233755));
#186730=CARTESIAN_POINT('Ctrl Pts',(101.448389431029,-3.07343676687899,
59.569247295142));
#186731=CARTESIAN_POINT('Ctrl Pts',(101.157852983112,1.02785454631301,59.46475598703));
#186732=CARTESIAN_POINT('Ctrl Pts',(102.055298534003,5.03965304529702,59.5911861394423));
#186733=CARTESIAN_POINT('Ctrl Pts',(104.063370724214,8.61266111885201,59.9335013186626));
#186734=CARTESIAN_POINT('Ctrl Pts',(107.008014613714,11.4357855789,60.4578685028059));
#186735=CARTESIAN_POINT('Ctrl Pts',(110.633630225412,13.26322379345,61.1146038413743));
#186736=CARTESIAN_POINT('Ctrl Pts',(114.625327018159,13.93586512842,61.8424985081874));
#186737=CARTESIAN_POINT('Ctrl Pts',(118.636340646059,13.39514432645,62.5741480061266));
#186738=CARTESIAN_POINT('Ctrl Pts',(122.318224893007,11.68814064254,63.2418209139908));
#186739=CARTESIAN_POINT('Ctrl Pts',(125.351190043614,8.96347876689701,63.783356097844));
#186740=CARTESIAN_POINT('Ctrl Pts',(127.471946201774,5.45838843197201,64.1475749308939));
#186741=CARTESIAN_POINT('Ctrl Pts',(128.496627306379,1.47804939228401,64.2987372929904));
#186742=CARTESIAN_POINT('Ctrl Pts',(128.336799905422,-2.63097984012399,
64.2196533766126));
#186743=CARTESIAN_POINT('Ctrl Pts',(127.007162843178,-6.51093600877899,
63.9131803619128));
#186744=CARTESIAN_POINT('Ctrl Pts',(124.624267467324,-9.82400069590499,
63.4019736489391));
#186745=CARTESIAN_POINT('Ctrl Pts',(121.396369784457,-12.2817133566,62.7265143066441));
#186746=CARTESIAN_POINT('Ctrl Pts',(117.60529811228,-13.67008688219,61.9415844839235));
#186747=CARTESIAN_POINT('Ctrl Pts',(113.581914968302,-13.86823894118,61.1114976601534));
#186748=CARTESIAN_POINT('Ctrl Pts',(109.677309669108,-12.85891691211,60.3044990257867));
#186749=CARTESIAN_POINT('Ctrl Pts',(106.23222983105,-10.73000002767,59.5868235383575));
#186750=CARTESIAN_POINT('Ctrl Pts',(103.547413297838,-7.66684794197098,
59.0169290046143));
#186751=CARTESIAN_POINT('Ctrl Pts',(101.857403622416,-3.93616191297999,
58.6404063003945));
#186752=CARTESIAN_POINT('Ctrl Pts',(101.310128925989,0.137236232267715,
58.4860098831306));
#186753=CARTESIAN_POINT('Ctrl Pts',(101.954022153609,4.19868555004701,58.5631542106142));
#186754=CARTESIAN_POINT('Ctrl Pts',(103.733804134502,7.89456545219501,58.8610940469303));
#186755=CARTESIAN_POINT('Ctrl Pts',(106.495296606141,10.90308459713,59.3498600241915));
#186756=CARTESIAN_POINT('Ctrl Pts',(109.998846143165,12.96229848513,59.982868003024));
#186757=CARTESIAN_POINT('Ctrl Pts',(113.940190203264,13.89291633382,60.7009750412564));
#186758=CARTESIAN_POINT('Ctrl Pts',(117.97694853005,13.61391149316,61.4376288266965));
#186759=CARTESIAN_POINT('Ctrl Pts',(121.758433383767,12.14957624252,62.1246622279085));
#186760=CARTESIAN_POINT('Ctrl Pts',(124.956183045448,9.62740671222201,62.6982284358081));
#186761=CARTESIAN_POINT('Ctrl Pts',(127.292560300925,6.26700213440002,63.104359973566));
#186762=CARTESIAN_POINT('Ctrl Pts',(128.564925213674,2.36094475154901,63.3036674311141));
#186763=CARTESIAN_POINT('Ctrl Pts',(128.66328009665,-1.75067417859599,63.2747693173408));
#186764=CARTESIAN_POINT('Ctrl Pts',(127.579840767871,-5.70986692940099,
63.0161525329957));
#186765=CARTESIAN_POINT('Ctrl Pts',(125.409736608484,-9.17191238110799,
62.5463084488705));
#186766=CARTESIAN_POINT('Ctrl Pts',(122.342644622221,-11.83539264088,61.9021067235759));
#186767=CARTESIAN_POINT('Ctrl Pts',(119.87860515966,-12.92403253729,61.3911326064781));
#186768=CARTESIAN_POINT('Ctrl Pts',(118.595402349439,-13.27293538064,61.125696515574));
#186769=CARTESIAN_POINT('Ctrl Pts',(119.306264638481,-12.63603893397,64.2128930868616));
#186770=CARTESIAN_POINT('Ctrl Pts',(118.084779649904,-13.11197862707,63.959453785075));
#186771=CARTESIAN_POINT('Ctrl Pts',(115.502617252005,-13.69165693723,63.4255187807093));
#186772=CARTESIAN_POINT('Ctrl Pts',(111.549126755281,-13.3691312854,62.6090177791154));
#186773=CARTESIAN_POINT('Ctrl Pts',(107.860577282853,-11.8825725314,61.8440163527233));
#186774=CARTESIAN_POINT('Ctrl Pts',(104.758855691358,-9.36143091994799,
61.1930832804673));
#186775=CARTESIAN_POINT('Ctrl Pts',(102.514817660809,-6.02521103080599,
60.7088678358931));
#186776=CARTESIAN_POINT('Ctrl Pts',(101.324625684322,-2.16439085221699,
60.4295003353339));
#186777=CARTESIAN_POINT('Ctrl Pts',(101.292690910985,1.88487769115301,60.3752763515067));
#186778=CARTESIAN_POINT('Ctrl Pts',(102.422576628608,5.77003446298902,60.546888520854));
#186779=CARTESIAN_POINT('Ctrl Pts',(104.616689541549,9.15280826802001,60.9253665337324));
#186780=CARTESIAN_POINT('Ctrl Pts',(107.684776574895,11.73866914963,61.4737287540785));
#186781=CARTESIAN_POINT('Ctrl Pts',(111.36048985989,13.30247244478,62.1402021424649));
#186782=CARTESIAN_POINT('Ctrl Pts',(115.324576970593,13.7080615749,62.8627300039652));
#186783=CARTESIAN_POINT('Ctrl Pts',(119.232677469826,12.92012287364,63.574375116313));
#186784=CARTESIAN_POINT('Ctrl Pts',(122.745305539082,11.00726026166,64.2091477918536));
#186785=CARTESIAN_POINT('Ctrl Pts',(125.557408189824,8.13602206913601,64.7077514404668));
#186786=CARTESIAN_POINT('Ctrl Pts',(127.424925490658,4.55640007460902,65.0227453804995));
#186787=CARTESIAN_POINT('Ctrl Pts',(128.186040276495,0.580063324285615,
65.1226753844131));
#186788=CARTESIAN_POINT('Ctrl Pts',(127.775267178477,-3.44677813946799,
64.9948123224437));
#186789=CARTESIAN_POINT('Ctrl Pts',(126.229154276958,-7.17351695080098,
64.6462604572009));
#186790=CARTESIAN_POINT('Ctrl Pts',(123.683100948408,-10.27567495739,64.1033388926787));
#186791=CARTESIAN_POINT('Ctrl Pts',(120.359568968502,-12.4831547499,63.4092900333947));
#186792=CARTESIAN_POINT('Ctrl Pts',(116.548713302336,-13.60375639144,62.620514572626));
#186793=CARTESIAN_POINT('Ctrl Pts',(112.583119012022,-13.5399118021,61.8016608201517));
#186794=CARTESIAN_POINT('Ctrl Pts',(108.808843878152,-12.29717977616,61.0199959300326));
#186795=CARTESIAN_POINT('Ctrl Pts',(105.555287984189,-9.98376199129099,
60.3395491118441));
#186796=CARTESIAN_POINT('Ctrl Pts',(103.106513646349,-6.80108214965099,
59.8155367619703));
#186797=CARTESIAN_POINT('Ctrl Pts',(101.676512793396,-3.02624850238099,
59.4895549052523));
#186798=CARTESIAN_POINT('Ctrl Pts',(101.39057520603,1.01207329692701,59.3859575295266));
#186799=CARTESIAN_POINT('Ctrl Pts',(102.274379838014,4.96227631731602,59.5097361426729));
#186800=CARTESIAN_POINT('Ctrl Pts',(104.251759011771,8.48042591720101,59.8460851740942));
#186801=CARTESIAN_POINT('Ctrl Pts',(107.151330154106,11.26020530339,60.3616910599886));
#186802=CARTESIAN_POINT('Ctrl Pts',(110.721417663228,13.05958579483,61.0076327749495));
#186803=CARTESIAN_POINT('Ctrl Pts',(114.651965695841,13.72189967566,61.7236412675494));
#186804=CARTESIAN_POINT('Ctrl Pts',(118.601533980985,13.18948087504,62.443346941166));
#186805=CARTESIAN_POINT('Ctrl Pts',(122.227026200225,11.50868581274,63.1000582945505));
#186806=CARTESIAN_POINT('Ctrl Pts',(125.2135625559,8.82585725755001,63.6325685898554));
#186807=CARTESIAN_POINT('Ctrl Pts',(127.301895595,5.37458261569201,63.9904849755484));
#186808=CARTESIAN_POINT('Ctrl Pts',(128.310982259146,1.45535603919601,64.1386160703609));
#186809=CARTESIAN_POINT('Ctrl Pts',(128.153746866589,-2.59058487454599,
64.0600359918914));
#186810=CARTESIAN_POINT('Ctrl Pts',(126.844662581706,-6.41096981667798,
63.7575580523452));
#186811=CARTESIAN_POINT('Ctrl Pts',(124.498491271469,-9.67316709231899,
63.2534898102216));
#186812=CARTESIAN_POINT('Ctrl Pts',(121.320291466714,-12.0931450593,62.5876908050552));
#186813=CARTESIAN_POINT('Ctrl Pts',(117.587564410871,-13.46020207762,61.8141020834892));
#186814=CARTESIAN_POINT('Ctrl Pts',(113.626092696544,-13.65531179265,60.9960496826084));
#186815=CARTESIAN_POINT('Ctrl Pts',(109.781575161582,-12.66148647246,60.2007309847145));
#186816=CARTESIAN_POINT('Ctrl Pts',(106.389527725756,-10.56525608868,59.4933640034673));
#186817=CARTESIAN_POINT('Ctrl Pts',(103.746070829524,-7.54913436075398,
58.9315090088654));
#186818=CARTESIAN_POINT('Ctrl Pts',(102.082146942077,-3.87572772689699,
58.56005689348));
#186819=CARTESIAN_POINT('Ctrl Pts',(101.543412958033,0.135129164517415,
58.4073206308037));
#186820=CARTESIAN_POINT('Ctrl Pts',(102.17755820323,4.13422068576602,58.482570132995));
#186821=CARTESIAN_POINT('Ctrl Pts',(103.930152240199,7.77335559150302,58.7752251419934));
#186822=CARTESIAN_POINT('Ctrl Pts',(106.649383995051,10.73568319001,59.255776427068));
#186823=CARTESIAN_POINT('Ctrl Pts',(110.099279581029,12.76328076801,59.8783550822648));
#186824=CARTESIAN_POINT('Ctrl Pts',(113.98024797582,13.67961029892,60.584726221445));
#186825=CARTESIAN_POINT('Ctrl Pts',(117.955165686495,13.40488918204,61.309359348822));
#186826=CARTESIAN_POINT('Ctrl Pts',(121.678729286384,11.96303672324,61.9851339426251));
#186827=CARTESIAN_POINT('Ctrl Pts',(124.827520120575,9.47959153049801,62.5491834710116));
#186828=CARTESIAN_POINT('Ctrl Pts',(127.128163700718,6.17078120106001,62.9483690512494));
#186829=CARTESIAN_POINT('Ctrl Pts',(128.381131339262,2.32469579186801,63.1439060418254));
#186830=CARTESIAN_POINT('Ctrl Pts',(128.478114207689,-1.72379505847099,
63.1147412341091));
#186831=CARTESIAN_POINT('Ctrl Pts',(127.4114476391,-5.62220001736299,62.8593847603446));
#186832=CARTESIAN_POINT('Ctrl Pts',(125.27480043787,-9.03109066914899,62.3960440825424));
#186833=CARTESIAN_POINT('Ctrl Pts',(122.254937386221,-11.65367696543,61.7610227779709));
#186834=CARTESIAN_POINT('Ctrl Pts',(119.828821813277,-12.72560233954,61.2574203550473));
#186835=CARTESIAN_POINT('Ctrl Pts',(118.565366791485,-13.06914827436,60.9958228645183));
#186836=CARTESIAN_POINT('Ctrl Pts',(119.255701008655,-12.43900529756,64.079029162937));
#186837=CARTESIAN_POINT('Ctrl Pts',(118.053309370171,-12.90752366749,63.8293012509647));
#186838=CARTESIAN_POINT('Ctrl Pts',(115.511504098567,-13.47816305921,63.3032109164311));
#186839=CARTESIAN_POINT('Ctrl Pts',(111.619800580443,-13.16066654684,62.4987201467721));
#186840=CARTESIAN_POINT('Ctrl Pts',(107.988906863712,-11.69728768953,61.7449259199226));
#186841=CARTESIAN_POINT('Ctrl Pts',(104.935690626277,-9.21545821554099,
61.1034213804345));
#186842=CARTESIAN_POINT('Ctrl Pts',(102.726784098077,-5.93125997179498,
60.6260348422253));
#186843=CARTESIAN_POINT('Ctrl Pts',(101.555291012315,-2.13064152598699,
60.350302055964));
#186844=CARTESIAN_POINT('Ctrl Pts',(101.523994436021,1.85548681101801,60.2962021256943));
#186845=CARTESIAN_POINT('Ctrl Pts',(102.636402094677,5.68006236980302,60.4644168875825));
#186846=CARTESIAN_POINT('Ctrl Pts',(104.796442463989,9.01008861466501,60.8362718358466));
#186847=CARTESIAN_POINT('Ctrl Pts',(107.816829083463,11.55562819184,61.3753619887283));
#186848=CARTESIAN_POINT('Ctrl Pts',(111.435367244147,13.09504711689,62.0307216033153));
#186849=CARTESIAN_POINT('Ctrl Pts',(115.337782620183,13.49431189952,62.741261634144));
#186850=CARTESIAN_POINT('Ctrl Pts',(119.185084383457,12.71865951902,63.4410886104253));
#186851=CARTESIAN_POINT('Ctrl Pts',(122.643080314639,10.83562415578,64.0652418210844));
#186852=CARTESIAN_POINT('Ctrl Pts',(125.41147411357,8.00915715343101,64.5553492871726));
#186853=CARTESIAN_POINT('Ctrl Pts',(127.250011473088,4.48535217104401,64.8647100691527));
#186854=CARTESIAN_POINT('Ctrl Pts',(127.999398441644,0.571018402320115,
64.9623604049417));
#186855=CARTESIAN_POINT('Ctrl Pts',(127.595170763105,-3.39303256031199,
64.8357696499831));
#186856=CARTESIAN_POINT('Ctrl Pts',(126.07330662396,-7.06166036836299,64.4919312901882));
#186857=CARTESIAN_POINT('Ctrl Pts',(123.567094119461,-10.11544645429,63.9567540360075));
#186858=CARTESIAN_POINT('Ctrl Pts',(120.295526180919,-12.28850503513,63.2728060135536));
#186859=CARTESIAN_POINT('Ctrl Pts',(116.544233389782,-13.3916331458,62.4956084606127));
#186860=CARTESIAN_POINT('Ctrl Pts',(112.640614812408,-13.32878408455,61.6888016264958));
#186861=CARTESIAN_POINT('Ctrl Pts',(108.925332153668,-12.10542996742,60.9186037691525));
#186862=CARTESIAN_POINT('Ctrl Pts',(105.722649164617,-9.82808528433599,
60.2480456912948));
#186863=CARTESIAN_POINT('Ctrl Pts',(103.312198780435,-6.69503293957399,
59.7314828005553));
#186864=CARTESIAN_POINT('Ctrl Pts',(101.904636155775,-2.97906023791099,
59.4098625153547));
#186865=CARTESIAN_POINT('Ctrl Pts',(101.623297428938,0.996292047509815,
59.3071590720213));
#186866=CARTESIAN_POINT('Ctrl Pts',(102.493461142014,4.88489958930502,59.4282861459017));
#186867=CARTESIAN_POINT('Ctrl Pts',(104.4401472993,8.34819071552401,59.7586690295201));
#186868=CARTESIAN_POINT('Ctrl Pts',(107.294645694468,11.08462502785,60.2655136171655));
#186869=CARTESIAN_POINT('Ctrl Pts',(110.80920510101,12.85594779619,60.9006617085182));
#186870=CARTESIAN_POINT('Ctrl Pts',(114.678604373486,13.5079342229,61.6047840269042));
#186871=CARTESIAN_POINT('Ctrl Pts',(118.566727315873,12.98381742364,62.312545876198));
#186872=CARTESIAN_POINT('Ctrl Pts',(122.13582750741,11.32923098296,62.9582956751037));
#186873=CARTESIAN_POINT('Ctrl Pts',(125.075935068154,8.68823574823501,63.4817810818708));
#186874=CARTESIAN_POINT('Ctrl Pts',(127.131844988214,5.29077679945202,63.8333950202108));
#186875=CARTESIAN_POINT('Ctrl Pts',(128.125337211901,1.43266268615201,63.9784948477393));
#186876=CARTESIAN_POINT('Ctrl Pts',(127.970693827763,-2.55018990892399,
63.9004186071819));
#186877=CARTESIAN_POINT('Ctrl Pts',(126.682162320262,-6.31100362453699,
63.6019357427932));
#186878=CARTESIAN_POINT('Ctrl Pts',(124.372715075645,-9.52233348869999,
63.1050059715203));
#186879=CARTESIAN_POINT('Ctrl Pts',(121.244213149014,-11.90457676197,62.4488673034646));
#186880=CARTESIAN_POINT('Ctrl Pts',(117.569830709511,-13.25031727305,61.6866196830542));
#186881=CARTESIAN_POINT('Ctrl Pts',(113.670270424834,-13.44238464412,60.8806017050628));
#186882=CARTESIAN_POINT('Ctrl Pts',(109.885840654102,-12.46405603282,60.0969629436411));
#186883=CARTESIAN_POINT('Ctrl Pts',(106.5468256205,-10.40051214973,59.3999044685746));
#186884=CARTESIAN_POINT('Ctrl Pts',(103.944728361231,-7.43142077957798,
58.8460890131106));
#186885=CARTESIAN_POINT('Ctrl Pts',(102.306890261749,-3.81529354086099,
58.4797074865576));
#186886=CARTESIAN_POINT('Ctrl Pts',(101.776696990086,0.133022096717915,
58.3286313784788));
#186887=CARTESIAN_POINT('Ctrl Pts',(102.401094252842,4.06975582143802,58.4019860553738));
#186888=CARTESIAN_POINT('Ctrl Pts',(104.126500345876,7.65214573077102,58.6893562370528));
#186889=CARTESIAN_POINT('Ctrl Pts',(106.803471383925,10.56828178286,59.1616928299374));
#186890=CARTESIAN_POINT('Ctrl Pts',(110.199713018851,12.56426305087,59.7738421614973));
#186891=CARTESIAN_POINT('Ctrl Pts',(114.020305748331,13.46630426402,60.468477401625));
#186892=CARTESIAN_POINT('Ctrl Pts',(117.933382842896,13.19586687093,61.1810898709391));
#186893=CARTESIAN_POINT('Ctrl Pts',(121.599025188964,11.77649720398,61.8456056573345));
#186894=CARTESIAN_POINT('Ctrl Pts',(124.698857195672,9.33177634880501,62.4001385062092));
#186895=CARTESIAN_POINT('Ctrl Pts',(126.963767100501,6.07456026775601,62.7923781289308));
#186896=CARTESIAN_POINT('Ctrl Pts',(128.197337464837,2.28844683222602,62.9841446525445));
#186897=CARTESIAN_POINT('Ctrl Pts',(128.292948318726,-1.69691593830999,
62.9547131508873));
#186898=CARTESIAN_POINT('Ctrl Pts',(127.243054510346,-5.53453310529599,
62.7026169877071));
#186899=CARTESIAN_POINT('Ctrl Pts',(125.139864267274,-8.89026895716699,
62.2457797162281));
#186900=CARTESIAN_POINT('Ctrl Pts',(122.167230150241,-11.47196128996,61.61993883238));
#186901=CARTESIAN_POINT('Ctrl Pts',(119.779038466918,-12.52717214178,61.1237081036312));
#186902=CARTESIAN_POINT('Ctrl Pts',(118.535331233552,-12.86536116807,60.8659492134769));
#186903=CARTESIAN_POINT('',(114.54332401699,-13.8999637388745,63.4488532896085));
#186904=CARTESIAN_POINT('Origin',(114.28108174878,1.45439216225896E-14,
64.7979697995068));
#186905=CARTESIAN_POINT('Ctrl Pts',(125.314806796842,-7.34586304067299,
66.2271012509232));
#186906=CARTESIAN_POINT('Ctrl Pts',(124.206005057303,-9.06047151994499,
65.9865345966579));
#186907=CARTESIAN_POINT('Ctrl Pts',(121.195667841809,-11.9531828368,65.351308690418));
#186908=CARTESIAN_POINT('Ctrl Pts',(115.253048553756,-13.77380876573,64.1210656902771));
#186909=CARTESIAN_POINT('Ctrl Pts',(109.139940975145,-12.69068481913,62.8576829581376));
#186910=CARTESIAN_POINT('Ctrl Pts',(104.147645605334,-8.93253702461299,
61.8121651368307));
#186911=CARTESIAN_POINT('Ctrl Pts',(101.331541571415,-3.29144748217499,
61.1896581710675));
#186912=CARTESIAN_POINT('Ctrl Pts',(101.288190926181,3.04345072980601,61.1061225557624));
#186913=CARTESIAN_POINT('Ctrl Pts',(104.029702302623,8.73681175115401,61.5639119824844));
#186914=CARTESIAN_POINT('Ctrl Pts',(108.981147777474,12.58851139971,62.4512712260906));
#186915=CARTESIAN_POINT('Ctrl Pts',(115.101761761745,13.78663799238,63.5658949400986));
#186916=CARTESIAN_POINT('Ctrl Pts',(121.104326210735,12.07863428537,64.6575720344359));
#186917=CARTESIAN_POINT('Ctrl Pts',(125.72650412153,7.82453632784801,65.4809278277585));
#186918=CARTESIAN_POINT('Ctrl Pts',(127.996946293465,1.92107788542301,65.8471502199406));
#186919=CARTESIAN_POINT('Ctrl Pts',(127.439989976586,-4.38732683985899,
65.6637792772028));
#186920=CARTESIAN_POINT('Ctrl Pts',(124.176131537949,-9.77092748121999,
64.954237237506));
#186921=CARTESIAN_POINT('Ctrl Pts',(118.895857162348,-13.09482740292,63.8527416886753));
#186922=CARTESIAN_POINT('Ctrl Pts',(114.77659556862,-13.47069719745,63.0019616433146));
#186923=CARTESIAN_POINT('Ctrl Pts',(112.783656420258,-13.17864608329,62.5895352285786));
#186924=CARTESIAN_POINT('Ctrl Pts',(125.510689982049,-7.46222138870299,
66.141141974147));
#186925=CARTESIAN_POINT('Ctrl Pts',(124.384250561224,-9.20398923768399,
65.8971468848321));
#186926=CARTESIAN_POINT('Ctrl Pts',(121.326081093995,-12.14252105354,65.2526232843154));
#186927=CARTESIAN_POINT('Ctrl Pts',(115.289107974865,-13.99198566682,64.0040396657971));
#186928=CARTESIAN_POINT('Ctrl Pts',(109.078946033499,-12.89170505496,62.7217913824783));
#186929=CARTESIAN_POINT('Ctrl Pts',(104.007349947628,-9.07402826206999,
61.660858986546));
#186930=CARTESIAN_POINT('Ctrl Pts',(101.146416032104,-3.34358395537999,
61.0296379310526));
#186931=CARTESIAN_POINT('Ctrl Pts',(101.102155872688,3.09165893860202,60.9459255232173));
#186932=CARTESIAN_POINT('Ctrl Pts',(103.886869902922,8.87520270355401,61.4121127370459));
#186933=CARTESIAN_POINT('Ctrl Pts',(108.91652335081,12.78791321029,62.3146741464906));
#186934=CARTESIAN_POINT('Ctrl Pts',(115.133864917805,14.0050181082,63.4480998917577));
#186935=CARTESIAN_POINT('Ctrl Pts',(121.231287046849,12.26995965095,64.5582155432809));
#186936=CARTESIAN_POINT('Ctrl Pts',(125.926457337962,7.94847685275301,65.3957596888578));
#186937=CARTESIAN_POINT('Ctrl Pts',(128.232640435342,1.95150772707801,65.768929447846));
#186938=CARTESIAN_POINT('Ctrl Pts',(127.666639098998,-4.45682202381698,
65.5838003226546));
#186939=CARTESIAN_POINT('Ctrl Pts',(124.350858356457,-9.92569880953099,
64.8641655591087));
#186940=CARTESIAN_POINT('Ctrl Pts',(118.986721682142,-13.30224925054,63.7463687493917));
#186941=CARTESIAN_POINT('Ctrl Pts',(114.802062493028,-13.68407281635,62.8828766357867));
#186942=CARTESIAN_POINT('Ctrl Pts',(112.777480941574,-13.38739561741,62.4642995302622));
#186943=CARTESIAN_POINT('Ctrl Pts',(125.706573167286,-7.57857973669199,
66.0551826973766));
#186944=CARTESIAN_POINT('Ctrl Pts',(124.562496065176,-9.34750695538599,
65.8077591730122));
#186945=CARTESIAN_POINT('Ctrl Pts',(121.456494346225,-12.33185927026,65.1539378782213));
#186946=CARTESIAN_POINT('Ctrl Pts',(115.325167396024,-14.21016256789,63.8870136413267));
#186947=CARTESIAN_POINT('Ctrl Pts',(109.017951091899,-13.09272529082,62.5858998068277));
#186948=CARTESIAN_POINT('Ctrl Pts',(103.86705428995,-9.21551949956499,61.5095528362669));
#186949=CARTESIAN_POINT('Ctrl Pts',(100.961290492803,-3.39572042863199,
60.8696176910395));
#186950=CARTESIAN_POINT('Ctrl Pts',(100.916120819196,3.13986714735501,60.7857284906722));
#186951=CARTESIAN_POINT('Ctrl Pts',(103.744037503191,9.01359365592001,61.2603134916017));
#186952=CARTESIAN_POINT('Ctrl Pts',(108.851898924109,12.98731502086,62.1780770668837));
#186953=CARTESIAN_POINT('Ctrl Pts',(115.165968073829,14.22339822402,63.3303048434097));
#186954=CARTESIAN_POINT('Ctrl Pts',(121.358247882935,12.46128501656,64.4588590521206));
#186955=CARTESIAN_POINT('Ctrl Pts',(126.126410554373,8.07241737768201,65.3105915499533));
#186956=CARTESIAN_POINT('Ctrl Pts',(128.468334577209,1.98193756875801,65.6907086757495));
#186957=CARTESIAN_POINT('Ctrl Pts',(127.893288221429,-4.52631720775899,
65.5038213681102));
#186958=CARTESIAN_POINT('Ctrl Pts',(124.525585174978,-10.08047013783,64.7740938807138));
#186959=CARTESIAN_POINT('Ctrl Pts',(119.077586201943,-13.50967109816,63.6399958100993));
#186960=CARTESIAN_POINT('Ctrl Pts',(114.827529417439,-13.89744843525,62.763791628249));
#186961=CARTESIAN_POINT('Ctrl Pts',(112.771305462889,-13.59614515153,62.3390638319355));
#186962=CARTESIAN_POINT('Ctrl Pts',(125.902456352492,-7.69493808472198,
65.9692234206102));
#186963=CARTESIAN_POINT('Ctrl Pts',(124.740741569096,-9.49102467312499,
65.7183714611964));
#186964=CARTESIAN_POINT('Ctrl Pts',(121.58690759841,-12.521197487,65.0552524721285));
#186965=CARTESIAN_POINT('Ctrl Pts',(115.361226817132,-14.42833946898,63.7699876168566));
#186966=CARTESIAN_POINT('Ctrl Pts',(108.956956150252,-13.29374552665,62.4500082311784));
#186967=CARTESIAN_POINT('Ctrl Pts',(103.726758632241,-9.35701073702199,
61.358246685992));
#186968=CARTESIAN_POINT('Ctrl Pts',(100.776164953491,-3.44785690183699,
60.7095974510343));
#186969=CARTESIAN_POINT('Ctrl Pts',(100.730085765701,3.18807535615101,60.6255314581369));
#186970=CARTESIAN_POINT('Ctrl Pts',(103.601205103488,9.15198460832001,61.108514246173));
#186971=CARTESIAN_POINT('Ctrl Pts',(108.787274497443,13.18671683143,62.0414799872937));
#186972=CARTESIAN_POINT('Ctrl Pts',(115.198071229887,14.44177833984,63.2125097950786));
#186973=CARTESIAN_POINT('Ctrl Pts',(121.485208719049,12.65261038215,64.3595025609656));
#186974=CARTESIAN_POINT('Ctrl Pts',(126.326363770805,8.19635790258801,65.2254234110526));
#186975=CARTESIAN_POINT('Ctrl Pts',(128.704028719076,2.01236741041301,65.612487903653));
#186976=CARTESIAN_POINT('Ctrl Pts',(128.11993734384,-4.59581239171698,65.4238424135619));
#186977=CARTESIAN_POINT('Ctrl Pts',(124.700311993483,-10.23524146614,64.6840222023159));
#186978=CARTESIAN_POINT('Ctrl Pts',(119.16845072174,-13.71709294579,63.533622870806));
#186979=CARTESIAN_POINT('Ctrl Pts',(114.85299634185,-14.11082405414,62.6447066207113));
#186980=CARTESIAN_POINT('Ctrl Pts',(112.765129984206,-13.80489468565,62.2138281336091));
#186981=CARTESIAN_POINT('Ctrl Pts',(122.863511281691,-10.228475512234,65.6767278482884));
#186982=CARTESIAN_POINT('Ctrl Pts',(123.110780037318,-10.0253785434155,
65.7247922653008));
#186983=CARTESIAN_POINT('Ctrl Pts',(123.350863821086,-9.81319073816203,
65.7714600582926));
#186984=CARTESIAN_POINT('Ctrl Pts',(123.815499473612,-9.37175300744527,
65.8617765307689));
#186985=CARTESIAN_POINT('Ctrl Pts',(124.040059565785,-9.14248705860146,
65.9054268087314));
#186986=CARTESIAN_POINT('Ctrl Pts',(124.256220060446,-8.90528662689628,
65.9474443621852));
#186987=CARTESIAN_POINT('Ctrl Pts',(108.487103650414,-12.59742940801,63.245643627947));
#186988=CARTESIAN_POINT('Ctrl Pts',(106.956911188634,-11.85516766911,62.9280906814806));
#186989=CARTESIAN_POINT('Ctrl Pts',(104.171395799652,-9.78264817709099,
62.3464142802986));
#186990=CARTESIAN_POINT('Ctrl Pts',(101.389134172046,-5.33442980417999,
61.7452581710137));
#186991=CARTESIAN_POINT('Ctrl Pts',(100.385889140724,-0.155999799768285,
61.4899095833419));
#186992=CARTESIAN_POINT('Ctrl Pts',(101.300395977681,5.04380189940801,61.6073360569171));
#186993=CARTESIAN_POINT('Ctrl Pts',(104.00904923499,9.55311537764301,62.0735110066611));
#186994=CARTESIAN_POINT('Ctrl Pts',(108.142577067656,12.75463210302,62.8166548989901));
#186995=CARTESIAN_POINT('Ctrl Pts',(113.136659801733,14.21007092034,63.7270745538334));
#186996=CARTESIAN_POINT('Ctrl Pts',(118.309166198777,13.72018623447,64.6721764285147));
#186997=CARTESIAN_POINT('Ctrl Pts',(122.953540186654,11.35204195259,65.5146192499319));
#186998=CARTESIAN_POINT('Ctrl Pts',(126.435525741389,7.42983117316102,66.1311155208569));
#186999=CARTESIAN_POINT('Ctrl Pts',(128.279993910017,2.49049495110001,66.4293090676415));
#187000=CARTESIAN_POINT('Ctrl Pts',(128.235991923602,-2.78978417332599,
66.3604193700536));
#187001=CARTESIAN_POINT('Ctrl Pts',(126.31107853456,-7.68814761989499,65.925915708057));
#187002=CARTESIAN_POINT('Ctrl Pts',(122.770362013952,-11.53402684478,65.1773301664936));
#187003=CARTESIAN_POINT('Ctrl Pts',(118.099935873545,-13.80091069517,64.2091502239663));
#187004=CARTESIAN_POINT('Ctrl Pts',(114.660876983065,-14.05266506285,63.5004372009833));
#187005=CARTESIAN_POINT('Ctrl Pts',(112.977552505738,-13.85500477741,63.1531182574564));
#187006=CARTESIAN_POINT('Ctrl Pts',(108.599155925917,-12.4069384568,63.1433891917103));
#187007=CARTESIAN_POINT('Ctrl Pts',(107.092159102354,-11.67590076529,62.8303450430814));
#187008=CARTESIAN_POINT('Ctrl Pts',(104.348878573649,-9.63472069949199,
62.2568783080545));
#187009=CARTESIAN_POINT('Ctrl Pts',(101.608859568653,-5.25376568020898,
61.663933373787));
#187010=CARTESIAN_POINT('Ctrl Pts',(100.620955912659,-0.153640862146685,
61.4115668622755));
#187011=CARTESIAN_POINT('Ctrl Pts',(101.521805004111,4.96753248042701,61.526338525809));
#187012=CARTESIAN_POINT('Ctrl Pts',(104.189670484291,9.40865876062801,61.9845850952611));
#187013=CARTESIAN_POINT('Ctrl Pts',(108.260864420817,12.5617640247,62.715612445124));
#187014=CARTESIAN_POINT('Ctrl Pts',(113.179600451426,13.99519454845,63.6113861113676));
#187015=CARTESIAN_POINT('Ctrl Pts',(118.274062126846,13.51271761195,64.5413175532287));
#187016=CARTESIAN_POINT('Ctrl Pts',(122.848377502147,11.18038302126,65.3701422919282));
#187017=CARTESIAN_POINT('Ctrl Pts',(126.277881401572,7.31748161662602,65.9764371115622));
#187018=CARTESIAN_POINT('Ctrl Pts',(128.094629493962,2.45283514473701,66.2692423944695));
#187019=CARTESIAN_POINT('Ctrl Pts',(128.051463771229,-2.74759869058399,
66.2005152508861));
#187020=CARTESIAN_POINT('Ctrl Pts',(126.155828686743,-7.57189195330198,
65.7717027431803));
#187021=CARTESIAN_POINT('Ctrl Pts',(122.668823699534,-11.35961604446,65.0335577181838));
#187022=CARTESIAN_POINT('Ctrl Pts',(118.069191899904,-13.59222140462,64.0791388701734));
#187023=CARTESIAN_POINT('Ctrl Pts',(114.682250371862,-13.84016889016,63.380556486757));
#187024=CARTESIAN_POINT('Ctrl Pts',(113.024437105427,-13.64549750782,63.0381964450459));
#187025=CARTESIAN_POINT('Ctrl Pts',(108.711208201378,-12.21644750558,63.0411347554654));
#187026=CARTESIAN_POINT('Ctrl Pts',(107.227407016037,-11.49663386145,62.7325994046647));
#187027=CARTESIAN_POINT('Ctrl Pts',(104.526361347626,-9.48679322185798,
62.1673423358065));
#187028=CARTESIAN_POINT('Ctrl Pts',(101.82858496525,-5.17310155619299,61.5826085765585));
#187029=CARTESIAN_POINT('Ctrl Pts',(100.856022684594,-0.151281924479185,
61.3332241412091));
#187030=CARTESIAN_POINT('Ctrl Pts',(101.74321403056,4.89126306148702,61.4453409947047));
#187031=CARTESIAN_POINT('Ctrl Pts',(104.370291733622,9.26420214364402,61.8956591838669));
#187032=CARTESIAN_POINT('Ctrl Pts',(108.379151774013,12.3688959464,62.6145699912648));
#187033=CARTESIAN_POINT('Ctrl Pts',(113.222541101156,13.78031817656,63.4956976689091));
#187034=CARTESIAN_POINT('Ctrl Pts',(118.238958054948,13.30524898942,64.4104586779493));
#187035=CARTESIAN_POINT('Ctrl Pts',(122.743214817667,11.00872408991,65.2256653339196));
#187036=CARTESIAN_POINT('Ctrl Pts',(126.120237061767,7.20513206006702,65.8217587022596));
#187037=CARTESIAN_POINT('Ctrl Pts',(127.909265077919,2.41517533835002,66.1091757212896));
#187038=CARTESIAN_POINT('Ctrl Pts',(127.866935618859,-2.70541320786099,
66.0406111317087));
#187039=CARTESIAN_POINT('Ctrl Pts',(126.000578838919,-7.45563628672199,
65.6174897782919));
#187040=CARTESIAN_POINT('Ctrl Pts',(122.56728538511,-11.18520524415,64.8897852698628));
#187041=CARTESIAN_POINT('Ctrl Pts',(118.03844792626,-13.38353211408,63.9491275163697));
#187042=CARTESIAN_POINT('Ctrl Pts',(114.70362376066,-13.62767271748,63.2606757725306));
#187043=CARTESIAN_POINT('Ctrl Pts',(113.07132170512,-13.43599023824,62.923274632626));
#187044=CARTESIAN_POINT('Ctrl Pts',(108.82326047688,-12.02595655437,62.9388803192384));
#187045=CARTESIAN_POINT('Ctrl Pts',(107.36265492976,-11.31736695764,62.6348537662557));
#187046=CARTESIAN_POINT('Ctrl Pts',(104.703844121629,-9.33886574425999,
62.0778063635736));
#187047=CARTESIAN_POINT('Ctrl Pts',(102.048310361865,-5.09243743222199,
61.5012837793436));
#187048=CARTESIAN_POINT('Ctrl Pts',(101.091089456537,-0.148922986857685,
61.2548814201544));
#187049=CARTESIAN_POINT('Ctrl Pts',(101.964623056987,4.81499364250501,61.3643434636064));
#187050=CARTESIAN_POINT('Ctrl Pts',(104.550912982913,9.11974552662901,61.806733272465));
#187051=CARTESIAN_POINT('Ctrl Pts',(108.497439127174,12.17602786808,62.5135275373988));
#187052=CARTESIAN_POINT('Ctrl Pts',(113.26548175085,13.56544180466,63.3800092264433));
#187053=CARTESIAN_POINT('Ctrl Pts',(118.203853983017,13.0977803669,64.2795998026635));
#187054=CARTESIAN_POINT('Ctrl Pts',(122.638052133161,10.83706515858,65.081188375906));
#187055=CARTESIAN_POINT('Ctrl Pts',(125.962592721952,7.09278250353201,65.6670802929552));
#187056=CARTESIAN_POINT('Ctrl Pts',(127.723900661866,2.37751553198702,65.9491090481079));
#187057=CARTESIAN_POINT('Ctrl Pts',(127.682407466479,-2.66322772511999,
65.8807070125294));
#187058=CARTESIAN_POINT('Ctrl Pts',(125.845328991104,-7.33938062012898,
65.4632768134054));
#187059=CARTESIAN_POINT('Ctrl Pts',(122.465747070694,-11.01079444384,64.7460128215434));
#187060=CARTESIAN_POINT('Ctrl Pts',(118.007703952621,-13.17484282353,63.819116162567));
#187061=CARTESIAN_POINT('Ctrl Pts',(114.724997149458,-13.41517654479,63.1407950583042));
#187062=CARTESIAN_POINT('Ctrl Pts',(113.118206304812,-13.22648296865,62.8083528202057));
#187063=CARTESIAN_POINT('',(105.924484859737,-10.2222654049121,62.3840982248477));
#187064=CARTESIAN_POINT('Ctrl Pts',(105.924635027038,-10.2220806761209,
62.3841274145597));
#187065=CARTESIAN_POINT('Ctrl Pts',(106.171216296684,-10.4260967714227,
62.4320581971677));
#187066=CARTESIAN_POINT('Ctrl Pts',(106.425035137045,-10.6210421244567,
62.4813958280292));
#187067=CARTESIAN_POINT('Ctrl Pts',(106.941125769492,-10.9884663950073,
62.5817141853213));
#187068=CARTESIAN_POINT('Ctrl Pts',(107.203172821437,-11.1612912792639,
62.6326512264755));
#187069=CARTESIAN_POINT('Ctrl Pts',(107.470912577424,-11.3244123346074,
62.6846948227235));
#187070=CARTESIAN_POINT('Ctrl Pts',(105.924385870765,-10.2223568854093,
62.3842011440511));
#187071=CARTESIAN_POINT('Ctrl Pts',(105.918649582816,-10.2174500398891,
62.3830453968698));
#187072=CARTESIAN_POINT('Ctrl Pts',(105.91291738673,-10.2125381703083,62.3818904450698));
#187073=CARTESIAN_POINT('Ctrl Pts',(105.907189290968,-10.2076212837564,
62.3807362902962));
#187074=CARTESIAN_POINT('Origin',(114.428959431277,1.45439216225896E-14,
64.0372088705551));
#187075=CARTESIAN_POINT('Origin',(114.772417274494,1.45439216225896E-14,
62.2702802613769));
#187076=CARTESIAN_POINT('Origin',(117.386513081203,1.45439216225896E-14,
48.8219902915203));
#187077=CARTESIAN_POINT('Origin',(105.886046742854,0.700000000000015,61.8672681344988));
#187078=CARTESIAN_POINT('',(105.826348707759,0.200000000000015,62.1743863680917));
#187079=CARTESIAN_POINT('',(105.829634839229,0.700000000000015,62.1574807716032));
#187080=CARTESIAN_POINT('Origin',(108.32086073557,1.45439216225896E-14,
49.3412985381828));
#187081=CARTESIAN_POINT('',(105.886046742854,0.200000000000015,61.8672681344988));
#187082=CARTESIAN_POINT('',(105.886046742854,0.200000000000015,61.8672681344988));
#187083=CARTESIAN_POINT('',(105.886046742854,0.700000000000015,61.8672681344988));
#187084=CARTESIAN_POINT('',(105.886046742854,0.700000000000015,61.8672681344988));
#187085=CARTESIAN_POINT('',(105.886046742854,0.700000000000015,61.8672681344988));
#187086=CARTESIAN_POINT('Origin',(106.376860245404,0.700000000000015,61.962673090948));
#187087=CARTESIAN_POINT('',(105.983292743205,0.700000000000015,61.8861709364391));
#187088=CARTESIAN_POINT('',(105.983292743205,0.700000000000015,61.8861709364391));
#187089=CARTESIAN_POINT('',(106.326420107966,0.700000000000015,62.2221638076415));
#187090=CARTESIAN_POINT('Origin',(116.959178380441,0.700000000000015,51.0204257716897));
#187091=CARTESIAN_POINT('',(106.258735053168,0.700000000000015,62.570371490472));
#187092=CARTESIAN_POINT('',(106.326420107966,0.700000000000015,62.2221638076415));
#187093=CARTESIAN_POINT('Origin',(116.959178380441,0.700000000000015,51.0204257716897));
#187094=CARTESIAN_POINT('Origin',(106.376860245404,0.200000000000015,61.962673090948));
#187095=CARTESIAN_POINT('',(106.25552825787,0.200000000000015,62.5868689397725));
#187096=CARTESIAN_POINT('Origin',(108.811674238119,1.45439216225896E-14,
49.4367034946321));
#187097=CARTESIAN_POINT('',(106.323126090759,0.200000000000015,62.2391099725262));
#187098=CARTESIAN_POINT('Origin',(108.811674238119,1.45439216225896E-14,
49.4367034946321));
#187099=CARTESIAN_POINT('',(106.323126090759,0.200000000000015,62.2391099725262));
#187100=CARTESIAN_POINT('Origin',(105.886046742854,0.200000000000015,61.8672681344988));
#187101=CARTESIAN_POINT('Origin',(116.959178380441,0.200000000000015,51.0204257716897));
#187102=CARTESIAN_POINT('',(105.957946172011,0.200000000000015,61.8812440375083));
#187103=CARTESIAN_POINT('Origin',(116.959178380441,0.200000000000015,51.0204257716897));
#187104=CARTESIAN_POINT('',(105.886046742854,0.200000000000015,61.8672681344988));
#187105=CARTESIAN_POINT('Origin',(105.689721341835,1.45439216225896E-14,
61.8291061519191));
#187106=CARTESIAN_POINT('Origin',(114.524364387726,1.45439216225896E-14,
63.5463953680056));
#187107=CARTESIAN_POINT('Origin',(105.886046742854,1.7,61.8672681344988));
#187108=CARTESIAN_POINT('',(105.836586502542,1.2,62.121717742656));
#187109=CARTESIAN_POINT('',(105.847234601382,1.7,62.0669382963709));
#187110=CARTESIAN_POINT('Origin',(108.32086073557,1.45439216225896E-14,
49.3412985381828));
#187111=CARTESIAN_POINT('',(105.886046742854,1.2,61.8672681344988));
#187112=CARTESIAN_POINT('',(105.886046742854,1.2,61.8672681344988));
#187113=CARTESIAN_POINT('',(105.886046742854,1.7,61.8672681344988));
#187114=CARTESIAN_POINT('',(105.886046742854,1.7,61.8672681344988));
#187115=CARTESIAN_POINT('',(105.886046742854,1.7,61.8672681344988));
#187116=CARTESIAN_POINT('Origin',(106.376860245404,1.7,61.962673090948));
#187117=CARTESIAN_POINT('',(106.119765346029,1.7,61.9126986555448));
#187118=CARTESIAN_POINT('',(106.344062462215,1.7,62.1314022161617));
#187119=CARTESIAN_POINT('Origin',(116.959178380441,1.7,51.0204257716897));
#187120=CARTESIAN_POINT('',(106.27590645159,1.7,62.4820327445918));
#187121=CARTESIAN_POINT('',(106.344062462215,1.7,62.1314022161617));
#187122=CARTESIAN_POINT('Origin',(116.959178380441,1.7,51.0204257716897));
#187123=CARTESIAN_POINT('',(106.119765346029,1.7,61.9126986555448));
#187124=CARTESIAN_POINT('Origin',(106.376860245404,1.2,61.962673090948));
#187125=CARTESIAN_POINT('',(106.265518217696,1.2,62.5354753082978));
#187126=CARTESIAN_POINT('Origin',(108.811674238119,1.45439216225896E-14,
49.4367034946321));
#187127=CARTESIAN_POINT('',(106.333388522201,1.2,62.1863146031025));
#187128=CARTESIAN_POINT('Origin',(108.811674238119,1.45439216225896E-14,
49.4367034946321));
#187129=CARTESIAN_POINT('',(106.333388522201,1.2,62.1863146031025));
#187130=CARTESIAN_POINT('Origin',(105.886046742854,1.2,61.8672681344988));
#187131=CARTESIAN_POINT('Origin',(116.959178380441,1.2,51.0204257716897));
#187132=CARTESIAN_POINT('',(106.037050746853,1.2,61.8966204859526));
#187133=CARTESIAN_POINT('Origin',(116.959178380441,1.2,51.0204257716897));
#187134=CARTESIAN_POINT('',(105.886046742854,1.2,61.8672681344988));
#187135=CARTESIAN_POINT('Origin',(105.689721341835,1.,61.8291061519191));
#187136=CARTESIAN_POINT('Origin',(114.524364387726,1.45439216225896E-14,
63.5463953680056));
#187137=CARTESIAN_POINT('Origin',(106.376860245404,2.2,61.962673090948));
#187138=CARTESIAN_POINT('',(106.376375477714,2.70027257384477,61.9628795173321));
#187139=CARTESIAN_POINT('',(106.307693166583,2.7,62.3185050883679));
#187140=CARTESIAN_POINT('',(106.376860245404,2.7,61.962673090948));
#187141=CARTESIAN_POINT('',(106.35849029638,2.2,62.0571778143663));
#187142=CARTESIAN_POINT('Origin',(108.811674238119,1.45439216225896E-14,
49.4367034946321));
#187143=CARTESIAN_POINT('',(106.289944307572,2.2,62.4098145966144));
#187144=CARTESIAN_POINT('',(106.35849029638,2.2,62.0571778143663));
#187145=CARTESIAN_POINT('Origin',(108.811674238119,1.45439216225896E-14,
49.4367034946321));
#187146=CARTESIAN_POINT('Origin',(106.376860245404,2.7,61.962673090948));
#187147=CARTESIAN_POINT('',(105.886046742854,2.7,61.8672681344988));
#187148=CARTESIAN_POINT('',(105.879830381159,2.7,61.8992483834357));
#187149=CARTESIAN_POINT('',(105.886046742854,2.7,61.8672681344988));
#187150=CARTESIAN_POINT('',(105.689721341835,2.7,61.8291061519191));
#187151=CARTESIAN_POINT('Origin',(116.959178380441,2.7,51.0204257716897));
#187152=CARTESIAN_POINT('Origin',(105.886046742854,2.7,61.8672681344988));
#187153=CARTESIAN_POINT('',(105.886046742854,2.2,61.8672681344988));
#187154=CARTESIAN_POINT('',(105.861627150251,2.2,61.9928954207813));
#187155=CARTESIAN_POINT('',(105.886046742854,2.2,61.8672681344988));
#187156=CARTESIAN_POINT('',(105.886046742854,2.7,61.8672681344988));
#187157=CARTESIAN_POINT('Origin',(108.32086073557,1.45439216225896E-14,
49.3412985381828));
#187158=CARTESIAN_POINT('Origin',(105.886046742854,2.2,61.8672681344988));
#187159=CARTESIAN_POINT('',(106.232303035066,2.2,61.9345738754923));
#187160=CARTESIAN_POINT('Origin',(116.959178380441,2.2,51.0204257716897));
#187161=CARTESIAN_POINT('',(105.886046742854,2.2,61.8672681344988));
#187162=CARTESIAN_POINT('Origin',(116.959178380441,2.2,51.0204257716897));
#187163=CARTESIAN_POINT('Origin',(105.689721341835,2.,61.8291061519191));
#187164=CARTESIAN_POINT('Origin',(114.524364387726,1.45439216225896E-14,
63.5463953680056));
#187165=CARTESIAN_POINT('Origin',(106.867673747954,0.200000000000015,62.0580780473973));
#187166=CARTESIAN_POINT('',(107.193139079362,0.200000000000015,63.0041213568046));
#187167=CARTESIAN_POINT('',(107.12837091224,0.200000000000015,63.3373230283091));
#187168=CARTESIAN_POINT('',(107.193139079362,0.200000000000015,63.0041213568046));
#187169=CARTESIAN_POINT('',(106.755733004587,0.200000000000015,62.6339603744237));
#187170=CARTESIAN_POINT('Origin',(116.959178380441,0.200000000000015,51.0204257716897));
#187171=CARTESIAN_POINT('',(106.689640619927,0.200000000000015,62.9739745205872));
#187172=CARTESIAN_POINT('',(106.755733004587,0.200000000000015,62.6339603744237));
#187173=CARTESIAN_POINT('Origin',(116.959178380441,0.200000000000015,51.0204257716897));
#187174=CARTESIAN_POINT('Origin',(107.358487250503,0.200000000000015,62.1534830038465));
#187175=CARTESIAN_POINT('',(107.196291522778,0.700000000000015,62.9879035222976));
#187176=CARTESIAN_POINT('',(107.13144664939,0.700000000000015,63.3214998113625));
#187177=CARTESIAN_POINT('',(107.196291522778,0.700000000000015,62.9879035222976));
#187178=CARTESIAN_POINT('Origin',(109.793301243218,1.45439216225896E-14,
49.6275134075306));
#187179=CARTESIAN_POINT('Origin',(109.793301243218,1.45439216225896E-14,
49.6275134075306));
#187180=CARTESIAN_POINT('Origin',(107.358487250503,0.700000000000015,62.1534830038465));
#187181=CARTESIAN_POINT('',(106.758951639987,0.700000000000015,62.617402013381));
#187182=CARTESIAN_POINT('',(106.692777740288,0.700000000000015,62.9578355159706));
#187183=CARTESIAN_POINT('',(106.758951639987,0.700000000000015,62.617402013381));
#187184=CARTESIAN_POINT('Origin',(116.959178380441,0.700000000000015,51.0204257716897));
#187185=CARTESIAN_POINT('Origin',(116.959178380441,0.700000000000015,51.0204257716897));
#187186=CARTESIAN_POINT('Origin',(106.867673747954,0.700000000000015,62.0580780473973));
#187187=CARTESIAN_POINT('Origin',(109.302487740669,1.45439216225896E-14,
49.5321084510813));
#187188=CARTESIAN_POINT('Origin',(109.302487740669,1.45439216225896E-14,
49.5321084510813));
#187189=CARTESIAN_POINT('Origin',(106.867673747954,1.2,62.0580780473973));
#187190=CARTESIAN_POINT('',(107.202959280012,1.2,62.9536010562203));
#187191=CARTESIAN_POINT('',(107.1379515719,1.2,63.2880350531379));
#187192=CARTESIAN_POINT('',(107.202959280012,1.2,62.9536010562203));
#187193=CARTESIAN_POINT('',(106.765759948068,1.2,62.5823764794873));
#187194=CARTESIAN_POINT('Origin',(116.959178380441,1.2,51.0204257716897));
#187195=CARTESIAN_POINT('',(106.699412965644,1.2,62.9237004110643));
#187196=CARTESIAN_POINT('',(106.765759948068,1.2,62.5823764794873));
#187197=CARTESIAN_POINT('Origin',(116.959178380441,1.2,51.0204257716897));
#187198=CARTESIAN_POINT('Origin',(107.358487250503,1.2,62.1534830038465));
#187199=CARTESIAN_POINT('',(107.213169604484,1.7,62.9010737525815));
#187200=CARTESIAN_POINT('',(107.147910976393,1.7,63.2367986144447));
#187201=CARTESIAN_POINT('',(107.213169604484,1.7,62.9010737525815));
#187202=CARTESIAN_POINT('Origin',(109.793301243218,1.45439216225896E-14,
49.6275134075306));
#187203=CARTESIAN_POINT('Origin',(109.793301243218,1.45439216225896E-14,
49.6275134075306));
#187204=CARTESIAN_POINT('Origin',(107.358487250503,1.7,62.1534830038465));
#187205=CARTESIAN_POINT('',(106.776186950858,1.7,62.5287344680997));
#187206=CARTESIAN_POINT('',(106.709573150634,1.7,62.8714310514089));
#187207=CARTESIAN_POINT('',(106.776186950858,1.7,62.5287344680997));
#187208=CARTESIAN_POINT('Origin',(116.959178380441,1.7,51.0204257716897));
#187209=CARTESIAN_POINT('Origin',(116.959178380441,1.7,51.0204257716897));
#187210=CARTESIAN_POINT('Origin',(106.867673747954,1.7,62.0580780473973));
#187211=CARTESIAN_POINT('Origin',(109.302487740669,1.45439216225896E-14,
49.5321084510813));
#187212=CARTESIAN_POINT('Origin',(109.302487740669,1.45439216225896E-14,
49.5321084510813));
#187213=CARTESIAN_POINT('Origin',(106.867673747954,2.2,62.0580780473973));
#187214=CARTESIAN_POINT('',(107.226964778796,2.2,62.8301040873326));
#187215=CARTESIAN_POINT('',(107.16136407846,2.2,63.1675887495536));
#187216=CARTESIAN_POINT('',(107.226964778796,2.2,62.8301040873326));
#187217=CARTESIAN_POINT('',(106.790277706451,2.2,62.4562441765705));
#187218=CARTESIAN_POINT('Origin',(116.959178380441,2.2,51.0204257716897));
#187219=CARTESIAN_POINT('',(106.723299952499,2.2,62.80081313015));
#187220=CARTESIAN_POINT('',(106.790277706451,2.2,62.4562441765705));
#187221=CARTESIAN_POINT('Origin',(116.959178380441,2.2,51.0204257716897));
#187222=CARTESIAN_POINT('Origin',(107.358487250503,2.2,62.1534830038465));
#187223=CARTESIAN_POINT('',(107.244403008174,2.7,62.740392622037));
#187224=CARTESIAN_POINT('',(107.178364799778,2.7,63.0801280568769));
#187225=CARTESIAN_POINT('',(107.244403008174,2.7,62.740392622037));
#187226=CARTESIAN_POINT('Origin',(109.793301243218,1.45439216225896E-14,
49.6275134075306));
#187227=CARTESIAN_POINT('Origin',(109.793301243218,1.45439216225896E-14,
49.6275134075306));
#187228=CARTESIAN_POINT('Origin',(107.358487250503,2.7,62.1534830038465));
#187229=CARTESIAN_POINT('',(106.808094303375,2.7,62.3645861887142));
#187230=CARTESIAN_POINT('',(106.740650702402,2.7,62.7115517054976));
#187231=CARTESIAN_POINT('',(106.808094303375,2.7,62.3645861887142));
#187232=CARTESIAN_POINT('Origin',(116.959178380441,2.7,51.0204257716897));
#187233=CARTESIAN_POINT('Origin',(116.959178380441,2.7,51.0204257716897));
#187234=CARTESIAN_POINT('Origin',(106.867673747954,2.7,62.0580780473973));
#187235=CARTESIAN_POINT('Origin',(109.302487740669,1.45439216225896E-14,
49.5321084510813));
#187236=CARTESIAN_POINT('Origin',(109.302487740669,1.45439216225896E-14,
49.5321084510813));
#187237=CARTESIAN_POINT('Origin',(107.358487250503,3.2,62.1534830038465));
#187238=CARTESIAN_POINT('',(107.290529118892,3.7,62.5030955380819));
#187239=CARTESIAN_POINT('',(107.223305387788,3.7,62.8489299280895));
#187240=CARTESIAN_POINT('',(107.290529118892,3.7,62.5030955380819));
#187241=CARTESIAN_POINT('',(107.265559688949,3.2,62.631551478141));
#187242=CARTESIAN_POINT('Origin',(109.793301243218,1.45439216225896E-14,
49.6275134075306));
#187243=CARTESIAN_POINT('',(107.198982882686,3.2,62.9740577449709));
#187244=CARTESIAN_POINT('',(107.265559688949,3.2,62.631551478141));
#187245=CARTESIAN_POINT('Origin',(109.793301243218,1.45439216225896E-14,
49.6275134075306));
#187246=CARTESIAN_POINT('Origin',(107.358487250503,3.7,62.1534830038465));
#187247=CARTESIAN_POINT('',(106.85524751672,3.7,62.1220051461779));
#187248=CARTESIAN_POINT('',(106.786539588514,3.7,62.4754750302491));
#187249=CARTESIAN_POINT('',(106.85524751672,3.7,62.1220051461779));
#187250=CARTESIAN_POINT('Origin',(116.959178380441,3.7,51.0204257716897));
#187251=CARTESIAN_POINT('Origin',(116.959178380441,3.7,51.0204257716897));
#187252=CARTESIAN_POINT('Origin',(106.867673747954,3.7,62.0580780473973));
#187253=CARTESIAN_POINT('',(106.829717275668,3.2,62.2533461948846));
#187254=CARTESIAN_POINT('',(106.76169964183,3.2,62.6032648400092));
#187255=CARTESIAN_POINT('',(106.829717275668,3.2,62.2533461948846));
#187256=CARTESIAN_POINT('Origin',(109.302487740669,1.45439216225896E-14,
49.5321084510813));
#187257=CARTESIAN_POINT('Origin',(109.302487740669,1.45439216225896E-14,
49.5321084510813));
#187258=CARTESIAN_POINT('Origin',(106.867673747954,3.2,62.0580780473973));
#187259=CARTESIAN_POINT('Origin',(116.959178380441,3.2,51.0204257716897));
#187260=CARTESIAN_POINT('Origin',(116.959178380441,3.2,51.0204257716897));
#187261=CARTESIAN_POINT('Origin',(106.867673747954,4.7,62.0580780473973));
#187262=CARTESIAN_POINT('',(106.815284123344,4.2,62.327597956097));
#187263=CARTESIAN_POINT('',(106.848070426457,4.7,62.1589278904623));
#187264=CARTESIAN_POINT('Origin',(109.302487740669,1.45439216225896E-14,
49.5321084510813));
#187265=CARTESIAN_POINT('',(106.867673747954,4.2,62.0580780473973));
#187266=CARTESIAN_POINT('',(106.867673747954,4.2,62.0580780473973));
#187267=CARTESIAN_POINT('',(106.867673747954,4.7,62.0580780473973));
#187268=CARTESIAN_POINT('',(106.867673747954,4.7,62.0580780473973));
#187269=CARTESIAN_POINT('',(106.867673747954,4.7,62.0580780473973));
#187270=CARTESIAN_POINT('Origin',(107.358487250503,4.7,62.1534830038465));
#187271=CARTESIAN_POINT('',(107.30381546326,4.7,62.1428558319088));
#187272=CARTESIAN_POINT('',(107.352392077707,4.7,62.1848397930544));
#187273=CARTESIAN_POINT('Origin',(116.959178380441,4.7,51.0204257716897));
#187274=CARTESIAN_POINT('',(107.283510824698,4.7,62.5392013514836));
#187275=CARTESIAN_POINT('',(107.352392077707,4.7,62.1848397930544));
#187276=CARTESIAN_POINT('Origin',(116.959178380441,4.7,51.0204257716897));
#187277=CARTESIAN_POINT('',(107.30381546326,4.7,62.1428558319088));
#187278=CARTESIAN_POINT('Origin',(107.358487250503,4.2,62.1534830038465));
#187279=CARTESIAN_POINT('',(107.251438653183,4.2,62.7041975468769));
#187280=CARTESIAN_POINT('Origin',(109.793301243218,1.45439216225896E-14,
49.6275134075306));
#187281=CARTESIAN_POINT('',(107.319426744379,4.2,62.3544308847057));
#187282=CARTESIAN_POINT('Origin',(109.793301243218,1.45439216225896E-14,
49.6275134075306));
#187283=CARTESIAN_POINT('',(107.319426744379,4.2,62.3544308847057));
#187284=CARTESIAN_POINT('Origin',(106.867673747954,4.2,62.0580780473973));
#187285=CARTESIAN_POINT('Origin',(116.959178380441,4.2,51.0204257716897));
#187286=CARTESIAN_POINT('',(107.012752757131,4.2,62.0862786907789));
#187287=CARTESIAN_POINT('Origin',(116.959178380441,4.2,51.0204257716897));
#187288=CARTESIAN_POINT('',(106.867673747954,4.2,62.0580780473973));
#187289=CARTESIAN_POINT('Origin',(106.671348346934,4.,62.0199160648176));
#187290=CARTESIAN_POINT('Origin',(114.524364387726,1.45439216225896E-14,
63.5463953680056));
#187291=CARTESIAN_POINT('Origin',(111.775808773449,8.2,63.0121276118898));
#187292=CARTESIAN_POINT('',(112.23936365414,8.2,63.2477653210878));
#187293=CARTESIAN_POINT('',(112.171058441185,8.2,63.5991634251371));
#187294=CARTESIAN_POINT('',(112.23936365414,8.2,63.2477653210878));
#187295=CARTESIAN_POINT('',(111.767477236086,8.2,63.0549894419973));
#187296=CARTESIAN_POINT('Origin',(116.959178380441,8.2,51.0204257716897));
#187297=CARTESIAN_POINT('',(111.698657306259,8.2,63.4090355215762));
#187298=CARTESIAN_POINT('',(111.767477236086,8.2,63.0549894419973));
#187299=CARTESIAN_POINT('Origin',(116.959178380441,8.2,51.0204257716897));
#187300=CARTESIAN_POINT('Origin',(112.266622275998,8.2,63.107532568339));
#187301=CARTESIAN_POINT('',(112.266622275998,8.7,63.107532568339));
#187302=CARTESIAN_POINT('',(112.232598328127,8.7,63.2825697325142));
#187303=CARTESIAN_POINT('',(112.266622275998,8.7,63.107532568339));
#187304=CARTESIAN_POINT('',(112.266622275998,8.42058489655001,63.107532568339));
#187305=CARTESIAN_POINT('',(112.266622275998,8.42058489655001,63.107532568339));
#187306=CARTESIAN_POINT('Origin',(114.701436268713,1.45439216225896E-14,
50.5815629720231));
#187307=CARTESIAN_POINT('Origin',(114.701436268713,1.45439216225896E-14,
50.5815629720231));
#187308=CARTESIAN_POINT('Origin',(112.266622275998,8.7,63.107532568339));
#187309=CARTESIAN_POINT('',(111.775808773449,8.7,63.0121276118898));
#187310=CARTESIAN_POINT('',(111.760659644282,8.7,63.0900627362657));
#187311=CARTESIAN_POINT('',(111.775808773449,8.7,63.0121276118898));
#187312=CARTESIAN_POINT('',(112.266622275998,8.7,63.107532568339));
#187313=CARTESIAN_POINT('Origin',(116.959178380441,8.7,51.0204257716897));
#187314=CARTESIAN_POINT('Origin',(111.775808773449,8.7,63.0121276118898));
#187315=CARTESIAN_POINT('',(111.775808773449,8.26778386268001,63.0121276118898));
#187316=CARTESIAN_POINT('Origin',(114.210622766164,1.45439216225896E-14,
50.4861580155739));
#187317=CARTESIAN_POINT('',(111.775808773449,8.7,63.0121276118898));
#187318=CARTESIAN_POINT('Origin',(114.210622766164,1.45439216225896E-14,
50.4861580155739));
#187319=CARTESIAN_POINT('Origin',(111.579483372429,8.,62.9739656293101));
#187320=CARTESIAN_POINT('Origin',(114.524364387726,1.45439216225896E-14,
63.5463953680056));
#187321=CARTESIAN_POINT('Origin',(112.757435778548,8.2,63.2029375247883));
#187322=CARTESIAN_POINT('',(113.194515126452,8.2,63.5747793628157));
#187323=CARTESIAN_POINT('',(113.126917293563,8.2,63.922538330062));
#187324=CARTESIAN_POINT('',(113.194515126452,8.2,63.5747793628157));
#187325=CARTESIAN_POINT('',(112.715066123186,8.2,63.4209094176961));
#187326=CARTESIAN_POINT('Origin',(116.959178380441,8.2,51.0204257716897));
#187327=CARTESIAN_POINT('',(112.647166429423,8.2,63.7702213167638));
#187328=CARTESIAN_POINT('',(112.715066123186,8.2,63.4209094176961));
#187329=CARTESIAN_POINT('Origin',(116.959178380441,8.2,51.0204257716897));
#187330=CARTESIAN_POINT('Origin',(113.248249281097,8.2,63.2983424812375));
#187331=CARTESIAN_POINT('',(113.248249281097,8.7,63.2983424812375));
#187332=CARTESIAN_POINT('',(113.187821582277,8.7,63.6092144905408));
#187333=CARTESIAN_POINT('',(113.248249281097,8.7,63.2983424812375));
#187334=CARTESIAN_POINT('',(113.248249281097,8.63170029600201,63.2983424812375));
#187335=CARTESIAN_POINT('',(113.248249281097,8.63170029600201,63.2983424812375));
#187336=CARTESIAN_POINT('Origin',(115.683063273812,1.45439216225896E-14,
50.7723728849216));
#187337=CARTESIAN_POINT('Origin',(115.683063273812,1.45439216225896E-14,
50.7723728849216));
#187338=CARTESIAN_POINT('Origin',(113.248249281097,8.7,63.2983424812375));
#187339=CARTESIAN_POINT('',(112.757435778548,8.7,63.2029375247883));
#187340=CARTESIAN_POINT('',(112.708341954184,8.7,63.4555020957113));
#187341=CARTESIAN_POINT('',(112.757435778548,8.7,63.2029375247883));
#187342=CARTESIAN_POINT('',(113.248249281097,8.7,63.2983424812375));
#187343=CARTESIAN_POINT('Origin',(116.959178380441,8.7,51.0204257716897));
#187344=CARTESIAN_POINT('Origin',(112.757435778548,8.7,63.2029375247883));
#187345=CARTESIAN_POINT('',(112.757435778548,8.54144308650501,63.2029375247883));
#187346=CARTESIAN_POINT('Origin',(115.192249771263,1.45439216225896E-14,
50.6769679284724));
#187347=CARTESIAN_POINT('',(112.757435778548,8.7,63.2029375247883));
#187348=CARTESIAN_POINT('Origin',(115.192249771263,1.45439216225896E-14,
50.6769679284724));
#187349=CARTESIAN_POINT('Origin',(112.561110377528,8.,63.1647755422086));
#187350=CARTESIAN_POINT('Origin',(114.524364387726,1.45439216225896E-14,
63.5463953680056));
#187351=CARTESIAN_POINT('Origin',(113.739062783647,8.2,63.3937474376868));
#187352=CARTESIAN_POINT('',(114.164465217381,8.2,63.8256614916251));
#187353=CARTESIAN_POINT('',(114.097174797181,8.2,64.1718389655816));
#187354=CARTESIAN_POINT('',(114.164465217381,8.2,63.8256614916251));
#187355=CARTESIAN_POINT('',(113.677659493004,8.2,63.7096384067719));
#187356=CARTESIAN_POINT('Origin',(116.959178380441,8.2,51.0204257716897));
#187357=CARTESIAN_POINT('',(113.610263873378,8.2,64.0563570821562));
#187358=CARTESIAN_POINT('',(113.677659493004,8.2,63.7096384067719));
#187359=CARTESIAN_POINT('Origin',(116.959178380441,8.2,51.0204257716897));
#187360=CARTESIAN_POINT('Origin',(114.229876286196,8.2,63.489152394136));
#187361=CARTESIAN_POINT('',(114.226766123991,8.7,63.5051527117506));
#187362=CARTESIAN_POINT('',(114.157802851094,8.7,63.8599362238241));
#187363=CARTESIAN_POINT('',(114.226766123991,8.7,63.5051527117506));
#187364=CARTESIAN_POINT('Origin',(116.664690278911,1.45439216225896E-14,
50.9631827978201));
#187365=CARTESIAN_POINT('Origin',(116.664690278911,1.45439216225896E-14,
50.9631827978201));
#187366=CARTESIAN_POINT('Origin',(114.229876286196,8.7,63.489152394136));
#187367=CARTESIAN_POINT('',(113.739062783647,8.7,63.3937474376868));
#187368=CARTESIAN_POINT('',(113.670986458514,8.7,63.7439680218447));
#187369=CARTESIAN_POINT('',(113.739062783647,8.7,63.3937474376868));
#187370=CARTESIAN_POINT('',(113.825924529237,8.7,63.4106317349037));
#187371=CARTESIAN_POINT('',(113.825924529237,8.7,63.4106317349037));
#187372=CARTESIAN_POINT('Origin',(116.959178380441,8.7,51.0204257716897));
#187373=CARTESIAN_POINT('Origin',(116.959178380441,8.7,51.0204257716897));
#187374=CARTESIAN_POINT('Origin',(113.739062783647,8.7,63.3937474376868));
#187375=CARTESIAN_POINT('',(113.739062783647,8.69230981960501,63.3937474376868));
#187376=CARTESIAN_POINT('Origin',(116.173876776362,1.45439216225896E-14,
50.8677778413709));
#187377=CARTESIAN_POINT('',(113.739062783647,8.7,63.3937474376868));
#187378=CARTESIAN_POINT('Origin',(116.173876776362,1.45439216225896E-14,
50.8677778413709));
#187379=CARTESIAN_POINT('Origin',(113.542737382627,8.,63.3555854551071));
#187380=CARTESIAN_POINT('Origin',(114.524364387726,1.45439216225896E-14,
63.5463953680056));
#187381=CARTESIAN_POINT('Origin',(114.720689788746,8.2,63.5845573505853));
#187382=CARTESIAN_POINT('',(115.149006332374,8.2,64.0014796835762));
#187383=CARTESIAN_POINT('',(115.081639452434,8.2,64.3480505068311));
#187384=CARTESIAN_POINT('',(115.149006332374,8.2,64.0014796835762));
#187385=CARTESIAN_POINT('',(114.654914694975,8.2,63.9229391847761));
#187386=CARTESIAN_POINT('Origin',(116.959178380441,8.2,51.0204257716897));
#187387=CARTESIAN_POINT('',(114.587633813946,8.2,64.2690675841949));
#187388=CARTESIAN_POINT('',(114.654914694975,8.2,63.9229391847761));
#187389=CARTESIAN_POINT('Origin',(116.959178380441,8.2,51.0204257716897));
#187390=CARTESIAN_POINT('Origin',(115.211503291295,8.2,63.6799623070345));
#187391=CARTESIAN_POINT('',(115.211381799034,8.7,63.6805873274131));
#187392=CARTESIAN_POINT('',(115.142336212475,8.7,64.0357943044535));
#187393=CARTESIAN_POINT('',(115.211381799034,8.7,63.6805873274131));
#187394=CARTESIAN_POINT('Origin',(117.64631728401,1.45439216225896E-14,
51.1539927107186));
#187395=CARTESIAN_POINT('Origin',(117.64631728401,1.45439216225896E-14,
51.1539927107186));
#187396=CARTESIAN_POINT('Origin',(115.211503291295,8.7,63.6799623070345));
#187397=CARTESIAN_POINT('',(114.717206300373,8.7,63.6024782552524));
#187398=CARTESIAN_POINT('',(114.648253295989,8.7,63.9572089406661));
#187399=CARTESIAN_POINT('',(114.717206300373,8.7,63.6024782552524));
#187400=CARTESIAN_POINT('Origin',(116.959178380441,8.7,51.0204257716897));
#187401=CARTESIAN_POINT('Origin',(116.959178380441,8.7,51.0204257716897));
#187402=CARTESIAN_POINT('Origin',(114.720689788746,8.7,63.5845573505853));
#187403=CARTESIAN_POINT('Origin',(117.155503781461,1.45439216225896E-14,
51.0585877542694));
#187404=CARTESIAN_POINT('Origin',(117.155503781461,1.45439216225896E-14,
51.0585877542694));
#187405=CARTESIAN_POINT('Origin',(115.702316793845,8.2,63.7753672634838));
#187406=CARTESIAN_POINT('',(116.148189911293,8.2,64.1019693048485));
#187407=CARTESIAN_POINT('',(116.080358733155,8.2,64.4509287233428));
#187408=CARTESIAN_POINT('',(116.148189911293,8.2,64.1019693048485));
#187409=CARTESIAN_POINT('',(115.646754512291,8.2,64.0612089957596));
#187410=CARTESIAN_POINT('Origin',(116.959178380441,8.2,51.0204257716897));
#187411=CARTESIAN_POINT('',(115.579204990518,8.2,64.4087194251001));
#187412=CARTESIAN_POINT('',(115.646754512291,8.2,64.0612089957596));
#187413=CARTESIAN_POINT('Origin',(116.959178380441,8.2,51.0204257716897));
#187414=CARTESIAN_POINT('Origin',(116.193130296394,8.2,63.870772219933));
#187415=CARTESIAN_POINT('',(116.193130296394,8.7,63.870772219933));
#187416=CARTESIAN_POINT('',(116.141472694311,8.7,64.1365262180004));
#187417=CARTESIAN_POINT('',(116.193130296394,8.7,63.870772219933));
#187418=CARTESIAN_POINT('',(116.193130296394,8.56190691376601,63.870772219933));
#187419=CARTESIAN_POINT('',(116.193130296394,8.56190691376601,63.870772219933));
#187420=CARTESIAN_POINT('Origin',(118.62794428911,1.45439216225896E-14,
51.3448026236171));
#187421=CARTESIAN_POINT('Origin',(118.62794428911,1.45439216225896E-14,
51.3448026236171));
#187422=CARTESIAN_POINT('Origin',(116.193130296394,8.7,63.870772219933));
#187423=CARTESIAN_POINT('',(115.702316793845,8.7,63.7753672634838));
#187424=CARTESIAN_POINT('',(115.640065868523,8.7,64.0956189132026));
#187425=CARTESIAN_POINT('',(115.702316793845,8.7,63.7753672634838));
#187426=CARTESIAN_POINT('',(116.193130296394,8.7,63.870772219933));
#187427=CARTESIAN_POINT('Origin',(116.959178380441,8.7,51.0204257716897));
#187428=CARTESIAN_POINT('Origin',(115.702316793845,8.7,63.7753672634838));
#187429=CARTESIAN_POINT('',(115.702316793845,8.64616967217301,63.7753672634838));
#187430=CARTESIAN_POINT('Origin',(118.13713078656,1.45439216225896E-14,
51.2493976671679));
#187431=CARTESIAN_POINT('',(115.702316793845,8.7,63.7753672634838));
#187432=CARTESIAN_POINT('Origin',(118.13713078656,1.45439216225896E-14,
51.2493976671679));
#187433=CARTESIAN_POINT('Origin',(115.505991392825,8.,63.7372052809041));
#187434=CARTESIAN_POINT('Origin',(114.524364387726,1.45439216225896E-14,
63.5463953680056));
#187435=CARTESIAN_POINT('Origin',(116.683943798944,8.2,63.9661771763823));
#187436=CARTESIAN_POINT('',(117.16233107026,8.2,64.1255092316122));
#187437=CARTESIAN_POINT('',(117.093623142053,8.2,64.4789791156834));
#187438=CARTESIAN_POINT('',(117.16233107026,8.2,64.1255092316122));
#187439=CARTESIAN_POINT('',(116.653360186866,8.2,64.1235154355592));
#187440=CARTESIAN_POINT('Origin',(116.959178380441,8.2,51.0204257716897));
#187441=CARTESIAN_POINT('',(116.585144612751,8.2,64.4744523900495));
#187442=CARTESIAN_POINT('',(116.653360186866,8.2,64.1235154355592));
#187443=CARTESIAN_POINT('Origin',(116.959178380441,8.2,51.0204257716897));
#187444=CARTESIAN_POINT('Origin',(117.174757301493,8.2,64.0615821328315));
#187445=CARTESIAN_POINT('',(117.174757301493,8.7,64.0615821328315));
#187446=CARTESIAN_POINT('',(117.155524853906,8.7,64.1605240045573));
#187447=CARTESIAN_POINT('',(117.174757301493,8.7,64.0615821328315));
#187448=CARTESIAN_POINT('',(117.174757301493,8.30097885794202,64.0615821328315));
#187449=CARTESIAN_POINT('',(117.174757301493,8.30097885794202,64.0615821328315));
#187450=CARTESIAN_POINT('Origin',(119.609571294209,1.45439216225896E-14,
51.5356125365156));
#187451=CARTESIAN_POINT('Origin',(119.609571294209,1.45439216225896E-14,
51.5356125365156));
#187452=CARTESIAN_POINT('Origin',(117.174757301493,8.7,64.0615821328315));
#187453=CARTESIAN_POINT('',(116.683943798944,8.7,63.9661771763823));
#187454=CARTESIAN_POINT('',(116.646603960045,8.7,64.1582730359324));
#187455=CARTESIAN_POINT('',(116.683943798944,8.7,63.9661771763823));
#187456=CARTESIAN_POINT('',(117.174757301493,8.7,64.0615821328315));
#187457=CARTESIAN_POINT('Origin',(116.959178380441,8.7,51.0204257716897));
#187458=CARTESIAN_POINT('Origin',(116.683943798944,8.7,63.9661771763823));
#187459=CARTESIAN_POINT('',(116.683943798944,8.44726287030301,63.9661771763823));
#187460=CARTESIAN_POINT('Origin',(119.118757791659,1.45439216225896E-14,
51.4402075800664));
#187461=CARTESIAN_POINT('',(116.683943798944,8.7,63.9661771763823));
#187462=CARTESIAN_POINT('Origin',(119.118757791659,1.45439216225896E-14,
51.4402075800664));
#187463=CARTESIAN_POINT('Origin',(116.487618397924,8.,63.9280151938026));
#187464=CARTESIAN_POINT('Origin',(114.524364387726,1.45439216225896E-14,
63.5463953680056));
#187465=CARTESIAN_POINT('Origin',(122.573705829538,2.7,65.1110366537733));
#187466=CARTESIAN_POINT('',(122.54312221746,2.2,65.2683749129502));
#187467=CARTESIAN_POINT('',(122.474906643345,2.2,65.6193118674405));
#187468=CARTESIAN_POINT('',(122.54312221746,2.2,65.2683749129502));
#187469=CARTESIAN_POINT('',(122.561279598304,2.7,65.174963752554));
#187470=CARTESIAN_POINT('Origin',(125.008519822253,1.45439216225896E-14,
52.5850670574574));
#187471=CARTESIAN_POINT('',(122.492571670098,2.7,65.5284336366251));
#187472=CARTESIAN_POINT('',(122.561279598304,2.7,65.174963752554));
#187473=CARTESIAN_POINT('Origin',(125.008519822253,1.45439216225896E-14,
52.5850670574574));
#187474=CARTESIAN_POINT('Origin',(122.573705829538,2.2,65.1110366537733));
#187475=CARTESIAN_POINT('',(123.064519332087,2.2,65.2064416102226));
#187476=CARTESIAN_POINT('',(123.027179493189,2.2,65.3985374697727));
#187477=CARTESIAN_POINT('',(123.064519332087,2.2,65.2064416102226));
#187478=CARTESIAN_POINT('',(122.816425740386,2.2,65.1582168605189));
#187479=CARTESIAN_POINT('',(122.816425740386,2.2,65.1582168605189));
#187480=CARTESIAN_POINT('Origin',(116.959178380441,2.2,51.0204257716897));
#187481=CARTESIAN_POINT('Origin',(116.959178380441,2.2,51.0204257716897));
#187482=CARTESIAN_POINT('Origin',(123.064519332087,2.2,65.2064416102226));
#187483=CARTESIAN_POINT('',(123.064519332087,2.7,65.2064416102226));
#187484=CARTESIAN_POINT('',(123.0452868845,2.7,65.3053834819483));
#187485=CARTESIAN_POINT('',(123.064519332087,2.7,65.2064416102226));
#187486=CARTESIAN_POINT('',(123.064519332087,2.2,65.2064416102226));
#187487=CARTESIAN_POINT('Origin',(125.499333324803,1.45439216225896E-14,
52.6804720139067));
#187488=CARTESIAN_POINT('Origin',(123.064519332087,2.7,65.2064416102226));
#187489=CARTESIAN_POINT('',(122.672829403438,2.7,65.1303044208618));
#187490=CARTESIAN_POINT('Origin',(116.959178380441,2.7,51.0204257716897));
#187491=CARTESIAN_POINT('',(123.064519332087,2.7,65.2064416102226));
#187492=CARTESIAN_POINT('Origin',(116.959178380441,2.7,51.0204257716897));
#187493=CARTESIAN_POINT('Origin',(122.377380428518,2.,65.0728746711936));
#187494=CARTESIAN_POINT('Origin',(114.524364387726,1.45439216225896E-14,
63.5463953680056));
#187495=CARTESIAN_POINT('Origin',(122.573705829538,1.7,65.1110366537733));
#187496=CARTESIAN_POINT('',(122.518143547984,1.2,65.3968783860492));
#187497=CARTESIAN_POINT('',(122.450594026211,1.2,65.7443888153896));
#187498=CARTESIAN_POINT('',(122.518143547984,1.2,65.3968783860492));
#187499=CARTESIAN_POINT('',(122.528765444436,1.7,65.3422337386888));
#187500=CARTESIAN_POINT('Origin',(125.008519822253,1.45439216225896E-14,
52.5850670574574));
#187501=CARTESIAN_POINT('',(122.460934266298,1.7,65.6911931571831));
#187502=CARTESIAN_POINT('',(122.528765444436,1.7,65.3422337386888));
#187503=CARTESIAN_POINT('Origin',(125.008519822253,1.45439216225896E-14,
52.5850670574574));
#187504=CARTESIAN_POINT('Origin',(122.573705829538,1.2,65.1110366537733));
#187505=CARTESIAN_POINT('',(123.064519332087,1.2,65.2064416102226));
#187506=CARTESIAN_POINT('',(123.002268406765,1.2,65.5266932599413));
#187507=CARTESIAN_POINT('',(123.064519332087,1.2,65.2064416102226));
#187508=CARTESIAN_POINT('',(123.011678028599,1.2,65.1961702500586));
#187509=CARTESIAN_POINT('',(123.011678028599,1.2,65.1961702500586));
#187510=CARTESIAN_POINT('Origin',(116.959178380441,1.2,51.0204257716897));
#187511=CARTESIAN_POINT('Origin',(116.959178380441,1.2,51.0204257716897));
#187512=CARTESIAN_POINT('Origin',(123.064519332087,1.2,65.2064416102226));
#187513=CARTESIAN_POINT('',(123.064519332087,1.7,65.2064416102226));
#187514=CARTESIAN_POINT('',(123.012861730004,1.7,65.4721956082899));
#187515=CARTESIAN_POINT('',(123.064519332087,1.7,65.2064416102226));
#187516=CARTESIAN_POINT('',(123.064519332087,1.2,65.2064416102226));
#187517=CARTESIAN_POINT('Origin',(125.499333324803,1.45439216225896E-14,
52.6804720139067));
#187518=CARTESIAN_POINT('Origin',(123.064519332087,1.7,65.2064416102226));
#187519=CARTESIAN_POINT('',(122.928963429423,1.7,65.1800920804664));
#187520=CARTESIAN_POINT('Origin',(116.959178380441,1.7,51.0204257716897));
#187521=CARTESIAN_POINT('',(123.064519332087,1.7,65.2064416102226));
#187522=CARTESIAN_POINT('Origin',(116.959178380441,1.7,51.0204257716897));
#187523=CARTESIAN_POINT('Origin',(122.377380428518,1.,65.0728746711936));
#187524=CARTESIAN_POINT('Origin',(114.524364387726,1.45439216225896E-14,
63.5463953680056));
#187525=CARTESIAN_POINT('Origin',(122.573705829538,0.200000000000015,65.1110366537733));
#187526=CARTESIAN_POINT('',(123.061035843715,0.200000000000015,65.2243625148896));
#187527=CARTESIAN_POINT('',(122.99208283933,0.200000000000015,65.5790932003033));
#187528=CARTESIAN_POINT('',(123.061035843715,0.200000000000015,65.2243625148896));
#187529=CARTESIAN_POINT('',(122.507930735767,0.200000000000015,65.4494184879642));
#187530=CARTESIAN_POINT('Origin',(116.959178380441,0.200000000000015,51.0204257716897));
#187531=CARTESIAN_POINT('',(122.440649854738,0.200000000000015,65.7955468873829));
#187532=CARTESIAN_POINT('',(122.507930735767,0.200000000000015,65.4494184879642));
#187533=CARTESIAN_POINT('Origin',(116.959178380441,0.200000000000015,51.0204257716897));
#187534=CARTESIAN_POINT('Origin',(123.064519332087,0.200000000000015,65.2064416102226));
#187535=CARTESIAN_POINT('',(123.064397839827,0.700000000000015,65.2070666306011));
#187536=CARTESIAN_POINT('',(122.995352253267,0.700000000000015,65.5622736076416));
#187537=CARTESIAN_POINT('',(123.064397839827,0.700000000000015,65.2070666306011));
#187538=CARTESIAN_POINT('Origin',(125.499333324803,1.45439216225896E-14,
52.6804720139067));
#187539=CARTESIAN_POINT('Origin',(125.499333324803,1.45439216225896E-14,
52.6804720139067));
#187540=CARTESIAN_POINT('Origin',(123.064519332087,0.700000000000015,65.2064416102226));
#187541=CARTESIAN_POINT('',(122.511208870617,0.700000000000015,65.432554030315));
#187542=CARTESIAN_POINT('',(122.443841990677,0.700000000000015,65.7791248535699));
#187543=CARTESIAN_POINT('',(122.511208870617,0.700000000000015,65.432554030315));
#187544=CARTESIAN_POINT('Origin',(116.959178380441,0.700000000000015,51.0204257716897));
#187545=CARTESIAN_POINT('Origin',(116.959178380441,0.700000000000015,51.0204257716897));
#187546=CARTESIAN_POINT('Origin',(122.573705829538,0.700000000000015,65.1110366537733));
#187547=CARTESIAN_POINT('Origin',(125.008519822253,1.45439216225896E-14,
52.5850670574574));
#187548=CARTESIAN_POINT('Origin',(125.008519822253,1.45439216225896E-14,
52.5850670574574));
#187549=CARTESIAN_POINT('Origin',(107.849300753053,0.200000000000015,62.2488879602958));
#187550=CARTESIAN_POINT('',(108.081232306075,0.200000000000015,63.6761184436699));
#187551=CARTESIAN_POINT('',(108.018661167669,0.200000000000015,63.9980174386746));
#187552=CARTESIAN_POINT('',(108.081232306075,0.200000000000015,63.6761184436699));
#187553=CARTESIAN_POINT('',(107.635054033078,0.200000000000015,63.351086283674));
#187554=CARTESIAN_POINT('Origin',(116.959178380441,0.200000000000015,51.0204257716897));
#187555=CARTESIAN_POINT('',(107.571453128439,0.200000000000015,63.6782829402525));
#187556=CARTESIAN_POINT('',(107.635054033078,0.200000000000015,63.351086283674));
#187557=CARTESIAN_POINT('Origin',(116.959178380441,0.200000000000015,51.0204257716897));
#187558=CARTESIAN_POINT('Origin',(108.340114255602,0.200000000000015,62.344292916745));
#187559=CARTESIAN_POINT('',(108.084275160503,0.700000000000015,63.6604643928218));
#187560=CARTESIAN_POINT('',(108.021634869547,0.700000000000015,63.9827191450807));
#187561=CARTESIAN_POINT('',(108.084275160503,0.700000000000015,63.6604643928218));
#187562=CARTESIAN_POINT('Origin',(110.774928248317,1.45439216225896E-14,
49.8183233204291));
#187563=CARTESIAN_POINT('Origin',(110.774928248317,1.45439216225896E-14,
49.8183233204291));
#187564=CARTESIAN_POINT('Origin',(108.340114255602,0.700000000000015,62.344292916745));
#187565=CARTESIAN_POINT('',(107.638148217403,0.700000000000015,63.335168164717));
#187566=CARTESIAN_POINT('',(107.574474684828,0.700000000000015,63.6627384577665));
#187567=CARTESIAN_POINT('',(107.638148217403,0.700000000000015,63.335168164717));
#187568=CARTESIAN_POINT('Origin',(116.959178380441,0.700000000000015,51.0204257716897));
#187569=CARTESIAN_POINT('Origin',(116.959178380441,0.700000000000015,51.0204257716897));
#187570=CARTESIAN_POINT('Origin',(107.849300753053,0.700000000000015,62.2488879602958));
#187571=CARTESIAN_POINT('Origin',(110.284114745768,1.45439216225896E-14,
49.7229183639799));
#187572=CARTESIAN_POINT('Origin',(110.284114745768,1.45439216225896E-14,
49.7229183639799));
#187573=CARTESIAN_POINT('Origin',(107.849300753053,1.2,62.2488879602958));
#187574=CARTESIAN_POINT('',(108.090710291957,1.2,63.62735867666));
#187575=CARTESIAN_POINT('',(108.027923255991,1.2,63.9503683627822));
#187576=CARTESIAN_POINT('',(108.090710291957,1.2,63.62735867666));
#187577=CARTESIAN_POINT('',(107.644692296156,1.2,63.3015019660882));
#187578=CARTESIAN_POINT('Origin',(116.959178380441,1.2,51.0204257716897));
#187579=CARTESIAN_POINT('',(107.580864617103,1.2,63.6298652700673));
#187580=CARTESIAN_POINT('',(107.644692296156,1.2,63.3015019660882));
#187581=CARTESIAN_POINT('Origin',(116.959178380441,1.2,51.0204257716897));
#187582=CARTESIAN_POINT('Origin',(108.340114255602,1.2,62.344292916745));
#187583=CARTESIAN_POINT('',(108.100562188088,1.7,63.5766753177783));
#187584=CARTESIAN_POINT('',(108.037549170674,1.7,63.9008475718654));
#187585=CARTESIAN_POINT('',(108.100562188088,1.7,63.5766753177783));
#187586=CARTESIAN_POINT('Origin',(110.774928248317,1.45439216225896E-14,
49.8183233204291));
#187587=CARTESIAN_POINT('Origin',(110.774928248317,1.45439216225896E-14,
49.8183233204291));
#187588=CARTESIAN_POINT('Origin',(108.340114255602,1.7,62.344292916745));
#187589=CARTESIAN_POINT('',(107.654712027589,1.7,63.2499551737372));
#187590=CARTESIAN_POINT('',(107.590646898367,1.7,63.5795400468435));
#187591=CARTESIAN_POINT('',(107.654712027589,1.7,63.2499551737372));
#187592=CARTESIAN_POINT('Origin',(116.959178380441,1.7,51.0204257716897));
#187593=CARTESIAN_POINT('Origin',(116.959178380441,1.7,51.0204257716897));
#187594=CARTESIAN_POINT('Origin',(107.849300753053,1.7,62.2488879602958));
#187595=CARTESIAN_POINT('Origin',(110.284114745768,1.45439216225896E-14,
49.7229183639799));
#187596=CARTESIAN_POINT('Origin',(110.284114745768,1.45439216225896E-14,
49.7229183639799));
#187597=CARTESIAN_POINT('Origin',(107.849300753053,2.2,62.2488879602958));
#187598=CARTESIAN_POINT('',(108.113868797738,2.2,63.5082190872827));
#187599=CARTESIAN_POINT('',(108.050547990326,2.2,63.8339747757386));
#187600=CARTESIAN_POINT('',(108.113868797738,2.2,63.5082190872827));
#187601=CARTESIAN_POINT('',(107.668247350469,2.2,63.1803223215487));
#187602=CARTESIAN_POINT('Origin',(116.959178380441,2.2,51.0204257716897));
#187603=CARTESIAN_POINT('',(107.603858672105,2.2,63.5115717023834));
#187604=CARTESIAN_POINT('',(107.668247350469,2.2,63.1803223215487));
#187605=CARTESIAN_POINT('Origin',(116.959178380441,2.2,51.0204257716897));
#187606=CARTESIAN_POINT('Origin',(108.340114255602,2.2,62.344292916745));
#187607=CARTESIAN_POINT('',(108.130682275735,2.7,63.4217216731765));
#187608=CARTESIAN_POINT('',(108.066968286624,2.7,63.7495000960255));
#187609=CARTESIAN_POINT('',(108.130682275735,2.7,63.4217216731765));
#187610=CARTESIAN_POINT('Origin',(110.774928248317,1.45439216225896E-14,
49.8183233204291));
#187611=CARTESIAN_POINT('Origin',(110.774928248317,1.45439216225896E-14,
49.8183233204291));
#187612=CARTESIAN_POINT('Origin',(108.340114255602,2.7,62.344292916745));
#187613=CARTESIAN_POINT('',(107.685353195764,2.7,63.0923208155893));
#187614=CARTESIAN_POINT('',(107.620550970598,2.7,63.4256976996709));
#187615=CARTESIAN_POINT('',(107.685353195764,2.7,63.0923208155893));
#187616=CARTESIAN_POINT('Origin',(116.959178380441,2.7,51.0204257716897));
#187617=CARTESIAN_POINT('Origin',(116.959178380441,2.7,51.0204257716897));
#187618=CARTESIAN_POINT('Origin',(107.849300753053,2.7,62.2488879602958));
#187619=CARTESIAN_POINT('Origin',(110.284114745768,1.45439216225896E-14,
49.7229183639799));
#187620=CARTESIAN_POINT('Origin',(110.284114745768,1.45439216225896E-14,
49.7229183639799));
#187621=CARTESIAN_POINT('Origin',(107.849300753053,3.2,62.2488879602958));
#187622=CARTESIAN_POINT('',(108.151070036431,3.2,63.3168362604153));
#187623=CARTESIAN_POINT('',(108.086872760294,3.2,63.6471009670686));
#187624=CARTESIAN_POINT('',(108.151070036431,3.2,63.3168362604153));
#187625=CARTESIAN_POINT('',(107.706100636741,3.2,62.9855850174297));
#187626=CARTESIAN_POINT('Origin',(116.959178380441,3.2,51.0204257716897));
#187627=CARTESIAN_POINT('',(107.640789730382,3.2,63.3215788263236));
#187628=CARTESIAN_POINT('',(107.706100636741,3.2,62.9855850174297));
#187629=CARTESIAN_POINT('Origin',(116.959178380441,3.2,51.0204257716897));
#187630=CARTESIAN_POINT('Origin',(108.340114255602,3.2,62.344292916745));
#187631=CARTESIAN_POINT('',(108.175116167184,3.7,63.1931302592104));
#187632=CARTESIAN_POINT('',(108.110339490587,3.7,63.5263757079516));
#187633=CARTESIAN_POINT('',(108.175116167184,3.7,63.1931302592104));
#187634=CARTESIAN_POINT('Origin',(110.774928248317,1.45439216225896E-14,
49.8183233204291));
#187635=CARTESIAN_POINT('Origin',(110.774928248317,1.45439216225896E-14,
49.8183233204291));
#187636=CARTESIAN_POINT('Origin',(108.340114255602,3.7,62.344292916745));
#187637=CARTESIAN_POINT('',(107.730578435575,3.7,62.859658287547));
#187638=CARTESIAN_POINT('',(107.664657153423,3.7,63.1987921920089));
#187639=CARTESIAN_POINT('',(107.730578435575,3.7,62.859658287547));
#187640=CARTESIAN_POINT('Origin',(116.959178380441,3.7,51.0204257716897));
#187641=CARTESIAN_POINT('Origin',(116.959178380441,3.7,51.0204257716897));
#187642=CARTESIAN_POINT('Origin',(107.849300753053,3.7,62.2488879602958));
#187643=CARTESIAN_POINT('Origin',(110.284114745768,1.45439216225896E-14,
49.7229183639799));
#187644=CARTESIAN_POINT('Origin',(110.284114745768,1.45439216225896E-14,
49.7229183639799));
#187645=CARTESIAN_POINT('Origin',(107.849300753053,4.2,62.2488879602958));
#187646=CARTESIAN_POINT('',(108.202923274195,4.2,63.0500758090438));
#187647=CARTESIAN_POINT('',(108.137463560871,4.2,63.3868351595864));
#187648=CARTESIAN_POINT('',(108.202923274195,4.2,63.0500758090438));
#187649=CARTESIAN_POINT('',(107.758895068754,4.2,62.7139825655704));
#187650=CARTESIAN_POINT('Origin',(116.959178380441,4.2,51.0204257716897));
#187651=CARTESIAN_POINT('',(107.692253482546,4.2,63.0568220946606));
#187652=CARTESIAN_POINT('',(107.758895068754,4.2,62.7139825655704));
#187653=CARTESIAN_POINT('Origin',(116.959178380441,4.2,51.0204257716897));
#187654=CARTESIAN_POINT('Origin',(108.340114255602,4.2,62.344292916745));
#187655=CARTESIAN_POINT('',(108.234614861118,4.7,62.8870375418728));
#187656=CARTESIAN_POINT('',(108.168359143959,4.7,63.2278919567083));
#187657=CARTESIAN_POINT('',(108.234614861118,4.7,62.8870375418728));
#187658=CARTESIAN_POINT('Origin',(110.774928248317,1.45439216225896E-14,
49.8183233204291));
#187659=CARTESIAN_POINT('Origin',(110.774928248317,1.45439216225896E-14,
49.8183233204291));
#187660=CARTESIAN_POINT('Origin',(108.340114255602,4.7,62.344292916745));
#187661=CARTESIAN_POINT('',(107.791181346046,4.7,62.5478848969395));
#187662=CARTESIAN_POINT('',(107.723699286108,4.7,62.8950482669577));
#187663=CARTESIAN_POINT('',(107.791181346046,4.7,62.5478848969395));
#187664=CARTESIAN_POINT('Origin',(116.959178380441,4.7,51.0204257716897));
#187665=CARTESIAN_POINT('Origin',(116.959178380441,4.7,51.0204257716897));
#187666=CARTESIAN_POINT('Origin',(107.849300753053,4.7,62.2488879602958));
#187667=CARTESIAN_POINT('Origin',(110.284114745768,1.45439216225896E-14,
49.7229183639799));
#187668=CARTESIAN_POINT('Origin',(110.284114745768,1.45439216225896E-14,
49.7229183639799));
#187669=CARTESIAN_POINT('Origin',(107.849300753053,5.2,62.2488879602958));
#187670=CARTESIAN_POINT('',(108.203162162018,5.2,63.0488468438676));
#187671=CARTESIAN_POINT('',(107.759138382928,5.2,62.7127308289054));
#187672=CARTESIAN_POINT('Origin',(116.959178380441,5.2,51.0204257716897));
#187673=CARTESIAN_POINT('',(108.270338379292,5.2,62.703256890106));
#187674=CARTESIAN_POINT('',(108.270338379292,5.2,62.703256890106));
#187675=CARTESIAN_POINT('',(107.827593782639,5.2,62.3605600848366));
#187676=CARTESIAN_POINT('Origin',(116.959178380441,5.2,51.0204257716897));
#187677=CARTESIAN_POINT('',(107.827593782639,5.2,62.3605600848366));
#187678=CARTESIAN_POINT('Origin',(108.340114255602,5.2,62.344292916745));
#187679=CARTESIAN_POINT('',(108.242033679243,5.7,62.848871221758));
#187680=CARTESIAN_POINT('Origin',(110.774928248317,1.45439216225896E-14,
49.8183233204291));
#187681=CARTESIAN_POINT('',(108.310269142593,5.7,62.4978319465326));
#187682=CARTESIAN_POINT('',(108.310269142593,5.7,62.4978319465326));
#187683=CARTESIAN_POINT('Origin',(110.774928248317,1.45439216225896E-14,
49.8183233204291));
#187684=CARTESIAN_POINT('Origin',(108.340114255602,5.7,62.344292916745));
#187685=CARTESIAN_POINT('',(108.034759286615,5.7,62.2849376272788));
#187686=CARTESIAN_POINT('',(107.849300753053,5.7,62.2488879602958));
#187687=CARTESIAN_POINT('',(108.034759286615,5.7,62.2849376272788));
#187688=CARTESIAN_POINT('Origin',(116.959178380441,5.7,51.0204257716897));
#187689=CARTESIAN_POINT('',(107.798741589013,5.7,62.5089910127149));
#187690=CARTESIAN_POINT('Origin',(116.959178380441,5.7,51.0204257716897));
#187691=CARTESIAN_POINT('',(107.849300753053,5.7,62.2488879602958));
#187692=CARTESIAN_POINT('Origin',(107.849300753053,5.7,62.2488879602958));
#187693=CARTESIAN_POINT('Origin',(110.284114745768,1.45439216225896E-14,
49.7229183639799));
#187694=CARTESIAN_POINT('',(107.849300753053,5.47323030759702,62.2488879602958));
#187695=CARTESIAN_POINT('Origin',(110.284114745768,1.45439216225896E-14,
49.7229183639799));
#187696=CARTESIAN_POINT('',(107.849300753053,5.7,62.2488879602958));
#187697=CARTESIAN_POINT('Origin',(107.652975352033,5.,62.2107259777161));
#187698=CARTESIAN_POINT('Origin',(114.524364387726,1.45439216225896E-14,
63.5463953680056));
#187699=CARTESIAN_POINT('Origin',(109.812554763251,7.2,62.6305077860928));
#187700=CARTESIAN_POINT('',(110.259896542597,7.2,62.9495542546965));
#187701=CARTESIAN_POINT('',(110.192026238092,7.2,63.2987149598918));
#187702=CARTESIAN_POINT('',(110.259896542597,7.2,62.9495542546965));
#187703=CARTESIAN_POINT('',(109.802733452754,7.2,62.6810337963105));
#187704=CARTESIAN_POINT('Origin',(116.959178380441,7.2,51.0204257716897));
#187705=CARTESIAN_POINT('',(109.733954314151,7.2,63.0348700242867));
#187706=CARTESIAN_POINT('',(109.802733452754,7.2,62.6810337963105));
#187707=CARTESIAN_POINT('Origin',(116.959178380441,7.2,51.0204257716897));
#187708=CARTESIAN_POINT('Origin',(110.3033682658,7.2,62.725912742542));
#187709=CARTESIAN_POINT('',(110.3033682658,7.7,62.725912742542));
#187710=CARTESIAN_POINT('',(110.245860503599,7.7,63.0217630551504));
#187711=CARTESIAN_POINT('',(110.3033682658,7.7,62.725912742542));
#187712=CARTESIAN_POINT('',(110.3033682658,7.59646299273501,62.725912742542));
#187713=CARTESIAN_POINT('',(110.3033682658,7.59646299273501,62.725912742542));
#187714=CARTESIAN_POINT('Origin',(112.738182258515,1.45439216225896E-14,
50.1999431462261));
#187715=CARTESIAN_POINT('Origin',(112.738182258515,1.45439216225896E-14,
50.1999431462261));
#187716=CARTESIAN_POINT('Origin',(110.3033682658,7.7,62.725912742542));
#187717=CARTESIAN_POINT('',(109.812554763251,7.7,62.6305077860928));
#187718=CARTESIAN_POINT('',(109.788505318111,7.7,62.7542308382569));
#187719=CARTESIAN_POINT('',(109.812554763251,7.7,62.6305077860928));
#187720=CARTESIAN_POINT('',(110.3033682658,7.7,62.725912742542));
#187721=CARTESIAN_POINT('Origin',(116.959178380441,7.7,51.0204257716897));
#187722=CARTESIAN_POINT('Origin',(109.812554763251,7.7,62.6305077860928));
#187723=CARTESIAN_POINT('',(109.812554763251,7.29083328570901,62.6305077860928));
#187724=CARTESIAN_POINT('Origin',(112.247368755966,1.45439216225896E-14,
50.1045381897769));
#187725=CARTESIAN_POINT('',(109.812554763251,7.7,62.6305077860928));
#187726=CARTESIAN_POINT('Origin',(112.247368755966,1.45439216225896E-14,
50.1045381897769));
#187727=CARTESIAN_POINT('Origin',(109.616229362231,7.,62.5923458035131));
#187728=CARTESIAN_POINT('Origin',(114.524364387726,1.45439216225896E-14,
63.5463953680056));
#187729=CARTESIAN_POINT('Origin',(110.79418176835,7.2,62.8213176989913));
#187730=CARTESIAN_POINT('',(111.186312844935,7.2,63.424397192804));
#187731=CARTESIAN_POINT('',(111.119883400425,7.2,63.7661453529164));
#187732=CARTESIAN_POINT('',(111.186312844935,7.2,63.424397192804));
#187733=CARTESIAN_POINT('',(110.721137271773,7.2,63.1970971819562));
#187734=CARTESIAN_POINT('Origin',(116.959178380441,7.2,51.0204257716897));
#187735=CARTESIAN_POINT('',(110.654046326041,7.2,63.5422484538535));
#187736=CARTESIAN_POINT('',(110.721137271773,7.2,63.1970971819562));
#187737=CARTESIAN_POINT('Origin',(116.959178380441,7.2,51.0204257716897));
#187738=CARTESIAN_POINT('Origin',(111.284995270899,7.2,62.9167226554405));
#187739=CARTESIAN_POINT('',(111.240421969713,7.7,63.1460312667499));
#187740=CARTESIAN_POINT('',(111.172581016328,7.7,63.4950409742804));
#187741=CARTESIAN_POINT('',(111.240421969713,7.7,63.1460312667499));
#187742=CARTESIAN_POINT('Origin',(113.719809263614,1.45439216225896E-14,
50.3907530591246));
#187743=CARTESIAN_POINT('Origin',(113.719809263614,1.45439216225896E-14,
50.3907530591246));
#187744=CARTESIAN_POINT('Origin',(111.284995270899,7.7,62.9167226554405));
#187745=CARTESIAN_POINT('',(110.775811819326,7.7,62.9158224224096));
#187746=CARTESIAN_POINT('',(110.707265830517,7.7,63.2684592046577));
#187747=CARTESIAN_POINT('',(110.775811819326,7.7,62.9158224224096));
#187748=CARTESIAN_POINT('Origin',(116.959178380441,7.7,51.0204257716897));
#187749=CARTESIAN_POINT('Origin',(116.959178380441,7.7,51.0204257716897));
#187750=CARTESIAN_POINT('Origin',(110.79418176835,7.7,62.8213176989913));
#187751=CARTESIAN_POINT('Origin',(113.228995761065,1.45439216225896E-14,
50.2953481026754));
#187752=CARTESIAN_POINT('Origin',(113.228995761065,1.45439216225896E-14,
50.2953481026754));
#187753=CARTESIAN_POINT('Origin',(111.775808773449,7.2,63.0121276118898));
#187754=CARTESIAN_POINT('',(112.12801611812,7.2,63.8205958761048));
#187755=CARTESIAN_POINT('',(112.062591509714,7.2,64.1571746284032));
#187756=CARTESIAN_POINT('',(112.12801611812,7.2,63.8205958761048));
#187757=CARTESIAN_POINT('',(111.655304822504,7.2,63.6320636030099));
#187758=CARTESIAN_POINT('Origin',(116.959178380441,7.2,51.0204257716897));
#187759=CARTESIAN_POINT('',(111.589428346857,7.2,63.9709669991386));
#187760=CARTESIAN_POINT('',(111.655304822504,7.2,63.6320636030099));
#187761=CARTESIAN_POINT('Origin',(116.959178380441,7.2,51.0204257716897));
#187762=CARTESIAN_POINT('Origin',(112.266622275998,7.2,63.107532568339));
#187763=CARTESIAN_POINT('',(112.18126791696,7.7,63.5466404876378));
#187764=CARTESIAN_POINT('',(112.114496201417,7.7,63.8901494707866));
#187765=CARTESIAN_POINT('',(112.18126791696,7.7,63.5466404876378));
#187766=CARTESIAN_POINT('Origin',(114.701436268713,1.45439216225896E-14,
50.5815629720231));
#187767=CARTESIAN_POINT('Origin',(114.701436268713,1.45439216225896E-14,
50.5815629720231));
#187768=CARTESIAN_POINT('Origin',(112.266622275998,7.7,63.107532568339));
#187769=CARTESIAN_POINT('',(111.708941922635,7.7,63.3561260211292));
#187770=CARTESIAN_POINT('',(111.641689634785,7.7,63.7021073221314));
#187771=CARTESIAN_POINT('',(111.708941922635,7.7,63.3561260211292));
#187772=CARTESIAN_POINT('Origin',(116.959178380441,7.7,51.0204257716897));
#187773=CARTESIAN_POINT('Origin',(116.959178380441,7.7,51.0204257716897));
#187774=CARTESIAN_POINT('Origin',(111.775808773449,7.7,63.0121276118898));
#187775=CARTESIAN_POINT('Origin',(114.210622766164,1.45439216225896E-14,
50.4861580155739));
#187776=CARTESIAN_POINT('Origin',(114.210622766164,1.45439216225896E-14,
50.4861580155739));
#187777=CARTESIAN_POINT('Origin',(112.757435778548,7.2,63.2029375247883));
#187778=CARTESIAN_POINT('',(113.084301723809,7.2,64.141775336531));
#187779=CARTESIAN_POINT('',(113.019499498642,7.2,64.4751522206127));
#187780=CARTESIAN_POINT('',(113.084301723809,7.2,64.141775336531));
#187781=CARTESIAN_POINT('',(112.604368680805,7.2,63.9903955475575));
#187782=CARTESIAN_POINT('Origin',(116.959178380441,7.2,51.0204257716897));
#187783=CARTESIAN_POINT('',(112.539300670928,7.2,64.325139768617));
#187784=CARTESIAN_POINT('',(112.604368680805,7.2,63.9903955475575));
#187785=CARTESIAN_POINT('Origin',(116.959178380441,7.2,51.0204257716897));
#187786=CARTESIAN_POINT('Origin',(113.248249281097,7.2,63.2983424812375));
#187787=CARTESIAN_POINT('',(113.137023438408,7.7,63.8705469814669));
#187788=CARTESIAN_POINT('',(113.070912965334,7.7,64.2106541839858));
#187789=CARTESIAN_POINT('',(113.137023438408,7.7,63.8705469814669));
#187790=CARTESIAN_POINT('Origin',(115.683063273812,1.45439216225896E-14,
50.7723728849216));
#187791=CARTESIAN_POINT('Origin',(115.683063273812,1.45439216225896E-14,
50.7723728849216));
#187792=CARTESIAN_POINT('Origin',(113.248249281097,7.7,63.2983424812375));
#187793=CARTESIAN_POINT('',(112.657316677859,7.7,63.7180030759923));
#187794=CARTESIAN_POINT('',(112.590923921114,7.7,64.059562494862));
#187795=CARTESIAN_POINT('',(112.657316677859,7.7,63.7180030759923));
#187796=CARTESIAN_POINT('Origin',(116.959178380441,7.7,51.0204257716897));
#187797=CARTESIAN_POINT('Origin',(116.959178380441,7.7,51.0204257716897));
#187798=CARTESIAN_POINT('Origin',(112.757435778548,7.7,63.2029375247883));
#187799=CARTESIAN_POINT('Origin',(115.192249771263,1.45439216225896E-14,
50.6769679284724));
#187800=CARTESIAN_POINT('Origin',(115.192249771263,1.45439216225896E-14,
50.6769679284724));
#187801=CARTESIAN_POINT('Origin',(113.739062783647,7.2,63.3937474376868));
#187802=CARTESIAN_POINT('',(114.054744863706,7.2,64.3901209609489));
#187803=CARTESIAN_POINT('',(113.990213608426,7.2,64.7221038327708));
#187804=CARTESIAN_POINT('',(114.054744863706,7.2,64.3901209609489));
#187805=CARTESIAN_POINT('',(113.567770401368,7.2,64.2749659533184));
#187806=CARTESIAN_POINT('Origin',(116.959178380441,7.2,51.0204257716897));
#187807=CARTESIAN_POINT('',(113.503146384053,7.2,64.6074260420585));
#187808=CARTESIAN_POINT('',(113.567770401368,7.2,64.2749659533184));
#187809=CARTESIAN_POINT('Origin',(116.959178380441,7.2,51.0204257716897));
#187810=CARTESIAN_POINT('Origin',(114.229876286196,7.2,63.489152394136));
#187811=CARTESIAN_POINT('',(114.107236013427,7.7,64.1200787534334));
#187812=CARTESIAN_POINT('',(114.041413185149,7.7,64.4587061591514));
#187813=CARTESIAN_POINT('',(114.107236013427,7.7,64.1200787534334));
#187814=CARTESIAN_POINT('Origin',(116.664690278911,1.45439216225896E-14,
50.9631827978201));
#187815=CARTESIAN_POINT('Origin',(116.664690278911,1.45439216225896E-14,
50.9631827978201));
#187816=CARTESIAN_POINT('Origin',(114.229876286196,7.7,63.489152394136));
#187817=CARTESIAN_POINT('',(113.620340466169,7.7,64.0045177649381));
#187818=CARTESIAN_POINT('',(113.554419184017,7.7,64.3436516693999));
#187819=CARTESIAN_POINT('',(113.620340466169,7.7,64.0045177649381));
#187820=CARTESIAN_POINT('Origin',(116.959178380441,7.7,51.0204257716897));
#187821=CARTESIAN_POINT('Origin',(116.959178380441,7.7,51.0204257716897));
#187822=CARTESIAN_POINT('Origin',(113.739062783647,7.7,63.3937474376868));
#187823=CARTESIAN_POINT('Origin',(116.173876776362,1.45439216225896E-14,
50.8677778413709));
#187824=CARTESIAN_POINT('Origin',(116.173876776362,1.45439216225896E-14,
50.8677778413709));
#187825=CARTESIAN_POINT('Origin',(114.720689788746,7.2,63.5845573505853));
#187826=CARTESIAN_POINT('',(115.039163337421,7.2,64.5665700844302));
#187827=CARTESIAN_POINT('',(114.974564658518,7.2,64.8988998189938));
#187828=CARTESIAN_POINT('',(115.039163337421,7.2,64.5665700844302));
#187829=CARTESIAN_POINT('',(114.545209642576,7.2,64.4873199362524));
#187830=CARTESIAN_POINT('Origin',(116.959178380441,7.2,51.0204257716897));
#187831=CARTESIAN_POINT('',(114.48068680041,7.2,64.8192595265691));
#187832=CARTESIAN_POINT('',(114.545209642576,7.2,64.4873199362524));
#187833=CARTESIAN_POINT('Origin',(116.959178380441,7.2,51.0204257716897));
#187834=CARTESIAN_POINT('Origin',(115.211503291295,7.2,63.6799623070345));
#187835=CARTESIAN_POINT('',(115.091711844631,7.7,64.2962327996897));
#187836=CARTESIAN_POINT('',(115.025817457352,7.7,64.635228342716));
#187837=CARTESIAN_POINT('',(115.091711844631,7.7,64.2962327996897));
#187838=CARTESIAN_POINT('Origin',(117.64631728401,1.45439216225896E-14,
51.1539927107186));
#187839=CARTESIAN_POINT('Origin',(117.64631728401,1.45439216225896E-14,
51.1539927107186));
#187840=CARTESIAN_POINT('Origin',(115.211503291295,7.7,63.6799623070345));
#187841=CARTESIAN_POINT('',(114.597693635811,7.7,64.2173145454823));
#187842=CARTESIAN_POINT('',(114.531879736022,7.7,64.5558960183304));
#187843=CARTESIAN_POINT('',(114.597693635811,7.7,64.2173145454823));
#187844=CARTESIAN_POINT('Origin',(116.959178380441,7.7,51.0204257716897));
#187845=CARTESIAN_POINT('Origin',(116.959178380441,7.7,51.0204257716897));
#187846=CARTESIAN_POINT('Origin',(114.720689788746,7.7,63.5845573505853));
#187847=CARTESIAN_POINT('Origin',(117.155503781461,1.45439216225896E-14,
51.0585877542694));
#187848=CARTESIAN_POINT('Origin',(117.155503781461,1.45439216225896E-14,
51.0585877542694));
#187849=CARTESIAN_POINT('Origin',(115.702316793845,7.2,63.7753672634838));
#187850=CARTESIAN_POINT('',(116.037602325903,7.2,64.6708902723069));
#187851=CARTESIAN_POINT('',(115.972594617792,7.2,65.0053242692244));
#187852=CARTESIAN_POINT('',(116.037602325903,7.2,64.6708902723069));
#187853=CARTESIAN_POINT('',(115.536618587108,7.2,64.6278063844825));
#187854=CARTESIAN_POINT('Origin',(116.959178380441,7.2,51.0204257716897));
#187855=CARTESIAN_POINT('',(115.471858926109,7.2,64.9609642959974));
#187856=CARTESIAN_POINT('',(115.536618587108,7.2,64.6278063844825));
#187857=CARTESIAN_POINT('Origin',(116.959178380441,7.2,51.0204257716897));
#187858=CARTESIAN_POINT('Origin',(116.193130296394,7.2,63.870772219933));
#187859=CARTESIAN_POINT('',(116.090498972252,7.7,64.398761975897));
#187860=CARTESIAN_POINT('',(116.02417027306,7.7,64.7399918488676));
#187861=CARTESIAN_POINT('',(116.090498972252,7.7,64.398761975897));
#187862=CARTESIAN_POINT('Origin',(118.62794428911,1.45439216225896E-14,
51.3448026236171));
#187863=CARTESIAN_POINT('Origin',(118.62794428911,1.45439216225896E-14,
51.3448026236171));
#187864=CARTESIAN_POINT('Origin',(116.193130296394,7.7,63.870772219933));
#187865=CARTESIAN_POINT('',(115.589304075579,7.7,64.3567643957619));
#187866=CARTESIAN_POINT('',(115.523238795715,7.7,64.6966391005331));
#187867=CARTESIAN_POINT('',(115.589304075579,7.7,64.3567643957619));
#187868=CARTESIAN_POINT('Origin',(116.959178380441,7.7,51.0204257716897));
#187869=CARTESIAN_POINT('Origin',(116.959178380441,7.7,51.0204257716897));
#187870=CARTESIAN_POINT('Origin',(115.702316793845,7.7,63.7753672634838));
#187871=CARTESIAN_POINT('Origin',(118.13713078656,1.45439216225896E-14,
51.2493976671679));
#187872=CARTESIAN_POINT('Origin',(118.13713078656,1.45439216225896E-14,
51.2493976671679));
#187873=CARTESIAN_POINT('Origin',(116.683943798944,7.2,63.9661771763823));
#187874=CARTESIAN_POINT('',(117.050338122776,7.2,64.7016601241992));
#187875=CARTESIAN_POINT('',(116.984559900636,7.2,65.040058052371));
#187876=CARTESIAN_POINT('',(117.050338122776,7.2,64.7016601241992));
#187877=CARTESIAN_POINT('',(116.54215633591,7.2,64.695606798692));
#187878=CARTESIAN_POINT('Origin',(116.959178380441,7.2,51.0204257716897));
#187879=CARTESIAN_POINT('',(116.476810507479,7.2,65.0317802651764));
#187880=CARTESIAN_POINT('',(116.54215633591,7.2,64.695606798692));
#187881=CARTESIAN_POINT('Origin',(116.959178380441,7.2,51.0204257716897));
#187882=CARTESIAN_POINT('Origin',(117.174757301493,7.2,64.0615821328315));
#187883=CARTESIAN_POINT('',(117.103891411332,7.7,64.4261537133422));
#187884=CARTESIAN_POINT('',(117.036743654029,7.7,64.7715972539806));
#187885=CARTESIAN_POINT('',(117.103891411332,7.7,64.4261537133422));
#187886=CARTESIAN_POINT('Origin',(119.609571294209,1.45439216225896E-14,
51.5356125365156));
#187887=CARTESIAN_POINT('Origin',(119.609571294209,1.45439216225896E-14,
51.5356125365156));
#187888=CARTESIAN_POINT('Origin',(117.174757301493,7.7,64.0615821328315));
#187889=CARTESIAN_POINT('',(116.595340998606,7.7,64.421996794018));
#187890=CARTESIAN_POINT('',(116.528653025038,7.7,64.7650749642014));
#187891=CARTESIAN_POINT('',(116.595340998606,7.7,64.421996794018));
#187892=CARTESIAN_POINT('Origin',(116.959178380441,7.7,51.0204257716897));
#187893=CARTESIAN_POINT('Origin',(116.959178380441,7.7,51.0204257716897));
#187894=CARTESIAN_POINT('Origin',(116.683943798944,7.7,63.9661771763823));
#187895=CARTESIAN_POINT('Origin',(119.118757791659,1.45439216225896E-14,
51.4402075800664));
#187896=CARTESIAN_POINT('Origin',(119.118757791659,1.45439216225896E-14,
51.4402075800664));
#187897=CARTESIAN_POINT('Origin',(117.665570804043,7.2,64.1569870892808));
#187898=CARTESIAN_POINT('',(118.077901556091,7.2,64.6561487801456));
#187899=CARTESIAN_POINT('',(118.010952010662,7.2,65.0005726141802));
#187900=CARTESIAN_POINT('',(118.077901556091,7.2,64.6561487801456));
#187901=CARTESIAN_POINT('',(117.562222158485,7.2,64.6886671256));
#187902=CARTESIAN_POINT('Origin',(116.959178380441,7.2,51.0204257716897));
#187903=CARTESIAN_POINT('',(117.495911727413,7.2,65.0298030177092));
#187904=CARTESIAN_POINT('',(117.562222158485,7.2,64.6886671256));
#187905=CARTESIAN_POINT('Origin',(116.959178380441,7.2,51.0204257716897));
#187906=CARTESIAN_POINT('Origin',(118.156384306592,7.2,64.25239204573));
#187907=CARTESIAN_POINT('',(118.132455171377,7.7,64.375496160079));
#187908=CARTESIAN_POINT('',(118.06405996519,7.7,64.7273572368534));
#187909=CARTESIAN_POINT('',(118.132455171377,7.7,64.375496160079));
#187910=CARTESIAN_POINT('Origin',(120.591198299308,1.45439216225896E-14,
51.7264224494141));
#187911=CARTESIAN_POINT('Origin',(120.591198299308,1.45439216225896E-14,
51.7264224494141));
#187912=CARTESIAN_POINT('Origin',(118.156384306592,7.7,64.25239204573));
#187913=CARTESIAN_POINT('',(117.616229642986,7.7,64.4108240908324));
#187914=CARTESIAN_POINT('',(117.548515439084,7.7,64.7591817320498));
#187915=CARTESIAN_POINT('',(117.616229642986,7.7,64.4108240908324));
#187916=CARTESIAN_POINT('Origin',(116.959178380441,7.7,51.0204257716897));
#187917=CARTESIAN_POINT('Origin',(116.959178380441,7.7,51.0204257716897));
#187918=CARTESIAN_POINT('Origin',(117.665570804043,7.7,64.1569870892808));
#187919=CARTESIAN_POINT('Origin',(120.100384796758,1.45439216225896E-14,
51.6310174929649));
#187920=CARTESIAN_POINT('Origin',(120.100384796758,1.45439216225896E-14,
51.6310174929649));
#187921=CARTESIAN_POINT('Origin',(118.647197809142,7.2,64.3477970021793));
#187922=CARTESIAN_POINT('',(119.121125941224,7.2,64.5300692255833));
#187923=CARTESIAN_POINT('',(119.05253957496,7.2,64.8829137307956));
#187924=CARTESIAN_POINT('',(119.121125941224,7.2,64.5300692255833));
#187925=CARTESIAN_POINT('',(118.597490268611,7.2,64.6035188533173));
#187926=CARTESIAN_POINT('Origin',(116.959178380441,7.2,51.0204257716897));
#187927=CARTESIAN_POINT('',(118.529785785263,7.2,64.9518264868721));
#187928=CARTESIAN_POINT('',(118.597490268611,7.2,64.6035188533173));
#187929=CARTESIAN_POINT('Origin',(116.959178380441,7.2,51.0204257716897));
#187930=CARTESIAN_POINT('Origin',(119.138011311691,7.2,64.4432019586286));
#187931=CARTESIAN_POINT('',(119.138011311691,7.7,64.4432019586286));
#187932=CARTESIAN_POINT('',(119.10693856578,7.7,64.6030565806735));
#187933=CARTESIAN_POINT('',(119.138011311691,7.7,64.4432019586286));
#187934=CARTESIAN_POINT('',(119.138011311691,7.35569507252702,64.4432019586286));
#187935=CARTESIAN_POINT('',(119.138011311691,7.35569507252702,64.4432019586286));
#187936=CARTESIAN_POINT('Origin',(121.572825304407,1.45439216225896E-14,
51.9172323623126));
#187937=CARTESIAN_POINT('Origin',(121.572825304407,1.45439216225896E-14,
51.9172323623126));
#187938=CARTESIAN_POINT('Origin',(119.138011311691,7.7,64.4432019586286));
#187939=CARTESIAN_POINT('',(118.647197809142,7.7,64.3477970021793));
#187940=CARTESIAN_POINT('',(118.58348926054,7.7,64.6755474361724));
#187941=CARTESIAN_POINT('',(118.647197809142,7.7,64.3477970021793));
#187942=CARTESIAN_POINT('',(119.138011311691,7.7,64.4432019586286));
#187943=CARTESIAN_POINT('Origin',(116.959178380441,7.7,51.0204257716897));
#187944=CARTESIAN_POINT('Origin',(118.647197809142,7.7,64.3477970021793));
#187945=CARTESIAN_POINT('',(118.647197809142,7.65220556441102,64.3477970021793));
#187946=CARTESIAN_POINT('Origin',(121.082011801857,1.45439216225896E-14,
51.8218274058634));
#187947=CARTESIAN_POINT('',(118.647197809142,7.7,64.3477970021793));
#187948=CARTESIAN_POINT('Origin',(121.082011801857,1.45439216225896E-14,
51.8218274058634));
#187949=CARTESIAN_POINT('Origin',(118.450872408122,7.,64.3096350195996));
#187950=CARTESIAN_POINT('Origin',(114.524364387726,1.45439216225896E-14,
63.5463953680056));
#187951=CARTESIAN_POINT('Origin',(121.592078824439,4.7,64.9202267408748));
#187952=CARTESIAN_POINT('',(121.542371283908,4.2,65.1759485920128));
#187953=CARTESIAN_POINT('',(121.47466680056,4.2,65.5242562255676));
#187954=CARTESIAN_POINT('',(121.542371283908,4.2,65.1759485920128));
#187955=CARTESIAN_POINT('',(121.575193453972,4.7,65.0070940078296));
#187956=CARTESIAN_POINT('Origin',(124.026892817154,1.45439216225896E-14,
52.3942571445589));
#187957=CARTESIAN_POINT('',(121.506607087708,4.7,65.3599385130419));
#187958=CARTESIAN_POINT('',(121.575193453972,4.7,65.0070940078296));
#187959=CARTESIAN_POINT('Origin',(124.026892817154,1.45439216225896E-14,
52.3942571445589));
#187960=CARTESIAN_POINT('Origin',(121.592078824439,4.2,64.9202267408748));
#187961=CARTESIAN_POINT('',(122.082892326988,4.2,65.0156316973241));
#187962=CARTESIAN_POINT('',(122.019183778387,4.2,65.3433821313171));
#187963=CARTESIAN_POINT('',(122.082892326988,4.2,65.0156316973241));
#187964=CARTESIAN_POINT('',(122.035976018321,4.2,65.0065120452323));
#187965=CARTESIAN_POINT('',(122.035976018321,4.2,65.0065120452323));
#187966=CARTESIAN_POINT('Origin',(116.959178380441,4.2,51.0204257716897));
#187967=CARTESIAN_POINT('Origin',(116.959178380441,4.2,51.0204257716897));
#187968=CARTESIAN_POINT('Origin',(122.082892326988,4.2,65.0156316973241));
#187969=CARTESIAN_POINT('',(122.082892326988,4.7,65.0156316973241));
#187970=CARTESIAN_POINT('',(122.051819581077,4.7,65.175486319369));
#187971=CARTESIAN_POINT('',(122.082892326988,4.7,65.0156316973241));
#187972=CARTESIAN_POINT('',(122.082892326988,4.2,65.0156316973241));
#187973=CARTESIAN_POINT('Origin',(124.517706319704,1.45439216225896E-14,
52.4896621010082));
#187974=CARTESIAN_POINT('Origin',(122.082892326988,4.7,65.0156316973241));
#187975=CARTESIAN_POINT('',(121.744913312192,4.7,64.9499349041024));
#187976=CARTESIAN_POINT('Origin',(116.959178380441,4.7,51.0204257716897));
#187977=CARTESIAN_POINT('',(122.082892326988,4.7,65.0156316973241));
#187978=CARTESIAN_POINT('Origin',(116.959178380441,4.7,51.0204257716897));
#187979=CARTESIAN_POINT('Origin',(121.395753423419,4.,64.8820647582951));
#187980=CARTESIAN_POINT('Origin',(114.524364387726,1.45439216225896E-14,
63.5463953680056));
#187981=CARTESIAN_POINT('Origin',(121.592078824439,3.2,64.9202267408748));
#187982=CARTESIAN_POINT('',(122.033551165931,3.2,65.2694686988757));
#187983=CARTESIAN_POINT('',(121.96583696203,3.2,65.6178263400931));
#187984=CARTESIAN_POINT('',(122.033551165931,3.2,65.2694686988757));
#187985=CARTESIAN_POINT('',(121.488730178881,3.2,65.451906777194));
#187986=CARTESIAN_POINT('Origin',(116.959178380441,3.2,51.0204257716897));
#187987=CARTESIAN_POINT('',(121.422419747809,3.2,65.7930426693032));
#187988=CARTESIAN_POINT('',(121.488730178881,3.2,65.451906777194));
#187989=CARTESIAN_POINT('Origin',(116.959178380441,3.2,51.0204257716897));
#187990=CARTESIAN_POINT('Origin',(122.082892326988,3.2,65.0156316973241));
#187991=CARTESIAN_POINT('',(122.058963191773,3.7,65.138735811673));
#187992=CARTESIAN_POINT('',(121.990567985586,3.7,65.4905968884474));
#187993=CARTESIAN_POINT('',(122.058963191773,3.7,65.138735811673));
#187994=CARTESIAN_POINT('Origin',(124.517706319704,1.45439216225896E-14,
52.4896621010082));
#187995=CARTESIAN_POINT('Origin',(124.517706319704,1.45439216225896E-14,
52.4896621010082));
#187996=CARTESIAN_POINT('Origin',(122.082892326988,3.7,65.0156316973241));
#187997=CARTESIAN_POINT('',(121.513596073938,3.7,65.3239834752904));
#187998=CARTESIAN_POINT('',(121.446646528509,3.7,65.6684073093249));
#187999=CARTESIAN_POINT('',(121.513596073938,3.7,65.3239834752904));
#188000=CARTESIAN_POINT('Origin',(116.959178380441,3.7,51.0204257716897));
#188001=CARTESIAN_POINT('Origin',(116.959178380441,3.7,51.0204257716897));
#188002=CARTESIAN_POINT('Origin',(121.592078824439,3.7,64.9202267408748));
#188003=CARTESIAN_POINT('Origin',(124.026892817154,1.45439216225896E-14,
52.3942571445589));
#188004=CARTESIAN_POINT('Origin',(124.026892817154,1.45439216225896E-14,
52.3942571445589));
#188005=CARTESIAN_POINT('Origin',(121.592078824439,2.2,64.9202267408748));
#188006=CARTESIAN_POINT('',(121.994289526651,2.2,65.4714513149597));
#188007=CARTESIAN_POINT('',(121.927601553083,2.2,65.8145294851432));
#188008=CARTESIAN_POINT('',(121.994289526651,2.2,65.4714513149597));
#188009=CARTESIAN_POINT('',(121.450291361405,2.2,65.6496563631845));
#188010=CARTESIAN_POINT('Origin',(116.959178380441,2.2,51.0204257716897));
#188011=CARTESIAN_POINT('',(121.384945532974,2.2,65.9858298296689));
#188012=CARTESIAN_POINT('',(121.450291361405,2.2,65.6496563631845));
#188013=CARTESIAN_POINT('Origin',(116.959178380441,2.2,51.0204257716897));
#188014=CARTESIAN_POINT('Origin',(122.082892326988,2.2,65.0156316973241));
#188015=CARTESIAN_POINT('',(122.012026436827,2.7,65.3802032778347));
#188016=CARTESIAN_POINT('',(121.944878679524,2.7,65.7256468184731));
#188017=CARTESIAN_POINT('',(122.012026436827,2.7,65.3802032778347));
#188018=CARTESIAN_POINT('Origin',(124.517706319704,1.45439216225896E-14,
52.4896621010082));
#188019=CARTESIAN_POINT('Origin',(124.517706319704,1.45439216225896E-14,
52.4896621010082));
#188020=CARTESIAN_POINT('Origin',(122.082892326988,2.7,65.0156316973241));
#188021=CARTESIAN_POINT('',(121.467659645721,2.7,65.5603047322425));
#188022=CARTESIAN_POINT('',(121.401881423582,2.7,65.8987026604143));
#188023=CARTESIAN_POINT('',(121.467659645721,2.7,65.5603047322425));
#188024=CARTESIAN_POINT('Origin',(116.959178380441,2.7,51.0204257716897));
#188025=CARTESIAN_POINT('Origin',(116.959178380441,2.7,51.0204257716897));
#188026=CARTESIAN_POINT('Origin',(121.592078824439,2.7,64.9202267408748));
#188027=CARTESIAN_POINT('Origin',(124.026892817154,1.45439216225896E-14,
52.3942571445589));
#188028=CARTESIAN_POINT('Origin',(124.026892817154,1.45439216225896E-14,
52.3942571445589));
#188029=CARTESIAN_POINT('Origin',(121.592078824439,1.2,64.9202267408748));
#188030=CARTESIAN_POINT('',(121.969879608722,1.2,65.5970288296021));
#188031=CARTESIAN_POINT('',(121.903814328859,1.2,65.9369035343734));
#188032=CARTESIAN_POINT('',(121.969879608722,1.2,65.5970288296021));
#188033=CARTESIAN_POINT('',(121.426380617702,1.2,65.7726658618735));
#188034=CARTESIAN_POINT('Origin',(116.959178380441,1.2,51.0204257716897));
#188035=CARTESIAN_POINT('',(121.361620956703,1.2,66.1058237733884));
#188036=CARTESIAN_POINT('',(121.426380617702,1.2,65.7726658618735));
#188037=CARTESIAN_POINT('Origin',(116.959178380441,1.2,51.0204257716897));
#188038=CARTESIAN_POINT('Origin',(122.082892326988,1.2,65.0156316973241));
#188039=CARTESIAN_POINT('',(121.980261002846,1.7,65.543621453288));
#188040=CARTESIAN_POINT('',(121.913932303654,1.7,65.8848513262587));
#188041=CARTESIAN_POINT('',(121.980261002846,1.7,65.543621453288));
#188042=CARTESIAN_POINT('Origin',(124.517706319704,1.45439216225896E-14,
52.4896621010082));
#188043=CARTESIAN_POINT('Origin',(124.517706319704,1.45439216225896E-14,
52.4896621010082));
#188044=CARTESIAN_POINT('Origin',(122.082892326988,1.7,65.0156316973241));
#188045=CARTESIAN_POINT('',(121.436550853948,1.7,65.7203447932486));
#188046=CARTESIAN_POINT('',(121.371543145836,1.7,66.0547787901662));
#188047=CARTESIAN_POINT('',(121.436550853948,1.7,65.7203447932486));
#188048=CARTESIAN_POINT('Origin',(116.959178380441,1.7,51.0204257716897));
#188049=CARTESIAN_POINT('Origin',(116.959178380441,1.7,51.0204257716897));
#188050=CARTESIAN_POINT('Origin',(121.592078824439,1.7,64.9202267408748));
#188051=CARTESIAN_POINT('Origin',(124.026892817154,1.45439216225896E-14,
52.3942571445589));
#188052=CARTESIAN_POINT('Origin',(124.026892817154,1.45439216225896E-14,
52.3942571445589));
#188053=CARTESIAN_POINT('Origin',(121.592078824439,0.200000000000015,64.9202267408748));
#188054=CARTESIAN_POINT('',(121.959896174053,0.200000000000015,65.6483888922211));
#188055=CARTESIAN_POINT('',(121.894082274265,0.200000000000015,65.9869703650692));
#188056=CARTESIAN_POINT('',(121.959896174053,0.200000000000015,65.6483888922211));
#188057=CARTESIAN_POINT('',(121.416598678269,0.200000000000015,65.822989326542));
#188058=CARTESIAN_POINT('Origin',(116.959178380441,0.200000000000015,51.0204257716897));
#188059=CARTESIAN_POINT('',(121.352075836103,0.200000000000015,66.1549289168586));
#188060=CARTESIAN_POINT('',(121.416598678269,0.200000000000015,65.822989326542));
#188061=CARTESIAN_POINT('Origin',(116.959178380441,0.200000000000015,51.0204257716897));
#188062=CARTESIAN_POINT('Origin',(122.082892326988,0.200000000000015,65.0156316973241));
#188063=CARTESIAN_POINT('',(121.963100880324,0.700000000000015,65.6319021899793));
#188064=CARTESIAN_POINT('',(121.897206493045,0.700000000000015,65.9708977330055));
#188065=CARTESIAN_POINT('',(121.963100880324,0.700000000000015,65.6319021899793));
#188066=CARTESIAN_POINT('Origin',(124.517706319704,1.45439216225896E-14,
52.4896621010082));
#188067=CARTESIAN_POINT('Origin',(124.517706319704,1.45439216225896E-14,
52.4896621010082));
#188068=CARTESIAN_POINT('Origin',(122.082892326988,0.700000000000015,65.0156316973241));
#188069=CARTESIAN_POINT('',(121.419738870565,0.700000000000015,65.8068345182705));
#188070=CARTESIAN_POINT('',(121.355140191661,0.700000000000015,66.1391642528341));
#188071=CARTESIAN_POINT('',(121.419738870565,0.700000000000015,65.8068345182705));
#188072=CARTESIAN_POINT('Origin',(116.959178380441,0.700000000000015,51.0204257716897));
#188073=CARTESIAN_POINT('Origin',(116.959178380441,0.700000000000015,51.0204257716897));
#188074=CARTESIAN_POINT('Origin',(121.592078824439,0.700000000000015,64.9202267408748));
#188075=CARTESIAN_POINT('Origin',(124.026892817154,1.45439216225896E-14,
52.3942571445589));
#188076=CARTESIAN_POINT('Origin',(124.026892817154,1.45439216225896E-14,
52.3942571445589));
#188077=CARTESIAN_POINT('Origin',(108.830927758152,0.200000000000015,62.4396978731943));
#188078=CARTESIAN_POINT('',(108.985574283718,0.200000000000015,64.264523370831));
#188079=CARTESIAN_POINT('',(108.924710285017,0.200000000000015,64.5776399372382));
#188080=CARTESIAN_POINT('',(108.985574283718,0.200000000000015,64.264523370831));
#188081=CARTESIAN_POINT('',(108.53146510291,0.200000000000015,63.9802919908596));
#188082=CARTESIAN_POINT('Origin',(116.959178380441,0.200000000000015,51.0204257716897));
#188083=CARTESIAN_POINT('',(108.469801984318,0.200000000000015,64.2975196521962));
#188084=CARTESIAN_POINT('',(108.53146510291,0.200000000000015,63.9802919908596));
#188085=CARTESIAN_POINT('Origin',(116.959178380441,0.200000000000015,51.0204257716897));
#188086=CARTESIAN_POINT('Origin',(109.321741260701,0.200000000000015,62.5351028296435));
#188087=CARTESIAN_POINT('',(108.988532178342,0.700000000000015,64.2493063981041));
#188088=CARTESIAN_POINT('',(108.927604540738,0.700000000000015,64.5627503566519));
#188089=CARTESIAN_POINT('',(108.988532178342,0.700000000000015,64.2493063981041));
#188090=CARTESIAN_POINT('Origin',(111.756555253416,1.45439216225896E-14,
50.0091332333276));
#188091=CARTESIAN_POINT('Origin',(111.756555253416,1.45439216225896E-14,
50.0091332333276));
#188092=CARTESIAN_POINT('Origin',(109.321741260701,0.700000000000015,62.5351028296435));
#188093=CARTESIAN_POINT('',(108.534462746944,0.700000000000015,63.9648705261644));
#188094=CARTESIAN_POINT('',(108.472733446567,0.700000000000015,64.2824386615687));
#188095=CARTESIAN_POINT('',(108.534462746944,0.700000000000015,63.9648705261644));
#188096=CARTESIAN_POINT('Origin',(116.959178380441,0.700000000000015,51.0204257716897));
#188097=CARTESIAN_POINT('Origin',(116.959178380441,0.700000000000015,51.0204257716897));
#188098=CARTESIAN_POINT('Origin',(108.830927758152,0.700000000000015,62.4396978731943));
#188099=CARTESIAN_POINT('Origin',(111.265741750867,1.45439216225896E-14,
49.9137282768784));
#188100=CARTESIAN_POINT('Origin',(111.265741750867,1.45439216225896E-14,
49.9137282768784));
#188101=CARTESIAN_POINT('Origin',(108.830927758152,1.2,62.4396978731943));
#188102=CARTESIAN_POINT('',(108.994787025916,1.2,64.217128157474));
#188103=CARTESIAN_POINT('',(108.933724381216,1.2,64.5312666638533));
#188104=CARTESIAN_POINT('',(108.994787025916,1.2,64.217128157474));
#188105=CARTESIAN_POINT('',(108.540801935833,1.2,63.932258389249));
#188106=CARTESIAN_POINT('Origin',(116.959178380441,1.2,51.0204257716897));
#188107=CARTESIAN_POINT('',(108.478932215543,1.2,64.2505489188773));
#188108=CARTESIAN_POINT('',(108.540801935833,1.2,63.932258389249));
#188109=CARTESIAN_POINT('Origin',(116.959178380441,1.2,51.0204257716897));
#188110=CARTESIAN_POINT('Origin',(109.321741260701,1.2,62.5351028296435));
#188111=CARTESIAN_POINT('',(109.004361305076,1.7,64.1678730069675));
#188112=CARTESIAN_POINT('',(108.943090855225,1.7,64.4830805728385));
#188113=CARTESIAN_POINT('',(109.004361305076,1.7,64.1678730069675));
#188114=CARTESIAN_POINT('Origin',(111.756555253416,1.45439216225896E-14,
50.0091332333276));
#188115=CARTESIAN_POINT('Origin',(111.756555253416,1.45439216225896E-14,
50.0091332333276));
#188116=CARTESIAN_POINT('Origin',(109.321741260701,1.7,62.5351028296435));
#188117=CARTESIAN_POINT('',(108.550506073729,1.7,63.8823351767978));
#188118=CARTESIAN_POINT('',(108.488420168295,1.7,64.2017378770224));
#188119=CARTESIAN_POINT('',(108.550506073729,1.7,63.8823351767978));
#188120=CARTESIAN_POINT('Origin',(116.959178380441,1.7,51.0204257716897));
#188121=CARTESIAN_POINT('Origin',(116.959178380441,1.7,51.0204257716897));
#188122=CARTESIAN_POINT('Origin',(108.830927758152,1.7,62.4396978731943));
#188123=CARTESIAN_POINT('Origin',(111.265741750867,1.45439216225896E-14,
49.9137282768784));
#188124=CARTESIAN_POINT('Origin',(111.265741750867,1.45439216225896E-14,
49.9137282768784));
#188125=CARTESIAN_POINT('Origin',(108.830927758152,2.2,62.4396978731943));
#188126=CARTESIAN_POINT('',(109.017289821827,2.2,64.1013618861081));
#188127=CARTESIAN_POINT('',(108.955736534662,2.2,64.4180245165501));
#188128=CARTESIAN_POINT('',(109.017289821827,2.2,64.1013618861081));
#188129=CARTESIAN_POINT('',(108.563611413924,2.2,63.814914382713));
#188130=CARTESIAN_POINT('Origin',(116.959178380441,2.2,51.0204257716897));
#188131=CARTESIAN_POINT('',(108.501231170594,2.2,64.1358313125929));
#188132=CARTESIAN_POINT('',(108.563611413924,2.2,63.814914382713));
#188133=CARTESIAN_POINT('Origin',(116.959178380441,2.2,51.0204257716897));
#188134=CARTESIAN_POINT('Origin',(109.321741260701,2.2,62.5351028296435));
#188135=CARTESIAN_POINT('',(109.03362035359,2.7,64.0173490025909));
#188136=CARTESIAN_POINT('',(108.971706090658,2.7,64.3358686830996));
#188137=CARTESIAN_POINT('',(109.03362035359,2.7,64.0173490025909));
#188138=CARTESIAN_POINT('Origin',(111.756555253416,1.45439216225896E-14,
50.0091332333276));
#188139=CARTESIAN_POINT('Origin',(111.756555253416,1.45439216225896E-14,
50.0091332333276));
#188140=CARTESIAN_POINT('Origin',(109.321741260701,2.7,62.5351028296435));
#188141=CARTESIAN_POINT('',(108.580167748568,2.7,63.7297398498768));
#188142=CARTESIAN_POINT('',(108.517411692007,2.7,64.0525901615711));
#188143=CARTESIAN_POINT('',(108.580167748568,2.7,63.7297398498768));
#188144=CARTESIAN_POINT('Origin',(116.959178380441,2.7,51.0204257716897));
#188145=CARTESIAN_POINT('Origin',(116.959178380441,2.7,51.0204257716897));
#188146=CARTESIAN_POINT('Origin',(108.830927758152,2.7,62.4396978731943));
#188147=CARTESIAN_POINT('Origin',(111.265741750867,1.45439216225896E-14,
49.9137282768784));
#188148=CARTESIAN_POINT('Origin',(111.265741750867,1.45439216225896E-14,
49.9137282768784));
#188149=CARTESIAN_POINT('Origin',(108.830927758152,3.2,62.4396978731943));
#188150=CARTESIAN_POINT('',(109.053414557622,3.2,63.9155171589135));
#188151=CARTESIAN_POINT('',(108.991057104461,3.2,64.2363168441179));
#188152=CARTESIAN_POINT('',(109.053414557622,3.2,63.9155171589135));
#188153=CARTESIAN_POINT('',(108.60023938276,3.2,63.6264807588764));
#188154=CARTESIAN_POINT('Origin',(116.959178380441,3.2,51.0204257716897));
#188155=CARTESIAN_POINT('',(108.537021672699,3.2,63.9517060600868));
#188156=CARTESIAN_POINT('',(108.60023938276,3.2,63.6264807588764));
#188157=CARTESIAN_POINT('Origin',(116.959178380441,3.2,51.0204257716897));
#188158=CARTESIAN_POINT('Origin',(109.321741260701,3.2,62.5351028296435));
#188159=CARTESIAN_POINT('',(109.076749185361,3.7,63.7954715051251));
#188160=CARTESIAN_POINT('',(109.013861148526,3.7,64.1190007930822));
#188161=CARTESIAN_POINT('',(109.076749185361,3.7,63.7954715051251));
#188162=CARTESIAN_POINT('Origin',(111.756555253416,1.45439216225896E-14,
50.0091332333276));
#188163=CARTESIAN_POINT('Origin',(111.756555253416,1.45439216225896E-14,
50.0091332333276));
#188164=CARTESIAN_POINT('Origin',(109.321741260701,3.7,62.5351028296435));
#188165=CARTESIAN_POINT('',(108.623906438908,3.7,63.5047249177198));
#188166=CARTESIAN_POINT('',(108.560135680847,3.7,63.8327953900438));
#188167=CARTESIAN_POINT('',(108.623906438908,3.7,63.5047249177198));
#188168=CARTESIAN_POINT('Origin',(116.959178380441,3.7,51.0204257716897));
#188169=CARTESIAN_POINT('Origin',(116.959178380441,3.7,51.0204257716897));
#188170=CARTESIAN_POINT('Origin',(108.830927758152,3.7,62.4396978731943));
#188171=CARTESIAN_POINT('Origin',(111.265741750867,1.45439216225896E-14,
49.9137282768784));
#188172=CARTESIAN_POINT('Origin',(111.265741750867,1.45439216225896E-14,
49.9137282768784));
#188173=CARTESIAN_POINT('Origin',(108.830927758152,4.2,62.4396978731943));
#188174=CARTESIAN_POINT('',(109.103717660933,4.2,63.6567314181698));
#188175=CARTESIAN_POINT('',(109.040205187114,4.2,63.9834731398894));
#188176=CARTESIAN_POINT('',(109.103717660933,4.2,63.6567314181698));
#188177=CARTESIAN_POINT('',(108.651266555877,4.2,63.3639700204965));
#188178=CARTESIAN_POINT('Origin',(116.959178380441,4.2,51.0204257716897));
#188179=CARTESIAN_POINT('',(108.586844415053,4.2,63.695391549907));
#188180=CARTESIAN_POINT('',(108.651266555877,4.2,63.3639700204965));
#188181=CARTESIAN_POINT('Origin',(116.959178380441,4.2,51.0204257716897));
#188182=CARTESIAN_POINT('Origin',(109.321741260701,4.2,62.5351028296435));
#188183=CARTESIAN_POINT('',(109.134432104066,4.7,63.4987200949224));
#188184=CARTESIAN_POINT('',(109.070193363986,4.7,63.8291981140025));
#188185=CARTESIAN_POINT('',(109.134432104066,4.7,63.4987200949224));
#188186=CARTESIAN_POINT('Origin',(111.756555253416,1.45439216225896E-14,
50.0091332333276));
#188187=CARTESIAN_POINT('Origin',(111.756555253416,1.45439216225896E-14,
50.0091332333276));
#188188=CARTESIAN_POINT('Origin',(109.321741260701,4.7,62.5351028296435));
#188189=CARTESIAN_POINT('',(108.682437072072,4.7,63.2036124164553));
#188190=CARTESIAN_POINT('',(108.617256626478,4.7,63.5389350662436));
#188191=CARTESIAN_POINT('',(108.682437072072,4.7,63.2036124164553));
#188192=CARTESIAN_POINT('Origin',(116.959178380441,4.7,51.0204257716897));
#188193=CARTESIAN_POINT('Origin',(116.959178380441,4.7,51.0204257716897));
#188194=CARTESIAN_POINT('Origin',(108.830927758152,4.7,62.4396978731943));
#188195=CARTESIAN_POINT('Origin',(111.265741750867,1.45439216225896E-14,
49.9137282768784));
#188196=CARTESIAN_POINT('Origin',(111.265741750867,1.45439216225896E-14,
49.9137282768784));
#188197=CARTESIAN_POINT('Origin',(108.830927758152,5.2,62.4396978731943));
#188198=CARTESIAN_POINT('',(109.169025907263,5.2,63.3207512938729));
#188199=CARTESIAN_POINT('',(109.10394926914,5.2,63.6555399031828));
#188200=CARTESIAN_POINT('',(109.169025907263,5.2,63.3207512938729));
#188201=CARTESIAN_POINT('',(108.717557815134,5.2,63.0229327583325));
#188202=CARTESIAN_POINT('Origin',(116.959178380441,5.2,51.0204257716897));
#188203=CARTESIAN_POINT('',(108.651501562792,5.2,63.3627610207596));
#188204=CARTESIAN_POINT('',(108.717557815134,5.2,63.0229327583325));
#188205=CARTESIAN_POINT('Origin',(116.959178380441,5.2,51.0204257716897));
#188206=CARTESIAN_POINT('Origin',(109.321741260701,5.2,62.5351028296435));
#188207=CARTESIAN_POINT('',(109.207657018372,5.7,63.122012447834));
#188208=CARTESIAN_POINT('',(109.141618809976,5.7,63.4617478826739));
#188209=CARTESIAN_POINT('',(109.207657018372,5.7,63.122012447834));
#188210=CARTESIAN_POINT('Origin',(111.756555253416,1.45439216225896E-14,
50.0091332333276));
#188211=CARTESIAN_POINT('Origin',(111.756555253416,1.45439216225896E-14,
50.0091332333276));
#188212=CARTESIAN_POINT('Origin',(109.321741260701,5.7,62.5351028296435));
#188213=CARTESIAN_POINT('',(108.756794667777,5.7,62.821077657805));
#188214=CARTESIAN_POINT('',(108.689732073798,5.7,63.166083073309));
#188215=CARTESIAN_POINT('',(108.756794667777,5.7,62.821077657805));
#188216=CARTESIAN_POINT('Origin',(116.959178380441,5.7,51.0204257716897));
#188217=CARTESIAN_POINT('Origin',(116.959178380441,5.7,51.0204257716897));
#188218=CARTESIAN_POINT('Origin',(108.830927758152,5.7,62.4396978731943));
#188219=CARTESIAN_POINT('Origin',(111.265741750867,1.45439216225896E-14,
49.9137282768784));
#188220=CARTESIAN_POINT('Origin',(111.265741750867,1.45439216225896E-14,
49.9137282768784));
#188221=CARTESIAN_POINT('Origin',(108.634602357132,6.,62.4015358906146));
#188222=CARTESIAN_POINT('',(109.031966112671,6.7,62.4787759657038));
#188223=CARTESIAN_POINT('',(108.830927758152,6.7,62.4396978731943));
#188224=CARTESIAN_POINT('',(109.031966112671,6.7,62.4787759657038));
#188225=CARTESIAN_POINT('',(108.830927758152,6.52351515672301,62.4396978731943));
#188226=CARTESIAN_POINT('',(108.830927758152,6.7,62.4396978731943));
#188227=CARTESIAN_POINT('Origin',(114.524364387726,1.45439216225896E-14,
63.5463953680056));
#188228=CARTESIAN_POINT('Origin',(108.830927758152,6.2,62.4396978731943));
#188229=CARTESIAN_POINT('',(109.250512137945,6.2,62.901543070532));
#188230=CARTESIAN_POINT('',(109.183373859264,6.2,63.2469378481324));
#188231=CARTESIAN_POINT('',(109.250512137945,6.2,62.901543070532));
#188232=CARTESIAN_POINT('',(108.800344146074,6.2,62.5970361323712));
#188233=CARTESIAN_POINT('Origin',(116.959178380441,6.2,51.0204257716897));
#188234=CARTESIAN_POINT('',(108.732128571959,6.2,62.9479730868615));
#188235=CARTESIAN_POINT('',(108.800344146074,6.2,62.5970361323712));
#188236=CARTESIAN_POINT('Origin',(116.959178380441,6.2,51.0204257716897));
#188237=CARTESIAN_POINT('Origin',(109.321741260701,6.2,62.5351028296435));
#188238=CARTESIAN_POINT('',(109.297812125485,6.7,62.6582069439925));
#188239=CARTESIAN_POINT('',(109.229416919299,6.7,63.0100680207669));
#188240=CARTESIAN_POINT('',(109.297812125485,6.7,62.6582069439925));
#188241=CARTESIAN_POINT('Origin',(111.756555253416,1.45439216225896E-14,
50.0091332333276));
#188242=CARTESIAN_POINT('Origin',(111.756555253416,1.45439216225896E-14,
50.0091332333276));
#188243=CARTESIAN_POINT('Origin',(109.321741260701,6.7,62.5351028296435));
#188244=CARTESIAN_POINT('',(108.77890411787,6.7,62.7073349651492));
#188245=CARTESIAN_POINT('',(108.830927758152,6.7,62.4396978731943));
#188246=CARTESIAN_POINT('Origin',(116.959178380441,6.7,51.0204257716897));
#188247=CARTESIAN_POINT('Origin',(116.959178380441,6.7,51.0204257716897));
#188248=CARTESIAN_POINT('Origin',(108.830927758152,6.7,62.4396978731943));
#188249=CARTESIAN_POINT('Origin',(111.265741750867,1.45439216225896E-14,
49.9137282768784));
#188250=CARTESIAN_POINT('Origin',(111.265741750867,1.45439216225896E-14,
49.9137282768784));
#188251=CARTESIAN_POINT('Origin',(109.812554763251,6.2,62.6305077860928));
#188252=CARTESIAN_POINT('',(110.163347709257,6.2,63.4462524643294));
#188253=CARTESIAN_POINT('',(110.09795814934,6.2,63.78265090868));
#188254=CARTESIAN_POINT('',(110.163347709257,6.2,63.4462524643294));
#188255=CARTESIAN_POINT('',(109.704906439227,6.2,63.1843076401468));
#188256=CARTESIAN_POINT('Origin',(116.959178380441,6.2,51.0204257716897));
#188257=CARTESIAN_POINT('',(109.638705300736,6.2,63.5248812734762));
#188258=CARTESIAN_POINT('',(109.704906439227,6.2,63.1843076401468));
#188259=CARTESIAN_POINT('Origin',(116.959178380441,6.2,51.0204257716897));
#188260=CARTESIAN_POINT('Origin',(110.3033682658,6.2,62.725912742542));
#188261=CARTESIAN_POINT('',(110.209360669591,6.7,63.2095374857282));
#188262=CARTESIAN_POINT('',(110.142811568378,6.7,63.5519012231441));
#188263=CARTESIAN_POINT('',(110.209360669591,6.7,63.2095374857282));
#188264=CARTESIAN_POINT('Origin',(112.738182258515,1.45439216225896E-14,
50.1999431462261));
#188265=CARTESIAN_POINT('Origin',(112.738182258515,1.45439216225896E-14,
50.1999431462261));
#188266=CARTESIAN_POINT('Origin',(110.3033682658,6.7,62.725912742542));
#188267=CARTESIAN_POINT('',(109.751516135199,6.7,62.9445227381437));
#188268=CARTESIAN_POINT('',(109.684110927497,6.7,63.2912907396567));
#188269=CARTESIAN_POINT('',(109.751516135199,6.7,62.9445227381437));
#188270=CARTESIAN_POINT('Origin',(116.959178380441,6.7,51.0204257716897));
#188271=CARTESIAN_POINT('Origin',(116.959178380441,6.7,51.0204257716897));
#188272=CARTESIAN_POINT('Origin',(109.812554763251,6.7,62.6305077860928));
#188273=CARTESIAN_POINT('Origin',(112.247368755966,1.45439216225896E-14,
50.1045381897769));
#188274=CARTESIAN_POINT('Origin',(112.247368755966,1.45439216225896E-14,
50.1045381897769));
#188275=CARTESIAN_POINT('Origin',(110.79418176835,6.2,62.8213176989913));
#188276=CARTESIAN_POINT('',(111.091791575357,6.2,63.9106645431981));
#188277=CARTESIAN_POINT('',(111.027693485939,6.2,64.2404189809629));
#188278=CARTESIAN_POINT('',(111.091791575357,6.2,63.9106645431981));
#188279=CARTESIAN_POINT('',(110.625684971198,6.2,63.6881542477025));
#188280=CARTESIAN_POINT('Origin',(116.959178380441,6.2,51.0204257716897));
#188281=CARTESIAN_POINT('',(110.560993238717,6.2,64.0209626990318));
#188282=CARTESIAN_POINT('',(110.625684971198,6.2,63.6881542477025));
#188283=CARTESIAN_POINT('Origin',(116.959178380441,6.2,51.0204257716897));
#188284=CARTESIAN_POINT('Origin',(111.284995270899,6.2,62.9167226554405));
#188285=CARTESIAN_POINT('',(111.136856952335,6.7,63.6788244340304));
#188286=CARTESIAN_POINT('',(111.071667833675,6.7,64.0141917026534));
#188287=CARTESIAN_POINT('',(111.136856952335,6.7,63.6788244340304));
#188288=CARTESIAN_POINT('Origin',(113.719809263614,1.45439216225896E-14,
50.3907530591246));
#188289=CARTESIAN_POINT('Origin',(113.719809263614,1.45439216225896E-14,
50.3907530591246));
#188290=CARTESIAN_POINT('Origin',(111.284995270899,6.7,62.9167226554405));
#188291=CARTESIAN_POINT('',(110.671185615415,6.7,63.4540748938883));
#188292=CARTESIAN_POINT('',(110.605371715626,6.7,63.7926563667364));
#188293=CARTESIAN_POINT('',(110.671185615415,6.7,63.4540748938883));
#188294=CARTESIAN_POINT('Origin',(116.959178380441,6.7,51.0204257716897));
#188295=CARTESIAN_POINT('Origin',(116.959178380441,6.7,51.0204257716897));
#188296=CARTESIAN_POINT('Origin',(110.79418176835,6.7,62.8213176989913));
#188297=CARTESIAN_POINT('Origin',(113.228995761065,1.45439216225896E-14,
50.2953481026754));
#188298=CARTESIAN_POINT('Origin',(113.228995761065,1.45439216225896E-14,
50.2953481026754));
#188299=CARTESIAN_POINT('Origin',(111.775808773449,6.2,63.0121276118898));
#188300=CARTESIAN_POINT('',(112.034909663219,6.2,64.2995846722948));
#188301=CARTESIAN_POINT('',(111.97171567341,6.2,64.6246879439969));
#188302=CARTESIAN_POINT('',(112.034909663219,6.2,64.2995846722948));
#188303=CARTESIAN_POINT('',(111.561562053474,6.2,64.114325935268));
#188304=CARTESIAN_POINT('Origin',(116.959178380441,6.2,51.0204257716897));
#188305=CARTESIAN_POINT('',(111.497961148835,6.2,64.4415225918465));
#188306=CARTESIAN_POINT('',(111.561562053474,6.2,64.114325935268));
#188307=CARTESIAN_POINT('Origin',(116.959178380441,6.2,51.0204257716897));
#188308=CARTESIAN_POINT('Origin',(112.266622275998,6.2,63.107532568339));
#188309=CARTESIAN_POINT('',(112.079313119363,6.7,64.0711498336179));
#188310=CARTESIAN_POINT('',(112.015074379284,6.7,64.401627852698));
#188311=CARTESIAN_POINT('',(112.079313119363,6.7,64.0711498336179));
#188312=CARTESIAN_POINT('Origin',(114.701436268713,1.45439216225896E-14,
50.5815629720231));
#188313=CARTESIAN_POINT('Origin',(114.701436268713,1.45439216225896E-14,
50.5815629720231));
#188314=CARTESIAN_POINT('Origin',(112.266622275998,6.7,63.107532568339));
#188315=CARTESIAN_POINT('',(111.606263280211,6.7,63.8843592073384));
#188316=CARTESIAN_POINT('',(111.54159696586,6.7,64.2170368943773));
#188317=CARTESIAN_POINT('',(111.606263280211,6.7,63.8843592073384));
#188318=CARTESIAN_POINT('Origin',(116.959178380441,6.7,51.0204257716897));
#188319=CARTESIAN_POINT('Origin',(116.959178380441,6.7,51.0204257716897));
#188320=CARTESIAN_POINT('Origin',(111.775808773449,6.7,63.0121276118898));
#188321=CARTESIAN_POINT('Origin',(114.210622766164,1.45439216225896E-14,
50.4861580155739));
#188322=CARTESIAN_POINT('Origin',(114.210622766164,1.45439216225896E-14,
50.4861580155739));
#188323=CARTESIAN_POINT('Origin',(112.757435778548,6.2,63.2029375247883));
#188324=CARTESIAN_POINT('',(112.992071921149,6.2,64.6162541704145));
#188325=CARTESIAN_POINT('',(112.929439325135,6.2,64.9384693358256));
#188326=CARTESIAN_POINT('',(112.992071921149,6.2,64.6162541704145));
#188327=CARTESIAN_POINT('',(112.511764478508,6.2,64.4668004909896));
#188328=CARTESIAN_POINT('Origin',(116.959178380441,6.2,51.0204257716897));
#188329=CARTESIAN_POINT('',(112.448892012004,6.2,64.7902496769364));
#188330=CARTESIAN_POINT('',(112.511764478508,6.2,64.4668004909896));
#188331=CARTESIAN_POINT('Origin',(116.959178380441,6.2,51.0204257716897));
#188332=CARTESIAN_POINT('Origin',(113.248249281097,6.2,63.2983424812375));
#188333=CARTESIAN_POINT('',(113.036064948792,6.7,64.3899307927943));
#188334=CARTESIAN_POINT('',(112.972415653174,6.7,64.7173763981386));
#188335=CARTESIAN_POINT('',(113.036064948792,6.7,64.3899307927943));
#188336=CARTESIAN_POINT('Origin',(115.683063273812,1.45439216225896E-14,
50.7723728849216));
#188337=CARTESIAN_POINT('Origin',(115.683063273812,1.45439216225896E-14,
50.7723728849216));
#188338=CARTESIAN_POINT('Origin',(113.248249281097,6.7,63.2983424812375));
#188339=CARTESIAN_POINT('',(112.555932818159,6.7,64.2395752157784));
#188340=CARTESIAN_POINT('',(112.492031730466,6.7,64.5683161725848));
#188341=CARTESIAN_POINT('',(112.555932818159,6.7,64.2395752157784));
#188342=CARTESIAN_POINT('Origin',(116.959178380441,6.7,51.0204257716897));
#188343=CARTESIAN_POINT('Origin',(116.959178380441,6.7,51.0204257716897));
#188344=CARTESIAN_POINT('Origin',(112.757435778548,6.7,63.2029375247883));
#188345=CARTESIAN_POINT('Origin',(115.192249771263,1.45439216225896E-14,
50.6769679284724));
#188346=CARTESIAN_POINT('Origin',(115.192249771263,1.45439216225896E-14,
50.6769679284724));
#188347=CARTESIAN_POINT('Origin',(113.739062783647,6.2,63.3937474376868));
#188348=CARTESIAN_POINT('',(113.962896812214,6.2,64.862635865129));
#188349=CARTESIAN_POINT('',(113.900508966606,6.2,65.1835919051392));
#188350=CARTESIAN_POINT('',(113.962896812214,6.2,64.862635865129));
#188351=CARTESIAN_POINT('',(113.475791658336,6.2,64.7481532038329));
#188352=CARTESIAN_POINT('Origin',(116.959178380441,6.2,51.0204257716897));
#188353=CARTESIAN_POINT('',(113.413320003765,6.2,65.0695404014283));
#188354=CARTESIAN_POINT('',(113.475791658336,6.2,64.7481532038329));
#188355=CARTESIAN_POINT('Origin',(116.959178380441,6.2,51.0204257716897));
#188356=CARTESIAN_POINT('Origin',(114.229876286196,6.2,63.489152394136));
#188357=CARTESIAN_POINT('',(114.006711044749,6.7,64.6372323040136));
#188358=CARTESIAN_POINT('',(113.943318565996,6.7,64.9633567077106));
#188359=CARTESIAN_POINT('',(114.006711044749,6.7,64.6372323040136));
#188360=CARTESIAN_POINT('Origin',(116.664690278911,1.45439216225896E-14,
50.9631827978201));
#188361=CARTESIAN_POINT('Origin',(116.664690278911,1.45439216225896E-14,
50.9631827978201));
#188362=CARTESIAN_POINT('Origin',(114.229876286196,6.7,63.489152394136));
#188363=CARTESIAN_POINT('',(113.519667105543,6.7,64.5224347220989));
#188364=CARTESIAN_POINT('',(113.456186697034,6.7,64.8490114829219));
#188365=CARTESIAN_POINT('',(113.519667105543,6.7,64.5224347220989));
#188366=CARTESIAN_POINT('Origin',(116.959178380441,6.7,51.0204257716897));
#188367=CARTESIAN_POINT('Origin',(116.959178380441,6.7,51.0204257716897));
#188368=CARTESIAN_POINT('Origin',(113.739062783647,6.7,63.3937474376868));
#188369=CARTESIAN_POINT('Origin',(116.173876776362,1.45439216225896E-14,
50.8677778413709));
#188370=CARTESIAN_POINT('Origin',(116.173876776362,1.45439216225896E-14,
50.8677778413709));
#188371=CARTESIAN_POINT('Origin',(114.720689788746,6.2,63.5845573505853));
#188372=CARTESIAN_POINT('',(114.947220292879,6.2,65.0395736830551));
#188373=CARTESIAN_POINT('',(114.884771528794,6.2,65.3608431198944));
#188374=CARTESIAN_POINT('',(114.947220292879,6.2,65.0395736830551));
#188375=CARTESIAN_POINT('',(114.453373444518,6.2,64.9597738601041));
#188376=CARTESIAN_POINT('Origin',(116.959178380441,6.2,51.0204257716897));
#188377=CARTESIAN_POINT('',(114.390993201188,6.2,65.2806907899839));
#188378=CARTESIAN_POINT('',(114.453373444518,6.2,64.9597738601041));
#188379=CARTESIAN_POINT('Origin',(116.959178380441,6.2,51.0204257716897));
#188380=CARTESIAN_POINT('Origin',(115.211503291295,6.2,63.6799623070345));
#188381=CARTESIAN_POINT('',(114.991079019732,6.7,64.8139412196562));
#188382=CARTESIAN_POINT('',(114.927622628352,6.7,65.140394423677));
#188383=CARTESIAN_POINT('',(114.991079019732,6.7,64.8139412196562));
#188384=CARTESIAN_POINT('Origin',(117.64631728401,1.45439216225896E-14,
51.1539927107186));
#188385=CARTESIAN_POINT('Origin',(117.64631728401,1.45439216225896E-14,
51.1539927107186));
#188386=CARTESIAN_POINT('Origin',(115.211503291295,6.7,63.6799623070345));
#188387=CARTESIAN_POINT('',(114.49718212478,6.7,64.734398862813));
#188388=CARTESIAN_POINT('',(114.433797621533,6.7,65.0604822362976));
#188389=CARTESIAN_POINT('',(114.49718212478,6.7,64.734398862813));
#188390=CARTESIAN_POINT('Origin',(116.959178380441,6.7,51.0204257716897));
#188391=CARTESIAN_POINT('Origin',(116.959178380441,6.7,51.0204257716897));
#188392=CARTESIAN_POINT('Origin',(114.720689788746,6.7,63.5845573505853));
#188393=CARTESIAN_POINT('Origin',(117.155503781461,1.45439216225896E-14,
51.0585877542694));
#188394=CARTESIAN_POINT('Origin',(117.155503781461,1.45439216225896E-14,
51.0585877542694));
#188395=CARTESIAN_POINT('Origin',(115.702316793845,6.2,63.7753672634838));
#188396=CARTESIAN_POINT('',(115.945083064097,6.2,65.146858236978));
#188397=CARTESIAN_POINT('',(115.882265002796,6.2,65.4700275338157));
#188398=CARTESIAN_POINT('',(115.945083064097,6.2,65.146858236978));
#188399=CARTESIAN_POINT('',(115.444448747065,6.2,65.1019767389875));
#188400=CARTESIAN_POINT('Origin',(116.959178380441,6.2,51.0204257716897));
#188401=CARTESIAN_POINT('',(115.381854583266,6.2,65.4239941887781));
#188402=CARTESIAN_POINT('',(115.444448747065,6.2,65.1019767389875));
#188403=CARTESIAN_POINT('Origin',(116.959178380441,6.2,51.0204257716897));
#188404=CARTESIAN_POINT('Origin',(116.193130296394,6.2,63.870772219933));
#188405=CARTESIAN_POINT('',(115.989211633983,6.7,64.9198375584453));
#188406=CARTESIAN_POINT('',(115.925367663769,6.7,65.2482846727662));
#188407=CARTESIAN_POINT('',(115.989211633983,6.7,64.9198375584453));
#188408=CARTESIAN_POINT('Origin',(118.62794428911,1.45439216225896E-14,
51.3448026236171));
#188409=CARTESIAN_POINT('Origin',(118.62794428911,1.45439216225896E-14,
51.3448026236171));
#188410=CARTESIAN_POINT('Origin',(116.193130296394,6.7,63.870772219933));
#188411=CARTESIAN_POINT('',(115.488413693631,6.7,64.8757978252638));
#188412=CARTESIAN_POINT('',(115.424804731494,6.7,65.2030359338696));
#188413=CARTESIAN_POINT('',(115.488413693631,6.7,64.8757978252638));
#188414=CARTESIAN_POINT('Origin',(116.959178380441,6.7,51.0204257716897));
#188415=CARTESIAN_POINT('Origin',(116.959178380441,6.7,51.0204257716897));
#188416=CARTESIAN_POINT('Origin',(115.702316793845,6.7,63.7753672634838));
#188417=CARTESIAN_POINT('Origin',(118.13713078656,1.45439216225896E-14,
51.2493976671679));
#188418=CARTESIAN_POINT('Origin',(118.13713078656,1.45439216225896E-14,
51.2493976671679));
#188419=CARTESIAN_POINT('Origin',(116.683943798944,6.2,63.9661771763823));
#188420=CARTESIAN_POINT('',(116.956733701725,6.2,65.1832107213578));
#188421=CARTESIAN_POINT('',(116.893221227906,6.2,65.5099524430775));
#188422=CARTESIAN_POINT('',(116.956733701725,6.2,65.1832107213578));
#188423=CARTESIAN_POINT('',(116.449160831798,6.2,65.1740248054003));
#188424=CARTESIAN_POINT('Origin',(116.959178380441,6.2,51.0204257716897));
#188425=CARTESIAN_POINT('',(116.386037842833,6.2,65.4987628112495));
#188426=CARTESIAN_POINT('',(116.449160831798,6.2,65.1740248054003));
#188427=CARTESIAN_POINT('Origin',(116.959178380441,6.2,51.0204257716897));
#188428=CARTESIAN_POINT('Origin',(117.174757301493,6.2,64.0615821328315));
#188429=CARTESIAN_POINT('',(117.001370196777,6.7,64.9535770074154));
#188430=CARTESIAN_POINT('',(116.936796826496,6.7,65.2857765410541));
#188431=CARTESIAN_POINT('',(117.001370196777,6.7,64.9535770074154));
#188432=CARTESIAN_POINT('Origin',(119.609571294209,1.45439216225896E-14,
51.5356125365156));
#188433=CARTESIAN_POINT('Origin',(119.609571294209,1.45439216225896E-14,
51.5356125365156));
#188434=CARTESIAN_POINT('Origin',(117.174757301493,6.7,64.0615821328315));
#188435=CARTESIAN_POINT('',(116.493512355389,6.7,64.9458571352127));
#188436=CARTESIAN_POINT('',(116.429348192645,6.7,65.2759514890787));
#188437=CARTESIAN_POINT('',(116.493512355389,6.7,64.9458571352127));
#188438=CARTESIAN_POINT('Origin',(116.959178380441,6.7,51.0204257716897));
#188439=CARTESIAN_POINT('Origin',(116.959178380441,6.7,51.0204257716897));
#188440=CARTESIAN_POINT('Origin',(116.683943798944,6.7,63.9661771763823));
#188441=CARTESIAN_POINT('Origin',(119.118757791659,1.45439216225896E-14,
51.4402075800664));
#188442=CARTESIAN_POINT('Origin',(119.118757791659,1.45439216225896E-14,
51.4402075800664));
#188443=CARTESIAN_POINT('Origin',(117.665570804043,6.2,64.1569870892808));
#188444=CARTESIAN_POINT('',(117.982648245008,6.2,65.1461821388146));
#188445=CARTESIAN_POINT('',(117.918083304325,6.2,65.4783383061452));
#188446=CARTESIAN_POINT('',(117.982648245008,6.2,65.1461821388146));
#188447=CARTESIAN_POINT('',(117.467868425555,6.2,65.1740725789575));
#188448=CARTESIAN_POINT('Origin',(116.959178380441,6.2,51.0204257716897));
#188449=CARTESIAN_POINT('',(117.403877271222,6.2,65.5032768861503));
#188450=CARTESIAN_POINT('',(117.467868425555,6.2,65.1740725789575));
#188451=CARTESIAN_POINT('Origin',(116.959178380441,6.2,51.0204257716897));
#188452=CARTESIAN_POINT('Origin',(118.156384306592,6.2,64.25239204573));
#188453=CARTESIAN_POINT('',(118.028055880648,6.7,64.9125812702591));
#188454=CARTESIAN_POINT('',(117.962375473602,6.7,65.2504759859093));
#188455=CARTESIAN_POINT('',(118.028055880648,6.7,64.9125812702591));
#188456=CARTESIAN_POINT('Origin',(120.591198299308,1.45439216225896E-14,
51.7264224494141));
#188457=CARTESIAN_POINT('Origin',(120.591198299308,1.45439216225896E-14,
51.7264224494141));
#188458=CARTESIAN_POINT('Origin',(118.156384306592,6.7,64.25239204573));
#188459=CARTESIAN_POINT('',(117.512855450604,6.7,64.9426355535102));
#188460=CARTESIAN_POINT('',(117.447778812482,6.7,65.2774241628201));
#188461=CARTESIAN_POINT('',(117.512855450604,6.7,64.9426355535102));
#188462=CARTESIAN_POINT('Origin',(116.959178380441,6.7,51.0204257716897));
#188463=CARTESIAN_POINT('Origin',(116.959178380441,6.7,51.0204257716897));
#188464=CARTESIAN_POINT('Origin',(117.665570804043,6.7,64.1569870892808));
#188465=CARTESIAN_POINT('Origin',(120.100384796758,1.45439216225896E-14,
51.6310174929649));
#188466=CARTESIAN_POINT('Origin',(120.100384796758,1.45439216225896E-14,
51.6310174929649));
#188467=CARTESIAN_POINT('Origin',(118.647197809142,6.2,64.3477970021793));
#188468=CARTESIAN_POINT('',(119.023569994761,6.2,65.0319485572271));
#188469=CARTESIAN_POINT('',(118.957540802795,6.2,65.3716376067848));
#188470=CARTESIAN_POINT('',(119.023569994761,6.2,65.0319485572271));
#188471=CARTESIAN_POINT('',(118.501174705973,6.2,65.0990169952141));
#188472=CARTESIAN_POINT('Origin',(116.959178380441,6.2,51.0204257716897));
#188473=CARTESIAN_POINT('',(118.435933476088,6.2,65.4346523515122));
#188474=CARTESIAN_POINT('',(118.501174705973,6.2,65.0990169952141));
#188475=CARTESIAN_POINT('Origin',(116.959178380441,6.2,51.0204257716897));
#188476=CARTESIAN_POINT('Origin',(119.138011311691,6.2,64.4432019586286));
#188477=CARTESIAN_POINT('',(119.07005318008,6.7,64.7928144928639));
#188478=CARTESIAN_POINT('',(119.002829448977,6.7,65.1386488828715));
#188479=CARTESIAN_POINT('',(119.07005318008,6.7,64.7928144928639));
#188480=CARTESIAN_POINT('Origin',(121.572825304407,1.45439216225896E-14,
51.9172323623126));
#188481=CARTESIAN_POINT('Origin',(121.572825304407,1.45439216225896E-14,
51.9172323623126));
#188482=CARTESIAN_POINT('Origin',(119.138011311691,6.7,64.4432019586286));
#188483=CARTESIAN_POINT('',(118.547078708453,6.7,64.8628625533834));
#188484=CARTESIAN_POINT('',(118.480685951708,6.7,65.204421972253));
#188485=CARTESIAN_POINT('',(118.547078708453,6.7,64.8628625533834));
#188486=CARTESIAN_POINT('Origin',(116.959178380441,6.7,51.0204257716897));
#188487=CARTESIAN_POINT('Origin',(116.959178380441,6.7,51.0204257716897));
#188488=CARTESIAN_POINT('Origin',(118.647197809142,6.7,64.3477970021793));
#188489=CARTESIAN_POINT('Origin',(121.082011801857,1.45439216225896E-14,
51.8218274058634));
#188490=CARTESIAN_POINT('Origin',(121.082011801857,1.45439216225896E-14,
51.8218274058634));
#188491=CARTESIAN_POINT('Origin',(119.628824814241,6.7,64.5386069150778));
#188492=CARTESIAN_POINT('',(119.549979931809,6.2,64.9442266474737));
#188493=CARTESIAN_POINT('',(119.4830397813,6.2,65.2886021490805));
#188494=CARTESIAN_POINT('',(119.549979931809,6.2,64.9442266474737));
#188495=CARTESIAN_POINT('',(119.597133868151,6.7,64.7016418854643));
#188496=CARTESIAN_POINT('Origin',(122.063638806956,1.45439216225896E-14,
52.0126373187619));
#188497=CARTESIAN_POINT('',(119.528948095297,6.7,65.0524255265237));
#188498=CARTESIAN_POINT('',(119.597133868151,6.7,64.7016418854643));
#188499=CARTESIAN_POINT('Origin',(122.063638806956,1.45439216225896E-14,
52.0126373187619));
#188500=CARTESIAN_POINT('Origin',(119.628824814241,6.2,64.5386069150778));
#188501=CARTESIAN_POINT('',(120.080577810667,6.2,64.8349597523862));
#188502=CARTESIAN_POINT('',(120.01258971947,6.2,65.1847264145575));
#188503=CARTESIAN_POINT('',(120.080577810667,6.2,64.8349597523862));
#188504=CARTESIAN_POINT('Origin',(116.959178380441,6.2,51.0204257716897));
#188505=CARTESIAN_POINT('Origin',(116.959178380441,6.2,51.0204257716897));
#188506=CARTESIAN_POINT('Origin',(120.11963831679,6.2,64.6340118715271));
#188507=CARTESIAN_POINT('',(120.11963831679,6.7,64.6340118715271));
#188508=CARTESIAN_POINT('',(120.05921061797,6.7,64.9448838808303));
#188509=CARTESIAN_POINT('',(120.11963831679,6.7,64.6340118715271));
#188510=CARTESIAN_POINT('',(120.11963831679,6.61107026131202,64.6340118715271));
#188511=CARTESIAN_POINT('',(120.11963831679,6.61107026131202,64.6340118715271));
#188512=CARTESIAN_POINT('Origin',(122.554452309506,1.45439216225896E-14,
52.1080422752111));
#188513=CARTESIAN_POINT('Origin',(122.554452309506,1.45439216225896E-14,
52.1080422752111));
#188514=CARTESIAN_POINT('Origin',(120.11963831679,6.7,64.6340118715271));
#188515=CARTESIAN_POINT('',(120.016762662781,6.7,64.6140147703074));
#188516=CARTESIAN_POINT('Origin',(116.959178380441,6.7,51.0204257716897));
#188517=CARTESIAN_POINT('',(120.11963831679,6.7,64.6340118715271));
#188518=CARTESIAN_POINT('Origin',(116.959178380441,6.7,51.0204257716897));
#188519=CARTESIAN_POINT('Origin',(119.432499413221,6.,64.5004449324981));
#188520=CARTESIAN_POINT('Origin',(114.524364387726,1.45439216225896E-14,
63.5463953680056));
#188521=CARTESIAN_POINT('Origin',(120.61045181934,5.7,64.7294168279763));
#188522=CARTESIAN_POINT('',(120.531606936909,5.2,65.1350365603722));
#188523=CARTESIAN_POINT('',(120.464666786399,5.2,65.479412061979));
#188524=CARTESIAN_POINT('',(120.531606936909,5.2,65.1350365603722));
#188525=CARTESIAN_POINT('',(120.571391313216,5.7,64.9303647088355));
#188526=CARTESIAN_POINT('Origin',(123.045265812055,1.45439216225896E-14,
52.2034472316604));
#188527=CARTESIAN_POINT('',(120.503403222019,5.7,65.2801313710067));
#188528=CARTESIAN_POINT('',(120.571391313216,5.7,64.9303647088355));
#188529=CARTESIAN_POINT('Origin',(123.045265812055,1.45439216225896E-14,
52.2034472316604));
#188530=CARTESIAN_POINT('Origin',(120.61045181934,5.2,64.7294168279763));
#188531=CARTESIAN_POINT('',(121.069574375799,5.2,64.9878567548121));
#188532=CARTESIAN_POINT('',(121.001388602946,5.2,65.3386403958715));
#188533=CARTESIAN_POINT('',(121.069574375799,5.2,64.9878567548121));
#188534=CARTESIAN_POINT('Origin',(116.959178380441,5.2,51.0204257716897));
#188535=CARTESIAN_POINT('Origin',(116.959178380441,5.2,51.0204257716897));
#188536=CARTESIAN_POINT('Origin',(121.101265321889,5.2,64.8248217844256));
#188537=CARTESIAN_POINT('',(121.101265321889,5.7,64.8248217844256));
#188538=CARTESIAN_POINT('',(121.040837623069,5.7,65.1356937937288));
#188539=CARTESIAN_POINT('',(121.101265321889,5.7,64.8248217844256));
#188540=CARTESIAN_POINT('',(121.101265321889,5.59519883471502,64.8248217844256));
#188541=CARTESIAN_POINT('',(121.101265321889,5.59519883471502,64.8248217844256));
#188542=CARTESIAN_POINT('Origin',(123.536079314605,1.45439216225896E-14,
52.2988521881097));
#188543=CARTESIAN_POINT('Origin',(123.536079314605,1.45439216225896E-14,
52.2988521881097));
#188544=CARTESIAN_POINT('Origin',(121.101265321889,5.7,64.8248217844256));
#188545=CARTESIAN_POINT('',(121.013969488837,5.7,64.8078531087324));
#188546=CARTESIAN_POINT('Origin',(116.959178380441,5.7,51.0204257716897));
#188547=CARTESIAN_POINT('',(121.101265321889,5.7,64.8248217844256));
#188548=CARTESIAN_POINT('Origin',(116.959178380441,5.7,51.0204257716897));
#188549=CARTESIAN_POINT('Origin',(120.41412641832,5.,64.6912548453966));
#188550=CARTESIAN_POINT('Origin',(114.524364387726,1.45439216225896E-14,
63.5463953680056));
#188551=CARTESIAN_POINT('Origin',(120.61045181934,4.2,64.7294168279763));
#188552=CARTESIAN_POINT('',(121.001146221201,4.2,65.3398873356296));
#188553=CARTESIAN_POINT('',(120.934753464455,4.2,65.6814467544992));
#188554=CARTESIAN_POINT('',(121.001146221201,4.2,65.3398873356296));
#188555=CARTESIAN_POINT('',(120.464428716171,4.2,65.4806368210111));
#188556=CARTESIAN_POINT('Origin',(116.959178380441,4.2,51.0204257716897));
#188557=CARTESIAN_POINT('',(120.399187486286,4.2,65.8162721773092));
#188558=CARTESIAN_POINT('',(120.464428716171,4.2,65.4806368210111));
#188559=CARTESIAN_POINT('Origin',(116.959178380441,4.2,51.0204257716897));
#188560=CARTESIAN_POINT('Origin',(121.101265321889,4.2,64.8248217844256));
#188561=CARTESIAN_POINT('',(121.033307190278,4.7,65.1744343186609));
#188562=CARTESIAN_POINT('',(120.966083459175,4.7,65.5202687086685));
#188563=CARTESIAN_POINT('',(121.033307190278,4.7,65.1744343186609));
#188564=CARTESIAN_POINT('Origin',(123.536079314605,1.45439216225896E-14,
52.2988521881097));
#188565=CARTESIAN_POINT('Origin',(123.536079314605,1.45439216225896E-14,
52.2988521881097));
#188566=CARTESIAN_POINT('Origin',(121.101265321889,4.7,64.8248217844256));
#188567=CARTESIAN_POINT('',(120.496010502409,4.7,65.3181634265749));
#188568=CARTESIAN_POINT('',(120.429981310443,4.7,65.6578524761325));
#188569=CARTESIAN_POINT('',(120.496010502409,4.7,65.3181634265749));
#188570=CARTESIAN_POINT('Origin',(116.959178380441,4.7,51.0204257716897));
#188571=CARTESIAN_POINT('Origin',(116.959178380441,4.7,51.0204257716897));
#188572=CARTESIAN_POINT('Origin',(120.61045181934,4.7,64.7294168279763));
#188573=CARTESIAN_POINT('Origin',(123.045265812055,1.45439216225896E-14,
52.2034472316604));
#188574=CARTESIAN_POINT('Origin',(123.045265812055,1.45439216225896E-14,
52.2034472316604));
#188575=CARTESIAN_POINT('Origin',(120.61045181934,3.2,64.7294168279763));
#188576=CARTESIAN_POINT('',(120.948549968451,3.2,65.6104702486549));
#188577=CARTESIAN_POINT('',(120.883473330329,3.2,65.9452588579649));
#188578=CARTESIAN_POINT('',(120.948549968451,3.2,65.6104702486549));
#188579=CARTESIAN_POINT('',(120.412749440852,3.2,65.746502317653));
#188580=CARTESIAN_POINT('Origin',(116.959178380441,3.2,51.0204257716897));
#188581=CARTESIAN_POINT('',(120.348758286519,3.2,66.0757066248458));
#188582=CARTESIAN_POINT('',(120.412749440852,3.2,65.746502317653));
#188583=CARTESIAN_POINT('Origin',(116.959178380441,3.2,51.0204257716897));
#188584=CARTESIAN_POINT('Origin',(121.101265321889,3.2,64.8248217844256));
#188585=CARTESIAN_POINT('',(120.972936895945,3.7,65.4850110089547));
#188586=CARTESIAN_POINT('',(120.907256488899,3.7,65.8229057246048));
#188587=CARTESIAN_POINT('',(120.972936895945,3.7,65.4850110089547));
#188588=CARTESIAN_POINT('Origin',(123.536079314605,1.45439216225896E-14,
52.2988521881097));
#188589=CARTESIAN_POINT('Origin',(123.536079314605,1.45439216225896E-14,
52.2988521881097));
#188590=CARTESIAN_POINT('Origin',(121.101265321889,3.7,64.8248217844256));
#188591=CARTESIAN_POINT('',(120.436715757755,3.7,65.6232069210608));
#188592=CARTESIAN_POINT('',(120.372150817072,3.7,65.9553630883915));
#188593=CARTESIAN_POINT('',(120.436715757755,3.7,65.6232069210608));
#188594=CARTESIAN_POINT('Origin',(116.959178380441,3.7,51.0204257716897));
#188595=CARTESIAN_POINT('Origin',(116.959178380441,3.7,51.0204257716897));
#188596=CARTESIAN_POINT('Origin',(120.61045181934,3.7,64.7294168279763));
#188597=CARTESIAN_POINT('Origin',(123.045265812055,1.45439216225896E-14,
52.2034472316604));
#188598=CARTESIAN_POINT('Origin',(123.045265812055,1.45439216225896E-14,
52.2034472316604));
#188599=CARTESIAN_POINT('Origin',(120.61045181934,2.2,64.7294168279763));
#188600=CARTESIAN_POINT('',(120.910833878335,2.2,65.804501743256));
#188601=CARTESIAN_POINT('',(120.846669715591,2.2,66.134596097122));
#188602=CARTESIAN_POINT('',(120.910833878335,2.2,65.804501743256));
#188603=CARTESIAN_POINT('',(120.375668852194,2.2,65.9372644569943));
#188604=CARTESIAN_POINT('Origin',(116.959178380441,2.2,51.0204257716897));
#188605=CARTESIAN_POINT('',(120.312545863229,2.2,66.2620024628435));
#188606=CARTESIAN_POINT('',(120.375668852194,2.2,65.9372644569943));
#188607=CARTESIAN_POINT('Origin',(116.959178380441,2.2,51.0204257716897));
#188608=CARTESIAN_POINT('Origin',(121.101265321889,2.2,64.8248217844256));
#188609=CARTESIAN_POINT('',(120.927878217173,2.7,65.7168166590094));
#188610=CARTESIAN_POINT('',(120.863304846892,2.7,66.0490161926481));
#188611=CARTESIAN_POINT('',(120.927878217173,2.7,65.7168166590094));
#188612=CARTESIAN_POINT('Origin',(123.536079314605,1.45439216225896E-14,
52.2988521881097));
#188613=CARTESIAN_POINT('Origin',(123.536079314605,1.45439216225896E-14,
52.2988521881097));
#188614=CARTESIAN_POINT('Origin',(121.101265321889,2.7,64.8248217844256));
#188615=CARTESIAN_POINT('',(120.392428219572,2.7,65.8510454165026));
#188616=CARTESIAN_POINT('',(120.328915745752,2.7,66.1777871382222));
#188617=CARTESIAN_POINT('',(120.392428219572,2.7,65.8510454165026));
#188618=CARTESIAN_POINT('Origin',(116.959178380441,2.7,51.0204257716897));
#188619=CARTESIAN_POINT('Origin',(116.959178380441,2.7,51.0204257716897));
#188620=CARTESIAN_POINT('Origin',(120.61045181934,2.7,64.7294168279763));
#188621=CARTESIAN_POINT('Origin',(123.045265812055,1.45439216225896E-14,
52.2034472316604));
#188622=CARTESIAN_POINT('Origin',(123.045265812055,1.45439216225896E-14,
52.2034472316604));
#188623=CARTESIAN_POINT('Origin',(120.61045181934,1.2,64.7294168279763));
#188624=CARTESIAN_POINT('',(120.887362221676,1.2,65.9252523462056));
#188625=CARTESIAN_POINT('',(120.823753259538,1.2,66.2524904548114));
#188626=CARTESIAN_POINT('',(120.887362221676,1.2,65.9252523462056));
#188627=CARTESIAN_POINT('',(120.35258377256,1.2,66.05602630348));
#188628=CARTESIAN_POINT('Origin',(116.959178380441,1.2,51.0204257716897));
#188629=CARTESIAN_POINT('',(120.289989608761,1.2,66.3780437532706));
#188630=CARTESIAN_POINT('',(120.35258377256,1.2,66.05602630348));
#188631=CARTESIAN_POINT('Origin',(116.959178380441,1.2,51.0204257716897));
#188632=CARTESIAN_POINT('Origin',(121.101265321889,1.2,64.8248217844256));
#188633=CARTESIAN_POINT('',(120.897346659478,1.7,65.8738871229378));
#188634=CARTESIAN_POINT('',(120.833502689264,1.7,66.2023342372587));
#188635=CARTESIAN_POINT('',(120.897346659478,1.7,65.8738871229378));
#188636=CARTESIAN_POINT('Origin',(123.536079314605,1.45439216225896E-14,
52.2988521881097));
#188637=CARTESIAN_POINT('Origin',(123.536079314605,1.45439216225896E-14,
52.2988521881097));
#188638=CARTESIAN_POINT('Origin',(121.101265321889,1.7,64.8248217844256));
#188639=CARTESIAN_POINT('',(120.362404587042,1.7,66.0055028450213));
#188640=CARTESIAN_POINT('',(120.299586525741,1.7,66.3286721418589));
#188641=CARTESIAN_POINT('',(120.362404587042,1.7,66.0055028450213));
#188642=CARTESIAN_POINT('Origin',(116.959178380441,1.7,51.0204257716897));
#188643=CARTESIAN_POINT('Origin',(116.959178380441,1.7,51.0204257716897));
#188644=CARTESIAN_POINT('Origin',(120.61045181934,1.7,64.7294168279763));
#188645=CARTESIAN_POINT('Origin',(123.045265812055,1.45439216225896E-14,
52.2034472316604));
#188646=CARTESIAN_POINT('Origin',(123.045265812055,1.45439216225896E-14,
52.2034472316604));
#188647=CARTESIAN_POINT('Origin',(120.61045181934,0.200000000000015,64.7294168279763));
#188648=CARTESIAN_POINT('',(120.877757657924,0.200000000000015,65.9746632966532));
#188649=CARTESIAN_POINT('',(120.814373154676,0.200000000000015,66.3007466701378));
#188650=CARTESIAN_POINT('',(120.877757657924,0.200000000000015,65.9746632966532));
#188651=CARTESIAN_POINT('',(120.343135475112,0.200000000000015,66.1046333374951));
#188652=CARTESIAN_POINT('Origin',(116.959178380441,0.200000000000015,51.0204257716897));
#188653=CARTESIAN_POINT('',(120.280755231782,0.200000000000015,66.4255502673749));
#188654=CARTESIAN_POINT('',(120.343135475112,0.200000000000015,66.1046333374951));
#188655=CARTESIAN_POINT('Origin',(116.959178380441,0.200000000000015,51.0204257716897));
#188656=CARTESIAN_POINT('Origin',(121.101265321889,0.200000000000015,64.8248217844256));
#188657=CARTESIAN_POINT('',(120.880841050326,0.700000000000015,65.9588006970472));
#188658=CARTESIAN_POINT('',(120.817384658946,0.700000000000015,66.285253901068));
#188659=CARTESIAN_POINT('',(120.880841050326,0.700000000000015,65.9588006970472));
#188660=CARTESIAN_POINT('Origin',(123.536079314605,1.45439216225896E-14,
52.2988521881097));
#188661=CARTESIAN_POINT('Origin',(123.536079314605,1.45439216225896E-14,
52.2988521881097));
#188662=CARTESIAN_POINT('Origin',(121.101265321889,0.700000000000015,64.8248217844256));
#188663=CARTESIAN_POINT('',(120.346168820923,0.700000000000015,66.0890282039968));
#188664=CARTESIAN_POINT('',(120.283720056839,0.700000000000015,66.4102976408361));
#188665=CARTESIAN_POINT('',(120.346168820923,0.700000000000015,66.0890282039968));
#188666=CARTESIAN_POINT('Origin',(116.959178380441,0.700000000000015,51.0204257716897));
#188667=CARTESIAN_POINT('Origin',(116.959178380441,0.700000000000015,51.0204257716897));
#188668=CARTESIAN_POINT('Origin',(120.61045181934,0.700000000000015,64.7294168279763));
#188669=CARTESIAN_POINT('Origin',(123.045265812055,1.45439216225896E-14,
52.2034472316604));
#188670=CARTESIAN_POINT('Origin',(123.045265812055,1.45439216225896E-14,
52.2034472316604));
#188671=CARTESIAN_POINT('Origin',(109.812554763251,0.200000000000015,62.6305077860928));
#188672=CARTESIAN_POINT('',(109.904835051783,0.200000000000015,64.7761781578189));
#188673=CARTESIAN_POINT('',(109.845282885134,0.200000000000015,65.0825459670545));
#188674=CARTESIAN_POINT('',(109.904835051783,0.200000000000015,64.7761781578189));
#188675=CARTESIAN_POINT('',(109.443407616813,0.200000000000015,64.5295957438079));
#188676=CARTESIAN_POINT('Origin',(116.959178380441,0.200000000000015,51.0204257716897));
#188677=CARTESIAN_POINT('',(109.383244376598,0.200000000000015,64.8391072383233));
#188678=CARTESIAN_POINT('',(109.443407616813,0.200000000000015,64.5295957438079));
#188679=CARTESIAN_POINT('Origin',(116.959178380441,0.200000000000015,51.0204257716897));
#188680=CARTESIAN_POINT('Origin',(110.3033682658,0.200000000000015,62.725912742542));
#188681=CARTESIAN_POINT('',(109.907727771406,0.700000000000015,64.7612964797325));
#188682=CARTESIAN_POINT('',(109.848115997298,0.700000000000015,65.0679709412246));
#188683=CARTESIAN_POINT('',(109.907727771406,0.700000000000015,64.7612964797325));
#188684=CARTESIAN_POINT('Origin',(112.738182258515,1.45439216225896E-14,
50.1999431462261));
#188685=CARTESIAN_POINT('Origin',(112.738182258515,1.45439216225896E-14,
50.1999431462261));
#188686=CARTESIAN_POINT('Origin',(110.3033682658,0.700000000000015,62.725912742542));
#188687=CARTESIAN_POINT('',(109.446330684182,0.700000000000015,64.5145579408814));
#188688=CARTESIAN_POINT('',(109.38610598051,0.700000000000015,64.8243856358901));
#188689=CARTESIAN_POINT('',(109.446330684182,0.700000000000015,64.5145579408814));
#188690=CARTESIAN_POINT('Origin',(116.959178380441,0.700000000000015,51.0204257716897));
#188691=CARTESIAN_POINT('Origin',(116.959178380441,0.700000000000015,51.0204257716897));
#188692=CARTESIAN_POINT('Origin',(109.812554763251,0.700000000000015,62.6305077860928));
#188693=CARTESIAN_POINT('Origin',(112.247368755966,1.45439216225896E-14,
50.1045381897769));
#188694=CARTESIAN_POINT('Origin',(112.247368755966,1.45439216225896E-14,
50.1045381897769));
#188695=CARTESIAN_POINT('Origin',(109.812554763251,1.2,62.6305077860928));
#188696=CARTESIAN_POINT('',(109.913844353467,1.2,64.7298295499524));
#188697=CARTESIAN_POINT('',(109.854106151249,1.2,65.0371544244425));
#188698=CARTESIAN_POINT('',(109.913844353467,1.2,64.7298295499524));
#188699=CARTESIAN_POINT('',(109.45251164372,1.2,64.4827598193477));
#188700=CARTESIAN_POINT('Origin',(116.959178380441,1.2,51.0204257716897));
#188701=CARTESIAN_POINT('',(109.392156562714,1.2,64.7932582442455));
#188702=CARTESIAN_POINT('',(109.45251164372,1.2,64.4827598193477));
#188703=CARTESIAN_POINT('Origin',(116.959178380441,1.2,51.0204257716897));
#188704=CARTESIAN_POINT('Origin',(110.3033682658,1.2,62.725912742542));
#188705=CARTESIAN_POINT('',(109.923205813012,1.7,64.6816692559874));
#188706=CARTESIAN_POINT('',(109.863273080932,1.7,64.9899948948704));
#188707=CARTESIAN_POINT('',(109.923205813012,1.7,64.6816692559874));
#188708=CARTESIAN_POINT('Origin',(112.738182258515,1.45439216225896E-14,
50.1999431462261));
#188709=CARTESIAN_POINT('Origin',(112.738182258515,1.45439216225896E-14,
50.1999431462261));
#188710=CARTESIAN_POINT('Origin',(110.3033682658,1.7,62.725912742542));
#188711=CARTESIAN_POINT('',(109.461972183711,1.7,64.4340898032213));
#188712=CARTESIAN_POINT('',(109.401416462735,1.7,64.7456204261326));
#188713=CARTESIAN_POINT('',(109.461972183711,1.7,64.4340898032213));
#188714=CARTESIAN_POINT('Origin',(116.959178380441,1.7,51.0204257716897));
#188715=CARTESIAN_POINT('Origin',(116.959178380441,1.7,51.0204257716897));
#188716=CARTESIAN_POINT('Origin',(109.812554763251,1.7,62.6305077860928));
#188717=CARTESIAN_POINT('Origin',(112.247368755966,1.45439216225896E-14,
50.1045381897769));
#188718=CARTESIAN_POINT('Origin',(112.247368755966,1.45439216225896E-14,
50.1045381897769));
#188719=CARTESIAN_POINT('Origin',(109.812554763251,2.2,62.6305077860928));
#188720=CARTESIAN_POINT('',(109.935844669259,2.2,64.6166483017972));
#188721=CARTESIAN_POINT('',(109.875647305929,2.2,64.9263353436442));
#188722=CARTESIAN_POINT('',(109.935844669259,2.2,64.6166483017972));
#188723=CARTESIAN_POINT('',(109.474745874983,2.2,64.3683751864209));
#188724=CARTESIAN_POINT('Origin',(116.959178380441,2.2,51.0204257716897));
#188725=CARTESIAN_POINT('',(109.413917145163,2.2,64.6813103110717));
#188726=CARTESIAN_POINT('',(109.474745874983,2.2,64.3683751864209));
#188727=CARTESIAN_POINT('Origin',(116.959178380441,2.2,51.0204257716897));
#188728=CARTESIAN_POINT('Origin',(110.3033682658,2.2,62.725912742542));
#188729=CARTESIAN_POINT('',(109.95180552014,2.7,64.5345372520554));
#188730=CARTESIAN_POINT('',(109.89127064788,2.7,64.8459606181596));
#188731=CARTESIAN_POINT('',(109.95180552014,2.7,64.5345372520554));
#188732=CARTESIAN_POINT('Origin',(112.738182258515,1.45439216225896E-14,
50.1999431462261));
#188733=CARTESIAN_POINT('Origin',(112.738182258515,1.45439216225896E-14,
50.1999431462261));
#188734=CARTESIAN_POINT('Origin',(110.3033682658,2.7,62.725912742542));
#188735=CARTESIAN_POINT('',(109.490878776999,2.7,64.2853790147403));
#188736=CARTESIAN_POINT('',(109.429701743214,2.7,64.6001059990095));
#188737=CARTESIAN_POINT('',(109.490878776999,2.7,64.2853790147403));
#188738=CARTESIAN_POINT('Origin',(116.959178380441,2.7,51.0204257716897));
#188739=CARTESIAN_POINT('Origin',(116.959178380441,2.7,51.0204257716897));
#188740=CARTESIAN_POINT('Origin',(109.812554763251,2.7,62.6305077860928));
#188741=CARTESIAN_POINT('Origin',(112.247368755966,1.45439216225896E-14,
50.1045381897769));
#188742=CARTESIAN_POINT('Origin',(112.247368755966,1.45439216225896E-14,
50.1045381897769));
#188743=CARTESIAN_POINT('Origin',(109.812554763251,3.2,62.6305077860928));
#188744=CARTESIAN_POINT('',(109.971145850964,3.2,64.4350403719647));
#188745=CARTESIAN_POINT('',(109.910196955985,3.2,64.7485936896801));
#188746=CARTESIAN_POINT('',(109.971145850964,3.2,64.4350403719647));
#188747=CARTESIAN_POINT('',(109.510430291786,3.2,64.184795692762));
#188748=CARTESIAN_POINT('Origin',(116.959178380441,3.2,51.0204257716897));
#188749=CARTESIAN_POINT('',(109.448825823059,3.2,64.5017216282059));
#188750=CARTESIAN_POINT('',(109.510430291786,3.2,64.184795692762));
#188751=CARTESIAN_POINT('Origin',(116.959178380441,3.2,51.0204257716897));
#188752=CARTESIAN_POINT('Origin',(110.3033682658,3.2,62.725912742542));
#188753=CARTESIAN_POINT('',(109.993937112423,3.7,64.317790081408));
#188754=CARTESIAN_POINT('',(109.932493071797,3.7,64.6338906899368));
#188755=CARTESIAN_POINT('',(109.993937112423,3.7,64.317790081408));
#188756=CARTESIAN_POINT('Origin',(112.738182258515,1.45439216225896E-14,
50.1999431462261));
#188757=CARTESIAN_POINT('Origin',(112.738182258515,1.45439216225896E-14,
50.1999431462261));
#188758=CARTESIAN_POINT('Origin',(110.3033682658,3.7,62.725912742542));
#188759=CARTESIAN_POINT('',(109.533474303738,3.7,64.066245120129));
#188760=CARTESIAN_POINT('',(109.471358401437,3.7,64.3858021400896));
#188761=CARTESIAN_POINT('',(109.533474303738,3.7,64.066245120129));
#188762=CARTESIAN_POINT('Origin',(116.959178380441,3.7,51.0204257716897));
#188763=CARTESIAN_POINT('Origin',(116.959178380441,3.7,51.0204257716897));
#188764=CARTESIAN_POINT('Origin',(109.812554763251,3.7,62.6305077860928));
#188765=CARTESIAN_POINT('Origin',(112.247368755966,1.45439216225896E-14,
50.1045381897769));
#188766=CARTESIAN_POINT('Origin',(112.247368755966,1.45439216225896E-14,
50.1045381897769));
#188767=CARTESIAN_POINT('Origin',(109.812554763251,4.2,62.6305077860928));
#188768=CARTESIAN_POINT('',(110.020266117139,4.2,64.182339770391));
#188769=CARTESIAN_POINT('',(109.958240075275,4.2,64.5014345007899));
#188770=CARTESIAN_POINT('',(110.020266117139,4.2,64.182339770391));
#188771=CARTESIAN_POINT('',(109.560100658523,4.2,63.9292650832573));
#188772=CARTESIAN_POINT('Origin',(116.959178380441,4.2,51.0204257716897));
#188773=CARTESIAN_POINT('',(109.497383261795,4.2,64.2519165083483));
#188774=CARTESIAN_POINT('',(109.560100658523,4.2,63.9292650832573));
#188775=CARTESIAN_POINT('Origin',(116.959178380441,4.2,51.0204257716897));
#188776=CARTESIAN_POINT('Origin',(110.3033682658,4.2,62.725912742542));
#188777=CARTESIAN_POINT('',(110.050236821974,4.7,64.0281546298999));
#188778=CARTESIAN_POINT('',(109.987534869184,4.7,64.3507266032104));
#188779=CARTESIAN_POINT('',(110.050236821974,4.7,64.0281546298999));
#188780=CARTESIAN_POINT('Origin',(112.738182258515,1.45439216225896E-14,
50.1999431462261));
#188781=CARTESIAN_POINT('Origin',(112.738182258515,1.45439216225896E-14,
50.1999431462261));
#188782=CARTESIAN_POINT('Origin',(110.3033682658,4.7,62.725912742542));
#188783=CARTESIAN_POINT('',(109.590417054145,4.7,63.7733015267161));
#188784=CARTESIAN_POINT('',(109.527000630799,4.7,64.0995491140498));
#188785=CARTESIAN_POINT('',(109.590417054145,4.7,63.7733015267161));
#188786=CARTESIAN_POINT('Origin',(116.959178380441,4.7,51.0204257716897));
#188787=CARTESIAN_POINT('Origin',(116.959178380441,4.7,51.0204257716897));
#188788=CARTESIAN_POINT('Origin',(109.812554763251,4.7,62.6305077860928));
#188789=CARTESIAN_POINT('Origin',(112.247368755966,1.45439216225896E-14,
50.1045381897769));
#188790=CARTESIAN_POINT('Origin',(112.247368755966,1.45439216225896E-14,
50.1045381897769));
#188791=CARTESIAN_POINT('Origin',(109.812554763251,5.2,62.6305077860928));
#188792=CARTESIAN_POINT('',(110.083972587697,5.2,63.8546000269541));
#188793=CARTESIAN_POINT('',(110.020492179188,5.2,64.1811767877771));
#188794=CARTESIAN_POINT('',(110.083972587697,5.2,63.8546000269541));
#188795=CARTESIAN_POINT('',(109.624551443867,5.2,63.5976961913039));
#188796=CARTESIAN_POINT('Origin',(116.959178380441,5.2,51.0204257716897));
#188797=CARTESIAN_POINT('',(109.560329299005,5.2,63.9280888358195));
#188798=CARTESIAN_POINT('',(109.624551443867,5.2,63.5976961913039));
#188799=CARTESIAN_POINT('Origin',(116.959178380441,5.2,51.0204257716897));
#188800=CARTESIAN_POINT('Origin',(110.3033682658,5.2,62.725912742542));
#188801=CARTESIAN_POINT('',(110.121619040844,5.7,63.6609267817127));
#188802=CARTESIAN_POINT('',(110.057247074165,5.7,63.9920901888077));
#188803=CARTESIAN_POINT('',(110.121619040844,5.7,63.6609267817127));
#188804=CARTESIAN_POINT('Origin',(112.738182258515,1.45439216225896E-14,
50.1999431462261));
#188805=CARTESIAN_POINT('Origin',(112.738182258515,1.45439216225896E-14,
50.1999431462261));
#188806=CARTESIAN_POINT('Origin',(110.3033682658,5.7,62.725912742542));
#188807=CARTESIAN_POINT('',(109.66265508748,5.7,63.401670916753));
#188808=CARTESIAN_POINT('',(109.597509299565,5.7,63.7368152691325));
#188809=CARTESIAN_POINT('',(109.66265508748,5.7,63.401670916753));
#188810=CARTESIAN_POINT('Origin',(116.959178380441,5.7,51.0204257716897));
#188811=CARTESIAN_POINT('Origin',(116.959178380441,5.7,51.0204257716897));
#188812=CARTESIAN_POINT('Origin',(109.812554763251,5.7,62.6305077860928));
#188813=CARTESIAN_POINT('Origin',(112.247368755966,1.45439216225896E-14,
50.1045381897769));
#188814=CARTESIAN_POINT('Origin',(112.247368755966,1.45439216225896E-14,
50.1045381897769));
#188815=CARTESIAN_POINT('Origin',(110.79418176835,5.2,62.8213176989913));
#188816=CARTESIAN_POINT('',(111.013976121973,5.2,64.3109883486827));
#188817=CARTESIAN_POINT('',(110.951679320672,5.2,64.6314760086754));
#188818=CARTESIAN_POINT('',(111.013976121973,5.2,64.3109883486827));
#188819=CARTESIAN_POINT('',(110.54715253499,5.2,64.0921665916452));
#188820=CARTESIAN_POINT('Origin',(116.959178380441,5.2,51.0204257716897));
#188821=CARTESIAN_POINT('',(110.484311174475,5.2,64.4154557519527));
#188822=CARTESIAN_POINT('',(110.54715253499,5.2,64.0921665916452));
#188823=CARTESIAN_POINT('Origin',(116.959178380441,5.2,51.0204257716897));
#188824=CARTESIAN_POINT('Origin',(111.284995270899,5.2,62.9167226554405));
#188825=CARTESIAN_POINT('',(111.050894299475,5.7,64.1210617381391));
#188826=CARTESIAN_POINT('',(110.98775555323,5.7,64.4458808077575));
#188827=CARTESIAN_POINT('',(111.050894299475,5.7,64.1210617381391));
#188828=CARTESIAN_POINT('Origin',(113.719809263614,1.45439216225896E-14,
50.3907530591246));
#188829=CARTESIAN_POINT('Origin',(113.719809263614,1.45439216225896E-14,
50.3907530591246));
#188830=CARTESIAN_POINT('Origin',(111.284995270899,5.7,62.9167226554405));
#188831=CARTESIAN_POINT('',(110.584405587776,5.7,63.900517205712));
#188832=CARTESIAN_POINT('',(110.520699696142,5.7,64.2282539708631));
#188833=CARTESIAN_POINT('',(110.584405587776,5.7,63.900517205712));
#188834=CARTESIAN_POINT('Origin',(116.959178380441,5.7,51.0204257716897));
#188835=CARTESIAN_POINT('Origin',(116.959178380441,5.7,51.0204257716897));
#188836=CARTESIAN_POINT('Origin',(110.79418176835,5.7,62.8213176989913));
#188837=CARTESIAN_POINT('Origin',(113.228995761065,1.45439216225896E-14,
50.2953481026754));
#188838=CARTESIAN_POINT('Origin',(113.228995761065,1.45439216225896E-14,
50.2953481026754));
#188839=CARTESIAN_POINT('Origin',(111.775808773449,5.2,63.0121276118898));
#188840=CARTESIAN_POINT('',(111.958186342362,5.2,64.6942899710361));
#188841=CARTESIAN_POINT('',(111.896720498972,5.2,65.0105027445071));
#188842=CARTESIAN_POINT('',(111.958186342362,5.2,64.6942899710361));
#188843=CARTESIAN_POINT('',(111.484347160118,5.2,64.5115601426693));
#188844=CARTESIAN_POINT('Origin',(116.959178380441,5.2,51.0204257716897));
#188845=CARTESIAN_POINT('',(111.422507081558,5.2,64.8296981795755));
#188846=CARTESIAN_POINT('',(111.484347160118,5.2,64.5115601426693));
#188847=CARTESIAN_POINT('Origin',(116.959178380441,5.2,51.0204257716897));
#188848=CARTESIAN_POINT('Origin',(112.266622275998,5.2,63.107532568339));
#188849=CARTESIAN_POINT('',(111.994594150334,5.7,64.5069889710055));
#188850=CARTESIAN_POINT('',(111.932320047887,5.7,64.8273598561001));
#188851=CARTESIAN_POINT('',(111.994594150334,5.7,64.5069889710055));
#188852=CARTESIAN_POINT('Origin',(114.701436268713,1.45439216225896E-14,
50.5815629720231));
#188853=CARTESIAN_POINT('Origin',(114.701436268713,1.45439216225896E-14,
50.5815629720231));
#188854=CARTESIAN_POINT('Origin',(112.266622275998,5.7,63.107532568339));
#188855=CARTESIAN_POINT('',(111.520984728148,5.7,64.3230771355044));
#188856=CARTESIAN_POINT('',(111.458321335333,5.7,64.6454507359363));
#188857=CARTESIAN_POINT('',(111.520984728148,5.7,64.3230771355044));
#188858=CARTESIAN_POINT('Origin',(116.959178380441,5.7,51.0204257716897));
#188859=CARTESIAN_POINT('Origin',(116.959178380441,5.7,51.0204257716897));
#188860=CARTESIAN_POINT('Origin',(111.775808773449,5.7,63.0121276118898));
#188861=CARTESIAN_POINT('Origin',(114.210622766164,1.45439216225896E-14,
50.4861580155739));
#188862=CARTESIAN_POINT('Origin',(114.210622766164,1.45439216225896E-14,
50.4861580155739));
#188863=CARTESIAN_POINT('Origin',(112.757435778548,5.2,63.2029375247883));
#188864=CARTESIAN_POINT('',(112.916026866261,5.2,65.0074701106602));
#188865=CARTESIAN_POINT('',(112.855077971282,5.2,65.3210234283756));
#188866=CARTESIAN_POINT('',(112.916026866261,5.2,65.0074701106602));
#188867=CARTESIAN_POINT('',(112.435429605694,5.2,64.8595074077664));
#188868=CARTESIAN_POINT('Origin',(116.959178380441,5.2,51.0204257716897));
#188869=CARTESIAN_POINT('',(112.374259740071,5.2,65.1741975152246));
#188870=CARTESIAN_POINT('',(112.435429605694,5.2,64.8595074077664));
#188871=CARTESIAN_POINT('Origin',(116.959178380441,5.2,51.0204257716897));
#188872=CARTESIAN_POINT('Origin',(113.248249281097,5.2,63.2983424812375));
#188873=CARTESIAN_POINT('',(112.952117544559,5.7,64.8218005932256));
#188874=CARTESIAN_POINT('',(112.890380877488,5.7,65.1394066267945));
#188875=CARTESIAN_POINT('',(112.952117544559,5.7,64.8218005932256));
#188876=CARTESIAN_POINT('Origin',(115.683063273812,1.45439216225896E-14,
50.7723728849216));
#188877=CARTESIAN_POINT('Origin',(115.683063273812,1.45439216225896E-14,
50.7723728849216));
#188878=CARTESIAN_POINT('Origin',(113.248249281097,5.7,63.2983424812375));
#188879=CARTESIAN_POINT('',(112.471655806575,5.7,64.6731406905662));
#188880=CARTESIAN_POINT('',(112.409689455418,5.7,64.9919283404247));
#188881=CARTESIAN_POINT('',(112.471655806575,5.7,64.6731406905662));
#188882=CARTESIAN_POINT('Origin',(116.959178380441,5.7,51.0204257716897));
#188883=CARTESIAN_POINT('Origin',(116.959178380441,5.7,51.0204257716897));
#188884=CARTESIAN_POINT('Origin',(112.757435778548,5.7,63.2029375247883));
#188885=CARTESIAN_POINT('Origin',(115.192249771263,1.45439216225896E-14,
50.6769679284724));
#188886=CARTESIAN_POINT('Origin',(115.192249771263,1.45439216225896E-14,
50.6769679284724));
#188887=CARTESIAN_POINT('Origin',(113.739062783647,5.2,63.3937474376868));
#188888=CARTESIAN_POINT('',(113.887147487649,5.2,65.2523304123455));
#188889=CARTESIAN_POINT('',(113.826424197673,5.2,65.5647230987283));
#188890=CARTESIAN_POINT('',(113.887147487649,5.2,65.2523304123455));
#188891=CARTESIAN_POINT('',(113.39994106609,5.2,65.138368725503));
#188892=CARTESIAN_POINT('Origin',(116.959178380441,5.2,51.0204257716897));
#188893=CARTESIAN_POINT('',(113.339140507264,5.2,65.4511589236753));
#188894=CARTESIAN_POINT('',(113.39994106609,5.2,65.138368725503));
#188895=CARTESIAN_POINT('Origin',(116.959178380441,5.2,51.0204257716897));
#188896=CARTESIAN_POINT('Origin',(114.229876286196,5.2,63.489152394136));
#188897=CARTESIAN_POINT('',(113.92309985496,5.7,65.0673724397024));
#188898=CARTESIAN_POINT('',(113.861597621984,5.7,65.3837724204277));
#188899=CARTESIAN_POINT('',(113.92309985496,5.7,65.0673724397024));
#188900=CARTESIAN_POINT('Origin',(116.664690278911,1.45439216225896E-14,
50.9631827978201));
#188901=CARTESIAN_POINT('Origin',(116.664690278911,1.45439216225896E-14,
50.9631827978201));
#188902=CARTESIAN_POINT('Origin',(114.229876286196,5.7,63.489152394136));
#188903=CARTESIAN_POINT('',(113.43594079827,5.7,64.9531670829504));
#188904=CARTESIAN_POINT('',(113.37435828013,5.7,65.2699800929758));
#188905=CARTESIAN_POINT('',(113.43594079827,5.7,64.9531670829504));
#188906=CARTESIAN_POINT('Origin',(116.959178380441,5.7,51.0204257716897));
#188907=CARTESIAN_POINT('Origin',(116.959178380441,5.7,51.0204257716897));
#188908=CARTESIAN_POINT('Origin',(113.739062783647,5.7,63.3937474376868));
#188909=CARTESIAN_POINT('Origin',(116.173876776362,1.45439216225896E-14,
50.8677778413709));
#188910=CARTESIAN_POINT('Origin',(116.173876776362,1.45439216225896E-14,
50.8677778413709));
#188911=CARTESIAN_POINT('Origin',(114.720689788746,5.2,63.5845573505853));
#188912=CARTESIAN_POINT('',(114.871397359373,5.2,65.429646913552));
#188913=CARTESIAN_POINT('',(114.810617903123,5.2,65.7423285489213));
#188914=CARTESIAN_POINT('',(114.871397359373,5.2,65.429646913552));
#188915=CARTESIAN_POINT('',(114.377633306,5.2,65.3494211494406));
#188916=CARTESIAN_POINT('Origin',(116.959178380441,5.2,51.0204257716897));
#188917=CARTESIAN_POINT('',(114.316917025863,5.2,65.6617777735075));
#188918=CARTESIAN_POINT('',(114.377633306,5.2,65.3494211494406));
#188919=CARTESIAN_POINT('Origin',(116.959178380441,5.2,51.0204257716897));
#188920=CARTESIAN_POINT('Origin',(115.211503291295,5.2,63.6799623070345));
#188921=CARTESIAN_POINT('',(114.907384155297,5.7,65.2445118219335));
#188922=CARTESIAN_POINT('',(114.845823564294,5.7,65.5612120271824));
#188923=CARTESIAN_POINT('',(114.907384155297,5.7,65.2445118219335));
#188924=CARTESIAN_POINT('Origin',(117.64631728401,1.45439216225896E-14,
51.1539927107186));
#188925=CARTESIAN_POINT('Origin',(117.64631728401,1.45439216225896E-14,
51.1539927107186));
#188926=CARTESIAN_POINT('Origin',(115.211503291295,5.7,63.6799623070345));
#188927=CARTESIAN_POINT('',(114.413581376678,5.7,65.1644852809468));
#188928=CARTESIAN_POINT('',(114.352086426791,5.7,65.4808477936172));
#188929=CARTESIAN_POINT('',(114.413581376678,5.7,65.1644852809468));
#188930=CARTESIAN_POINT('Origin',(116.959178380441,5.7,51.0204257716897));
#188931=CARTESIAN_POINT('Origin',(116.959178380441,5.7,51.0204257716897));
#188932=CARTESIAN_POINT('Origin',(114.720689788746,5.7,63.5845573505853));
#188933=CARTESIAN_POINT('Origin',(117.155503781461,1.45439216225896E-14,
51.0585877542694));
#188934=CARTESIAN_POINT('Origin',(117.155503781461,1.45439216225896E-14,
51.0585877542694));
#188935=CARTESIAN_POINT('Origin',(115.702316793845,5.2,63.7753672634838));
#188936=CARTESIAN_POINT('',(115.868813923706,5.2,65.5392269914383));
#188937=CARTESIAN_POINT('',(115.807694164759,5.2,65.8536593236842));
#188938=CARTESIAN_POINT('',(115.868813923706,5.2,65.5392269914383));
#188939=CARTESIAN_POINT('',(115.368450128478,5.2,65.4929537863623));
#188940=CARTESIAN_POINT('Origin',(116.959178380441,5.2,51.0204257716897));
#188941=CARTESIAN_POINT('',(115.307536650107,5.2,65.8063249023359));
#188942=CARTESIAN_POINT('',(115.368450128478,5.2,65.4929537863623));
#188943=CARTESIAN_POINT('Origin',(116.959178380441,5.2,51.0204257716897));
#188944=CARTESIAN_POINT('Origin',(116.193130296394,5.2,63.870772219933));
#188945=CARTESIAN_POINT('',(115.905009389283,5.7,65.3530183928804));
#188946=CARTESIAN_POINT('',(115.843095126351,5.7,65.6715380733892));
#188947=CARTESIAN_POINT('',(115.905009389283,5.7,65.3530183928804));
#188948=CARTESIAN_POINT('Origin',(118.62794428911,1.45439216225896E-14,
51.3448026236171));
#188949=CARTESIAN_POINT('Origin',(118.62794428911,1.45439216225896E-14,
51.3448026236171));
#188950=CARTESIAN_POINT('Origin',(116.193130296394,5.7,63.870772219933));
#188951=CARTESIAN_POINT('',(115.404519090427,5.7,65.3073959893009));
#188952=CARTESIAN_POINT('',(115.342819230478,5.7,65.6248126675899));
#188953=CARTESIAN_POINT('',(115.404519090427,5.7,65.3073959893009));
#188954=CARTESIAN_POINT('Origin',(116.959178380441,5.7,51.0204257716897));
#188955=CARTESIAN_POINT('Origin',(116.959178380441,5.7,51.0204257716897));
#188956=CARTESIAN_POINT('Origin',(115.702316793845,5.7,63.7753672634838));
#188957=CARTESIAN_POINT('Origin',(118.13713078656,1.45439216225896E-14,
51.2493976671679));
#188958=CARTESIAN_POINT('Origin',(118.13713078656,1.45439216225896E-14,
51.2493976671679));
#188959=CARTESIAN_POINT('Origin',(116.683943798944,5.2,63.9661771763823));
#188960=CARTESIAN_POINT('',(116.879625633083,5.2,65.5798953659895));
#188961=CARTESIAN_POINT('',(116.81786685009,5.2,65.8976151755468));
#188962=CARTESIAN_POINT('',(116.879625633083,5.2,65.5798953659895));
#188963=CARTESIAN_POINT('',(116.372523288069,5.2,65.5682888212799));
#188964=CARTESIAN_POINT('Origin',(116.959178380441,5.2,51.0204257716897));
#188965=CARTESIAN_POINT('',(116.311122783449,5.2,65.8841654575899));
#188966=CARTESIAN_POINT('',(116.372523288069,5.2,65.5682888212799));
#188967=CARTESIAN_POINT('Origin',(116.959178380441,5.2,51.0204257716897));
#188968=CARTESIAN_POINT('Origin',(117.174757301493,5.2,64.0615821328315));
#188969=CARTESIAN_POINT('',(116.91621327714,5.7,65.3916691941193));
#188970=CARTESIAN_POINT('',(116.853634466426,5.7,65.7136076595311));
#188971=CARTESIAN_POINT('',(116.91621327714,5.7,65.3916691941193));
#188972=CARTESIAN_POINT('Origin',(119.609571294209,1.45439216225896E-14,
51.5356125365156));
#188973=CARTESIAN_POINT('Origin',(119.609571294209,1.45439216225896E-14,
51.5356125365156));
#188974=CARTESIAN_POINT('Origin',(117.174757301493,5.7,64.0615821328315));
#188975=CARTESIAN_POINT('',(116.408890997126,5.7,65.3811941112541));
#188976=CARTESIAN_POINT('',(116.346684842631,5.7,65.7012154361843));
#188977=CARTESIAN_POINT('',(116.408890997126,5.7,65.3811941112541));
#188978=CARTESIAN_POINT('Origin',(116.959178380441,5.7,51.0204257716897));
#188979=CARTESIAN_POINT('Origin',(116.959178380441,5.7,51.0204257716897));
#188980=CARTESIAN_POINT('Origin',(116.683943798944,5.7,63.9661771763823));
#188981=CARTESIAN_POINT('Origin',(119.118757791659,1.45439216225896E-14,
51.4402075800664));
#188982=CARTESIAN_POINT('Origin',(119.118757791659,1.45439216225896E-14,
51.4402075800664));
#188983=CARTESIAN_POINT('Origin',(117.665570804043,5.2,64.1569870892808));
#188984=CARTESIAN_POINT('',(117.904268935444,5.2,65.5494067183983));
#188985=CARTESIAN_POINT('',(117.841543812465,5.2,65.8720978914024));
#188986=CARTESIAN_POINT('',(117.904268935444,5.2,65.5494067183983));
#188987=CARTESIAN_POINT('',(117.390182135468,5.2,65.5737319002038));
#188988=CARTESIAN_POINT('Origin',(116.959178380441,5.2,51.0204257716897));
#188989=CARTESIAN_POINT('',(117.327983517023,5.2,65.8937144557068));
#188990=CARTESIAN_POINT('',(117.390182135468,5.2,65.5737319002038));
#188991=CARTESIAN_POINT('Origin',(116.959178380441,5.2,51.0204257716897));
#188992=CARTESIAN_POINT('Origin',(118.156384306592,5.2,64.25239204573));
#188993=CARTESIAN_POINT('',(117.941450480778,5.7,65.3581252045768));
#188994=CARTESIAN_POINT('',(117.87786568195,5.7,65.6852390043561));
#188995=CARTESIAN_POINT('',(117.941450480778,5.7,65.3581252045768));
#188996=CARTESIAN_POINT('Origin',(120.591198299308,1.45439216225896E-14,
51.7264224494141));
#188997=CARTESIAN_POINT('Origin',(120.591198299308,1.45439216225896E-14,
51.7264224494141));
#188998=CARTESIAN_POINT('Origin',(118.156384306592,5.7,64.25239204573));
#188999=CARTESIAN_POINT('',(117.42703997039,5.7,65.3841157237722));
#189000=CARTESIAN_POINT('',(117.364003436039,5.7,65.7084089614048));
#189001=CARTESIAN_POINT('',(117.42703997039,5.7,65.3841157237722));
#189002=CARTESIAN_POINT('Origin',(116.959178380441,5.7,51.0204257716897));
#189003=CARTESIAN_POINT('Origin',(116.959178380441,5.7,51.0204257716897));
#189004=CARTESIAN_POINT('Origin',(117.665570804043,5.7,64.1569870892808));
#189005=CARTESIAN_POINT('Origin',(120.100384796758,1.45439216225896E-14,
51.6310174929649));
#189006=CARTESIAN_POINT('Origin',(120.100384796758,1.45439216225896E-14,
51.6310174929649));
#189007=CARTESIAN_POINT('Origin',(118.647197809142,5.2,64.3477970021793));
#189008=CARTESIAN_POINT('',(118.943422586228,5.2,65.44426917207));
#189009=CARTESIAN_POINT('',(118.879357457006,5.2,65.7738540451763));
#189010=CARTESIAN_POINT('',(118.943422586228,5.2,65.44426917207));
#189011=CARTESIAN_POINT('',(118.421978693774,5.2,65.5064431246532));
#189012=CARTESIAN_POINT('Origin',(116.959178380441,5.2,51.0204257716897));
#189013=CARTESIAN_POINT('',(118.358634022938,5.2,65.8323215791715));
#189014=CARTESIAN_POINT('',(118.421978693774,5.2,65.5064431246532));
#189015=CARTESIAN_POINT('Origin',(116.959178380441,5.2,51.0204257716897));
#189016=CARTESIAN_POINT('Origin',(119.138011311691,5.2,64.4432019586286));
#189017=CARTESIAN_POINT('',(118.981429396835,5.7,65.2487420576654));
#189018=CARTESIAN_POINT('',(118.916447481056,5.7,65.5830433651943));
#189019=CARTESIAN_POINT('',(118.981429396835,5.7,65.2487420576654));
#189020=CARTESIAN_POINT('Origin',(121.572825304407,1.45439216225896E-14,
51.9172323623126));
#189021=CARTESIAN_POINT('Origin',(121.572825304407,1.45439216225896E-14,
51.9172323623126));
#189022=CARTESIAN_POINT('Origin',(119.138011311691,5.7,64.4432019586286));
#189023=CARTESIAN_POINT('',(118.459541548164,5.7,65.3131999555876));
#189024=CARTESIAN_POINT('',(118.395311107302,5.7,65.6436352791055));
#189025=CARTESIAN_POINT('',(118.459541548164,5.7,65.3131999555876));
#189026=CARTESIAN_POINT('Origin',(116.959178380441,5.7,51.0204257716897));
#189027=CARTESIAN_POINT('Origin',(116.959178380441,5.7,51.0204257716897));
#189028=CARTESIAN_POINT('Origin',(118.647197809142,5.7,64.3477970021793));
#189029=CARTESIAN_POINT('Origin',(121.082011801857,1.45439216225896E-14,
51.8218274058634));
#189030=CARTESIAN_POINT('Origin',(121.082011801857,1.45439216225896E-14,
51.8218274058634));
#189031=CARTESIAN_POINT('Origin',(119.628824814241,5.2,64.5386069150778));
#189032=CARTESIAN_POINT('',(119.998065981774,5.2,65.2594441947878));
#189033=CARTESIAN_POINT('',(119.932216346204,5.2,65.5982095113747));
#189034=CARTESIAN_POINT('',(119.998065981774,5.2,65.2594441947878));
#189035=CARTESIAN_POINT('',(119.468732843108,5.2,65.3622045981111));
#189036=CARTESIAN_POINT('Origin',(116.959178380441,5.2,51.0204257716897));
#189037=CARTESIAN_POINT('',(119.403836680514,5.2,65.696064745953));
#189038=CARTESIAN_POINT('',(119.468732843108,5.2,65.3622045981111));
#189039=CARTESIAN_POINT('Origin',(116.959178380441,5.2,51.0204257716897));
#189040=CARTESIAN_POINT('Origin',(120.11963831679,5.2,64.6340118715271));
#189041=CARTESIAN_POINT('',(120.037174980321,5.7,65.0582468432809));
#189042=CARTESIAN_POINT('',(119.970328561956,5.7,65.4021401372109));
#189043=CARTESIAN_POINT('',(120.037174980321,5.7,65.0582468432809));
#189044=CARTESIAN_POINT('Origin',(122.554452309506,1.45439216225896E-14,
52.1080422752111));
#189045=CARTESIAN_POINT('Origin',(122.554452309506,1.45439216225896E-14,
52.1080422752111));
#189046=CARTESIAN_POINT('Origin',(120.11963831679,5.7,64.6340118715271));
#189047=CARTESIAN_POINT('',(119.507252479224,5.7,65.1640392383386));
#189048=CARTESIAN_POINT('',(119.441402843655,5.7,65.5028045549254));
#189049=CARTESIAN_POINT('',(119.507252479224,5.7,65.1640392383386));
#189050=CARTESIAN_POINT('Origin',(116.959178380441,5.7,51.0204257716897));
#189051=CARTESIAN_POINT('Origin',(116.959178380441,5.7,51.0204257716897));
#189052=CARTESIAN_POINT('Origin',(119.628824814241,5.7,64.5386069150778));
#189053=CARTESIAN_POINT('Origin',(122.063638806956,1.45439216225896E-14,
52.0126373187619));
#189054=CARTESIAN_POINT('Origin',(122.063638806956,1.45439216225896E-14,
52.0126373187619));
#189055=CARTESIAN_POINT('Origin',(119.628824814241,4.2,64.5386069150778));
#189056=CARTESIAN_POINT('',(119.931982055812,4.2,65.5994148249354));
#189057=CARTESIAN_POINT('',(119.867751614951,4.2,65.9298501484533));
#189058=CARTESIAN_POINT('',(119.931982055812,4.2,65.5994148249354));
#189059=CARTESIAN_POINT('',(119.403605698873,4.2,65.6972530375517));
#189060=CARTESIAN_POINT('Origin',(116.959178380441,4.2,51.0204257716897));
#189061=CARTESIAN_POINT('',(119.340261028037,4.2,66.02313149207));
#189062=CARTESIAN_POINT('',(119.403605698873,4.2,65.6972530375517));
#189063=CARTESIAN_POINT('Origin',(116.959178380441,4.2,51.0204257716897));
#189064=CARTESIAN_POINT('Origin',(120.11963831679,4.2,64.6340118715271));
#189065=CARTESIAN_POINT('',(119.963056401934,4.7,65.4395519705639));
#189066=CARTESIAN_POINT('',(119.898074486155,4.7,65.7738532780928));
#189067=CARTESIAN_POINT('',(119.963056401934,4.7,65.4395519705639));
#189068=CARTESIAN_POINT('Origin',(122.554452309506,1.45439216225896E-14,
52.1080422752111));
#189069=CARTESIAN_POINT('Origin',(122.554452309506,1.45439216225896E-14,
52.1080422752111));
#189070=CARTESIAN_POINT('Origin',(120.11963831679,4.7,64.6340118715271));
#189071=CARTESIAN_POINT('',(119.434236088778,4.7,65.5396741285193));
#189072=CARTESIAN_POINT('',(119.370170959555,4.7,65.8692590016255));
#189073=CARTESIAN_POINT('',(119.434236088778,4.7,65.5396741285193));
#189074=CARTESIAN_POINT('Origin',(116.959178380441,4.7,51.0204257716897));
#189075=CARTESIAN_POINT('Origin',(116.959178380441,4.7,51.0204257716897));
#189076=CARTESIAN_POINT('Origin',(119.628824814241,4.7,64.5386069150778));
#189077=CARTESIAN_POINT('Origin',(122.063638806956,1.45439216225896E-14,
52.0126373187619));
#189078=CARTESIAN_POINT('Origin',(122.063638806956,1.45439216225896E-14,
52.0126373187619));
#189079=CARTESIAN_POINT('Origin',(119.628824814241,3.2,64.5386069150778));
#189080=CARTESIAN_POINT('',(119.881107483137,3.2,65.8611405060185));
#189081=CARTESIAN_POINT('',(119.818070948787,3.2,66.1854337436511));
#189082=CARTESIAN_POINT('',(119.881107483137,3.2,65.8611405060185));
#189083=CARTESIAN_POINT('',(119.353436145666,3.2,65.9553517260008));
#189084=CARTESIAN_POINT('Origin',(116.959178380441,3.2,51.0204257716897));
#189085=CARTESIAN_POINT('',(119.291237527222,3.2,66.2753342815038));
#189086=CARTESIAN_POINT('',(119.353436145666,3.2,65.9553517260008));
#189087=CARTESIAN_POINT('Origin',(116.959178380441,3.2,51.0204257716897));
#189088=CARTESIAN_POINT('Origin',(120.11963831679,3.2,64.6340118715271));
#189089=CARTESIAN_POINT('',(119.904704490976,3.7,65.7397450303738));
#189090=CARTESIAN_POINT('',(119.841119692148,3.7,66.0668588301531));
#189091=CARTESIAN_POINT('',(119.904704490976,3.7,65.7397450303738));
#189092=CARTESIAN_POINT('Origin',(122.554452309506,1.45439216225896E-14,
52.1080422752111));
#189093=CARTESIAN_POINT('Origin',(122.554452309506,1.45439216225896E-14,
52.1080422752111));
#189094=CARTESIAN_POINT('Origin',(120.11963831679,3.7,64.6340118715271));
#189095=CARTESIAN_POINT('',(119.376709443092,3.7,65.835621587746));
#189096=CARTESIAN_POINT('',(119.313984320114,3.7,66.1583127607501));
#189097=CARTESIAN_POINT('',(119.376709443092,3.7,65.835621587746));
#189098=CARTESIAN_POINT('Origin',(116.959178380441,3.7,51.0204257716897));
#189099=CARTESIAN_POINT('Origin',(116.959178380441,3.7,51.0204257716897));
#189100=CARTESIAN_POINT('Origin',(119.628824814241,3.7,64.5386069150778));
#189101=CARTESIAN_POINT('Origin',(122.063638806956,1.45439216225896E-14,
52.0126373187619));
#189102=CARTESIAN_POINT('Origin',(122.063638806956,1.45439216225896E-14,
52.0126373187619));
#189103=CARTESIAN_POINT('Origin',(119.628824814241,2.2,64.5386069150778));
#189104=CARTESIAN_POINT('',(119.844585514972,2.2,66.0490288063989));
#189105=CARTESIAN_POINT('',(119.782379360477,2.2,66.3690501313291));
#189106=CARTESIAN_POINT('',(119.844585514972,2.2,66.0490288063989));
#189107=CARTESIAN_POINT('',(119.317404303366,2.2,66.1407185599755));
#189108=CARTESIAN_POINT('Origin',(116.959178380441,2.2,51.0204257716897));
#189109=CARTESIAN_POINT('',(119.256003798747,2.2,66.4565951962854));
#189110=CARTESIAN_POINT('',(119.317404303366,2.2,66.1407185599755));
#189111=CARTESIAN_POINT('Origin',(116.959178380441,2.2,51.0204257716897));
#189112=CARTESIAN_POINT('Origin',(120.11963831679,2.2,64.6340118715271));
#189113=CARTESIAN_POINT('',(119.861094292437,2.7,65.9640989328148));
#189114=CARTESIAN_POINT('',(119.798515481723,2.7,66.2860373982266));
#189115=CARTESIAN_POINT('',(119.861094292437,2.7,65.9640989328148));
#189116=CARTESIAN_POINT('Origin',(122.554452309506,1.45439216225896E-14,
52.1080422752111));
#189117=CARTESIAN_POINT('Origin',(122.554452309506,1.45439216225896E-14,
52.1080422752111));
#189118=CARTESIAN_POINT('Origin',(120.11963831679,2.7,64.6340118715271));
#189119=CARTESIAN_POINT('',(119.33369314583,2.7,66.0569201482357));
#189120=CARTESIAN_POINT('',(119.271934362838,2.7,66.3746399577931));
#189121=CARTESIAN_POINT('',(119.33369314583,2.7,66.0569201482357));
#189122=CARTESIAN_POINT('Origin',(116.959178380441,2.7,51.0204257716897));
#189123=CARTESIAN_POINT('Origin',(116.959178380441,2.7,51.0204257716897));
#189124=CARTESIAN_POINT('Origin',(119.628824814241,2.7,64.5386069150778));
#189125=CARTESIAN_POINT('Origin',(122.063638806956,1.45439216225896E-14,
52.0126373187619));
#189126=CARTESIAN_POINT('Origin',(122.063638806956,1.45439216225896E-14,
52.0126373187619));
#189127=CARTESIAN_POINT('Origin',(119.628824814241,1.2,64.5386069150778));
#189128=CARTESIAN_POINT('',(119.821840613373,1.2,66.1660405973442));
#189129=CARTESIAN_POINT('',(119.760140753424,1.2,66.4834572756331));
#189130=CARTESIAN_POINT('',(119.821840613373,1.2,66.1660405973442));
#189131=CARTESIAN_POINT('',(119.294958148874,1.2,66.2561934379564));
#189132=CARTESIAN_POINT('Origin',(116.959178380441,1.2,51.0204257716897));
#189133=CARTESIAN_POINT('',(119.234044670503,1.2,66.5695645539299));
#189134=CARTESIAN_POINT('',(119.294958148874,1.2,66.2561934379564));
#189135=CARTESIAN_POINT('Origin',(116.959178380441,1.2,51.0204257716897));
#189136=CARTESIAN_POINT('Origin',(120.11963831679,1.2,64.6340118715271));
#189137=CARTESIAN_POINT('',(119.831517409679,1.7,66.1162580444744));
#189138=CARTESIAN_POINT('',(119.769603146747,1.7,66.4347777249832));
#189139=CARTESIAN_POINT('',(119.831517409679,1.7,66.1162580444744));
#189140=CARTESIAN_POINT('Origin',(122.554452309506,1.45439216225896E-14,
52.1080422752111));
#189141=CARTESIAN_POINT('Origin',(122.554452309506,1.45439216225896E-14,
52.1080422752111));
#189142=CARTESIAN_POINT('Origin',(120.11963831679,1.7,64.6340118715271));
#189143=CARTESIAN_POINT('',(119.304508441553,1.7,66.2070616865831));
#189144=CARTESIAN_POINT('',(119.243388682605,1.7,66.5214940188289));
#189145=CARTESIAN_POINT('',(119.304508441553,1.7,66.2070616865831));
#189146=CARTESIAN_POINT('Origin',(116.959178380441,1.7,51.0204257716897));
#189147=CARTESIAN_POINT('Origin',(116.959178380441,1.7,51.0204257716897));
#189148=CARTESIAN_POINT('Origin',(119.628824814241,1.7,64.5386069150778));
#189149=CARTESIAN_POINT('Origin',(122.063638806956,1.45439216225896E-14,
52.0126373187619));
#189150=CARTESIAN_POINT('Origin',(122.063638806956,1.45439216225896E-14,
52.0126373187619));
#189151=CARTESIAN_POINT('Origin',(119.628824814241,0.200000000000015,64.5386069150778));
#189152=CARTESIAN_POINT('',(119.812529904723,0.200000000000015,66.2139398018886));
#189153=CARTESIAN_POINT('',(119.751034954835,0.200000000000015,66.530302314559));
#189154=CARTESIAN_POINT('',(119.812529904723,0.200000000000015,66.2139398018886));
#189155=CARTESIAN_POINT('',(119.285768331495,0.200000000000015,66.3034707139332));
#189156=CARTESIAN_POINT('Origin',(116.959178380441,0.200000000000015,51.0204257716897));
#189157=CARTESIAN_POINT('',(119.225052051358,0.200000000000015,66.615827338));
#189158=CARTESIAN_POINT('',(119.285768331495,0.200000000000015,66.3034707139332));
#189159=CARTESIAN_POINT('Origin',(116.959178380441,0.200000000000015,51.0204257716897));
#189160=CARTESIAN_POINT('Origin',(120.11963831679,0.200000000000015,64.6340118715271));
#189161=CARTESIAN_POINT('',(119.815519180792,0.700000000000015,66.1985613864261));
#189162=CARTESIAN_POINT('',(119.753958589789,0.700000000000015,66.5152615916749));
#189163=CARTESIAN_POINT('',(119.815519180792,0.700000000000015,66.1985613864261));
#189164=CARTESIAN_POINT('Origin',(122.554452309506,1.45439216225896E-14,
52.1080422752111));
#189165=CARTESIAN_POINT('Origin',(122.554452309506,1.45439216225896E-14,
52.1080422752111));
#189166=CARTESIAN_POINT('Origin',(120.11963831679,0.700000000000015,64.6340118715271));
#189167=CARTESIAN_POINT('',(119.288718882318,0.700000000000015,66.2882915215953));
#189168=CARTESIAN_POINT('',(119.227939426069,0.700000000000015,66.6009731569646));
#189169=CARTESIAN_POINT('',(119.288718882318,0.700000000000015,66.2882915215953));
#189170=CARTESIAN_POINT('Origin',(116.959178380441,0.700000000000015,51.0204257716897));
#189171=CARTESIAN_POINT('Origin',(116.959178380441,0.700000000000015,51.0204257716897));
#189172=CARTESIAN_POINT('Origin',(119.628824814241,0.700000000000015,64.5386069150778));
#189173=CARTESIAN_POINT('Origin',(122.063638806956,1.45439216225896E-14,
52.0126373187619));
#189174=CARTESIAN_POINT('Origin',(122.063638806956,1.45439216225896E-14,
52.0126373187619));
#189175=CARTESIAN_POINT('Origin',(111.284995270899,0.200000000000015,62.9167226554405));
#189176=CARTESIAN_POINT('',(110.840889914737,0.700000000000015,65.2014352476504));
#189177=CARTESIAN_POINT('',(110.782261475414,0.700000000000015,65.5030509154767));
#189178=CARTESIAN_POINT('',(110.840889914737,0.700000000000015,65.2014352476504));
#189179=CARTESIAN_POINT('',(110.838045843825,0.200000000000015,65.2160666510678));
#189180=CARTESIAN_POINT('Origin',(113.719809263614,1.45439216225896E-14,
50.3907530591246));
#189181=CARTESIAN_POINT('',(110.779474112948,0.200000000000015,65.5173905806832));
#189182=CARTESIAN_POINT('',(110.838045843825,0.200000000000015,65.2160666510678));
#189183=CARTESIAN_POINT('Origin',(113.719809263614,1.45439216225896E-14,
50.3907530591246));
#189184=CARTESIAN_POINT('Origin',(111.284995270899,0.700000000000015,62.9167226554405));
#189185=CARTESIAN_POINT('',(110.372612258069,0.700000000000015,64.9900939933211));
#189186=CARTESIAN_POINT('',(110.313530599756,0.700000000000015,65.2940412590885));
#189187=CARTESIAN_POINT('',(110.372612258069,0.700000000000015,64.9900939933211));
#189188=CARTESIAN_POINT('Origin',(116.959178380441,0.700000000000015,51.0204257716897));
#189189=CARTESIAN_POINT('Origin',(116.959178380441,0.700000000000015,51.0204257716897));
#189190=CARTESIAN_POINT('Origin',(110.79418176835,0.700000000000015,62.8213176989913));
#189191=CARTESIAN_POINT('',(110.369745770862,0.200000000000015,65.0048407180042));
#189192=CARTESIAN_POINT('',(110.310722145193,0.200000000000015,65.3084894331871));
#189193=CARTESIAN_POINT('',(110.369745770862,0.200000000000015,65.0048407180042));
#189194=CARTESIAN_POINT('Origin',(113.228995761065,1.45439216225896E-14,
50.2953481026754));
#189195=CARTESIAN_POINT('Origin',(113.228995761065,1.45439216225896E-14,
50.2953481026754));
#189196=CARTESIAN_POINT('Origin',(110.79418176835,0.200000000000015,62.8213176989913));
#189197=CARTESIAN_POINT('Origin',(116.959178380441,0.200000000000015,51.0204257716897));
#189198=CARTESIAN_POINT('Origin',(116.959178380441,0.200000000000015,51.0204257716897));
#189199=CARTESIAN_POINT('Origin',(110.79418176835,1.2,62.8213176989913));
#189200=CARTESIAN_POINT('',(110.846903310467,1.2,65.1704991628781));
#189201=CARTESIAN_POINT('',(110.788154610309,1.2,65.4727335159764));
#189202=CARTESIAN_POINT('',(110.846903310467,1.2,65.1704991628781));
#189203=CARTESIAN_POINT('',(110.378673197833,1.2,64.958913316921));
#189204=CARTESIAN_POINT('Origin',(116.959178380441,1.2,51.0204257716897));
#189205=CARTESIAN_POINT('',(110.319468461813,1.2,65.2634937594351));
#189206=CARTESIAN_POINT('',(110.378673197833,1.2,64.958913316921));
#189207=CARTESIAN_POINT('Origin',(116.959178380441,1.2,51.0204257716897));
#189208=CARTESIAN_POINT('Origin',(111.284995270899,1.2,62.9167226554405));
#189209=CARTESIAN_POINT('',(110.856105996431,1.7,65.1231556841011));
#189210=CARTESIAN_POINT('',(110.797172304788,1.7,65.4263417311382));
#189211=CARTESIAN_POINT('',(110.856105996431,1.7,65.1231556841011));
#189212=CARTESIAN_POINT('Origin',(113.719809263614,1.45439216225896E-14,
50.3907530591246));
#189213=CARTESIAN_POINT('Origin',(113.719809263614,1.45439216225896E-14,
50.3907530591246));
#189214=CARTESIAN_POINT('Origin',(111.284995270899,1.7,62.9167226554405));
#189215=CARTESIAN_POINT('',(110.387949034711,1.7,64.9111935111905));
#189216=CARTESIAN_POINT('',(110.328554951129,1.7,65.2167480576087));
#189217=CARTESIAN_POINT('',(110.387949034711,1.7,64.9111935111905));
#189218=CARTESIAN_POINT('Origin',(116.959178380441,1.7,51.0204257716897));
#189219=CARTESIAN_POINT('Origin',(116.959178380441,1.7,51.0204257716897));
#189220=CARTESIAN_POINT('Origin',(110.79418176835,1.7,62.8213176989913));
#189221=CARTESIAN_POINT('Origin',(113.228995761065,1.45439216225896E-14,
50.2953481026754));
#189222=CARTESIAN_POINT('Origin',(113.228995761065,1.45439216225896E-14,
50.2953481026754));
#189223=CARTESIAN_POINT('Origin',(110.79418176835,2.2,62.8213176989913));
#189224=CARTESIAN_POINT('',(110.868528853359,2.2,65.0592459445302));
#189225=CARTESIAN_POINT('',(110.809343601815,2.2,65.3637261486052));
#189226=CARTESIAN_POINT('',(110.868528853359,2.2,65.0592459445302));
#189227=CARTESIAN_POINT('',(110.40047139724,2.2,64.8467718622361));
#189228=CARTESIAN_POINT('Origin',(116.959178380441,2.2,51.0204257716897));
#189229=CARTESIAN_POINT('',(110.340819785234,2.2,65.1536512709261));
#189230=CARTESIAN_POINT('',(110.40047139724,2.2,64.8467718622361));
#189231=CARTESIAN_POINT('Origin',(116.959178380441,2.2,51.0204257716897));
#189232=CARTESIAN_POINT('Origin',(111.284995270899,2.2,62.9167226554405));
#189233=CARTESIAN_POINT('',(110.884214204038,2.7,64.9785522133862));
#189234=CARTESIAN_POINT('',(110.824708275305,2.7,65.2846821503487));
#189235=CARTESIAN_POINT('',(110.884214204038,2.7,64.9785522133862));
#189236=CARTESIAN_POINT('Origin',(113.719809263614,1.45439216225896E-14,
50.3907530591246));
#189237=CARTESIAN_POINT('Origin',(113.719809263614,1.45439216225896E-14,
50.3907530591246));
#189238=CARTESIAN_POINT('Origin',(111.284995270899,2.7,62.9167226554405));
#189239=CARTESIAN_POINT('',(110.416283646265,2.7,64.7654252989529));
#189240=CARTESIAN_POINT('',(110.356303673257,2.7,65.0739939701296));
#189241=CARTESIAN_POINT('',(110.416283646265,2.7,64.7654252989529));
#189242=CARTESIAN_POINT('Origin',(116.959178380441,2.7,51.0204257716897));
#189243=CARTESIAN_POINT('Origin',(116.959178380441,2.7,51.0204257716897));
#189244=CARTESIAN_POINT('Origin',(110.79418176835,2.7,62.8213176989913));
#189245=CARTESIAN_POINT('Origin',(113.228995761065,1.45439216225896E-14,
50.2953481026754));
#189246=CARTESIAN_POINT('Origin',(113.228995761065,1.45439216225896E-14,
50.2953481026754));
#189247=CARTESIAN_POINT('Origin',(110.79418176835,3.2,62.8213176989913));
#189248=CARTESIAN_POINT('',(110.903216553537,3.2,64.8807940877961));
#189249=CARTESIAN_POINT('',(110.84331749671,3.2,65.188946483383));
#189250=CARTESIAN_POINT('',(110.903216553537,3.2,64.8807940877961));
#189251=CARTESIAN_POINT('',(110.435441646089,3.2,64.6668664258578));
#189252=CARTESIAN_POINT('Origin',(116.959178380441,3.2,51.0204257716897));
#189253=CARTESIAN_POINT('',(110.375059009152,3.2,64.9775066130281));
#189254=CARTESIAN_POINT('',(110.435441646089,3.2,64.6668664258578));
#189255=CARTESIAN_POINT('Origin',(116.959178380441,3.2,51.0204257716897));
#189256=CARTESIAN_POINT('Origin',(111.284995270899,3.2,62.9167226554405));
#189257=CARTESIAN_POINT('',(110.925603574051,3.7,64.7656234262428));
#189258=CARTESIAN_POINT('',(110.865234719798,3.7,65.0761927080012));
#189259=CARTESIAN_POINT('',(110.925603574051,3.7,64.7656234262428));
#189260=CARTESIAN_POINT('Origin',(113.719809263614,1.45439216225896E-14,
50.3907530591246));
#189261=CARTESIAN_POINT('Origin',(113.719809263614,1.45439216225896E-14,
50.3907530591246));
#189262=CARTESIAN_POINT('Origin',(111.284995270899,3.7,62.9167226554405));
#189263=CARTESIAN_POINT('',(110.458014791367,3.7,64.5507382401787));
#189264=CARTESIAN_POINT('',(110.397150792666,3.7,64.8638548065859));
#189265=CARTESIAN_POINT('',(110.458014791367,3.7,64.5507382401787));
#189266=CARTESIAN_POINT('Origin',(116.959178380441,3.7,51.0204257716897));
#189267=CARTESIAN_POINT('Origin',(116.959178380441,3.7,51.0204257716897));
#189268=CARTESIAN_POINT('Origin',(110.79418176835,3.7,62.8213176989913));
#189269=CARTESIAN_POINT('Origin',(113.228995761065,1.45439216225896E-14,
50.2953481026754));
#189270=CARTESIAN_POINT('Origin',(113.228995761065,1.45439216225896E-14,
50.2953481026754));
#189271=CARTESIAN_POINT('Origin',(110.79418176835,4.2,62.8213176989913));
#189272=CARTESIAN_POINT('',(110.951457377512,4.2,64.6326178015551));
#189273=CARTESIAN_POINT('',(110.890536820758,4.2,64.9460253324646));
#189274=CARTESIAN_POINT('',(110.951457377512,4.2,64.6326178015551));
#189275=CARTESIAN_POINT('',(110.48408733561,4.2,64.4166072973359));
#189276=CARTESIAN_POINT('Origin',(116.959178380441,4.2,51.0204257716897));
#189277=CARTESIAN_POINT('',(110.422657817275,4.2,64.7326331955291));
#189278=CARTESIAN_POINT('',(110.48408733561,4.2,64.4166072973359));
#189279=CARTESIAN_POINT('Origin',(116.959178380441,4.2,51.0204257716897));
#189280=CARTESIAN_POINT('Origin',(111.284995270899,4.2,62.9167226554405));
#189281=CARTESIAN_POINT('',(110.980876134901,4.7,64.4812721703395));
#189282=CARTESIAN_POINT('',(110.919315543898,4.7,64.7979723755884));
#189283=CARTESIAN_POINT('',(110.980876134901,4.7,64.4812721703395));
#189284=CARTESIAN_POINT('Origin',(113.719809263614,1.45439216225896E-14,
50.3907530591246));
#189285=CARTESIAN_POINT('Origin',(113.719809263614,1.45439216225896E-14,
50.3907530591246));
#189286=CARTESIAN_POINT('Origin',(111.284995270899,4.7,62.9167226554405));
#189287=CARTESIAN_POINT('',(110.513760083927,4.7,64.2639550025948));
#189288=CARTESIAN_POINT('',(110.451674178493,4.7,64.5833577028194));
#189289=CARTESIAN_POINT('',(110.513760083927,4.7,64.2639550025948));
#189290=CARTESIAN_POINT('Origin',(116.959178380441,4.7,51.0204257716897));
#189291=CARTESIAN_POINT('Origin',(116.959178380441,4.7,51.0204257716897));
#189292=CARTESIAN_POINT('Origin',(110.79418176835,4.7,62.8213176989913));
#189293=CARTESIAN_POINT('Origin',(113.228995761065,1.45439216225896E-14,
50.2953481026754));
#189294=CARTESIAN_POINT('Origin',(113.228995761065,1.45439216225896E-14,
50.2953481026754));
#189295=CARTESIAN_POINT('Origin',(111.775808773449,4.2,63.0121276118898));
#189296=CARTESIAN_POINT('',(111.896501450699,4.2,65.0116296445541));
#189297=CARTESIAN_POINT('',(111.836358656514,4.2,65.3210359538879));
#189298=CARTESIAN_POINT('',(111.896501450699,4.2,65.0116296445541));
#189299=CARTESIAN_POINT('',(111.422286729203,4.2,64.830831788513));
#189300=CARTESIAN_POINT('Origin',(116.959178380441,4.2,51.0204257716897));
#189301=CARTESIAN_POINT('',(111.361793489841,4.2,65.142040972989));
#189302=CARTESIAN_POINT('',(111.422286729203,4.2,64.830831788513));
#189303=CARTESIAN_POINT('Origin',(116.959178380441,4.2,51.0204257716897));
#189304=CARTESIAN_POINT('Origin',(112.266622275998,4.2,63.107532568339));
#189305=CARTESIAN_POINT('',(111.925532478671,4.7,64.862278698319));
#189306=CARTESIAN_POINT('',(111.864774103035,4.7,65.1748518838705));
#189307=CARTESIAN_POINT('',(111.925532478671,4.7,64.862278698319));
#189308=CARTESIAN_POINT('Origin',(114.701436268713,1.45439216225896E-14,
50.5815629720231));
#189309=CARTESIAN_POINT('Origin',(114.701436268713,1.45439216225896E-14,
50.5815629720231));
#189310=CARTESIAN_POINT('Origin',(112.266622275998,4.7,63.107532568339));
#189311=CARTESIAN_POINT('',(111.451492400761,4.7,64.6805823833951));
#189312=CARTESIAN_POINT('',(111.390372641813,4.7,64.9950147156409));
#189313=CARTESIAN_POINT('',(111.451492400761,4.7,64.6805823833951));
#189314=CARTESIAN_POINT('Origin',(116.959178380441,4.7,51.0204257716897));
#189315=CARTESIAN_POINT('Origin',(116.959178380441,4.7,51.0204257716897));
#189316=CARTESIAN_POINT('Origin',(111.775808773449,4.7,63.0121276118898));
#189317=CARTESIAN_POINT('Origin',(114.210622766164,1.45439216225896E-14,
50.4861580155739));
#189318=CARTESIAN_POINT('Origin',(114.210622766164,1.45439216225896E-14,
50.4861580155739));
#189319=CARTESIAN_POINT('Origin',(112.757435778548,4.2,63.2029375247883));
#189320=CARTESIAN_POINT('',(112.854860725266,4.2,65.322141056661));
#189321=CARTESIAN_POINT('',(112.79520246584,4.2,65.6290546631941));
#189322=CARTESIAN_POINT('',(112.854860725266,4.2,65.322141056661));
#189323=CARTESIAN_POINT('',(112.374041723553,4.2,65.1753191073788));
#189324=CARTESIAN_POINT('Origin',(116.959178380441,4.2,51.0204257716897));
#189325=CARTESIAN_POINT('',(112.314176285267,4.2,65.4832985514289));
#189326=CARTESIAN_POINT('',(112.374041723553,4.2,65.1753191073788));
#189327=CARTESIAN_POINT('Origin',(116.959178380441,4.2,51.0204257716897));
#189328=CARTESIAN_POINT('Origin',(113.248249281097,4.2,63.2983424812375));
#189329=CARTESIAN_POINT('',(112.883650447187,4.7,65.1740315162422));
#189330=CARTESIAN_POINT('',(112.82339151564,4.7,65.4840352975252));
#189331=CARTESIAN_POINT('',(112.883650447187,4.7,65.1740315162422));
#189332=CARTESIAN_POINT('Origin',(115.683063273812,1.45439216225896E-14,
50.7723728849216));
#189333=CARTESIAN_POINT('Origin',(115.683063273812,1.45439216225896E-14,
50.7723728849216));
#189334=CARTESIAN_POINT('Origin',(113.248249281097,4.7,63.2983424812375));
#189335=CARTESIAN_POINT('',(112.40293460111,4.7,65.0266788798666));
#189336=CARTESIAN_POINT('',(112.342462146009,4.7,65.337781139129));
#189337=CARTESIAN_POINT('',(112.40293460111,4.7,65.0266788798666));
#189338=CARTESIAN_POINT('Origin',(116.959178380441,4.7,51.0204257716897));
#189339=CARTESIAN_POINT('Origin',(116.959178380441,4.7,51.0204257716897));
#189340=CARTESIAN_POINT('Origin',(112.757435778548,4.7,63.2029375247883));
#189341=CARTESIAN_POINT('Origin',(115.192249771263,1.45439216225896E-14,
50.6769679284724));
#189342=CARTESIAN_POINT('Origin',(115.192249771263,1.45439216225896E-14,
50.6769679284724));
#189343=CARTESIAN_POINT('Origin',(113.739062783647,4.2,63.3937474376868));
#189344=CARTESIAN_POINT('',(113.826207738508,4.2,65.5658366790392));
#189345=CARTESIAN_POINT('',(113.76676110055,4.2,65.8716615929319));
#189346=CARTESIAN_POINT('',(113.826207738508,4.2,65.5658366790392));
#189347=CARTESIAN_POINT('',(113.338923778585,4.2,65.4522738905049));
#189348=CARTESIAN_POINT('Origin',(116.959178380441,4.2,51.0204257716897));
#189349=CARTESIAN_POINT('',(113.27940465001,4.2,65.7584717344309));
#189350=CARTESIAN_POINT('',(113.338923778585,4.2,65.4522738905049));
#189351=CARTESIAN_POINT('Origin',(116.959178380441,4.2,51.0204257716897));
#189352=CARTESIAN_POINT('Origin',(114.229876286196,4.2,63.489152394136));
#189353=CARTESIAN_POINT('',(113.854892127718,4.7,65.4182690257343));
#189354=CARTESIAN_POINT('',(113.794851251881,4.7,65.7271510132369));
#189355=CARTESIAN_POINT('',(113.854892127718,4.7,65.4182690257343));
#189356=CARTESIAN_POINT('Origin',(116.664690278911,1.45439216225896E-14,
50.9631827978201));
#189357=CARTESIAN_POINT('Origin',(116.664690278911,1.45439216225896E-14,
50.9631827978201));
#189358=CARTESIAN_POINT('Origin',(114.229876286196,4.7,63.489152394136));
#189359=CARTESIAN_POINT('',(113.367644245392,4.7,65.3045206349844));
#189360=CARTESIAN_POINT('',(113.307528680178,4.7,65.6137868641028));
#189361=CARTESIAN_POINT('',(113.367644245392,4.7,65.3045206349844));
#189362=CARTESIAN_POINT('Origin',(116.959178380441,4.7,51.0204257716897));
#189363=CARTESIAN_POINT('Origin',(116.959178380441,4.7,51.0204257716897));
#189364=CARTESIAN_POINT('Origin',(113.739062783647,4.7,63.3937474376868));
#189365=CARTESIAN_POINT('Origin',(116.173876776362,1.45439216225896E-14,
50.8677778413709));
#189366=CARTESIAN_POINT('Origin',(116.173876776362,1.45439216225896E-14,
50.8677778413709));
#189367=CARTESIAN_POINT('Origin',(114.720689788746,4.2,63.5845573505853));
#189368=CARTESIAN_POINT('',(114.810401248048,4.2,65.7434431370981));
#189369=CARTESIAN_POINT('',(114.750901915942,4.2,66.0495391375266));
#189370=CARTESIAN_POINT('',(114.810401248048,4.2,65.7434431370981));
#189371=CARTESIAN_POINT('',(114.31670059115,4.2,65.6628912280229));
#189372=CARTESIAN_POINT('Origin',(116.959178380441,4.2,51.0204257716897));
#189373=CARTESIAN_POINT('',(114.25726053012,4.2,65.9686823067247));
#189374=CARTESIAN_POINT('',(114.31670059115,4.2,65.6628912280229));
#189375=CARTESIAN_POINT('Origin',(116.959178380441,4.2,51.0204257716897));
#189376=CARTESIAN_POINT('Origin',(115.211503291295,4.2,63.6799623070345));
#189377=CARTESIAN_POINT('',(114.83911186201,4.7,65.595740569812));
#189378=CARTESIAN_POINT('',(114.779016694271,4.7,65.9049018635434));
#189379=CARTESIAN_POINT('',(114.83911186201,4.7,65.595740569812));
#189380=CARTESIAN_POINT('Origin',(117.64631728401,1.45439216225896E-14,
51.1539927107186));
#189381=CARTESIAN_POINT('Origin',(117.64631728401,1.45439216225896E-14,
51.1539927107186));
#189382=CARTESIAN_POINT('Origin',(115.211503291295,4.7,63.6799623070345));
#189383=CARTESIAN_POINT('',(114.345381707316,4.7,65.5153404129881));
#189384=CARTESIAN_POINT('',(114.285347607624,4.7,65.8241875404224));
#189385=CARTESIAN_POINT('',(114.345381707316,4.7,65.5153404129881));
#189386=CARTESIAN_POINT('Origin',(116.959178380441,4.7,51.0204257716897));
#189387=CARTESIAN_POINT('Origin',(116.959178380441,4.7,51.0204257716897));
#189388=CARTESIAN_POINT('Origin',(114.720689788746,4.7,63.5845573505853));
#189389=CARTESIAN_POINT('Origin',(117.155503781461,1.45439216225896E-14,
51.0585877542694));
#189390=CARTESIAN_POINT('Origin',(117.155503781461,1.45439216225896E-14,
51.0585877542694));
#189391=CARTESIAN_POINT('Origin',(115.702316793845,4.2,63.7753672634838));
#189392=CARTESIAN_POINT('',(115.807476322943,4.2,65.8547800170803));
#189393=CARTESIAN_POINT('',(115.747657855648,4.2,66.1625178175346));
#189394=CARTESIAN_POINT('',(115.807476322943,4.2,65.8547800170803));
#189395=CARTESIAN_POINT('',(115.307319527602,4.2,65.8074418952141));
#189396=CARTESIAN_POINT('Origin',(116.959178380441,4.2,51.0204257716897));
#189397=CARTESIAN_POINT('',(115.247694483068,4.2,66.1141846267932));
#189398=CARTESIAN_POINT('',(115.307319527602,4.2,65.8074418952141));
#189399=CARTESIAN_POINT('Origin',(116.959178380441,4.2,51.0204257716897));
#189400=CARTESIAN_POINT('Origin',(116.193130296394,4.2,63.870772219933));
#189401=CARTESIAN_POINT('',(115.836345810381,4.7,65.7062601206949));
#189402=CARTESIAN_POINT('',(115.775921768676,4.7,66.01711331587));
#189403=CARTESIAN_POINT('',(115.836345810381,4.7,65.7062601206949));
#189404=CARTESIAN_POINT('Origin',(118.62794428911,1.45439216225896E-14,
51.3448026236171));
#189405=CARTESIAN_POINT('Origin',(118.62794428911,1.45439216225896E-14,
51.3448026236171));
#189406=CARTESIAN_POINT('Origin',(116.193130296394,4.7,63.870772219933));
#189407=CARTESIAN_POINT('',(115.336092714776,4.7,65.6594174182724));
#189408=CARTESIAN_POINT('',(115.275868011104,4.7,65.9692451132811));
#189409=CARTESIAN_POINT('',(115.336092714776,4.7,65.6594174182724));
#189410=CARTESIAN_POINT('Origin',(116.959178380441,4.7,51.0204257716897));
#189411=CARTESIAN_POINT('Origin',(116.959178380441,4.7,51.0204257716897));
#189412=CARTESIAN_POINT('Origin',(115.702316793845,4.7,63.7753672634838));
#189413=CARTESIAN_POINT('Origin',(118.13713078656,1.45439216225896E-14,
51.2493976671679));
#189414=CARTESIAN_POINT('Origin',(118.13713078656,1.45439216225896E-14,
51.2493976671679));
#189415=CARTESIAN_POINT('Origin',(116.683943798944,4.2,63.9661771763823));
#189416=CARTESIAN_POINT('',(116.817646780977,4.2,65.8987473273376));
#189417=CARTESIAN_POINT('',(116.757229645983,4.2,66.2095649907366));
#189418=CARTESIAN_POINT('',(116.817646780977,4.2,65.8987473273376));
#189419=CARTESIAN_POINT('',(116.310903962914,4.2,65.8852911860356));
#189420=CARTESIAN_POINT('Origin',(116.959178380441,4.2,51.0204257716897));
#189421=CARTESIAN_POINT('',(116.250822381959,4.2,66.1943825821719));
#189422=CARTESIAN_POINT('',(116.310903962914,4.2,65.8852911860356));
#189423=CARTESIAN_POINT('Origin',(116.959178380441,4.2,51.0204257716897));
#189424=CARTESIAN_POINT('Origin',(117.174757301493,4.2,64.0615821328315));
#189425=CARTESIAN_POINT('',(116.846814517752,4.7,65.7486930787876));
#189426=CARTESIAN_POINT('',(116.785773249647,4.7,66.062721612669));
#189427=CARTESIAN_POINT('',(116.846814517752,4.7,65.7486930787876));
#189428=CARTESIAN_POINT('Origin',(119.609571294209,1.45439216225896E-14,
51.5356125365156));
#189429=CARTESIAN_POINT('Origin',(119.609571294209,1.45439216225896E-14,
51.5356125365156));
#189430=CARTESIAN_POINT('Origin',(117.174757301493,4.7,64.0615821328315));
#189431=CARTESIAN_POINT('',(116.339904495447,4.7,65.7360971244494));
#189432=CARTESIAN_POINT('',(116.27920923027,4.7,66.0483456364567));
#189433=CARTESIAN_POINT('',(116.339904495447,4.7,65.7360971244494));
#189434=CARTESIAN_POINT('Origin',(116.959178380441,4.7,51.0204257716897));
#189435=CARTESIAN_POINT('Origin',(116.959178380441,4.7,51.0204257716897));
#189436=CARTESIAN_POINT('Origin',(116.683943798944,4.7,63.9661771763823));
#189437=CARTESIAN_POINT('Origin',(119.118757791659,1.45439216225896E-14,
51.4402075800664));
#189438=CARTESIAN_POINT('Origin',(119.118757791659,1.45439216225896E-14,
51.4402075800664));
#189439=CARTESIAN_POINT('Origin',(117.665570804043,4.2,64.1569870892808));
#189440=CARTESIAN_POINT('',(117.841320378148,4.2,65.8732473555792));
#189441=CARTESIAN_POINT('',(117.779999449725,4.2,66.1887146098929));
#189442=CARTESIAN_POINT('',(117.841320378148,4.2,65.8732473555792));
#189443=CARTESIAN_POINT('',(117.327761915775,4.2,65.894854489609));
#189444=CARTESIAN_POINT('Origin',(116.959178380441,4.2,51.0204257716897));
#189445=CARTESIAN_POINT('',(117.266933185955,4.2,66.2077896142598));
#189446=CARTESIAN_POINT('',(117.327761915775,4.2,65.894854489609));
#189447=CARTESIAN_POINT('Origin',(116.959178380441,4.2,51.0204257716897));
#189448=CARTESIAN_POINT('Origin',(118.156384306592,4.2,64.25239204573));
#189449=CARTESIAN_POINT('',(117.870938918374,4.7,65.7208739358971));
#189450=CARTESIAN_POINT('',(117.808965115304,4.7,66.0396999223345));
#189451=CARTESIAN_POINT('',(117.870938918374,4.7,65.7208739358971));
#189452=CARTESIAN_POINT('Origin',(120.591198299308,1.45439216225896E-14,
51.7264224494141));
#189453=CARTESIAN_POINT('Origin',(120.591198299308,1.45439216225896E-14,
51.7264224494141));
#189454=CARTESIAN_POINT('Origin',(118.156384306592,4.7,64.25239204573));
#189455=CARTESIAN_POINT('',(117.357134870407,4.7,65.7437444919779));
#189456=CARTESIAN_POINT('',(117.295669027016,4.7,66.0599572654489));
#189457=CARTESIAN_POINT('',(117.357134870407,4.7,65.7437444919779));
#189458=CARTESIAN_POINT('Origin',(116.959178380441,4.7,51.0204257716897));
#189459=CARTESIAN_POINT('Origin',(116.959178380441,4.7,51.0204257716897));
#189460=CARTESIAN_POINT('Origin',(117.665570804043,4.7,64.1569870892808));
#189461=CARTESIAN_POINT('Origin',(120.100384796758,1.45439216225896E-14,
51.6310174929649));
#189462=CARTESIAN_POINT('Origin',(120.100384796758,1.45439216225896E-14,
51.6310174929649));
#189463=CARTESIAN_POINT('Origin',(118.647197809142,4.2,64.3477970021793));
#189464=CARTESIAN_POINT('',(118.879129362164,4.2,65.7750274855535));
#189465=CARTESIAN_POINT('',(118.816558223758,4.2,66.0969264805582));
#189466=CARTESIAN_POINT('',(118.879129362164,4.2,65.7750274855535));
#189467=CARTESIAN_POINT('',(118.358408432976,4.2,65.8334821331224));
#189468=CARTESIAN_POINT('Origin',(116.959178380441,4.2,51.0204257716897));
#189469=CARTESIAN_POINT('',(118.296509028281,4.2,66.1519253750136));
#189470=CARTESIAN_POINT('',(118.358408432976,4.2,65.8334821331224));
#189471=CARTESIAN_POINT('Origin',(116.959178380441,4.2,51.0204257716897));
#189472=CARTESIAN_POINT('Origin',(119.138011311691,4.2,64.4432019586286));
#189473=CARTESIAN_POINT('',(118.909372592695,4.7,65.6194403288909));
#189474=CARTESIAN_POINT('',(118.846107361872,4.7,65.9449101020099));
#189475=CARTESIAN_POINT('',(118.909372592695,4.7,65.6194403288909));
#189476=CARTESIAN_POINT('Origin',(121.572825304407,1.45439216225896E-14,
51.9172323623126));
#189477=CARTESIAN_POINT('Origin',(121.572825304407,1.45439216225896E-14,
51.9172323623126));
#189478=CARTESIAN_POINT('Origin',(119.138011311691,4.7,64.4432019586286));
#189479=CARTESIAN_POINT('',(118.388315859615,4.7,65.6796225291042));
#189480=CARTESIAN_POINT('',(118.325744721209,4.7,66.0015215241089));
#189481=CARTESIAN_POINT('',(118.388315859615,4.7,65.6796225291042));
#189482=CARTESIAN_POINT('Origin',(116.959178380441,4.7,51.0204257716897));
#189483=CARTESIAN_POINT('Origin',(116.959178380441,4.7,51.0204257716897));
#189484=CARTESIAN_POINT('Origin',(118.647197809142,4.7,64.3477970021793));
#189485=CARTESIAN_POINT('Origin',(121.082011801857,1.45439216225896E-14,
51.8218274058634));
#189486=CARTESIAN_POINT('Origin',(121.082011801857,1.45439216225896E-14,
51.8218274058634));
#189487=CARTESIAN_POINT('Origin',(118.647197809142,3.2,64.3477970021793));
#189488=CARTESIAN_POINT('',(118.829575378056,3.2,66.0299593613256));
#189489=CARTESIAN_POINT('',(118.768109534665,3.2,66.3461721347966));
#189490=CARTESIAN_POINT('',(118.829575378056,3.2,66.0299593613256));
#189491=CARTESIAN_POINT('',(118.309388920874,3.2,66.0856644025075));
#189492=CARTESIAN_POINT('Origin',(116.959178380441,3.2,51.0204257716897));
#189493=CARTESIAN_POINT('',(118.248560191054,3.2,66.3985995271583));
#189494=CARTESIAN_POINT('',(118.309388920874,3.2,66.0856644025075));
#189495=CARTESIAN_POINT('Origin',(116.959178380441,3.2,51.0204257716897));
#189496=CARTESIAN_POINT('Origin',(119.138011311691,3.2,64.4432019586286));
#189497=CARTESIAN_POINT('',(118.852565923473,3.7,65.9116838487956));
#189498=CARTESIAN_POINT('',(118.790592120403,3.7,66.230509835233));
#189499=CARTESIAN_POINT('',(118.852565923473,3.7,65.9116838487956));
#189500=CARTESIAN_POINT('Origin',(121.572825304407,1.45439216225896E-14,
51.9172323623126));
#189501=CARTESIAN_POINT('Origin',(121.572825304407,1.45439216225896E-14,
51.9172323623126));
#189502=CARTESIAN_POINT('Origin',(119.138011311691,3.7,64.4432019586286));
#189503=CARTESIAN_POINT('',(118.332133880698,3.7,65.9686523120285));
#189504=CARTESIAN_POINT('',(118.270812952274,3.7,66.2841195663421));
#189505=CARTESIAN_POINT('',(118.332133880698,3.7,65.9686523120285));
#189506=CARTESIAN_POINT('Origin',(116.959178380441,3.7,51.0204257716897));
#189507=CARTESIAN_POINT('Origin',(116.959178380441,3.7,51.0204257716897));
#189508=CARTESIAN_POINT('Origin',(118.647197809142,3.7,64.3477970021793));
#189509=CARTESIAN_POINT('Origin',(121.082011801857,1.45439216225896E-14,
51.8218274058634));
#189510=CARTESIAN_POINT('Origin',(121.082011801857,1.45439216225896E-14,
51.8218274058634));
#189511=CARTESIAN_POINT('Origin',(118.647197809142,2.2,64.3477970021793));
#189512=CARTESIAN_POINT('',(118.793972008194,2.2,66.2131219066956));
#189513=CARTESIAN_POINT('',(118.733276743018,2.2,66.5253704187029));
#189514=CARTESIAN_POINT('',(118.793972008194,2.2,66.2131219066956));
#189515=CARTESIAN_POINT('',(118.274157973112,2.2,66.2669110118326));
#189516=CARTESIAN_POINT('Origin',(116.959178380441,2.2,51.0204257716897));
#189517=CARTESIAN_POINT('',(118.214076392157,2.2,66.5760024079689));
#189518=CARTESIAN_POINT('',(118.274157973112,2.2,66.2669110118326));
#189519=CARTESIAN_POINT('Origin',(116.959178380441,2.2,51.0204257716897));
#189520=CARTESIAN_POINT('Origin',(119.138011311691,2.2,64.4432019586286));
#189521=CARTESIAN_POINT('',(118.81006852795,2.7,66.1303129045846));
#189522=CARTESIAN_POINT('',(118.749027259845,2.7,66.444341438466));
#189523=CARTESIAN_POINT('',(118.81006852795,2.7,66.1303129045846));
#189524=CARTESIAN_POINT('Origin',(121.572825304407,1.45439216225896E-14,
51.9172323623126));
#189525=CARTESIAN_POINT('Origin',(121.572825304407,1.45439216225896E-14,
51.9172323623126));
#189526=CARTESIAN_POINT('Origin',(119.138011311691,2.7,64.4432019586286));
#189527=CARTESIAN_POINT('',(118.290087288625,2.7,66.1849621966853));
#189528=CARTESIAN_POINT('',(118.229670153632,2.7,66.4957798600844));
#189529=CARTESIAN_POINT('',(118.290087288625,2.7,66.1849621966853));
#189530=CARTESIAN_POINT('Origin',(116.959178380441,2.7,51.0204257716897));
#189531=CARTESIAN_POINT('Origin',(116.959178380441,2.7,51.0204257716897));
#189532=CARTESIAN_POINT('Origin',(118.647197809142,2.7,64.3477970021793));
#189533=CARTESIAN_POINT('Origin',(121.082011801857,1.45439216225896E-14,
51.8218274058634));
#189534=CARTESIAN_POINT('Origin',(121.082011801857,1.45439216225896E-14,
51.8218274058634));
#189535=CARTESIAN_POINT('Origin',(118.647197809142,1.2,64.3477970021793));
#189536=CARTESIAN_POINT('',(118.771787232622,1.2,66.3272521134172));
#189537=CARTESIAN_POINT('',(118.711562528951,1.2,66.6370798084259));
#189538=CARTESIAN_POINT('',(118.771787232622,1.2,66.3272521134172));
#189539=CARTESIAN_POINT('',(118.252200542899,1.2,66.3798716339097));
#189540=CARTESIAN_POINT('Origin',(116.959178380441,1.2,51.0204257716897));
#189541=CARTESIAN_POINT('',(118.192575498365,1.2,66.6866143654888));
#189542=CARTESIAN_POINT('',(118.252200542899,1.2,66.3798716339097));
#189543=CARTESIAN_POINT('Origin',(116.959178380441,1.2,51.0204257716897));
#189544=CARTESIAN_POINT('Origin',(119.138011311691,1.2,64.4432019586286));
#189545=CARTESIAN_POINT('',(118.781226825678,1.7,66.2786898593904));
#189546=CARTESIAN_POINT('',(118.720802783973,1.7,66.5895430545655));
#189547=CARTESIAN_POINT('',(118.781226825678,1.7,66.2786898593904));
#189548=CARTESIAN_POINT('Origin',(121.572825304407,1.45439216225896E-14,
51.9172323623126));
#189549=CARTESIAN_POINT('Origin',(121.572825304407,1.45439216225896E-14,
51.9172323623126));
#189550=CARTESIAN_POINT('Origin',(119.138011311691,1.7,64.4432019586286));
#189551=CARTESIAN_POINT('',(118.26154383569,1.7,66.3318047993266));
#189552=CARTESIAN_POINT('',(118.201725368395,1.7,66.6395425997809));
#189553=CARTESIAN_POINT('',(118.26154383569,1.7,66.3318047993266));
#189554=CARTESIAN_POINT('Origin',(116.959178380441,1.7,51.0204257716897));
#189555=CARTESIAN_POINT('Origin',(116.959178380441,1.7,51.0204257716897));
#189556=CARTESIAN_POINT('Origin',(118.647197809142,1.7,64.3477970021793));
#189557=CARTESIAN_POINT('Origin',(121.082011801857,1.45439216225896E-14,
51.8218274058634));
#189558=CARTESIAN_POINT('Origin',(121.082011801857,1.45439216225896E-14,
51.8218274058634));
#189559=CARTESIAN_POINT('Origin',(118.647197809142,0.200000000000015,64.3477970021793));
#189560=CARTESIAN_POINT('',(118.762703230262,0.200000000000015,66.3739850210313));
#189561=CARTESIAN_POINT('',(118.70266913057,0.200000000000015,66.6828321484657));
#189562=CARTESIAN_POINT('',(118.762703230262,0.200000000000015,66.3739850210313));
#189563=CARTESIAN_POINT('',(118.243208611546,0.200000000000015,66.4261308796169));
#189564=CARTESIAN_POINT('Origin',(116.959178380441,0.200000000000015,51.0204257716897));
#189565=CARTESIAN_POINT('',(118.183768550516,0.200000000000015,66.7319219583188));
#189566=CARTESIAN_POINT('',(118.243208611546,0.200000000000015,66.4261308796169));
#189567=CARTESIAN_POINT('Origin',(116.959178380441,0.200000000000015,51.0204257716897));
#189568=CARTESIAN_POINT('Origin',(119.138011311691,0.200000000000015,64.4432019586286));
#189569=CARTESIAN_POINT('',(118.765619882406,0.700000000000015,66.358980221406));
#189570=CARTESIAN_POINT('',(118.705524714667,0.700000000000015,66.6681415151374));
#189571=CARTESIAN_POINT('',(118.765619882406,0.700000000000015,66.358980221406));
#189572=CARTESIAN_POINT('Origin',(121.572825304407,1.45439216225896E-14,
51.9172323623126));
#189573=CARTESIAN_POINT('Origin',(121.572825304407,1.45439216225896E-14,
51.9172323623126));
#189574=CARTESIAN_POINT('Origin',(119.138011311691,0.700000000000015,64.4432019586286));
#189575=CARTESIAN_POINT('',(118.246095765894,0.700000000000015,66.4112778322429));
#189576=CARTESIAN_POINT('',(118.186596433788,0.700000000000015,66.7173738326713));
#189577=CARTESIAN_POINT('',(118.246095765894,0.700000000000015,66.4112778322429));
#189578=CARTESIAN_POINT('Origin',(116.959178380441,0.700000000000015,51.0204257716897));
#189579=CARTESIAN_POINT('Origin',(116.959178380441,0.700000000000015,51.0204257716897));
#189580=CARTESIAN_POINT('Origin',(118.647197809142,0.700000000000015,64.3477970021793));
#189581=CARTESIAN_POINT('Origin',(121.082011801857,1.45439216225896E-14,
51.8218274058634));
#189582=CARTESIAN_POINT('Origin',(121.082011801857,1.45439216225896E-14,
51.8218274058634));
#189583=CARTESIAN_POINT('Origin',(111.775808773449,0.200000000000015,63.0121276118898));
#189584=CARTESIAN_POINT('',(111.784511933794,0.200000000000015,65.58776288843));
#189585=CARTESIAN_POINT('',(111.726632415304,0.200000000000015,65.8855257118037));
#189586=CARTESIAN_POINT('',(111.784511933794,0.200000000000015,65.58776288843));
#189587=CARTESIAN_POINT('',(111.30965635868,0.200000000000015,65.4102619219916));
#189588=CARTESIAN_POINT('Origin',(116.959178380441,0.200000000000015,51.0204257716897));
#189589=CARTESIAN_POINT('',(111.251464695365,0.200000000000015,65.7096305832602));
#189590=CARTESIAN_POINT('',(111.30965635868,0.200000000000015,65.4102619219916));
#189591=CARTESIAN_POINT('Origin',(116.959178380441,0.200000000000015,51.0204257716897));
#189592=CARTESIAN_POINT('Origin',(112.266622275998,0.200000000000015,63.107532568339));
#189593=CARTESIAN_POINT('',(111.787321688715,0.700000000000015,65.5733080246022));
#189594=CARTESIAN_POINT('',(111.729387450815,0.700000000000015,65.8713523535303));
#189595=CARTESIAN_POINT('',(111.787321688715,0.700000000000015,65.5733080246022));
#189596=CARTESIAN_POINT('Origin',(114.701436268713,1.45439216225896E-14,
50.5815629720231));
#189597=CARTESIAN_POINT('Origin',(114.701436268713,1.45439216225896E-14,
50.5815629720231));
#189598=CARTESIAN_POINT('Origin',(112.266622275998,0.700000000000015,63.107532568339));
#189599=CARTESIAN_POINT('',(111.31248158481,0.700000000000015,65.3957274660892));
#189600=CARTESIAN_POINT('',(111.254234311024,0.700000000000015,65.6953822170022));
#189601=CARTESIAN_POINT('',(111.31248158481,0.700000000000015,65.3957274660892));
#189602=CARTESIAN_POINT('Origin',(116.959178380441,0.700000000000015,51.0204257716897));
#189603=CARTESIAN_POINT('Origin',(116.959178380441,0.700000000000015,51.0204257716897));
#189604=CARTESIAN_POINT('Origin',(111.775808773449,0.700000000000015,63.0121276118898));
#189605=CARTESIAN_POINT('Origin',(114.210622766164,1.45439216225896E-14,
50.4861580155739));
#189606=CARTESIAN_POINT('Origin',(114.210622766164,1.45439216225896E-14,
50.4861580155739));
#189607=CARTESIAN_POINT('Origin',(111.775808773449,1.2,63.0121276118898));
#189608=CARTESIAN_POINT('',(111.793262308365,1.2,65.5427463384361));
#189609=CARTESIAN_POINT('',(111.735212040126,1.2,65.8413875887286));
#189610=CARTESIAN_POINT('',(111.793262308365,1.2,65.5427463384361));
#189611=CARTESIAN_POINT('',(111.318455014226,1.2,65.3649969891498));
#189612=CARTESIAN_POINT('Origin',(116.959178380441,1.2,51.0204257716897));
#189613=CARTESIAN_POINT('',(111.260089814989,1.2,65.6652584108877));
#189614=CARTESIAN_POINT('',(111.318455014226,1.2,65.3649969891498));
#189615=CARTESIAN_POINT('Origin',(116.959178380441,1.2,51.0204257716897));
#189616=CARTESIAN_POINT('Origin',(112.266622275998,1.2,63.107532568339));
#189617=CARTESIAN_POINT('',(111.802353039398,1.7,65.4959788149727));
#189618=CARTESIAN_POINT('',(111.74412432015,1.7,65.7955381115431));
#189619=CARTESIAN_POINT('',(111.802353039398,1.7,65.4959788149727));
#189620=CARTESIAN_POINT('Origin',(114.701436268713,1.45439216225896E-14,
50.5815629720231));
#189621=CARTESIAN_POINT('Origin',(114.701436268713,1.45439216225896E-14,
50.5815629720231));
#189622=CARTESIAN_POINT('Origin',(112.266622275998,1.7,63.107532568339));
#189623=CARTESIAN_POINT('',(111.327596215435,1.7,65.3179698204353));
#189624=CARTESIAN_POINT('',(111.269049635537,1.7,65.6191643601265));
#189625=CARTESIAN_POINT('',(111.327596215435,1.7,65.3179698204353));
#189626=CARTESIAN_POINT('Origin',(116.959178380441,1.7,51.0204257716897));
#189627=CARTESIAN_POINT('Origin',(116.959178380441,1.7,51.0204257716897));
#189628=CARTESIAN_POINT('Origin',(111.775808773449,1.7,63.0121276118898));
#189629=CARTESIAN_POINT('Origin',(114.210622766164,1.45439216225896E-14,
50.4861580155739));
#189630=CARTESIAN_POINT('Origin',(114.210622766164,1.45439216225896E-14,
50.4861580155739));
#189631=CARTESIAN_POINT('Origin',(111.775808773449,2.2,63.0121276118898));
#189632=CARTESIAN_POINT('',(111.814623641277,2.2,65.4328523558162));
#189633=CARTESIAN_POINT('',(111.756152320341,2.2,65.7336597236466));
#189634=CARTESIAN_POINT('',(111.814623641277,2.2,65.4328523558162));
#189635=CARTESIAN_POINT('',(111.339935449923,2.2,65.2544902788798));
#189636=CARTESIAN_POINT('Origin',(116.959178380441,2.2,51.0204257716897));
#189637=CARTESIAN_POINT('',(111.281142256204,2.2,65.5569535303645));
#189638=CARTESIAN_POINT('',(111.339935449923,2.2,65.2544902788798));
#189639=CARTESIAN_POINT('Origin',(116.959178380441,2.2,51.0204257716897));
#189640=CARTESIAN_POINT('Origin',(112.266622275998,2.2,63.107532568339));
#189641=CARTESIAN_POINT('',(111.830114881284,2.7,65.3531572325288));
#189642=CARTESIAN_POINT('',(111.771334410325,2.7,65.6555550314119));
#189643=CARTESIAN_POINT('',(111.830114881284,2.7,65.3531572325288));
#189644=CARTESIAN_POINT('Origin',(114.701436268713,1.45439216225896E-14,
50.5815629720231));
#189645=CARTESIAN_POINT('Origin',(114.701436268713,1.45439216225896E-14,
50.5815629720231));
#189646=CARTESIAN_POINT('Origin',(112.266622275998,2.7,63.107532568339));
#189647=CARTESIAN_POINT('',(111.355514181256,2.7,65.1743450539802));
#189648=CARTESIAN_POINT('',(111.296406675647,2.7,65.4784252918939));
#189649=CARTESIAN_POINT('',(111.355514181256,2.7,65.1743450539802));
#189650=CARTESIAN_POINT('Origin',(116.959178380441,2.7,51.0204257716897));
#189651=CARTESIAN_POINT('Origin',(116.959178380441,2.7,51.0204257716897));
#189652=CARTESIAN_POINT('Origin',(111.775808773449,2.7,63.0121276118898));
#189653=CARTESIAN_POINT('Origin',(114.210622766164,1.45439216225896E-14,
50.4861580155739));
#189654=CARTESIAN_POINT('Origin',(114.210622766164,1.45439216225896E-14,
50.4861580155739));
#189655=CARTESIAN_POINT('Origin',(111.775808773449,3.2,63.0121276118898));
#189656=CARTESIAN_POINT('',(111.848879229412,3.2,65.2566235117408));
#189657=CARTESIAN_POINT('',(111.789719927259,3.2,65.5609702184402));
#189658=CARTESIAN_POINT('',(111.848879229412,3.2,65.2566235117408));
#189659=CARTESIAN_POINT('',(111.374385790137,3.2,65.0772595272087));
#189660=CARTESIAN_POINT('Origin',(116.959178380441,3.2,51.0204257716897));
#189661=CARTESIAN_POINT('',(111.314893052466,3.2,65.3833216023821));
#189662=CARTESIAN_POINT('',(111.374385790137,3.2,65.0772595272087));
#189663=CARTESIAN_POINT('Origin',(116.959178380441,3.2,51.0204257716897));
#189664=CARTESIAN_POINT('Origin',(112.266622275998,3.2,63.107532568339));
#189665=CARTESIAN_POINT('',(111.870981781604,3.7,65.1429163055294));
#189666=CARTESIAN_POINT('',(111.811370007496,3.7,65.4495907670216));
#189667=CARTESIAN_POINT('',(111.870981781604,3.7,65.1429163055294));
#189668=CARTESIAN_POINT('Origin',(114.701436268713,1.45439216225896E-14,
50.5815629720231));
#189669=CARTESIAN_POINT('Origin',(114.701436268713,1.45439216225896E-14,
50.5815629720231));
#189670=CARTESIAN_POINT('Origin',(112.266622275998,3.7,63.107532568339));
#189671=CARTESIAN_POINT('',(111.396616525,3.7,64.9628928816151));
#189672=CARTESIAN_POINT('',(111.336663560482,3.7,65.2713226068464));
#189673=CARTESIAN_POINT('',(111.396616525,3.7,64.9628928816151));
#189674=CARTESIAN_POINT('Origin',(116.959178380441,3.7,51.0204257716897));
#189675=CARTESIAN_POINT('Origin',(116.959178380441,3.7,51.0204257716897));
#189676=CARTESIAN_POINT('Origin',(111.775808773449,3.7,63.0121276118898));
#189677=CARTESIAN_POINT('Origin',(114.210622766164,1.45439216225896E-14,
50.4861580155739));
#189678=CARTESIAN_POINT('Origin',(114.210622766164,1.45439216225896E-14,
50.4861580155739));
#189679=CARTESIAN_POINT('Origin',(112.757435778548,3.2,63.2029375247883));
#189680=CARTESIAN_POINT('',(112.807623831785,3.2,65.5651525940272));
#189681=CARTESIAN_POINT('',(112.748925857912,3.2,65.8671259843151));
#189682=CARTESIAN_POINT('',(112.807623831785,3.2,65.5651525940272));
#189683=CARTESIAN_POINT('',(112.326640075344,3.2,65.4191782301113));
#189684=CARTESIAN_POINT('Origin',(116.959178380441,3.2,51.0204257716897));
#189685=CARTESIAN_POINT('',(112.267744801195,3.2,65.7221666372604));
#189686=CARTESIAN_POINT('',(112.326640075344,3.2,65.4191782301113));
#189687=CARTESIAN_POINT('Origin',(116.959178380441,3.2,51.0204257716897));
#189688=CARTESIAN_POINT('Origin',(113.248249281097,3.2,63.2983424812375));
#189689=CARTESIAN_POINT('',(112.82954913754,3.7,65.4523572371316));
#189690=CARTESIAN_POINT('',(112.770409275048,3.7,65.7566039359465));
#189691=CARTESIAN_POINT('',(112.82954913754,3.7,65.4523572371316));
#189692=CARTESIAN_POINT('Origin',(115.683063273812,1.45439216225896E-14,
50.7723728849216));
#189693=CARTESIAN_POINT('Origin',(115.683063273812,1.45439216225896E-14,
50.7723728849216));
#189694=CARTESIAN_POINT('Origin',(113.248249281097,3.7,63.2983424812375));
#189695=CARTESIAN_POINT('',(112.348641171179,3.7,65.305992969006));
#189696=CARTESIAN_POINT('',(112.289299502814,3.7,65.6112778638504));
#189697=CARTESIAN_POINT('',(112.348641171179,3.7,65.305992969006));
#189698=CARTESIAN_POINT('Origin',(116.959178380441,3.7,51.0204257716897));
#189699=CARTESIAN_POINT('Origin',(116.959178380441,3.7,51.0204257716897));
#189700=CARTESIAN_POINT('Origin',(112.757435778548,3.7,63.2029375247883));
#189701=CARTESIAN_POINT('Origin',(115.192249771263,1.45439216225896E-14,
50.6769679284724));
#189702=CARTESIAN_POINT('Origin',(115.192249771263,1.45439216225896E-14,
50.6769679284724));
#189703=CARTESIAN_POINT('Origin',(113.739062783647,3.2,63.3937474376868));
#189704=CARTESIAN_POINT('',(113.779139125086,3.2,65.8079824948715));
#189705=CARTESIAN_POINT('',(113.72064275009,3.2,66.1089187540186));
#189706=CARTESIAN_POINT('',(113.779139125086,3.2,65.8079824948715));
#189707=CARTESIAN_POINT('',(113.291797521939,3.2,65.6947162535388));
#189708=CARTESIAN_POINT('Origin',(116.959178380441,3.2,51.0204257716897));
#189709=CARTESIAN_POINT('',(113.233232081845,3.2,65.9960078200407));
#189710=CARTESIAN_POINT('',(113.291797521939,3.2,65.6947162535388));
#189711=CARTESIAN_POINT('Origin',(116.959178380441,3.2,51.0204257716897));
#189712=CARTESIAN_POINT('Origin',(114.229876286196,3.2,63.489152394136));
#189713=CARTESIAN_POINT('',(113.800987011728,3.7,65.6955854227966));
#189714=CARTESIAN_POINT('',(113.742053320085,3.7,65.9987714698337));
#189715=CARTESIAN_POINT('',(113.800987011728,3.7,65.6955854227966));
#189716=CARTESIAN_POINT('Origin',(116.664690278911,1.45439216225896E-14,
50.9631827978201));
#189717=CARTESIAN_POINT('Origin',(116.664690278911,1.45439216225896E-14,
50.9631827978201));
#189718=CARTESIAN_POINT('Origin',(114.229876286196,3.7,63.489152394136));
#189719=CARTESIAN_POINT('',(113.31367192882,3.7,65.582182747345));
#189720=CARTESIAN_POINT('',(113.254667609391,3.7,65.8857321410265));
#189721=CARTESIAN_POINT('',(113.31367192882,3.7,65.582182747345));
#189722=CARTESIAN_POINT('Origin',(116.959178380441,3.7,51.0204257716897));
#189723=CARTESIAN_POINT('Origin',(116.959178380441,3.7,51.0204257716897));
#189724=CARTESIAN_POINT('Origin',(113.739062783647,3.7,63.3937474376868));
#189725=CARTESIAN_POINT('Origin',(116.173876776362,1.45439216225896E-14,
50.8677778413709));
#189726=CARTESIAN_POINT('Origin',(116.173876776362,1.45439216225896E-14,
50.8677778413709));
#189727=CARTESIAN_POINT('Origin',(114.720689788746,3.2,63.5845573505853));
#189728=CARTESIAN_POINT('',(114.763290733282,3.2,65.9858045155801));
#189729=CARTESIAN_POINT('',(114.704744153384,3.2,66.2869990552712));
#189730=CARTESIAN_POINT('',(114.763290733282,3.2,65.9858045155801));
#189731=CARTESIAN_POINT('',(114.269637207538,3.2,65.905010138951));
#189732=CARTESIAN_POINT('Origin',(116.959178380441,3.2,51.0204257716897));
#189733=CARTESIAN_POINT('',(114.211147099076,3.2,66.2059141597396));
#189734=CARTESIAN_POINT('',(114.269637207538,3.2,65.905010138951));
#189735=CARTESIAN_POINT('Origin',(116.959178380441,3.2,51.0204257716897));
#189736=CARTESIAN_POINT('Origin',(115.211503291295,3.2,63.6799623070345));
#189737=CARTESIAN_POINT('',(114.785157897793,3.7,65.873308267962));
#189738=CARTESIAN_POINT('',(114.726172865673,3.7,66.1767584375391));
#189739=CARTESIAN_POINT('',(114.785157897793,3.7,65.873308267962));
#189740=CARTESIAN_POINT('Origin',(117.64631728401,1.45439216225896E-14,
51.1539927107186));
#189741=CARTESIAN_POINT('Origin',(117.64631728401,1.45439216225896E-14,
51.1539927107186));
#189742=CARTESIAN_POINT('Origin',(115.211503291295,3.7,63.6799623070345));
#189743=CARTESIAN_POINT('',(114.291482688029,3.7,65.792625445389));
#189744=CARTESIAN_POINT('',(114.232555404523,3.7,66.0957785255825));
#189745=CARTESIAN_POINT('',(114.291482688029,3.7,65.792625445389));
#189746=CARTESIAN_POINT('Origin',(116.959178380441,3.7,51.0204257716897));
#189747=CARTESIAN_POINT('Origin',(116.959178380441,3.7,51.0204257716897));
#189748=CARTESIAN_POINT('Origin',(114.720689788746,3.7,63.5845573505853));
#189749=CARTESIAN_POINT('Origin',(117.155503781461,1.45439216225896E-14,
51.0585877542694));
#189750=CARTESIAN_POINT('Origin',(117.155503781461,1.45439216225896E-14,
51.0585877542694));
#189751=CARTESIAN_POINT('Origin',(115.702316793845,3.2,63.7753672634838));
#189752=CARTESIAN_POINT('',(115.760112028091,3.2,66.0984469744097));
#189753=CARTESIAN_POINT('',(115.701261479518,3.2,66.401205289563));
#189754=CARTESIAN_POINT('',(115.760112028091,3.2,66.0984469744097));
#189755=CARTESIAN_POINT('',(115.260109046897,3.2,66.0503175513039));
#189756=CARTESIAN_POINT('Origin',(116.959178380441,3.2,51.0204257716897));
#189757=CARTESIAN_POINT('',(115.201442710298,3.2,66.3521281827397));
#189758=CARTESIAN_POINT('',(115.260109046897,3.2,66.0503175513039));
#189759=CARTESIAN_POINT('Origin',(116.959178380441,3.2,51.0204257716897));
#189760=CARTESIAN_POINT('Origin',(116.193130296394,3.2,63.870772219933));
#189761=CARTESIAN_POINT('',(115.782095941346,3.7,65.985350109572));
#189762=CARTESIAN_POINT('',(115.722800022625,3.7,66.2903996440776));
#189763=CARTESIAN_POINT('',(115.782095941346,3.7,65.985350109572));
#189764=CARTESIAN_POINT('Origin',(118.62794428911,1.45439216225896E-14,
51.3448026236171));
#189765=CARTESIAN_POINT('Origin',(118.62794428911,1.45439216225896E-14,
51.3448026236171));
#189766=CARTESIAN_POINT('Origin',(116.193130296394,3.7,63.870772219933));
#189767=CARTESIAN_POINT('',(115.282022201653,3.7,65.9375847055742));
#189768=CARTESIAN_POINT('',(115.222914696043,3.7,66.2416649434879));
#189769=CARTESIAN_POINT('',(115.282022201653,3.7,65.9375847055742));
#189770=CARTESIAN_POINT('Origin',(116.959178380441,3.7,51.0204257716897));
#189771=CARTESIAN_POINT('Origin',(116.959178380441,3.7,51.0204257716897));
#189772=CARTESIAN_POINT('Origin',(115.702316793845,3.7,63.7753672634838));
#189773=CARTESIAN_POINT('Origin',(118.13713078656,1.45439216225896E-14,
51.2493976671679));
#189774=CARTESIAN_POINT('Origin',(118.13713078656,1.45439216225896E-14,
51.2493976671679));
#189775=CARTESIAN_POINT('Origin',(116.683943798944,3.2,63.9661771763823));
#189776=CARTESIAN_POINT('',(116.76980637141,3.2,66.1448636703097));
#189777=CARTESIAN_POINT('',(116.710386028075,3.2,66.4505533107689));
#189778=CARTESIAN_POINT('',(116.76980637141,3.2,66.1448636703097));
#189779=CARTESIAN_POINT('',(116.263330423862,3.2,66.1300346060814));
#189780=CARTESIAN_POINT('Origin',(116.959178380441,3.2,51.0204257716897));
#189781=CARTESIAN_POINT('',(116.204229383259,3.2,66.4340815845874));
#189782=CARTESIAN_POINT('',(116.263330423862,3.2,66.1300346060814));
#189783=CARTESIAN_POINT('Origin',(116.959178380441,3.2,51.0204257716897));
#189784=CARTESIAN_POINT('Origin',(117.174757301493,3.2,64.0615821328315));
#189785=CARTESIAN_POINT('',(116.792009270423,3.7,66.0306402270355));
#189786=CARTESIAN_POINT('',(116.732130391513,3.7,66.3386888167544));
#189787=CARTESIAN_POINT('',(116.792009270423,3.7,66.0306402270355));
#189788=CARTESIAN_POINT('Origin',(119.609571294209,1.45439216225896E-14,
51.5356125365156));
#189789=CARTESIAN_POINT('Origin',(119.609571294209,1.45439216225896E-14,
51.5356125365156));
#189790=CARTESIAN_POINT('Origin',(117.174757301493,3.7,64.0615821328315));
#189791=CARTESIAN_POINT('',(116.285410584927,3.7,66.0164425916591));
#189792=CARTESIAN_POINT('',(116.225858418278,3.7,66.3228104008948));
#189793=CARTESIAN_POINT('',(116.285410584927,3.7,66.0164425916591));
#189794=CARTESIAN_POINT('Origin',(116.959178380441,3.7,51.0204257716897));
#189795=CARTESIAN_POINT('Origin',(116.959178380441,3.7,51.0204257716897));
#189796=CARTESIAN_POINT('Origin',(116.683943798944,3.7,63.9661771763823));
#189797=CARTESIAN_POINT('Origin',(119.118757791659,1.45439216225896E-14,
51.4402075800664));
#189798=CARTESIAN_POINT('Origin',(119.118757791659,1.45439216225896E-14,
51.4402075800664));
#189799=CARTESIAN_POINT('Origin',(117.665570804043,3.2,64.1569870892808));
#189800=CARTESIAN_POINT('',(117.792761072847,3.2,66.1230620780361));
#189801=CARTESIAN_POINT('',(117.732481576534,3.2,66.4331716553377));
#189802=CARTESIAN_POINT('',(117.792761072847,3.2,66.1230620780361));
#189803=CARTESIAN_POINT('',(117.279594132899,3.2,66.1426550138522));
#189804=CARTESIAN_POINT('Origin',(116.959178380441,3.2,51.0204257716897));
#189805=CARTESIAN_POINT('',(117.219782366722,3.2,66.450358340214));
#189806=CARTESIAN_POINT('',(117.279594132899,3.2,66.1426550138522));
#189807=CARTESIAN_POINT('Origin',(116.959178380441,3.2,51.0204257716897));
#189808=CARTESIAN_POINT('Origin',(118.156384306592,3.2,64.25239204573));
#189809=CARTESIAN_POINT('',(117.815294509265,3.7,66.0071381757101));
#189810=CARTESIAN_POINT('',(117.754536133629,3.7,66.3197113612616));
#189811=CARTESIAN_POINT('',(117.815294509265,3.7,66.0071381757101));
#189812=CARTESIAN_POINT('Origin',(120.591198299308,1.45439216225896E-14,
51.7264224494141));
#189813=CARTESIAN_POINT('Origin',(120.591198299308,1.45439216225896E-14,
51.7264224494141));
#189814=CARTESIAN_POINT('Origin',(118.156384306592,3.7,64.25239204573));
#189815=CARTESIAN_POINT('',(117.301947570297,3.7,66.0276571215869));
#189816=CARTESIAN_POINT('',(117.241668073985,3.7,66.3377666988885));
#189817=CARTESIAN_POINT('',(117.301947570297,3.7,66.0276571215869));
#189818=CARTESIAN_POINT('Origin',(116.959178380441,3.7,51.0204257716897));
#189819=CARTESIAN_POINT('Origin',(116.959178380441,3.7,51.0204257716897));
#189820=CARTESIAN_POINT('Origin',(117.665570804043,3.7,64.1569870892808));
#189821=CARTESIAN_POINT('Origin',(120.100384796758,1.45439216225896E-14,
51.6310174929649));
#189822=CARTESIAN_POINT('Origin',(120.100384796758,1.45439216225896E-14,
51.6310174929649));
#189823=CARTESIAN_POINT('Origin',(117.665570804043,2.2,64.1569870892808));
#189824=CARTESIAN_POINT('',(117.757851092575,2.2,66.3026574610069));
#189825=CARTESIAN_POINT('',(117.698298925926,2.2,66.6090252702425));
#189826=CARTESIAN_POINT('',(117.757851092575,2.2,66.3026574610069));
#189827=CARTESIAN_POINT('',(117.244957428961,2.2,66.3208445189799));
#189828=CARTESIAN_POINT('Origin',(116.959178380441,2.2,51.0204257716897));
#189829=CARTESIAN_POINT('',(117.185856388358,2.2,66.6248914974859));
#189830=CARTESIAN_POINT('',(117.244957428961,2.2,66.3208445189799));
#189831=CARTESIAN_POINT('Origin',(116.959178380441,2.2,51.0204257716897));
#189832=CARTESIAN_POINT('Origin',(118.156384306592,2.2,64.25239204573));
#189833=CARTESIAN_POINT('',(117.773636275522,2.7,66.221450139934));
#189834=CARTESIAN_POINT('',(117.713757396612,2.7,66.5294987296529));
#189835=CARTESIAN_POINT('',(117.773636275522,2.7,66.221450139934));
#189836=CARTESIAN_POINT('Origin',(120.591198299308,1.45439216225896E-14,
51.7264224494141));
#189837=CARTESIAN_POINT('Origin',(120.591198299308,1.45439216225896E-14,
51.7264224494141));
#189838=CARTESIAN_POINT('Origin',(118.156384306592,2.7,64.25239204573));
#189839=CARTESIAN_POINT('',(117.26061987396,2.7,66.2402686267589));
#189840=CARTESIAN_POINT('',(117.201199530625,2.7,66.5459582672182));
#189841=CARTESIAN_POINT('',(117.26061987396,2.7,66.2402686267589));
#189842=CARTESIAN_POINT('Origin',(116.959178380441,2.7,51.0204257716897));
#189843=CARTESIAN_POINT('Origin',(116.959178380441,2.7,51.0204257716897));
#189844=CARTESIAN_POINT('Origin',(117.665570804043,2.7,64.1569870892808));
#189845=CARTESIAN_POINT('Origin',(120.100384796758,1.45439216225896E-14,
51.6310174929649));
#189846=CARTESIAN_POINT('Origin',(120.100384796758,1.45439216225896E-14,
51.6310174929649));
#189847=CARTESIAN_POINT('Origin',(117.665570804043,1.2,64.1569870892808));
#189848=CARTESIAN_POINT('',(117.7360897144,1.2,66.4146094878205));
#189849=CARTESIAN_POINT('',(117.67698220879,1.2,66.7186897257342));
#189850=CARTESIAN_POINT('',(117.7360897144,1.2,66.4146094878205));
#189851=CARTESIAN_POINT('',(117.223363057096,1.2,66.4319373771009));
#189852=CARTESIAN_POINT('Origin',(116.959178380441,1.2,51.0204257716897));
#189853=CARTESIAN_POINT('',(117.164696720496,1.2,66.7337480085367));
#189854=CARTESIAN_POINT('',(117.223363057096,1.2,66.4319373771009));
#189855=CARTESIAN_POINT('Origin',(116.959178380441,1.2,51.0204257716897));
#189856=CARTESIAN_POINT('Origin',(118.156384306592,1.2,64.25239204573));
#189857=CARTESIAN_POINT('',(117.745349951544,1.7,66.366969935369));
#189858=CARTESIAN_POINT('',(117.686054032823,1.7,66.6720194698746));
#189859=CARTESIAN_POINT('',(117.745349951544,1.7,66.366969935369));
#189860=CARTESIAN_POINT('Origin',(120.591198299308,1.45439216225896E-14,
51.7264224494141));
#189861=CARTESIAN_POINT('Origin',(120.591198299308,1.45439216225896E-14,
51.7264224494141));
#189862=CARTESIAN_POINT('Origin',(118.156384306592,1.7,64.25239204573));
#189863=CARTESIAN_POINT('',(117.232552535739,1.7,66.3846618437574));
#189864=CARTESIAN_POINT('',(117.173701987167,1.7,66.6874201589108));
#189865=CARTESIAN_POINT('',(117.232552535739,1.7,66.3846618437574));
#189866=CARTESIAN_POINT('Origin',(116.959178380441,1.7,51.0204257716897));
#189867=CARTESIAN_POINT('Origin',(116.959178380441,1.7,51.0204257716897));
#189868=CARTESIAN_POINT('Origin',(117.665570804043,1.7,64.1569870892808));
#189869=CARTESIAN_POINT('Origin',(120.100384796758,1.45439216225896E-14,
51.6310174929649));
#189870=CARTESIAN_POINT('Origin',(120.100384796758,1.45439216225896E-14,
51.6310174929649));
#189871=CARTESIAN_POINT('Origin',(117.665570804043,0.200000000000015,64.1569870892808));
#189872=CARTESIAN_POINT('',(117.727177205876,0.200000000000015,66.4604601405338));
#189873=CARTESIAN_POINT('',(117.668249922372,0.200000000000015,66.7636132207175));
#189874=CARTESIAN_POINT('',(117.727177205876,0.200000000000015,66.4604601405338));
#189875=CARTESIAN_POINT('',(117.214518222835,0.200000000000015,66.4774398776465));
#189876=CARTESIAN_POINT('Origin',(116.959178380441,0.200000000000015,51.0204257716897));
#189877=CARTESIAN_POINT('',(117.156028114373,0.200000000000015,66.7783438984351));
#189878=CARTESIAN_POINT('',(117.214518222835,0.200000000000015,66.4774398776465));
#189879=CARTESIAN_POINT('Origin',(116.959178380441,0.200000000000015,51.0204257716897));
#189880=CARTESIAN_POINT('Origin',(118.156384306592,0.200000000000015,64.25239204573));
#189881=CARTESIAN_POINT('',(117.73003891309,0.700000000000015,66.4457380066575));
#189882=CARTESIAN_POINT('',(117.67105388097,0.700000000000015,66.7491881762347));
#189883=CARTESIAN_POINT('',(117.73003891309,0.700000000000015,66.4457380066575));
#189884=CARTESIAN_POINT('Origin',(120.591198299308,1.45439216225896E-14,
51.7264224494141));
#189885=CARTESIAN_POINT('Origin',(120.591198299308,1.45439216225896E-14,
51.7264224494141));
#189886=CARTESIAN_POINT('Origin',(118.156384306592,0.700000000000015,64.25239204573));
#189887=CARTESIAN_POINT('',(117.217358246029,0.700000000000015,66.4628292978264));
#189888=CARTESIAN_POINT('',(117.158811666132,0.700000000000015,66.7640238375175));
#189889=CARTESIAN_POINT('',(117.217358246029,0.700000000000015,66.4628292978264));
#189890=CARTESIAN_POINT('Origin',(116.959178380441,0.700000000000015,51.0204257716897));
#189891=CARTESIAN_POINT('Origin',(116.959178380441,0.700000000000015,51.0204257716897));
#189892=CARTESIAN_POINT('Origin',(117.665570804043,0.700000000000015,64.1569870892808));
#189893=CARTESIAN_POINT('Origin',(120.100384796758,1.45439216225896E-14,
51.6310174929649));
#189894=CARTESIAN_POINT('Origin',(120.100384796758,1.45439216225896E-14,
51.6310174929649));
#189895=CARTESIAN_POINT('Origin',(112.757435778548,0.200000000000015,63.2029375247883));
#189896=CARTESIAN_POINT('',(112.743757590842,0.200000000000015,65.8937142807404));
#189897=CARTESIAN_POINT('',(112.686310316266,0.200000000000015,66.1892534130432));
#189898=CARTESIAN_POINT('',(112.743757590842,0.200000000000015,65.8937142807404));
#189899=CARTESIAN_POINT('',(112.262559541475,0.200000000000015,65.7488423528614));
#189900=CARTESIAN_POINT('Origin',(116.959178380441,0.200000000000015,51.0204257716897));
#189901=CARTESIAN_POINT('',(112.204927352587,0.200000000000015,66.0453327820839));
#189902=CARTESIAN_POINT('',(112.262559541475,0.200000000000015,65.7488423528614));
#189903=CARTESIAN_POINT('Origin',(116.959178380441,0.200000000000015,51.0204257716897));
#189904=CARTESIAN_POINT('Origin',(113.248249281097,0.200000000000015,63.2983424812375));
#189905=CARTESIAN_POINT('',(112.746545930485,0.700000000000015,65.8793695884159));
#189906=CARTESIAN_POINT('',(112.689045154583,0.700000000000015,66.1751839598116));
#189907=CARTESIAN_POINT('',(112.746545930485,0.700000000000015,65.8793695884159));
#189908=CARTESIAN_POINT('Origin',(115.683063273812,1.45439216225896E-14,
50.7723728849216));
#189909=CARTESIAN_POINT('Origin',(115.683063273812,1.45439216225896E-14,
50.7723728849216));
#189910=CARTESIAN_POINT('Origin',(113.248249281097,0.700000000000015,63.2983424812375));
#189911=CARTESIAN_POINT('',(112.265357041383,0.700000000000015,65.7344505352944));
#189912=CARTESIAN_POINT('',(112.20767083231,0.700000000000015,66.0312188728892));
#189913=CARTESIAN_POINT('',(112.265357041383,0.700000000000015,65.7344505352944));
#189914=CARTESIAN_POINT('Origin',(116.959178380441,0.700000000000015,51.0204257716897));
#189915=CARTESIAN_POINT('Origin',(116.959178380441,0.700000000000015,51.0204257716897));
#189916=CARTESIAN_POINT('Origin',(112.757435778548,0.700000000000015,63.2029375247883));
#189917=CARTESIAN_POINT('Origin',(115.192249771263,1.45439216225896E-14,
50.6769679284724));
#189918=CARTESIAN_POINT('Origin',(115.192249771263,1.45439216225896E-14,
50.6769679284724));
#189919=CARTESIAN_POINT('Origin',(112.757435778548,1.2,63.2029375247883));
#189920=CARTESIAN_POINT('',(112.752441137483,1.2,65.8490415289272));
#189921=CARTESIAN_POINT('',(112.694826921622,1.2,66.1454394954038));
#189922=CARTESIAN_POINT('',(112.752441137483,1.2,65.8490415289272));
#189923=CARTESIAN_POINT('',(112.271271673005,1.2,65.7040225452736));
#189924=CARTESIAN_POINT('Origin',(116.959178380441,1.2,51.0204257716897));
#189925=CARTESIAN_POINT('',(112.213470920606,1.2,66.0013801542565));
#189926=CARTESIAN_POINT('',(112.271271673005,1.2,65.7040225452736));
#189927=CARTESIAN_POINT('Origin',(116.959178380441,1.2,51.0204257716897));
#189928=CARTESIAN_POINT('Origin',(113.248249281097,1.2,63.2983424812375));
#189929=CARTESIAN_POINT('',(112.761462018886,1.7,65.8026333488664));
#189930=CARTESIAN_POINT('',(112.703673355823,1.7,66.0999287639157));
#189931=CARTESIAN_POINT('',(112.761462018886,1.7,65.8026333488664));
#189932=CARTESIAN_POINT('Origin',(115.683063273812,1.45439216225896E-14,
50.7723728849216));
#189933=CARTESIAN_POINT('Origin',(115.683063273812,1.45439216225896E-14,
50.7723728849216));
#189934=CARTESIAN_POINT('Origin',(113.248249281097,1.7,63.2983424812375));
#189935=CARTESIAN_POINT('',(112.28032243059,1.7,65.657460666346));
#189936=CARTESIAN_POINT('',(112.222345525672,1.7,65.9557244969574));
#189937=CARTESIAN_POINT('',(112.28032243059,1.7,65.657460666346));
#189938=CARTESIAN_POINT('Origin',(116.959178380441,1.7,51.0204257716897));
#189939=CARTESIAN_POINT('Origin',(116.959178380441,1.7,51.0204257716897));
#189940=CARTESIAN_POINT('Origin',(112.757435778548,1.7,63.2029375247883));
#189941=CARTESIAN_POINT('Origin',(115.192249771263,1.45439216225896E-14,
50.6769679284724));
#189942=CARTESIAN_POINT('Origin',(115.192249771263,1.45439216225896E-14,
50.6769679284724));
#189943=CARTESIAN_POINT('Origin',(112.757435778548,2.2,63.2029375247883));
#189944=CARTESIAN_POINT('',(112.773637648674,2.2,65.7399954763229));
#189945=CARTESIAN_POINT('',(112.715611865814,2.2,66.0385107608908));
#189946=CARTESIAN_POINT('',(112.773637648674,2.2,65.7399954763229));
#189947=CARTESIAN_POINT('',(112.292538680002,2.2,65.5946138249966));
#189948=CARTESIAN_POINT('Origin',(116.959178380441,2.2,51.0204257716897));
#189949=CARTESIAN_POINT('',(112.234322320598,2.2,65.8941095360005));
#189950=CARTESIAN_POINT('',(112.292538680002,2.2,65.5946138249966));
#189951=CARTESIAN_POINT('Origin',(116.959178380441,2.2,51.0204257716897));
#189952=CARTESIAN_POINT('Origin',(113.248249281097,2.2,63.2983424812375));
#189953=CARTESIAN_POINT('',(112.78900784376,2.7,65.6609230720582));
#189954=CARTESIAN_POINT('',(112.730679961499,2.7,65.9609925155598));
#189955=CARTESIAN_POINT('',(112.78900784376,2.7,65.6609230720582));
#189956=CARTESIAN_POINT('Origin',(115.683063273812,1.45439216225896E-14,
50.7723728849216));
#189957=CARTESIAN_POINT('Origin',(115.683063273812,1.45439216225896E-14,
50.7723728849216));
#189958=CARTESIAN_POINT('Origin',(113.248249281097,2.7,63.2983424812375));
#189959=CARTESIAN_POINT('',(112.307960642765,2.7,65.5152751004566));
#189960=CARTESIAN_POINT('',(112.249439181471,2.7,65.816340416776));
#189961=CARTESIAN_POINT('',(112.307960642765,2.7,65.5152751004566));
#189962=CARTESIAN_POINT('Origin',(116.959178380441,2.7,51.0204257716897));
#189963=CARTESIAN_POINT('Origin',(116.959178380441,2.7,51.0204257716897));
#189964=CARTESIAN_POINT('Origin',(112.757435778548,2.7,63.2029375247883));
#189965=CARTESIAN_POINT('Origin',(115.192249771263,1.45439216225896E-14,
50.6769679284724));
#189966=CARTESIAN_POINT('Origin',(115.192249771263,1.45439216225896E-14,
50.6769679284724));
#189967=CARTESIAN_POINT('Origin',(113.739062783647,2.2,63.3937474376868));
#189968=CARTESIAN_POINT('',(113.745270654261,2.2,65.9822198029767));
#189969=CARTESIAN_POINT('',(113.687439645288,2.2,66.2797330677587));
#189970=CARTESIAN_POINT('',(113.745270654261,2.2,65.9822198029767));
#189971=CARTESIAN_POINT('',(113.257888725595,2.2,65.8691610174192));
#189972=CARTESIAN_POINT('Origin',(116.959178380441,2.2,51.0204257716897));
#189973=CARTESIAN_POINT('',(113.199990984535,2.2,66.1670175873205));
#189974=CARTESIAN_POINT('',(113.257888725595,2.2,65.8691610174192));
#189975=CARTESIAN_POINT('Origin',(116.959178380441,2.2,51.0204257716897));
#189976=CARTESIAN_POINT('Origin',(114.229876286196,2.2,63.489152394136));
#189977=CARTESIAN_POINT('',(113.760587954822,2.7,65.9034195160936));
#189978=CARTESIAN_POINT('',(113.702457894475,2.7,66.2024712591523));
#189979=CARTESIAN_POINT('',(113.760587954822,2.7,65.9034195160936));
#189980=CARTESIAN_POINT('Origin',(116.664690278911,1.45439216225896E-14,
50.9631827978201));
#189981=CARTESIAN_POINT('Origin',(116.664690278911,1.45439216225896E-14,
50.9631827978201));
#189982=CARTESIAN_POINT('Origin',(114.229876286196,2.7,63.489152394136));
#189983=CARTESIAN_POINT('',(113.273224147002,2.7,65.7902675073336));
#189984=CARTESIAN_POINT('',(113.215026312613,2.7,66.0896679158723));
#189985=CARTESIAN_POINT('',(113.273224147002,2.7,65.7902675073336));
#189986=CARTESIAN_POINT('Origin',(116.959178380441,2.7,51.0204257716897));
#189987=CARTESIAN_POINT('Origin',(116.959178380441,2.7,51.0204257716897));
#189988=CARTESIAN_POINT('Origin',(113.739062783647,2.7,63.3937474376868));
#189989=CARTESIAN_POINT('Origin',(116.173876776362,1.45439216225896E-14,
50.8677778413709));
#189990=CARTESIAN_POINT('Origin',(116.173876776362,1.45439216225896E-14,
50.8677778413709));
#189991=CARTESIAN_POINT('Origin',(114.720689788746,2.2,63.5845573505853));
#189992=CARTESIAN_POINT('',(114.729392949091,2.2,66.1601926271255));
#189993=CARTESIAN_POINT('',(114.671513430601,2.2,66.4579554504992));
#189994=CARTESIAN_POINT('',(114.729392949091,2.2,66.1601926271255));
#189995=CARTESIAN_POINT('',(114.235772395539,2.2,66.0792286241228));
#189996=CARTESIAN_POINT('Origin',(116.959178380441,2.2,51.0204257716897));
#189997=CARTESIAN_POINT('',(114.177947441683,2.2,66.3767107381891));
#189998=CARTESIAN_POINT('',(114.235772395539,2.2,66.0792286241228));
#189999=CARTESIAN_POINT('Origin',(116.959178380441,2.2,51.0204257716897));
#190000=CARTESIAN_POINT('Origin',(115.211503291295,2.2,63.6799623070345));
#190001=CARTESIAN_POINT('',(114.744723422072,2.7,66.0813245743583));
#190002=CARTESIAN_POINT('',(114.686544095021,2.7,66.3806297713697));
#190003=CARTESIAN_POINT('',(114.744723422072,2.7,66.0813245743583));
#190004=CARTESIAN_POINT('Origin',(117.64631728401,1.45439216225896E-14,
51.1539927107186));
#190005=CARTESIAN_POINT('Origin',(117.64631728401,1.45439216225896E-14,
51.1539927107186));
#190006=CARTESIAN_POINT('Origin',(115.211503291295,2.7,63.6799623070345));
#190007=CARTESIAN_POINT('',(114.251088051933,2.7,66.0004367957037));
#190008=CARTESIAN_POINT('',(114.192964141128,2.7,66.2994569022688));
#190009=CARTESIAN_POINT('',(114.251088051933,2.7,66.0004367957037));
#190010=CARTESIAN_POINT('Origin',(116.959178380441,2.7,51.0204257716897));
#190011=CARTESIAN_POINT('Origin',(116.959178380441,2.7,51.0204257716897));
#190012=CARTESIAN_POINT('Origin',(114.720689788746,2.7,63.5845573505853));
#190013=CARTESIAN_POINT('Origin',(117.155503781461,1.45439216225896E-14,
51.0585877542694));
#190014=CARTESIAN_POINT('Origin',(117.155503781461,1.45439216225896E-14,
51.0585877542694));
#190015=CARTESIAN_POINT('Origin',(115.702316793845,2.2,63.7753672634838));
#190016=CARTESIAN_POINT('',(115.726036750819,2.2,66.2737482041414));
#190017=CARTESIAN_POINT('',(115.66786358896,2.2,66.5730216841463));
#190018=CARTESIAN_POINT('',(115.726036750819,2.2,66.2737482041414));
#190019=CARTESIAN_POINT('',(115.22614133726,2.2,66.2250653962915));
#190020=CARTESIAN_POINT('Origin',(116.959178380441,2.2,51.0204257716897));
#190021=CARTESIAN_POINT('',(115.168146117596,2.2,66.5234234476348));
#190022=CARTESIAN_POINT('',(115.22614133726,2.2,66.2250653962915));
#190023=CARTESIAN_POINT('Origin',(116.959178380441,2.2,51.0204257716897));
#190024=CARTESIAN_POINT('Origin',(116.193130296394,2.2,63.870772219933));
#190025=CARTESIAN_POINT('',(115.741446978392,2.7,66.1944698516157));
#190026=CARTESIAN_POINT('',(115.682969396959,2.7,66.4953094267459));
#190027=CARTESIAN_POINT('',(115.741446978392,2.7,66.1944698516157));
#190028=CARTESIAN_POINT('Origin',(118.62794428911,1.45439216225896E-14,
51.3448026236171));
#190029=CARTESIAN_POINT('Origin',(118.62794428911,1.45439216225896E-14,
51.3448026236171));
#190030=CARTESIAN_POINT('Origin',(116.193130296394,2.7,63.870772219933));
#190031=CARTESIAN_POINT('',(115.241503231448,2.7,66.1460356962372));
#190032=CARTESIAN_POINT('',(115.183206392039,2.7,66.4459454389002));
#190033=CARTESIAN_POINT('',(115.241503231448,2.7,66.1460356962372));
#190034=CARTESIAN_POINT('Origin',(116.959178380441,2.7,51.0204257716897));
#190035=CARTESIAN_POINT('Origin',(116.959178380441,2.7,51.0204257716897));
#190036=CARTESIAN_POINT('Origin',(115.702316793845,2.7,63.7753672634838));
#190037=CARTESIAN_POINT('Origin',(118.13713078656,1.45439216225896E-14,
51.2493976671679));
#190038=CARTESIAN_POINT('Origin',(118.13713078656,1.45439216225896E-14,
51.2493976671679));
#190039=CARTESIAN_POINT('Origin',(116.683943798944,2.2,63.9661771763823));
#190040=CARTESIAN_POINT('',(116.735398317472,2.2,66.321876879036));
#190041=CARTESIAN_POINT('',(116.676674996893,2.2,66.6239806661718));
#190042=CARTESIAN_POINT('',(116.735398317472,2.2,66.321876879036));
#190043=CARTESIAN_POINT('',(116.229108862081,2.2,66.306088400618));
#190044=CARTESIAN_POINT('Origin',(116.959178380441,2.2,51.0204257716897));
#190045=CARTESIAN_POINT('',(116.170693795267,2.2,66.6066063675209));
#190046=CARTESIAN_POINT('',(116.229108862081,2.2,66.306088400618));
#190047=CARTESIAN_POINT('Origin',(116.959178380441,2.2,51.0204257716897));
#190048=CARTESIAN_POINT('Origin',(117.174757301493,2.2,64.0615821328315));
#190049=CARTESIAN_POINT('',(116.750958052759,2.7,66.2418293798362));
#190050=CARTESIAN_POINT('',(116.691921545728,2.7,66.5455443635489));
#190051=CARTESIAN_POINT('',(116.750958052759,2.7,66.2418293798362));
#190052=CARTESIAN_POINT('Origin',(119.609571294209,1.45439216225896E-14,
51.5356125365156));
#190053=CARTESIAN_POINT('Origin',(119.609571294209,1.45439216225896E-14,
51.5356125365156));
#190054=CARTESIAN_POINT('Origin',(117.174757301493,2.7,64.0615821328315));
#190055=CARTESIAN_POINT('',(116.244584814922,2.7,66.2264719225867));
#190056=CARTESIAN_POINT('',(116.185861494343,2.7,66.5285757097225));
#190057=CARTESIAN_POINT('',(116.244584814922,2.7,66.2264719225867));
#190058=CARTESIAN_POINT('Origin',(116.959178380441,2.7,51.0204257716897));
#190059=CARTESIAN_POINT('Origin',(116.959178380441,2.7,51.0204257716897));
#190060=CARTESIAN_POINT('Origin',(116.683943798944,2.7,63.9661771763823));
#190061=CARTESIAN_POINT('Origin',(119.118757791659,1.45439216225896E-14,
51.4402075800664));
#190062=CARTESIAN_POINT('Origin',(119.118757791659,1.45439216225896E-14,
51.4402075800664));
#190063=CARTESIAN_POINT('Origin',(116.683943798944,1.2,63.9661771763823));
#190064=CARTESIAN_POINT('',(116.713943739096,1.2,66.432250565585));
#190065=CARTESIAN_POINT('',(116.655646899688,1.2,66.732160308248));
#190066=CARTESIAN_POINT('',(116.713943739096,1.2,66.432250565585));
#190067=CARTESIAN_POINT('',(116.207768342359,1.2,66.41587530919));
#190068=CARTESIAN_POINT('Origin',(116.959178380441,1.2,51.0204257716897));
#190069=CARTESIAN_POINT('',(116.149773122695,1.2,66.7142333605333));
#190070=CARTESIAN_POINT('',(116.207768342359,1.2,66.41587530919));
#190071=CARTESIAN_POINT('Origin',(116.959178380441,1.2,51.0204257716897));
#190072=CARTESIAN_POINT('Origin',(117.174757301493,1.2,64.0615821328315));
#190073=CARTESIAN_POINT('',(116.723073983491,1.7,66.3852797645142));
#190074=CARTESIAN_POINT('',(116.664596402058,1.7,66.6861193396444));
#190075=CARTESIAN_POINT('',(116.723073983491,1.7,66.3852797645142));
#190076=CARTESIAN_POINT('Origin',(119.609571294209,1.45439216225896E-14,
51.5356125365156));
#190077=CARTESIAN_POINT('Origin',(119.609571294209,1.45439216225896E-14,
51.5356125365156));
#190078=CARTESIAN_POINT('Origin',(117.174757301493,1.7,64.0615821328315));
#190079=CARTESIAN_POINT('',(116.216850253369,1.7,66.3691531605907));
#190080=CARTESIAN_POINT('',(116.15867709151,1.7,66.6684266405955));
#190081=CARTESIAN_POINT('',(116.216850253369,1.7,66.3691531605907));
#190082=CARTESIAN_POINT('Origin',(116.959178380441,1.7,51.0204257716897));
#190083=CARTESIAN_POINT('Origin',(116.959178380441,1.7,51.0204257716897));
#190084=CARTESIAN_POINT('Origin',(116.683943798944,1.7,63.9661771763823));
#190085=CARTESIAN_POINT('Origin',(119.118757791659,1.45439216225896E-14,
51.4402075800664));
#190086=CARTESIAN_POINT('Origin',(119.118757791659,1.45439216225896E-14,
51.4402075800664));
#190087=CARTESIAN_POINT('Origin',(116.683943798944,0.200000000000015,63.9661771763823));
#190088=CARTESIAN_POINT('',(116.705155564681,0.200000000000015,66.47746157795));
#190089=CARTESIAN_POINT('',(116.647031653875,0.200000000000015,66.7764816845151));
#190090=CARTESIAN_POINT('',(116.705155564681,0.200000000000015,66.47746157795));
#190091=CARTESIAN_POINT('',(116.199026405737,0.200000000000015,66.4608484499199));
#190092=CARTESIAN_POINT('Origin',(116.959178380441,0.200000000000015,51.0204257716897));
#190093=CARTESIAN_POINT('',(116.141201451881,0.200000000000015,66.7583305639861));
#190094=CARTESIAN_POINT('',(116.199026405737,0.200000000000015,66.4608484499199));
#190095=CARTESIAN_POINT('Origin',(116.959178380441,0.200000000000015,51.0204257716897));
#190096=CARTESIAN_POINT('Origin',(117.174757301493,0.200000000000015,64.0615821328315));
#190097=CARTESIAN_POINT('',(116.70797743227,0.700000000000015,66.4629444001553));
#190098=CARTESIAN_POINT('',(116.649798105219,0.700000000000015,66.7622495971667));
#190099=CARTESIAN_POINT('',(116.70797743227,0.700000000000015,66.4629444001553));
#190100=CARTESIAN_POINT('Origin',(119.609571294209,1.45439216225896E-14,
51.5356125365156));
#190101=CARTESIAN_POINT('Origin',(119.609571294209,1.45439216225896E-14,
51.5356125365156));
#190102=CARTESIAN_POINT('Origin',(117.174757301493,0.700000000000015,64.0615821328315));
#190103=CARTESIAN_POINT('',(116.20183345674,0.700000000000015,66.4464074964732));
#190104=CARTESIAN_POINT('',(116.143953938249,0.700000000000015,66.744170319847));
#190105=CARTESIAN_POINT('',(116.20183345674,0.700000000000015,66.4464074964732));
#190106=CARTESIAN_POINT('Origin',(116.959178380441,0.700000000000015,51.0204257716897));
#190107=CARTESIAN_POINT('Origin',(116.959178380441,0.700000000000015,51.0204257716897));
#190108=CARTESIAN_POINT('Origin',(116.683943798944,0.700000000000015,63.9661771763823));
#190109=CARTESIAN_POINT('Origin',(119.118757791659,1.45439216225896E-14,
51.4402075800664));
#190110=CARTESIAN_POINT('Origin',(119.118757791659,1.45439216225896E-14,
51.4402075800664));
#190111=CARTESIAN_POINT('Origin',(113.739062783647,0.200000000000015,63.3937474376868));
#190112=CARTESIAN_POINT('',(113.715491849759,0.200000000000015,66.1354177067687));
#190113=CARTESIAN_POINT('',(113.658233599506,0.200000000000015,66.4299843980828));
#190114=CARTESIAN_POINT('',(113.715491849759,0.200000000000015,66.1354177067687));
#190115=CARTESIAN_POINT('',(113.22807523146,0.200000000000015,66.022537383013));
#190116=CARTESIAN_POINT('Origin',(116.959178380441,0.200000000000015,51.0204257716897));
#190117=CARTESIAN_POINT('',(113.170752214749,0.200000000000015,66.317437267206));
#190118=CARTESIAN_POINT('',(113.22807523146,0.200000000000015,66.022537383013));
#190119=CARTESIAN_POINT('Origin',(116.959178380441,0.200000000000015,51.0204257716897));
#190120=CARTESIAN_POINT('Origin',(114.229876286196,0.200000000000015,63.489152394136));
#190121=CARTESIAN_POINT('',(113.718270827401,0.700000000000015,66.1211211775216));
#190122=CARTESIAN_POINT('',(113.66095960276,0.700000000000015,66.4159603970774));
#190123=CARTESIAN_POINT('',(113.718270827401,0.700000000000015,66.1211211775216));
#190124=CARTESIAN_POINT('Origin',(116.664690278911,1.45439216225896E-14,
50.9631827978201));
#190125=CARTESIAN_POINT('Origin',(116.664690278911,1.45439216225896E-14,
50.9631827978201));
#190126=CARTESIAN_POINT('Origin',(114.229876286196,0.700000000000015,63.489152394136));
#190127=CARTESIAN_POINT('',(113.230857416645,0.700000000000015,66.0082243524688));
#190128=CARTESIAN_POINT('',(113.17348124539,0.700000000000015,66.3033976917261));
#190129=CARTESIAN_POINT('',(113.230857416645,0.700000000000015,66.0082243524688));
#190130=CARTESIAN_POINT('Origin',(116.959178380441,0.700000000000015,51.0204257716897));
#190131=CARTESIAN_POINT('Origin',(116.959178380441,0.700000000000015,51.0204257716897));
#190132=CARTESIAN_POINT('Origin',(113.739062783647,0.700000000000015,63.3937474376868));
#190133=CARTESIAN_POINT('Origin',(116.173876776362,1.45439216225896E-14,
50.8677778413709));
#190134=CARTESIAN_POINT('Origin',(116.173876776362,1.45439216225896E-14,
50.8677778413709));
#190135=CARTESIAN_POINT('Origin',(113.739062783647,1.2,63.3937474376868));
#190136=CARTESIAN_POINT('',(113.724146182571,1.2,66.0908952463201));
#190137=CARTESIAN_POINT('',(113.666722638469,1.2,66.3863122965288));
#190138=CARTESIAN_POINT('',(113.724146182571,1.2,66.0908952463201));
#190139=CARTESIAN_POINT('',(113.236739573243,1.2,65.9779634311333));
#190140=CARTESIAN_POINT('Origin',(116.959178380441,1.2,51.0204257716897));
#190141=CARTESIAN_POINT('',(113.179250699444,1.2,66.273716571817));
#190142=CARTESIAN_POINT('',(113.236739573243,1.2,65.9779634311333));
#190143=CARTESIAN_POINT('Origin',(116.959178380441,1.2,51.0204257716897));
#190144=CARTESIAN_POINT('Origin',(114.229876286196,1.2,63.489152394136));
#190145=CARTESIAN_POINT('',(113.733136532284,1.7,66.0446441374075));
#190146=CARTESIAN_POINT('',(113.675540272641,1.7,66.3409497276097));
#190147=CARTESIAN_POINT('',(113.733136532284,1.7,66.0446441374075));
#190148=CARTESIAN_POINT('Origin',(116.664690278911,1.45439216225896E-14,
50.9631827978201));
#190149=CARTESIAN_POINT('Origin',(116.664690278911,1.45439216225896E-14,
50.9631827978201));
#190150=CARTESIAN_POINT('Origin',(114.229876286196,1.7,63.489152394136));
#190151=CARTESIAN_POINT('',(113.245740383227,1.7,65.9316585090553));
#190152=CARTESIAN_POINT('',(113.188078201874,1.7,66.2283032353676));
#190153=CARTESIAN_POINT('',(113.245740383227,1.7,65.9316585090553));
#190154=CARTESIAN_POINT('Origin',(116.959178380441,1.7,51.0204257716897));
#190155=CARTESIAN_POINT('Origin',(116.959178380441,1.7,51.0204257716897));
#190156=CARTESIAN_POINT('Origin',(113.739062783647,1.7,63.3937474376868));
#190157=CARTESIAN_POINT('Origin',(116.173876776362,1.45439216225896E-14,
50.8677778413709));
#190158=CARTESIAN_POINT('Origin',(116.173876776362,1.45439216225896E-14,
50.8677778413709));
#190159=CARTESIAN_POINT('Origin',(114.720689788746,1.2,63.5845573505853));
#190160=CARTESIAN_POINT('',(114.708250536407,1.2,66.268960368429));
#190161=CARTESIAN_POINT('',(114.65077950191,1.2,66.5646217343204));
#190162=CARTESIAN_POINT('',(114.708250536407,1.2,66.268960368429));
#190163=CARTESIAN_POINT('',(114.214650163263,1.2,66.1878925467383));
#190164=CARTESIAN_POINT('Origin',(116.959178380441,1.2,51.0204257716897));
#190165=CARTESIAN_POINT('',(114.157232547186,1.2,66.4832791000537));
#190166=CARTESIAN_POINT('',(114.214650163263,1.2,66.1878925467383));
#190167=CARTESIAN_POINT('Origin',(116.959178380441,1.2,51.0204257716897));
#190168=CARTESIAN_POINT('Origin',(115.211503291295,1.2,63.6799623070345));
#190169=CARTESIAN_POINT('',(114.717248489969,1.7,66.2226701412973));
#190170=CARTESIAN_POINT('',(114.659604309712,1.7,66.5192222604567));
#190171=CARTESIAN_POINT('',(114.717248489969,1.7,66.2226701412973));
#190172=CARTESIAN_POINT('Origin',(117.64631728401,1.45439216225896E-14,
51.1539927107186));
#190173=CARTESIAN_POINT('Origin',(117.64631728401,1.45439216225896E-14,
51.1539927107186));
#190174=CARTESIAN_POINT('Origin',(115.211503291295,1.7,63.6799623070345));
#190175=CARTESIAN_POINT('',(114.223639563849,1.7,66.1416463206347));
#190176=CARTESIAN_POINT('',(114.166049285884,1.7,66.4379211379298));
#190177=CARTESIAN_POINT('',(114.223639563849,1.7,66.1416463206347));
#190178=CARTESIAN_POINT('Origin',(116.959178380441,1.7,51.0204257716897));
#190179=CARTESIAN_POINT('Origin',(116.959178380441,1.7,51.0204257716897));
#190180=CARTESIAN_POINT('Origin',(114.720689788746,1.7,63.5845573505853));
#190181=CARTESIAN_POINT('Origin',(117.155503781461,1.45439216225896E-14,
51.0585877542694));
#190182=CARTESIAN_POINT('Origin',(117.155503781461,1.45439216225896E-14,
51.0585877542694));
#190183=CARTESIAN_POINT('Origin',(115.702316793845,1.2,63.7753672634838));
#190184=CARTESIAN_POINT('',(115.704785723703,1.2,66.3830747154636));
#190185=CARTESIAN_POINT('',(115.647027250828,1.2,66.6802148162415));
#190186=CARTESIAN_POINT('',(115.704785723703,1.2,66.3830747154636));
#190187=CARTESIAN_POINT('',(115.204956130839,1.2,66.3340532911867));
#190188=CARTESIAN_POINT('Origin',(116.959178380441,1.2,51.0204257716897));
#190189=CARTESIAN_POINT('',(115.147371832686,1.2,66.630297345165));
#190190=CARTESIAN_POINT('',(115.204956130839,1.2,66.3340532911867));
#190191=CARTESIAN_POINT('Origin',(116.959178380441,1.2,51.0204257716897));
#190192=CARTESIAN_POINT('Origin',(116.193130296394,1.2,63.870772219933));
#190193=CARTESIAN_POINT('',(115.713829709111,1.7,66.3365476761963));
#190194=CARTESIAN_POINT('',(115.655895471211,1.7,66.6345920051243));
#190195=CARTESIAN_POINT('',(115.713829709111,1.7,66.3365476761963));
#190196=CARTESIAN_POINT('Origin',(118.62794428911,1.45439216225896E-14,
51.3448026236171));
#190197=CARTESIAN_POINT('Origin',(118.62794428911,1.45439216225896E-14,
51.3448026236171));
#190198=CARTESIAN_POINT('Origin',(116.193130296394,1.7,63.870772219933));
#190199=CARTESIAN_POINT('',(115.213972221154,1.7,66.2876697590143));
#190200=CARTESIAN_POINT('',(115.156213748278,1.7,66.5848098597922));
#190201=CARTESIAN_POINT('',(115.213972221154,1.7,66.2876697590143));
#190202=CARTESIAN_POINT('Origin',(116.959178380441,1.7,51.0204257716897));
#190203=CARTESIAN_POINT('Origin',(116.959178380441,1.7,51.0204257716897));
#190204=CARTESIAN_POINT('Origin',(115.702316793845,1.7,63.7753672634838));
#190205=CARTESIAN_POINT('Origin',(118.13713078656,1.45439216225896E-14,
51.2493976671679));
#190206=CARTESIAN_POINT('Origin',(118.13713078656,1.45439216225896E-14,
51.2493976671679));
#190207=CARTESIAN_POINT('Origin',(115.702316793845,0.200000000000015,63.7753672634838));
#190208=CARTESIAN_POINT('',(115.696080071498,0.200000000000015,66.4278611899825));
#190209=CARTESIAN_POINT('',(115.638489793532,0.200000000000015,66.7241360072775));
#190210=CARTESIAN_POINT('',(115.696080071498,0.200000000000015,66.4278611899825));
#190211=CARTESIAN_POINT('',(115.196277168362,0.200000000000015,66.3787024596368));
#190212=CARTESIAN_POINT('Origin',(116.959178380441,0.200000000000015,51.0204257716897));
#190213=CARTESIAN_POINT('',(115.138859552286,0.200000000000015,66.6740890129522));
#190214=CARTESIAN_POINT('',(115.196277168362,0.200000000000015,66.3787024596368));
#190215=CARTESIAN_POINT('Origin',(116.959178380441,0.200000000000015,51.0204257716897));
#190216=CARTESIAN_POINT('Origin',(116.193130296394,0.200000000000015,63.870772219933));
#190217=CARTESIAN_POINT('',(115.698875495068,0.700000000000015,66.4134800541959));
#190218=CARTESIAN_POINT('',(115.641231314811,0.700000000000015,66.7100321733552));
#190219=CARTESIAN_POINT('',(115.698875495068,0.700000000000015,66.4134800541959));
#190220=CARTESIAN_POINT('Origin',(118.62794428911,1.45439216225896E-14,
51.3448026236171));
#190221=CARTESIAN_POINT('Origin',(118.62794428911,1.45439216225896E-14,
51.3448026236171));
#190222=CARTESIAN_POINT('Origin',(116.193130296394,0.700000000000015,63.870772219933));
#190223=CARTESIAN_POINT('',(115.199064038956,0.700000000000015,66.3643653248782));
#190224=CARTESIAN_POINT('',(115.141593004459,0.700000000000015,66.6600266907696));
#190225=CARTESIAN_POINT('',(115.199064038956,0.700000000000015,66.3643653248782));
#190226=CARTESIAN_POINT('Origin',(116.959178380441,0.700000000000015,51.0204257716897));
#190227=CARTESIAN_POINT('Origin',(116.959178380441,0.700000000000015,51.0204257716897));
#190228=CARTESIAN_POINT('Origin',(115.702316793845,0.700000000000015,63.7753672634838));
#190229=CARTESIAN_POINT('Origin',(118.13713078656,1.45439216225896E-14,
51.2493976671679));
#190230=CARTESIAN_POINT('Origin',(118.13713078656,1.45439216225896E-14,
51.2493976671679));
#190231=CARTESIAN_POINT('Origin',(117.174757301493,-8.3,64.0615821328315));
#190232=CARTESIAN_POINT('',(116.66557384992,-8.3,64.0606818998006));
#190233=CARTESIAN_POINT('',(116.597027861112,-8.3,64.4133186820487));
#190234=CARTESIAN_POINT('',(116.66557384992,-8.3,64.0606818998006));
#190235=CARTESIAN_POINT('',(117.174968553192,-8.30043647285503,64.0619238523546));
#190236=CARTESIAN_POINT('Origin',(116.959178380441,-8.3,51.0204257716897));
#190237=CARTESIAN_POINT('',(117.105590222673,-8.3,64.4174141302515));
#190238=CARTESIAN_POINT('',(117.174757301493,-8.3,64.0615821328315));
#190239=CARTESIAN_POINT('Origin',(116.959178380441,-8.3,51.0204257716897));
#190240=CARTESIAN_POINT('Origin',(116.683943798944,-8.3,63.9661771763823));
#190241=CARTESIAN_POINT('',(116.683943798944,-8.8,63.9661771763823));
#190242=CARTESIAN_POINT('',(116.65952420634,-8.8,64.0918044626649));
#190243=CARTESIAN_POINT('',(116.683943798944,-8.8,63.9661771763823));
#190244=CARTESIAN_POINT('',(116.683943798944,-8.44726287030299,63.9661771763823));
#190245=CARTESIAN_POINT('',(116.683943798944,-8.44726287030299,63.9661771763823));
#190246=CARTESIAN_POINT('Origin',(119.118757791659,1.45439216225896E-14,
51.4402075800664));
#190247=CARTESIAN_POINT('Origin',(119.118757791659,1.45439216225896E-14,
51.4402075800664));
#190248=CARTESIAN_POINT('Origin',(116.683943798944,-8.8,63.9661771763823));
#190249=CARTESIAN_POINT('',(117.174757301493,-8.8,64.0615821328315));
#190250=CARTESIAN_POINT('',(117.168540939797,-8.8,64.0935623817685));
#190251=CARTESIAN_POINT('',(117.174757301493,-8.8,64.0615821328315));
#190252=CARTESIAN_POINT('',(116.683943798944,-8.8,63.9661771763823));
#190253=CARTESIAN_POINT('Origin',(116.959178380441,-8.8,51.0204257716897));
#190254=CARTESIAN_POINT('Origin',(117.174757301493,-8.8,64.0615821328315));
#190255=CARTESIAN_POINT('',(117.174757301493,-9.,64.0615821328315));
#190256=CARTESIAN_POINT('Origin',(119.609571294209,1.45439216225896E-14,
51.5356125365156));
#190257=CARTESIAN_POINT('Origin',(116.487618397924,-9.,63.9280151938026));
#190258=CARTESIAN_POINT('Origin',(114.524364387726,1.45439216225896E-14,
63.5463953680056));
#190259=CARTESIAN_POINT('Origin',(116.193130296394,-8.3,63.870772219933));
#190260=CARTESIAN_POINT('',(115.658845070641,-8.3,63.9990087756383));
#190261=CARTESIAN_POINT('',(115.590974766137,-8.3,64.3481694808335));
#190262=CARTESIAN_POINT('',(115.658845070641,-8.3,63.9990087756383));
#190263=CARTESIAN_POINT('',(116.160332513205,-8.3,64.0395013451467));
#190264=CARTESIAN_POINT('Origin',(116.959178380441,-8.3,51.0204257716897));
#190265=CARTESIAN_POINT('',(116.09217650258,-8.3,64.3901318735768));
#190266=CARTESIAN_POINT('',(116.160332513205,-8.3,64.0395013451467));
#190267=CARTESIAN_POINT('Origin',(116.959178380441,-8.3,51.0204257716897));
#190268=CARTESIAN_POINT('Origin',(115.702316793845,-8.3,63.7753672634838));
#190269=CARTESIAN_POINT('',(115.702316793845,-8.8,63.7753672634838));
#190270=CARTESIAN_POINT('',(115.652856553532,-8.8,64.029816871641));
#190271=CARTESIAN_POINT('',(115.702316793845,-8.8,63.7753672634838));
#190272=CARTESIAN_POINT('',(115.702316793845,-8.64616967217299,63.7753672634838));
#190273=CARTESIAN_POINT('',(115.702316793845,-8.64616967217299,63.7753672634838));
#190274=CARTESIAN_POINT('Origin',(118.13713078656,1.45439216225896E-14,
51.2493976671679));
#190275=CARTESIAN_POINT('Origin',(118.13713078656,1.45439216225896E-14,
51.2493976671679));
#190276=CARTESIAN_POINT('Origin',(115.702316793845,-8.8,63.7753672634838));
#190277=CARTESIAN_POINT('',(116.193130296394,-8.8,63.870772219933));
#190278=CARTESIAN_POINT('',(116.154318154922,-8.8,64.0704423818052));
#190279=CARTESIAN_POINT('',(116.193130296394,-8.8,63.870772219933));
#190280=CARTESIAN_POINT('',(115.702316793845,-8.8,63.7753672634838));
#190281=CARTESIAN_POINT('Origin',(116.959178380441,-8.8,51.0204257716897));
#190282=CARTESIAN_POINT('Origin',(116.193130296394,-8.8,63.870772219933));
#190283=CARTESIAN_POINT('',(116.193130296394,-8.56190691376599,63.870772219933));
#190284=CARTESIAN_POINT('Origin',(118.62794428911,1.45439216225896E-14,
51.3448026236171));
#190285=CARTESIAN_POINT('',(116.193130296394,-8.8,63.870772219933));
#190286=CARTESIAN_POINT('Origin',(118.62794428911,1.45439216225896E-14,
51.3448026236171));
#190287=CARTESIAN_POINT('Origin',(115.505991392825,-9.,63.7372052809041));
#190288=CARTESIAN_POINT('Origin',(114.524364387726,1.45439216225896E-14,
63.5463953680056));
#190289=CARTESIAN_POINT('Origin',(115.211503291295,-8.3,63.6799623070345));
#190290=CARTESIAN_POINT('',(114.6669556341,-8.3,63.8609942321634));
#190291=CARTESIAN_POINT('',(114.599357801212,-8.3,64.2087531994098));
#190292=CARTESIAN_POINT('',(114.6669556341,-8.3,63.8609942321634));
#190293=CARTESIAN_POINT('',(115.161063153857,-8.3,63.939453023728));
#190294=CARTESIAN_POINT('Origin',(116.959178380441,-8.3,51.0204257716897));
#190295=CARTESIAN_POINT('',(115.093378099059,-8.3,64.2876607065586));
#190296=CARTESIAN_POINT('',(115.161063153857,-8.3,63.939453023728));
#190297=CARTESIAN_POINT('Origin',(116.959178380441,-8.3,51.0204257716897));
#190298=CARTESIAN_POINT('Origin',(114.720689788746,-8.3,63.5845573505853));
#190299=CARTESIAN_POINT('',(114.720689788746,-8.8,63.5845573505853));
#190300=CARTESIAN_POINT('',(114.66099175365,-8.8,63.8916755841782));
#190301=CARTESIAN_POINT('',(114.720689788746,-8.8,63.5845573505853));
#190302=CARTESIAN_POINT('',(114.720689788746,-8.72675483785299,63.5845573505853));
#190303=CARTESIAN_POINT('',(114.720689788746,-8.72675483785299,63.5845573505853));
#190304=CARTESIAN_POINT('Origin',(117.155503781461,1.45439216225896E-14,
51.0585877542694));
#190305=CARTESIAN_POINT('Origin',(117.155503781461,1.45439216225896E-14,
51.0585877542694));
#190306=CARTESIAN_POINT('Origin',(114.720689788746,-8.8,63.5845573505853));
#190307=CARTESIAN_POINT('',(115.211503291295,-8.8,63.6799623070345));
#190308=CARTESIAN_POINT('',(115.15509138767,-8.8,63.970174944139));
#190309=CARTESIAN_POINT('',(115.211503291295,-8.8,63.6799623070345));
#190310=CARTESIAN_POINT('',(114.720689788746,-8.8,63.5845573505853));
#190311=CARTESIAN_POINT('Origin',(116.959178380441,-8.8,51.0204257716897));
#190312=CARTESIAN_POINT('Origin',(115.211503291295,-8.8,63.6799623070345));
#190313=CARTESIAN_POINT('',(115.211503291295,-8.70093385792599,63.6799623070345));
#190314=CARTESIAN_POINT('Origin',(117.64631728401,1.45439216225896E-14,
51.1539927107186));
#190315=CARTESIAN_POINT('',(115.211503291295,-8.8,63.6799623070345));
#190316=CARTESIAN_POINT('Origin',(117.64631728401,1.45439216225896E-14,
51.1539927107186));
#190317=CARTESIAN_POINT('Origin',(114.524364387726,-9.,63.5463953680056));
#190318=CARTESIAN_POINT('Origin',(114.524364387726,1.45439216225896E-14,
63.5463953680056));
#190319=CARTESIAN_POINT('Origin',(114.229876286196,-8.3,63.489152394136));
#190320=CARTESIAN_POINT('',(113.68972162259,-8.3,63.6475844392384));
#190321=CARTESIAN_POINT('',(113.622007418688,-8.3,63.9959420804558));
#190322=CARTESIAN_POINT('',(113.68972162259,-8.3,63.6475844392384));
#190323=CARTESIAN_POINT('',(114.176507918113,-8.3,63.7637074763767));
#190324=CARTESIAN_POINT('Origin',(116.959178380441,-8.3,51.0204257716897));
#190325=CARTESIAN_POINT('',(114.108900410553,-8.3,64.1115162152435));
#190326=CARTESIAN_POINT('',(114.176507918113,-8.3,63.7637074763767));
#190327=CARTESIAN_POINT('Origin',(116.959178380441,-8.3,51.0204257716897));
#190328=CARTESIAN_POINT('Origin',(113.739062783647,-8.3,63.3937474376868));
#190329=CARTESIAN_POINT('',(113.739062783647,-8.8,63.3937474376868));
#190330=CARTESIAN_POINT('',(113.683747220861,-8.8,63.6783199182644));
#190331=CARTESIAN_POINT('',(113.739062783647,-8.8,63.3937474376868));
#190332=CARTESIAN_POINT('',(113.739062783647,-8.69230981960499,63.3937474376868));
#190333=CARTESIAN_POINT('',(113.739062783647,-8.69230981960499,63.3937474376868));
#190334=CARTESIAN_POINT('Origin',(116.173876776362,1.45439216225896E-14,
50.8677778413709));
#190335=CARTESIAN_POINT('Origin',(116.173876776362,1.45439216225896E-14,
50.8677778413709));
#190336=CARTESIAN_POINT('Origin',(113.739062783647,-8.8,63.3937474376868));
#190337=CARTESIAN_POINT('',(114.229876286196,-8.8,63.489152394136));
#190338=CARTESIAN_POINT('',(114.170543163013,-8.8,63.7943933280519));
#190339=CARTESIAN_POINT('',(114.229876286196,-8.8,63.489152394136));
#190340=CARTESIAN_POINT('',(113.739062783647,-8.8,63.3937474376868));
#190341=CARTESIAN_POINT('Origin',(116.959178380441,-8.8,51.0204257716897));
#190342=CARTESIAN_POINT('Origin',(114.229876286196,-8.8,63.489152394136));
#190343=CARTESIAN_POINT('',(114.229876286196,-8.72388961415699,63.489152394136));
#190344=CARTESIAN_POINT('Origin',(116.664690278911,1.45439216225896E-14,
50.9631827978201));
#190345=CARTESIAN_POINT('',(114.229876286196,-8.8,63.489152394136));
#190346=CARTESIAN_POINT('Origin',(116.664690278911,1.45439216225896E-14,
50.9631827978201));
#190347=CARTESIAN_POINT('Origin',(113.542737382627,-9.,63.3555854551071));
#190348=CARTESIAN_POINT('Origin',(114.524364387726,1.45439216225896E-14,
63.5463953680056));
#190349=CARTESIAN_POINT('Origin',(113.248249281097,-8.3,63.2983424812375));
#190350=CARTESIAN_POINT('',(112.727221388347,-8.3,63.3583763115525));
#190351=CARTESIAN_POINT('',(112.65899587179,-8.3,63.7093644152198));
#190352=CARTESIAN_POINT('',(112.727221388347,-8.3,63.3583763115525));
#190353=CARTESIAN_POINT('',(113.206614610098,-8.3,63.5125332262568));
#190354=CARTESIAN_POINT('Origin',(116.959178380441,-8.3,51.0204257716897));
#190355=CARTESIAN_POINT('',(113.138695302267,-8.3,63.8619460304553));
#190356=CARTESIAN_POINT('',(113.206614610098,-8.3,63.5125332262568));
#190357=CARTESIAN_POINT('Origin',(116.959178380441,-8.3,51.0204257716897));
#190358=CARTESIAN_POINT('Origin',(112.757435778548,-8.3,63.2029375247883));
#190359=CARTESIAN_POINT('',(112.757435778548,-8.8,63.2029375247883));
#190360=CARTESIAN_POINT('',(112.72120074226,-8.8,63.3893496959914));
#190361=CARTESIAN_POINT('',(112.757435778548,-8.8,63.2029375247883));
#190362=CARTESIAN_POINT('',(112.757435778548,-8.54144308650499,63.2029375247883));
#190363=CARTESIAN_POINT('',(112.757435778548,-8.54144308650499,63.2029375247883));
#190364=CARTESIAN_POINT('Origin',(115.192249771263,1.45439216225896E-14,
50.6769679284724));
#190365=CARTESIAN_POINT('Origin',(115.192249771263,1.45439216225896E-14,
50.6769679284724));
#190366=CARTESIAN_POINT('Origin',(112.757435778548,-8.8,63.2029375247883));
#190367=CARTESIAN_POINT('',(113.248249281097,-8.8,63.2983424812375));
#190368=CARTESIAN_POINT('',(113.200621661374,-8.8,63.5433641208314));
#190369=CARTESIAN_POINT('',(113.248249281097,-8.8,63.2983424812375));
#190370=CARTESIAN_POINT('',(112.757435778548,-8.8,63.2029375247883));
#190371=CARTESIAN_POINT('Origin',(116.959178380441,-8.8,51.0204257716897));
#190372=CARTESIAN_POINT('Origin',(113.248249281097,-8.8,63.2983424812375));
#190373=CARTESIAN_POINT('',(113.248249281097,-8.63170029600199,63.2983424812375));
#190374=CARTESIAN_POINT('Origin',(115.683063273812,1.45439216225896E-14,
50.7723728849216));
#190375=CARTESIAN_POINT('',(113.248249281097,-8.8,63.2983424812375));
#190376=CARTESIAN_POINT('Origin',(115.683063273812,1.45439216225896E-14,
50.7723728849216));
#190377=CARTESIAN_POINT('Origin',(112.561110377528,-9.,63.1647755422086));
#190378=CARTESIAN_POINT('Origin',(114.524364387726,1.45439216225896E-14,
63.5463953680056));
#190379=CARTESIAN_POINT('Origin',(112.266622275998,-8.3,63.107532568339));
#190380=CARTESIAN_POINT('',(111.775808773449,-8.3,63.0121276118898));
#190381=CARTESIAN_POINT('',(111.710643451443,-8.3,63.3473724579512));
#190382=CARTESIAN_POINT('',(111.775808773449,-8.3,63.0121276118898));
#190383=CARTESIAN_POINT('',(111.871019148132,-8.3,63.030634726309));
#190384=CARTESIAN_POINT('',(111.871019148132,-8.3,63.030634726309));
#190385=CARTESIAN_POINT('',(112.251593893842,-8.3,63.1848465062967));
#190386=CARTESIAN_POINT('Origin',(116.959178380441,-8.3,51.0204257716897));
#190387=CARTESIAN_POINT('',(112.182956955252,-8.3,63.5379511822739));
#190388=CARTESIAN_POINT('',(112.251593893842,-8.3,63.1848465062967));
#190389=CARTESIAN_POINT('Origin',(116.959178380441,-8.3,51.0204257716897));
#190390=CARTESIAN_POINT('Origin',(111.775808773449,-8.3,63.0121276118898));
#190391=CARTESIAN_POINT('',(111.775808773449,-8.8,63.0121276118898));
#190392=CARTESIAN_POINT('',(111.773697539863,-8.8,63.0229889129114));
#190393=CARTESIAN_POINT('',(111.775808773449,-8.8,63.0121276118898));
#190394=CARTESIAN_POINT('',(111.775808773449,-8.3,63.0121276118898));
#190395=CARTESIAN_POINT('Origin',(114.210622766164,1.45439216225896E-14,
50.4861580155739));
#190396=CARTESIAN_POINT('Origin',(111.775808773449,-8.8,63.0121276118898));
#190397=CARTESIAN_POINT('',(112.266622275998,-8.8,63.107532568339));
#190398=CARTESIAN_POINT('',(112.245536018932,-8.8,63.2160114154701));
#190399=CARTESIAN_POINT('',(112.266622275998,-8.8,63.107532568339));
#190400=CARTESIAN_POINT('',(111.775808773449,-8.8,63.0121276118898));
#190401=CARTESIAN_POINT('Origin',(116.959178380441,-8.8,51.0204257716897));
#190402=CARTESIAN_POINT('Origin',(112.266622275998,-8.8,63.107532568339));
#190403=CARTESIAN_POINT('',(112.266622275998,-8.42058489654999,63.107532568339));
#190404=CARTESIAN_POINT('Origin',(114.701436268713,1.45439216225896E-14,
50.5815629720231));
#190405=CARTESIAN_POINT('',(112.266622275998,-8.8,63.107532568339));
#190406=CARTESIAN_POINT('Origin',(114.701436268713,1.45439216225896E-14,
50.5815629720231));
#190407=CARTESIAN_POINT('Origin',(111.579483372429,-9.,62.9739656293101));
#190408=CARTESIAN_POINT('Origin',(114.524364387726,1.45439216225896E-14,
63.5463953680056));
#190409=CARTESIAN_POINT('Origin',(106.376860245404,-2.3,61.962673090948));
#190410=CARTESIAN_POINT('',(105.886046742854,-2.3,61.8672681344988));
#190411=CARTESIAN_POINT('',(105.864960485789,-2.3,61.9757469816299));
#190412=CARTESIAN_POINT('',(105.886046742854,-2.3,61.8672681344988));
#190413=CARTESIAN_POINT('',(106.258490854543,-2.3,61.9396642973404));
#190414=CARTESIAN_POINT('',(106.258490854543,-2.3,61.9396642973404));
#190415=CARTESIAN_POINT('',(106.361831863248,-2.3,62.0399870289056));
#190416=CARTESIAN_POINT('Origin',(116.959178380441,-2.3,51.0204257716897));
#190417=CARTESIAN_POINT('',(106.293194924658,-2.3,62.3930917048829));
#190418=CARTESIAN_POINT('',(106.361831863248,-2.3,62.0399870289056));
#190419=CARTESIAN_POINT('Origin',(116.959178380441,-2.3,51.0204257716897));
#190420=CARTESIAN_POINT('Origin',(105.886046742854,-2.3,61.8672681344988));
#190421=CARTESIAN_POINT('',(105.886046742854,-2.8,61.8672681344988));
#190422=CARTESIAN_POINT('',(105.883935509269,-2.8,61.8781294355204));
#190423=CARTESIAN_POINT('',(105.886046742854,-2.8,61.8672681344988));
#190424=CARTESIAN_POINT('',(105.886046742854,-2.3,61.8672681344988));
#190425=CARTESIAN_POINT('Origin',(108.32086073557,1.45439216225896E-14,
49.3412985381828));
#190426=CARTESIAN_POINT('Origin',(105.886046742854,-2.8,61.8672681344988));
#190427=CARTESIAN_POINT('',(106.376860245404,-2.8,61.962673090948));
#190428=CARTESIAN_POINT('',(106.311694923398,-2.8,62.2979179370094));
#190429=CARTESIAN_POINT('',(106.376860245404,-2.8,61.962673090948));
#190430=CARTESIAN_POINT('',(105.886046742854,-2.8,61.8672681344988));
#190431=CARTESIAN_POINT('Origin',(116.959178380441,-2.8,51.0204257716897));
#190432=CARTESIAN_POINT('Origin',(106.376860245404,-2.8,61.962673090948));
#190433=CARTESIAN_POINT('',(106.376860245404,-2.70300758415499,61.962673090948));
#190434=CARTESIAN_POINT('Origin',(108.811674238119,1.45439216225896E-14,
49.4367034946321));
#190435=CARTESIAN_POINT('',(106.376860245404,-2.8,61.962673090948));
#190436=CARTESIAN_POINT('Origin',(108.811674238119,1.45439216225896E-14,
49.4367034946321));
#190437=CARTESIAN_POINT('Origin',(105.689721341835,-3.,61.8291061519191));
#190438=CARTESIAN_POINT('Origin',(114.524364387726,1.45439216225896E-14,
63.5463953680056));
#190439=CARTESIAN_POINT('Origin',(106.376860245404,-1.8,61.962673090948));
#190440=CARTESIAN_POINT('',(106.335225574405,-1.3,62.1768638359673));
#190441=CARTESIAN_POINT('',(106.267306266574,-1.3,62.5262766401657));
#190442=CARTESIAN_POINT('',(106.335225574405,-1.3,62.1768638359673));
#190443=CARTESIAN_POINT('',(106.346645855203,-1.8,62.1181118777122));
#190444=CARTESIAN_POINT('Origin',(108.811674238119,1.45439216225896E-14,
49.4367034946321));
#190445=CARTESIAN_POINT('',(106.278420338646,-1.8,62.4690999813795));
#190446=CARTESIAN_POINT('',(106.346645855203,-1.8,62.1181118777122));
#190447=CARTESIAN_POINT('Origin',(108.811674238119,1.45439216225896E-14,
49.4367034946321));
#190448=CARTESIAN_POINT('Origin',(106.376860245404,-1.3,61.962673090948));
#190449=CARTESIAN_POINT('',(105.886046742854,-1.3,61.8672681344988));
#190450=CARTESIAN_POINT('',(105.838419123131,-1.3,62.1122897740926));
#190451=CARTESIAN_POINT('',(105.886046742854,-1.3,61.8672681344988));
#190452=CARTESIAN_POINT('',(106.051254277249,-1.3,61.8993813863595));
#190453=CARTESIAN_POINT('',(106.051254277249,-1.3,61.8993813863595));
#190454=CARTESIAN_POINT('Origin',(116.959178380441,-1.3,51.0204257716897));
#190455=CARTESIAN_POINT('Origin',(116.959178380441,-1.3,51.0204257716897));
#190456=CARTESIAN_POINT('Origin',(105.886046742854,-1.3,61.8672681344988));
#190457=CARTESIAN_POINT('',(105.886046742854,-1.8,61.8672681344988));
#190458=CARTESIAN_POINT('',(105.849811706567,-1.8,62.0536803057019));
#190459=CARTESIAN_POINT('',(105.886046742854,-1.8,61.8672681344988));
#190460=CARTESIAN_POINT('',(105.886046742854,-1.3,61.8672681344988));
#190461=CARTESIAN_POINT('Origin',(108.32086073557,1.45439216225896E-14,
49.3412985381828));
#190462=CARTESIAN_POINT('Origin',(105.886046742854,-1.8,61.8672681344988));
#190463=CARTESIAN_POINT('',(106.139853191496,-1.8,61.916603356642));
#190464=CARTESIAN_POINT('Origin',(116.959178380441,-1.8,51.0204257716897));
#190465=CARTESIAN_POINT('',(105.886046742854,-1.8,61.8672681344988));
#190466=CARTESIAN_POINT('Origin',(116.959178380441,-1.8,51.0204257716897));
#190467=CARTESIAN_POINT('Origin',(105.689721341835,-2.,61.8291061519191));
#190468=CARTESIAN_POINT('Origin',(114.524364387726,1.45439216225896E-14,
63.5463953680056));
#190469=CARTESIAN_POINT('Origin',(106.376860245404,-0.799999999999986,61.962673090948));
#190470=CARTESIAN_POINT('',(106.323491877321,-0.299999999999985,62.2372281731886));
#190471=CARTESIAN_POINT('',(106.255884369761,-0.299999999999985,62.5850369120555));
#190472=CARTESIAN_POINT('',(106.323491877321,-0.299999999999985,62.2372281731886));
#190473=CARTESIAN_POINT('',(106.327519084347,-0.799999999999986,62.2165100924996));
#190474=CARTESIAN_POINT('Origin',(108.811674238119,1.45439216225896E-14,
49.4367034946321));
#190475=CARTESIAN_POINT('',(106.259804880446,-0.799999999999986,62.564867733717));
#190476=CARTESIAN_POINT('',(106.327519084347,-0.799999999999986,62.2165100924996));
#190477=CARTESIAN_POINT('Origin',(108.811674238119,1.45439216225896E-14,
49.4367034946321));
#190478=CARTESIAN_POINT('Origin',(106.376860245404,-0.299999999999985,61.962673090948));
#190479=CARTESIAN_POINT('',(105.886046742854,-0.299999999999985,61.8672681344988));
#190480=CARTESIAN_POINT('',(105.826713619671,-0.299999999999985,62.1725090684146));
#190481=CARTESIAN_POINT('',(105.886046742854,-0.299999999999985,61.8672681344988));
#190482=CARTESIAN_POINT('',(105.960758752966,-0.299999999999985,61.8817907505921));
#190483=CARTESIAN_POINT('',(105.960758752966,-0.299999999999985,61.8817907505921));
#190484=CARTESIAN_POINT('Origin',(116.959178380441,-0.299999999999985,51.0204257716897));
#190485=CARTESIAN_POINT('Origin',(116.959178380441,-0.299999999999985,51.0204257716897));
#190486=CARTESIAN_POINT('Origin',(105.886046742854,-0.299999999999985,61.8672681344988));
#190487=CARTESIAN_POINT('',(105.886046742854,-0.799999999999986,61.8672681344988));
#190488=CARTESIAN_POINT('',(105.830731180069,-0.799999999999986,62.1518406150764));
#190489=CARTESIAN_POINT('',(105.886046742854,-0.799999999999986,61.8672681344988));
#190490=CARTESIAN_POINT('',(105.886046742854,-0.299999999999985,61.8672681344988));
#190491=CARTESIAN_POINT('Origin',(108.32086073557,1.45439216225896E-14,
49.3412985381828));
#190492=CARTESIAN_POINT('Origin',(105.886046742854,-0.799999999999986,61.8672681344988));
#190493=CARTESIAN_POINT('',(105.991758332114,-0.799999999999986,61.88781648844));
#190494=CARTESIAN_POINT('Origin',(116.959178380441,-0.799999999999986,51.0204257716897));
#190495=CARTESIAN_POINT('',(105.886046742854,-0.799999999999986,61.8672681344988));
#190496=CARTESIAN_POINT('Origin',(116.959178380441,-0.799999999999986,51.0204257716897));
#190497=CARTESIAN_POINT('Origin',(105.689721341835,-0.999999999999985,61.8291061519191));
#190498=CARTESIAN_POINT('Origin',(114.524364387726,1.45439216225896E-14,
63.5463953680056));
#190499=CARTESIAN_POINT('Origin',(119.138011311691,-7.3,64.4432019586286));
#190500=CARTESIAN_POINT('',(118.608137303018,-7.3,64.5487448830385));
#190501=CARTESIAN_POINT('',(118.540149211821,-7.3,64.8985115452097));
#190502=CARTESIAN_POINT('',(118.608137303018,-7.3,64.5487448830385));
#190503=CARTESIAN_POINT('',(119.131916138895,-7.3,64.4745587478364));
#190504=CARTESIAN_POINT('Origin',(116.959178380441,-7.3,51.0204257716897));
#190505=CARTESIAN_POINT('',(119.063034885886,-7.3,64.8289203062656));
#190506=CARTESIAN_POINT('',(119.131916138895,-7.3,64.4745587478364));
#190507=CARTESIAN_POINT('Origin',(116.959178380441,-7.3,51.0204257716897));
#190508=CARTESIAN_POINT('Origin',(118.647197809142,-7.3,64.3477970021793));
#190509=CARTESIAN_POINT('',(118.647197809142,-7.8,64.3477970021793));
#190510=CARTESIAN_POINT('',(118.594808184532,-7.8,64.6173169108791));
#190511=CARTESIAN_POINT('',(118.647197809142,-7.8,64.3477970021793));
#190512=CARTESIAN_POINT('',(118.647197809142,-7.65220556441099,64.3477970021793));
#190513=CARTESIAN_POINT('',(118.647197809142,-7.65220556441099,64.3477970021793));
#190514=CARTESIAN_POINT('Origin',(121.082011801857,1.45439216225896E-14,
51.8218274058634));
#190515=CARTESIAN_POINT('Origin',(121.082011801857,1.45439216225896E-14,
51.8218274058634));
#190516=CARTESIAN_POINT('Origin',(118.647197809142,-7.8,64.3477970021793));
#190517=CARTESIAN_POINT('',(119.138011311691,-7.8,64.4432019586286));
#190518=CARTESIAN_POINT('',(119.118407990194,-7.8,64.5440518016936));
#190519=CARTESIAN_POINT('',(119.138011311691,-7.8,64.4432019586286));
#190520=CARTESIAN_POINT('',(118.647197809142,-7.8,64.3477970021793));
#190521=CARTESIAN_POINT('Origin',(116.959178380441,-7.8,51.0204257716897));
#190522=CARTESIAN_POINT('Origin',(119.138011311691,-7.8,64.4432019586286));
#190523=CARTESIAN_POINT('',(119.138011311691,-7.35569507252699,64.4432019586286));
#190524=CARTESIAN_POINT('Origin',(121.572825304407,1.45439216225896E-14,
51.9172323623126));
#190525=CARTESIAN_POINT('',(119.138011311691,-7.8,64.4432019586286));
#190526=CARTESIAN_POINT('Origin',(121.572825304407,1.45439216225896E-14,
51.9172323623126));
#190527=CARTESIAN_POINT('Origin',(118.450872408122,-8.,64.3096350195996));
#190528=CARTESIAN_POINT('Origin',(114.524364387726,1.45439216225896E-14,
63.5463953680056));
#190529=CARTESIAN_POINT('Origin',(117.665570804043,-7.8,64.1569870892808));
#190530=CARTESIAN_POINT('',(118.143958075359,-7.8,64.3163191445107));
#190531=CARTESIAN_POINT('',(118.075250147152,-7.8,64.6697890285819));
#190532=CARTESIAN_POINT('',(118.143958075359,-7.8,64.3163191445107));
#190533=CARTESIAN_POINT('',(117.627614331757,-7.8,64.3522552367681));
#190534=CARTESIAN_POINT('Origin',(116.959178380441,-7.8,51.0204257716897));
#190535=CARTESIAN_POINT('',(117.55959669792,-7.8,64.7021738818927));
#190536=CARTESIAN_POINT('',(117.627614331757,-7.8,64.3522552367681));
#190537=CARTESIAN_POINT('Origin',(116.959178380441,-7.8,51.0204257716897));
#190538=CARTESIAN_POINT('Origin',(118.156384306592,-7.8,64.25239204573));
#190539=CARTESIAN_POINT('',(118.088426174981,-7.3,64.6020045799654));
#190540=CARTESIAN_POINT('',(118.021202443878,-7.3,64.947838969973));
#190541=CARTESIAN_POINT('',(118.088426174981,-7.3,64.6020045799654));
#190542=CARTESIAN_POINT('Origin',(120.591198299308,1.45439216225896E-14,
51.7264224494141));
#190543=CARTESIAN_POINT('Origin',(120.591198299308,1.45439216225896E-14,
51.7264224494141));
#190544=CARTESIAN_POINT('Origin',(118.156384306592,-7.3,64.25239204573));
#190545=CARTESIAN_POINT('',(117.572643242488,-7.3,64.6350555635753));
#190546=CARTESIAN_POINT('',(117.506066436225,-7.3,64.9775618304052));
#190547=CARTESIAN_POINT('',(117.572643242488,-7.3,64.6350555635753));
#190548=CARTESIAN_POINT('Origin',(116.959178380441,-7.3,51.0204257716897));
#190549=CARTESIAN_POINT('Origin',(116.959178380441,-7.3,51.0204257716897));
#190550=CARTESIAN_POINT('Origin',(117.665570804043,-7.3,64.1569870892808));
#190551=CARTESIAN_POINT('Origin',(120.100384796758,1.45439216225896E-14,
51.6310174929649));
#190552=CARTESIAN_POINT('Origin',(120.100384796758,1.45439216225896E-14,
51.6310174929649));
#190553=CARTESIAN_POINT('Origin',(116.683943798944,-7.8,63.9661771763823));
#190554=CARTESIAN_POINT('',(117.115177856914,-7.8,64.3680902741484));
#190555=CARTESIAN_POINT('',(117.047734255941,-7.8,64.7150557909319));
#190556=CARTESIAN_POINT('',(117.115177856914,-7.8,64.3680902741484));
#190557=CARTESIAN_POINT('',(116.606547757441,-7.8,64.3643433055556));
#190558=CARTESIAN_POINT('Origin',(116.959178380441,-7.8,51.0204257716897));
#190559=CARTESIAN_POINT('',(116.539570003489,-7.8,64.708912259135));
#190560=CARTESIAN_POINT('',(116.606547757441,-7.8,64.3643433055556));
#190561=CARTESIAN_POINT('Origin',(116.959178380441,-7.8,51.0204257716897));
#190562=CARTESIAN_POINT('Origin',(117.174757301493,-7.8,64.0615821328315));
#190563=CARTESIAN_POINT('',(117.060673059164,-7.3,64.6484917510221));
#190564=CARTESIAN_POINT('',(116.994634850768,-7.3,64.9882271858619));
#190565=CARTESIAN_POINT('',(117.060673059164,-7.3,64.6484917510221));
#190566=CARTESIAN_POINT('Origin',(119.609571294209,1.45439216225896E-14,
51.5356125365156));
#190567=CARTESIAN_POINT('Origin',(119.609571294209,1.45439216225896E-14,
51.5356125365156));
#190568=CARTESIAN_POINT('Origin',(117.174757301493,-7.3,64.0615821328315));
#190569=CARTESIAN_POINT('',(116.552421327236,-7.3,64.6427982598684));
#190570=CARTESIAN_POINT('',(116.486820626901,-7.3,64.9802829220894));
#190571=CARTESIAN_POINT('',(116.552421327236,-7.3,64.6427982598684));
#190572=CARTESIAN_POINT('Origin',(116.959178380441,-7.3,51.0204257716897));
#190573=CARTESIAN_POINT('Origin',(116.959178380441,-7.3,51.0204257716897));
#190574=CARTESIAN_POINT('Origin',(116.683943798944,-7.3,63.9661771763823));
#190575=CARTESIAN_POINT('Origin',(119.118757791659,1.45439216225896E-14,
51.4402075800664));
#190576=CARTESIAN_POINT('Origin',(119.118757791659,1.45439216225896E-14,
51.4402075800664));
#190577=CARTESIAN_POINT('Origin',(115.702316793845,-7.8,63.7753672634838));
#190578=CARTESIAN_POINT('',(116.101643499298,-7.8,64.3414286406355));
#190579=CARTESIAN_POINT('',(116.035029699075,-7.8,64.6841252239447));
#190580=CARTESIAN_POINT('',(116.101643499298,-7.8,64.3414286406355));
#190581=CARTESIAN_POINT('',(115.600402993959,-7.8,64.2996656955739));
#190582=CARTESIAN_POINT('Origin',(116.959178380441,-7.8,51.0204257716897));
#190583=CARTESIAN_POINT('',(115.534056011535,-7.8,64.6409896271509));
#190584=CARTESIAN_POINT('',(115.600402993959,-7.8,64.2996656955739));
#190585=CARTESIAN_POINT('Origin',(116.959178380441,-7.8,51.0204257716897));
#190586=CARTESIAN_POINT('Origin',(116.193130296394,-7.8,63.870772219933));
#190587=CARTESIAN_POINT('',(116.047812650375,-7.3,64.618362968668));
#190588=CARTESIAN_POINT('',(115.982554022284,-7.3,64.9540878305312));
#190589=CARTESIAN_POINT('',(116.047812650375,-7.3,64.618362968668));
#190590=CARTESIAN_POINT('Origin',(118.62794428911,1.45439216225896E-14,
51.3448026236171));
#190591=CARTESIAN_POINT('Origin',(118.62794428911,1.45439216225896E-14,
51.3448026236171));
#190592=CARTESIAN_POINT('Origin',(116.193130296394,-7.3,63.870772219933));
#190593=CARTESIAN_POINT('',(115.546788823354,-7.3,64.5754853158576));
#190594=CARTESIAN_POINT('',(115.481781115242,-7.3,64.9099193127751));
#190595=CARTESIAN_POINT('',(115.546788823354,-7.3,64.5754853158576));
#190596=CARTESIAN_POINT('Origin',(116.959178380441,-7.3,51.0204257716897));
#190597=CARTESIAN_POINT('Origin',(116.959178380441,-7.3,51.0204257716897));
#190598=CARTESIAN_POINT('Origin',(115.702316793845,-7.3,63.7753672634838));
#190599=CARTESIAN_POINT('Origin',(118.13713078656,1.45439216225896E-14,
51.2493976671679));
#190600=CARTESIAN_POINT('Origin',(118.13713078656,1.45439216225896E-14,
51.2493976671679));
#190601=CARTESIAN_POINT('Origin',(114.720689788746,-7.8,63.5845573505853));
#190602=CARTESIAN_POINT('',(115.102781183328,-7.8,64.2392862730183));
#190603=CARTESIAN_POINT('',(115.03660728363,-7.8,64.5797197756079));
#190604=CARTESIAN_POINT('',(115.102781183328,-7.8,64.2392862730183));
#190605=CARTESIAN_POINT('',(114.608749045379,-7.8,64.1604396776117));
#190606=CARTESIAN_POINT('Origin',(116.959178380441,-7.8,51.0204257716897));
#190607=CARTESIAN_POINT('',(114.542656660719,-7.8,64.5004538237752));
#190608=CARTESIAN_POINT('',(114.608749045379,-7.8,64.1604396776117));
#190609=CARTESIAN_POINT('Origin',(116.959178380441,-7.8,51.0204257716897));
#190610=CARTESIAN_POINT('Origin',(115.211503291295,-7.8,63.6799623070345));
#190611=CARTESIAN_POINT('',(115.04930756357,-7.3,64.5143828254856));
#190612=CARTESIAN_POINT('',(114.984462690182,-7.3,64.8479791145506));
#190613=CARTESIAN_POINT('',(115.04930756357,-7.3,64.5143828254856));
#190614=CARTESIAN_POINT('Origin',(117.64631728401,1.45439216225896E-14,
51.1539927107186));
#190615=CARTESIAN_POINT('Origin',(117.64631728401,1.45439216225896E-14,
51.1539927107186));
#190616=CARTESIAN_POINT('Origin',(115.211503291295,-7.3,63.6799623070345));
#190617=CARTESIAN_POINT('',(114.555341617604,-7.3,64.4351957035434));
#190618=CARTESIAN_POINT('',(114.490573450483,-7.3,64.7683973750478));
#190619=CARTESIAN_POINT('',(114.555341617604,-7.3,64.4351957035434));
#190620=CARTESIAN_POINT('Origin',(116.959178380441,-7.3,51.0204257716897));
#190621=CARTESIAN_POINT('Origin',(116.959178380441,-7.3,51.0204257716897));
#190622=CARTESIAN_POINT('Origin',(114.720689788746,-7.3,63.5845573505853));
#190623=CARTESIAN_POINT('Origin',(117.155503781461,1.45439216225896E-14,
51.0585877542694));
#190624=CARTESIAN_POINT('Origin',(117.155503781461,1.45439216225896E-14,
51.0585877542694));
#190625=CARTESIAN_POINT('Origin',(113.739062783647,-7.8,63.3937474376868));
#190626=CARTESIAN_POINT('',(114.118292968078,-7.8,64.0631959368381));
#190627=CARTESIAN_POINT('',(114.052191541068,-7.8,64.403256601628));
#190628=CARTESIAN_POINT('',(114.118292968078,-7.8,64.0631959368381));
#190629=CARTESIAN_POINT('',(113.631414459623,-7.8,63.9475472917409));
#190630=CARTESIAN_POINT('Origin',(116.959178380441,-7.8,51.0204257716897));
#190631=CARTESIAN_POINT('',(113.565213321132,-7.8,64.2881209250702));
#190632=CARTESIAN_POINT('',(113.631414459623,-7.8,63.9475472917409));
#190633=CARTESIAN_POINT('Origin',(116.959178380441,-7.8,51.0204257716897));
#190634=CARTESIAN_POINT('Origin',(114.229876286196,-7.8,63.489152394136));
#190635=CARTESIAN_POINT('',(114.064878197778,-7.3,64.3379897366015));
#190636=CARTESIAN_POINT('',(114.000101521181,-7.3,64.6712351853426));
#190637=CARTESIAN_POINT('',(114.064878197778,-7.3,64.3379897366015));
#190638=CARTESIAN_POINT('Origin',(116.664690278911,1.45439216225896E-14,
50.9631827978201));
#190639=CARTESIAN_POINT('Origin',(116.664690278911,1.45439216225896E-14,
50.9631827978201));
#190640=CARTESIAN_POINT('Origin',(114.229876286196,-7.3,63.489152394136));
#190641=CARTESIAN_POINT('',(113.577918721109,-7.3,64.2227576347738));
#190642=CARTESIAN_POINT('',(113.513048218327,-7.3,64.5564857749867));
#190643=CARTESIAN_POINT('',(113.577918721109,-7.3,64.2227576347738));
#190644=CARTESIAN_POINT('Origin',(116.959178380441,-7.3,51.0204257716897));
#190645=CARTESIAN_POINT('Origin',(116.959178380441,-7.3,51.0204257716897));
#190646=CARTESIAN_POINT('Origin',(113.739062783647,-7.3,63.3937474376868));
#190647=CARTESIAN_POINT('Origin',(116.173876776362,1.45439216225896E-14,
50.8677778413709));
#190648=CARTESIAN_POINT('Origin',(116.173876776362,1.45439216225896E-14,
50.8677778413709));
#190649=CARTESIAN_POINT('Origin',(112.757435778548,-7.8,63.2029375247883));
#190650=CARTESIAN_POINT('',(113.148130180408,-7.8,63.8134080324416));
#190651=CARTESIAN_POINT('',(113.081737423663,-7.8,64.1549674513112));
#190652=CARTESIAN_POINT('',(113.148130180408,-7.8,63.8134080324416));
#190653=CARTESIAN_POINT('',(112.668472298385,-7.8,63.6606126700068));
#190654=CARTESIAN_POINT('Origin',(116.959178380441,-7.8,51.0204257716897));
#190655=CARTESIAN_POINT('',(112.601793610039,-7.8,64.0036430720998));
#190656=CARTESIAN_POINT('',(112.668472298385,-7.8,63.6606126700068));
#190657=CARTESIAN_POINT('Origin',(116.959178380441,-7.8,51.0204257716897));
#190658=CARTESIAN_POINT('Origin',(113.248249281097,-7.8,63.2983424812375));
#190659=CARTESIAN_POINT('',(113.094478838136,-7.3,64.0894188834233));
#190660=CARTESIAN_POINT('',(113.02942807446,-7.3,64.4240743809113));
#190661=CARTESIAN_POINT('',(113.094478838136,-7.3,64.0894188834233));
#190662=CARTESIAN_POINT('Origin',(115.683063273812,1.45439216225896E-14,
50.7723728849216));
#190663=CARTESIAN_POINT('Origin',(115.683063273812,1.45439216225896E-14,
50.7723728849216));
#190664=CARTESIAN_POINT('Origin',(113.248249281097,-7.3,63.2983424812375));
#190665=CARTESIAN_POINT('',(112.614588752975,-7.3,63.9378180966099));
#190666=CARTESIAN_POINT('',(112.54926912135,-7.3,64.2738567928821));
#190667=CARTESIAN_POINT('',(112.614588752975,-7.3,63.9378180966099));
#190668=CARTESIAN_POINT('Origin',(116.959178380441,-7.3,51.0204257716897));
#190669=CARTESIAN_POINT('Origin',(116.959178380441,-7.3,51.0204257716897));
#190670=CARTESIAN_POINT('Origin',(112.757435778548,-7.3,63.2029375247883));
#190671=CARTESIAN_POINT('Origin',(115.192249771263,1.45439216225896E-14,
50.6769679284724));
#190672=CARTESIAN_POINT('Origin',(115.192249771263,1.45439216225896E-14,
50.6769679284724));
#190673=CARTESIAN_POINT('Origin',(111.775808773449,-7.8,63.0121276118898));
#190674=CARTESIAN_POINT('',(112.192489185624,-7.8,63.4889123529498));
#190675=CARTESIAN_POINT('',(112.125426591645,-7.8,63.8339177684538));
#190676=CARTESIAN_POINT('',(112.192489185624,-7.8,63.4889123529498));
#190677=CARTESIAN_POINT('',(111.720246491895,-7.8,63.2979693441656));
#190678=CARTESIAN_POINT('Origin',(116.959178380441,-7.8,51.0204257716897));
#190679=CARTESIAN_POINT('',(111.652696970122,-7.8,63.6454797735061));
#190680=CARTESIAN_POINT('',(111.720246491895,-7.8,63.2979693441656));
#190681=CARTESIAN_POINT('Origin',(116.959178380441,-7.8,51.0204257716897));
#190682=CARTESIAN_POINT('Origin',(112.266622275998,-7.8,63.107532568339));
#190683=CARTESIAN_POINT('',(112.138293850054,-7.3,63.7677217928681));
#190684=CARTESIAN_POINT('',(112.072613443008,-7.3,64.1056165085183));
#190685=CARTESIAN_POINT('',(112.138293850054,-7.3,63.7677217928681));
#190686=CARTESIAN_POINT('Origin',(114.701436268713,1.45439216225896E-14,
50.5815629720231));
#190687=CARTESIAN_POINT('Origin',(114.701436268713,1.45439216225896E-14,
50.5815629720231));
#190688=CARTESIAN_POINT('Origin',(112.266622275998,-7.3,63.107532568339));
#190689=CARTESIAN_POINT('',(111.665655658314,-7.3,63.5788134348104));
#190690=CARTESIAN_POINT('',(111.599518024745,-7.3,63.9190603652681));
#190691=CARTESIAN_POINT('',(111.665655658314,-7.3,63.5788134348104));
#190692=CARTESIAN_POINT('Origin',(116.959178380441,-7.3,51.0204257716897));
#190693=CARTESIAN_POINT('Origin',(116.959178380441,-7.3,51.0204257716897));
#190694=CARTESIAN_POINT('Origin',(111.775808773449,-7.3,63.0121276118898));
#190695=CARTESIAN_POINT('Origin',(114.210622766164,1.45439216225896E-14,
50.4861580155739));
#190696=CARTESIAN_POINT('Origin',(114.210622766164,1.45439216225896E-14,
50.4861580155739));
#190697=CARTESIAN_POINT('Origin',(110.79418176835,-7.8,62.8213176989913));
#190698=CARTESIAN_POINT('',(111.25182865232,-7.8,63.0873492647716));
#190699=CARTESIAN_POINT('',(111.18368255378,-7.8,63.4379288002016));
#190700=CARTESIAN_POINT('',(111.25182865232,-7.8,63.0873492647716));
#190701=CARTESIAN_POINT('',(110.787340913104,-7.8,62.8565106726941));
#190702=CARTESIAN_POINT('Origin',(116.959178380441,-7.8,51.0204257716897));
#190703=CARTESIAN_POINT('',(110.718480119372,-7.8,63.2107669777972));
#190704=CARTESIAN_POINT('',(110.787340913104,-7.8,62.8565106726941));
#190705=CARTESIAN_POINT('Origin',(116.959178380441,-7.8,51.0204257716897));
#190706=CARTESIAN_POINT('Origin',(111.284995270899,-7.8,62.9167226554405));
#190707=CARTESIAN_POINT('',(111.196753201947,-7.3,63.3706864802381));
#190708=CARTESIAN_POINT('',(111.130055939274,-7.3,63.7138124384881));
#190709=CARTESIAN_POINT('',(111.196753201947,-7.3,63.3706864802381));
#190710=CARTESIAN_POINT('Origin',(113.719809263614,1.45439216225896E-14,
50.3907530591246));
#190711=CARTESIAN_POINT('Origin',(113.719809263614,1.45439216225896E-14,
50.3907530591246));
#190712=CARTESIAN_POINT('Origin',(111.284995270899,-7.3,62.9167226554405));
#190713=CARTESIAN_POINT('',(110.731684809429,-7.3,63.142835075533));
#190714=CARTESIAN_POINT('',(110.664317929489,-7.3,63.4894058987878));
#190715=CARTESIAN_POINT('',(110.731684809429,-7.3,63.142835075533));
#190716=CARTESIAN_POINT('Origin',(116.959178380441,-7.3,51.0204257716897));
#190717=CARTESIAN_POINT('Origin',(116.959178380441,-7.3,51.0204257716897));
#190718=CARTESIAN_POINT('Origin',(110.79418176835,-7.3,62.8213176989913));
#190719=CARTESIAN_POINT('Origin',(113.228995761065,1.45439216225896E-14,
50.2953481026754));
#190720=CARTESIAN_POINT('Origin',(113.228995761065,1.45439216225896E-14,
50.2953481026754));
#190721=CARTESIAN_POINT('Origin',(110.3033682658,-7.3,62.725912742542));
#190722=CARTESIAN_POINT('',(109.812554763251,-7.3,62.6305077860928));
#190723=CARTESIAN_POINT('',(109.744478438118,-7.3,62.9807283702507));
#190724=CARTESIAN_POINT('',(109.812554763251,-7.3,62.6305077860928));
#190725=CARTESIAN_POINT('',(109.82625098298,-7.3,62.6331700748033));
#190726=CARTESIAN_POINT('',(109.82625098298,-7.3,62.6331700748033));
#190727=CARTESIAN_POINT('',(110.270570482611,-7.3,62.8946418677557));
#190728=CARTESIAN_POINT('Origin',(116.959178380441,-7.3,51.0204257716897));
#190729=CARTESIAN_POINT('',(110.202414471986,-7.3,63.2452723961858));
#190730=CARTESIAN_POINT('',(110.270570482611,-7.3,62.8946418677557));
#190731=CARTESIAN_POINT('Origin',(116.959178380441,-7.3,51.0204257716897));
#190732=CARTESIAN_POINT('Origin',(109.812554763251,-7.3,62.6305077860928));
#190733=CARTESIAN_POINT('',(109.812554763251,-7.8,62.6305077860928));
#190734=CARTESIAN_POINT('',(109.800007656622,-7.8,62.6950567317697));
#190735=CARTESIAN_POINT('',(109.812554763251,-7.8,62.6305077860928));
#190736=CARTESIAN_POINT('',(109.812554763251,-7.3,62.6305077860928));
#190737=CARTESIAN_POINT('Origin',(112.247368755966,1.45439216225896E-14,
50.1045381897769));
#190738=CARTESIAN_POINT('Origin',(109.812554763251,-7.8,62.6305077860928));
#190739=CARTESIAN_POINT('',(110.3033682658,-7.8,62.725912742542));
#190740=CARTESIAN_POINT('',(110.257207717211,-7.8,62.9633869931011));
#190741=CARTESIAN_POINT('',(110.3033682658,-7.8,62.725912742542));
#190742=CARTESIAN_POINT('',(109.812554763251,-7.8,62.6305077860928));
#190743=CARTESIAN_POINT('Origin',(116.959178380441,-7.8,51.0204257716897));
#190744=CARTESIAN_POINT('Origin',(110.3033682658,-7.8,62.725912742542));
#190745=CARTESIAN_POINT('',(110.3033682658,-7.59646299273499,62.725912742542));
#190746=CARTESIAN_POINT('Origin',(112.738182258515,1.45439216225896E-14,
50.1999431462261));
#190747=CARTESIAN_POINT('',(110.3033682658,-7.8,62.725912742542));
#190748=CARTESIAN_POINT('Origin',(112.738182258515,1.45439216225896E-14,
50.1999431462261));
#190749=CARTESIAN_POINT('Origin',(109.616229362231,-8.,62.5923458035131));
#190750=CARTESIAN_POINT('Origin',(114.524364387726,1.45439216225896E-14,
63.5463953680056));
#190751=CARTESIAN_POINT('Origin',(107.358487250503,-4.3,62.1534830038465));
#190752=CARTESIAN_POINT('',(106.867673747954,-4.3,62.0580780473973));
#190753=CARTESIAN_POINT('',(106.821513199365,-4.3,62.2955522979563));
#190754=CARTESIAN_POINT('',(106.867673747954,-4.3,62.0580780473973));
#190755=CARTESIAN_POINT('',(107.067471170822,-4.3,62.0969149260251));
#190756=CARTESIAN_POINT('',(107.067471170822,-4.3,62.0969149260251));
#190757=CARTESIAN_POINT('',(107.325689467314,-4.3,62.3222121290602));
#190758=CARTESIAN_POINT('Origin',(116.959178380441,-4.3,51.0204257716897));
#190759=CARTESIAN_POINT('',(107.257533456689,-4.3,62.6728426574903));
#190760=CARTESIAN_POINT('',(107.325689467314,-4.3,62.3222121290602));
#190761=CARTESIAN_POINT('Origin',(116.959178380441,-4.3,51.0204257716897));
#190762=CARTESIAN_POINT('Origin',(106.867673747954,-4.3,62.0580780473973));
#190763=CARTESIAN_POINT('',(106.867673747954,-4.8,62.0580780473973));
#190764=CARTESIAN_POINT('',(106.855126641325,-4.8,62.1226269930741));
#190765=CARTESIAN_POINT('',(106.867673747954,-4.8,62.0580780473973));
#190766=CARTESIAN_POINT('',(106.867673747954,-4.3,62.0580780473973));
#190767=CARTESIAN_POINT('Origin',(109.302487740669,1.45439216225896E-14,
49.5321084510813));
#190768=CARTESIAN_POINT('Origin',(106.867673747954,-4.8,62.0580780473973));
#190769=CARTESIAN_POINT('',(107.358487250503,-4.8,62.1534830038465));
#190770=CARTESIAN_POINT('',(107.29041092537,-4.8,62.5037035880044));
#190771=CARTESIAN_POINT('',(107.358487250503,-4.8,62.1534830038465));
#190772=CARTESIAN_POINT('',(106.867673747954,-4.8,62.0580780473973));
#190773=CARTESIAN_POINT('Origin',(116.959178380441,-4.8,51.0204257716897));
#190774=CARTESIAN_POINT('Origin',(107.358487250503,-4.8,62.1534830038465));
#190775=CARTESIAN_POINT('',(107.358487250503,-4.78604742976898,62.1534830038465));
#190776=CARTESIAN_POINT('Origin',(109.793301243218,1.45439216225896E-14,
49.6275134075306));
#190777=CARTESIAN_POINT('',(107.358487250503,-4.8,62.1534830038465));
#190778=CARTESIAN_POINT('Origin',(109.793301243218,1.45439216225896E-14,
49.6275134075306));
#190779=CARTESIAN_POINT('Origin',(106.671348346934,-5.,62.0199160648176));
#190780=CARTESIAN_POINT('Origin',(114.524364387726,1.45439216225896E-14,
63.5463953680056));
#190781=CARTESIAN_POINT('Origin',(107.358487250503,-3.8,62.1534830038465));
#190782=CARTESIAN_POINT('',(107.270245181551,-3.3,62.6074468286441));
#190783=CARTESIAN_POINT('',(107.203547918878,-3.3,62.9505727868941));
#190784=CARTESIAN_POINT('',(107.270245181551,-3.3,62.6074468286441));
#190785=CARTESIAN_POINT('',(107.295990291582,-3.8,62.4750003803882));
#190786=CARTESIAN_POINT('Origin',(109.793301243218,1.45439216225896E-14,
49.6275134075306));
#190787=CARTESIAN_POINT('',(107.228623411642,-3.8,62.8215712036431));
#190788=CARTESIAN_POINT('',(107.295990291582,-3.8,62.4750003803882));
#190789=CARTESIAN_POINT('Origin',(109.793301243218,1.45439216225896E-14,
49.6275134075306));
#190790=CARTESIAN_POINT('Origin',(107.358487250503,-3.3,62.1534830038465));
#190791=CARTESIAN_POINT('',(106.834507129375,-3.3,62.2287046567283));
#190792=CARTESIAN_POINT('',(106.766361030834,-3.3,62.5792841921583));
#190793=CARTESIAN_POINT('',(106.834507129375,-3.3,62.2287046567283));
#190794=CARTESIAN_POINT('Origin',(116.959178380441,-3.3,51.0204257716897));
#190795=CARTESIAN_POINT('Origin',(116.959178380441,-3.3,51.0204257716897));
#190796=CARTESIAN_POINT('Origin',(106.867673747954,-3.3,62.0580780473973));
#190797=CARTESIAN_POINT('',(106.860832892708,-3.8,62.0932710211001));
#190798=CARTESIAN_POINT('',(106.791972098975,-3.8,62.4475273262032));
#190799=CARTESIAN_POINT('',(106.860832892708,-3.8,62.0932710211001));
#190800=CARTESIAN_POINT('Origin',(109.302487740669,1.45439216225896E-14,
49.5321084510813));
#190801=CARTESIAN_POINT('Origin',(109.302487740669,1.45439216225896E-14,
49.5321084510813));
#190802=CARTESIAN_POINT('Origin',(106.867673747954,-3.8,62.0580780473973));
#190803=CARTESIAN_POINT('Origin',(116.959178380441,-3.8,51.0204257716897));
#190804=CARTESIAN_POINT('Origin',(116.959178380441,-3.8,51.0204257716897));
#190805=CARTESIAN_POINT('Origin',(106.867673747954,-2.8,62.0580780473973));
#190806=CARTESIAN_POINT('',(107.248334135368,-2.8,62.7201688267671));
#190807=CARTESIAN_POINT('',(107.182196501799,-2.8,63.0604157572248));
#190808=CARTESIAN_POINT('',(107.248334135368,-2.8,62.7201688267671));
#190809=CARTESIAN_POINT('',(106.8121114664,-2.8,62.3439197796731));
#190810=CARTESIAN_POINT('Origin',(116.959178380441,-2.8,51.0204257716897));
#190811=CARTESIAN_POINT('',(106.744561944627,-2.8,62.6914302090136));
#190812=CARTESIAN_POINT('',(106.8121114664,-2.8,62.3439197796731));
#190813=CARTESIAN_POINT('Origin',(116.959178380441,-2.8,51.0204257716897));
#190814=CARTESIAN_POINT('Origin',(107.358487250503,-2.8,62.1534830038465));
#190815=CARTESIAN_POINT('',(107.230158824559,-2.3,62.8136722283756));
#190816=CARTESIAN_POINT('',(107.164478417513,-2.3,63.1515669440258));
#190817=CARTESIAN_POINT('',(107.230158824559,-2.3,62.8136722283756));
#190818=CARTESIAN_POINT('Origin',(109.793301243218,1.45439216225896E-14,
49.6275134075306));
#190819=CARTESIAN_POINT('Origin',(109.793301243218,1.45439216225896E-14,
49.6275134075306));
#190820=CARTESIAN_POINT('Origin',(107.358487250503,-2.3,62.1534830038465));
#190821=CARTESIAN_POINT('',(106.793540657579,-2.3,62.439457832008));
#190822=CARTESIAN_POINT('',(106.7264780636,-2.3,62.784463247512));
#190823=CARTESIAN_POINT('',(106.793540657579,-2.3,62.439457832008));
#190824=CARTESIAN_POINT('Origin',(116.959178380441,-2.3,51.0204257716897));
#190825=CARTESIAN_POINT('Origin',(116.959178380441,-2.3,51.0204257716897));
#190826=CARTESIAN_POINT('Origin',(106.867673747954,-2.3,62.0580780473973));
#190827=CARTESIAN_POINT('Origin',(109.302487740669,1.45439216225896E-14,
49.5321084510813));
#190828=CARTESIAN_POINT('Origin',(109.302487740669,1.45439216225896E-14,
49.5321084510813));
#190829=CARTESIAN_POINT('Origin',(106.867673747954,-1.8,62.0580780473973));
#190830=CARTESIAN_POINT('',(107.21564022493,-1.8,62.8883635756681));
#190831=CARTESIAN_POINT('',(107.150320593305,-1.8,63.2244022719403));
#190832=CARTESIAN_POINT('',(107.21564022493,-1.8,62.8883635756681));
#190833=CARTESIAN_POINT('',(106.778710267791,-1.8,62.5157531926157));
#190834=CARTESIAN_POINT('Origin',(116.959178380441,-1.8,51.0204257716897));
#190835=CARTESIAN_POINT('',(106.712031579445,-1.8,62.8587835947088));
#190836=CARTESIAN_POINT('',(106.778710267791,-1.8,62.5157531926157));
#190837=CARTESIAN_POINT('Origin',(116.959178380441,-1.8,51.0204257716897));
#190838=CARTESIAN_POINT('Origin',(107.358487250503,-1.8,62.1534830038465));
#190839=CARTESIAN_POINT('',(107.204716807541,-1.3,62.9445594060323));
#190840=CARTESIAN_POINT('',(107.139666043865,-1.3,63.2792149035202));
#190841=CARTESIAN_POINT('',(107.204716807541,-1.3,62.9445594060323));
#190842=CARTESIAN_POINT('Origin',(109.793301243218,1.45439216225896E-14,
49.6275134075306));
#190843=CARTESIAN_POINT('Origin',(109.793301243218,1.45439216225896E-14,
49.6275134075306));
#190844=CARTESIAN_POINT('Origin',(107.358487250503,-1.3,62.1534830038465));
#190845=CARTESIAN_POINT('',(106.767554647265,-1.3,62.5731435986013));
#190846=CARTESIAN_POINT('',(106.701161890519,-1.3,62.9147030174709));
#190847=CARTESIAN_POINT('',(106.767554647265,-1.3,62.5731435986013));
#190848=CARTESIAN_POINT('Origin',(116.959178380441,-1.3,51.0204257716897));
#190849=CARTESIAN_POINT('Origin',(116.959178380441,-1.3,51.0204257716897));
#190850=CARTESIAN_POINT('Origin',(106.867673747954,-1.3,62.0580780473973));
#190851=CARTESIAN_POINT('Origin',(109.302487740669,1.45439216225896E-14,
49.5321084510813));
#190852=CARTESIAN_POINT('Origin',(109.302487740669,1.45439216225896E-14,
49.5321084510813));
#190853=CARTESIAN_POINT('Origin',(106.867673747954,-0.799999999999986,62.0580780473973));
#190854=CARTESIAN_POINT('',(107.197343187966,-0.799999999999986,62.9824932009336));
#190855=CARTESIAN_POINT('',(107.132472685183,-0.799999999999986,63.3162213411464));
#190856=CARTESIAN_POINT('',(107.197343187966,-0.799999999999986,62.9824932009336));
#190857=CARTESIAN_POINT('',(106.76002542393,-0.799999999999986,62.6118779014513));
#190858=CARTESIAN_POINT('Origin',(116.959178380441,-0.799999999999986,51.0204257716897));
#190859=CARTESIAN_POINT('',(106.693824285439,-0.799999999999986,62.9524515347807));
#190860=CARTESIAN_POINT('',(106.76002542393,-0.799999999999986,62.6118779014513));
#190861=CARTESIAN_POINT('Origin',(116.959178380441,-0.799999999999986,51.0204257716897));
#190862=CARTESIAN_POINT('Origin',(107.358487250503,-0.799999999999986,62.1534830038465));
#190863=CARTESIAN_POINT('',(107.193489162085,-0.299999999999985,63.0023203463119));
#190864=CARTESIAN_POINT('',(107.128712485488,-0.299999999999985,63.3355657950531));
#190865=CARTESIAN_POINT('',(107.193489162085,-0.299999999999985,63.0023203463119));
#190866=CARTESIAN_POINT('Origin',(109.793301243218,1.45439216225896E-14,
49.6275134075306));
#190867=CARTESIAN_POINT('Origin',(109.793301243218,1.45439216225896E-14,
49.6275134075306));
#190868=CARTESIAN_POINT('Origin',(107.358487250503,-0.299999999999985,62.1534830038465));
#190869=CARTESIAN_POINT('',(106.756090429836,-0.299999999999985,62.6321215900993));
#190870=CARTESIAN_POINT('',(106.689989002826,-0.299999999999985,62.9721822548892));
#190871=CARTESIAN_POINT('',(106.756090429836,-0.299999999999985,62.6321215900993));
#190872=CARTESIAN_POINT('Origin',(116.959178380441,-0.299999999999985,51.0204257716897));
#190873=CARTESIAN_POINT('Origin',(116.959178380441,-0.299999999999985,51.0204257716897));
#190874=CARTESIAN_POINT('Origin',(106.867673747954,-0.299999999999985,62.0580780473973));
#190875=CARTESIAN_POINT('Origin',(109.302487740669,1.45439216225896E-14,
49.5321084510813));
#190876=CARTESIAN_POINT('Origin',(109.302487740669,1.45439216225896E-14,
49.5321084510813));
#190877=CARTESIAN_POINT('Origin',(123.064519332087,-0.299999999999985,65.2064416102226));
#190878=CARTESIAN_POINT('',(122.508294760723,-0.299999999999985,65.4475457512624));
#190879=CARTESIAN_POINT('',(122.441004340522,-0.299999999999985,65.7937232252189));
#190880=CARTESIAN_POINT('',(122.508294760723,-0.299999999999985,65.4475457512624));
#190881=CARTESIAN_POINT('',(123.061409169883,-0.299999999999985,65.2224419278371));
#190882=CARTESIAN_POINT('Origin',(116.959178380441,-0.299999999999985,51.0204257716897));
#190883=CARTESIAN_POINT('',(122.992445896985,-0.299999999999985,65.5772254399106));
#190884=CARTESIAN_POINT('',(123.061409169883,-0.299999999999985,65.2224419278371));
#190885=CARTESIAN_POINT('Origin',(116.959178380441,-0.299999999999985,51.0204257716897));
#190886=CARTESIAN_POINT('Origin',(122.573705829538,-0.299999999999985,65.1110366537733));
#190887=CARTESIAN_POINT('',(122.512302538895,-0.799999999999986,65.4269276228584));
#190888=CARTESIAN_POINT('',(122.444906919269,-0.799999999999986,65.7736462982427));
#190889=CARTESIAN_POINT('',(122.512302538895,-0.799999999999986,65.4269276228584));
#190890=CARTESIAN_POINT('Origin',(125.008519822253,1.45439216225896E-14,
52.5850670574574));
#190891=CARTESIAN_POINT('Origin',(125.008519822253,1.45439216225896E-14,
52.5850670574574));
#190892=CARTESIAN_POINT('Origin',(122.573705829538,-0.799999999999986,65.1110366537733));
#190893=CARTESIAN_POINT('',(123.064519332087,-0.799999999999986,65.2064416102226));
#190894=CARTESIAN_POINT('',(122.996443006954,-0.799999999999986,65.5566621943805));
#190895=CARTESIAN_POINT('',(123.064519332087,-0.799999999999986,65.2064416102226));
#190896=CARTESIAN_POINT('',(123.056970443337,-0.799999999999986,65.2049742475712));
#190897=CARTESIAN_POINT('',(123.056970443337,-0.799999999999986,65.2049742475712));
#190898=CARTESIAN_POINT('Origin',(116.959178380441,-0.799999999999986,51.0204257716897));
#190899=CARTESIAN_POINT('Origin',(116.959178380441,-0.799999999999986,51.0204257716897));
#190900=CARTESIAN_POINT('Origin',(123.064519332087,-0.799999999999986,65.2064416102226));
#190901=CARTESIAN_POINT('',(123.064519332087,-0.711512473537285,65.2064416102226));
#190902=CARTESIAN_POINT('Origin',(125.499333324803,1.45439216225896E-14,
52.6804720139067));
#190903=CARTESIAN_POINT('',(123.064519332087,-0.799999999999986,65.2064416102226));
#190904=CARTESIAN_POINT('Origin',(125.499333324803,1.45439216225896E-14,
52.6804720139067));
#190905=CARTESIAN_POINT('Origin',(122.377380428518,-0.999999999999985,65.0728746711936));
#190906=CARTESIAN_POINT('Origin',(114.524364387726,1.45439216225896E-14,
63.5463953680056));
#190907=CARTESIAN_POINT('Origin',(122.573705829538,-1.3,65.1110366537733));
#190908=CARTESIAN_POINT('',(122.531336174176,-1.8,65.3290085466811));
#190909=CARTESIAN_POINT('',(122.463436480413,-1.8,65.6783204457488));
#190910=CARTESIAN_POINT('',(122.531336174176,-1.8,65.3290085466811));
#190911=CARTESIAN_POINT('',(122.519971674893,-1.3,65.3874735353515));
#190912=CARTESIAN_POINT('Origin',(125.008519822253,1.45439216225896E-14,
52.5850670574574));
#190913=CARTESIAN_POINT('',(122.452373842004,-1.3,65.7352325025978));
#190914=CARTESIAN_POINT('',(122.519971674893,-1.3,65.3874735353515));
#190915=CARTESIAN_POINT('Origin',(125.008519822253,1.45439216225896E-14,
52.5850670574574));
#190916=CARTESIAN_POINT('Origin',(122.573705829538,-1.8,65.1110366537733));
#190917=CARTESIAN_POINT('',(123.064519332087,-1.8,65.2064416102226));
#190918=CARTESIAN_POINT('',(123.015425507724,-1.8,65.4590061811456));
#190919=CARTESIAN_POINT('',(123.064519332087,-1.8,65.2064416102226));
#190920=CARTESIAN_POINT('',(122.908875583955,-1.8,65.1761873793691));
#190921=CARTESIAN_POINT('',(122.908875583955,-1.8,65.1761873793691));
#190922=CARTESIAN_POINT('Origin',(116.959178380441,-1.8,51.0204257716897));
#190923=CARTESIAN_POINT('Origin',(116.959178380441,-1.8,51.0204257716897));
#190924=CARTESIAN_POINT('Origin',(123.064519332087,-1.8,65.2064416102226));
#190925=CARTESIAN_POINT('',(123.064519332087,-1.3,65.2064416102226));
#190926=CARTESIAN_POINT('',(123.004091633267,-1.3,65.5173136195258));
#190927=CARTESIAN_POINT('',(123.064519332087,-1.3,65.2064416102226));
#190928=CARTESIAN_POINT('',(123.064519332087,-1.8,65.2064416102226));
#190929=CARTESIAN_POINT('Origin',(125.499333324803,1.45439216225896E-14,
52.6804720139067));
#190930=CARTESIAN_POINT('Origin',(123.064519332087,-1.3,65.2064416102226));
#190931=CARTESIAN_POINT('',(122.997474498203,-1.3,65.1934093496517));
#190932=CARTESIAN_POINT('Origin',(116.959178380441,-1.3,51.0204257716897));
#190933=CARTESIAN_POINT('',(123.064519332087,-1.3,65.2064416102226));
#190934=CARTESIAN_POINT('Origin',(116.959178380441,-1.3,51.0204257716897));
#190935=CARTESIAN_POINT('Origin',(122.377380428518,-2.,65.0728746711936));
#190936=CARTESIAN_POINT('Origin',(114.524364387726,1.45439216225896E-14,
63.5463953680056));
#190937=CARTESIAN_POINT('Origin',(122.573705829538,-2.3,65.1110366537733));
#190938=CARTESIAN_POINT('',(122.565374292175,-2.8,65.1538984838808));
#190939=CARTESIAN_POINT('',(122.496554362349,-2.8,65.5079445634598));
#190940=CARTESIAN_POINT('',(122.565374292175,-2.8,65.1538984838808));
#190941=CARTESIAN_POINT('',(122.54644720768,-2.3,65.2512694065221));
#190942=CARTESIAN_POINT('Origin',(125.008519822253,1.45439216225896E-14,
52.5850670574574));
#190943=CARTESIAN_POINT('',(122.478141994724,-2.3,65.6026675105714));
#190944=CARTESIAN_POINT('',(122.54644720768,-2.3,65.2512694065221));
#190945=CARTESIAN_POINT('Origin',(125.008519822253,1.45439216225896E-14,
52.5850670574574));
#190946=CARTESIAN_POINT('Origin',(122.573705829538,-2.8,65.1110366537733));
#190947=CARTESIAN_POINT('',(123.064519332087,-2.8,65.2064416102226));
#190948=CARTESIAN_POINT('',(123.04937020292,-2.8,65.2843767345985));
#190949=CARTESIAN_POINT('',(123.064519332087,-2.8,65.2064416102226));
#190950=CARTESIAN_POINT('',(122.640244299654,-2.8,65.1239704867072));
#190951=CARTESIAN_POINT('',(122.640244299654,-2.8,65.1239704867072));
#190952=CARTESIAN_POINT('Origin',(116.959178380441,-2.8,51.0204257716897));
#190953=CARTESIAN_POINT('Origin',(116.959178380441,-2.8,51.0204257716897));
#190954=CARTESIAN_POINT('Origin',(123.064519332087,-2.8,65.2064416102226));
#190955=CARTESIAN_POINT('',(123.064519332087,-2.3,65.2064416102226));
#190956=CARTESIAN_POINT('',(123.030495384216,-2.3,65.3814787743977));
#190957=CARTESIAN_POINT('',(123.064519332087,-2.3,65.2064416102226));
#190958=CARTESIAN_POINT('',(123.064519332087,-2.8,65.2064416102226));
#190959=CARTESIAN_POINT('Origin',(125.499333324803,1.45439216225896E-14,
52.6804720139067));
#190960=CARTESIAN_POINT('Origin',(123.064519332087,-2.3,65.2064416102226));
#190961=CARTESIAN_POINT('',(122.790237920908,-2.3,65.1531264386707));
#190962=CARTESIAN_POINT('Origin',(116.959178380441,-2.3,51.0204257716897));
#190963=CARTESIAN_POINT('',(123.064519332087,-2.3,65.2064416102226));
#190964=CARTESIAN_POINT('Origin',(116.959178380441,-2.3,51.0204257716897));
#190965=CARTESIAN_POINT('Origin',(122.377380428518,-3.,65.0728746711936));
#190966=CARTESIAN_POINT('Origin',(114.524364387726,1.45439216225896E-14,
63.5463953680056));
#190967=CARTESIAN_POINT('Origin',(120.11963831679,-6.3,64.6340118715271));
#190968=CARTESIAN_POINT('',(119.55904893793,-6.3,64.8975708884388));
#190969=CARTESIAN_POINT('',(119.491872720657,-6.3,65.2431608422003));
#190970=CARTESIAN_POINT('',(119.55904893793,-6.3,64.8975708884388));
#190971=CARTESIAN_POINT('',(120.089793203781,-6.3,64.7875509013147));
#190972=CARTESIAN_POINT('Origin',(116.959178380441,-6.3,51.0204257716897));
#190973=CARTESIAN_POINT('',(120.021557740431,-6.3,65.13859017654));
#190974=CARTESIAN_POINT('',(120.089793203781,-6.3,64.7875509013147));
#190975=CARTESIAN_POINT('Origin',(116.959178380441,-6.3,51.0204257716897));
#190976=CARTESIAN_POINT('Origin',(119.628824814241,-6.3,64.5386069150778));
#190977=CARTESIAN_POINT('',(119.607117843827,-6.8,64.6502790396187));
#190978=CARTESIAN_POINT('',(119.538662444116,-6.8,65.0024497836874));
#190979=CARTESIAN_POINT('',(119.607117843827,-6.8,64.6502790396187));
#190980=CARTESIAN_POINT('Origin',(122.063638806956,1.45439216225896E-14,
52.0126373187619));
#190981=CARTESIAN_POINT('Origin',(122.063638806956,1.45439216225896E-14,
52.0126373187619));
#190982=CARTESIAN_POINT('Origin',(119.628824814241,-6.8,64.5386069150778));
#190983=CARTESIAN_POINT('',(120.11963831679,-6.8,64.6340118715271));
#190984=CARTESIAN_POINT('',(120.06907915275,-6.8,64.8941149239462));
#190985=CARTESIAN_POINT('',(120.11963831679,-6.8,64.6340118715271));
#190986=CARTESIAN_POINT('',(119.897035062789,-6.8,64.5907419662716));
#190987=CARTESIAN_POINT('',(119.897035062789,-6.8,64.5907419662716));
#190988=CARTESIAN_POINT('Origin',(116.959178380441,-6.8,51.0204257716897));
#190989=CARTESIAN_POINT('Origin',(116.959178380441,-6.8,51.0204257716897));
#190990=CARTESIAN_POINT('Origin',(120.11963831679,-6.8,64.6340118715271));
#190991=CARTESIAN_POINT('',(120.11963831679,-6.61107026131199,64.6340118715271));
#190992=CARTESIAN_POINT('Origin',(122.554452309506,1.45439216225896E-14,
52.1080422752111));
#190993=CARTESIAN_POINT('',(120.11963831679,-6.8,64.6340118715271));
#190994=CARTESIAN_POINT('Origin',(122.554452309506,1.45439216225896E-14,
52.1080422752111));
#190995=CARTESIAN_POINT('Origin',(119.432499413221,-7.,64.5004449324981));
#190996=CARTESIAN_POINT('Origin',(114.524364387726,1.45439216225896E-14,
63.5463953680056));
#190997=CARTESIAN_POINT('Origin',(118.647197809142,-6.8,64.3477970021793));
#190998=CARTESIAN_POINT('',(119.079891904685,-6.8,64.7421988952723));
#190999=CARTESIAN_POINT('',(119.012409844747,-6.8,65.0893622652905));
#191000=CARTESIAN_POINT('',(119.079891904685,-6.8,64.7421988952723));
#191001=CARTESIAN_POINT('',(118.556792124843,-6.8,64.8128916074539));
#191002=CARTESIAN_POINT('Origin',(116.959178380441,-6.8,51.0204257716897));
#191003=CARTESIAN_POINT('',(118.490150538636,-6.8,65.1557311365441));
#191004=CARTESIAN_POINT('',(118.556792124843,-6.8,64.8128916074539));
#191005=CARTESIAN_POINT('Origin',(116.959178380441,-6.8,51.0204257716897));
#191006=CARTESIAN_POINT('Origin',(119.138011311691,-6.8,64.4432019586286));
#191007=CARTESIAN_POINT('',(119.032511917208,-6.3,64.9859465837563));
#191008=CARTESIAN_POINT('',(118.966256200048,-6.3,65.3268009985918));
#191009=CARTESIAN_POINT('',(119.032511917208,-6.3,64.9859465837563));
#191010=CARTESIAN_POINT('Origin',(121.572825304407,1.45439216225896E-14,
51.9172323623126));
#191011=CARTESIAN_POINT('Origin',(121.572825304407,1.45439216225896E-14,
51.9172323623126));
#191012=CARTESIAN_POINT('Origin',(119.138011311691,-6.3,64.4432019586286));
#191013=CARTESIAN_POINT('',(118.510006827735,-6.3,65.053579894478));
#191014=CARTESIAN_POINT('',(118.444547114411,-6.3,65.3903392450207));
#191015=CARTESIAN_POINT('',(118.510006827735,-6.3,65.053579894478));
#191016=CARTESIAN_POINT('Origin',(116.959178380441,-6.3,51.0204257716897));
#191017=CARTESIAN_POINT('Origin',(116.959178380441,-6.3,51.0204257716897));
#191018=CARTESIAN_POINT('Origin',(118.647197809142,-6.3,64.3477970021793));
#191019=CARTESIAN_POINT('Origin',(121.082011801857,1.45439216225896E-14,
51.8218274058634));
#191020=CARTESIAN_POINT('Origin',(121.082011801857,1.45439216225896E-14,
51.8218274058634));
#191021=CARTESIAN_POINT('Origin',(117.665570804043,-6.8,64.1569870892808));
#191022=CARTESIAN_POINT('',(118.037661989115,-6.8,64.8631623729813));
#191023=CARTESIAN_POINT('',(117.971740706963,-6.8,65.2022962774431));
#191024=CARTESIAN_POINT('',(118.037661989115,-6.8,64.8631623729813));
#191025=CARTESIAN_POINT('',(117.522370687732,-6.8,64.8936841464147));
#191026=CARTESIAN_POINT('Origin',(116.959178380441,-6.8,51.0204257716897));
#191027=CARTESIAN_POINT('',(117.457059781373,-6.8,65.2296779553086));
#191028=CARTESIAN_POINT('',(117.522370687732,-6.8,64.8936841464147));
#191029=CARTESIAN_POINT('Origin',(116.959178380441,-6.8,51.0204257716897));
#191030=CARTESIAN_POINT('Origin',(118.156384306592,-6.8,64.25239204573));
#191031=CARTESIAN_POINT('',(117.991386218174,-6.3,65.1012293881955));
#191032=CARTESIAN_POINT('',(117.926609541577,-6.3,65.4344748369367));
#191033=CARTESIAN_POINT('',(117.991386218174,-6.3,65.1012293881955));
#191034=CARTESIAN_POINT('Origin',(120.591198299308,1.45439216225896E-14,
51.7264224494141));
#191035=CARTESIAN_POINT('Origin',(120.591198299308,1.45439216225896E-14,
51.7264224494141));
#191036=CARTESIAN_POINT('Origin',(118.156384306592,-6.3,64.25239204573));
#191037=CARTESIAN_POINT('',(117.476526584872,-6.3,65.1295304329511));
#191038=CARTESIAN_POINT('',(117.412329308735,-6.3,65.4597951396044));
#191039=CARTESIAN_POINT('',(117.476526584872,-6.3,65.1295304329511));
#191040=CARTESIAN_POINT('Origin',(116.959178380441,-6.3,51.0204257716897));
#191041=CARTESIAN_POINT('Origin',(116.959178380441,-6.3,51.0204257716897));
#191042=CARTESIAN_POINT('Origin',(117.665570804043,-6.3,64.1569870892808));
#191043=CARTESIAN_POINT('Origin',(120.100384796758,1.45439216225896E-14,
51.6310174929649));
#191044=CARTESIAN_POINT('Origin',(120.100384796758,1.45439216225896E-14,
51.6310174929649));
#191045=CARTESIAN_POINT('Origin',(116.683943798944,-6.8,63.9661771763823));
#191046=CARTESIAN_POINT('',(117.010809744205,-6.8,64.9050149881251));
#191047=CARTESIAN_POINT('',(116.946007519038,-6.8,65.2383918722067));
#191048=CARTESIAN_POINT('',(117.010809744205,-6.8,64.9050149881251));
#191049=CARTESIAN_POINT('',(116.50289039636,-6.8,64.8976115376352));
#191050=CARTESIAN_POINT('Origin',(116.959178380441,-6.8,51.0204257716897));
#191051=CARTESIAN_POINT('',(116.438501717996,-6.8,65.2288609184699));
#191052=CARTESIAN_POINT('',(116.50289039636,-6.8,64.8976115376352));
#191053=CARTESIAN_POINT('Origin',(116.959178380441,-6.8,51.0204257716897));
#191054=CARTESIAN_POINT('Origin',(117.174757301493,-6.8,64.0615821328315));
#191055=CARTESIAN_POINT('',(116.965325321626,-6.3,65.139010889263));
#191056=CARTESIAN_POINT('',(116.901611332515,-6.3,65.466789312112));
#191057=CARTESIAN_POINT('',(116.965325321626,-6.3,65.139010889263));
#191058=CARTESIAN_POINT('Origin',(119.609571294209,1.45439216225896E-14,
51.5356125365156));
#191059=CARTESIAN_POINT('Origin',(119.609571294209,1.45439216225896E-14,
51.5356125365156));
#191060=CARTESIAN_POINT('Origin',(117.174757301493,-6.3,64.0615821328315));
#191061=CARTESIAN_POINT('',(116.457698341079,-6.3,65.1301033469199));
#191062=CARTESIAN_POINT('',(116.394377533667,-6.3,65.4558590353759));
#191063=CARTESIAN_POINT('',(116.457698341079,-6.3,65.1301033469199));
#191064=CARTESIAN_POINT('Origin',(116.959178380441,-6.3,51.0204257716897));
#191065=CARTESIAN_POINT('Origin',(116.959178380441,-6.3,51.0204257716897));
#191066=CARTESIAN_POINT('Origin',(116.683943798944,-6.3,63.9661771763823));
#191067=CARTESIAN_POINT('Origin',(119.118757791659,1.45439216225896E-14,
51.4402075800664));
#191068=CARTESIAN_POINT('Origin',(119.118757791659,1.45439216225896E-14,
51.4402075800664));
#191069=CARTESIAN_POINT('Origin',(115.702316793845,-6.8,63.7753672634838));
#191070=CARTESIAN_POINT('',(115.998541570931,-6.8,64.8718394333745));
#191071=CARTESIAN_POINT('',(115.934476441709,-6.8,65.2014243064807));
#191072=CARTESIAN_POINT('',(115.998541570931,-6.8,64.8718394333745));
#191073=CARTESIAN_POINT('',(115.497708336948,-6.8,64.8279812692763));
#191074=CARTESIAN_POINT('Origin',(116.959178380441,-6.8,51.0204257716897));
#191075=CARTESIAN_POINT('',(115.433880657895,-6.8,65.1563445732553));
#191076=CARTESIAN_POINT('',(115.497708336948,-6.8,64.8279812692763));
#191077=CARTESIAN_POINT('Origin',(116.959178380441,-6.8,51.0204257716897));
#191078=CARTESIAN_POINT('Origin',(116.193130296394,-6.8,63.870772219933));
#191079=CARTESIAN_POINT('',(115.95357822888,-6.3,65.1031546209663));
#191080=CARTESIAN_POINT('',(115.890565211466,-6.3,65.4273268750535));
#191081=CARTESIAN_POINT('',(115.95357822888,-6.3,65.1031546209663));
#191082=CARTESIAN_POINT('Origin',(118.62794428911,1.45439216225896E-14,
51.3448026236171));
#191083=CARTESIAN_POINT('Origin',(118.62794428911,1.45439216225896E-14,
51.3448026236171));
#191084=CARTESIAN_POINT('Origin',(116.193130296394,-6.3,63.870772219933));
#191085=CARTESIAN_POINT('',(115.4529128302,-6.3,65.0584330233987));
#191086=CARTESIAN_POINT('',(115.390125794234,-6.3,65.381442709521));
#191087=CARTESIAN_POINT('',(115.4529128302,-6.3,65.0584330233987));
#191088=CARTESIAN_POINT('Origin',(116.959178380441,-6.3,51.0204257716897));
#191089=CARTESIAN_POINT('Origin',(116.959178380441,-6.3,51.0204257716897));
#191090=CARTESIAN_POINT('Origin',(115.702316793845,-6.3,63.7753672634838));
#191091=CARTESIAN_POINT('Origin',(118.13713078656,1.45439216225896E-14,
51.2493976671679));
#191092=CARTESIAN_POINT('Origin',(118.13713078656,1.45439216225896E-14,
51.2493976671679));
#191093=CARTESIAN_POINT('Origin',(114.720689788746,-6.8,63.5845573505853));
#191094=CARTESIAN_POINT('',(115.000350755645,-6.8,64.7662425114558));
#191095=CARTESIAN_POINT('',(114.936677223071,-6.8,65.0938128045052));
#191096=CARTESIAN_POINT('',(115.000350755645,-6.8,64.7662425114558));
#191097=CARTESIAN_POINT('',(114.506443068771,-6.8,64.6867556739635));
#191098=CARTESIAN_POINT('Origin',(116.959178380441,-6.8,51.0204257716897));
#191099=CARTESIAN_POINT('',(114.442842164132,-6.8,65.013952330542));
#191100=CARTESIAN_POINT('',(114.506443068771,-6.8,64.6867556739635));
#191101=CARTESIAN_POINT('Origin',(116.959178380441,-6.8,51.0204257716897));
#191102=CARTESIAN_POINT('Origin',(115.211503291295,-6.8,63.6799623070345));
#191103=CARTESIAN_POINT('',(114.955664196196,-6.3,64.9961337831114));
#191104=CARTESIAN_POINT('',(114.89302390524,-6.3,65.3183885353702));
#191105=CARTESIAN_POINT('',(114.955664196196,-6.3,64.9961337831114));
#191106=CARTESIAN_POINT('Origin',(117.64631728401,1.45439216225896E-14,
51.1539927107186));
#191107=CARTESIAN_POINT('Origin',(117.64631728401,1.45439216225896E-14,
51.1539927107186));
#191108=CARTESIAN_POINT('Origin',(115.211503291295,-6.3,63.6799623070345));
#191109=CARTESIAN_POINT('',(114.461807839218,-6.3,64.9163828775102));
#191110=CARTESIAN_POINT('',(114.399236700813,-6.3,65.2382818725149));
#191111=CARTESIAN_POINT('',(114.461807839218,-6.3,64.9163828775102));
#191112=CARTESIAN_POINT('Origin',(116.959178380441,-6.3,51.0204257716897));
#191113=CARTESIAN_POINT('Origin',(116.959178380441,-6.3,51.0204257716897));
#191114=CARTESIAN_POINT('Origin',(114.720689788746,-6.3,63.5845573505853));
#191115=CARTESIAN_POINT('Origin',(117.155503781461,1.45439216225896E-14,
51.0585877542694));
#191116=CARTESIAN_POINT('Origin',(117.155503781461,1.45439216225896E-14,
51.0585877542694));
#191117=CARTESIAN_POINT('Origin',(113.739062783647,-6.8,63.3937474376868));
#191118=CARTESIAN_POINT('',(114.015973185983,-6.8,64.589582955916));
#191119=CARTESIAN_POINT('',(113.952364223845,-6.8,64.9168210645219));
#191120=CARTESIAN_POINT('',(114.015973185983,-6.8,64.589582955916));
#191121=CARTESIAN_POINT('',(113.528942447158,-6.8,64.4747174642696));
#191122=CARTESIAN_POINT('Origin',(116.959178380441,-6.8,51.0204257716897));
#191123=CARTESIAN_POINT('',(113.465244649916,-6.8,64.802412587586));
#191124=CARTESIAN_POINT('',(113.528942447158,-6.8,64.4747174642696));
#191125=CARTESIAN_POINT('Origin',(116.959178380441,-6.8,51.0204257716897));
#191126=CARTESIAN_POINT('Origin',(114.229876286196,-6.8,63.489152394136));
#191127=CARTESIAN_POINT('',(113.971332261843,-6.3,64.8192394554237));
#191128=CARTESIAN_POINT('',(113.908753451129,-6.3,65.1411779208355));
#191129=CARTESIAN_POINT('',(113.971332261843,-6.3,64.8192394554237));
#191130=CARTESIAN_POINT('Origin',(116.664690278911,1.45439216225896E-14,
50.9631827978201));
#191131=CARTESIAN_POINT('Origin',(116.664690278911,1.45439216225896E-14,
50.9631827978201));
#191132=CARTESIAN_POINT('Origin',(114.229876286196,-6.3,63.489152394136));
#191133=CARTESIAN_POINT('',(113.484238738346,-6.3,64.7046969613014));
#191134=CARTESIAN_POINT('',(113.421575345531,-6.3,65.0270705617333));
#191135=CARTESIAN_POINT('',(113.484238738346,-6.3,64.7046969613014));
#191136=CARTESIAN_POINT('Origin',(116.959178380441,-6.3,51.0204257716897));
#191137=CARTESIAN_POINT('Origin',(116.959178380441,-6.3,51.0204257716897));
#191138=CARTESIAN_POINT('Origin',(113.739062783647,-6.3,63.3937474376868));
#191139=CARTESIAN_POINT('Origin',(116.173876776362,1.45439216225896E-14,
50.8677778413709));
#191140=CARTESIAN_POINT('Origin',(116.173876776362,1.45439216225896E-14,
50.8677778413709));
#191141=CARTESIAN_POINT('Origin',(112.757435778548,-6.8,63.2029375247883));
#191142=CARTESIAN_POINT('',(113.045365648647,-6.8,64.3420830787778));
#191143=CARTESIAN_POINT('',(112.981497218279,-6.8,64.6706560290523));
#191144=CARTESIAN_POINT('',(113.045365648647,-6.8,64.3420830787778));
#191145=CARTESIAN_POINT('',(112.565271334663,-6.8,64.191532952939));
#191146=CARTESIAN_POINT('Origin',(116.959178380441,-6.8,51.0204257716897));
#191147=CARTESIAN_POINT('',(112.501148491679,-6.8,64.5214147361248));
#191148=CARTESIAN_POINT('',(112.565271334663,-6.8,64.191532952939));
#191149=CARTESIAN_POINT('Origin',(116.959178380441,-6.8,51.0204257716897));
#191150=CARTESIAN_POINT('Origin',(113.248249281097,-6.8,63.2983424812375));
#191151=CARTESIAN_POINT('',(113.000541338854,-6.3,64.572683010979));
#191152=CARTESIAN_POINT('',(112.937715514028,-6.3,64.8958922474905));
#191153=CARTESIAN_POINT('',(113.000541338854,-6.3,64.572683010979));
#191154=CARTESIAN_POINT('Origin',(115.683063273812,1.45439216225896E-14,
50.7723728849216));
#191155=CARTESIAN_POINT('Origin',(115.683063273812,1.45439216225896E-14,
50.7723728849216));
#191156=CARTESIAN_POINT('Origin',(113.248249281097,-6.3,63.2983424812375));
#191157=CARTESIAN_POINT('',(112.520267197199,-6.3,64.42305801369));
#191158=CARTESIAN_POINT('',(112.457199265932,-6.3,64.7475127736486));
#191159=CARTESIAN_POINT('',(112.520267197199,-6.3,64.42305801369));
#191160=CARTESIAN_POINT('Origin',(116.959178380441,-6.3,51.0204257716897));
#191161=CARTESIAN_POINT('Origin',(116.959178380441,-6.3,51.0204257716897));
#191162=CARTESIAN_POINT('Origin',(112.757435778548,-6.3,63.2029375247883));
#191163=CARTESIAN_POINT('Origin',(115.192249771263,1.45439216225896E-14,
50.6769679284724));
#191164=CARTESIAN_POINT('Origin',(115.192249771263,1.45439216225896E-14,
50.6769679284724));
#191165=CARTESIAN_POINT('Origin',(111.775808773449,-6.8,63.0121276118898));
#191166=CARTESIAN_POINT('',(112.088702367317,-6.8,64.0228465813954));
#191167=CARTESIAN_POINT('',(112.024238324945,-6.8,64.354483674506));
#191168=CARTESIAN_POINT('',(112.088702367317,-6.8,64.0228465813954));
#191169=CARTESIAN_POINT('',(111.615716802316,-6.8,63.8357252949231));
#191170=CARTESIAN_POINT('Origin',(116.959178380441,-6.8,51.0204257716897));
#191171=CARTESIAN_POINT('',(111.550820639722,-6.8,64.169585442765));
#191172=CARTESIAN_POINT('',(111.615716802316,-6.8,63.8357252949231));
#191173=CARTESIAN_POINT('Origin',(116.959178380441,-6.8,51.0204257716897));
#191174=CARTESIAN_POINT('Origin',(112.266622275998,-6.8,63.107532568339));
#191175=CARTESIAN_POINT('',(112.043457034551,-6.3,64.2556124782166));
#191176=CARTESIAN_POINT('',(111.980064555798,-6.3,64.5817368819136));
#191177=CARTESIAN_POINT('',(112.043457034551,-6.3,64.2556124782166));
#191178=CARTESIAN_POINT('Origin',(114.701436268713,1.45439216225896E-14,
50.5815629720231));
#191179=CARTESIAN_POINT('Origin',(114.701436268713,1.45439216225896E-14,
50.5815629720231));
#191180=CARTESIAN_POINT('Origin',(112.266622275998,-6.3,63.107532568339));
#191181=CARTESIAN_POINT('',(111.570165962703,-6.3,64.0700628803767));
#191182=CARTESIAN_POINT('',(111.506362697021,-6.3,64.3983005890775));
#191183=CARTESIAN_POINT('',(111.570165962703,-6.3,64.0700628803767));
#191184=CARTESIAN_POINT('Origin',(116.959178380441,-6.3,51.0204257716897));
#191185=CARTESIAN_POINT('Origin',(116.959178380441,-6.3,51.0204257716897));
#191186=CARTESIAN_POINT('Origin',(111.775808773449,-6.3,63.0121276118898));
#191187=CARTESIAN_POINT('Origin',(114.210622766164,1.45439216225896E-14,
50.4861580155739));
#191188=CARTESIAN_POINT('Origin',(114.210622766164,1.45439216225896E-14,
50.4861580155739));
#191189=CARTESIAN_POINT('Origin',(110.79418176835,-6.8,62.8213176989913));
#191190=CARTESIAN_POINT('',(111.146389113021,-6.8,63.6297859632063));
#191191=CARTESIAN_POINT('',(111.080964504615,-6.8,63.9663647155047));
#191192=CARTESIAN_POINT('',(111.146389113021,-6.8,63.6297859632063));
#191193=CARTESIAN_POINT('',(110.680811825332,-6.8,63.4045525841295));
#191194=CARTESIAN_POINT('Origin',(116.959178380441,-6.8,51.0204257716897));
#191195=CARTESIAN_POINT('',(110.61475557299,-6.8,63.7443808465566));
#191196=CARTESIAN_POINT('',(110.680811825332,-6.8,63.4045525841295));
#191197=CARTESIAN_POINT('Origin',(116.959178380441,-6.8,51.0204257716897));
#191198=CARTESIAN_POINT('Origin',(111.284995270899,-6.8,62.9167226554405));
#191199=CARTESIAN_POINT('',(111.100464604885,-6.3,63.8660458969672));
#191200=CARTESIAN_POINT('',(111.036159355032,-6.3,64.1968660774633));
#191201=CARTESIAN_POINT('',(111.100464604885,-6.3,63.8660458969672));
#191202=CARTESIAN_POINT('Origin',(113.719809263614,1.45439216225896E-14,
50.3907530591246));
#191203=CARTESIAN_POINT('Origin',(113.719809263614,1.45439216225896E-14,
50.3907530591246));
#191204=CARTESIAN_POINT('Origin',(111.284995270899,-6.3,62.9167226554405));
#191205=CARTESIAN_POINT('',(110.634440589158,-6.3,63.6431107229422));
#191206=CARTESIAN_POINT('',(110.569535866522,-6.3,63.9770149081617));
#191207=CARTESIAN_POINT('',(110.634440589158,-6.3,63.6431107229422));
#191208=CARTESIAN_POINT('Origin',(116.959178380441,-6.3,51.0204257716897));
#191209=CARTESIAN_POINT('Origin',(116.959178380441,-6.3,51.0204257716897));
#191210=CARTESIAN_POINT('Origin',(110.79418176835,-6.3,62.8213176989913));
#191211=CARTESIAN_POINT('Origin',(113.228995761065,1.45439216225896E-14,
50.2953481026754));
#191212=CARTESIAN_POINT('Origin',(113.228995761065,1.45439216225896E-14,
50.2953481026754));
#191213=CARTESIAN_POINT('Origin',(109.812554763251,-6.8,62.6305077860928));
#191214=CARTESIAN_POINT('',(110.219097651412,-6.8,63.1594453067728));
#191215=CARTESIAN_POINT('',(110.152297951675,-6.8,63.5030982553971));
#191216=CARTESIAN_POINT('',(110.219097651412,-6.8,63.1594453067728));
#191217=CARTESIAN_POINT('',(109.761382244793,-6.8,62.8937662576995));
#191218=CARTESIAN_POINT('Origin',(116.959178380441,-6.8,51.0204257716897));
#191219=CARTESIAN_POINT('',(109.693716601825,-6.8,63.241874075816));
#191220=CARTESIAN_POINT('',(109.761382244793,-6.8,62.8937662576995));
#191221=CARTESIAN_POINT('Origin',(116.959178380441,-6.8,51.0204257716897));
#191222=CARTESIAN_POINT('Origin',(110.3033682658,-6.8,62.725912742542));
#191223=CARTESIAN_POINT('',(110.172200491729,-6.3,63.4007090739833));
#191224=CARTESIAN_POINT('',(110.106590949423,-6.3,63.7382392239751));
#191225=CARTESIAN_POINT('',(110.172200491729,-6.3,63.4007090739833));
#191226=CARTESIAN_POINT('Origin',(112.738182258515,1.45439216225896E-14,
50.1999431462261));
#191227=CARTESIAN_POINT('Origin',(112.738182258515,1.45439216225896E-14,
50.1999431462261));
#191228=CARTESIAN_POINT('Origin',(110.3033682658,-6.3,62.725912742542));
#191229=CARTESIAN_POINT('',(109.713872337286,-6.3,63.1381823234563));
#191230=CARTESIAN_POINT('',(109.647442892777,-6.3,63.4799304835687));
#191231=CARTESIAN_POINT('',(109.713872337286,-6.3,63.1381823234563));
#191232=CARTESIAN_POINT('Origin',(116.959178380441,-6.3,51.0204257716897));
#191233=CARTESIAN_POINT('Origin',(116.959178380441,-6.3,51.0204257716897));
#191234=CARTESIAN_POINT('Origin',(109.812554763251,-6.3,62.6305077860928));
#191235=CARTESIAN_POINT('Origin',(112.247368755966,1.45439216225896E-14,
50.1045381897769));
#191236=CARTESIAN_POINT('Origin',(112.247368755966,1.45439216225896E-14,
50.1045381897769));
#191237=CARTESIAN_POINT('Origin',(109.321741260701,-6.8,62.5351028296435));
#191238=CARTESIAN_POINT('',(109.259608804648,-6.3,62.8547450108513));
#191239=CARTESIAN_POINT('',(109.192232348899,-6.3,63.2013650971262));
#191240=CARTESIAN_POINT('',(109.259608804648,-6.3,62.8547450108513));
#191241=CARTESIAN_POINT('',(109.307827747489,-6.8,62.6066812927165));
#191242=CARTESIAN_POINT('Origin',(111.756555253416,1.45439216225896E-14,
50.0091332333276));
#191243=CARTESIAN_POINT('',(109.239160411739,-6.8,62.9599423477459));
#191244=CARTESIAN_POINT('',(109.307827747489,-6.8,62.6066812927165));
#191245=CARTESIAN_POINT('Origin',(111.756555253416,1.45439216225896E-14,
50.0091332333276));
#191246=CARTESIAN_POINT('Origin',(109.321741260701,-6.3,62.5351028296435));
#191247=CARTESIAN_POINT('',(108.809591344001,-6.3,62.5494636605398));
#191248=CARTESIAN_POINT('',(108.741125896572,-6.3,62.9016860953786));
#191249=CARTESIAN_POINT('',(108.809591344001,-6.3,62.5494636605398));
#191250=CARTESIAN_POINT('Origin',(116.959178380441,-6.3,51.0204257716897));
#191251=CARTESIAN_POINT('Origin',(116.959178380441,-6.3,51.0204257716897));
#191252=CARTESIAN_POINT('Origin',(108.830927758152,-6.3,62.4396978731943));
#191253=CARTESIAN_POINT('',(108.830927758152,-6.8,62.4396978731943));
#191254=CARTESIAN_POINT('',(108.78880613563,-6.8,62.6563937541252));
#191255=CARTESIAN_POINT('',(108.830927758152,-6.8,62.4396978731943));
#191256=CARTESIAN_POINT('',(108.830927758152,-6.52351515672298,62.4396978731943));
#191257=CARTESIAN_POINT('',(108.830927758152,-6.52351515672298,62.4396978731943));
#191258=CARTESIAN_POINT('Origin',(111.265741750867,1.45439216225896E-14,
49.9137282768784));
#191259=CARTESIAN_POINT('Origin',(111.265741750867,1.45439216225896E-14,
49.9137282768784));
#191260=CARTESIAN_POINT('Origin',(108.830927758152,-6.8,62.4396978731943));
#191261=CARTESIAN_POINT('',(109.151693712662,-6.8,62.5020487697396));
#191262=CARTESIAN_POINT('Origin',(116.959178380441,-6.8,51.0204257716897));
#191263=CARTESIAN_POINT('',(108.830927758152,-6.8,62.4396978731943));
#191264=CARTESIAN_POINT('Origin',(116.959178380441,-6.8,51.0204257716897));
#191265=CARTESIAN_POINT('Origin',(108.634602357132,-7.,62.4015358906146));
#191266=CARTESIAN_POINT('Origin',(114.524364387726,1.45439216225896E-14,
63.5463953680056));
#191267=CARTESIAN_POINT('Origin',(108.340114255602,-5.8,62.344292916745));
#191268=CARTESIAN_POINT('',(108.277981799549,-5.3,62.6639350979528));
#191269=CARTESIAN_POINT('',(108.2106053438,-5.3,63.0105551842277));
#191270=CARTESIAN_POINT('',(108.277981799549,-5.3,62.6639350979528));
#191271=CARTESIAN_POINT('',(108.318777841451,-5.8,62.4540587040905));
#191272=CARTESIAN_POINT('Origin',(110.774928248317,1.45439216225896E-14,
49.8183233204291));
#191273=CARTESIAN_POINT('',(108.250312394022,-5.8,62.8062811389293));
#191274=CARTESIAN_POINT('',(108.318777841451,-5.8,62.4540587040905));
#191275=CARTESIAN_POINT('Origin',(110.774928248317,1.45439216225896E-14,
49.8183233204291));
#191276=CARTESIAN_POINT('Origin',(108.340114255602,-5.3,62.344292916745));
#191277=CARTESIAN_POINT('',(107.835387239841,-5.3,62.3204664233688));
#191278=CARTESIAN_POINT('',(107.766719904091,-5.3,62.6737274783981));
#191279=CARTESIAN_POINT('',(107.835387239841,-5.3,62.3204664233688));
#191280=CARTESIAN_POINT('Origin',(116.959178380441,-5.3,51.0204257716897));
#191281=CARTESIAN_POINT('Origin',(116.959178380441,-5.3,51.0204257716897));
#191282=CARTESIAN_POINT('Origin',(107.849300753053,-5.3,62.2488879602958));
#191283=CARTESIAN_POINT('',(107.849300753053,-5.8,62.2488879602958));
#191284=CARTESIAN_POINT('',(107.807179130531,-5.8,62.4655838412267));
#191285=CARTESIAN_POINT('',(107.849300753053,-5.8,62.2488879602958));
#191286=CARTESIAN_POINT('',(107.849300753053,-5.47323030759699,62.2488879602958));
#191287=CARTESIAN_POINT('',(107.849300753053,-5.47323030759699,62.2488879602958));
#191288=CARTESIAN_POINT('Origin',(110.284114745768,1.45439216225896E-14,
49.7229183639799));
#191289=CARTESIAN_POINT('Origin',(110.284114745768,1.45439216225896E-14,
49.7229183639799));
#191290=CARTESIAN_POINT('Origin',(107.849300753053,-5.8,62.2488879602958));
#191291=CARTESIAN_POINT('',(108.120705741714,-5.8,62.3016440091592));
#191292=CARTESIAN_POINT('Origin',(116.959178380441,-5.8,51.0204257716897));
#191293=CARTESIAN_POINT('',(107.849300753053,-5.8,62.2488879602958));
#191294=CARTESIAN_POINT('Origin',(116.959178380441,-5.8,51.0204257716897));
#191295=CARTESIAN_POINT('Origin',(107.652975352033,-6.,62.2107259777161));
#191296=CARTESIAN_POINT('Origin',(114.524364387726,1.45439216225896E-14,
63.5463953680056));
#191297=CARTESIAN_POINT('Origin',(107.849300753053,-4.8,62.2488879602958));
#191298=CARTESIAN_POINT('',(108.241431829638,-4.8,62.8519674541085));
#191299=CARTESIAN_POINT('',(108.175002385128,-4.8,63.1937156142209));
#191300=CARTESIAN_POINT('',(108.241431829638,-4.8,62.8519674541085));
#191301=CARTESIAN_POINT('',(107.798128234595,-4.8,62.5121464319025));
#191302=CARTESIAN_POINT('Origin',(116.959178380441,-4.8,51.0204257716897));
#191303=CARTESIAN_POINT('',(107.730462591627,-4.8,62.8602542500189));
#191304=CARTESIAN_POINT('',(107.798128234595,-4.8,62.5121464319025));
#191305=CARTESIAN_POINT('Origin',(116.959178380441,-4.8,51.0204257716897));
#191306=CARTESIAN_POINT('Origin',(108.340114255602,-4.8,62.344292916745));
#191307=CARTESIAN_POINT('',(108.208946481531,-4.3,63.0190892481863));
#191308=CARTESIAN_POINT('',(108.143336939225,-4.3,63.3566193981781));
#191309=CARTESIAN_POINT('',(108.208946481531,-4.3,63.0190892481863));
#191310=CARTESIAN_POINT('Origin',(110.774928248317,1.45439216225896E-14,
49.8183233204291));
#191311=CARTESIAN_POINT('Origin',(110.774928248317,1.45439216225896E-14,
49.8183233204291));
#191312=CARTESIAN_POINT('Origin',(108.340114255602,-4.3,62.344292916745));
#191313=CARTESIAN_POINT('',(107.765030138665,-4.3,62.6824205245265));
#191314=CARTESIAN_POINT('',(107.698230438928,-4.3,63.0260734731508));
#191315=CARTESIAN_POINT('',(107.765030138665,-4.3,62.6824205245265));
#191316=CARTESIAN_POINT('Origin',(116.959178380441,-4.3,51.0204257716897));
#191317=CARTESIAN_POINT('Origin',(116.959178380441,-4.3,51.0204257716897));
#191318=CARTESIAN_POINT('Origin',(107.849300753053,-4.3,62.2488879602958));
#191319=CARTESIAN_POINT('Origin',(110.284114745768,1.45439216225896E-14,
49.7229183639799));
#191320=CARTESIAN_POINT('Origin',(110.284114745768,1.45439216225896E-14,
49.7229183639799));
#191321=CARTESIAN_POINT('Origin',(107.849300753053,-3.8,62.2488879602958));
#191322=CARTESIAN_POINT('',(108.180373076411,-3.8,63.1660859406959));
#191323=CARTESIAN_POINT('',(108.115468353774,-3.8,63.4999901259154));
#191324=CARTESIAN_POINT('',(108.180373076411,-3.8,63.1660859406959));
#191325=CARTESIAN_POINT('',(107.735930810035,-3.8,62.832122845434));
#191326=CARTESIAN_POINT('Origin',(116.959178380441,-3.8,51.0204257716897));
#191327=CARTESIAN_POINT('',(107.669874557693,-3.8,63.1719511078611));
#191328=CARTESIAN_POINT('',(107.735930810035,-3.8,62.832122845434));
#191329=CARTESIAN_POINT('Origin',(116.959178380441,-3.8,51.0204257716897));
#191330=CARTESIAN_POINT('Origin',(108.340114255602,-3.8,62.344292916745));
#191331=CARTESIAN_POINT('',(108.155583589588,-3.3,63.2936161582717));
#191332=CARTESIAN_POINT('',(108.091278339735,-3.3,63.6244363387677));
#191333=CARTESIAN_POINT('',(108.155583589588,-3.3,63.2936161582717));
#191334=CARTESIAN_POINT('Origin',(110.774928248317,1.45439216225896E-14,
49.8183233204291));
#191335=CARTESIAN_POINT('Origin',(110.774928248317,1.45439216225896E-14,
49.8183233204291));
#191336=CARTESIAN_POINT('Origin',(108.340114255602,-3.3,62.344292916745));
#191337=CARTESIAN_POINT('',(107.710694595175,-3.3,62.9619512680616));
#191338=CARTESIAN_POINT('',(107.645269986769,-3.3,63.2985300203599));
#191339=CARTESIAN_POINT('',(107.710694595175,-3.3,62.9619512680616));
#191340=CARTESIAN_POINT('Origin',(116.959178380441,-3.3,51.0204257716897));
#191341=CARTESIAN_POINT('Origin',(116.959178380441,-3.3,51.0204257716897));
#191342=CARTESIAN_POINT('Origin',(107.849300753053,-3.3,62.2488879602958));
#191343=CARTESIAN_POINT('Origin',(110.284114745768,1.45439216225896E-14,
49.7229183639799));
#191344=CARTESIAN_POINT('Origin',(110.284114745768,1.45439216225896E-14,
49.7229183639799));
#191345=CARTESIAN_POINT('Origin',(107.849300753053,-2.8,62.2488879602958));
#191346=CARTESIAN_POINT('',(108.134471444857,-2.8,63.4022281852319));
#191347=CARTESIAN_POINT('',(108.070668179174,-2.8,63.7304658939327));
#191348=CARTESIAN_POINT('',(108.134471444857,-2.8,63.4022281852319));
#191349=CARTESIAN_POINT('',(107.68920878192,-2.8,63.0724856433291));
#191350=CARTESIAN_POINT('Origin',(116.959178380441,-2.8,51.0204257716897));
#191351=CARTESIAN_POINT('',(107.624312619326,-2.8,63.4063457911709));
#191352=CARTESIAN_POINT('',(107.68920878192,-2.8,63.0724856433291));
#191353=CARTESIAN_POINT('Origin',(116.959178380441,-2.8,51.0204257716897));
#191354=CARTESIAN_POINT('Origin',(108.340114255602,-2.8,62.344292916745));
#191355=CARTESIAN_POINT('',(108.116949014155,-2.3,63.4923728266226));
#191356=CARTESIAN_POINT('',(108.053556535402,-2.3,63.8184972303196));
#191357=CARTESIAN_POINT('',(108.116949014155,-2.3,63.4923728266226));
#191358=CARTESIAN_POINT('Origin',(110.774928248317,1.45439216225896E-14,
49.8183233204291));
#191359=CARTESIAN_POINT('Origin',(110.774928248317,1.45439216225896E-14,
49.8183233204291));
#191360=CARTESIAN_POINT('Origin',(108.340114255602,-2.3,62.344292916745));
#191361=CARTESIAN_POINT('',(107.671380844371,-2.3,63.1642019733521));
#191362=CARTESIAN_POINT('',(107.606916801999,-2.3,63.4958390664627));
#191363=CARTESIAN_POINT('',(107.671380844371,-2.3,63.1642019733521));
#191364=CARTESIAN_POINT('Origin',(116.959178380441,-2.3,51.0204257716897));
#191365=CARTESIAN_POINT('Origin',(116.959178380441,-2.3,51.0204257716897));
#191366=CARTESIAN_POINT('Origin',(107.849300753053,-2.3,62.2488879602958));
#191367=CARTESIAN_POINT('Origin',(110.284114745768,1.45439216225896E-14,
49.7229183639799));
#191368=CARTESIAN_POINT('Origin',(110.284114745768,1.45439216225896E-14,
49.7229183639799));
#191369=CARTESIAN_POINT('Origin',(107.849300753053,-1.8,62.2488879602958));
#191370=CARTESIAN_POINT('',(108.102945674253,-1.8,63.5644134056468));
#191371=CARTESIAN_POINT('',(108.039877742986,-1.8,63.8888681656054));
#191372=CARTESIAN_POINT('',(108.102945674253,-1.8,63.5644134056468));
#191373=CARTESIAN_POINT('',(107.657136309168,-1.8,63.2374833884464));
#191374=CARTESIAN_POINT('Origin',(116.959178380441,-1.8,51.0204257716897));
#191375=CARTESIAN_POINT('',(107.593013466184,-1.8,63.5673651716323));
#191376=CARTESIAN_POINT('',(107.657136309168,-1.8,63.2374833884464));
#191377=CARTESIAN_POINT('Origin',(116.959178380441,-1.8,51.0204257716897));
#191378=CARTESIAN_POINT('Origin',(108.340114255602,-1.8,62.344292916745));
#191379=CARTESIAN_POINT('',(108.092406313359,-1.3,63.6186334464865));
#191380=CARTESIAN_POINT('',(108.029580488533,-1.3,63.941842682998));
#191381=CARTESIAN_POINT('',(108.092406313359,-1.3,63.6186334464865));
#191382=CARTESIAN_POINT('Origin',(110.774928248317,1.45439216225896E-14,
49.8183233204291));
#191383=CARTESIAN_POINT('Origin',(110.774928248317,1.45439216225896E-14,
49.8183233204291));
#191384=CARTESIAN_POINT('Origin',(108.340114255602,-1.3,62.344292916745));
#191385=CARTESIAN_POINT('',(107.646417120603,-1.3,63.292628557836));
#191386=CARTESIAN_POINT('',(107.582548690235,-1.3,63.6212015081105));
#191387=CARTESIAN_POINT('',(107.646417120603,-1.3,63.292628557836));
#191388=CARTESIAN_POINT('Origin',(116.959178380441,-1.3,51.0204257716897));
#191389=CARTESIAN_POINT('Origin',(116.959178380441,-1.3,51.0204257716897));
#191390=CARTESIAN_POINT('Origin',(107.849300753053,-1.3,62.2488879602958));
#191391=CARTESIAN_POINT('Origin',(110.284114745768,1.45439216225896E-14,
49.7229183639799));
#191392=CARTESIAN_POINT('Origin',(110.284114745768,1.45439216225896E-14,
49.7229183639799));
#191393=CARTESIAN_POINT('Origin',(107.849300753053,-0.799999999999986,62.2488879602958));
#191394=CARTESIAN_POINT('',(108.085290210302,-0.799999999999986,63.6552424403597));
#191395=CARTESIAN_POINT('',(108.022626817486,-0.799999999999986,63.9776160407915));
#191396=CARTESIAN_POINT('',(108.085290210302,-0.799999999999986,63.6552424403597));
#191397=CARTESIAN_POINT('',(107.639180416563,-0.799999999999986,63.3298579868786));
#191398=CARTESIAN_POINT('Origin',(116.959178380441,-0.799999999999986,51.0204257716897));
#191399=CARTESIAN_POINT('',(107.575482619322,-0.799999999999986,63.657553110195));
#191400=CARTESIAN_POINT('',(107.639180416563,-0.799999999999986,63.3298579868786));
#191401=CARTESIAN_POINT('Origin',(116.959178380441,-0.799999999999986,51.0204257716897));
#191402=CARTESIAN_POINT('Origin',(108.340114255602,-0.799999999999986,62.344292916745));
#191403=CARTESIAN_POINT('',(108.081570231249,-0.299999999999985,63.6743799780327));
#191404=CARTESIAN_POINT('',(108.018991420535,-0.299999999999985,63.9963184434445));
#191405=CARTESIAN_POINT('',(108.081570231249,-0.299999999999985,63.6743799780327));
#191406=CARTESIAN_POINT('Origin',(110.774928248317,1.45439216225896E-14,
49.8183233204291));
#191407=CARTESIAN_POINT('Origin',(110.774928248317,1.45439216225896E-14,
49.8183233204291));
#191408=CARTESIAN_POINT('Origin',(108.340114255602,-0.299999999999985,62.344292916745));
#191409=CARTESIAN_POINT('',(107.635397652839,-0.299999999999985,63.3493185220758));
#191410=CARTESIAN_POINT('',(107.571788690702,-0.299999999999985,63.6765566306816));
#191411=CARTESIAN_POINT('',(107.635397652839,-0.299999999999985,63.3493185220758));
#191412=CARTESIAN_POINT('Origin',(116.959178380441,-0.299999999999985,51.0204257716897));
#191413=CARTESIAN_POINT('Origin',(116.959178380441,-0.299999999999985,51.0204257716897));
#191414=CARTESIAN_POINT('Origin',(107.849300753053,-0.299999999999985,62.2488879602958));
#191415=CARTESIAN_POINT('Origin',(110.284114745768,1.45439216225896E-14,
49.7229183639799));
#191416=CARTESIAN_POINT('Origin',(110.284114745768,1.45439216225896E-14,
49.7229183639799));
#191417=CARTESIAN_POINT('Origin',(121.592078824439,-0.799999999999986,64.9202267408748));
#191418=CARTESIAN_POINT('',(121.964170009511,-0.799999999999986,65.6264020245753));
#191419=CARTESIAN_POINT('',(121.898248727359,-0.799999999999986,65.9655359290372));
#191420=CARTESIAN_POINT('',(121.964170009511,-0.799999999999986,65.6264020245753));
#191421=CARTESIAN_POINT('',(121.42078644216,-0.799999999999986,65.8014452565064));
#191422=CARTESIAN_POINT('Origin',(116.959178380441,-0.799999999999986,51.0204257716897));
#191423=CARTESIAN_POINT('',(121.356162424845,-0.799999999999986,66.1339053452465));
#191424=CARTESIAN_POINT('',(121.42078644216,-0.799999999999986,65.8014452565064));
#191425=CARTESIAN_POINT('Origin',(116.959178380441,-0.799999999999986,51.0204257716897));
#191426=CARTESIAN_POINT('Origin',(122.082892326988,-0.799999999999986,65.0156316973241));
#191427=CARTESIAN_POINT('',(121.960252054219,-0.299999999999985,65.6465580566214));
#191428=CARTESIAN_POINT('',(121.894429225941,-0.299999999999985,65.9851854623394));
#191429=CARTESIAN_POINT('',(121.960252054219,-0.299999999999985,65.6465580566214));
#191430=CARTESIAN_POINT('Origin',(124.517706319704,1.45439216225896E-14,
52.4896621010082));
#191431=CARTESIAN_POINT('Origin',(124.517706319704,1.45439216225896E-14,
52.4896621010082));
#191432=CARTESIAN_POINT('Origin',(122.082892326988,-0.299999999999985,65.0156316973241));
#191433=CARTESIAN_POINT('',(121.416947401949,-0.299999999999985,65.8211953076876));
#191434=CARTESIAN_POINT('',(121.352416146668,-0.299999999999985,66.1531781795096));
#191435=CARTESIAN_POINT('',(121.416947401949,-0.299999999999985,65.8211953076876));
#191436=CARTESIAN_POINT('Origin',(116.959178380441,-0.299999999999985,51.0204257716897));
#191437=CARTESIAN_POINT('Origin',(116.959178380441,-0.299999999999985,51.0204257716897));
#191438=CARTESIAN_POINT('Origin',(121.592078824439,-0.299999999999985,64.9202267408748));
#191439=CARTESIAN_POINT('Origin',(124.026892817154,1.45439216225896E-14,
52.3942571445589));
#191440=CARTESIAN_POINT('Origin',(124.026892817154,1.45439216225896E-14,
52.3942571445589));
#191441=CARTESIAN_POINT('Origin',(121.592078824439,-1.8,64.9202267408748));
#191442=CARTESIAN_POINT('',(121.9827732263,-1.8,65.5306972485281));
#191443=CARTESIAN_POINT('',(121.916380469554,-1.8,65.8722566673977));
#191444=CARTESIAN_POINT('',(121.9827732263,-1.8,65.5306972485281));
#191445=CARTESIAN_POINT('',(121.439011726697,-1.8,65.7076847636441));
#191446=CARTESIAN_POINT('Origin',(116.959178380441,-1.8,51.0204257716897));
#191447=CARTESIAN_POINT('',(121.373943716819,-1.8,66.0424289847036));
#191448=CARTESIAN_POINT('',(121.439011726697,-1.8,65.7076847636441));
#191449=CARTESIAN_POINT('Origin',(116.959178380441,-1.8,51.0204257716897));
#191450=CARTESIAN_POINT('Origin',(122.082892326988,-1.8,65.0156316973241));
#191451=CARTESIAN_POINT('',(121.971666484299,-1.3,65.5878361975535));
#191452=CARTESIAN_POINT('',(121.905556011225,-1.3,65.9279434000723));
#191453=CARTESIAN_POINT('',(121.971666484299,-1.3,65.5878361975535));
#191454=CARTESIAN_POINT('Origin',(124.517706319704,1.45439216225896E-14,
52.4896621010082));
#191455=CARTESIAN_POINT('Origin',(124.517706319704,1.45439216225896E-14,
52.4896621010082));
#191456=CARTESIAN_POINT('Origin',(122.082892326988,-1.3,65.0156316973241));
#191457=CARTESIAN_POINT('',(121.42813126715,-1.3,65.7636595961683));
#191458=CARTESIAN_POINT('',(121.363329041984,-1.3,66.09703648025));
#191459=CARTESIAN_POINT('',(121.42813126715,-1.3,65.7636595961683));
#191460=CARTESIAN_POINT('Origin',(116.959178380441,-1.3,51.0204257716897));
#191461=CARTESIAN_POINT('Origin',(116.959178380441,-1.3,51.0204257716897));
#191462=CARTESIAN_POINT('Origin',(121.592078824439,-1.3,64.9202267408748));
#191463=CARTESIAN_POINT('Origin',(124.026892817154,1.45439216225896E-14,
52.3942571445589));
#191464=CARTESIAN_POINT('Origin',(124.026892817154,1.45439216225896E-14,
52.3942571445589));
#191465=CARTESIAN_POINT('Origin',(121.592078824439,-2.8,64.9202267408748));
#191466=CARTESIAN_POINT('',(122.016025476175,-2.8,65.3596301065635));
#191467=CARTESIAN_POINT('',(121.948773188325,-2.8,65.7056114075657));
#191468=CARTESIAN_POINT('',(122.016025476175,-2.8,65.3596301065635));
#191469=CARTESIAN_POINT('',(121.471574873494,-2.8,65.540162731995));
#191470=CARTESIAN_POINT('Origin',(116.959178380441,-2.8,51.0204257716897));
#191471=CARTESIAN_POINT('',(121.405698397847,-2.8,65.8790661281236));
#191472=CARTESIAN_POINT('',(121.471574873494,-2.8,65.540162731995));
#191473=CARTESIAN_POINT('Origin',(116.959178380441,-2.8,51.0204257716897));
#191474=CARTESIAN_POINT('Origin',(122.082892326988,-2.8,65.0156316973241));
#191475=CARTESIAN_POINT('',(121.99753796795,-2.3,65.4547396166228));
#191476=CARTESIAN_POINT('',(121.930766252407,-2.3,65.7982485997717));
#191477=CARTESIAN_POINT('',(121.99753796795,-2.3,65.4547396166228));
#191478=CARTESIAN_POINT('Origin',(124.517706319704,1.45439216225896E-14,
52.4896621010082));
#191479=CARTESIAN_POINT('Origin',(124.517706319704,1.45439216225896E-14,
52.4896621010082));
#191480=CARTESIAN_POINT('Origin',(122.082892326988,-2.3,65.0156316973241));
#191481=CARTESIAN_POINT('',(121.453472666561,-2.3,65.6332900486406));
#191482=CARTESIAN_POINT('',(121.388048058155,-2.3,65.969868800939));
#191483=CARTESIAN_POINT('',(121.453472666561,-2.3,65.6332900486406));
#191484=CARTESIAN_POINT('Origin',(116.959178380441,-2.3,51.0204257716897));
#191485=CARTESIAN_POINT('Origin',(116.959178380441,-2.3,51.0204257716897));
#191486=CARTESIAN_POINT('Origin',(121.592078824439,-2.3,64.9202267408748));
#191487=CARTESIAN_POINT('Origin',(124.026892817154,1.45439216225896E-14,
52.3942571445589));
#191488=CARTESIAN_POINT('Origin',(124.026892817154,1.45439216225896E-14,
52.3942571445589));
#191489=CARTESIAN_POINT('Origin',(121.592078824439,-3.8,64.9202267408748));
#191490=CARTESIAN_POINT('',(122.064522377965,-3.8,65.1101364207424));
#191491=CARTESIAN_POINT('',(121.995976389156,-3.8,65.4627732029904));
#191492=CARTESIAN_POINT('',(122.064522377965,-3.8,65.1101364207424));
#191493=CARTESIAN_POINT('',(121.519034327862,-3.8,65.2960062238397));
#191494=CARTESIAN_POINT('Origin',(116.959178380441,-3.8,51.0204257716897));
#191495=CARTESIAN_POINT('',(121.451943382131,-3.8,65.641157495737));
#191496=CARTESIAN_POINT('',(121.519034327862,-3.8,65.2960062238397));
#191497=CARTESIAN_POINT('Origin',(116.959178380441,-3.8,51.0204257716897));
#191498=CARTESIAN_POINT('Origin',(122.082892326988,-3.8,65.0156316973241));
#191499=CARTESIAN_POINT('',(122.038319025802,-3.3,65.2449403086335));
#191500=CARTESIAN_POINT('',(121.970478072417,-3.3,65.5939500161639));
#191501=CARTESIAN_POINT('',(122.038319025802,-3.3,65.2449403086335));
#191502=CARTESIAN_POINT('Origin',(124.517706319704,1.45439216225896E-14,
52.4896621010082));
#191503=CARTESIAN_POINT('Origin',(124.517706319704,1.45439216225896E-14,
52.4896621010082));
#191504=CARTESIAN_POINT('Origin',(122.082892326988,-3.3,65.0156316973241));
#191505=CARTESIAN_POINT('',(121.493396398475,-3.3,65.4279012782383));
#191506=CARTESIAN_POINT('',(121.426966953965,-3.3,65.7696494383507));
#191507=CARTESIAN_POINT('',(121.493396398475,-3.3,65.4279012782383));
#191508=CARTESIAN_POINT('Origin',(116.959178380441,-3.3,51.0204257716897));
#191509=CARTESIAN_POINT('Origin',(116.959178380441,-3.3,51.0204257716897));
#191510=CARTESIAN_POINT('Origin',(121.592078824439,-3.3,64.9202267408748));
#191511=CARTESIAN_POINT('Origin',(124.026892817154,1.45439216225896E-14,
52.3942571445589));
#191512=CARTESIAN_POINT('Origin',(124.026892817154,1.45439216225896E-14,
52.3942571445589));
#191513=CARTESIAN_POINT('Origin',(121.592078824439,-4.3,64.9202267408748));
#191514=CARTESIAN_POINT('',(121.582257513942,-4.8,64.9707527510925));
#191515=CARTESIAN_POINT('',(121.513478375339,-4.8,65.3245889790688));
#191516=CARTESIAN_POINT('',(121.582257513942,-4.8,64.9707527510925));
#191517=CARTESIAN_POINT('',(121.548607101235,-4.3,65.1438682530293));
#191518=CARTESIAN_POINT('Origin',(124.026892817154,1.45439216225896E-14,
52.3942571445589));
#191519=CARTESIAN_POINT('',(121.480736796731,-4.3,65.4930289582246));
#191520=CARTESIAN_POINT('',(121.548607101235,-4.3,65.1438682530293));
#191521=CARTESIAN_POINT('Origin',(124.026892817154,1.45439216225896E-14,
52.3942571445589));
#191522=CARTESIAN_POINT('Origin',(121.592078824439,-4.8,64.9202267408748));
#191523=CARTESIAN_POINT('',(122.082892326988,-4.8,65.0156316973241));
#191524=CARTESIAN_POINT('',(122.058842881848,-4.8,65.1393547494882));
#191525=CARTESIAN_POINT('',(122.082892326988,-4.8,65.0156316973241));
#191526=CARTESIAN_POINT('',(121.681243230653,-4.8,64.9375586322092));
#191527=CARTESIAN_POINT('',(121.681243230653,-4.8,64.9375586322092));
#191528=CARTESIAN_POINT('Origin',(116.959178380441,-4.8,51.0204257716897));
#191529=CARTESIAN_POINT('Origin',(116.959178380441,-4.8,51.0204257716897));
#191530=CARTESIAN_POINT('Origin',(122.082892326988,-4.8,65.0156316973241));
#191531=CARTESIAN_POINT('',(122.082892326988,-4.3,65.0156316973241));
#191532=CARTESIAN_POINT('',(122.025384564787,-4.3,65.3114820099324));
#191533=CARTESIAN_POINT('',(122.082892326988,-4.3,65.0156316973241));
#191534=CARTESIAN_POINT('',(122.082892326988,-4.8,65.0156316973241));
#191535=CARTESIAN_POINT('Origin',(124.517706319704,1.45439216225896E-14,
52.4896621010082));
#191536=CARTESIAN_POINT('Origin',(122.082892326988,-4.3,65.0156316973241));
#191537=CARTESIAN_POINT('',(121.98125760463,-4.3,64.9958758099861));
#191538=CARTESIAN_POINT('Origin',(116.959178380441,-4.3,51.0204257716897));
#191539=CARTESIAN_POINT('',(122.082892326988,-4.3,65.0156316973241));
#191540=CARTESIAN_POINT('Origin',(116.959178380441,-4.3,51.0204257716897));
#191541=CARTESIAN_POINT('Origin',(121.395753423419,-5.,64.8820647582951));
#191542=CARTESIAN_POINT('Origin',(114.524364387726,1.45439216225896E-14,
63.5463953680056));
#191543=CARTESIAN_POINT('Origin',(121.101265321889,-5.3,64.8248217844256));
#191544=CARTESIAN_POINT('',(120.539222696584,-5.3,65.0958570688648));
#191545=CARTESIAN_POINT('',(120.472084417903,-5.3,65.4412518464652));
#191546=CARTESIAN_POINT('',(120.539222696584,-5.3,65.0958570688648));
#191547=CARTESIAN_POINT('',(121.077336186674,-5.3,64.9479258987745));
#191548=CARTESIAN_POINT('Origin',(116.959178380441,-5.3,51.0204257716897));
#191549=CARTESIAN_POINT('',(121.008940980487,-5.3,65.2997869755489));
#191550=CARTESIAN_POINT('',(121.077336186674,-5.3,64.9479258987745));
#191551=CARTESIAN_POINT('Origin',(116.959178380441,-5.3,51.0204257716897));
#191552=CARTESIAN_POINT('Origin',(120.61045181934,-5.3,64.7294168279763));
#191553=CARTESIAN_POINT('',(120.579868207262,-5.8,64.8867550871532));
#191554=CARTESIAN_POINT('',(120.511652633147,-5.8,65.2376920416435));
#191555=CARTESIAN_POINT('',(120.579868207262,-5.8,64.8867550871532));
#191556=CARTESIAN_POINT('Origin',(123.045265812055,1.45439216225896E-14,
52.2034472316604));
#191557=CARTESIAN_POINT('Origin',(123.045265812055,1.45439216225896E-14,
52.2034472316604));
#191558=CARTESIAN_POINT('Origin',(120.61045181934,-5.8,64.7294168279763));
#191559=CARTESIAN_POINT('',(121.101265321889,-5.8,64.8248217844256));
#191560=CARTESIAN_POINT('',(121.049241681607,-5.8,65.0924588763805));
#191561=CARTESIAN_POINT('',(121.101265321889,-5.8,64.8248217844256));
#191562=CARTESIAN_POINT('',(120.928023033738,-5.8,64.791146726852));
#191563=CARTESIAN_POINT('',(120.928023033738,-5.8,64.791146726852));
#191564=CARTESIAN_POINT('Origin',(116.959178380441,-5.8,51.0204257716897));
#191565=CARTESIAN_POINT('Origin',(116.959178380441,-5.8,51.0204257716897));
#191566=CARTESIAN_POINT('Origin',(121.101265321889,-5.8,64.8248217844256));
#191567=CARTESIAN_POINT('',(121.101265321889,-5.59519883471499,64.8248217844256));
#191568=CARTESIAN_POINT('Origin',(123.536079314605,1.45439216225896E-14,
52.2988521881097));
#191569=CARTESIAN_POINT('',(121.101265321889,-5.8,64.8248217844256));
#191570=CARTESIAN_POINT('Origin',(123.536079314605,1.45439216225896E-14,
52.2988521881097));
#191571=CARTESIAN_POINT('Origin',(120.41412641832,-6.,64.6912548453966));
#191572=CARTESIAN_POINT('Origin',(114.524364387726,1.45439216225896E-14,
63.5463953680056));
#191573=CARTESIAN_POINT('Origin',(119.628824814241,-5.8,64.5386069150778));
#191574=CARTESIAN_POINT('',(120.045505226416,-5.8,65.0153916561379));
#191575=CARTESIAN_POINT('',(119.978442632437,-5.8,65.3603970716418));
#191576=CARTESIAN_POINT('',(120.045505226416,-5.8,65.0153916561379));
#191577=CARTESIAN_POINT('',(119.515454871223,-5.8,65.121841800216));
#191578=CARTESIAN_POINT('Origin',(116.959178380441,-5.8,51.0204257716897));
#191579=CARTESIAN_POINT('',(119.449398618882,-5.8,65.4616700626431));
#191580=CARTESIAN_POINT('',(119.515454871223,-5.8,65.121841800216));
#191581=CARTESIAN_POINT('Origin',(116.959178380441,-5.8,51.0204257716897));
#191582=CARTESIAN_POINT('Origin',(120.11963831679,-5.8,64.6340118715271));
#191583=CARTESIAN_POINT('',(120.005554074461,-5.3,65.2209214897176));
#191584=CARTESIAN_POINT('',(119.939515866065,-5.3,65.5606569245574));
#191585=CARTESIAN_POINT('',(120.005554074461,-5.3,65.2209214897176));
#191586=CARTESIAN_POINT('Origin',(122.554452309506,1.45439216225896E-14,
52.1080422752111));
#191587=CARTESIAN_POINT('Origin',(122.554452309506,1.45439216225896E-14,
52.1080422752111));
#191588=CARTESIAN_POINT('Origin',(120.11963831679,-5.3,64.6340118715271));
#191589=CARTESIAN_POINT('',(119.476109460802,-5.3,65.3242553793072));
#191590=CARTESIAN_POINT('',(119.41103282268,-5.3,65.6590439886171));
#191591=CARTESIAN_POINT('',(119.476109460802,-5.3,65.3242553793072));
#191592=CARTESIAN_POINT('Origin',(116.959178380441,-5.3,51.0204257716897));
#191593=CARTESIAN_POINT('Origin',(116.959178380441,-5.3,51.0204257716897));
#191594=CARTESIAN_POINT('Origin',(119.628824814241,-5.3,64.5386069150778));
#191595=CARTESIAN_POINT('Origin',(122.063638806956,1.45439216225896E-14,
52.0126373187619));
#191596=CARTESIAN_POINT('Origin',(122.063638806956,1.45439216225896E-14,
52.0126373187619));
#191597=CARTESIAN_POINT('Origin',(118.647197809142,-5.8,64.3477970021793));
#191598=CARTESIAN_POINT('',(118.989520625611,-5.8,65.2071165018896));
#191599=CARTESIAN_POINT('',(118.924340180018,-5.8,65.5424391516779));
#191600=CARTESIAN_POINT('',(118.989520625611,-5.8,65.2071165018896));
#191601=CARTESIAN_POINT('',(118.467536606867,-5.8,65.2720691494816));
#191602=CARTESIAN_POINT('Origin',(116.959178380441,-5.8,51.0204257716897));
#191603=CARTESIAN_POINT('',(118.403114466043,-5.8,65.6034906788921));
#191604=CARTESIAN_POINT('',(118.467536606867,-5.8,65.2720691494816));
#191605=CARTESIAN_POINT('Origin',(116.959178380441,-5.8,51.0204257716897));
#191606=CARTESIAN_POINT('Origin',(119.138011311691,-5.8,64.4432019586286));
#191607=CARTESIAN_POINT('',(118.950702155056,-5.3,65.4068192239074));
#191608=CARTESIAN_POINT('',(118.886463414977,-5.3,65.7372972429876));
#191609=CARTESIAN_POINT('',(118.950702155056,-5.3,65.4068192239074));
#191610=CARTESIAN_POINT('Origin',(121.572825304407,1.45439216225896E-14,
51.9172323623126));
#191611=CARTESIAN_POINT('Origin',(121.572825304407,1.45439216225896E-14,
51.9172323623126));
#191612=CARTESIAN_POINT('Origin',(119.138011311691,-5.3,64.4432019586286));
#191613=CARTESIAN_POINT('',(118.429174209374,-5.3,65.4694255907055));
#191614=CARTESIAN_POINT('',(118.365661735554,-5.3,65.7961673124252));
#191615=CARTESIAN_POINT('',(118.429174209374,-5.3,65.4694255907055));
#191616=CARTESIAN_POINT('Origin',(116.959178380441,-5.3,51.0204257716897));
#191617=CARTESIAN_POINT('Origin',(116.959178380441,-5.3,51.0204257716897));
#191618=CARTESIAN_POINT('Origin',(118.647197809142,-5.3,64.3477970021793));
#191619=CARTESIAN_POINT('Origin',(121.082011801857,1.45439216225896E-14,
51.8218274058634));
#191620=CARTESIAN_POINT('Origin',(121.082011801857,1.45439216225896E-14,
51.8218274058634));
#191621=CARTESIAN_POINT('Origin',(117.665570804043,-5.8,64.1569870892808));
#191622=CARTESIAN_POINT('',(117.949362987349,-5.8,65.3174190902556));
#191623=CARTESIAN_POINT('',(117.885592229287,-5.8,65.6454895625796));
#191624=CARTESIAN_POINT('',(117.949362987349,-5.8,65.3174190902556));
#191625=CARTESIAN_POINT('',(117.434882428651,-5.8,65.3437699749629));
#191626=CARTESIAN_POINT('Origin',(116.959178380441,-5.8,51.0204257716897));
#191627=CARTESIAN_POINT('',(117.371664718591,-5.8,65.6689952761733));
#191628=CARTESIAN_POINT('',(117.434882428651,-5.8,65.3437699749629));
#191629=CARTESIAN_POINT('Origin',(116.959178380441,-5.8,51.0204257716897));
#191630=CARTESIAN_POINT('Origin',(118.156384306592,-5.8,64.25239204573));
#191631=CARTESIAN_POINT('',(117.911392231253,-5.3,65.5127607212116));
#191632=CARTESIAN_POINT('',(117.848504194417,-5.3,65.8362900091687));
#191633=CARTESIAN_POINT('',(117.911392231253,-5.3,65.5127607212116));
#191634=CARTESIAN_POINT('Origin',(120.591198299308,1.45439216225896E-14,
51.7264224494141));
#191635=CARTESIAN_POINT('Origin',(120.591198299308,1.45439216225896E-14,
51.7264224494141));
#191636=CARTESIAN_POINT('Origin',(118.156384306592,-5.3,64.25239204573));
#191637=CARTESIAN_POINT('',(117.397244100963,-5.3,65.5374014185508));
#191638=CARTESIAN_POINT('',(117.334886647803,-5.3,65.8582011037552));
#191639=CARTESIAN_POINT('',(117.397244100963,-5.3,65.5374014185508));
#191640=CARTESIAN_POINT('Origin',(116.959178380441,-5.3,51.0204257716897));
#191641=CARTESIAN_POINT('Origin',(116.959178380441,-5.3,51.0204257716897));
#191642=CARTESIAN_POINT('Origin',(117.665570804043,-5.3,64.1569870892808));
#191643=CARTESIAN_POINT('Origin',(120.100384796758,1.45439216225896E-14,
51.6310174929649));
#191644=CARTESIAN_POINT('Origin',(120.100384796758,1.45439216225896E-14,
51.6310174929649));
#191645=CARTESIAN_POINT('Origin',(116.683943798944,-5.8,63.9661771763823));
#191646=CARTESIAN_POINT('',(116.92399729191,-5.8,65.3516241095141));
#191647=CARTESIAN_POINT('',(116.861241235349,-5.8,65.6744744212084));
#191648=CARTESIAN_POINT('',(116.92399729191,-5.8,65.3516241095141));
#191649=CARTESIAN_POINT('',(116.416627454716,-5.8,65.3413936859011));
#191650=CARTESIAN_POINT('Origin',(116.959178380441,-5.8,51.0204257716897));
#191651=CARTESIAN_POINT('',(116.354247211386,-5.8,65.6623106157809));
#191652=CARTESIAN_POINT('',(116.416627454716,-5.8,65.3413936859011));
#191653=CARTESIAN_POINT('Origin',(116.959178380441,-5.8,51.0204257716897));
#191654=CARTESIAN_POINT('Origin',(117.174757301493,-5.8,64.0615821328315));
#191655=CARTESIAN_POINT('',(116.886636394382,-5.3,65.5438283057789));
#191656=CARTESIAN_POINT('',(116.82472213145,-5.3,65.8623479862876));
#191657=CARTESIAN_POINT('',(116.886636394382,-5.3,65.5438283057789));
#191658=CARTESIAN_POINT('Origin',(119.609571294209,1.45439216225896E-14,
51.5356125365156));
#191659=CARTESIAN_POINT('Origin',(119.609571294209,1.45439216225896E-14,
51.5356125365156));
#191660=CARTESIAN_POINT('Origin',(117.174757301493,-5.3,64.0615821328315));
#191661=CARTESIAN_POINT('',(116.379492360069,-5.3,65.5324362328468));
#191662=CARTESIAN_POINT('',(116.317939072905,-5.3,65.8490988632889));
#191663=CARTESIAN_POINT('',(116.379492360069,-5.3,65.5324362328468));
#191664=CARTESIAN_POINT('Origin',(116.959178380441,-5.3,51.0204257716897));
#191665=CARTESIAN_POINT('Origin',(116.959178380441,-5.3,51.0204257716897));
#191666=CARTESIAN_POINT('Origin',(116.683943798944,-5.3,63.9661771763823));
#191667=CARTESIAN_POINT('Origin',(119.118757791659,1.45439216225896E-14,
51.4402075800664));
#191668=CARTESIAN_POINT('Origin',(119.118757791659,1.45439216225896E-14,
51.4402075800664));
#191669=CARTESIAN_POINT('Origin',(115.702316793845,-5.8,63.7753672634838));
#191670=CARTESIAN_POINT('',(115.912708611971,-5.8,65.3134095235366));
#191671=CARTESIAN_POINT('',(115.850622706538,-5.8,65.6328122237612));
#191672=CARTESIAN_POINT('',(115.912708611971,-5.8,65.3134095235366));
#191673=CARTESIAN_POINT('',(115.412190971526,-5.8,65.2679277795385));
#191674=CARTESIAN_POINT('Origin',(116.959178380441,-5.8,51.0204257716897));
#191675=CARTESIAN_POINT('',(115.350321251236,-5.8,65.5862183091668));
#191676=CARTESIAN_POINT('',(115.412190971526,-5.8,65.2679277795385));
#191677=CARTESIAN_POINT('Origin',(116.959178380441,-5.8,51.0204257716897));
#191678=CARTESIAN_POINT('Origin',(116.193130296394,-5.8,63.870772219933));
#191679=CARTESIAN_POINT('',(115.875750340769,-5.3,65.503542397257));
#191680=CARTESIAN_POINT('',(115.814479890918,-5.3,65.8187499631281));
#191681=CARTESIAN_POINT('',(115.875750340769,-5.3,65.503542397257));
#191682=CARTESIAN_POINT('Origin',(118.62794428911,1.45439216225896E-14,
51.3448026236171));
#191683=CARTESIAN_POINT('Origin',(118.62794428911,1.45439216225896E-14,
51.3448026236171));
#191684=CARTESIAN_POINT('Origin',(116.193130296394,-5.3,63.870772219933));
#191685=CARTESIAN_POINT('',(115.37536255906,-5.3,65.4573925913142));
#191686=CARTESIAN_POINT('',(115.31429991436,-5.3,65.7715310976936));
#191687=CARTESIAN_POINT('',(115.37536255906,-5.3,65.4573925913142));
#191688=CARTESIAN_POINT('Origin',(116.959178380441,-5.3,51.0204257716897));
#191689=CARTESIAN_POINT('Origin',(116.959178380441,-5.3,51.0204257716897));
#191690=CARTESIAN_POINT('Origin',(115.702316793845,-5.3,63.7753672634838));
#191691=CARTESIAN_POINT('Origin',(118.13713078656,1.45439216225896E-14,
51.2493976671679));
#191692=CARTESIAN_POINT('Origin',(118.13713078656,1.45439216225896E-14,
51.2493976671679));
#191693=CARTESIAN_POINT('Origin',(114.720689788746,-5.8,63.5845573505853));
#191694=CARTESIAN_POINT('',(114.915038280088,-5.8,65.2051349600047));
#191695=CARTESIAN_POINT('',(114.853308979711,-5.8,65.522703095409));
#191696=CARTESIAN_POINT('',(114.915038280088,-5.8,65.2051349600047));
#191697=CARTESIAN_POINT('',(114.421227133504,-5.8,65.1251514682507));
#191698=CARTESIAN_POINT('Origin',(116.959178380441,-5.8,51.0204257716897));
#191699=CARTESIAN_POINT('',(114.359564014912,-5.8,65.4423791295872));
#191700=CARTESIAN_POINT('',(114.421227133504,-5.8,65.1251514682507));
#191701=CARTESIAN_POINT('Origin',(116.959178380441,-5.8,51.0204257716897));
#191702=CARTESIAN_POINT('Origin',(115.211503291295,-5.8,63.6799623070345));
#191703=CARTESIAN_POINT('',(114.878294208936,-5.3,65.3941658754951));
#191704=CARTESIAN_POINT('',(114.817366571332,-5.3,65.7076098340429));
#191705=CARTESIAN_POINT('',(114.878294208936,-5.3,65.3941658754951));
#191706=CARTESIAN_POINT('Origin',(117.64631728401,1.45439216225896E-14,
51.1539927107186));
#191707=CARTESIAN_POINT('Origin',(117.64631728401,1.45439216225896E-14,
51.1539927107186));
#191708=CARTESIAN_POINT('Origin',(115.211503291295,-5.3,63.6799623070345));
#191709=CARTESIAN_POINT('',(114.384522811763,-5.3,65.3139778917727));
#191710=CARTESIAN_POINT('',(114.323658813062,-5.3,65.6270944581799));
#191711=CARTESIAN_POINT('',(114.384522811763,-5.3,65.3139778917727));
#191712=CARTESIAN_POINT('Origin',(116.959178380441,-5.3,51.0204257716897));
#191713=CARTESIAN_POINT('Origin',(116.959178380441,-5.3,51.0204257716897));
#191714=CARTESIAN_POINT('Origin',(114.720689788746,-5.3,63.5845573505853));
#191715=CARTESIAN_POINT('Origin',(117.155503781461,1.45439216225896E-14,
51.0585877542694));
#191716=CARTESIAN_POINT('Origin',(117.155503781461,1.45439216225896E-14,
51.0585877542694));
#191717=CARTESIAN_POINT('Origin',(113.739062783647,-5.8,63.3937474376868));
#191718=CARTESIAN_POINT('',(113.930746540204,-5.8,65.0280338507332));
#191719=CARTESIAN_POINT('',(113.869076078592,-5.8,65.3452992884439));
#191720=CARTESIAN_POINT('',(113.930746540204,-5.8,65.0280338507332));
#191721=CARTESIAN_POINT('',(113.443597718493,-5.8,64.9137758398423));
#191722=CARTESIAN_POINT('Origin',(116.959178380441,-5.8,51.0204257716897));
#191723=CARTESIAN_POINT('',(113.381846310114,-5.8,65.2314577104878));
#191724=CARTESIAN_POINT('',(113.443597718493,-5.8,64.9137758398423));
#191725=CARTESIAN_POINT('Origin',(116.959178380441,-5.8,51.0204257716897));
#191726=CARTESIAN_POINT('Origin',(114.229876286196,-5.8,63.489152394136));
#191727=CARTESIAN_POINT('',(113.894037808231,-5.3,65.2168829628162));
#191728=CARTESIAN_POINT('',(113.833166748388,-5.3,65.5300358554694));
#191729=CARTESIAN_POINT('',(113.894037808231,-5.3,65.2168829628162));
#191730=CARTESIAN_POINT('Origin',(116.664690278911,1.45439216225896E-14,
50.9631827978201));
#191731=CARTESIAN_POINT('Origin',(116.664690278911,1.45439216225896E-14,
50.9631827978201));
#191732=CARTESIAN_POINT('Origin',(114.229876286196,-5.3,63.489152394136));
#191733=CARTESIAN_POINT('',(113.40684036881,-5.3,65.1028750671095));
#191734=CARTESIAN_POINT('',(113.345891473831,-5.3,65.4164283848248));
#191735=CARTESIAN_POINT('',(113.40684036881,-5.3,65.1028750671095));
#191736=CARTESIAN_POINT('Origin',(116.959178380441,-5.3,51.0204257716897));
#191737=CARTESIAN_POINT('Origin',(116.959178380441,-5.3,51.0204257716897));
#191738=CARTESIAN_POINT('Origin',(113.739062783647,-5.3,63.3937474376868));
#191739=CARTESIAN_POINT('Origin',(116.173876776362,1.45439216225896E-14,
50.8677778413709));
#191740=CARTESIAN_POINT('Origin',(116.173876776362,1.45439216225896E-14,
50.8677778413709));
#191741=CARTESIAN_POINT('Origin',(112.757435778548,-5.8,63.2029375247883));
#191742=CARTESIAN_POINT('',(112.959794118948,-5.8,64.7823082386979));
#191743=CARTESIAN_POINT('',(112.897887286472,-5.8,65.1007896930215));
#191744=CARTESIAN_POINT('',(112.959794118948,-5.8,64.7823082386979));
#191745=CARTESIAN_POINT('',(112.479361672869,-5.8,64.633497643002));
#191746=CARTESIAN_POINT('Origin',(116.959178380441,-5.8,51.0204257716897));
#191747=CARTESIAN_POINT('',(112.417223244359,-5.8,64.9531705496847));
#191748=CARTESIAN_POINT('',(112.479361672869,-5.8,64.633497643002));
#191749=CARTESIAN_POINT('Origin',(116.959178380441,-5.8,51.0204257716897));
#191750=CARTESIAN_POINT('Origin',(113.248249281097,-5.8,63.2983424812375));
#191751=CARTESIAN_POINT('',(112.922943414692,-5.3,64.9718877312178));
#191752=CARTESIAN_POINT('',(112.861845092366,-5.3,65.2862097821557));
#191753=CARTESIAN_POINT('',(112.922943414692,-5.3,64.9718877312178));
#191754=CARTESIAN_POINT('Origin',(115.683063273812,1.45439216225896E-14,
50.7723728849216));
#191755=CARTESIAN_POINT('Origin',(115.683063273812,1.45439216225896E-14,
50.7723728849216));
#191756=CARTESIAN_POINT('Origin',(113.248249281097,-5.3,63.2983424812375));
#191757=CARTESIAN_POINT('',(112.442371850103,-5.3,64.8237928346375));
#191758=CARTESIAN_POINT('',(112.38105092168,-5.3,65.1392600889511));
#191759=CARTESIAN_POINT('',(112.442371850103,-5.3,64.8237928346375));
#191760=CARTESIAN_POINT('Origin',(116.959178380441,-5.3,51.0204257716897));
#191761=CARTESIAN_POINT('Origin',(116.959178380441,-5.3,51.0204257716897));
#191762=CARTESIAN_POINT('Origin',(112.757435778548,-5.3,63.2029375247883));
#191763=CARTESIAN_POINT('Origin',(115.192249771263,1.45439216225896E-14,
50.6769679284724));
#191764=CARTESIAN_POINT('Origin',(115.192249771263,1.45439216225896E-14,
50.6769679284724));
#191765=CARTESIAN_POINT('Origin',(111.775808773449,-5.8,63.0121276118898));
#191766=CARTESIAN_POINT('',(112.002339277582,-5.8,64.4671439443595));
#191767=CARTESIAN_POINT('',(111.939890513497,-5.8,64.7884133811989));
#191768=CARTESIAN_POINT('',(112.002339277582,-5.8,64.4671439443595));
#191769=CARTESIAN_POINT('',(111.528779540089,-5.8,64.2829765045437));
#191770=CARTESIAN_POINT('Origin',(116.959178380441,-5.8,51.0204257716897));
#191771=CARTESIAN_POINT('',(111.465938179574,-5.8,64.6062656648512));
#191772=CARTESIAN_POINT('',(111.528779540089,-5.8,64.2829765045437));
#191773=CARTESIAN_POINT('Origin',(116.959178380441,-5.8,51.0204257716897));
#191774=CARTESIAN_POINT('Origin',(112.266622275998,-5.8,63.107532568339));
#191775=CARTESIAN_POINT('',(111.965163015835,-5.3,64.6583982766151));
#191776=CARTESIAN_POINT('',(111.903543900335,-5.3,64.9753995627983));
#191777=CARTESIAN_POINT('',(111.965163015835,-5.3,64.6583982766151));
#191778=CARTESIAN_POINT('Origin',(114.701436268713,1.45439216225896E-14,
50.5815629720231));
#191779=CARTESIAN_POINT('Origin',(114.701436268713,1.45439216225896E-14,
50.5815629720231));
#191780=CARTESIAN_POINT('Origin',(112.266622275998,-5.3,63.107532568339));
#191781=CARTESIAN_POINT('',(111.491367383505,-5.3,64.4754444044786));
#191782=CARTESIAN_POINT('',(111.429371208549,-5.3,64.7943854837179));
#191783=CARTESIAN_POINT('',(111.491367383505,-5.3,64.4754444044786));
#191784=CARTESIAN_POINT('Origin',(116.959178380441,-5.3,51.0204257716897));
#191785=CARTESIAN_POINT('Origin',(116.959178380441,-5.3,51.0204257716897));
#191786=CARTESIAN_POINT('Origin',(111.775808773449,-5.3,63.0121276118898));
#191787=CARTESIAN_POINT('Origin',(114.210622766164,1.45439216225896E-14,
50.4861580155739));
#191788=CARTESIAN_POINT('Origin',(114.210622766164,1.45439216225896E-14,
50.4861580155739));
#191789=CARTESIAN_POINT('Origin',(110.79418176835,-5.8,62.8213176989913));
#191790=CARTESIAN_POINT('',(111.058749813035,-5.8,64.0806488259782));
#191791=CARTESIAN_POINT('',(110.995429005623,-5.8,64.4064045144342));
#191792=CARTESIAN_POINT('',(111.058749813035,-5.8,64.0806488259782));
#191793=CARTESIAN_POINT('',(110.592333572166,-5.8,63.8597314653125));
#191794=CARTESIAN_POINT('Origin',(116.959178380441,-5.8,51.0204257716897));
#191795=CARTESIAN_POINT('',(110.528440653502,-5.8,64.1884303963207));
#191796=CARTESIAN_POINT('',(110.592333572166,-5.8,63.8597314653125));
#191797=CARTESIAN_POINT('Origin',(116.959178380441,-5.8,51.0204257716897));
#191798=CARTESIAN_POINT('Origin',(111.284995270899,-5.8,62.9167226554405));
#191799=CARTESIAN_POINT('',(111.021049521363,-5.3,64.2745990450339));
#191800=CARTESIAN_POINT('',(110.958593129912,-5.3,64.5959077210777));
#191801=CARTESIAN_POINT('',(111.021049521363,-5.3,64.2745990450339));
#191802=CARTESIAN_POINT('Origin',(113.719809263614,1.45439216225896E-14,
50.3907530591246));
#191803=CARTESIAN_POINT('Origin',(113.719809263614,1.45439216225896E-14,
50.3907530591246));
#191804=CARTESIAN_POINT('Origin',(111.284995270899,-5.3,62.9167226554405));
#191805=CARTESIAN_POINT('',(110.554289376198,-5.3,64.0554509097686));
#191806=CARTESIAN_POINT('',(110.491284191915,-5.3,64.3795828660941));
#191807=CARTESIAN_POINT('',(110.554289376198,-5.3,64.0554509097686));
#191808=CARTESIAN_POINT('Origin',(116.959178380441,-5.3,51.0204257716897));
#191809=CARTESIAN_POINT('Origin',(116.959178380441,-5.3,51.0204257716897));
#191810=CARTESIAN_POINT('Origin',(110.79418176835,-5.3,62.8213176989913));
#191811=CARTESIAN_POINT('Origin',(113.228995761065,1.45439216225896E-14,
50.2953481026754));
#191812=CARTESIAN_POINT('Origin',(113.228995761065,1.45439216225896E-14,
50.2953481026754));
#191813=CARTESIAN_POINT('Origin',(109.812554763251,-5.8,62.6305077860928));
#191814=CARTESIAN_POINT('',(110.129632204215,-5.8,63.6197028356265));
#191815=CARTESIAN_POINT('',(110.065067263532,-5.8,63.9518590029572));
#191816=CARTESIAN_POINT('',(110.129632204215,-5.8,63.6197028356265));
#191817=CARTESIAN_POINT('',(109.670767300217,-5.8,63.3599374084025));
#191818=CARTESIAN_POINT('Origin',(116.959178380441,-5.8,51.0204257716897));
#191819=CARTESIAN_POINT('',(109.605421471785,-5.8,63.6961108748868));
#191820=CARTESIAN_POINT('',(109.670767300217,-5.8,63.3599374084025));
#191821=CARTESIAN_POINT('Origin',(116.959178380441,-5.8,51.0204257716897));
#191822=CARTESIAN_POINT('Origin',(110.3033682658,-5.8,62.725912742542));
#191823=CARTESIAN_POINT('',(110.091183933495,-5.3,63.8175010540987));
#191824=CARTESIAN_POINT('',(110.027534637877,-5.3,64.1449466594431));
#191825=CARTESIAN_POINT('',(110.091183933495,-5.3,63.8175010540987));
#191826=CARTESIAN_POINT('Origin',(112.738182258515,1.45439216225896E-14,
50.1999431462261));
#191827=CARTESIAN_POINT('Origin',(112.738182258515,1.45439216225896E-14,
50.1999431462261));
#191828=CARTESIAN_POINT('Origin',(110.3033682658,-5.3,62.725912742542));
#191829=CARTESIAN_POINT('',(109.631849341272,-5.3,63.560151951261));
#191830=CARTESIAN_POINT('',(109.567452302182,-5.3,63.8914443440855));
#191831=CARTESIAN_POINT('',(109.631849341272,-5.3,63.560151951261));
#191832=CARTESIAN_POINT('Origin',(116.959178380441,-5.3,51.0204257716897));
#191833=CARTESIAN_POINT('Origin',(116.959178380441,-5.3,51.0204257716897));
#191834=CARTESIAN_POINT('Origin',(109.812554763251,-5.3,62.6305077860928));
#191835=CARTESIAN_POINT('Origin',(112.247368755966,1.45439216225896E-14,
50.1045381897769));
#191836=CARTESIAN_POINT('Origin',(112.247368755966,1.45439216225896E-14,
50.1045381897769));
#191837=CARTESIAN_POINT('Origin',(108.830927758152,-5.8,62.4396978731943));
#191838=CARTESIAN_POINT('',(109.215883585073,-5.8,63.0796906422719));
#191839=CARTESIAN_POINT('',(109.149636973735,-5.8,63.4204982119526));
#191840=CARTESIAN_POINT('',(109.215883585073,-5.8,63.0796906422719));
#191841=CARTESIAN_POINT('',(108.765152664381,-5.8,62.7780797073851));
#191842=CARTESIAN_POINT('Origin',(116.959178380441,-5.8,51.0204257716897));
#191843=CARTESIAN_POINT('',(108.697871783352,-5.8,63.1242081068039));
#191844=CARTESIAN_POINT('',(108.765152664381,-5.8,62.7780797073851));
#191845=CARTESIAN_POINT('Origin',(116.959178380441,-5.8,51.0204257716897));
#191846=CARTESIAN_POINT('Origin',(109.321741260701,-5.8,62.5351028296435));
#191847=CARTESIAN_POINT('',(109.176423614682,-5.3,63.2826935783785));
#191848=CARTESIAN_POINT('',(109.111164986591,-5.3,63.6184184402417));
#191849=CARTESIAN_POINT('',(109.176423614682,-5.3,63.2826935783785));
#191850=CARTESIAN_POINT('Origin',(111.756555253416,1.45439216225896E-14,
50.0091332333276));
#191851=CARTESIAN_POINT('Origin',(111.756555253416,1.45439216225896E-14,
50.0091332333276));
#191852=CARTESIAN_POINT('Origin',(109.321741260701,-5.3,62.5351028296435));
#191853=CARTESIAN_POINT('',(108.725070082524,-5.3,62.9842856858227));
#191854=CARTESIAN_POINT('',(108.658823471186,-5.3,63.3250932555033));
#191855=CARTESIAN_POINT('',(108.725070082524,-5.3,62.9842856858227));
#191856=CARTESIAN_POINT('Origin',(116.959178380441,-5.3,51.0204257716897));
#191857=CARTESIAN_POINT('Origin',(116.959178380441,-5.3,51.0204257716897));
#191858=CARTESIAN_POINT('Origin',(108.830927758152,-5.3,62.4396978731943));
#191859=CARTESIAN_POINT('Origin',(111.265741750867,1.45439216225896E-14,
49.9137282768784));
#191860=CARTESIAN_POINT('Origin',(111.265741750867,1.45439216225896E-14,
49.9137282768784));
#191861=CARTESIAN_POINT('Origin',(108.830927758152,-4.8,62.4396978731943));
#191862=CARTESIAN_POINT('',(109.141035838722,-4.8,63.4647469948118));
#191863=CARTESIAN_POINT('',(109.076638799632,-4.8,63.7960393876363));
#191864=CARTESIAN_POINT('',(109.141035838722,-4.8,63.4647469948118));
#191865=CARTESIAN_POINT('',(108.689140295118,-4.8,63.169127495504));
#191866=CARTESIAN_POINT('Origin',(116.959178380441,-4.8,51.0204257716897));
#191867=CARTESIAN_POINT('',(108.623794466686,-4.8,63.5053009619883));
#191868=CARTESIAN_POINT('',(108.689140295118,-4.8,63.169127495504));
#191869=CARTESIAN_POINT('Origin',(116.959178380441,-4.8,51.0204257716897));
#191870=CARTESIAN_POINT('Origin',(109.321741260701,-4.8,62.5351028296435));
#191871=CARTESIAN_POINT('',(109.109556928396,-4.3,63.6266911412002));
#191872=CARTESIAN_POINT('',(109.045907632778,-4.3,63.9541367465445));
#191873=CARTESIAN_POINT('',(109.109556928396,-4.3,63.6266911412002));
#191874=CARTESIAN_POINT('Origin',(111.756555253416,1.45439216225896E-14,
50.0091332333276));
#191875=CARTESIAN_POINT('Origin',(111.756555253416,1.45439216225896E-14,
50.0091332333276));
#191876=CARTESIAN_POINT('Origin',(109.321741260701,-4.3,62.5351028296435));
#191877=CARTESIAN_POINT('',(108.657191696567,-4.3,63.3334879662788));
#191878=CARTESIAN_POINT('',(108.592626755884,-4.3,63.6656441336094));
#191879=CARTESIAN_POINT('',(108.657191696567,-4.3,63.3334879662788));
#191880=CARTESIAN_POINT('Origin',(116.959178380441,-4.3,51.0204257716897));
#191881=CARTESIAN_POINT('Origin',(116.959178380441,-4.3,51.0204257716897));
#191882=CARTESIAN_POINT('Origin',(108.830927758152,-4.3,62.4396978731943));
#191883=CARTESIAN_POINT('Origin',(111.265741750867,1.45439216225896E-14,
49.9137282768784));
#191884=CARTESIAN_POINT('Origin',(111.265741750867,1.45439216225896E-14,
49.9137282768784));
#191885=CARTESIAN_POINT('Origin',(108.830927758152,-3.8,62.4396978731943));
#191886=CARTESIAN_POINT('',(109.08184886855,-3.8,63.7692360404209));
#191887=CARTESIAN_POINT('',(109.018843684266,-3.8,64.0933679967464));
#191888=CARTESIAN_POINT('',(109.08184886855,-3.8,63.7692360404209));
#191889=CARTESIAN_POINT('',(108.629079561968,-3.8,63.4781116395155));
#191890=CARTESIAN_POINT('Origin',(116.959178380441,-3.8,51.0204257716897));
#191891=CARTESIAN_POINT('',(108.565186643304,-3.8,63.8068105705237));
#191892=CARTESIAN_POINT('',(108.629079561968,-3.8,63.4781116395155));
#191893=CARTESIAN_POINT('Origin',(116.959178380441,-3.8,51.0204257716897));
#191894=CARTESIAN_POINT('Origin',(109.321741260701,-3.8,62.5351028296435));
#191895=CARTESIAN_POINT('',(109.057795511165,-3.3,63.8929792192369));
#191896=CARTESIAN_POINT('',(108.995339119714,-3.3,64.2142878952807));
#191897=CARTESIAN_POINT('',(109.057795511165,-3.3,63.8929792192369));
#191898=CARTESIAN_POINT('Origin',(111.756555253416,1.45439216225896E-14,
50.0091332333276));
#191899=CARTESIAN_POINT('Origin',(111.756555253416,1.45439216225896E-14,
50.0091332333276));
#191900=CARTESIAN_POINT('Origin',(109.321741260701,-3.3,62.5351028296435));
#191901=CARTESIAN_POINT('',(108.604682300287,-3.3,63.6036240437319));
#191902=CARTESIAN_POINT('',(108.541361492875,-3.3,63.9293797321879));
#191903=CARTESIAN_POINT('',(108.604682300287,-3.3,63.6036240437319));
#191904=CARTESIAN_POINT('Origin',(116.959178380441,-3.3,51.0204257716897));
#191905=CARTESIAN_POINT('Origin',(116.959178380441,-3.3,51.0204257716897));
#191906=CARTESIAN_POINT('Origin',(108.830927758152,-3.3,62.4396978731943));
#191907=CARTESIAN_POINT('Origin',(111.265741750867,1.45439216225896E-14,
49.9137282768784));
#191908=CARTESIAN_POINT('Origin',(111.265741750867,1.45439216225896E-14,
49.9137282768784));
#191909=CARTESIAN_POINT('Origin',(108.830927758152,-2.8,62.4396978731943));
#191910=CARTESIAN_POINT('',(109.037299870757,-2.8,63.9984196222324));
#191911=CARTESIAN_POINT('',(108.975303695801,-2.8,64.3173607014716));
#191912=CARTESIAN_POINT('',(109.037299870757,-2.8,63.9984196222324));
#191913=CARTESIAN_POINT('',(108.583898524792,-2.8,63.7105467658482));
#191914=CARTESIAN_POINT('Origin',(116.959178380441,-2.8,51.0204257716897));
#191915=CARTESIAN_POINT('',(108.521057164277,-2.8,64.0338359261557));
#191916=CARTESIAN_POINT('',(108.583898524792,-2.8,63.7105467658482));
#191917=CARTESIAN_POINT('Origin',(116.959178380441,-2.8,51.0204257716897));
#191918=CARTESIAN_POINT('Origin',(109.321741260701,-2.8,62.5351028296435));
#191919=CARTESIAN_POINT('',(109.020282000538,-2.3,64.0859685379196));
#191920=CARTESIAN_POINT('',(108.958662885038,-2.3,64.4029698241028));
#191921=CARTESIAN_POINT('',(109.020282000538,-2.3,64.0859685379196));
#191922=CARTESIAN_POINT('Origin',(111.756555253416,1.45439216225896E-14,
50.0091332333276));
#191923=CARTESIAN_POINT('Origin',(111.756555253416,1.45439216225896E-14,
50.0091332333276));
#191924=CARTESIAN_POINT('Origin',(109.321741260701,-2.3,62.5351028296435));
#191925=CARTESIAN_POINT('',(108.566644759735,-2.3,63.7993092492148));
#191926=CARTESIAN_POINT('',(108.504195995651,-2.3,64.1205786860541));
#191927=CARTESIAN_POINT('',(108.566644759735,-2.3,63.7993092492148));
#191928=CARTESIAN_POINT('Origin',(116.959178380441,-2.3,51.0204257716897));
#191929=CARTESIAN_POINT('Origin',(116.959178380441,-2.3,51.0204257716897));
#191930=CARTESIAN_POINT('Origin',(108.830927758152,-2.3,62.4396978731943));
#191931=CARTESIAN_POINT('Origin',(111.265741750867,1.45439216225896E-14,
49.9137282768784));
#191932=CARTESIAN_POINT('Origin',(111.265741750867,1.45439216225896E-14,
49.9137282768784));
#191933=CARTESIAN_POINT('Origin',(108.830927758152,-1.8,62.4396978731943));
#191934=CARTESIAN_POINT('',(109.006677332257,-1.8,64.1559581394927));
#191935=CARTESIAN_POINT('',(108.945356403834,-1.8,64.4714253938064));
#191936=CARTESIAN_POINT('',(109.006677332257,-1.8,64.1559581394927));
#191937=CARTESIAN_POINT('',(108.552853652473,-1.8,63.870257991408));
#191938=CARTESIAN_POINT('Origin',(116.959178380441,-1.8,51.0204257716897));
#191939=CARTESIAN_POINT('',(108.490715223963,-1.8,64.1899308980908));
#191940=CARTESIAN_POINT('',(108.552853652473,-1.8,63.870257991408));
#191941=CARTESIAN_POINT('Origin',(116.959178380441,-1.8,51.0204257716897));
#191942=CARTESIAN_POINT('Origin',(109.321741260701,-1.8,62.5351028296435));
#191943=CARTESIAN_POINT('',(108.996435394296,-1.3,64.2086480796238));
#191944=CARTESIAN_POINT('',(108.93533707197,-1.3,64.5229701305617));
#191945=CARTESIAN_POINT('',(108.996435394296,-1.3,64.2086480796238));
#191946=CARTESIAN_POINT('Origin',(111.756555253416,1.45439216225896E-14,
50.0091332333276));
#191947=CARTESIAN_POINT('Origin',(111.756555253416,1.45439216225896E-14,
50.0091332333276));
#191948=CARTESIAN_POINT('Origin',(109.321741260701,-1.3,62.5351028296435));
#191949=CARTESIAN_POINT('',(108.542472596003,-1.3,63.9236636306546));
#191950=CARTESIAN_POINT('',(108.480565763526,-1.3,64.2421450849782));
#191951=CARTESIAN_POINT('',(108.542472596003,-1.3,63.9236636306546));
#191952=CARTESIAN_POINT('Origin',(116.959178380441,-1.3,51.0204257716897));
#191953=CARTESIAN_POINT('Origin',(116.959178380441,-1.3,51.0204257716897));
#191954=CARTESIAN_POINT('Origin',(108.830927758152,-1.3,62.4396978731943));
#191955=CARTESIAN_POINT('Origin',(111.265741750867,1.45439216225896E-14,
49.9137282768784));
#191956=CARTESIAN_POINT('Origin',(111.265741750867,1.45439216225896E-14,
49.9137282768784));
#191957=CARTESIAN_POINT('Origin',(108.830927758152,-0.799999999999986,62.4396978731943));
#191958=CARTESIAN_POINT('',(108.989518845865,-0.799999999999986,64.2442304590662));
#191959=CARTESIAN_POINT('',(108.928569950886,-0.799999999999986,64.5577837767815));
#191960=CARTESIAN_POINT('',(108.989518845865,-0.799999999999986,64.2442304590662));
#191961=CARTESIAN_POINT('',(108.535462692998,-0.799999999999986,63.9597262753498));
#191962=CARTESIAN_POINT('Origin',(116.959178380441,-0.799999999999986,51.0204257716897));
#191963=CARTESIAN_POINT('',(108.473711284619,-0.799999999999986,64.2774081459953));
#191964=CARTESIAN_POINT('',(108.535462692998,-0.799999999999986,63.9597262753498));
#191965=CARTESIAN_POINT('Origin',(116.959178380441,-0.799999999999986,51.0204257716897));
#191966=CARTESIAN_POINT('Origin',(109.321741260701,-0.799999999999986,62.5351028296435));
#191967=CARTESIAN_POINT('',(108.985902782736,-0.299999999999985,64.2628333983237));
#191968=CARTESIAN_POINT('',(108.925031722893,-0.299999999999985,64.5759862909769));
#191969=CARTESIAN_POINT('',(108.985902782736,-0.299999999999985,64.2628333983237));
#191970=CARTESIAN_POINT('Origin',(111.756555253416,1.45439216225896E-14,
50.0091332333276));
#191971=CARTESIAN_POINT('Origin',(111.756555253416,1.45439216225896E-14,
50.0091332333276));
#191972=CARTESIAN_POINT('Origin',(109.321741260701,-0.299999999999985,62.5351028296435));
#191973=CARTESIAN_POINT('',(108.531798012159,-0.299999999999985,63.9785793297914));
#191974=CARTESIAN_POINT('',(108.470127550547,-0.299999999999985,64.2958447675021));
#191975=CARTESIAN_POINT('',(108.531798012159,-0.299999999999985,63.9785793297914));
#191976=CARTESIAN_POINT('Origin',(116.959178380441,-0.299999999999985,51.0204257716897));
#191977=CARTESIAN_POINT('Origin',(116.959178380441,-0.299999999999985,51.0204257716897));
#191978=CARTESIAN_POINT('Origin',(108.830927758152,-0.299999999999985,62.4396978731943));
#191979=CARTESIAN_POINT('Origin',(111.265741750867,1.45439216225896E-14,
49.9137282768784));
#191980=CARTESIAN_POINT('Origin',(111.265741750867,1.45439216225896E-14,
49.9137282768784));
#191981=CARTESIAN_POINT('Origin',(120.61045181934,-0.799999999999986,64.7294168279763));
#191982=CARTESIAN_POINT('',(120.881869643786,-0.799999999999986,65.9535090688376));
#191983=CARTESIAN_POINT('',(120.818389235277,-0.799999999999986,66.2800858296606));
#191984=CARTESIAN_POINT('',(120.881869643786,-0.799999999999986,65.9535090688376));
#191985=CARTESIAN_POINT('',(120.347180694029,-0.799999999999986,66.0838225941224));
#191986=CARTESIAN_POINT('Origin',(116.959178380441,-0.799999999999986,51.0204257716897));
#191987=CARTESIAN_POINT('',(120.284709039459,-0.799999999999986,66.4052097917178));
#191988=CARTESIAN_POINT('',(120.347180694029,-0.799999999999986,66.0838225941224));
#191989=CARTESIAN_POINT('Origin',(116.959178380441,-0.799999999999986,51.0204257716897));
#191990=CARTESIAN_POINT('Origin',(121.101265321889,-0.799999999999986,64.8248217844256));
#191991=CARTESIAN_POINT('',(120.878100080442,-0.299999999999985,65.9729016943031));
#191992=CARTESIAN_POINT('',(120.814707601689,-0.299999999999985,66.2990260980001));
#191993=CARTESIAN_POINT('',(120.878100080442,-0.299999999999985,65.9729016943031));
#191994=CARTESIAN_POINT('Origin',(123.536079314605,1.45439216225896E-14,
52.2988521881097));
#191995=CARTESIAN_POINT('Origin',(123.536079314605,1.45439216225896E-14,
52.2988521881097));
#191996=CARTESIAN_POINT('Origin',(121.101265321889,-0.299999999999985,64.8248217844256));
#191997=CARTESIAN_POINT('',(120.343472345358,-0.299999999999985,66.1029002989693));
#191998=CARTESIAN_POINT('',(120.28108449975,-0.299999999999985,66.4238563389795));
#191999=CARTESIAN_POINT('',(120.343472345358,-0.299999999999985,66.1029002989693));
#192000=CARTESIAN_POINT('Origin',(116.959178380441,-0.299999999999985,51.0204257716897));
#192001=CARTESIAN_POINT('Origin',(116.959178380441,-0.299999999999985,51.0204257716897));
#192002=CARTESIAN_POINT('Origin',(120.61045181934,-0.299999999999985,64.7294168279763));
#192003=CARTESIAN_POINT('Origin',(123.045265812055,1.45439216225896E-14,
52.2034472316604));
#192004=CARTESIAN_POINT('Origin',(123.045265812055,1.45439216225896E-14,
52.2034472316604));
#192005=CARTESIAN_POINT('Origin',(120.61045181934,-1.8,64.7294168279763));
#192006=CARTESIAN_POINT('',(120.8997623615,-1.8,65.8614594754157));
#192007=CARTESIAN_POINT('',(120.835861273808,-1.8,66.1902004322221));
#192008=CARTESIAN_POINT('',(120.8997623615,-1.8,65.8614594754157));
#192009=CARTESIAN_POINT('',(120.3647805193,-1.8,65.9932797941777));
#192010=CARTESIAN_POINT('Origin',(116.959178380441,-1.8,51.0204257716897));
#192011=CARTESIAN_POINT('',(120.301908052796,-1.8,66.3167289801245));
#192012=CARTESIAN_POINT('',(120.3647805193,-1.8,65.9932797941777));
#192013=CARTESIAN_POINT('Origin',(116.959178380441,-1.8,51.0204257716897));
#192014=CARTESIAN_POINT('Origin',(121.101265321889,-1.8,64.8248217844256));
#192015=CARTESIAN_POINT('',(120.889080989585,-1.3,65.9164100959823));
#192016=CARTESIAN_POINT('',(120.825431693966,-1.3,66.2438557013266));
#192017=CARTESIAN_POINT('',(120.889080989585,-1.3,65.9164100959823));
#192018=CARTESIAN_POINT('Origin',(123.536079314605,1.45439216225896E-14,
52.2988521881097));
#192019=CARTESIAN_POINT('Origin',(123.536079314605,1.45439216225896E-14,
52.2988521881097));
#192020=CARTESIAN_POINT('Origin',(121.101265321889,-1.3,64.8248217844256));
#192021=CARTESIAN_POINT('',(120.354274459392,-1.3,66.0473285171533));
#192022=CARTESIAN_POINT('',(120.291641863378,-1.3,66.3695436825644));
#192023=CARTESIAN_POINT('',(120.354274459392,-1.3,66.0473285171533));
#192024=CARTESIAN_POINT('Origin',(116.959178380441,-1.3,51.0204257716897));
#192025=CARTESIAN_POINT('Origin',(116.959178380441,-1.3,51.0204257716897));
#192026=CARTESIAN_POINT('Origin',(120.61045181934,-1.3,64.7294168279763));
#192027=CARTESIAN_POINT('Origin',(123.045265812055,1.45439216225896E-14,
52.2034472316604));
#192028=CARTESIAN_POINT('Origin',(123.045265812055,1.45439216225896E-14,
52.2034472316604));
#192029=CARTESIAN_POINT('Origin',(120.61045181934,-2.8,64.7294168279763));
#192030=CARTESIAN_POINT('',(120.931719828652,-2.8,65.6970533798742));
#192031=CARTESIAN_POINT('',(120.867053514301,-2.8,66.0297310669131));
#192032=CARTESIAN_POINT('',(120.931719828652,-2.8,65.6970533798742));
#192033=CARTESIAN_POINT('',(120.396205099365,-2.8,65.8316151513545));
#192034=CARTESIAN_POINT('Origin',(116.959178380441,-2.8,51.0204257716897));
#192035=CARTESIAN_POINT('',(120.332604194726,-2.8,66.158811807933));
#192036=CARTESIAN_POINT('',(120.396205099365,-2.8,65.8316151513545));
#192037=CARTESIAN_POINT('Origin',(116.959178380441,-2.8,51.0204257716897));
#192038=CARTESIAN_POINT('Origin',(121.101265321889,-2.8,64.8248217844256));
#192039=CARTESIAN_POINT('',(120.913956165254,-2.3,65.7884390497044));
#192040=CARTESIAN_POINT('',(120.849717425175,-2.3,66.1189170687846));
#192041=CARTESIAN_POINT('',(120.913956165254,-2.3,65.7884390497044));
#192042=CARTESIAN_POINT('Origin',(123.536079314605,1.45439216225896E-14,
52.2988521881097));
#192043=CARTESIAN_POINT('Origin',(123.536079314605,1.45439216225896E-14,
52.2988521881097));
#192044=CARTESIAN_POINT('Origin',(121.101265321889,-2.3,64.8248217844256));
#192045=CARTESIAN_POINT('',(120.37873920656,-2.3,65.9214689319321));
#192046=CARTESIAN_POINT('',(120.315545216751,-2.3,66.2465722036342));
#192047=CARTESIAN_POINT('',(120.37873920656,-2.3,65.9214689319321));
#192048=CARTESIAN_POINT('Origin',(116.959178380441,-2.3,51.0204257716897));
#192049=CARTESIAN_POINT('Origin',(116.959178380441,-2.3,51.0204257716897));
#192050=CARTESIAN_POINT('Origin',(120.61045181934,-2.3,64.7294168279763));
#192051=CARTESIAN_POINT('Origin',(123.045265812055,1.45439216225896E-14,
52.2034472316604));
#192052=CARTESIAN_POINT('Origin',(123.045265812055,1.45439216225896E-14,
52.2034472316604));
#192053=CARTESIAN_POINT('Origin',(120.61045181934,-3.8,64.7294168279763));
#192054=CARTESIAN_POINT('',(120.978269168954,-3.8,65.4575789793226));
#192055=CARTESIAN_POINT('',(120.912455269166,-3.8,65.7961604521707));
#192056=CARTESIAN_POINT('',(120.978269168954,-3.8,65.4575789793226));
#192057=CARTESIAN_POINT('',(120.441955022188,-3.8,65.5962533766876));
#192058=CARTESIAN_POINT('Origin',(116.959178380441,-3.8,51.0204257716897));
#192059=CARTESIAN_POINT('',(120.377263289707,-3.8,65.9290618280169));
#192060=CARTESIAN_POINT('',(120.441955022188,-3.8,65.5962533766876));
#192061=CARTESIAN_POINT('Origin',(116.959178380441,-3.8,51.0204257716897));
#192062=CARTESIAN_POINT('Origin',(121.101265321889,-3.8,64.8248217844256));
#192063=CARTESIAN_POINT('',(120.953127003325,-3.3,65.5869235630155));
#192064=CARTESIAN_POINT('',(120.887937884665,-3.3,65.9222908316384));
#192065=CARTESIAN_POINT('',(120.953127003325,-3.3,65.5869235630155));
#192066=CARTESIAN_POINT('Origin',(123.536079314605,1.45439216225896E-14,
52.2988521881097));
#192067=CARTESIAN_POINT('Origin',(123.536079314605,1.45439216225896E-14,
52.2988521881097));
#192068=CARTESIAN_POINT('Origin',(121.101265321889,-3.3,64.8248217844256));
#192069=CARTESIAN_POINT('',(120.417248123798,-3.3,65.7233587157339));
#192070=CARTESIAN_POINT('',(120.35315003438,-3.3,66.0531131534987));
#192071=CARTESIAN_POINT('',(120.417248123798,-3.3,65.7233587157339));
#192072=CARTESIAN_POINT('Origin',(116.959178380441,-3.3,51.0204257716897));
#192073=CARTESIAN_POINT('Origin',(116.959178380441,-3.3,51.0204257716897));
#192074=CARTESIAN_POINT('Origin',(120.61045181934,-3.3,64.7294168279763));
#192075=CARTESIAN_POINT('Origin',(123.045265812055,1.45439216225896E-14,
52.2034472316604));
#192076=CARTESIAN_POINT('Origin',(123.045265812055,1.45439216225896E-14,
52.2034472316604));
#192077=CARTESIAN_POINT('Origin',(120.61045181934,-4.8,64.7294168279763));
#192078=CARTESIAN_POINT('',(121.040226693838,-4.8,65.1388367364764));
#192079=CARTESIAN_POINT('',(120.972821486136,-4.8,65.4856047379895));
#192080=CARTESIAN_POINT('',(121.040226693838,-4.8,65.1388367364764));
#192081=CARTESIAN_POINT('',(120.502803495316,-4.8,65.2832166820304));
#192082=CARTESIAN_POINT('Origin',(116.959178380441,-4.8,51.0204257716897));
#192083=CARTESIAN_POINT('',(120.436602356825,-4.8,65.6237903153597));
#192084=CARTESIAN_POINT('',(120.502803495316,-4.8,65.2832166820304));
#192085=CARTESIAN_POINT('Origin',(116.959178380441,-4.8,51.0204257716897));
#192086=CARTESIAN_POINT('Origin',(121.101265321889,-4.8,64.8248217844256));
#192087=CARTESIAN_POINT('',(121.007257725681,-4.3,65.3084465276117));
#192088=CARTESIAN_POINT('',(120.940708624467,-4.3,65.6508102650276));
#192089=CARTESIAN_POINT('',(121.007257725681,-4.3,65.3084465276117));
#192090=CARTESIAN_POINT('Origin',(123.536079314605,1.45439216225896E-14,
52.2988521881097));
#192091=CARTESIAN_POINT('Origin',(123.536079314605,1.45439216225896E-14,
52.2988521881097));
#192092=CARTESIAN_POINT('Origin',(121.101265321889,-4.3,64.8248217844256));
#192093=CARTESIAN_POINT('',(120.470431262797,-4.3,65.4497565497637));
#192094=CARTESIAN_POINT('',(120.40504170288,-4.3,65.7861549941143));
#192095=CARTESIAN_POINT('',(120.470431262797,-4.3,65.4497565497637));
#192096=CARTESIAN_POINT('Origin',(116.959178380441,-4.3,51.0204257716897));
#192097=CARTESIAN_POINT('Origin',(116.959178380441,-4.3,51.0204257716897));
#192098=CARTESIAN_POINT('Origin',(120.61045181934,-4.3,64.7294168279763));
#192099=CARTESIAN_POINT('Origin',(123.045265812055,1.45439216225896E-14,
52.2034472316604));
#192100=CARTESIAN_POINT('Origin',(123.045265812055,1.45439216225896E-14,
52.2034472316604));
#192101=CARTESIAN_POINT('Origin',(119.628824814241,-4.8,64.5386069150778));
#192102=CARTESIAN_POINT('',(119.96973864102,-4.8,65.4051750021872));
#192103=CARTESIAN_POINT('',(119.904592853105,-4.8,65.7403193545668));
#192104=CARTESIAN_POINT('',(119.96973864102,-4.8,65.4051750021872));
#192105=CARTESIAN_POINT('',(119.440821494858,-4.8,65.5057953202889));
#192106=CARTESIAN_POINT('Origin',(116.959178380441,-4.8,51.0204257716897));
#192107=CARTESIAN_POINT('',(119.376599349995,-4.8,65.8361879648046));
#192108=CARTESIAN_POINT('',(119.440821494858,-4.8,65.5057953202889));
#192109=CARTESIAN_POINT('Origin',(116.959178380441,-4.8,51.0204257716897));
#192110=CARTESIAN_POINT('Origin',(120.11963831679,-4.8,64.6340118715271));
#192111=CARTESIAN_POINT('',(119.937889091834,-4.3,65.5690259106978));
#192112=CARTESIAN_POINT('',(119.873517125155,-4.3,65.9001893177927));
#192113=CARTESIAN_POINT('',(119.937889091834,-4.3,65.5690259106978));
#192114=CARTESIAN_POINT('Origin',(122.554452309506,1.45439216225896E-14,
52.1080422752111));
#192115=CARTESIAN_POINT('Origin',(122.554452309506,1.45439216225896E-14,
52.1080422752111));
#192116=CARTESIAN_POINT('Origin',(120.11963831679,-4.3,64.6340118715271));
#192117=CARTESIAN_POINT('',(119.409429136137,-4.3,65.6672941994899));
#192118=CARTESIAN_POINT('',(119.345948727628,-4.3,65.9938709603129));
#192119=CARTESIAN_POINT('',(119.409429136137,-4.3,65.6672941994899));
#192120=CARTESIAN_POINT('Origin',(116.959178380441,-4.3,51.0204257716897));
#192121=CARTESIAN_POINT('Origin',(116.959178380441,-4.3,51.0204257716897));
#192122=CARTESIAN_POINT('Origin',(119.628824814241,-4.3,64.5386069150778));
#192123=CARTESIAN_POINT('Origin',(122.063638806956,1.45439216225896E-14,
52.0126373187619));
#192124=CARTESIAN_POINT('Origin',(122.063638806956,1.45439216225896E-14,
52.0126373187619));
#192125=CARTESIAN_POINT('Origin',(118.647197809142,-4.8,64.3477970021793));
#192126=CARTESIAN_POINT('',(118.915873602585,-4.8,65.5859956992519));
#192127=CARTESIAN_POINT('',(118.85245717924,-4.8,65.9122432865856));
#192128=CARTESIAN_POINT('',(118.915873602585,-4.8,65.5859956992519));
#192129=CARTESIAN_POINT('',(118.394743704415,-4.8,65.6465542993439));
#192130=CARTESIAN_POINT('Origin',(116.959178380441,-4.8,51.0204257716897));
#192131=CARTESIAN_POINT('',(118.332026307686,-4.8,65.9692057244349));
#192132=CARTESIAN_POINT('',(118.394743704415,-4.8,65.6465542993439));
#192133=CARTESIAN_POINT('Origin',(116.959178380441,-4.8,51.0204257716897));
#192134=CARTESIAN_POINT('Origin',(119.138011311691,-4.8,64.4432019586286));
#192135=CARTESIAN_POINT('',(118.884879867865,-4.3,65.7454438459865));
#192136=CARTESIAN_POINT('',(118.822177915075,-4.3,66.0680158192969));
#192137=CARTESIAN_POINT('',(118.884879867865,-4.3,65.7454438459865));
#192138=CARTESIAN_POINT('Origin',(121.572825304407,1.45439216225896E-14,
51.9172323623126));
#192139=CARTESIAN_POINT('Origin',(121.572825304407,1.45439216225896E-14,
51.9172323623126));
#192140=CARTESIAN_POINT('Origin',(119.138011311691,-4.3,64.4432019586286));
#192141=CARTESIAN_POINT('',(118.364095660481,-4.3,65.8042240300283));
#192142=CARTESIAN_POINT('',(118.302069618616,-4.3,66.1233187604272));
#192143=CARTESIAN_POINT('',(118.364095660481,-4.3,65.8042240300283));
#192144=CARTESIAN_POINT('Origin',(116.959178380441,-4.3,51.0204257716897));
#192145=CARTESIAN_POINT('Origin',(116.959178380441,-4.3,51.0204257716897));
#192146=CARTESIAN_POINT('Origin',(118.647197809142,-4.3,64.3477970021793));
#192147=CARTESIAN_POINT('Origin',(121.082011801857,1.45439216225896E-14,
51.8218274058634));
#192148=CARTESIAN_POINT('Origin',(121.082011801857,1.45439216225896E-14,
51.8218274058634));
#192149=CARTESIAN_POINT('Origin',(117.665570804043,-4.8,64.1569870892808));
#192150=CARTESIAN_POINT('',(117.87730384708,-4.8,65.6881293797663));
#192151=CARTESIAN_POINT('',(117.815187944779,-4.8,66.0076863997269));
#192152=CARTESIAN_POINT('',(117.87730384708,-4.8,65.6881293797663));
#192153=CARTESIAN_POINT('',(117.363446332578,-4.8,65.7112749959501));
#192154=CARTESIAN_POINT('Origin',(116.959178380441,-4.8,51.0204257716897));
#192155=CARTESIAN_POINT('',(117.301841863851,-4.8,66.028200931394));
#192156=CARTESIAN_POINT('',(117.363446332578,-4.8,65.7112749959501));
#192157=CARTESIAN_POINT('Origin',(116.959178380441,-4.8,51.0204257716897));
#192158=CARTESIAN_POINT('Origin',(118.156384306592,-4.8,64.25239204573));
#192159=CARTESIAN_POINT('',(117.846953153215,-4.3,65.844269384596));
#192160=CARTESIAN_POINT('',(117.785509112589,-4.3,66.1603699931248));
#192161=CARTESIAN_POINT('',(117.846953153215,-4.3,65.844269384596));
#192162=CARTESIAN_POINT('Origin',(120.591198299308,1.45439216225896E-14,
51.7264224494141));
#192163=CARTESIAN_POINT('Origin',(120.591198299308,1.45439216225896E-14,
51.7264224494141));
#192164=CARTESIAN_POINT('Origin',(118.156384306592,-4.3,64.25239204573));
#192165=CARTESIAN_POINT('',(117.333348389206,-4.3,65.8661147187035));
#192166=CARTESIAN_POINT('',(117.272399494227,-4.3,66.1796680364188));
#192167=CARTESIAN_POINT('',(117.333348389206,-4.3,65.8661147187035));
#192168=CARTESIAN_POINT('Origin',(116.959178380441,-4.3,51.0204257716897));
#192169=CARTESIAN_POINT('Origin',(116.959178380441,-4.3,51.0204257716897));
#192170=CARTESIAN_POINT('Origin',(117.665570804043,-4.3,64.1569870892808));
#192171=CARTESIAN_POINT('Origin',(120.100384796758,1.45439216225896E-14,
51.6310174929649));
#192172=CARTESIAN_POINT('Origin',(120.100384796758,1.45439216225896E-14,
51.6310174929649));
#192173=CARTESIAN_POINT('Origin',(116.683943798944,-4.8,63.9661771763823));
#192174=CARTESIAN_POINT('',(116.853081315242,-4.8,65.7164533614791));
#192175=CARTESIAN_POINT('',(116.791904281457,-4.8,66.0311803457483));
#192176=CARTESIAN_POINT('',(116.853081315242,-4.8,65.7164533614791));
#192177=CARTESIAN_POINT('',(116.346134910676,-4.8,65.7040445767105));
#192178=CARTESIAN_POINT('Origin',(116.959178380441,-4.8,51.0204257716897));
#192179=CARTESIAN_POINT('',(116.285306180856,-4.8,66.0169797013613));
#192180=CARTESIAN_POINT('',(116.346134910676,-4.8,65.7040445767105));
#192181=CARTESIAN_POINT('Origin',(116.959178380441,-4.8,51.0204257716897));
#192182=CARTESIAN_POINT('Origin',(117.174757301493,-4.8,64.0615821328315));
#192183=CARTESIAN_POINT('',(116.823194555833,-4.3,65.8702066423449));
#192184=CARTESIAN_POINT('',(116.762659683573,-4.3,66.1816300084491));
#192185=CARTESIAN_POINT('',(116.823194555833,-4.3,65.8702066423449));
#192186=CARTESIAN_POINT('Origin',(119.609571294209,1.45439216225896E-14,
51.5356125365156));
#192187=CARTESIAN_POINT('Origin',(119.609571294209,1.45439216225896E-14,
51.5356125365156));
#192188=CARTESIAN_POINT('Origin',(117.174757301493,-4.3,64.0615821328315));
#192189=CARTESIAN_POINT('',(116.316420202403,-4.3,65.8569127356375));
#192190=CARTESIAN_POINT('',(116.256222839073,-4.3,66.1665997774845));
#192191=CARTESIAN_POINT('',(116.316420202403,-4.3,65.8569127356375));
#192192=CARTESIAN_POINT('Origin',(116.959178380441,-4.3,51.0204257716897));
#192193=CARTESIAN_POINT('Origin',(116.959178380441,-4.3,51.0204257716897));
#192194=CARTESIAN_POINT('Origin',(116.683943798944,-4.3,63.9661771763823));
#192195=CARTESIAN_POINT('Origin',(119.118757791659,1.45439216225896E-14,
51.4402075800664));
#192196=CARTESIAN_POINT('Origin',(119.118757791659,1.45439216225896E-14,
51.4402075800664));
#192197=CARTESIAN_POINT('Origin',(115.702316793845,-4.8,63.7753672634838));
#192198=CARTESIAN_POINT('',(115.842547716854,-4.8,65.6743542370615));
#192199=CARTESIAN_POINT('',(115.781991995879,-4.8,65.9858848599729));
#192200=CARTESIAN_POINT('',(115.842547716854,-4.8,65.6743542370615));
#192201=CARTESIAN_POINT('',(115.342273674314,-4.8,65.6276192967388));
#192202=CARTESIAN_POINT('Origin',(116.959178380441,-4.8,51.0204257716897));
#192203=CARTESIAN_POINT('',(115.281918593308,-4.8,65.9381177216365));
#192204=CARTESIAN_POINT('',(115.342273674314,-4.8,65.6276192967388));
#192205=CARTESIAN_POINT('Origin',(116.959178380441,-4.8,51.0204257716897));
#192206=CARTESIAN_POINT('Origin',(116.193130296394,-4.8,63.870772219933));
#192207=CARTESIAN_POINT('',(115.812967843606,-4.3,65.8265287333784));
#192208=CARTESIAN_POINT('',(115.753035111526,-4.3,66.1348543722614));
#192209=CARTESIAN_POINT('',(115.812967843606,-4.3,65.8265287333784));
#192210=CARTESIAN_POINT('Origin',(118.62794428911,1.45439216225896E-14,
51.3448026236171));
#192211=CARTESIAN_POINT('Origin',(118.62794428911,1.45439216225896E-14,
51.3448026236171));
#192212=CARTESIAN_POINT('Origin',(116.193130296394,-4.3,63.870772219933));
#192213=CARTESIAN_POINT('',(115.312792881512,-4.3,65.7792840708942));
#192214=CARTESIAN_POINT('',(115.253054679294,-4.3,66.0866089453843));
#192215=CARTESIAN_POINT('',(115.312792881512,-4.3,65.7792840708942));
#192216=CARTESIAN_POINT('Origin',(116.959178380441,-4.3,51.0204257716897));
#192217=CARTESIAN_POINT('Origin',(116.959178380441,-4.3,51.0204257716897));
#192218=CARTESIAN_POINT('Origin',(115.702316793845,-4.3,63.7753672634838));
#192219=CARTESIAN_POINT('Origin',(118.13713078656,1.45439216225896E-14,
51.2493976671679));
#192220=CARTESIAN_POINT('Origin',(118.13713078656,1.45439216225896E-14,
51.2493976671679));
#192221=CARTESIAN_POINT('Origin',(114.720689788746,-4.8,63.5845573505853));
#192222=CARTESIAN_POINT('',(114.845279212226,-4.8,65.5640124618232));
#192223=CARTESIAN_POINT('',(114.785054508555,-4.8,65.8738401568318));
#192224=CARTESIAN_POINT('',(114.845279212226,-4.8,65.5640124618232));
#192225=CARTESIAN_POINT('',(114.351542642308,-4.8,65.4836453083005));
#192226=CARTESIAN_POINT('Origin',(116.959178380441,-4.8,51.0204257716897));
#192227=CARTESIAN_POINT('',(114.291379402093,-4.8,65.7931568028158));
#192228=CARTESIAN_POINT('',(114.351542642308,-4.8,65.4836453083005));
#192229=CARTESIAN_POINT('Origin',(116.959178380441,-4.8,51.0204257716897));
#192230=CARTESIAN_POINT('Origin',(115.211503291295,-4.8,63.6799623070345));
#192231=CARTESIAN_POINT('',(114.815862796901,-4.3,65.7153460442249));
#192232=CARTESIAN_POINT('',(114.756251022793,-4.3,66.0220205057171));
#192233=CARTESIAN_POINT('',(114.815862796901,-4.3,65.7153460442249));
#192234=CARTESIAN_POINT('Origin',(117.64631728401,1.45439216225896E-14,
51.1539927107186));
#192235=CARTESIAN_POINT('Origin',(117.64631728401,1.45439216225896E-14,
51.1539927107186));
#192236=CARTESIAN_POINT('Origin',(115.211503291295,-4.3,63.6799623070345));
#192237=CARTESIAN_POINT('',(114.322156574729,-4.3,65.6348227658621));
#192238=CARTESIAN_POINT('',(114.26260440808,-4.3,65.9411905750978));
#192239=CARTESIAN_POINT('',(114.322156574729,-4.3,65.6348227658621));
#192240=CARTESIAN_POINT('Origin',(116.959178380441,-4.3,51.0204257716897));
#192241=CARTESIAN_POINT('Origin',(116.959178380441,-4.3,51.0204257716897));
#192242=CARTESIAN_POINT('Origin',(114.720689788746,-4.3,63.5845573505853));
#192243=CARTESIAN_POINT('Origin',(117.155503781461,1.45439216225896E-14,
51.0585877542694));
#192244=CARTESIAN_POINT('Origin',(117.155503781461,1.45439216225896E-14,
51.0585877542694));
#192245=CARTESIAN_POINT('Origin',(113.739062783647,-4.8,63.3937474376868));
#192246=CARTESIAN_POINT('',(113.861053774525,-4.8,65.3865702590969));
#192247=CARTESIAN_POINT('',(113.800883714328,-4.8,65.6961168391996));
#192248=CARTESIAN_POINT('',(113.861053774525,-4.8,65.3865702590969));
#192249=CARTESIAN_POINT('',(113.373813738472,-4.8,65.272781502971));
#192250=CARTESIAN_POINT('Origin',(116.959178380441,-4.8,51.0204257716897));
#192251=CARTESIAN_POINT('',(113.313568505077,-4.8,65.5827148137224));
#192252=CARTESIAN_POINT('',(113.373813738472,-4.8,65.272781502971));
#192253=CARTESIAN_POINT('Origin',(116.959178380441,-4.8,51.0204257716897));
#192254=CARTESIAN_POINT('Origin',(114.229876286196,-4.8,63.489152394136));
#192255=CARTESIAN_POINT('',(113.83166433961,-4.3,65.5377650400095));
#192256=CARTESIAN_POINT('',(113.772105558741,-4.3,65.8441668762851));
#192257=CARTESIAN_POINT('',(113.83166433961,-4.3,65.5377650400095));
#192258=CARTESIAN_POINT('Origin',(116.664690278911,1.45439216225896E-14,
50.9631827978201));
#192259=CARTESIAN_POINT('Origin',(116.664690278911,1.45439216225896E-14,
50.9631827978201));
#192260=CARTESIAN_POINT('Origin',(114.229876286196,-4.3,63.489152394136));
#192261=CARTESIAN_POINT('',(113.344387186316,-4.3,65.4241672345822));
#192262=CARTESIAN_POINT('',(113.284755503242,-4.3,65.7309441183195));
#192263=CARTESIAN_POINT('',(113.344387186316,-4.3,65.4241672345822));
#192264=CARTESIAN_POINT('Origin',(116.959178380441,-4.3,51.0204257716897));
#192265=CARTESIAN_POINT('Origin',(116.959178380441,-4.3,51.0204257716897));
#192266=CARTESIAN_POINT('Origin',(113.739062783647,-4.3,63.3937474376868));
#192267=CARTESIAN_POINT('Origin',(116.173876776362,1.45439216225896E-14,
50.8677778413709));
#192268=CARTESIAN_POINT('Origin',(116.173876776362,1.45439216225896E-14,
50.8677778413709));
#192269=CARTESIAN_POINT('Origin',(112.757435778548,-4.8,63.2029375247883));
#192270=CARTESIAN_POINT('',(112.889835003128,-4.8,65.1422148929144));
#192271=CARTESIAN_POINT('',(112.829445471306,-4.8,65.4528905510097));
#192272=CARTESIAN_POINT('',(112.889835003128,-4.8,65.1422148929144));
#192273=CARTESIAN_POINT('',(112.409141595728,-4.8,64.9947468201283));
#192274=CARTESIAN_POINT('Origin',(116.959178380441,-4.8,51.0204257716897));
#192275=CARTESIAN_POINT('',(112.348537143845,-4.8,65.3065281405739));
#192276=CARTESIAN_POINT('',(112.409141595728,-4.8,64.9947468201283));
#192277=CARTESIAN_POINT('Origin',(116.959178380441,-4.8,51.0204257716897));
#192278=CARTESIAN_POINT('Origin',(113.248249281097,-4.8,63.2983424812375));
#192279=CARTESIAN_POINT('',(112.860337198513,-4.3,65.2939671848206));
#192280=CARTESIAN_POINT('',(112.800565591803,-4.3,65.6014639096681));
#192281=CARTESIAN_POINT('',(112.860337198513,-4.3,65.2939671848206));
#192282=CARTESIAN_POINT('Origin',(115.683063273812,1.45439216225896E-14,
50.7723728849216));
#192283=CARTESIAN_POINT('Origin',(115.683063273812,1.45439216225896E-14,
50.7723728849216));
#192284=CARTESIAN_POINT('Origin',(113.248249281097,-4.3,63.2983424812375));
#192285=CARTESIAN_POINT('',(112.379537656463,-4.3,65.14704512475));
#192286=CARTESIAN_POINT('',(112.319557683455,-4.3,65.4556137959266));
#192287=CARTESIAN_POINT('',(112.379537656463,-4.3,65.14704512475));
#192288=CARTESIAN_POINT('Origin',(116.959178380441,-4.3,51.0204257716897));
#192289=CARTESIAN_POINT('Origin',(116.959178380441,-4.3,51.0204257716897));
#192290=CARTESIAN_POINT('Origin',(112.757435778548,-4.3,63.2029375247883));
#192291=CARTESIAN_POINT('Origin',(115.192249771263,1.45439216225896E-14,
50.6769679284724));
#192292=CARTESIAN_POINT('Origin',(115.192249771263,1.45439216225896E-14,
50.6769679284724));
#192293=CARTESIAN_POINT('Origin',(111.775808773449,-4.8,63.0121276118898));
#192294=CARTESIAN_POINT('',(111.931769528859,-4.8,64.8301920168471));
#192295=CARTESIAN_POINT('',(111.870877270834,-4.8,65.1434539641476));
#192296=CARTESIAN_POINT('',(111.931769528859,-4.8,64.8301920168471));
#192297=CARTESIAN_POINT('',(111.457767453663,-4.8,64.6483001958862));
#192298=CARTESIAN_POINT('Origin',(116.959178380441,-4.8,51.0204257716897));
#192299=CARTESIAN_POINT('',(111.396511403375,-4.8,64.9634336827943));
#192300=CARTESIAN_POINT('',(111.457767453663,-4.8,64.6483001958862));
#192301=CARTESIAN_POINT('Origin',(116.959178380441,-4.8,51.0204257716897));
#192302=CARTESIAN_POINT('Origin',(112.266622275998,-4.8,63.107532568339));
#192303=CARTESIAN_POINT('',(111.902023442088,-4.3,64.9832216033437));
#192304=CARTESIAN_POINT('',(111.841764510541,-4.3,65.2932253846267));
#192305=CARTESIAN_POINT('',(111.902023442088,-4.3,64.9832216033437));
#192306=CARTESIAN_POINT('Origin',(114.701436268713,1.45439216225896E-14,
50.5815629720231));
#192307=CARTESIAN_POINT('Origin',(114.701436268713,1.45439216225896E-14,
50.5815629720231));
#192308=CARTESIAN_POINT('Origin',(112.266622275998,-4.3,63.107532568339));
#192309=CARTESIAN_POINT('',(111.427841658067,-4.3,64.8022542995263));
#192310=CARTESIAN_POINT('',(111.367230235014,-4.3,65.1140714833514));
#192311=CARTESIAN_POINT('',(111.427841658067,-4.3,64.8022542995263));
#192312=CARTESIAN_POINT('Origin',(116.959178380441,-4.3,51.0204257716897));
#192313=CARTESIAN_POINT('Origin',(116.959178380441,-4.3,51.0204257716897));
#192314=CARTESIAN_POINT('Origin',(111.775808773449,-4.3,63.0121276118898));
#192315=CARTESIAN_POINT('Origin',(114.210622766164,1.45439216225896E-14,
50.4861580155739));
#192316=CARTESIAN_POINT('Origin',(114.210622766164,1.45439216225896E-14,
50.4861580155739));
#192317=CARTESIAN_POINT('Origin',(110.79418176835,-4.8,62.8213176989913));
#192318=CARTESIAN_POINT('',(110.987197567482,-4.8,64.4487513812576));
#192319=CARTESIAN_POINT('',(110.925497707532,-4.8,64.7661680595466));
#192320=CARTESIAN_POINT('',(110.987197567482,-4.8,64.4487513812576));
#192321=CARTESIAN_POINT('',(110.520136816659,-4.8,64.2311497203179));
#192322=CARTESIAN_POINT('Origin',(116.959178380441,-4.8,51.0204257716897));
#192323=CARTESIAN_POINT('',(110.457908037569,-4.8,64.5512874381168));
#192324=CARTESIAN_POINT('',(110.520136816659,-4.8,64.2311497203179));
#192325=CARTESIAN_POINT('Origin',(116.959178380441,-4.8,51.0204257716897));
#192326=CARTESIAN_POINT('Origin',(111.284995270899,-4.8,62.9167226554405));
#192327=CARTESIAN_POINT('',(110.957052487158,-4.3,64.6038336013966));
#192328=CARTESIAN_POINT('',(110.896011219052,-4.3,64.917862135278));
#192329=CARTESIAN_POINT('',(110.957052487158,-4.3,64.6038336013966));
#192330=CARTESIAN_POINT('Origin',(113.719809263614,1.45439216225896E-14,
50.3907530591246));
#192331=CARTESIAN_POINT('Origin',(113.719809263614,1.45439216225896E-14,
50.3907530591246));
#192332=CARTESIAN_POINT('Origin',(111.284995270899,-4.3,62.9167226554405));
#192333=CARTESIAN_POINT('',(110.489730329475,-4.3,64.3875767554558));
#192334=CARTESIAN_POINT('',(110.428177042311,-4.3,64.7042393858979));
#192335=CARTESIAN_POINT('',(110.489730329475,-4.3,64.3875767554558));
#192336=CARTESIAN_POINT('Origin',(116.959178380441,-4.3,51.0204257716897));
#192337=CARTESIAN_POINT('Origin',(116.959178380441,-4.3,51.0204257716897));
#192338=CARTESIAN_POINT('Origin',(110.79418176835,-4.3,62.8213176989913));
#192339=CARTESIAN_POINT('Origin',(113.228995761065,1.45439216225896E-14,
50.2953481026754));
#192340=CARTESIAN_POINT('Origin',(113.228995761065,1.45439216225896E-14,
50.2953481026754));
#192341=CARTESIAN_POINT('Origin',(109.812554763251,-4.8,62.6305077860928));
#192342=CARTESIAN_POINT('',(110.056678451302,-4.8,63.9950154852452));
#192343=CARTESIAN_POINT('',(109.993829318619,-4.8,64.3183446296844));
#192344=CARTESIAN_POINT('',(110.056678451302,-4.8,63.9950154852452));
#192345=CARTESIAN_POINT('',(109.596934009723,-4.8,63.7397748640298));
#192346=CARTESIAN_POINT('Origin',(116.959178380441,-4.8,51.0204257716897));
#192347=CARTESIAN_POINT('',(109.533365304474,-4.8,64.0668058699322));
#192348=CARTESIAN_POINT('',(109.596934009723,-4.8,63.7397748640298));
#192349=CARTESIAN_POINT('Origin',(116.959178380441,-4.8,51.0204257716897));
#192350=CARTESIAN_POINT('Origin',(110.3033682658,-4.8,62.725912742542));
#192351=CARTESIAN_POINT('',(110.025965270125,-4.3,64.1530203163257));
#192352=CARTESIAN_POINT('',(109.963811810516,-4.3,64.4727705509212));
#192353=CARTESIAN_POINT('',(110.025965270125,-4.3,64.1530203163257));
#192354=CARTESIAN_POINT('Origin',(112.738182258515,1.45439216225896E-14,
50.1999431462261));
#192355=CARTESIAN_POINT('Origin',(112.738182258515,1.45439216225896E-14,
50.1999431462261));
#192356=CARTESIAN_POINT('Origin',(110.3033682658,-4.3,62.725912742542));
#192357=CARTESIAN_POINT('',(109.565864948752,-4.3,63.8996105287959));
#192358=CARTESIAN_POINT('',(109.50301581607,-4.3,64.2229396732352));
#192359=CARTESIAN_POINT('',(109.565864948752,-4.3,63.8996105287959));
#192360=CARTESIAN_POINT('Origin',(116.959178380441,-4.3,51.0204257716897));
#192361=CARTESIAN_POINT('Origin',(116.959178380441,-4.3,51.0204257716897));
#192362=CARTESIAN_POINT('Origin',(109.812554763251,-4.3,62.6305077860928));
#192363=CARTESIAN_POINT('Origin',(112.247368755966,1.45439216225896E-14,
50.1045381897769));
#192364=CARTESIAN_POINT('Origin',(112.247368755966,1.45439216225896E-14,
50.1045381897769));
#192365=CARTESIAN_POINT('Origin',(109.812554763251,-3.8,62.6305077860928));
#192366=CARTESIAN_POINT('',(109.998916826926,-3.8,64.2921717990066));
#192367=CARTESIAN_POINT('',(109.937363539761,-3.8,64.6088344294486));
#192368=CARTESIAN_POINT('',(109.998916826926,-3.8,64.2921717990066));
#192369=CARTESIAN_POINT('',(109.53850981156,-3.8,64.0403398074194));
#192370=CARTESIAN_POINT('Origin',(116.959178380441,-3.8,51.0204257716897));
#192371=CARTESIAN_POINT('',(109.47628103247,-3.8,64.3604775252183));
#192372=CARTESIAN_POINT('',(109.53850981156,-3.8,64.0403398074194));
#192373=CARTESIAN_POINT('Origin',(116.959178380441,-3.8,51.0204257716897));
#192374=CARTESIAN_POINT('Origin',(110.3033682658,-3.8,62.725912742542));
#192375=CARTESIAN_POINT('',(109.975425482059,-3.3,64.4130236884981));
#192376=CARTESIAN_POINT('',(109.914384213953,-3.3,64.7270522223795));
#192377=CARTESIAN_POINT('',(109.975425482059,-3.3,64.4130236884981));
#192378=CARTESIAN_POINT('Origin',(112.738182258515,1.45439216225896E-14,
50.1999431462261));
#192379=CARTESIAN_POINT('Origin',(112.738182258515,1.45439216225896E-14,
50.1999431462261));
#192380=CARTESIAN_POINT('Origin',(110.3033682658,-3.3,62.725912742542));
#192381=CARTESIAN_POINT('',(109.514757059833,-3.3,64.1625365119099));
#192382=CARTESIAN_POINT('',(109.453057199884,-3.3,64.4799531901988));
#192383=CARTESIAN_POINT('',(109.514757059833,-3.3,64.1625365119099));
#192384=CARTESIAN_POINT('Origin',(116.959178380441,-3.3,51.0204257716897));
#192385=CARTESIAN_POINT('Origin',(116.959178380441,-3.3,51.0204257716897));
#192386=CARTESIAN_POINT('Origin',(109.812554763251,-3.3,62.6305077860928));
#192387=CARTESIAN_POINT('Origin',(112.247368755966,1.45439216225896E-14,
50.1045381897769));
#192388=CARTESIAN_POINT('Origin',(112.247368755966,1.45439216225896E-14,
50.1045381897769));
#192389=CARTESIAN_POINT('Origin',(109.812554763251,-2.8,62.6305077860928));
#192390=CARTESIAN_POINT('',(109.955401150418,-2.8,64.5160394301785));
#192391=CARTESIAN_POINT('',(109.894789727366,-2.8,64.8278566140037));
#192392=CARTESIAN_POINT('',(109.955401150418,-2.8,64.5160394301785));
#192393=CARTESIAN_POINT('',(109.494513443465,-2.8,64.2666803700892));
#192394=CARTESIAN_POINT('Origin',(116.959178380441,-2.8,51.0204257716897));
#192395=CARTESIAN_POINT('',(109.433257393177,-2.8,64.5818138569973));
#192396=CARTESIAN_POINT('',(109.494513443465,-2.8,64.2666803700892));
#192397=CARTESIAN_POINT('Origin',(116.959178380441,-2.8,51.0204257716897));
#192398=CARTESIAN_POINT('Origin',(110.3033682658,-2.8,62.725912742542));
#192399=CARTESIAN_POINT('',(109.93876943189,-2.3,64.6016017775467));
#192400=CARTESIAN_POINT('',(109.878510500343,-2.3,64.9116055588297));
#192401=CARTESIAN_POINT('',(109.93876943189,-2.3,64.6016017775467));
#192402=CARTESIAN_POINT('Origin',(112.738182258515,1.45439216225896E-14,
50.1999431462261));
#192403=CARTESIAN_POINT('Origin',(112.738182258515,1.45439216225896E-14,
50.1999431462261));
#192404=CARTESIAN_POINT('Origin',(110.3033682658,-2.3,62.725912742542));
#192405=CARTESIAN_POINT('',(109.477702016111,-2.3,64.3531672346009));
#192406=CARTESIAN_POINT('',(109.416809758086,-2.3,64.6664291819013));
#192407=CARTESIAN_POINT('',(109.477702016111,-2.3,64.3531672346009));
#192408=CARTESIAN_POINT('Origin',(116.959178380441,-2.3,51.0204257716897));
#192409=CARTESIAN_POINT('Origin',(116.959178380441,-2.3,51.0204257716897));
#192410=CARTESIAN_POINT('Origin',(109.812554763251,-2.3,62.6305077860928));
#192411=CARTESIAN_POINT('Origin',(112.247368755966,1.45439216225896E-14,
50.1045381897769));
#192412=CARTESIAN_POINT('Origin',(112.247368755966,1.45439216225896E-14,
50.1045381897769));
#192413=CARTESIAN_POINT('Origin',(109.812554763251,-1.8,62.6305077860928));
#192414=CARTESIAN_POINT('',(109.925470143716,-1.8,64.6700203425037));
#192415=CARTESIAN_POINT('',(109.865490170707,-1.8,64.9785890136804));
#192416=CARTESIAN_POINT('',(109.925470143716,-1.8,64.6700203425037));
#192417=CARTESIAN_POINT('',(109.464260580431,-1.8,64.4223170814327));
#192418=CARTESIAN_POINT('Origin',(116.959178380441,-1.8,51.0204257716897));
#192419=CARTESIAN_POINT('',(109.403656128548,-1.8,64.7340984018784));
#192420=CARTESIAN_POINT('',(109.464260580431,-1.8,64.4223170814327));
#192421=CARTESIAN_POINT('Origin',(116.959178380441,-1.8,51.0204257716897));
#192422=CARTESIAN_POINT('Origin',(110.3033682658,-1.8,62.725912742542));
#192423=CARTESIAN_POINT('',(109.915456183216,-1.3,64.7215374461251));
#192424=CARTESIAN_POINT('',(109.855684576506,-1.3,65.0290341709726));
#192425=CARTESIAN_POINT('',(109.915456183216,-1.3,64.7215374461251));
#192426=CARTESIAN_POINT('Origin',(112.738182258515,1.45439216225896E-14,
50.1999431462261));
#192427=CARTESIAN_POINT('Origin',(112.738182258515,1.45439216225896E-14,
50.1999431462261));
#192428=CARTESIAN_POINT('Origin',(110.3033682658,-1.3,62.725912742542));
#192429=CARTESIAN_POINT('',(109.454140485281,-1.3,64.4743801977696));
#192430=CARTESIAN_POINT('',(109.39375095346,-1.3,64.7850558558649));
#192431=CARTESIAN_POINT('',(109.454140485281,-1.3,64.4743801977696));
#192432=CARTESIAN_POINT('Origin',(116.959178380441,-1.3,51.0204257716897));
#192433=CARTESIAN_POINT('Origin',(116.959178380441,-1.3,51.0204257716897));
#192434=CARTESIAN_POINT('Origin',(109.812554763251,-1.3,62.6305077860928));
#192435=CARTESIAN_POINT('Origin',(112.247368755966,1.45439216225896E-14,
50.1045381897769));
#192436=CARTESIAN_POINT('Origin',(112.247368755966,1.45439216225896E-14,
50.1045381897769));
#192437=CARTESIAN_POINT('Origin',(109.812554763251,-0.799999999999986,62.6305077860928));
#192438=CARTESIAN_POINT('',(109.90869266847,-0.799999999999986,64.7563325394375));
#192439=CARTESIAN_POINT('',(109.849060985396,-0.799999999999986,65.0631094231747));
#192440=CARTESIAN_POINT('',(109.90869266847,-0.799999999999986,64.7563325394375));
#192441=CARTESIAN_POINT('',(109.447305718076,-0.799999999999986,64.509541851377));
#192442=CARTESIAN_POINT('Origin',(116.959178380441,-0.799999999999986,51.0204257716897));
#192443=CARTESIAN_POINT('',(109.387060484681,-0.799999999999986,64.8194751621284));
#192444=CARTESIAN_POINT('',(109.447305718076,-0.799999999999986,64.509541851377));
#192445=CARTESIAN_POINT('Origin',(116.959178380441,-0.799999999999986,51.0204257716897));
#192446=CARTESIAN_POINT('Origin',(110.3033682658,-0.799999999999986,62.725912742542));
#192447=CARTESIAN_POINT('',(109.905156319214,-0.299999999999985,64.7745253884155));
#192448=CARTESIAN_POINT('',(109.845597538345,-0.299999999999985,65.0809272246911));
#192449=CARTESIAN_POINT('',(109.905156319214,-0.299999999999985,64.7745253884155));
#192450=CARTESIAN_POINT('Origin',(112.738182258515,1.45439216225896E-14,
50.1999431462261));
#192451=CARTESIAN_POINT('Origin',(112.738182258515,1.45439216225896E-14,
50.1999431462261));
#192452=CARTESIAN_POINT('Origin',(110.3033682658,-0.299999999999985,62.725912742542));
#192453=CARTESIAN_POINT('',(109.443732251579,-0.299999999999985,64.5279256510537));
#192454=CARTESIAN_POINT('',(109.383562191382,-0.299999999999985,64.8374722311563));
#192455=CARTESIAN_POINT('',(109.443732251579,-0.299999999999985,64.5279256510537));
#192456=CARTESIAN_POINT('Origin',(116.959178380441,-0.299999999999985,51.0204257716897));
#192457=CARTESIAN_POINT('Origin',(116.959178380441,-0.299999999999985,51.0204257716897));
#192458=CARTESIAN_POINT('Origin',(109.812554763251,-0.299999999999985,62.6305077860928));
#192459=CARTESIAN_POINT('Origin',(112.247368755966,1.45439216225896E-14,
50.1045381897769));
#192460=CARTESIAN_POINT('Origin',(112.247368755966,1.45439216225896E-14,
50.1045381897769));
#192461=CARTESIAN_POINT('Origin',(119.628824814241,-0.799999999999986,64.5386069150778));
#192462=CARTESIAN_POINT('',(119.816516331414,-0.799999999999986,66.1934315167906));
#192463=CARTESIAN_POINT('',(119.754933813274,-0.799999999999986,66.5102445268161));
#192464=CARTESIAN_POINT('',(119.816516331414,-0.799999999999986,66.1934315167906));
#192465=CARTESIAN_POINT('',(119.289703096684,-0.799999999999986,66.283228202894));
#192466=CARTESIAN_POINT('Origin',(116.959178380441,-0.799999999999986,51.0204257716897));
#192467=CARTESIAN_POINT('',(119.228902537858,-0.799999999999986,66.5960184010664));
#192468=CARTESIAN_POINT('',(119.289703096684,-0.799999999999986,66.283228202894));
#192469=CARTESIAN_POINT('Origin',(116.959178380441,-0.799999999999986,51.0204257716897));
#192470=CARTESIAN_POINT('Origin',(120.11963831679,-0.799999999999986,64.6340118715271));
#192471=CARTESIAN_POINT('',(119.812861885554,-0.299999999999985,66.2122319170934));
#192472=CARTESIAN_POINT('',(119.751359652578,-0.299999999999985,66.5286318978187));
#192473=CARTESIAN_POINT('',(119.812861885554,-0.299999999999985,66.2122319170934));
#192474=CARTESIAN_POINT('Origin',(122.554452309506,1.45439216225896E-14,
52.1080422752111));
#192475=CARTESIAN_POINT('Origin',(122.554452309506,1.45439216225896E-14,
52.1080422752111));
#192476=CARTESIAN_POINT('Origin',(120.11963831679,-0.299999999999985,64.6340118715271));
#192477=CARTESIAN_POINT('',(119.286096015694,-0.299999999999985,66.3017849332873));
#192478=CARTESIAN_POINT('',(119.225372725718,-0.299999999999985,66.6141776196701));
#192479=CARTESIAN_POINT('',(119.286096015694,-0.299999999999985,66.3017849332873));
#192480=CARTESIAN_POINT('Origin',(116.959178380441,-0.299999999999985,51.0204257716897));
#192481=CARTESIAN_POINT('Origin',(116.959178380441,-0.299999999999985,51.0204257716897));
#192482=CARTESIAN_POINT('Origin',(119.628824814241,-0.299999999999985,64.5386069150778));
#192483=CARTESIAN_POINT('Origin',(122.063638806956,1.45439216225896E-14,
52.0126373187619));
#192484=CARTESIAN_POINT('Origin',(122.063638806956,1.45439216225896E-14,
52.0126373187619));
#192485=CARTESIAN_POINT('Origin',(119.628824814241,-1.8,64.5386069150778));
#192486=CARTESIAN_POINT('',(119.833858344817,-1.8,66.104215037305));
#192487=CARTESIAN_POINT('',(119.771891993661,-1.8,66.4230026871635));
#192488=CARTESIAN_POINT('',(119.833858344817,-1.8,66.104215037305));
#192489=CARTESIAN_POINT('',(119.306818641387,-1.8,66.195176798056));
#192490=CARTESIAN_POINT('Origin',(116.959178380441,-1.8,51.0204257716897));
#192491=CARTESIAN_POINT('',(119.245648775764,-1.8,66.5098669055141));
#192492=CARTESIAN_POINT('',(119.306818641387,-1.8,66.195176798056));
#192493=CARTESIAN_POINT('Origin',(116.959178380441,-1.8,51.0204257716897));
#192494=CARTESIAN_POINT('Origin',(120.11963831679,-1.8,64.6340118715271));
#192495=CARTESIAN_POINT('',(119.823506580252,-1.3,66.1574699835151));
#192496=CARTESIAN_POINT('',(119.761769913181,-1.3,66.475076017084));
#192497=CARTESIAN_POINT('',(119.823506580252,-1.3,66.1574699835151));
#192498=CARTESIAN_POINT('Origin',(122.554452309506,1.45439216225896E-14,
52.1080422752111));
#192499=CARTESIAN_POINT('Origin',(122.554452309506,1.45439216225896E-14,
52.1080422752111));
#192500=CARTESIAN_POINT('Origin',(120.11963831679,-1.3,64.6340118715271));
#192501=CARTESIAN_POINT('',(119.296602399404,-1.3,66.2477345445005));
#192502=CARTESIAN_POINT('',(119.235653504425,-1.3,66.5612878622158));
#192503=CARTESIAN_POINT('',(119.296602399404,-1.3,66.2477345445005));
#192504=CARTESIAN_POINT('Origin',(116.959178380441,-1.3,51.0204257716897));
#192505=CARTESIAN_POINT('Origin',(116.959178380441,-1.3,51.0204257716897));
#192506=CARTESIAN_POINT('Origin',(119.628824814241,-1.3,64.5386069150778));
#192507=CARTESIAN_POINT('Origin',(122.063638806956,1.45439216225896E-14,
52.0126373187619));
#192508=CARTESIAN_POINT('Origin',(122.063638806956,1.45439216225896E-14,
52.0126373187619));
#192509=CARTESIAN_POINT('Origin',(119.628824814241,-2.8,64.5386069150778));
#192510=CARTESIAN_POINT('',(119.86481427149,-2.8,65.9449613951417));
#192511=CARTESIAN_POINT('',(119.802150878674,-2.8,66.2673349955735));
#192512=CARTESIAN_POINT('',(119.86481427149,-2.8,65.9449613951417));
#192513=CARTESIAN_POINT('',(119.33736320091,-2.8,66.0380394458573));
#192514=CARTESIAN_POINT('Origin',(116.959178380441,-2.8,51.0204257716897));
#192515=CARTESIAN_POINT('',(119.27552312235,-2.8,66.3561774827635));
#192516=CARTESIAN_POINT('',(119.33736320091,-2.8,66.0380394458573));
#192517=CARTESIAN_POINT('Origin',(116.959178380441,-2.8,51.0204257716897));
#192518=CARTESIAN_POINT('Origin',(120.11963831679,-2.8,64.6340118715271));
#192519=CARTESIAN_POINT('',(119.847610191126,-2.3,66.0334682741935));
#192520=CARTESIAN_POINT('',(119.78533608868,-2.3,66.3538391592881));
#192521=CARTESIAN_POINT('',(119.847610191126,-2.3,66.0334682741935));
#192522=CARTESIAN_POINT('Origin',(122.554452309506,1.45439216225896E-14,
52.1080422752111));
#192523=CARTESIAN_POINT('Origin',(122.554452309506,1.45439216225896E-14,
52.1080422752111));
#192524=CARTESIAN_POINT('Origin',(120.11963831679,-2.3,64.6340118715271));
#192525=CARTESIAN_POINT('',(119.320388880605,-2.3,66.1253643177749));
#192526=CARTESIAN_POINT('',(119.258923037214,-2.3,66.4415770912459));
#192527=CARTESIAN_POINT('',(119.320388880605,-2.3,66.1253643177749));
#192528=CARTESIAN_POINT('Origin',(116.959178380441,-2.3,51.0204257716897));
#192529=CARTESIAN_POINT('Origin',(116.959178380441,-2.3,51.0204257716897));
#192530=CARTESIAN_POINT('Origin',(119.628824814241,-2.3,64.5386069150778));
#192531=CARTESIAN_POINT('Origin',(122.063638806956,1.45439216225896E-14,
52.0126373187619));
#192532=CARTESIAN_POINT('Origin',(122.063638806956,1.45439216225896E-14,
52.0126373187619));
#192533=CARTESIAN_POINT('Origin',(119.628824814241,-3.8,64.5386069150778));
#192534=CARTESIAN_POINT('',(119.909862136217,-3.8,65.7132113782478));
#192535=CARTESIAN_POINT('',(119.846156244582,-3.8,66.0409481433989));
#192536=CARTESIAN_POINT('',(119.909862136217,-3.8,65.7132113782478));
#192537=CARTESIAN_POINT('',(119.381795580881,-3.8,65.8094558077318));
#192538=CARTESIAN_POINT('Origin',(116.959178380441,-3.8,51.0204257716897));
#192539=CARTESIAN_POINT('',(119.318954220366,-3.8,66.1327449680392));
#192540=CARTESIAN_POINT('',(119.381795580881,-3.8,65.8094558077318));
#192541=CARTESIAN_POINT('Origin',(116.959178380441,-3.8,51.0204257716897));
#192542=CARTESIAN_POINT('Origin',(120.11963831679,-3.8,64.6340118715271));
#192543=CARTESIAN_POINT('',(119.885537345366,-3.3,65.8383509542256));
#192544=CARTESIAN_POINT('',(119.822398599122,-3.3,66.163170023844));
#192545=CARTESIAN_POINT('',(119.885537345366,-3.3,65.8383509542256));
#192546=CARTESIAN_POINT('Origin',(122.554452309506,1.45439216225896E-14,
52.1080422752111));
#192547=CARTESIAN_POINT('Origin',(122.554452309506,1.45439216225896E-14,
52.1080422752111));
#192548=CARTESIAN_POINT('Origin',(120.11963831679,-3.3,64.6340118715271));
#192549=CARTESIAN_POINT('',(119.357805665315,-3.3,65.9328726083199));
#192550=CARTESIAN_POINT('',(119.295508864014,-3.3,66.2533602683127));
#192551=CARTESIAN_POINT('',(119.357805665315,-3.3,65.9328726083199));
#192552=CARTESIAN_POINT('Origin',(116.959178380441,-3.3,51.0204257716897));
#192553=CARTESIAN_POINT('Origin',(116.959178380441,-3.3,51.0204257716897));
#192554=CARTESIAN_POINT('Origin',(119.628824814241,-3.3,64.5386069150778));
#192555=CARTESIAN_POINT('Origin',(122.063638806956,1.45439216225896E-14,
52.0126373187619));
#192556=CARTESIAN_POINT('Origin',(122.063638806956,1.45439216225896E-14,
52.0126373187619));
#192557=CARTESIAN_POINT('Origin',(118.647197809142,-3.8,64.3477970021793));
#192558=CARTESIAN_POINT('',(118.857589627268,-3.8,65.8858392622321));
#192559=CARTESIAN_POINT('',(118.795503721835,-3.8,66.2052419624567));
#192560=CARTESIAN_POINT('',(118.857589627268,-3.8,65.8858392622321));
#192561=CARTESIAN_POINT('',(118.337103376402,-3.8,65.9430866005239));
#192562=CARTESIAN_POINT('Origin',(116.959178380441,-3.8,51.0204257716897));
#192563=CARTESIAN_POINT('',(118.275673858067,-3.8,66.2591124987171));
#192564=CARTESIAN_POINT('',(118.337103376402,-3.8,65.9430866005239));
#192565=CARTESIAN_POINT('Origin',(116.959178380441,-3.8,51.0204257716897));
#192566=CARTESIAN_POINT('Origin',(119.138011311691,-3.8,64.4432019586286));
#192567=CARTESIAN_POINT('',(118.833892175693,-3.3,66.0077514735275));
#192568=CARTESIAN_POINT('',(118.77233158469,-3.3,66.3244516787764));
#192569=CARTESIAN_POINT('',(118.833892175693,-3.3,66.0077514735275));
#192570=CARTESIAN_POINT('Origin',(121.572825304407,1.45439216225896E-14,
51.9172323623126));
#192571=CARTESIAN_POINT('Origin',(121.572825304407,1.45439216225896E-14,
51.9172323623126));
#192572=CARTESIAN_POINT('Origin',(119.138011311691,-3.3,64.4432019586286));
#192573=CARTESIAN_POINT('',(118.313659915754,-3.3,66.0636921482939));
#192574=CARTESIAN_POINT('',(118.252739359001,-3.3,66.3770996792034));
#192575=CARTESIAN_POINT('',(118.313659915754,-3.3,66.0636921482939));
#192576=CARTESIAN_POINT('Origin',(116.959178380441,-3.3,51.0204257716897));
#192577=CARTESIAN_POINT('Origin',(116.959178380441,-3.3,51.0204257716897));
#192578=CARTESIAN_POINT('Origin',(118.647197809142,-3.3,64.3477970021793));
#192579=CARTESIAN_POINT('Origin',(121.082011801857,1.45439216225896E-14,
51.8218274058634));
#192580=CARTESIAN_POINT('Origin',(121.082011801857,1.45439216225896E-14,
51.8218274058634));
#192581=CARTESIAN_POINT('Origin',(117.665570804043,-3.8,64.1569870892808));
#192582=CARTESIAN_POINT('',(117.820217329609,-3.8,65.9818125869175));
#192583=CARTESIAN_POINT('',(117.759353330908,-3.8,66.2949291533247));
#192584=CARTESIAN_POINT('',(117.820217329609,-3.8,65.9818125869175));
#192585=CARTESIAN_POINT('',(117.306830681782,-3.8,66.0025358161473));
#192586=CARTESIAN_POINT('Origin',(116.959178380441,-3.8,51.0204257716897));
#192587=CARTESIAN_POINT('',(117.246448044845,-3.8,66.3131760033177));
#192588=CARTESIAN_POINT('',(117.306830681782,-3.8,66.0025358161473));
#192589=CARTESIAN_POINT('Origin',(116.959178380441,-3.8,51.0204257716897));
#192590=CARTESIAN_POINT('Origin',(118.156384306592,-3.8,64.25239204573));
#192591=CARTESIAN_POINT('',(117.796992609744,-3.3,66.1012928165323));
#192592=CARTESIAN_POINT('',(117.736623755491,-3.3,66.4118620982908));
#192593=CARTESIAN_POINT('',(117.796992609744,-3.3,66.1012928165323));
#192594=CARTESIAN_POINT('Origin',(120.591198299308,1.45439216225896E-14,
51.7264224494141));
#192595=CARTESIAN_POINT('Origin',(120.591198299308,1.45439216225896E-14,
51.7264224494141));
#192596=CARTESIAN_POINT('Origin',(118.156384306592,-3.3,64.25239204573));
#192597=CARTESIAN_POINT('',(117.283792086681,-3.3,66.1210585216364));
#192598=CARTESIAN_POINT('',(117.223893029854,-3.3,66.4292109172233));
#192599=CARTESIAN_POINT('',(117.283792086681,-3.3,66.1210585216364));
#192600=CARTESIAN_POINT('Origin',(116.959178380441,-3.3,51.0204257716897));
#192601=CARTESIAN_POINT('Origin',(116.959178380441,-3.3,51.0204257716897));
#192602=CARTESIAN_POINT('Origin',(117.665570804043,-3.3,64.1569870892808));
#192603=CARTESIAN_POINT('Origin',(120.100384796758,1.45439216225896E-14,
51.6310174929649));
#192604=CARTESIAN_POINT('Origin',(120.100384796758,1.45439216225896E-14,
51.6310174929649));
#192605=CARTESIAN_POINT('Origin',(116.683943798944,-3.8,63.9661771763823));
#192606=CARTESIAN_POINT('',(116.796859179409,-3.8,66.0056897327932));
#192607=CARTESIAN_POINT('',(116.7368792064,-3.8,66.3142584039699));
#192608=CARTESIAN_POINT('',(116.796859179409,-3.8,66.0056897327932));
#192609=CARTESIAN_POINT('',(116.290233427834,-3.8,65.9916313396271));
#192610=CARTESIAN_POINT('Origin',(116.959178380441,-3.8,51.0204257716897));
#192611=CARTESIAN_POINT('',(116.230581815828,-3.8,66.2985107483171));
#192612=CARTESIAN_POINT('',(116.290233427834,-3.8,65.9916313396271));
#192613=CARTESIAN_POINT('Origin',(116.959178380441,-3.8,51.0204257716897));
#192614=CARTESIAN_POINT('Origin',(117.174757301493,-3.8,64.0615821328315));
#192615=CARTESIAN_POINT('',(116.773976234632,-3.3,66.1234116907773));
#192616=CARTESIAN_POINT('',(116.7144703059,-3.3,66.4295416277397));
#192617=CARTESIAN_POINT('',(116.773976234632,-3.3,66.1234116907773));
#192618=CARTESIAN_POINT('Origin',(119.609571294209,1.45439216225896E-14,
51.5356125365156));
#192619=CARTESIAN_POINT('Origin',(119.609571294209,1.45439216225896E-14,
51.5356125365156));
#192620=CARTESIAN_POINT('Origin',(117.174757301493,-3.3,64.0615821328315));
#192621=CARTESIAN_POINT('',(116.267477381404,-3.3,66.108700465472));
#192622=CARTESIAN_POINT('',(116.20829212986,-3.3,66.413180669547));
#192623=CARTESIAN_POINT('',(116.267477381404,-3.3,66.108700465472));
#192624=CARTESIAN_POINT('Origin',(116.959178380441,-3.3,51.0204257716897));
#192625=CARTESIAN_POINT('Origin',(116.959178380441,-3.3,51.0204257716897));
#192626=CARTESIAN_POINT('Origin',(116.683943798944,-3.3,63.9661771763823));
#192627=CARTESIAN_POINT('Origin',(119.118757791659,1.45439216225896E-14,
51.4402075800664));
#192628=CARTESIAN_POINT('Origin',(119.118757791659,1.45439216225896E-14,
51.4402075800664));
#192629=CARTESIAN_POINT('Origin',(115.702316793845,-3.8,63.7753672634838));
#192630=CARTESIAN_POINT('',(115.786897562756,-3.8,65.9606480321323));
#192631=CARTESIAN_POINT('',(115.727503479173,-3.8,66.2662025785505));
#192632=CARTESIAN_POINT('',(115.786897562756,-3.8,65.9606480321323));
#192633=CARTESIAN_POINT('',(115.286808223328,-3.8,65.9129628814135));
#192634=CARTESIAN_POINT('Origin',(116.959178380441,-3.8,51.0204257716897));
#192635=CARTESIAN_POINT('',(115.227603487308,-3.8,66.2175433239276));
#192636=CARTESIAN_POINT('',(115.286808223328,-3.8,65.9129628814135));
#192637=CARTESIAN_POINT('Origin',(116.959178380441,-3.8,51.0204257716897));
#192638=CARTESIAN_POINT('Origin',(116.193130296394,-3.8,63.870772219933));
#192639=CARTESIAN_POINT('',(115.764241021926,-3.3,66.0772052485936));
#192640=CARTESIAN_POINT('',(115.705307330283,-3.3,66.3803912956307));
#192641=CARTESIAN_POINT('',(115.764241021926,-3.3,66.0772052485936));
#192642=CARTESIAN_POINT('Origin',(118.62794428911,1.45439216225896E-14,
51.3448026236171));
#192643=CARTESIAN_POINT('Origin',(118.62794428911,1.45439216225896E-14,
51.3448026236171));
#192644=CARTESIAN_POINT('Origin',(116.193130296394,-3.3,63.870772219933));
#192645=CARTESIAN_POINT('',(115.264224833413,-3.3,66.0291437709213));
#192646=CARTESIAN_POINT('',(115.205476133255,-3.3,66.3313781240196));
#192647=CARTESIAN_POINT('',(115.264224833413,-3.3,66.0291437709213));
#192648=CARTESIAN_POINT('Origin',(116.959178380441,-3.3,51.0204257716897));
#192649=CARTESIAN_POINT('Origin',(116.959178380441,-3.3,51.0204257716897));
#192650=CARTESIAN_POINT('Origin',(115.702316793845,-3.3,63.7753672634838));
#192651=CARTESIAN_POINT('Origin',(118.13713078656,1.45439216225896E-14,
51.2493976671679));
#192652=CARTESIAN_POINT('Origin',(118.13713078656,1.45439216225896E-14,
51.2493976671679));
#192653=CARTESIAN_POINT('Origin',(114.720689788746,-3.8,63.5845573505853));
#192654=CARTESIAN_POINT('',(114.789933781015,-3.8,65.8487386013644));
#192655=CARTESIAN_POINT('',(114.730852122701,-3.8,66.1526858671318));
#192656=CARTESIAN_POINT('',(114.789933781015,-3.8,65.8487386013644));
#192657=CARTESIAN_POINT('',(114.296253791258,-3.8,65.7680803695982));
#192658=CARTESIAN_POINT('Origin',(116.959178380441,-3.8,51.0204257716897));
#192659=CARTESIAN_POINT('',(114.237230165589,-3.8,66.0717290847811));
#192660=CARTESIAN_POINT('',(114.296253791258,-3.8,65.7680803695982));
#192661=CARTESIAN_POINT('Origin',(116.959178380441,-3.8,51.0204257716897));
#192662=CARTESIAN_POINT('Origin',(115.211503291295,-3.8,63.6799623070345));
#192663=CARTESIAN_POINT('',(114.767397935133,-3.3,65.9646748992444));
#192664=CARTESIAN_POINT('',(114.70876949581,-3.3,66.2662905670707));
#192665=CARTESIAN_POINT('',(114.767397935133,-3.3,65.9646748992444));
#192666=CARTESIAN_POINT('Origin',(117.64631728401,1.45439216225896E-14,
51.1539927107186));
#192667=CARTESIAN_POINT('Origin',(117.64631728401,1.45439216225896E-14,
51.1539927107186));
#192668=CARTESIAN_POINT('Origin',(115.211503291295,-3.3,63.6799623070345));
#192669=CARTESIAN_POINT('',(114.273740361672,-3.3,65.8839013462125));
#192670=CARTESIAN_POINT('',(114.215168630795,-3.3,66.185225275828));
#192671=CARTESIAN_POINT('',(114.273740361672,-3.3,65.8839013462125));
#192672=CARTESIAN_POINT('Origin',(116.959178380441,-3.3,51.0204257716897));
#192673=CARTESIAN_POINT('Origin',(116.959178380441,-3.3,51.0204257716897));
#192674=CARTESIAN_POINT('Origin',(114.720689788746,-3.3,63.5845573505853));
#192675=CARTESIAN_POINT('Origin',(117.155503781461,1.45439216225896E-14,
51.0585877542694));
#192676=CARTESIAN_POINT('Origin',(117.155503781461,1.45439216225896E-14,
51.0585877542694));
#192677=CARTESIAN_POINT('Origin',(113.739062783647,-3.8,63.3937474376868));
#192678=CARTESIAN_POINT('',(113.805758645357,-3.8,65.6710376183478));
#192679=CARTESIAN_POINT('',(113.746728580063,-3.8,65.9747194623623));
#192680=CARTESIAN_POINT('',(113.805758645357,-3.8,65.6710376183478));
#192681=CARTESIAN_POINT('',(113.318449408565,-3.8,65.5576048673859));
#192682=CARTESIAN_POINT('Origin',(116.959178380441,-3.8,51.0204257716897));
#192683=CARTESIAN_POINT('',(113.259348367962,-3.8,65.8616518458919));
#192684=CARTESIAN_POINT('',(113.318449408565,-3.8,65.5576048673859));
#192685=CARTESIAN_POINT('Origin',(116.959178380441,-3.8,51.0204257716897));
#192686=CARTESIAN_POINT('Origin',(114.229876286196,-3.8,63.489152394136));
#192687=CARTESIAN_POINT('',(113.783242728376,-3.3,65.7868713914321));
#192688=CARTESIAN_POINT('',(113.724664704686,-3.3,66.0882276946056));
#192689=CARTESIAN_POINT('',(113.783242728376,-3.3,65.7868713914321));
#192690=CARTESIAN_POINT('Origin',(116.664690278911,1.45439216225896E-14,
50.9631827978201));
#192691=CARTESIAN_POINT('Origin',(116.664690278911,1.45439216225896E-14,
50.9631827978201));
#192692=CARTESIAN_POINT('Origin',(114.229876286196,-3.3,63.489152394136));
#192693=CARTESIAN_POINT('',(113.295906075692,-3.3,65.6735796823071));
#192694=CARTESIAN_POINT('',(113.237258696916,-3.3,65.9752927846826));
#192695=CARTESIAN_POINT('',(113.295906075692,-3.3,65.6735796823071));
#192696=CARTESIAN_POINT('Origin',(116.959178380441,-3.3,51.0204257716897));
#192697=CARTESIAN_POINT('Origin',(116.959178380441,-3.3,51.0204257716897));
#192698=CARTESIAN_POINT('Origin',(113.739062783647,-3.3,63.3937474376868));
#192699=CARTESIAN_POINT('Origin',(116.173876776362,1.45439216225896E-14,
50.8677778413709));
#192700=CARTESIAN_POINT('Origin',(116.173876776362,1.45439216225896E-14,
50.8677778413709));
#192701=CARTESIAN_POINT('Origin',(112.757435778548,-3.8,63.2029375247883));
#192702=CARTESIAN_POINT('',(112.834337837981,-3.8,65.4277216319878));
#192703=CARTESIAN_POINT('',(112.775100585027,-3.8,65.732469358792));
#192704=CARTESIAN_POINT('',(112.834337837981,-3.8,65.4277216319878));
#192705=CARTESIAN_POINT('',(112.353446580952,-3.8,65.2812714022259));
#192706=CARTESIAN_POINT('Origin',(116.959178380441,-3.8,51.0204257716897));
#192707=CARTESIAN_POINT('',(112.294006519922,-3.8,65.5870624809277));
#192708=CARTESIAN_POINT('',(112.353446580952,-3.8,65.2812714022259));
#192709=CARTESIAN_POINT('Origin',(116.959178380441,-3.8,51.0204257716897));
#192710=CARTESIAN_POINT('Origin',(113.248249281097,-3.8,63.2983424812375));
#192711=CARTESIAN_POINT('',(112.811741886383,-3.3,65.5439671454273));
#192712=CARTESIAN_POINT('',(112.752961415424,-3.3,65.8463649443104));
#192713=CARTESIAN_POINT('',(112.811741886383,-3.3,65.5439671454273));
#192714=CARTESIAN_POINT('Origin',(115.683063273812,1.45439216225896E-14,
50.7723728849216));
#192715=CARTESIAN_POINT('Origin',(115.683063273812,1.45439216225896E-14,
50.7723728849216));
#192716=CARTESIAN_POINT('Origin',(113.248249281097,-3.3,63.2983424812375));
#192717=CARTESIAN_POINT('',(112.330772276248,-3.3,65.3979200054423));
#192718=CARTESIAN_POINT('',(112.271793669026,-3.3,65.7013371219498));
#192719=CARTESIAN_POINT('',(112.330772276248,-3.3,65.3979200054423));
#192720=CARTESIAN_POINT('Origin',(116.959178380441,-3.3,51.0204257716897));
#192721=CARTESIAN_POINT('Origin',(116.959178380441,-3.3,51.0204257716897));
#192722=CARTESIAN_POINT('Origin',(112.757435778548,-3.3,63.2029375247883));
#192723=CARTESIAN_POINT('Origin',(115.192249771263,1.45439216225896E-14,
50.6769679284724));
#192724=CARTESIAN_POINT('Origin',(115.192249771263,1.45439216225896E-14,
50.6769679284724));
#192725=CARTESIAN_POINT('Origin',(111.775808773449,-3.8,63.0121276118898));
#192726=CARTESIAN_POINT('',(111.875809561864,-3.8,65.1180796531428));
#192727=CARTESIAN_POINT('',(111.816098042946,-3.8,65.425267254645));
#192728=CARTESIAN_POINT('',(111.875809561864,-3.8,65.1180796531428));
#192729=CARTESIAN_POINT('',(111.401472572927,-3.8,64.9379108054185));
#192730=CARTESIAN_POINT('Origin',(116.959178380441,-3.8,51.0204257716897));
#192731=CARTESIAN_POINT('',(111.341418137912,-3.8,65.2468625484944));
#192732=CARTESIAN_POINT('',(111.401472572927,-3.8,64.9379108054185));
#192733=CARTESIAN_POINT('Origin',(116.959178380441,-3.8,51.0204257716897));
#192734=CARTESIAN_POINT('Origin',(112.266622275998,-3.8,63.107532568339));
#192735=CARTESIAN_POINT('',(111.853030365824,-3.3,65.2352678728129));
#192736=CARTESIAN_POINT('',(111.79378660305,-3.3,65.5400490895696));
#192737=CARTESIAN_POINT('',(111.853030365824,-3.3,65.2352678728129));
#192738=CARTESIAN_POINT('Origin',(114.701436268713,1.45439216225896E-14,
50.5815629720231));
#192739=CARTESIAN_POINT('Origin',(114.701436268713,1.45439216225896E-14,
50.5815629720231));
#192740=CARTESIAN_POINT('Origin',(112.266622275998,-3.3,63.107532568339));
#192741=CARTESIAN_POINT('',(111.378560847823,-3.3,65.0557808246087));
#192742=CARTESIAN_POINT('',(111.318982211057,-3.3,65.3622848101095));
#192743=CARTESIAN_POINT('',(111.378560847823,-3.3,65.0557808246087));
#192744=CARTESIAN_POINT('Origin',(116.959178380441,-3.3,51.0204257716897));
#192745=CARTESIAN_POINT('Origin',(116.959178380441,-3.3,51.0204257716897));
#192746=CARTESIAN_POINT('Origin',(111.775808773449,-3.3,63.0121276118898));
#192747=CARTESIAN_POINT('Origin',(114.210622766164,1.45439216225896E-14,
50.4861580155739));
#192748=CARTESIAN_POINT('Origin',(114.210622766164,1.45439216225896E-14,
50.4861580155739));
#192749=CARTESIAN_POINT('Origin',(110.79418176835,-3.8,62.8213176989913));
#192750=CARTESIAN_POINT('',(110.930494093462,-3.8,64.7404640105189));
#192751=CARTESIAN_POINT('',(110.87002163836,-3.8,65.0515662697813));
#192752=CARTESIAN_POINT('',(110.930494093462,-3.8,64.7404640105189));
#192753=CARTESIAN_POINT('',(110.462946372987,-3.8,64.5253675787552));
#192754=CARTESIAN_POINT('Origin',(116.959178380441,-3.8,51.0204257716897));
#192755=CARTESIAN_POINT('',(110.401976198362,-3.8,64.8390303702136));
#192756=CARTESIAN_POINT('',(110.462946372987,-3.8,64.5253675787552));
#192757=CARTESIAN_POINT('Origin',(116.959178380441,-3.8,51.0204257716897));
#192758=CARTESIAN_POINT('Origin',(111.284995270899,-3.8,62.9167226554405));
#192759=CARTESIAN_POINT('',(110.907420773452,-3.3,64.8591653592831));
#192760=CARTESIAN_POINT('',(110.847434042615,-3.3,65.1677687963017));
#192761=CARTESIAN_POINT('',(110.907420773452,-3.3,64.8591653592831));
#192762=CARTESIAN_POINT('Origin',(113.719809263614,1.45439216225896E-14,
50.3907530591246));
#192763=CARTESIAN_POINT('Origin',(113.719809263614,1.45439216225896E-14,
50.3907530591246));
#192764=CARTESIAN_POINT('Origin',(111.284995270899,-3.3,62.9167226554405));
#192765=CARTESIAN_POINT('',(110.439680590912,-3.3,64.6450590540696));
#192766=CARTESIAN_POINT('',(110.379208135811,-3.3,64.956161313332));
#192767=CARTESIAN_POINT('',(110.439680590912,-3.3,64.6450590540696));
#192768=CARTESIAN_POINT('Origin',(116.959178380441,-3.3,51.0204257716897));
#192769=CARTESIAN_POINT('Origin',(116.959178380441,-3.3,51.0204257716897));
#192770=CARTESIAN_POINT('Origin',(110.79418176835,-3.3,62.8213176989913));
#192771=CARTESIAN_POINT('Origin',(113.228995761065,1.45439216225896E-14,
50.2953481026754));
#192772=CARTESIAN_POINT('Origin',(113.228995761065,1.45439216225896E-14,
50.2953481026754));
#192773=CARTESIAN_POINT('Origin',(110.79418176835,-2.8,62.8213176989913));
#192774=CARTESIAN_POINT('',(110.887747345274,-2.8,64.9603758681595));
#192775=CARTESIAN_POINT('',(110.828168708508,-2.8,65.2668798536603));
#192776=CARTESIAN_POINT('',(110.887747345274,-2.8,64.9603758681595));
#192777=CARTESIAN_POINT('',(110.419845567828,-2.8,64.74710089252));
#192778=CARTESIAN_POINT('Origin',(116.959178380441,-2.8,51.0204257716897));
#192779=CARTESIAN_POINT('',(110.359791132813,-2.8,65.0560526355959));
#192780=CARTESIAN_POINT('',(110.419845567828,-2.8,64.74710089252));
#192781=CARTESIAN_POINT('Origin',(116.959178380441,-2.8,51.0204257716897));
#192782=CARTESIAN_POINT('Origin',(111.284995270899,-2.8,62.9167226554405));
#192783=CARTESIAN_POINT('',(110.871403360725,-2.3,65.0444579599144));
#192784=CARTESIAN_POINT('',(110.812159597951,-2.3,65.3492391766711));
#192785=CARTESIAN_POINT('',(110.871403360725,-2.3,65.0444579599144));
#192786=CARTESIAN_POINT('Origin',(113.719809263614,1.45439216225896E-14,
50.3907530591246));
#192787=CARTESIAN_POINT('Origin',(113.719809263614,1.45439216225896E-14,
50.3907530591246));
#192788=CARTESIAN_POINT('Origin',(111.284995270899,-2.3,62.9167226554405));
#192789=CARTESIAN_POINT('',(110.403369054216,-2.3,64.8318647837951));
#192790=CARTESIAN_POINT('',(110.343657535297,-2.3,65.1390523852972));
#192791=CARTESIAN_POINT('',(110.403369054216,-2.3,64.8318647837951));
#192792=CARTESIAN_POINT('Origin',(116.959178380441,-2.3,51.0204257716897));
#192793=CARTESIAN_POINT('Origin',(116.959178380441,-2.3,51.0204257716897));
#192794=CARTESIAN_POINT('Origin',(110.79418176835,-2.3,62.8213176989913));
#192795=CARTESIAN_POINT('Origin',(113.228995761065,1.45439216225896E-14,
50.2953481026754));
#192796=CARTESIAN_POINT('Origin',(113.228995761065,1.45439216225896E-14,
50.2953481026754));
#192797=CARTESIAN_POINT('Origin',(110.79418176835,-1.8,62.8213176989913));
#192798=CARTESIAN_POINT('',(110.8583317686,-1.8,65.1117051360946));
#192799=CARTESIAN_POINT('',(110.799353161377,-1.8,65.4151222526021));
#192800=CARTESIAN_POINT('',(110.8583317686,-1.8,65.1117051360946));
#192801=CARTESIAN_POINT('',(110.390192570754,-1.8,64.8996515764289));
#192802=CARTESIAN_POINT('Origin',(116.959178380441,-1.8,51.0204257716897));
#192803=CARTESIAN_POINT('',(110.330752509724,-1.8,65.2054426551307));
#192804=CARTESIAN_POINT('',(110.390192570754,-1.8,64.8996515764289));
#192805=CARTESIAN_POINT('Origin',(116.959178380441,-1.8,51.0204257716897));
#192806=CARTESIAN_POINT('Origin',(111.284995270899,-1.8,62.9167226554405));
#192807=CARTESIAN_POINT('',(110.848487876185,-1.3,65.1623473196303));
#192808=CARTESIAN_POINT('',(110.789707405226,-1.3,65.4647451185134));
#192809=CARTESIAN_POINT('',(110.848487876185,-1.3,65.1623473196303));
#192810=CARTESIAN_POINT('Origin',(113.719809263614,1.45439216225896E-14,
50.3907530591246));
#192811=CARTESIAN_POINT('Origin',(113.719809263614,1.45439216225896E-14,
50.3907530591246));
#192812=CARTESIAN_POINT('Origin',(111.284995270899,-1.3,62.9167226554405));
#192813=CARTESIAN_POINT('',(110.380270325233,-1.3,64.9506968497415));
#192814=CARTESIAN_POINT('',(110.321033072279,-1.3,65.2554445765457));
#192815=CARTESIAN_POINT('',(110.380270325233,-1.3,64.9506968497415));
#192816=CARTESIAN_POINT('Origin',(116.959178380441,-1.3,51.0204257716897));
#192817=CARTESIAN_POINT('Origin',(116.959178380441,-1.3,51.0204257716897));
#192818=CARTESIAN_POINT('Origin',(110.79418176835,-1.3,62.8213176989913));
#192819=CARTESIAN_POINT('Origin',(113.228995761065,1.45439216225896E-14,
50.2953481026754));
#192820=CARTESIAN_POINT('Origin',(113.228995761065,1.45439216225896E-14,
50.2953481026754));
#192821=CARTESIAN_POINT('Origin',(111.284995270899,-0.799999999999986,62.9167226554405));
#192822=CARTESIAN_POINT('',(110.838361713079,-0.299999999999985,65.2144416527366));
#192823=CARTESIAN_POINT('',(110.779783689389,-0.299999999999985,65.51579795591));
#192824=CARTESIAN_POINT('',(110.838361713079,-0.299999999999985,65.2144416527366));
#192825=CARTESIAN_POINT('',(110.841838562944,-0.799999999999986,65.1965549000608));
#192826=CARTESIAN_POINT('Origin',(113.719809263614,1.45439216225896E-14,
50.3907530591246));
#192827=CARTESIAN_POINT('',(110.783191184168,-0.799999999999986,65.4982680024364));
#192828=CARTESIAN_POINT('',(110.841838562944,-0.799999999999986,65.1965549000608));
#192829=CARTESIAN_POINT('Origin',(113.719809263614,1.45439216225896E-14,
50.3907530591246));
#192830=CARTESIAN_POINT('Origin',(111.284995270899,-0.299999999999985,62.9167226554405));
#192831=CARTESIAN_POINT('',(110.370064127511,-0.299999999999985,65.003202923203));
#192832=CARTESIAN_POINT('',(110.311034062217,-0.299999999999985,65.3068847672175));
#192833=CARTESIAN_POINT('',(110.370064127511,-0.299999999999985,65.003202923203));
#192834=CARTESIAN_POINT('Origin',(116.959178380441,-0.299999999999985,51.0204257716897));
#192835=CARTESIAN_POINT('Origin',(116.959178380441,-0.299999999999985,51.0204257716897));
#192836=CARTESIAN_POINT('Origin',(110.79418176835,-0.299999999999985,62.8213176989913));
#192837=CARTESIAN_POINT('',(110.373568393268,-0.799999999999986,64.9851751286904));
#192838=CARTESIAN_POINT('',(110.314467352665,-0.799999999999986,65.2892221071964));
#192839=CARTESIAN_POINT('',(110.373568393268,-0.799999999999986,64.9851751286904));
#192840=CARTESIAN_POINT('Origin',(113.228995761065,1.45439216225896E-14,
50.2953481026754));
#192841=CARTESIAN_POINT('Origin',(113.228995761065,1.45439216225896E-14,
50.2953481026754));
#192842=CARTESIAN_POINT('Origin',(110.79418176835,-0.799999999999986,62.8213176989913));
#192843=CARTESIAN_POINT('Origin',(116.959178380441,-0.799999999999986,51.0204257716897));
#192844=CARTESIAN_POINT('Origin',(116.959178380441,-0.799999999999986,51.0204257716897));
#192845=CARTESIAN_POINT('Origin',(118.647197809142,-0.799999999999986,64.3477970021793));
#192846=CARTESIAN_POINT('',(118.766592773437,-0.799999999999986,66.3539751559262));
#192847=CARTESIAN_POINT('',(118.706477208223,-0.799999999999986,66.6632413850446));
#192848=CARTESIAN_POINT('',(118.766592773437,-0.799999999999986,66.3539751559262));
#192849=CARTESIAN_POINT('',(118.247058804081,-0.799999999999986,66.4063234549974));
#192850=CARTESIAN_POINT('Origin',(116.959178380441,-0.799999999999986,51.0204257716897));
#192851=CARTESIAN_POINT('',(118.187539675506,-0.799999999999986,66.7125212989234));
#192852=CARTESIAN_POINT('',(118.247058804081,-0.799999999999986,66.4063234549974));
#192853=CARTESIAN_POINT('Origin',(116.959178380441,-0.799999999999986,51.0204257716897));
#192854=CARTESIAN_POINT('Origin',(119.138011311691,-0.799999999999986,64.4432019586286));
#192855=CARTESIAN_POINT('',(118.763027153213,-0.299999999999985,66.3723185902268));
#192856=CARTESIAN_POINT('',(118.702986277376,-0.299999999999985,66.6812005777294));
#192857=CARTESIAN_POINT('',(118.763027153213,-0.299999999999985,66.3723185902268));
#192858=CARTESIAN_POINT('Origin',(121.572825304407,1.45439216225896E-14,
51.9172323623126));
#192859=CARTESIAN_POINT('Origin',(121.572825304407,1.45439216225896E-14,
51.9172323623126));
#192860=CARTESIAN_POINT('Origin',(119.138011311691,-0.299999999999985,64.4432019586286));
#192861=CARTESIAN_POINT('',(118.243529261453,-0.299999999999985,66.4244812870825));
#192862=CARTESIAN_POINT('',(118.184082623495,-0.299999999999985,66.7303062009751));
#192863=CARTESIAN_POINT('',(118.243529261453,-0.299999999999985,66.4244812870825));
#192864=CARTESIAN_POINT('Origin',(116.959178380441,-0.299999999999985,51.0204257716897));
#192865=CARTESIAN_POINT('Origin',(116.959178380441,-0.299999999999985,51.0204257716897));
#192866=CARTESIAN_POINT('Origin',(118.647197809142,-0.299999999999985,64.3477970021793));
#192867=CARTESIAN_POINT('Origin',(121.082011801857,1.45439216225896E-14,
51.8218274058634));
#192868=CARTESIAN_POINT('Origin',(121.082011801857,1.45439216225896E-14,
51.8218274058634));
#192869=CARTESIAN_POINT('Origin',(118.647197809142,-1.8,64.3477970021793));
#192870=CARTESIAN_POINT('',(118.783510134254,-1.8,66.2669433137069));
#192871=CARTESIAN_POINT('',(118.723037679152,-1.8,66.5780455729693));
#192872=CARTESIAN_POINT('',(118.783510134254,-1.8,66.2669433137069));
#192873=CARTESIAN_POINT('',(118.263803754148,-1.8,66.3201785847698));
#192874=CARTESIAN_POINT('Origin',(116.959178380441,-1.8,51.0204257716897));
#192875=CARTESIAN_POINT('',(118.203938315861,-1.8,66.6281580288199));
#192876=CARTESIAN_POINT('',(118.263803754148,-1.8,66.3201785847698));
#192877=CARTESIAN_POINT('Origin',(116.959178380441,-1.8,51.0204257716897));
#192878=CARTESIAN_POINT('Origin',(119.138011311691,-1.8,64.4432019586286));
#192879=CARTESIAN_POINT('',(118.773412477781,-1.3,66.3188909936332));
#192880=CARTESIAN_POINT('',(118.713153546234,-1.3,66.6288947749162));
#192881=CARTESIAN_POINT('',(118.773412477781,-1.3,66.3188909936332));
#192882=CARTESIAN_POINT('Origin',(121.572825304407,1.45439216225896E-14,
51.9172323623126));
#192883=CARTESIAN_POINT('Origin',(121.572825304407,1.45439216225896E-14,
51.9172323623126));
#192884=CARTESIAN_POINT('Origin',(119.138011311691,-1.3,64.4432019586286));
#192885=CARTESIAN_POINT('',(118.253809253311,-1.3,66.3715955776028));
#192886=CARTESIAN_POINT('',(118.194150993884,-1.3,66.6785091841359));
#192887=CARTESIAN_POINT('',(118.253809253311,-1.3,66.3715955776028));
#192888=CARTESIAN_POINT('Origin',(116.959178380441,-1.3,51.0204257716897));
#192889=CARTESIAN_POINT('Origin',(116.959178380441,-1.3,51.0204257716897));
#192890=CARTESIAN_POINT('Origin',(118.647197809142,-1.3,64.3477970021793));
#192891=CARTESIAN_POINT('Origin',(121.082011801857,1.45439216225896E-14,
51.8218274058634));
#192892=CARTESIAN_POINT('Origin',(121.082011801857,1.45439216225896E-14,
51.8218274058634));
#192893=CARTESIAN_POINT('Origin',(118.647197809142,-2.8,64.3477970021793));
#192894=CARTESIAN_POINT('',(118.813694939004,-2.8,66.1116567301338));
#192895=CARTESIAN_POINT('',(118.752575180056,-2.8,66.4260890623797));
#192896=CARTESIAN_POINT('',(118.813694939004,-2.8,66.1116567301338));
#192897=CARTESIAN_POINT('',(118.293675764896,-2.8,66.1665011788025));
#192898=CARTESIAN_POINT('Origin',(116.959178380441,-2.8,51.0204257716897));
#192899=CARTESIAN_POINT('',(118.233182525534,-2.8,66.4777103632785));
#192900=CARTESIAN_POINT('',(118.293675764896,-2.8,66.1665011788025));
#192901=CARTESIAN_POINT('Origin',(116.959178380441,-2.8,51.0204257716897));
#192902=CARTESIAN_POINT('Origin',(119.138011311691,-2.8,64.4432019586286));
#192903=CARTESIAN_POINT('',(118.796921514364,-2.3,66.1979480886086));
#192904=CARTESIAN_POINT('',(118.736163138728,-2.3,66.5105212741601));
#192905=CARTESIAN_POINT('',(118.796921514364,-2.3,66.1979480886086));
#192906=CARTESIAN_POINT('Origin',(121.572825304407,1.45439216225896E-14,
51.9172323623126));
#192907=CARTESIAN_POINT('Origin',(121.572825304407,1.45439216225896E-14,
51.9172323623126));
#192908=CARTESIAN_POINT('Origin',(119.138011311691,-2.3,64.4432019586286));
#192909=CARTESIAN_POINT('',(118.277076983843,-2.3,66.2518940783944));
#192910=CARTESIAN_POINT('',(118.216934189658,-2.3,66.5613003877282));
#192911=CARTESIAN_POINT('',(118.277076983843,-2.3,66.2518940783944));
#192912=CARTESIAN_POINT('Origin',(116.959178380441,-2.3,51.0204257716897));
#192913=CARTESIAN_POINT('Origin',(116.959178380441,-2.3,51.0204257716897));
#192914=CARTESIAN_POINT('Origin',(118.647197809142,-2.3,64.3477970021793));
#192915=CARTESIAN_POINT('Origin',(121.082011801857,1.45439216225896E-14,
51.8218274058634));
#192916=CARTESIAN_POINT('Origin',(121.082011801857,1.45439216225896E-14,
51.8218274058634));
#192917=CARTESIAN_POINT('Origin',(117.665570804043,-2.8,64.1569870892808));
#192918=CARTESIAN_POINT('',(117.777192058143,-2.8,66.2031573154554));
#192919=CARTESIAN_POINT('',(117.717239093625,-2.8,66.5115870406867));
#192920=CARTESIAN_POINT('',(117.777192058143,-2.8,66.2031573154554));
#192921=CARTESIAN_POINT('',(117.264147820731,-2.8,66.2221190045997));
#192922=CARTESIAN_POINT('Origin',(116.959178380441,-2.8,51.0204257716897));
#192923=CARTESIAN_POINT('',(117.20465508306,-2.8,66.5281810797731));
#192924=CARTESIAN_POINT('',(117.264147820731,-2.8,66.2221190045997));
#192925=CARTESIAN_POINT('Origin',(116.959178380441,-2.8,51.0204257716897));
#192926=CARTESIAN_POINT('Origin',(118.156384306592,-2.8,64.25239204573));
#192927=CARTESIAN_POINT('',(117.760743812198,-2.3,66.2877757829205));
#192928=CARTESIAN_POINT('',(117.701132038091,-2.3,66.5944502444126));
#192929=CARTESIAN_POINT('',(117.760743812198,-2.3,66.2877757829205));
#192930=CARTESIAN_POINT('Origin',(120.591198299308,1.45439216225896E-14,
51.7264224494141));
#192931=CARTESIAN_POINT('Origin',(120.591198299308,1.45439216225896E-14,
51.7264224494141));
#192932=CARTESIAN_POINT('Origin',(118.156384306592,-2.3,64.25239204573));
#192933=CARTESIAN_POINT('',(117.247827757456,-2.3,66.3060780326826));
#192934=CARTESIAN_POINT('',(117.188668455303,-2.3,66.6104247393819));
#192935=CARTESIAN_POINT('',(117.247827757456,-2.3,66.3060780326826));
#192936=CARTESIAN_POINT('Origin',(116.959178380441,-2.3,51.0204257716897));
#192937=CARTESIAN_POINT('Origin',(116.959178380441,-2.3,51.0204257716897));
#192938=CARTESIAN_POINT('Origin',(117.665570804043,-2.3,64.1569870892808));
#192939=CARTESIAN_POINT('Origin',(120.100384796758,1.45439216225896E-14,
51.6310174929649));
#192940=CARTESIAN_POINT('Origin',(120.100384796758,1.45439216225896E-14,
51.6310174929649));
#192941=CARTESIAN_POINT('Origin',(116.683943798944,-2.8,63.9661771763823));
#192942=CARTESIAN_POINT('',(116.754462709301,-2.8,66.223799574922));
#192943=CARTESIAN_POINT('',(116.695355203691,-2.8,66.5278798128357));
#192944=CARTESIAN_POINT('',(116.754462709301,-2.8,66.223799574922));
#192945=CARTESIAN_POINT('',(116.248070475418,-2.8,66.2085398433723));
#192946=CARTESIAN_POINT('Origin',(116.959178380441,-2.8,51.0204257716897));
#192947=CARTESIAN_POINT('',(116.189277281699,-2.8,66.511003094857));
#192948=CARTESIAN_POINT('',(116.248070475418,-2.8,66.2085398433723));
#192949=CARTESIAN_POINT('Origin',(116.959178380441,-2.8,51.0204257716897));
#192950=CARTESIAN_POINT('Origin',(117.174757301493,-2.8,64.0615821328315));
#192951=CARTESIAN_POINT('',(116.738249906779,-2.3,66.3072067970213));
#192952=CARTESIAN_POINT('',(116.67946943582,-2.3,66.6096045959044));
#192953=CARTESIAN_POINT('',(116.738249906779,-2.3,66.3072067970213));
#192954=CARTESIAN_POINT('Origin',(119.609571294209,1.45439216225896E-14,
51.5356125365156));
#192955=CARTESIAN_POINT('Origin',(119.609571294209,1.45439216225896E-14,
51.5356125365156));
#192956=CARTESIAN_POINT('Origin',(117.174757301493,-2.3,64.0615821328315));
#192957=CARTESIAN_POINT('',(116.231945164223,-2.3,66.2914969638595));
#192958=CARTESIAN_POINT('',(116.173473843287,-2.3,66.5923043316899));
#192959=CARTESIAN_POINT('',(116.231945164223,-2.3,66.2914969638595));
#192960=CARTESIAN_POINT('Origin',(116.959178380441,-2.3,51.0204257716897));
#192961=CARTESIAN_POINT('Origin',(116.959178380441,-2.3,51.0204257716897));
#192962=CARTESIAN_POINT('Origin',(116.683943798944,-2.3,63.9661771763823));
#192963=CARTESIAN_POINT('Origin',(119.118757791659,1.45439216225896E-14,
51.4402075800664));
#192964=CARTESIAN_POINT('Origin',(119.118757791659,1.45439216225896E-14,
51.4402075800664));
#192965=CARTESIAN_POINT('Origin',(115.702316793845,-2.8,63.7753672634838));
#192966=CARTESIAN_POINT('',(115.744917738381,-2.8,66.1766144284786));
#192967=CARTESIAN_POINT('',(115.686371158483,-2.8,66.4778089681697));
#192968=CARTESIAN_POINT('',(115.744917738381,-2.8,66.1766144284786));
#192969=CARTESIAN_POINT('',(115.244963034622,-2.8,66.1282366407438));
#192970=CARTESIAN_POINT('Origin',(116.959178380441,-2.8,51.0204257716897));
#192971=CARTESIAN_POINT('',(115.186597835385,-2.8,66.4284980624817));
#192972=CARTESIAN_POINT('',(115.244963034622,-2.8,66.1282366407438));
#192973=CARTESIAN_POINT('Origin',(116.959178380441,-2.8,51.0204257716897));
#192974=CARTESIAN_POINT('Origin',(116.193130296394,-2.8,63.870772219933));
#192975=CARTESIAN_POINT('',(115.728861059795,-2.3,66.2592184665667));
#192976=CARTESIAN_POINT('',(115.670632340546,-2.3,66.5587777631371));
#192977=CARTESIAN_POINT('',(115.728861059795,-2.3,66.2592184665667));
#192978=CARTESIAN_POINT('Origin',(118.62794428911,1.45439216225896E-14,
51.3448026236171));
#192979=CARTESIAN_POINT('Origin',(118.62794428911,1.45439216225896E-14,
51.3448026236171));
#192980=CARTESIAN_POINT('Origin',(116.193130296394,-2.3,63.870772219933));
#192981=CARTESIAN_POINT('',(115.228956826212,-2.3,66.2105810335809));
#192982=CARTESIAN_POINT('',(115.170906557973,-2.3,66.5092222838734));
#192983=CARTESIAN_POINT('',(115.228956826212,-2.3,66.2105810335809));
#192984=CARTESIAN_POINT('Origin',(116.959178380441,-2.3,51.0204257716897));
#192985=CARTESIAN_POINT('Origin',(116.959178380441,-2.3,51.0204257716897));
#192986=CARTESIAN_POINT('Origin',(115.702316793845,-2.3,63.7753672634838));
#192987=CARTESIAN_POINT('Origin',(118.13713078656,1.45439216225896E-14,
51.2493976671679));
#192988=CARTESIAN_POINT('Origin',(118.13713078656,1.45439216225896E-14,
51.2493976671679));
#192989=CARTESIAN_POINT('Origin',(114.720689788746,-2.8,63.5845573505853));
#192990=CARTESIAN_POINT('',(114.748176102656,-2.8,66.063562161234));
#192991=CARTESIAN_POINT('',(114.689928828871,-2.8,66.363216912147));
#192992=CARTESIAN_POINT('',(114.748176102656,-2.8,66.063562161234));
#192993=CARTESIAN_POINT('',(114.254537373977,-2.8,65.9826916606871));
#192994=CARTESIAN_POINT('Origin',(116.959178380441,-2.8,51.0204257716897));
#192995=CARTESIAN_POINT('',(114.196345710662,-2.8,66.2820603219557));
#192996=CARTESIAN_POINT('',(114.254537373977,-2.8,65.9826916606871));
#192997=CARTESIAN_POINT('Origin',(116.959178380441,-2.8,51.0204257716897));
#192998=CARTESIAN_POINT('Origin',(115.211503291295,-2.8,63.6799623070345));
#192999=CARTESIAN_POINT('',(114.732202704012,-2.3,66.1457377632978));
#193000=CARTESIAN_POINT('',(114.674268466112,-2.3,66.4437820922258));
#193001=CARTESIAN_POINT('',(114.732202704012,-2.3,66.1457377632978));
#193002=CARTESIAN_POINT('Origin',(117.64631728401,1.45439216225896E-14,
51.1539927107186));
#193003=CARTESIAN_POINT('Origin',(117.64631728401,1.45439216225896E-14,
51.1539927107186));
#193004=CARTESIAN_POINT('Origin',(115.211503291295,-2.3,63.6799623070345));
#193005=CARTESIAN_POINT('',(114.238579446542,-2.3,66.0647876706762));
#193006=CARTESIAN_POINT('',(114.180699928051,-2.3,66.36255049405));
#193007=CARTESIAN_POINT('',(114.238579446542,-2.3,66.0647876706762));
#193008=CARTESIAN_POINT('Origin',(116.959178380441,-2.3,51.0204257716897));
#193009=CARTESIAN_POINT('Origin',(116.959178380441,-2.3,51.0204257716897));
#193010=CARTESIAN_POINT('Origin',(114.720689788746,-2.3,63.5845573505853));
#193011=CARTESIAN_POINT('Origin',(117.155503781461,1.45439216225896E-14,
51.0585877542694));
#193012=CARTESIAN_POINT('Origin',(117.155503781461,1.45439216225896E-14,
51.0585877542694));
#193013=CARTESIAN_POINT('Origin',(113.739062783647,-2.8,63.3937474376868));
#193014=CARTESIAN_POINT('',(113.764037649552,-2.8,65.8856724637829));
#193015=CARTESIAN_POINT('',(113.705839815162,-2.8,66.1850728723215));
#193016=CARTESIAN_POINT('',(113.764037649552,-2.8,65.8856724637829));
#193017=CARTESIAN_POINT('',(113.276677949281,-2.8,65.7724993236168));
#193018=CARTESIAN_POINT('Origin',(116.959178380441,-2.8,51.0204257716897));
#193019=CARTESIAN_POINT('',(113.218412103209,-2.8,66.0722496201832));
#193020=CARTESIAN_POINT('',(113.276677949281,-2.8,65.7724993236168));
#193021=CARTESIAN_POINT('Origin',(116.959178380441,-2.8,51.0204257716897));
#193022=CARTESIAN_POINT('Origin',(114.229876286196,-2.8,63.489152394136));
#193023=CARTESIAN_POINT('',(113.748078005312,-2.3,65.9677773059216));
#193024=CARTESIAN_POINT('',(113.690192414544,-2.3,66.2655713682987));
#193025=CARTESIAN_POINT('',(113.748078005312,-2.3,65.9677773059216));
#193026=CARTESIAN_POINT('Origin',(116.664690278911,1.45439216225896E-14,
50.9631827978201));
#193027=CARTESIAN_POINT('Origin',(116.664690278911,1.45439216225896E-14,
50.9631827978201));
#193028=CARTESIAN_POINT('Origin',(114.229876286196,-2.3,63.489152394136));
#193029=CARTESIAN_POINT('',(113.26069938356,-2.3,65.8547015078552));
#193030=CARTESIAN_POINT('',(113.202746871335,-2.3,66.1528398495673));
#193031=CARTESIAN_POINT('',(113.26069938356,-2.3,65.8547015078552));
#193032=CARTESIAN_POINT('Origin',(116.959178380441,-2.3,51.0204257716897));
#193033=CARTESIAN_POINT('Origin',(116.959178380441,-2.3,51.0204257716897));
#193034=CARTESIAN_POINT('Origin',(113.739062783647,-2.3,63.3937474376868));
#193035=CARTESIAN_POINT('Origin',(116.173876776362,1.45439216225896E-14,
50.8677778413709));
#193036=CARTESIAN_POINT('Origin',(116.173876776362,1.45439216225896E-14,
50.8677778413709));
#193037=CARTESIAN_POINT('Origin',(112.757435778548,-2.8,63.2029375247883));
#193038=CARTESIAN_POINT('',(112.792469528639,-2.8,65.6431143360832));
#193039=CARTESIAN_POINT('',(112.734073177143,-2.8,65.943536021505));
#193040=CARTESIAN_POINT('',(112.792469528639,-2.8,65.6431143360832));
#193041=CARTESIAN_POINT('',(112.311434063134,-2.8,65.4974059909163));
#193042=CARTESIAN_POINT('Origin',(116.959178380441,-2.8,51.0204257716897));
#193043=CARTESIAN_POINT('',(112.252843447732,-2.8,65.7988270725098));
#193044=CARTESIAN_POINT('',(112.311434063134,-2.8,65.4974059909163));
#193045=CARTESIAN_POINT('Origin',(116.959178380441,-2.8,51.0204257716897));
#193046=CARTESIAN_POINT('Origin',(113.248249281097,-2.8,63.2983424812375));
#193047=CARTESIAN_POINT('',(112.776454652423,-2.3,65.7255033206915));
#193048=CARTESIAN_POINT('',(112.71837373382,-2.3,66.024302252655));
#193049=CARTESIAN_POINT('',(112.776454652423,-2.3,65.7255033206915));
#193050=CARTESIAN_POINT('Origin',(115.683063273812,1.45439216225896E-14,
50.7723728849216));
#193051=CARTESIAN_POINT('Origin',(115.683063273812,1.45439216225896E-14,
50.7723728849216));
#193052=CARTESIAN_POINT('Origin',(113.248249281097,-2.3,63.2983424812375));
#193053=CARTESIAN_POINT('',(112.295365130396,-2.3,65.580073070838));
#193054=CARTESIAN_POINT('',(112.237093089611,-2.3,65.8798552362785));
#193055=CARTESIAN_POINT('',(112.295365130396,-2.3,65.580073070838));
#193056=CARTESIAN_POINT('Origin',(116.959178380441,-2.3,51.0204257716897));
#193057=CARTESIAN_POINT('Origin',(116.959178380441,-2.3,51.0204257716897));
#193058=CARTESIAN_POINT('Origin',(112.757435778548,-2.3,63.2029375247883));
#193059=CARTESIAN_POINT('Origin',(115.192249771263,1.45439216225896E-14,
50.6769679284724));
#193060=CARTESIAN_POINT('Origin',(115.192249771263,1.45439216225896E-14,
50.6769679284724));
#193061=CARTESIAN_POINT('Origin',(111.775808773449,-2.8,63.0121276118898));
#193062=CARTESIAN_POINT('',(111.833604007695,-2.8,65.3352073228156));
#193063=CARTESIAN_POINT('',(111.774753459122,-2.8,65.637965637969));
#193064=CARTESIAN_POINT('',(111.833604007695,-2.8,65.3352073228156));
#193065=CARTESIAN_POINT('',(111.359023145067,-2.8,65.1562930902008));
#193066=CARTESIAN_POINT('Origin',(116.959178380441,-2.8,51.0204257716897));
#193067=CARTESIAN_POINT('',(111.299844384071,-2.8,65.4607399034676));
#193068=CARTESIAN_POINT('',(111.359023145067,-2.8,65.1562930902008));
#193069=CARTESIAN_POINT('Origin',(116.959178380441,-2.8,51.0204257716897));
#193070=CARTESIAN_POINT('Origin',(112.266622275998,-2.8,63.107532568339));
#193071=CARTESIAN_POINT('',(111.817462732837,-2.3,65.4182465688194));
#193072=CARTESIAN_POINT('',(111.758934994926,-2.3,65.7193441753763));
#193073=CARTESIAN_POINT('',(111.817462732837,-2.3,65.4182465688194));
#193074=CARTESIAN_POINT('Origin',(114.701436268713,1.45439216225896E-14,
50.5815629720231));
#193075=CARTESIAN_POINT('Origin',(114.701436268713,1.45439216225896E-14,
50.5815629720231));
#193076=CARTESIAN_POINT('Origin',(112.266622275998,-2.3,63.107532568339));
#193077=CARTESIAN_POINT('',(111.342790505145,-2.3,65.2398023663664));
#193078=CARTESIAN_POINT('',(111.283939956573,-2.3,65.5425606815198));
#193079=CARTESIAN_POINT('',(111.342790505145,-2.3,65.2398023663664));
#193080=CARTESIAN_POINT('Origin',(116.959178380441,-2.3,51.0204257716897));
#193081=CARTESIAN_POINT('Origin',(116.959178380441,-2.3,51.0204257716897));
#193082=CARTESIAN_POINT('Origin',(111.775808773449,-2.3,63.0121276118898));
#193083=CARTESIAN_POINT('Origin',(114.210622766164,1.45439216225896E-14,
50.4861580155739));
#193084=CARTESIAN_POINT('Origin',(114.210622766164,1.45439216225896E-14,
50.4861580155739));
#193085=CARTESIAN_POINT('Origin',(111.775808773449,-1.8,63.0121276118898));
#193086=CARTESIAN_POINT('',(111.804551627846,-1.8,65.4846681143887));
#193087=CARTESIAN_POINT('',(111.746279587062,-1.8,65.7844502798292));
#193088=CARTESIAN_POINT('',(111.804551627846,-1.8,65.4846681143887));
#193089=CARTESIAN_POINT('',(111.329807058035,-1.8,65.3065960780178));
#193090=CARTESIAN_POINT('Origin',(116.959178380441,-1.8,51.0204257716897));
#193091=CARTESIAN_POINT('',(111.271216442633,-1.8,65.6080171596113));
#193092=CARTESIAN_POINT('',(111.329807058035,-1.8,65.3065960780178));
#193093=CARTESIAN_POINT('Origin',(116.959178380441,-1.8,51.0204257716897));
#193094=CARTESIAN_POINT('Origin',(112.266622275998,-1.8,63.107532568339));
#193095=CARTESIAN_POINT('',(111.794827647324,-1.3,65.534693407793));
#193096=CARTESIAN_POINT('',(111.736746728721,-1.3,65.8334923397565));
#193097=CARTESIAN_POINT('',(111.794827647324,-1.3,65.534693407793));
#193098=CARTESIAN_POINT('Origin',(114.701436268713,1.45439216225896E-14,
50.5815629720231));
#193099=CARTESIAN_POINT('Origin',(114.701436268713,1.45439216225896E-14,
50.5815629720231));
#193100=CARTESIAN_POINT('Origin',(112.266622275998,-1.3,63.107532568339));
#193101=CARTESIAN_POINT('',(111.320029020991,-1.3,65.3568994667354));
#193102=CARTESIAN_POINT('',(111.261632669494,-1.3,65.6573211521572));
#193103=CARTESIAN_POINT('',(111.320029020991,-1.3,65.3568994667354));
#193104=CARTESIAN_POINT('Origin',(116.959178380441,-1.3,51.0204257716897));
#193105=CARTESIAN_POINT('Origin',(116.959178380441,-1.3,51.0204257716897));
#193106=CARTESIAN_POINT('Origin',(111.775808773449,-1.3,63.0121276118898));
#193107=CARTESIAN_POINT('Origin',(114.210622766164,1.45439216225896E-14,
50.4861580155739));
#193108=CARTESIAN_POINT('Origin',(114.210622766164,1.45439216225896E-14,
50.4861580155739));
#193109=CARTESIAN_POINT('Origin',(111.775808773449,-0.799999999999986,63.0121276118898));
#193110=CARTESIAN_POINT('',(111.788258875911,-0.799999999999986,65.5684866385074));
#193111=CARTESIAN_POINT('',(111.730306363686,-0.799999999999986,65.8666249802195));
#193112=CARTESIAN_POINT('',(111.788258875911,-0.799999999999986,65.5684866385074));
#193113=CARTESIAN_POINT('',(111.313423939083,-0.799999999999986,65.3908794978198));
#193114=CARTESIAN_POINT('Origin',(116.959178380441,-0.799999999999986,51.0204257716897));
#193115=CARTESIAN_POINT('',(111.255158093011,-0.799999999999986,65.6906297943862));
#193116=CARTESIAN_POINT('',(111.313423939083,-0.799999999999986,65.3908794978198));
#193117=CARTESIAN_POINT('Origin',(116.959178380441,-0.799999999999986,51.0204257716897));
#193118=CARTESIAN_POINT('Origin',(112.266622275998,-0.799999999999986,63.107532568339));
#193119=CARTESIAN_POINT('',(111.784823995114,-0.299999999999985,65.5861574801246));
#193120=CARTESIAN_POINT('',(111.726938404346,-0.299999999999985,65.8839515425017));
#193121=CARTESIAN_POINT('',(111.784823995114,-0.299999999999985,65.5861574801246));
#193122=CARTESIAN_POINT('Origin',(114.701436268713,1.45439216225896E-14,
50.5815629720231));
#193123=CARTESIAN_POINT('Origin',(114.701436268713,1.45439216225896E-14,
50.5815629720231));
#193124=CARTESIAN_POINT('Origin',(112.266622275998,-0.299999999999985,63.107532568339));
#193125=CARTESIAN_POINT('',(111.309970136804,-0.299999999999985,65.4086476815366));
#193126=CARTESIAN_POINT('',(111.251772302414,-0.299999999999985,65.7080480900753));
#193127=CARTESIAN_POINT('',(111.309970136804,-0.299999999999985,65.4086476815366));
#193128=CARTESIAN_POINT('Origin',(116.959178380441,-0.299999999999985,51.0204257716897));
#193129=CARTESIAN_POINT('Origin',(116.959178380441,-0.299999999999985,51.0204257716897));
#193130=CARTESIAN_POINT('Origin',(111.775808773449,-0.299999999999985,63.0121276118898));
#193131=CARTESIAN_POINT('Origin',(114.210622766164,1.45439216225896E-14,
50.4861580155739));
#193132=CARTESIAN_POINT('Origin',(114.210622766164,1.45439216225896E-14,
50.4861580155739));
#193133=CARTESIAN_POINT('Origin',(117.665570804043,-0.799999999999986,64.1569870892808));
#193134=CARTESIAN_POINT('',(117.730993451766,-0.799999999999986,66.4408273553883));
#193135=CARTESIAN_POINT('',(117.671989132337,-0.799999999999986,66.7443767490697));
#193136=CARTESIAN_POINT('',(117.730993451766,-0.799999999999986,66.4408273553883));
#193137=CARTESIAN_POINT('',(117.218305542335,-0.799999999999986,66.4579559051328));
#193138=CARTESIAN_POINT('Origin',(116.959178380441,-0.799999999999986,51.0204257716897));
#193139=CARTESIAN_POINT('',(117.159740102242,-0.799999999999986,66.7592474716348));
#193140=CARTESIAN_POINT('',(117.218305542335,-0.799999999999986,66.4579559051328));
#193141=CARTESIAN_POINT('Origin',(116.959178380441,-0.799999999999986,51.0204257716897));
#193142=CARTESIAN_POINT('Origin',(118.156384306592,-0.799999999999986,64.25239204573));
#193143=CARTESIAN_POINT('',(117.727495032124,-0.299999999999985,66.4588250743906));
#193144=CARTESIAN_POINT('',(117.668561340481,-0.299999999999985,66.7620111214277));
#193145=CARTESIAN_POINT('',(117.727495032124,-0.299999999999985,66.4588250743906));
#193146=CARTESIAN_POINT('Origin',(120.591198299308,1.45439216225896E-14,
51.7264224494141));
#193147=CARTESIAN_POINT('Origin',(120.591198299308,1.45439216225896E-14,
51.7264224494141));
#193148=CARTESIAN_POINT('Origin',(118.156384306592,-0.299999999999985,64.25239204573));
#193149=CARTESIAN_POINT('',(117.214833642932,-0.299999999999985,66.4758171900162));
#193150=CARTESIAN_POINT('',(117.156337267937,-0.299999999999985,66.7767534491633));
#193151=CARTESIAN_POINT('',(117.214833642932,-0.299999999999985,66.4758171900162));
#193152=CARTESIAN_POINT('Origin',(116.959178380441,-0.299999999999985,51.0204257716897));
#193153=CARTESIAN_POINT('Origin',(116.959178380441,-0.299999999999985,51.0204257716897));
#193154=CARTESIAN_POINT('Origin',(117.665570804043,-0.299999999999985,64.1569870892808));
#193155=CARTESIAN_POINT('Origin',(120.100384796758,1.45439216225896E-14,
51.6310174929649));
#193156=CARTESIAN_POINT('Origin',(120.100384796758,1.45439216225896E-14,
51.6310174929649));
#193157=CARTESIAN_POINT('Origin',(117.665570804043,-1.8,64.1569870892808));
#193158=CARTESIAN_POINT('',(117.747589699224,-1.8,66.3554474899478));
#193159=CARTESIAN_POINT('',(117.688248030859,-1.8,66.6607323847921));
#193160=CARTESIAN_POINT('',(117.747589699224,-1.8,66.3554474899478));
#193161=CARTESIAN_POINT('',(117.23477510084,-1.8,66.3732277946038));
#193162=CARTESIAN_POINT('Origin',(116.959178380441,-1.8,51.0204257716897));
#193163=CARTESIAN_POINT('',(117.175879826691,-1.8,66.6762162017529));
#193164=CARTESIAN_POINT('',(117.23477510084,-1.8,66.3732277946038));
#193165=CARTESIAN_POINT('Origin',(116.959178380441,-1.8,51.0204257716897));
#193166=CARTESIAN_POINT('Origin',(118.156384306592,-1.8,64.25239204573));
#193167=CARTESIAN_POINT('',(117.737684163035,-1.3,66.4064068016241));
#193168=CARTESIAN_POINT('',(117.678544300543,-1.3,66.710653500439));
#193169=CARTESIAN_POINT('',(117.737684163035,-1.3,66.4064068016241));
#193170=CARTESIAN_POINT('Origin',(120.591198299308,1.45439216225896E-14,
51.7264224494141));
#193171=CARTESIAN_POINT('Origin',(120.591198299308,1.45439216225896E-14,
51.7264224494141));
#193172=CARTESIAN_POINT('Origin',(118.156384306592,-1.3,64.25239204573));
#193173=CARTESIAN_POINT('',(117.22494535473,-1.3,66.4237972020704));
#193174=CARTESIAN_POINT('',(117.166247380857,-1.3,66.7257705923584));
#193175=CARTESIAN_POINT('',(117.22494535473,-1.3,66.4237972020704));
#193176=CARTESIAN_POINT('Origin',(116.959178380441,-1.3,51.0204257716897));
#193177=CARTESIAN_POINT('Origin',(116.959178380441,-1.3,51.0204257716897));
#193178=CARTESIAN_POINT('Origin',(117.665570804043,-1.3,64.1569870892808));
#193179=CARTESIAN_POINT('Origin',(120.100384796758,1.45439216225896E-14,
51.6310174929649));
#193180=CARTESIAN_POINT('Origin',(120.100384796758,1.45439216225896E-14,
51.6310174929649));
#193181=CARTESIAN_POINT('Origin',(116.683943798944,-1.8,63.9661771763823));
#193182=CARTESIAN_POINT('',(116.72528216571,-1.8,66.3739197084998));
#193183=CARTESIAN_POINT('',(116.666760704416,-1.8,66.6749850248193));
#193184=CARTESIAN_POINT('',(116.72528216571,-1.8,66.3739197084998));
#193185=CARTESIAN_POINT('',(116.219046700398,-1.8,66.3578534765906));
#193186=CARTESIAN_POINT('Origin',(116.959178380441,-1.8,51.0204257716897));
#193187=CARTESIAN_POINT('',(116.160830340994,-1.8,66.6573491875945));
#193188=CARTESIAN_POINT('',(116.219046700398,-1.8,66.3578534765906));
#193189=CARTESIAN_POINT('Origin',(116.959178380441,-1.8,51.0204257716897));
#193190=CARTESIAN_POINT('Origin',(117.174757301493,-1.8,64.0615821328315));
#193191=CARTESIAN_POINT('',(116.715515864156,-1.3,66.4241627236523));
#193192=CARTESIAN_POINT('',(116.657187981895,-1.3,66.7242321671538));
#193193=CARTESIAN_POINT('',(116.715515864156,-1.3,66.4241627236523));
#193194=CARTESIAN_POINT('Origin',(119.609571294209,1.45439216225896E-14,
51.5356125365156));
#193195=CARTESIAN_POINT('Origin',(119.609571294209,1.45439216225896E-14,
51.5356125365156));
#193196=CARTESIAN_POINT('Origin',(117.174757301493,-1.3,64.0615821328315));
#193197=CARTESIAN_POINT('',(116.209332166521,-1.3,66.4078301714677));
#193198=CARTESIAN_POINT('',(116.151306383661,-1.3,66.7063454560356));
#193199=CARTESIAN_POINT('',(116.209332166521,-1.3,66.4078301714677));
#193200=CARTESIAN_POINT('Origin',(116.959178380441,-1.3,51.0204257716897));
#193201=CARTESIAN_POINT('Origin',(116.959178380441,-1.3,51.0204257716897));
#193202=CARTESIAN_POINT('Origin',(116.683943798944,-1.3,63.9661771763823));
#193203=CARTESIAN_POINT('Origin',(119.118757791659,1.45439216225896E-14,
51.4402075800664));
#193204=CARTESIAN_POINT('Origin',(119.118757791659,1.45439216225896E-14,
51.4402075800664));
#193205=CARTESIAN_POINT('Origin',(115.702316793845,-1.8,63.7753672634838));
#193206=CARTESIAN_POINT('',(115.716016948437,-1.8,66.3252953614908));
#193207=CARTESIAN_POINT('',(115.658040043519,-1.8,66.6235591921022));
#193208=CARTESIAN_POINT('',(115.716016948437,-1.8,66.3252953614908));
#193209=CARTESIAN_POINT('',(115.216152688302,-1.8,66.2764522839691));
#193210=CARTESIAN_POINT('Origin',(116.959178380441,-1.8,51.0204257716897));
#193211=CARTESIAN_POINT('',(115.158351935903,-1.8,66.573809892952));
#193212=CARTESIAN_POINT('',(115.216152688302,-1.8,66.2764522839691));
#193213=CARTESIAN_POINT('Origin',(116.959178380441,-1.8,51.0204257716897));
#193214=CARTESIAN_POINT('Origin',(116.193130296394,-1.8,63.870772219933));
#193215=CARTESIAN_POINT('',(115.706343034183,-1.3,66.3750630875619));
#193216=CARTESIAN_POINT('',(115.64855437112,-1.3,66.6723585026113));
#193217=CARTESIAN_POINT('',(115.706343034183,-1.3,66.3750630875619));
#193218=CARTESIAN_POINT('Origin',(118.62794428911,1.45439216225896E-14,
51.3448026236171));
#193219=CARTESIAN_POINT('Origin',(118.62794428911,1.45439216225896E-14,
51.3448026236171));
#193220=CARTESIAN_POINT('Origin',(116.193130296394,-1.3,63.870772219933));
#193221=CARTESIAN_POINT('',(115.20650865023,-1.3,66.3260663111735));
#193222=CARTESIAN_POINT('',(115.148894434369,-1.3,66.6224642776501));
#193223=CARTESIAN_POINT('',(115.20650865023,-1.3,66.3260663111735));
#193224=CARTESIAN_POINT('Origin',(116.959178380441,-1.3,51.0204257716897));
#193225=CARTESIAN_POINT('Origin',(116.959178380441,-1.3,51.0204257716897));
#193226=CARTESIAN_POINT('Origin',(115.702316793845,-1.3,63.7753672634838));
#193227=CARTESIAN_POINT('Origin',(118.13713078656,1.45439216225896E-14,
51.2493976671679));
#193228=CARTESIAN_POINT('Origin',(118.13713078656,1.45439216225896E-14,
51.2493976671679));
#193229=CARTESIAN_POINT('Origin',(114.720689788746,-1.8,63.5845573505853));
#193230=CARTESIAN_POINT('',(114.71942455413,-1.8,66.2114753175407));
#193231=CARTESIAN_POINT('',(114.661738345058,-1.8,66.5082436551355));
#193232=CARTESIAN_POINT('',(114.71942455413,-1.8,66.2114753175407));
#193233=CARTESIAN_POINT('',(114.225813551673,-1.8,66.1304621786584));
#193234=CARTESIAN_POINT('Origin',(116.959178380441,-1.8,51.0204257716897));
#193235=CARTESIAN_POINT('',(114.168181362785,-1.8,66.4269526078809));
#193236=CARTESIAN_POINT('',(114.225813551673,-1.8,66.1304621786584));
#193237=CARTESIAN_POINT('Origin',(116.959178380441,-1.8,51.0204257716897));
#193238=CARTESIAN_POINT('Origin',(115.211503291295,-1.8,63.6799623070345));
#193239=CARTESIAN_POINT('',(114.709799940683,-1.3,66.2609894142129));
#193240=CARTESIAN_POINT('',(114.652299164781,-1.3,66.5568037856086));
#193241=CARTESIAN_POINT('',(114.709799940683,-1.3,66.2609894142129));
#193242=CARTESIAN_POINT('Origin',(117.64631728401,1.45439216225896E-14,
51.1539927107186));
#193243=CARTESIAN_POINT('Origin',(117.64631728401,1.45439216225896E-14,
51.1539927107186));
#193244=CARTESIAN_POINT('Origin',(115.211503291295,-1.3,63.6799623070345));
#193245=CARTESIAN_POINT('',(114.216198098491,-1.3,66.1799291500881));
#193246=CARTESIAN_POINT('',(114.158750823915,-1.3,66.4754682823909));
#193247=CARTESIAN_POINT('',(114.216198098491,-1.3,66.1799291500881));
#193248=CARTESIAN_POINT('Origin',(116.959178380441,-1.3,51.0204257716897));
#193249=CARTESIAN_POINT('Origin',(116.959178380441,-1.3,51.0204257716897));
#193250=CARTESIAN_POINT('Origin',(114.720689788746,-1.3,63.5845573505853));
#193251=CARTESIAN_POINT('Origin',(117.155503781461,1.45439216225896E-14,
51.0585877542694));
#193252=CARTESIAN_POINT('Origin',(117.155503781461,1.45439216225896E-14,
51.0585877542694));
#193253=CARTESIAN_POINT('Origin',(113.739062783647,-1.8,63.3937474376868));
#193254=CARTESIAN_POINT('',(113.735310750518,-1.8,66.0334588100773));
#193255=CARTESIAN_POINT('',(113.677672566881,-1.8,66.3299800794583));
#193256=CARTESIAN_POINT('',(113.735310750518,-1.8,66.0334588100773));
#193257=CARTESIAN_POINT('',(113.247917140825,-1.8,65.9204601178992));
#193258=CARTESIAN_POINT('Origin',(116.959178380441,-1.8,51.0204257716897));
#193259=CARTESIAN_POINT('',(113.190212891236,-1.8,66.2173212654414));
#193260=CARTESIAN_POINT('',(113.247917140825,-1.8,65.9204601178992));
#193261=CARTESIAN_POINT('Origin',(116.959178380441,-1.8,51.0204257716897));
#193262=CARTESIAN_POINT('Origin',(114.229876286196,-1.8,63.489152394136));
#193263=CARTESIAN_POINT('',(113.725694280819,-1.3,66.0829310110071));
#193264=CARTESIAN_POINT('',(113.668241069027,-1.3,66.3785006874882));
#193265=CARTESIAN_POINT('',(113.725694280819,-1.3,66.0829310110071));
#193266=CARTESIAN_POINT('Origin',(116.664690278911,1.45439216225896E-14,
50.9631827978201));
#193267=CARTESIAN_POINT('Origin',(116.664690278911,1.45439216225896E-14,
50.9631827978201));
#193268=CARTESIAN_POINT('Origin',(114.229876286196,-1.3,63.489152394136));
#193269=CARTESIAN_POINT('',(113.238289468134,-1.3,65.9699899529383));
#193270=CARTESIAN_POINT('',(113.180770825207,-1.3,66.2658962417468));
#193271=CARTESIAN_POINT('',(113.238289468134,-1.3,65.9699899529383));
#193272=CARTESIAN_POINT('Origin',(116.959178380441,-1.3,51.0204257716897));
#193273=CARTESIAN_POINT('Origin',(116.959178380441,-1.3,51.0204257716897));
#193274=CARTESIAN_POINT('Origin',(113.739062783647,-1.3,63.3937474376868));
#193275=CARTESIAN_POINT('Origin',(116.173876776362,1.45439216225896E-14,
50.8677778413709));
#193276=CARTESIAN_POINT('Origin',(116.173876776362,1.45439216225896E-14,
50.8677778413709));
#193277=CARTESIAN_POINT('Origin',(112.757435778548,-1.8,63.2029375247883));
#193278=CARTESIAN_POINT('',(112.763643649162,-1.8,65.7914098900782));
#193279=CARTESIAN_POINT('',(112.705812640189,-1.8,66.0889231548602));
#193280=CARTESIAN_POINT('',(112.763643649162,-1.8,65.7914098900782));
#193281=CARTESIAN_POINT('',(112.282511314055,-1.8,65.6461998933239));
#193282=CARTESIAN_POINT('Origin',(116.959178380441,-1.8,51.0204257716897));
#193283=CARTESIAN_POINT('',(112.2244916477,-1.8,65.9446837113571));
#193284=CARTESIAN_POINT('',(112.282511314055,-1.8,65.6461998933239));
#193285=CARTESIAN_POINT('Origin',(116.959178380441,-1.8,51.0204257716897));
#193286=CARTESIAN_POINT('Origin',(113.248249281097,-1.8,63.2983424812375));
#193287=CARTESIAN_POINT('',(112.753994479771,-1.3,65.8410503155003));
#193288=CARTESIAN_POINT('',(112.696350299514,-1.3,66.1376024346597));
#193289=CARTESIAN_POINT('',(112.753994479771,-1.3,65.8410503155003));
#193290=CARTESIAN_POINT('Origin',(115.683063273812,1.45439216225896E-14,
50.7723728849216));
#193291=CARTESIAN_POINT('Origin',(115.683063273812,1.45439216225896E-14,
50.7723728849216));
#193292=CARTESIAN_POINT('Origin',(113.248249281097,-1.3,63.2983424812375));
#193293=CARTESIAN_POINT('',(112.272830146612,-1.3,65.696004933629));
#193294=CARTESIAN_POINT('',(112.21499913764,-1.3,65.993518198411));
#193295=CARTESIAN_POINT('',(112.272830146612,-1.3,65.696004933629));
#193296=CARTESIAN_POINT('Origin',(116.959178380441,-1.3,51.0204257716897));
#193297=CARTESIAN_POINT('Origin',(116.959178380441,-1.3,51.0204257716897));
#193298=CARTESIAN_POINT('Origin',(112.757435778548,-1.3,63.2029375247883));
#193299=CARTESIAN_POINT('Origin',(115.192249771263,1.45439216225896E-14,
50.6769679284724));
#193300=CARTESIAN_POINT('Origin',(115.192249771263,1.45439216225896E-14,
50.6769679284724));
#193301=CARTESIAN_POINT('Origin',(112.757435778548,-0.799999999999986,63.2029375247883));
#193302=CARTESIAN_POINT('',(112.747475965584,-0.799999999999986,65.874584996489));
#193303=CARTESIAN_POINT('',(112.689957322657,-0.799999999999986,66.1704912852975));
#193304=CARTESIAN_POINT('',(112.747475965584,-0.799999999999986,65.874584996489));
#193305=CARTESIAN_POINT('',(112.266290135726,-0.799999999999986,65.7296502050007));
#193306=CARTESIAN_POINT('Origin',(116.959178380441,-0.799999999999986,51.0204257716897));
#193307=CARTESIAN_POINT('',(112.208585886137,-0.799999999999986,66.0265113525429));
#193308=CARTESIAN_POINT('',(112.266290135726,-0.799999999999986,65.7296502050007));
#193309=CARTESIAN_POINT('Origin',(116.959178380441,-0.799999999999986,51.0204257716897));
#193310=CARTESIAN_POINT('Origin',(113.248249281097,-0.799999999999986,63.2983424812375));
#193311=CARTESIAN_POINT('',(112.74406727572,-0.299999999999985,65.8921210981086));
#193312=CARTESIAN_POINT('',(112.686614063928,-0.299999999999985,66.1876907745897));
#193313=CARTESIAN_POINT('',(112.74406727572,-0.299999999999985,65.8921210981086));
#193314=CARTESIAN_POINT('Origin',(115.683063273812,1.45439216225896E-14,
50.7723728849216));
#193315=CARTESIAN_POINT('Origin',(115.683063273812,1.45439216225896E-14,
50.7723728849216));
#193316=CARTESIAN_POINT('Origin',(113.248249281097,-0.299999999999985,63.2983424812375));
#193317=CARTESIAN_POINT('',(112.26287024287,-0.299999999999985,65.7472439407296));
#193318=CARTESIAN_POINT('',(112.205232059232,-0.299999999999985,66.0437652101105));
#193319=CARTESIAN_POINT('',(112.26287024287,-0.299999999999985,65.7472439407296));
#193320=CARTESIAN_POINT('Origin',(116.959178380441,-0.299999999999985,51.0204257716897));
#193321=CARTESIAN_POINT('Origin',(116.959178380441,-0.299999999999985,51.0204257716897));
#193322=CARTESIAN_POINT('Origin',(112.757435778548,-0.299999999999985,63.2029375247883));
#193323=CARTESIAN_POINT('Origin',(115.192249771263,1.45439216225896E-14,
50.6769679284724));
#193324=CARTESIAN_POINT('Origin',(115.192249771263,1.45439216225896E-14,
50.6769679284724));
#193325=CARTESIAN_POINT('Origin',(116.683943798944,-0.799999999999986,63.9661771763823));
#193326=CARTESIAN_POINT('',(116.708918664849,-0.799999999999986,66.4581022024784));
#193327=CARTESIAN_POINT('',(116.650720830459,-0.799999999999986,66.757502611017));
#193328=CARTESIAN_POINT('',(116.708918664849,-0.799999999999986,66.4581022024784));
#193329=CARTESIAN_POINT('',(116.202769740892,-0.799999999999986,66.4415907561147));
#193330=CARTESIAN_POINT('Origin',(116.959178380441,-0.799999999999986,51.0204257716897));
#193331=CARTESIAN_POINT('',(116.144871999832,-0.799999999999986,66.739447326016));
#193332=CARTESIAN_POINT('',(116.202769740892,-0.799999999999986,66.4415907561147));
#193333=CARTESIAN_POINT('Origin',(116.959178380441,-0.799999999999986,51.0204257716897));
#193334=CARTESIAN_POINT('Origin',(117.174757301493,-0.799999999999986,64.0615821328315));
#193335=CARTESIAN_POINT('',(116.705468970119,-0.299999999999985,66.4758492547892));
#193336=CARTESIAN_POINT('',(116.647338909772,-0.299999999999985,66.7749009978478));
#193337=CARTESIAN_POINT('',(116.705468970119,-0.299999999999985,66.4758492547892));
#193338=CARTESIAN_POINT('Origin',(119.609571294209,1.45439216225896E-14,
51.5356125365156));
#193339=CARTESIAN_POINT('Origin',(119.609571294209,1.45439216225896E-14,
51.5356125365156));
#193340=CARTESIAN_POINT('Origin',(117.174757301493,-0.299999999999985,64.0615821328315));
#193341=CARTESIAN_POINT('',(116.199338167008,-0.299999999999985,66.459244585223));
#193342=CARTESIAN_POINT('',(116.141507158036,-0.299999999999985,66.756757850005));
#193343=CARTESIAN_POINT('',(116.199338167008,-0.299999999999985,66.459244585223));
#193344=CARTESIAN_POINT('Origin',(116.959178380441,-0.299999999999985,51.0204257716897));
#193345=CARTESIAN_POINT('Origin',(116.959178380441,-0.299999999999985,51.0204257716897));
#193346=CARTESIAN_POINT('Origin',(116.683943798944,-0.299999999999985,63.9661771763823));
#193347=CARTESIAN_POINT('Origin',(119.118757791659,1.45439216225896E-14,
51.4402075800664));
#193348=CARTESIAN_POINT('Origin',(119.118757791659,1.45439216225896E-14,
51.4402075800664));
#193349=CARTESIAN_POINT('Origin',(115.702316793845,-0.799999999999986,63.7753672634838));
#193350=CARTESIAN_POINT('',(115.699807895975,-0.799999999999986,66.4086832913015));
#193351=CARTESIAN_POINT('',(115.642145714621,-0.799999999999986,66.7053280176139));
#193352=CARTESIAN_POINT('',(115.699807895975,-0.799999999999986,66.4086832913015));
#193353=CARTESIAN_POINT('',(115.199993583441,-0.799999999999986,66.3595832569304));
#193354=CARTESIAN_POINT('Origin',(116.959178380441,-0.799999999999986,51.0204257716897));
#193355=CARTESIAN_POINT('',(115.142504709642,-0.799999999999986,66.655336397614));
#193356=CARTESIAN_POINT('',(115.199993583441,-0.799999999999986,66.3595832569304));
#193357=CARTESIAN_POINT('Origin',(116.959178380441,-0.799999999999986,51.0204257716897));
#193358=CARTESIAN_POINT('Origin',(116.193130296394,-0.799999999999986,63.870772219933));
#193359=CARTESIAN_POINT('',(115.696390542482,-0.299999999999985,66.4262639632045));
#193360=CARTESIAN_POINT('',(115.638794282839,-0.299999999999985,66.7225695534067));
#193361=CARTESIAN_POINT('',(115.696390542482,-0.299999999999985,66.4262639632045));
#193362=CARTESIAN_POINT('Origin',(118.62794428911,1.45439216225896E-14,
51.3448026236171));
#193363=CARTESIAN_POINT('Origin',(118.62794428911,1.45439216225896E-14,
51.3448026236171));
#193364=CARTESIAN_POINT('Origin',(116.193130296394,-0.299999999999985,63.870772219933));
#193365=CARTESIAN_POINT('',(115.19658669022,-0.299999999999985,66.3771101156678));
#193366=CARTESIAN_POINT('',(115.139163146118,-0.299999999999985,66.6725271658766));
#193367=CARTESIAN_POINT('',(115.19658669022,-0.299999999999985,66.3771101156678));
#193368=CARTESIAN_POINT('Origin',(116.959178380441,-0.299999999999985,51.0204257716897));
#193369=CARTESIAN_POINT('Origin',(116.959178380441,-0.299999999999985,51.0204257716897));
#193370=CARTESIAN_POINT('Origin',(115.702316793845,-0.299999999999985,63.7753672634838));
#193371=CARTESIAN_POINT('Origin',(118.13713078656,1.45439216225896E-14,
51.2493976671679));
#193372=CARTESIAN_POINT('Origin',(118.13713078656,1.45439216225896E-14,
51.2493976671679));
#193373=CARTESIAN_POINT('Origin',(114.720689788746,-0.799999999999986,63.5845573505853));
#193374=CARTESIAN_POINT('',(114.703297924294,-0.799999999999986,66.2944392218165));
#193375=CARTESIAN_POINT('',(114.645921753038,-0.799999999999986,66.5896125610739));
#193376=CARTESIAN_POINT('',(114.703297924294,-0.799999999999986,66.2944392218165));
#193377=CARTESIAN_POINT('',(114.209702236559,-0.799999999999986,66.2133472959115));
#193378=CARTESIAN_POINT('Origin',(116.959178380441,-0.799999999999986,51.0204257716897));
#193379=CARTESIAN_POINT('',(114.152379219848,-0.799999999999986,66.5082471801045));
#193380=CARTESIAN_POINT('',(114.209702236559,-0.799999999999986,66.2133472959115));
#193381=CARTESIAN_POINT('Origin',(116.959178380441,-0.799999999999986,51.0204257716897));
#193382=CARTESIAN_POINT('Origin',(115.211503291295,-0.799999999999986,63.6799623070345));
#193383=CARTESIAN_POINT('',(114.6998978325,-0.299999999999985,66.3119310904201));
#193384=CARTESIAN_POINT('',(114.642586607859,-0.299999999999985,66.6067703099759));
#193385=CARTESIAN_POINT('',(114.6998978325,-0.299999999999985,66.3119310904201));
#193386=CARTESIAN_POINT('Origin',(117.64631728401,1.45439216225896E-14,
51.1539927107186));
#193387=CARTESIAN_POINT('Origin',(117.64631728401,1.45439216225896E-14,
51.1539927107186));
#193388=CARTESIAN_POINT('Origin',(115.211503291295,-0.299999999999985,63.6799623070345));
#193389=CARTESIAN_POINT('',(114.206305352308,-0.299999999999985,66.2308226632179));
#193390=CARTESIAN_POINT('',(114.149047102056,-0.299999999999985,66.5253893545321));
#193391=CARTESIAN_POINT('',(114.206305352308,-0.299999999999985,66.2308226632179));
#193392=CARTESIAN_POINT('Origin',(116.959178380441,-0.299999999999985,51.0204257716897));
#193393=CARTESIAN_POINT('Origin',(116.959178380441,-0.299999999999985,51.0204257716897));
#193394=CARTESIAN_POINT('Origin',(114.720689788746,-0.299999999999985,63.5845573505853));
#193395=CARTESIAN_POINT('Origin',(117.155503781461,1.45439216225896E-14,
51.0585877542694));
#193396=CARTESIAN_POINT('Origin',(117.155503781461,1.45439216225896E-14,
51.0585877542694));
#193397=CARTESIAN_POINT('Origin',(113.739062783647,-0.799999999999986,63.3937474376868));
#193398=CARTESIAN_POINT('',(113.719197735921,-0.799999999999986,66.116352670368));
#193399=CARTESIAN_POINT('',(113.661868820446,-0.799999999999986,66.4112829009218));
#193400=CARTESIAN_POINT('',(113.719197735921,-0.799999999999986,66.116352670368));
#193401=CARTESIAN_POINT('',(113.231785396369,-0.799999999999986,66.0034503344807));
#193402=CARTESIAN_POINT('Origin',(116.959178380441,-0.799999999999986,51.0204257716897));
#193403=CARTESIAN_POINT('',(113.17439147404,-0.799999999999986,66.2987149946358));
#193404=CARTESIAN_POINT('',(113.231785396369,-0.799999999999986,66.0034503344807));
#193405=CARTESIAN_POINT('Origin',(116.959178380441,-0.799999999999986,51.0204257716897));
#193406=CARTESIAN_POINT('Origin',(114.229876286196,-0.799999999999986,63.489152394136));
#193407=CARTESIAN_POINT('',(113.715800495726,-0.299999999999985,66.1338298688407));
#193408=CARTESIAN_POINT('',(113.658536366685,-0.299999999999985,66.4284268037491));
#193409=CARTESIAN_POINT('',(113.715800495726,-0.299999999999985,66.1338298688407));
#193410=CARTESIAN_POINT('Origin',(116.664690278911,1.45439216225896E-14,
50.9631827978201));
#193411=CARTESIAN_POINT('Origin',(116.664690278911,1.45439216225896E-14,
50.9631827978201));
#193412=CARTESIAN_POINT('Origin',(114.229876286196,-0.299999999999985,63.489152394136));
#193413=CARTESIAN_POINT('',(113.228384233372,-0.299999999999985,66.0209477139188));
#193414=CARTESIAN_POINT('',(113.171055317897,-0.299999999999985,66.3158779444725));
#193415=CARTESIAN_POINT('',(113.228384233372,-0.299999999999985,66.0209477139188));
#193416=CARTESIAN_POINT('Origin',(116.959178380441,-0.299999999999985,51.0204257716897));
#193417=CARTESIAN_POINT('Origin',(116.959178380441,-0.299999999999985,51.0204257716897));
#193418=CARTESIAN_POINT('Origin',(113.739062783647,-0.299999999999985,63.3937474376868));
#193419=CARTESIAN_POINT('Origin',(116.173876776362,1.45439216225896E-14,
50.8677778413709));
#193420=CARTESIAN_POINT('Origin',(116.173876776362,1.45439216225896E-14,
50.8677778413709));
#193421=CARTESIAN_POINT('Origin',(114.581607361595,1.45439216225896E-14,
63.2519072664759));
#193422=CARTESIAN_POINT('Origin',(108.407383728608,3.45,47.5859740823384));
#193423=CARTESIAN_POINT('',(108.898197231158,3.45,47.6813790387876));
#193424=CARTESIAN_POINT('',(108.840954257288,3.45,47.9758671403173));
#193425=CARTESIAN_POINT('',(108.898197231158,3.45,47.6813790387876));
#193426=CARTESIAN_POINT('',(108.350140754738,3.45,47.8804621838681));
#193427=CARTESIAN_POINT('',(108.350140754738,3.45,47.8804621838681));
#193428=CARTESIAN_POINT('',(108.407383728608,3.45,47.5859740823384));
#193429=CARTESIAN_POINT('',(108.407383728608,3.45,47.5859740823384));
#193430=CARTESIAN_POINT('',(108.407383728608,3.45,47.5859740823384));
#193431=CARTESIAN_POINT('Origin',(108.898197231158,3.45,47.6813790387876));
#193432=CARTESIAN_POINT('',(108.898197231158,2.95,47.6813790387876));
#193433=CARTESIAN_POINT('',(108.840954257288,2.95,47.9758671403173));
#193434=CARTESIAN_POINT('',(108.898197231158,2.95,47.6813790387876));
#193435=CARTESIAN_POINT('',(108.840954257288,3.45,47.9758671403173));
#193436=CARTESIAN_POINT('',(108.898197231158,3.45,47.6813790387876));
#193437=CARTESIAN_POINT('Origin',(108.898197231158,2.95,47.6813790387876));
#193438=CARTESIAN_POINT('',(108.407383728608,2.95,47.5859740823384));
#193439=CARTESIAN_POINT('',(108.350140754738,2.95,47.8804621838681));
#193440=CARTESIAN_POINT('',(108.407383728608,2.95,47.5859740823384));
#193441=CARTESIAN_POINT('',(108.840954257288,2.95,47.9758671403173));
#193442=CARTESIAN_POINT('',(108.898197231158,2.95,47.6813790387876));
#193443=CARTESIAN_POINT('Origin',(108.407383728608,2.95,47.5859740823384));
#193444=CARTESIAN_POINT('',(108.350140754738,2.95,47.8804621838681));
#193445=CARTESIAN_POINT('',(108.407383728608,2.95,47.5859740823384));
#193446=CARTESIAN_POINT('Origin',(108.407383728608,2.65,47.5859740823384));
#193447=CARTESIAN_POINT('',(108.898197231158,2.65,47.6813790387876));
#193448=CARTESIAN_POINT('',(108.840954257288,2.65,47.9758671403173));
#193449=CARTESIAN_POINT('',(108.898197231158,2.65,47.6813790387876));
#193450=CARTESIAN_POINT('',(108.350140754738,2.65,47.8804621838681));
#193451=CARTESIAN_POINT('',(108.350140754738,2.65,47.8804621838681));
#193452=CARTESIAN_POINT('',(108.407383728608,2.65,47.5859740823384));
#193453=CARTESIAN_POINT('',(108.407383728608,2.65,47.5859740823384));
#193454=CARTESIAN_POINT('',(108.407383728608,2.65,47.5859740823384));
#193455=CARTESIAN_POINT('Origin',(108.898197231158,2.65,47.6813790387876));
#193456=CARTESIAN_POINT('',(108.898197231158,2.15,47.6813790387876));
#193457=CARTESIAN_POINT('',(108.840954257288,2.15,47.9758671403173));
#193458=CARTESIAN_POINT('',(108.898197231158,2.15,47.6813790387876));
#193459=CARTESIAN_POINT('',(108.840954257288,2.65,47.9758671403173));
#193460=CARTESIAN_POINT('',(108.898197231158,2.65,47.6813790387876));
#193461=CARTESIAN_POINT('Origin',(108.898197231158,2.15,47.6813790387876));
#193462=CARTESIAN_POINT('',(108.407383728608,2.15,47.5859740823384));
#193463=CARTESIAN_POINT('',(108.350140754738,2.15,47.8804621838681));
#193464=CARTESIAN_POINT('',(108.407383728608,2.15,47.5859740823384));
#193465=CARTESIAN_POINT('',(108.840954257288,2.15,47.9758671403173));
#193466=CARTESIAN_POINT('',(108.898197231158,2.15,47.6813790387876));
#193467=CARTESIAN_POINT('Origin',(108.407383728608,2.15,47.5859740823384));
#193468=CARTESIAN_POINT('',(108.350140754738,2.15,47.8804621838681));
#193469=CARTESIAN_POINT('',(108.407383728608,2.15,47.5859740823384));
#193470=CARTESIAN_POINT('Origin',(108.407383728608,1.85,47.5859740823384));
#193471=CARTESIAN_POINT('',(108.898197231158,1.85,47.6813790387876));
#193472=CARTESIAN_POINT('',(108.840954257288,1.85,47.9758671403173));
#193473=CARTESIAN_POINT('',(108.898197231158,1.85,47.6813790387876));
#193474=CARTESIAN_POINT('',(108.350140754738,1.85,47.8804621838681));
#193475=CARTESIAN_POINT('',(108.350140754738,1.85,47.8804621838681));
#193476=CARTESIAN_POINT('',(108.407383728608,1.85,47.5859740823384));
#193477=CARTESIAN_POINT('',(108.407383728608,1.85,47.5859740823384));
#193478=CARTESIAN_POINT('',(108.407383728608,1.85,47.5859740823384));
#193479=CARTESIAN_POINT('Origin',(108.898197231158,1.85,47.6813790387876));
#193480=CARTESIAN_POINT('',(108.898197231158,1.35,47.6813790387876));
#193481=CARTESIAN_POINT('',(108.840954257288,1.35,47.9758671403173));
#193482=CARTESIAN_POINT('',(108.898197231158,1.35,47.6813790387876));
#193483=CARTESIAN_POINT('',(108.840954257288,1.85,47.9758671403173));
#193484=CARTESIAN_POINT('',(108.898197231158,1.85,47.6813790387876));
#193485=CARTESIAN_POINT('Origin',(108.898197231158,1.35,47.6813790387876));
#193486=CARTESIAN_POINT('',(108.407383728608,1.35,47.5859740823384));
#193487=CARTESIAN_POINT('',(108.350140754738,1.35,47.8804621838681));
#193488=CARTESIAN_POINT('',(108.407383728608,1.35,47.5859740823384));
#193489=CARTESIAN_POINT('',(108.840954257288,1.35,47.9758671403173));
#193490=CARTESIAN_POINT('',(108.898197231158,1.35,47.6813790387876));
#193491=CARTESIAN_POINT('Origin',(108.407383728608,1.35,47.5859740823384));
#193492=CARTESIAN_POINT('',(108.350140754738,1.35,47.8804621838681));
#193493=CARTESIAN_POINT('',(108.407383728608,1.35,47.5859740823384));
#193494=CARTESIAN_POINT('Origin',(108.407383728608,1.05,47.5859740823384));
#193495=CARTESIAN_POINT('',(108.898197231158,1.05,47.6813790387876));
#193496=CARTESIAN_POINT('',(108.840954257288,1.05,47.9758671403173));
#193497=CARTESIAN_POINT('',(108.898197231158,1.05,47.6813790387876));
#193498=CARTESIAN_POINT('',(108.350140754738,1.05,47.8804621838681));
#193499=CARTESIAN_POINT('',(108.350140754738,1.05,47.8804621838681));
#193500=CARTESIAN_POINT('',(108.407383728608,1.05,47.5859740823384));
#193501=CARTESIAN_POINT('',(108.407383728608,1.05,47.5859740823384));
#193502=CARTESIAN_POINT('',(108.407383728608,1.05,47.5859740823384));
#193503=CARTESIAN_POINT('Origin',(108.898197231158,1.05,47.6813790387876));
#193504=CARTESIAN_POINT('',(108.898197231158,0.550000000000015,47.6813790387876));
#193505=CARTESIAN_POINT('',(108.840954257288,0.550000000000015,47.9758671403173));
#193506=CARTESIAN_POINT('',(108.898197231158,0.550000000000015,47.6813790387876));
#193507=CARTESIAN_POINT('',(108.840954257288,1.05,47.9758671403173));
#193508=CARTESIAN_POINT('',(108.898197231158,1.05,47.6813790387876));
#193509=CARTESIAN_POINT('Origin',(108.898197231158,0.550000000000015,47.6813790387876));
#193510=CARTESIAN_POINT('',(108.407383728608,0.550000000000015,47.5859740823384));
#193511=CARTESIAN_POINT('',(108.350140754738,0.550000000000015,47.8804621838681));
#193512=CARTESIAN_POINT('',(108.407383728608,0.550000000000015,47.5859740823384));
#193513=CARTESIAN_POINT('',(108.840954257288,0.550000000000015,47.9758671403173));
#193514=CARTESIAN_POINT('',(108.898197231158,0.550000000000015,47.6813790387876));
#193515=CARTESIAN_POINT('Origin',(108.407383728608,0.550000000000015,47.5859740823384));
#193516=CARTESIAN_POINT('',(108.350140754738,0.550000000000015,47.8804621838681));
#193517=CARTESIAN_POINT('',(108.407383728608,0.550000000000015,47.5859740823384));
#193518=CARTESIAN_POINT('Origin',(108.407383728608,0.250000000000015,47.5859740823384));
#193519=CARTESIAN_POINT('',(108.898197231158,0.250000000000015,47.6813790387876));
#193520=CARTESIAN_POINT('',(108.840954257288,0.250000000000015,47.9758671403173));
#193521=CARTESIAN_POINT('',(108.898197231158,0.250000000000015,47.6813790387876));
#193522=CARTESIAN_POINT('',(108.350140754738,0.250000000000015,47.8804621838681));
#193523=CARTESIAN_POINT('',(108.350140754738,0.250000000000015,47.8804621838681));
#193524=CARTESIAN_POINT('',(108.407383728608,0.250000000000015,47.5859740823384));
#193525=CARTESIAN_POINT('',(108.407383728608,0.250000000000015,47.5859740823384));
#193526=CARTESIAN_POINT('',(108.407383728608,0.250000000000015,47.5859740823384));
#193527=CARTESIAN_POINT('Origin',(108.898197231158,0.250000000000015,47.6813790387876));
#193528=CARTESIAN_POINT('',(108.898197231158,-0.249999999999985,47.6813790387876));
#193529=CARTESIAN_POINT('',(108.840954257288,-0.249999999999985,47.9758671403173));
#193530=CARTESIAN_POINT('',(108.898197231158,-0.249999999999985,47.6813790387876));
#193531=CARTESIAN_POINT('',(108.840954257288,0.250000000000015,47.9758671403173));
#193532=CARTESIAN_POINT('',(108.898197231158,0.250000000000015,47.6813790387876));
#193533=CARTESIAN_POINT('Origin',(108.898197231158,-0.249999999999985,47.6813790387876));
#193534=CARTESIAN_POINT('',(108.407383728608,-0.249999999999985,47.5859740823384));
#193535=CARTESIAN_POINT('',(108.350140754738,-0.249999999999985,47.8804621838681));
#193536=CARTESIAN_POINT('',(108.407383728608,-0.249999999999985,47.5859740823384));
#193537=CARTESIAN_POINT('',(108.840954257288,-0.249999999999985,47.9758671403173));
#193538=CARTESIAN_POINT('',(108.898197231158,-0.249999999999985,47.6813790387876));
#193539=CARTESIAN_POINT('Origin',(108.407383728608,-0.249999999999985,47.5859740823384));
#193540=CARTESIAN_POINT('',(108.350140754738,-0.249999999999985,47.8804621838681));
#193541=CARTESIAN_POINT('',(108.407383728608,-0.249999999999985,47.5859740823384));
#193542=CARTESIAN_POINT('Origin',(108.407383728608,-0.549999999999986,47.5859740823384));
#193543=CARTESIAN_POINT('',(108.898197231158,-0.549999999999986,47.6813790387876));
#193544=CARTESIAN_POINT('',(108.840954257288,-0.549999999999986,47.9758671403173));
#193545=CARTESIAN_POINT('',(108.898197231158,-0.549999999999986,47.6813790387876));
#193546=CARTESIAN_POINT('',(108.350140754738,-0.549999999999986,47.8804621838681));
#193547=CARTESIAN_POINT('',(108.350140754738,-0.549999999999986,47.8804621838681));
#193548=CARTESIAN_POINT('',(108.407383728608,-0.549999999999986,47.5859740823384));
#193549=CARTESIAN_POINT('',(108.407383728608,-0.549999999999986,47.5859740823384));
#193550=CARTESIAN_POINT('',(108.407383728608,-0.549999999999986,47.5859740823384));
#193551=CARTESIAN_POINT('Origin',(108.898197231158,-0.549999999999986,47.6813790387876));
#193552=CARTESIAN_POINT('',(108.898197231158,-1.05,47.6813790387876));
#193553=CARTESIAN_POINT('',(108.840954257288,-1.05,47.9758671403173));
#193554=CARTESIAN_POINT('',(108.898197231158,-1.05,47.6813790387876));
#193555=CARTESIAN_POINT('',(108.840954257288,-0.549999999999986,47.9758671403173));
#193556=CARTESIAN_POINT('',(108.898197231158,-0.549999999999986,47.6813790387876));
#193557=CARTESIAN_POINT('Origin',(108.898197231158,-1.05,47.6813790387876));
#193558=CARTESIAN_POINT('',(108.407383728608,-1.05,47.5859740823384));
#193559=CARTESIAN_POINT('',(108.350140754738,-1.05,47.8804621838681));
#193560=CARTESIAN_POINT('',(108.407383728608,-1.05,47.5859740823384));
#193561=CARTESIAN_POINT('',(108.840954257288,-1.05,47.9758671403173));
#193562=CARTESIAN_POINT('',(108.898197231158,-1.05,47.6813790387876));
#193563=CARTESIAN_POINT('Origin',(108.407383728608,-1.05,47.5859740823384));
#193564=CARTESIAN_POINT('',(108.350140754738,-1.05,47.8804621838681));
#193565=CARTESIAN_POINT('',(108.407383728608,-1.05,47.5859740823384));
#193566=CARTESIAN_POINT('Origin',(108.407383728608,-1.35,47.5859740823384));
#193567=CARTESIAN_POINT('',(108.898197231158,-1.35,47.6813790387876));
#193568=CARTESIAN_POINT('',(108.840954257288,-1.35,47.9758671403173));
#193569=CARTESIAN_POINT('',(108.898197231158,-1.35,47.6813790387876));
#193570=CARTESIAN_POINT('',(108.350140754738,-1.35,47.8804621838681));
#193571=CARTESIAN_POINT('',(108.350140754738,-1.35,47.8804621838681));
#193572=CARTESIAN_POINT('',(108.407383728608,-1.35,47.5859740823384));
#193573=CARTESIAN_POINT('',(108.407383728608,-1.35,47.5859740823384));
#193574=CARTESIAN_POINT('',(108.407383728608,-1.35,47.5859740823384));
#193575=CARTESIAN_POINT('Origin',(108.898197231158,-1.35,47.6813790387876));
#193576=CARTESIAN_POINT('',(108.898197231158,-1.85,47.6813790387876));
#193577=CARTESIAN_POINT('',(108.840954257288,-1.85,47.9758671403173));
#193578=CARTESIAN_POINT('',(108.898197231158,-1.85,47.6813790387876));
#193579=CARTESIAN_POINT('',(108.840954257288,-1.35,47.9758671403173));
#193580=CARTESIAN_POINT('',(108.898197231158,-1.35,47.6813790387876));
#193581=CARTESIAN_POINT('Origin',(108.898197231158,-1.85,47.6813790387876));
#193582=CARTESIAN_POINT('',(108.407383728608,-1.85,47.5859740823384));
#193583=CARTESIAN_POINT('',(108.350140754738,-1.85,47.8804621838681));
#193584=CARTESIAN_POINT('',(108.407383728608,-1.85,47.5859740823384));
#193585=CARTESIAN_POINT('',(108.840954257288,-1.85,47.9758671403173));
#193586=CARTESIAN_POINT('',(108.898197231158,-1.85,47.6813790387876));
#193587=CARTESIAN_POINT('Origin',(108.407383728608,-1.85,47.5859740823384));
#193588=CARTESIAN_POINT('',(108.350140754738,-1.85,47.8804621838681));
#193589=CARTESIAN_POINT('',(108.407383728608,-1.85,47.5859740823384));
#193590=CARTESIAN_POINT('Origin',(108.407383728608,-2.15,47.5859740823384));
#193591=CARTESIAN_POINT('',(108.898197231158,-2.15,47.6813790387876));
#193592=CARTESIAN_POINT('',(108.840954257288,-2.15,47.9758671403173));
#193593=CARTESIAN_POINT('',(108.898197231158,-2.15,47.6813790387876));
#193594=CARTESIAN_POINT('',(108.350140754738,-2.15,47.8804621838681));
#193595=CARTESIAN_POINT('',(108.350140754738,-2.15,47.8804621838681));
#193596=CARTESIAN_POINT('',(108.407383728608,-2.15,47.5859740823384));
#193597=CARTESIAN_POINT('',(108.407383728608,-2.15,47.5859740823384));
#193598=CARTESIAN_POINT('',(108.407383728608,-2.15,47.5859740823384));
#193599=CARTESIAN_POINT('Origin',(108.898197231158,-2.15,47.6813790387876));
#193600=CARTESIAN_POINT('',(108.898197231158,-2.65,47.6813790387876));
#193601=CARTESIAN_POINT('',(108.840954257288,-2.65,47.9758671403173));
#193602=CARTESIAN_POINT('',(108.898197231158,-2.65,47.6813790387876));
#193603=CARTESIAN_POINT('',(108.840954257288,-2.15,47.9758671403173));
#193604=CARTESIAN_POINT('',(108.898197231158,-2.15,47.6813790387876));
#193605=CARTESIAN_POINT('Origin',(108.898197231158,-2.65,47.6813790387876));
#193606=CARTESIAN_POINT('',(108.407383728608,-2.65,47.5859740823384));
#193607=CARTESIAN_POINT('',(108.350140754738,-2.65,47.8804621838681));
#193608=CARTESIAN_POINT('',(108.407383728608,-2.65,47.5859740823384));
#193609=CARTESIAN_POINT('',(108.840954257288,-2.65,47.9758671403173));
#193610=CARTESIAN_POINT('',(108.898197231158,-2.65,47.6813790387876));
#193611=CARTESIAN_POINT('Origin',(108.407383728608,-2.65,47.5859740823384));
#193612=CARTESIAN_POINT('',(108.350140754738,-2.65,47.8804621838681));
#193613=CARTESIAN_POINT('',(108.407383728608,-2.65,47.5859740823384));
#193614=CARTESIAN_POINT('Origin',(108.407383728608,-2.95,47.5859740823384));
#193615=CARTESIAN_POINT('',(108.898197231158,-2.95,47.6813790387876));
#193616=CARTESIAN_POINT('',(108.840954257288,-2.95,47.9758671403173));
#193617=CARTESIAN_POINT('',(108.898197231158,-2.95,47.6813790387876));
#193618=CARTESIAN_POINT('',(108.350140754738,-2.95,47.8804621838681));
#193619=CARTESIAN_POINT('',(108.350140754738,-2.95,47.8804621838681));
#193620=CARTESIAN_POINT('',(108.407383728608,-2.95,47.5859740823384));
#193621=CARTESIAN_POINT('',(108.407383728608,-2.95,47.5859740823384));
#193622=CARTESIAN_POINT('',(108.407383728608,-2.95,47.5859740823384));
#193623=CARTESIAN_POINT('Origin',(108.898197231158,-2.95,47.6813790387876));
#193624=CARTESIAN_POINT('',(108.898197231158,-3.45,47.6813790387876));
#193625=CARTESIAN_POINT('',(108.840954257288,-3.45,47.9758671403173));
#193626=CARTESIAN_POINT('',(108.898197231158,-3.45,47.6813790387876));
#193627=CARTESIAN_POINT('',(108.840954257288,-2.95,47.9758671403173));
#193628=CARTESIAN_POINT('',(108.898197231158,-2.95,47.6813790387876));
#193629=CARTESIAN_POINT('Origin',(108.898197231158,-3.45,47.6813790387876));
#193630=CARTESIAN_POINT('',(108.407383728608,-3.45,47.5859740823384));
#193631=CARTESIAN_POINT('',(108.350140754738,-3.45,47.8804621838681));
#193632=CARTESIAN_POINT('',(108.407383728608,-3.45,47.5859740823384));
#193633=CARTESIAN_POINT('',(108.840954257288,-3.45,47.9758671403173));
#193634=CARTESIAN_POINT('',(108.898197231158,-3.45,47.6813790387876));
#193635=CARTESIAN_POINT('Origin',(108.407383728608,-3.45,47.5859740823384));
#193636=CARTESIAN_POINT('',(108.350140754738,-3.45,47.8804621838681));
#193637=CARTESIAN_POINT('',(108.407383728608,-3.45,47.5859740823384));
#193638=CARTESIAN_POINT('Origin',(113.904494957163,-8.55,48.65450959457));
#193639=CARTESIAN_POINT('',(114.395308459712,-8.55,48.7499145510193));
#193640=CARTESIAN_POINT('',(114.338065485842,-8.55,49.044402652549));
#193641=CARTESIAN_POINT('',(114.395308459712,-8.55,48.7499145510193));
#193642=CARTESIAN_POINT('',(113.847251983293,-8.55,48.9489976960997));
#193643=CARTESIAN_POINT('',(113.847251983293,-8.55,48.9489976960997));
#193644=CARTESIAN_POINT('',(113.904494957163,-8.55,48.65450959457));
#193645=CARTESIAN_POINT('',(113.904494957163,-8.55,48.65450959457));
#193646=CARTESIAN_POINT('',(113.904494957163,-8.55,48.65450959457));
#193647=CARTESIAN_POINT('Origin',(114.395308459712,-8.55,48.7499145510193));
#193648=CARTESIAN_POINT('',(114.395308459712,-9.05,48.7499145510193));
#193649=CARTESIAN_POINT('',(114.338065485842,-9.05,49.044402652549));
#193650=CARTESIAN_POINT('',(114.395308459712,-9.05,48.7499145510193));
#193651=CARTESIAN_POINT('',(114.338065485842,-8.55,49.044402652549));
#193652=CARTESIAN_POINT('',(114.395308459712,-8.55,48.7499145510193));
#193653=CARTESIAN_POINT('Origin',(114.395308459712,-9.05,48.7499145510193));
#193654=CARTESIAN_POINT('',(113.904494957163,-9.05,48.65450959457));
#193655=CARTESIAN_POINT('',(113.847251983293,-9.05,48.9489976960997));
#193656=CARTESIAN_POINT('',(113.904494957163,-9.05,48.65450959457));
#193657=CARTESIAN_POINT('',(114.338065485842,-9.05,49.044402652549));
#193658=CARTESIAN_POINT('',(114.395308459712,-9.05,48.7499145510193));
#193659=CARTESIAN_POINT('Origin',(113.904494957163,-9.05,48.65450959457));
#193660=CARTESIAN_POINT('',(113.847251983293,-9.05,48.9489976960997));
#193661=CARTESIAN_POINT('',(113.904494957163,-9.05,48.65450959457));
#193662=CARTESIAN_POINT('Origin',(114.689796561242,-8.55,48.8071575248888));
#193663=CARTESIAN_POINT('',(115.180610063791,-8.55,48.9025624813381));
#193664=CARTESIAN_POINT('',(115.123367089922,-8.55,49.1970505828678));
#193665=CARTESIAN_POINT('',(115.180610063791,-8.55,48.9025624813381));
#193666=CARTESIAN_POINT('',(114.632553587372,-8.55,49.1016456264185));
#193667=CARTESIAN_POINT('',(114.632553587372,-8.55,49.1016456264185));
#193668=CARTESIAN_POINT('',(114.689796561242,-8.55,48.8071575248888));
#193669=CARTESIAN_POINT('',(114.689796561242,-8.55,48.8071575248888));
#193670=CARTESIAN_POINT('',(114.689796561242,-8.55,48.8071575248888));
#193671=CARTESIAN_POINT('Origin',(115.180610063791,-8.55,48.9025624813381));
#193672=CARTESIAN_POINT('',(115.180610063791,-9.05,48.9025624813381));
#193673=CARTESIAN_POINT('',(115.123367089922,-9.05,49.1970505828678));
#193674=CARTESIAN_POINT('',(115.180610063791,-9.05,48.9025624813381));
#193675=CARTESIAN_POINT('',(115.123367089922,-8.55,49.1970505828678));
#193676=CARTESIAN_POINT('',(115.180610063791,-8.55,48.9025624813381));
#193677=CARTESIAN_POINT('Origin',(115.180610063791,-9.05,48.9025624813381));
#193678=CARTESIAN_POINT('',(114.689796561242,-9.05,48.8071575248888));
#193679=CARTESIAN_POINT('',(114.632553587372,-9.05,49.1016456264185));
#193680=CARTESIAN_POINT('',(114.689796561242,-9.05,48.8071575248888));
#193681=CARTESIAN_POINT('',(115.123367089922,-9.05,49.1970505828678));
#193682=CARTESIAN_POINT('',(115.180610063791,-9.05,48.9025624813381));
#193683=CARTESIAN_POINT('Origin',(114.689796561242,-9.05,48.8071575248888));
#193684=CARTESIAN_POINT('',(114.632553587372,-9.05,49.1016456264185));
#193685=CARTESIAN_POINT('',(114.689796561242,-9.05,48.8071575248888));
#193686=CARTESIAN_POINT('Origin',(115.475098165321,-8.55,48.9598054552076));
#193687=CARTESIAN_POINT('',(115.96591166787,-8.55,49.0552104116569));
#193688=CARTESIAN_POINT('',(115.908668694001,-8.55,49.3496985131866));
#193689=CARTESIAN_POINT('',(115.96591166787,-8.55,49.0552104116569));
#193690=CARTESIAN_POINT('',(115.417855191451,-8.55,49.2542935567373));
#193691=CARTESIAN_POINT('',(115.417855191451,-8.55,49.2542935567373));
#193692=CARTESIAN_POINT('',(115.475098165321,-8.55,48.9598054552076));
#193693=CARTESIAN_POINT('',(115.475098165321,-8.55,48.9598054552076));
#193694=CARTESIAN_POINT('',(115.475098165321,-8.55,48.9598054552076));
#193695=CARTESIAN_POINT('Origin',(115.96591166787,-8.55,49.0552104116569));
#193696=CARTESIAN_POINT('',(115.96591166787,-9.05,49.0552104116569));
#193697=CARTESIAN_POINT('',(115.908668694001,-9.05,49.3496985131866));
#193698=CARTESIAN_POINT('',(115.96591166787,-9.05,49.0552104116569));
#193699=CARTESIAN_POINT('',(115.908668694001,-8.55,49.3496985131866));
#193700=CARTESIAN_POINT('',(115.96591166787,-8.55,49.0552104116569));
#193701=CARTESIAN_POINT('Origin',(115.96591166787,-9.05,49.0552104116569));
#193702=CARTESIAN_POINT('',(115.475098165321,-9.05,48.9598054552076));
#193703=CARTESIAN_POINT('',(115.417855191451,-9.05,49.2542935567373));
#193704=CARTESIAN_POINT('',(115.475098165321,-9.05,48.9598054552076));
#193705=CARTESIAN_POINT('',(115.908668694001,-9.05,49.3496985131866));
#193706=CARTESIAN_POINT('',(115.96591166787,-9.05,49.0552104116569));
#193707=CARTESIAN_POINT('Origin',(115.475098165321,-9.05,48.9598054552076));
#193708=CARTESIAN_POINT('',(115.417855191451,-9.05,49.2542935567373));
#193709=CARTESIAN_POINT('',(115.475098165321,-9.05,48.9598054552076));
#193710=CARTESIAN_POINT('Origin',(116.2603997694,-8.55,49.1124533855264));
#193711=CARTESIAN_POINT('',(116.75121327195,-8.55,49.2078583419757));
#193712=CARTESIAN_POINT('',(116.69397029808,-8.55,49.5023464435054));
#193713=CARTESIAN_POINT('',(116.75121327195,-8.55,49.2078583419757));
#193714=CARTESIAN_POINT('',(116.203156795531,-8.55,49.4069414870561));
#193715=CARTESIAN_POINT('',(116.203156795531,-8.55,49.4069414870561));
#193716=CARTESIAN_POINT('',(116.2603997694,-8.55,49.1124533855264));
#193717=CARTESIAN_POINT('',(116.2603997694,-8.55,49.1124533855264));
#193718=CARTESIAN_POINT('',(116.2603997694,-8.55,49.1124533855264));
#193719=CARTESIAN_POINT('Origin',(116.75121327195,-8.55,49.2078583419757));
#193720=CARTESIAN_POINT('',(116.75121327195,-9.05,49.2078583419757));
#193721=CARTESIAN_POINT('',(116.69397029808,-9.05,49.5023464435054));
#193722=CARTESIAN_POINT('',(116.75121327195,-9.05,49.2078583419757));
#193723=CARTESIAN_POINT('',(116.69397029808,-8.55,49.5023464435054));
#193724=CARTESIAN_POINT('',(116.75121327195,-8.55,49.2078583419757));
#193725=CARTESIAN_POINT('Origin',(116.75121327195,-9.05,49.2078583419757));
#193726=CARTESIAN_POINT('',(116.2603997694,-9.05,49.1124533855264));
#193727=CARTESIAN_POINT('',(116.203156795531,-9.05,49.4069414870561));
#193728=CARTESIAN_POINT('',(116.2603997694,-9.05,49.1124533855264));
#193729=CARTESIAN_POINT('',(116.69397029808,-9.05,49.5023464435054));
#193730=CARTESIAN_POINT('',(116.75121327195,-9.05,49.2078583419757));
#193731=CARTESIAN_POINT('Origin',(116.2603997694,-9.05,49.1124533855264));
#193732=CARTESIAN_POINT('',(116.203156795531,-9.05,49.4069414870561));
#193733=CARTESIAN_POINT('',(116.2603997694,-9.05,49.1124533855264));
#193734=CARTESIAN_POINT('Origin',(117.045701373479,-8.55,49.2651013158452));
#193735=CARTESIAN_POINT('',(117.536514876029,-8.55,49.3605062722945));
#193736=CARTESIAN_POINT('',(117.479271902159,-8.55,49.6549943738242));
#193737=CARTESIAN_POINT('',(117.536514876029,-8.55,49.3605062722945));
#193738=CARTESIAN_POINT('',(116.98845839961,-8.55,49.5595894173749));
#193739=CARTESIAN_POINT('',(116.98845839961,-8.55,49.5595894173749));
#193740=CARTESIAN_POINT('',(117.045701373479,-8.55,49.2651013158452));
#193741=CARTESIAN_POINT('',(117.045701373479,-8.55,49.2651013158452));
#193742=CARTESIAN_POINT('',(117.045701373479,-8.55,49.2651013158452));
#193743=CARTESIAN_POINT('Origin',(117.536514876029,-8.55,49.3605062722945));
#193744=CARTESIAN_POINT('',(117.536514876029,-9.05,49.3605062722945));
#193745=CARTESIAN_POINT('',(117.479271902159,-9.05,49.6549943738242));
#193746=CARTESIAN_POINT('',(117.536514876029,-9.05,49.3605062722945));
#193747=CARTESIAN_POINT('',(117.479271902159,-8.55,49.6549943738242));
#193748=CARTESIAN_POINT('',(117.536514876029,-8.55,49.3605062722945));
#193749=CARTESIAN_POINT('Origin',(117.536514876029,-9.05,49.3605062722945));
#193750=CARTESIAN_POINT('',(117.045701373479,-9.05,49.2651013158452));
#193751=CARTESIAN_POINT('',(116.98845839961,-9.05,49.5595894173749));
#193752=CARTESIAN_POINT('',(117.045701373479,-9.05,49.2651013158452));
#193753=CARTESIAN_POINT('',(117.479271902159,-9.05,49.6549943738242));
#193754=CARTESIAN_POINT('',(117.536514876029,-9.05,49.3605062722945));
#193755=CARTESIAN_POINT('Origin',(117.045701373479,-9.05,49.2651013158452));
#193756=CARTESIAN_POINT('',(116.98845839961,-9.05,49.5595894173749));
#193757=CARTESIAN_POINT('',(117.045701373479,-9.05,49.2651013158452));
#193758=CARTESIAN_POINT('Origin',(117.831002977559,-8.55,49.417749246164));
#193759=CARTESIAN_POINT('',(118.321816480108,-8.55,49.5131542026133));
#193760=CARTESIAN_POINT('',(118.264573506239,-8.55,49.807642304143));
#193761=CARTESIAN_POINT('',(118.321816480108,-8.55,49.5131542026133));
#193762=CARTESIAN_POINT('',(117.773760003689,-8.55,49.7122373476937));
#193763=CARTESIAN_POINT('',(117.773760003689,-8.55,49.7122373476937));
#193764=CARTESIAN_POINT('',(117.831002977559,-8.55,49.417749246164));
#193765=CARTESIAN_POINT('',(117.831002977559,-8.55,49.417749246164));
#193766=CARTESIAN_POINT('',(117.831002977559,-8.55,49.417749246164));
#193767=CARTESIAN_POINT('Origin',(118.321816480108,-8.55,49.5131542026133));
#193768=CARTESIAN_POINT('',(118.321816480108,-9.05,49.5131542026133));
#193769=CARTESIAN_POINT('',(118.264573506239,-9.05,49.807642304143));
#193770=CARTESIAN_POINT('',(118.321816480108,-9.05,49.5131542026133));
#193771=CARTESIAN_POINT('',(118.264573506239,-8.55,49.807642304143));
#193772=CARTESIAN_POINT('',(118.321816480108,-8.55,49.5131542026133));
#193773=CARTESIAN_POINT('Origin',(118.321816480108,-9.05,49.5131542026133));
#193774=CARTESIAN_POINT('',(117.831002977559,-9.05,49.417749246164));
#193775=CARTESIAN_POINT('',(117.773760003689,-9.05,49.7122373476937));
#193776=CARTESIAN_POINT('',(117.831002977559,-9.05,49.417749246164));
#193777=CARTESIAN_POINT('',(118.264573506239,-9.05,49.807642304143));
#193778=CARTESIAN_POINT('',(118.321816480108,-9.05,49.5131542026133));
#193779=CARTESIAN_POINT('Origin',(117.831002977559,-9.05,49.417749246164));
#193780=CARTESIAN_POINT('',(117.773760003689,-9.05,49.7122373476937));
#193781=CARTESIAN_POINT('',(117.831002977559,-9.05,49.417749246164));
#193782=CARTESIAN_POINT('Origin',(118.616304581638,-8.55,49.5703971764828));
#193783=CARTESIAN_POINT('',(119.107118084187,-8.55,49.6658021329321));
#193784=CARTESIAN_POINT('',(119.049875110318,-8.55,49.9602902344618));
#193785=CARTESIAN_POINT('',(119.107118084187,-8.55,49.6658021329321));
#193786=CARTESIAN_POINT('',(118.559061607768,-8.55,49.8648852780125));
#193787=CARTESIAN_POINT('',(118.559061607768,-8.55,49.8648852780125));
#193788=CARTESIAN_POINT('',(118.616304581638,-8.55,49.5703971764828));
#193789=CARTESIAN_POINT('',(118.616304581638,-8.55,49.5703971764828));
#193790=CARTESIAN_POINT('',(118.616304581638,-8.55,49.5703971764828));
#193791=CARTESIAN_POINT('Origin',(119.107118084187,-8.55,49.6658021329321));
#193792=CARTESIAN_POINT('',(119.107118084187,-9.05,49.6658021329321));
#193793=CARTESIAN_POINT('',(119.049875110318,-9.05,49.9602902344618));
#193794=CARTESIAN_POINT('',(119.107118084187,-9.05,49.6658021329321));
#193795=CARTESIAN_POINT('',(119.049875110318,-8.55,49.9602902344618));
#193796=CARTESIAN_POINT('',(119.107118084187,-8.55,49.6658021329321));
#193797=CARTESIAN_POINT('Origin',(119.107118084187,-9.05,49.6658021329321));
#193798=CARTESIAN_POINT('',(118.616304581638,-9.05,49.5703971764828));
#193799=CARTESIAN_POINT('',(118.559061607768,-9.05,49.8648852780125));
#193800=CARTESIAN_POINT('',(118.616304581638,-9.05,49.5703971764828));
#193801=CARTESIAN_POINT('',(119.049875110318,-9.05,49.9602902344618));
#193802=CARTESIAN_POINT('',(119.107118084187,-9.05,49.6658021329321));
#193803=CARTESIAN_POINT('Origin',(118.616304581638,-9.05,49.5703971764828));
#193804=CARTESIAN_POINT('',(118.559061607768,-9.05,49.8648852780125));
#193805=CARTESIAN_POINT('',(118.616304581638,-9.05,49.5703971764828));
#193806=CARTESIAN_POINT('Origin',(119.401606185717,-8.55,49.7230451068016));
#193807=CARTESIAN_POINT('',(119.892419688267,-8.55,49.8184500632509));
#193808=CARTESIAN_POINT('',(119.835176714397,-8.55,50.1129381647806));
#193809=CARTESIAN_POINT('',(119.892419688267,-8.55,49.8184500632509));
#193810=CARTESIAN_POINT('',(119.344363211847,-8.55,50.0175332083313));
#193811=CARTESIAN_POINT('',(119.344363211847,-8.55,50.0175332083313));
#193812=CARTESIAN_POINT('',(119.401606185717,-8.55,49.7230451068016));
#193813=CARTESIAN_POINT('',(119.401606185717,-8.55,49.7230451068016));
#193814=CARTESIAN_POINT('',(119.401606185717,-8.55,49.7230451068016));
#193815=CARTESIAN_POINT('Origin',(119.892419688267,-8.55,49.8184500632509));
#193816=CARTESIAN_POINT('',(119.892419688267,-9.05,49.8184500632509));
#193817=CARTESIAN_POINT('',(119.835176714397,-9.05,50.1129381647806));
#193818=CARTESIAN_POINT('',(119.892419688267,-9.05,49.8184500632509));
#193819=CARTESIAN_POINT('',(119.835176714397,-8.55,50.1129381647806));
#193820=CARTESIAN_POINT('',(119.892419688267,-8.55,49.8184500632509));
#193821=CARTESIAN_POINT('Origin',(119.892419688267,-9.05,49.8184500632509));
#193822=CARTESIAN_POINT('',(119.401606185717,-9.05,49.7230451068016));
#193823=CARTESIAN_POINT('',(119.344363211847,-9.05,50.0175332083313));
#193824=CARTESIAN_POINT('',(119.401606185717,-9.05,49.7230451068016));
#193825=CARTESIAN_POINT('',(119.835176714397,-9.05,50.1129381647806));
#193826=CARTESIAN_POINT('',(119.892419688267,-9.05,49.8184500632509));
#193827=CARTESIAN_POINT('Origin',(119.401606185717,-9.05,49.7230451068016));
#193828=CARTESIAN_POINT('',(119.344363211847,-9.05,50.0175332083313));
#193829=CARTESIAN_POINT('',(119.401606185717,-9.05,49.7230451068016));
#193830=CARTESIAN_POINT('Origin',(120.186907789796,-8.55,49.8756930371204));
#193831=CARTESIAN_POINT('',(120.677721292346,-8.55,49.9710979935697));
#193832=CARTESIAN_POINT('',(120.620478318476,-8.55,50.2655860950994));
#193833=CARTESIAN_POINT('',(120.677721292346,-8.55,49.9710979935697));
#193834=CARTESIAN_POINT('',(120.129664815927,-8.55,50.1701811386501));
#193835=CARTESIAN_POINT('',(120.129664815927,-8.55,50.1701811386501));
#193836=CARTESIAN_POINT('',(120.186907789796,-8.55,49.8756930371204));
#193837=CARTESIAN_POINT('',(120.186907789796,-8.55,49.8756930371204));
#193838=CARTESIAN_POINT('',(120.186907789796,-8.55,49.8756930371204));
#193839=CARTESIAN_POINT('Origin',(120.677721292346,-8.55,49.9710979935697));
#193840=CARTESIAN_POINT('',(120.677721292346,-9.05,49.9710979935697));
#193841=CARTESIAN_POINT('',(120.620478318476,-9.05,50.2655860950994));
#193842=CARTESIAN_POINT('',(120.677721292346,-9.05,49.9710979935697));
#193843=CARTESIAN_POINT('',(120.620478318476,-8.55,50.2655860950994));
#193844=CARTESIAN_POINT('',(120.677721292346,-8.55,49.9710979935697));
#193845=CARTESIAN_POINT('Origin',(120.677721292346,-9.05,49.9710979935697));
#193846=CARTESIAN_POINT('',(120.186907789796,-9.05,49.8756930371204));
#193847=CARTESIAN_POINT('',(120.129664815927,-9.05,50.1701811386501));
#193848=CARTESIAN_POINT('',(120.186907789796,-9.05,49.8756930371204));
#193849=CARTESIAN_POINT('',(120.620478318476,-9.05,50.2655860950994));
#193850=CARTESIAN_POINT('',(120.677721292346,-9.05,49.9710979935697));
#193851=CARTESIAN_POINT('Origin',(120.186907789796,-9.05,49.8756930371204));
#193852=CARTESIAN_POINT('',(120.129664815927,-9.05,50.1701811386501));
#193853=CARTESIAN_POINT('',(120.186907789796,-9.05,49.8756930371204));
#193854=CARTESIAN_POINT('Origin',(125.684019018351,-2.95,50.944228549352));
#193855=CARTESIAN_POINT('',(126.1748325209,-2.95,51.0396335058013));
#193856=CARTESIAN_POINT('',(126.117589547031,-2.95,51.334121607331));
#193857=CARTESIAN_POINT('',(126.1748325209,-2.95,51.0396335058013));
#193858=CARTESIAN_POINT('',(125.626776044481,-2.95,51.2387166508817));
#193859=CARTESIAN_POINT('',(125.626776044481,-2.95,51.2387166508817));
#193860=CARTESIAN_POINT('',(125.684019018351,-2.95,50.944228549352));
#193861=CARTESIAN_POINT('',(125.684019018351,-2.95,50.944228549352));
#193862=CARTESIAN_POINT('',(125.684019018351,-2.95,50.944228549352));
#193863=CARTESIAN_POINT('Origin',(126.1748325209,-2.95,51.0396335058013));
#193864=CARTESIAN_POINT('',(126.1748325209,-3.45,51.0396335058013));
#193865=CARTESIAN_POINT('',(126.117589547031,-3.45,51.334121607331));
#193866=CARTESIAN_POINT('',(126.1748325209,-3.45,51.0396335058013));
#193867=CARTESIAN_POINT('',(126.117589547031,-2.95,51.334121607331));
#193868=CARTESIAN_POINT('',(126.1748325209,-2.95,51.0396335058013));
#193869=CARTESIAN_POINT('Origin',(126.1748325209,-3.45,51.0396335058013));
#193870=CARTESIAN_POINT('',(125.684019018351,-3.45,50.944228549352));
#193871=CARTESIAN_POINT('',(125.626776044481,-3.45,51.2387166508817));
#193872=CARTESIAN_POINT('',(125.684019018351,-3.45,50.944228549352));
#193873=CARTESIAN_POINT('',(126.117589547031,-3.45,51.334121607331));
#193874=CARTESIAN_POINT('',(126.1748325209,-3.45,51.0396335058013));
#193875=CARTESIAN_POINT('Origin',(125.684019018351,-3.45,50.944228549352));
#193876=CARTESIAN_POINT('',(125.626776044481,-3.45,51.2387166508817));
#193877=CARTESIAN_POINT('',(125.684019018351,-3.45,50.944228549352));
#193878=CARTESIAN_POINT('Origin',(125.684019018351,-2.15,50.944228549352));
#193879=CARTESIAN_POINT('',(126.1748325209,-2.15,51.0396335058013));
#193880=CARTESIAN_POINT('',(126.117589547031,-2.15,51.334121607331));
#193881=CARTESIAN_POINT('',(126.1748325209,-2.15,51.0396335058013));
#193882=CARTESIAN_POINT('',(125.626776044481,-2.15,51.2387166508817));
#193883=CARTESIAN_POINT('',(125.626776044481,-2.15,51.2387166508817));
#193884=CARTESIAN_POINT('',(125.684019018351,-2.15,50.944228549352));
#193885=CARTESIAN_POINT('',(125.684019018351,-2.15,50.944228549352));
#193886=CARTESIAN_POINT('',(125.684019018351,-2.15,50.944228549352));
#193887=CARTESIAN_POINT('Origin',(126.1748325209,-2.15,51.0396335058013));
#193888=CARTESIAN_POINT('',(126.1748325209,-2.65,51.0396335058013));
#193889=CARTESIAN_POINT('',(126.117589547031,-2.65,51.334121607331));
#193890=CARTESIAN_POINT('',(126.1748325209,-2.65,51.0396335058013));
#193891=CARTESIAN_POINT('',(126.117589547031,-2.15,51.334121607331));
#193892=CARTESIAN_POINT('',(126.1748325209,-2.15,51.0396335058013));
#193893=CARTESIAN_POINT('Origin',(126.1748325209,-2.65,51.0396335058013));
#193894=CARTESIAN_POINT('',(125.684019018351,-2.65,50.944228549352));
#193895=CARTESIAN_POINT('',(125.626776044481,-2.65,51.2387166508817));
#193896=CARTESIAN_POINT('',(125.684019018351,-2.65,50.944228549352));
#193897=CARTESIAN_POINT('',(126.117589547031,-2.65,51.334121607331));
#193898=CARTESIAN_POINT('',(126.1748325209,-2.65,51.0396335058013));
#193899=CARTESIAN_POINT('Origin',(125.684019018351,-2.65,50.944228549352));
#193900=CARTESIAN_POINT('',(125.626776044481,-2.65,51.2387166508817));
#193901=CARTESIAN_POINT('',(125.684019018351,-2.65,50.944228549352));
#193902=CARTESIAN_POINT('Origin',(125.684019018351,-1.35,50.944228549352));
#193903=CARTESIAN_POINT('',(126.1748325209,-1.35,51.0396335058013));
#193904=CARTESIAN_POINT('',(126.117589547031,-1.35,51.334121607331));
#193905=CARTESIAN_POINT('',(126.1748325209,-1.35,51.0396335058013));
#193906=CARTESIAN_POINT('',(125.626776044481,-1.35,51.2387166508817));
#193907=CARTESIAN_POINT('',(125.626776044481,-1.35,51.2387166508817));
#193908=CARTESIAN_POINT('',(125.684019018351,-1.35,50.944228549352));
#193909=CARTESIAN_POINT('',(125.684019018351,-1.35,50.944228549352));
#193910=CARTESIAN_POINT('',(125.684019018351,-1.35,50.944228549352));
#193911=CARTESIAN_POINT('Origin',(126.1748325209,-1.35,51.0396335058013));
#193912=CARTESIAN_POINT('',(126.1748325209,-1.85,51.0396335058013));
#193913=CARTESIAN_POINT('',(126.117589547031,-1.85,51.334121607331));
#193914=CARTESIAN_POINT('',(126.1748325209,-1.85,51.0396335058013));
#193915=CARTESIAN_POINT('',(126.117589547031,-1.35,51.334121607331));
#193916=CARTESIAN_POINT('',(126.1748325209,-1.35,51.0396335058013));
#193917=CARTESIAN_POINT('Origin',(126.1748325209,-1.85,51.0396335058013));
#193918=CARTESIAN_POINT('',(125.684019018351,-1.85,50.944228549352));
#193919=CARTESIAN_POINT('',(125.626776044481,-1.85,51.2387166508817));
#193920=CARTESIAN_POINT('',(125.684019018351,-1.85,50.944228549352));
#193921=CARTESIAN_POINT('',(126.117589547031,-1.85,51.334121607331));
#193922=CARTESIAN_POINT('',(126.1748325209,-1.85,51.0396335058013));
#193923=CARTESIAN_POINT('Origin',(125.684019018351,-1.85,50.944228549352));
#193924=CARTESIAN_POINT('',(125.626776044481,-1.85,51.2387166508817));
#193925=CARTESIAN_POINT('',(125.684019018351,-1.85,50.944228549352));
#193926=CARTESIAN_POINT('Origin',(125.684019018351,-0.549999999999986,50.944228549352));
#193927=CARTESIAN_POINT('',(126.1748325209,-0.549999999999986,51.0396335058013));
#193928=CARTESIAN_POINT('',(126.117589547031,-0.549999999999986,51.334121607331));
#193929=CARTESIAN_POINT('',(126.1748325209,-0.549999999999986,51.0396335058013));
#193930=CARTESIAN_POINT('',(125.626776044481,-0.549999999999986,51.2387166508817));
#193931=CARTESIAN_POINT('',(125.626776044481,-0.549999999999986,51.2387166508817));
#193932=CARTESIAN_POINT('',(125.684019018351,-0.549999999999986,50.944228549352));
#193933=CARTESIAN_POINT('',(125.684019018351,-0.549999999999986,50.944228549352));
#193934=CARTESIAN_POINT('',(125.684019018351,-0.549999999999986,50.944228549352));
#193935=CARTESIAN_POINT('Origin',(126.1748325209,-0.549999999999986,51.0396335058013));
#193936=CARTESIAN_POINT('',(126.1748325209,-1.05,51.0396335058013));
#193937=CARTESIAN_POINT('',(126.117589547031,-1.05,51.334121607331));
#193938=CARTESIAN_POINT('',(126.1748325209,-1.05,51.0396335058013));
#193939=CARTESIAN_POINT('',(126.117589547031,-0.549999999999986,51.334121607331));
#193940=CARTESIAN_POINT('',(126.1748325209,-0.549999999999986,51.0396335058013));
#193941=CARTESIAN_POINT('Origin',(126.1748325209,-1.05,51.0396335058013));
#193942=CARTESIAN_POINT('',(125.684019018351,-1.05,50.944228549352));
#193943=CARTESIAN_POINT('',(125.626776044481,-1.05,51.2387166508817));
#193944=CARTESIAN_POINT('',(125.684019018351,-1.05,50.944228549352));
#193945=CARTESIAN_POINT('',(126.117589547031,-1.05,51.334121607331));
#193946=CARTESIAN_POINT('',(126.1748325209,-1.05,51.0396335058013));
#193947=CARTESIAN_POINT('Origin',(125.684019018351,-1.05,50.944228549352));
#193948=CARTESIAN_POINT('',(125.626776044481,-1.05,51.2387166508817));
#193949=CARTESIAN_POINT('',(125.684019018351,-1.05,50.944228549352));
#193950=CARTESIAN_POINT('Origin',(125.684019018351,0.250000000000015,50.944228549352));
#193951=CARTESIAN_POINT('',(126.1748325209,0.250000000000015,51.0396335058013));
#193952=CARTESIAN_POINT('',(126.117589547031,0.250000000000015,51.334121607331));
#193953=CARTESIAN_POINT('',(126.1748325209,0.250000000000015,51.0396335058013));
#193954=CARTESIAN_POINT('',(125.626776044481,0.250000000000015,51.2387166508817));
#193955=CARTESIAN_POINT('',(125.626776044481,0.250000000000015,51.2387166508817));
#193956=CARTESIAN_POINT('',(125.684019018351,0.250000000000015,50.944228549352));
#193957=CARTESIAN_POINT('',(125.684019018351,0.250000000000015,50.944228549352));
#193958=CARTESIAN_POINT('',(125.684019018351,0.250000000000015,50.944228549352));
#193959=CARTESIAN_POINT('Origin',(126.1748325209,0.250000000000015,51.0396335058013));
#193960=CARTESIAN_POINT('',(126.1748325209,-0.249999999999985,51.0396335058013));
#193961=CARTESIAN_POINT('',(126.117589547031,-0.249999999999985,51.334121607331));
#193962=CARTESIAN_POINT('',(126.1748325209,-0.249999999999985,51.0396335058013));
#193963=CARTESIAN_POINT('',(126.117589547031,0.250000000000015,51.334121607331));
#193964=CARTESIAN_POINT('',(126.1748325209,0.250000000000015,51.0396335058013));
#193965=CARTESIAN_POINT('Origin',(126.1748325209,-0.249999999999985,51.0396335058013));
#193966=CARTESIAN_POINT('',(125.684019018351,-0.249999999999985,50.944228549352));
#193967=CARTESIAN_POINT('',(125.626776044481,-0.249999999999985,51.2387166508817));
#193968=CARTESIAN_POINT('',(125.684019018351,-0.249999999999985,50.944228549352));
#193969=CARTESIAN_POINT('',(126.117589547031,-0.249999999999985,51.334121607331));
#193970=CARTESIAN_POINT('',(126.1748325209,-0.249999999999985,51.0396335058013));
#193971=CARTESIAN_POINT('Origin',(125.684019018351,-0.249999999999985,50.944228549352));
#193972=CARTESIAN_POINT('',(125.626776044481,-0.249999999999985,51.2387166508817));
#193973=CARTESIAN_POINT('',(125.684019018351,-0.249999999999985,50.944228549352));
#193974=CARTESIAN_POINT('Origin',(125.684019018351,1.05,50.944228549352));
#193975=CARTESIAN_POINT('',(126.1748325209,1.05,51.0396335058013));
#193976=CARTESIAN_POINT('',(126.117589547031,1.05,51.334121607331));
#193977=CARTESIAN_POINT('',(126.1748325209,1.05,51.0396335058013));
#193978=CARTESIAN_POINT('',(125.626776044481,1.05,51.2387166508817));
#193979=CARTESIAN_POINT('',(125.626776044481,1.05,51.2387166508817));
#193980=CARTESIAN_POINT('',(125.684019018351,1.05,50.944228549352));
#193981=CARTESIAN_POINT('',(125.684019018351,1.05,50.944228549352));
#193982=CARTESIAN_POINT('',(125.684019018351,1.05,50.944228549352));
#193983=CARTESIAN_POINT('Origin',(126.1748325209,1.05,51.0396335058013));
#193984=CARTESIAN_POINT('',(126.1748325209,0.550000000000015,51.0396335058013));
#193985=CARTESIAN_POINT('',(126.117589547031,0.550000000000015,51.334121607331));
#193986=CARTESIAN_POINT('',(126.1748325209,0.550000000000015,51.0396335058013));
#193987=CARTESIAN_POINT('',(126.117589547031,1.05,51.334121607331));
#193988=CARTESIAN_POINT('',(126.1748325209,1.05,51.0396335058013));
#193989=CARTESIAN_POINT('Origin',(126.1748325209,0.550000000000015,51.0396335058013));
#193990=CARTESIAN_POINT('',(125.684019018351,0.550000000000015,50.944228549352));
#193991=CARTESIAN_POINT('',(125.626776044481,0.550000000000015,51.2387166508817));
#193992=CARTESIAN_POINT('',(125.684019018351,0.550000000000015,50.944228549352));
#193993=CARTESIAN_POINT('',(126.117589547031,0.550000000000015,51.334121607331));
#193994=CARTESIAN_POINT('',(126.1748325209,0.550000000000015,51.0396335058013));
#193995=CARTESIAN_POINT('Origin',(125.684019018351,0.550000000000015,50.944228549352));
#193996=CARTESIAN_POINT('',(125.626776044481,0.550000000000015,51.2387166508817));
#193997=CARTESIAN_POINT('',(125.684019018351,0.550000000000015,50.944228549352));
#193998=CARTESIAN_POINT('Origin',(125.684019018351,1.85,50.944228549352));
#193999=CARTESIAN_POINT('',(126.1748325209,1.85,51.0396335058013));
#194000=CARTESIAN_POINT('',(126.117589547031,1.85,51.334121607331));
#194001=CARTESIAN_POINT('',(126.1748325209,1.85,51.0396335058013));
#194002=CARTESIAN_POINT('',(125.626776044481,1.85,51.2387166508817));
#194003=CARTESIAN_POINT('',(125.626776044481,1.85,51.2387166508817));
#194004=CARTESIAN_POINT('',(125.684019018351,1.85,50.944228549352));
#194005=CARTESIAN_POINT('',(125.684019018351,1.85,50.944228549352));
#194006=CARTESIAN_POINT('',(125.684019018351,1.85,50.944228549352));
#194007=CARTESIAN_POINT('Origin',(126.1748325209,1.85,51.0396335058013));
#194008=CARTESIAN_POINT('',(126.1748325209,1.35,51.0396335058013));
#194009=CARTESIAN_POINT('',(126.117589547031,1.35,51.334121607331));
#194010=CARTESIAN_POINT('',(126.1748325209,1.35,51.0396335058013));
#194011=CARTESIAN_POINT('',(126.117589547031,1.85,51.334121607331));
#194012=CARTESIAN_POINT('',(126.1748325209,1.85,51.0396335058013));
#194013=CARTESIAN_POINT('Origin',(126.1748325209,1.35,51.0396335058013));
#194014=CARTESIAN_POINT('',(125.684019018351,1.35,50.944228549352));
#194015=CARTESIAN_POINT('',(125.626776044481,1.35,51.2387166508817));
#194016=CARTESIAN_POINT('',(125.684019018351,1.35,50.944228549352));
#194017=CARTESIAN_POINT('',(126.117589547031,1.35,51.334121607331));
#194018=CARTESIAN_POINT('',(126.1748325209,1.35,51.0396335058013));
#194019=CARTESIAN_POINT('Origin',(125.684019018351,1.35,50.944228549352));
#194020=CARTESIAN_POINT('',(125.626776044481,1.35,51.2387166508817));
#194021=CARTESIAN_POINT('',(125.684019018351,1.35,50.944228549352));
#194022=CARTESIAN_POINT('Origin',(125.684019018351,2.65,50.944228549352));
#194023=CARTESIAN_POINT('',(126.1748325209,2.65,51.0396335058013));
#194024=CARTESIAN_POINT('',(126.117589547031,2.65,51.334121607331));
#194025=CARTESIAN_POINT('',(126.1748325209,2.65,51.0396335058013));
#194026=CARTESIAN_POINT('',(125.626776044481,2.65,51.2387166508817));
#194027=CARTESIAN_POINT('',(125.626776044481,2.65,51.2387166508817));
#194028=CARTESIAN_POINT('',(125.684019018351,2.65,50.944228549352));
#194029=CARTESIAN_POINT('',(125.684019018351,2.65,50.944228549352));
#194030=CARTESIAN_POINT('',(125.684019018351,2.65,50.944228549352));
#194031=CARTESIAN_POINT('Origin',(126.1748325209,2.65,51.0396335058013));
#194032=CARTESIAN_POINT('',(126.1748325209,2.15,51.0396335058013));
#194033=CARTESIAN_POINT('',(126.117589547031,2.15,51.334121607331));
#194034=CARTESIAN_POINT('',(126.1748325209,2.15,51.0396335058013));
#194035=CARTESIAN_POINT('',(126.117589547031,2.65,51.334121607331));
#194036=CARTESIAN_POINT('',(126.1748325209,2.65,51.0396335058013));
#194037=CARTESIAN_POINT('Origin',(126.1748325209,2.15,51.0396335058013));
#194038=CARTESIAN_POINT('',(125.684019018351,2.15,50.944228549352));
#194039=CARTESIAN_POINT('',(125.626776044481,2.15,51.2387166508817));
#194040=CARTESIAN_POINT('',(125.684019018351,2.15,50.944228549352));
#194041=CARTESIAN_POINT('',(126.117589547031,2.15,51.334121607331));
#194042=CARTESIAN_POINT('',(126.1748325209,2.15,51.0396335058013));
#194043=CARTESIAN_POINT('Origin',(125.684019018351,2.15,50.944228549352));
#194044=CARTESIAN_POINT('',(125.626776044481,2.15,51.2387166508817));
#194045=CARTESIAN_POINT('',(125.684019018351,2.15,50.944228549352));
#194046=CARTESIAN_POINT('Origin',(125.684019018351,3.45,50.944228549352));
#194047=CARTESIAN_POINT('',(126.1748325209,3.45,51.0396335058013));
#194048=CARTESIAN_POINT('',(126.117589547031,3.45,51.334121607331));
#194049=CARTESIAN_POINT('',(126.1748325209,3.45,51.0396335058013));
#194050=CARTESIAN_POINT('',(125.626776044481,3.45,51.2387166508817));
#194051=CARTESIAN_POINT('',(125.626776044481,3.45,51.2387166508817));
#194052=CARTESIAN_POINT('',(125.684019018351,3.45,50.944228549352));
#194053=CARTESIAN_POINT('',(125.684019018351,3.45,50.944228549352));
#194054=CARTESIAN_POINT('',(125.684019018351,3.45,50.944228549352));
#194055=CARTESIAN_POINT('Origin',(126.1748325209,3.45,51.0396335058013));
#194056=CARTESIAN_POINT('',(126.1748325209,2.95,51.0396335058013));
#194057=CARTESIAN_POINT('',(126.117589547031,2.95,51.334121607331));
#194058=CARTESIAN_POINT('',(126.1748325209,2.95,51.0396335058013));
#194059=CARTESIAN_POINT('',(126.117589547031,3.45,51.334121607331));
#194060=CARTESIAN_POINT('',(126.1748325209,3.45,51.0396335058013));
#194061=CARTESIAN_POINT('Origin',(126.1748325209,2.95,51.0396335058013));
#194062=CARTESIAN_POINT('',(125.684019018351,2.95,50.944228549352));
#194063=CARTESIAN_POINT('',(125.626776044481,2.95,51.2387166508817));
#194064=CARTESIAN_POINT('',(125.684019018351,2.95,50.944228549352));
#194065=CARTESIAN_POINT('',(126.117589547031,2.95,51.334121607331));
#194066=CARTESIAN_POINT('',(126.1748325209,2.95,51.0396335058013));
#194067=CARTESIAN_POINT('Origin',(125.684019018351,2.95,50.944228549352));
#194068=CARTESIAN_POINT('',(125.626776044481,2.95,51.2387166508817));
#194069=CARTESIAN_POINT('',(125.684019018351,2.95,50.944228549352));
#194070=CARTESIAN_POINT('Origin',(120.186907789796,9.05,49.8756930371204));
#194071=CARTESIAN_POINT('',(120.677721292346,9.05,49.9710979935697));
#194072=CARTESIAN_POINT('',(120.620478318476,9.05,50.2655860950994));
#194073=CARTESIAN_POINT('',(120.677721292346,9.05,49.9710979935697));
#194074=CARTESIAN_POINT('',(120.129664815927,9.05,50.1701811386501));
#194075=CARTESIAN_POINT('',(120.129664815927,9.05,50.1701811386501));
#194076=CARTESIAN_POINT('',(120.186907789796,9.05,49.8756930371204));
#194077=CARTESIAN_POINT('',(120.186907789796,9.05,49.8756930371204));
#194078=CARTESIAN_POINT('',(120.186907789796,9.05,49.8756930371204));
#194079=CARTESIAN_POINT('Origin',(120.677721292346,9.05,49.9710979935697));
#194080=CARTESIAN_POINT('',(120.677721292346,8.55,49.9710979935697));
#194081=CARTESIAN_POINT('',(120.620478318476,8.55,50.2655860950994));
#194082=CARTESIAN_POINT('',(120.677721292346,8.55,49.9710979935697));
#194083=CARTESIAN_POINT('',(120.620478318476,9.05,50.2655860950994));
#194084=CARTESIAN_POINT('',(120.677721292346,9.05,49.9710979935697));
#194085=CARTESIAN_POINT('Origin',(120.677721292346,8.55,49.9710979935697));
#194086=CARTESIAN_POINT('',(120.186907789796,8.55,49.8756930371204));
#194087=CARTESIAN_POINT('',(120.129664815927,8.55,50.1701811386501));
#194088=CARTESIAN_POINT('',(120.186907789796,8.55,49.8756930371204));
#194089=CARTESIAN_POINT('',(120.620478318476,8.55,50.2655860950994));
#194090=CARTESIAN_POINT('',(120.677721292346,8.55,49.9710979935697));
#194091=CARTESIAN_POINT('Origin',(120.186907789796,8.55,49.8756930371204));
#194092=CARTESIAN_POINT('',(120.129664815927,8.55,50.1701811386501));
#194093=CARTESIAN_POINT('',(120.186907789796,8.55,49.8756930371204));
#194094=CARTESIAN_POINT('Origin',(119.401606185717,9.05,49.7230451068016));
#194095=CARTESIAN_POINT('',(119.892419688267,9.05,49.8184500632509));
#194096=CARTESIAN_POINT('',(119.835176714397,9.05,50.1129381647806));
#194097=CARTESIAN_POINT('',(119.892419688267,9.05,49.8184500632509));
#194098=CARTESIAN_POINT('',(119.344363211847,9.05,50.0175332083313));
#194099=CARTESIAN_POINT('',(119.344363211847,9.05,50.0175332083313));
#194100=CARTESIAN_POINT('',(119.401606185717,9.05,49.7230451068016));
#194101=CARTESIAN_POINT('',(119.401606185717,9.05,49.7230451068016));
#194102=CARTESIAN_POINT('',(119.401606185717,9.05,49.7230451068016));
#194103=CARTESIAN_POINT('Origin',(119.892419688267,9.05,49.8184500632509));
#194104=CARTESIAN_POINT('',(119.892419688267,8.55,49.8184500632509));
#194105=CARTESIAN_POINT('',(119.835176714397,8.55,50.1129381647806));
#194106=CARTESIAN_POINT('',(119.892419688267,8.55,49.8184500632509));
#194107=CARTESIAN_POINT('',(119.835176714397,9.05,50.1129381647806));
#194108=CARTESIAN_POINT('',(119.892419688267,9.05,49.8184500632509));
#194109=CARTESIAN_POINT('Origin',(119.892419688267,8.55,49.8184500632509));
#194110=CARTESIAN_POINT('',(119.401606185717,8.55,49.7230451068016));
#194111=CARTESIAN_POINT('',(119.344363211847,8.55,50.0175332083313));
#194112=CARTESIAN_POINT('',(119.401606185717,8.55,49.7230451068016));
#194113=CARTESIAN_POINT('',(119.835176714397,8.55,50.1129381647806));
#194114=CARTESIAN_POINT('',(119.892419688267,8.55,49.8184500632509));
#194115=CARTESIAN_POINT('Origin',(119.401606185717,8.55,49.7230451068016));
#194116=CARTESIAN_POINT('',(119.344363211847,8.55,50.0175332083313));
#194117=CARTESIAN_POINT('',(119.401606185717,8.55,49.7230451068016));
#194118=CARTESIAN_POINT('Origin',(118.616304581638,9.05,49.5703971764828));
#194119=CARTESIAN_POINT('',(119.107118084187,9.05,49.6658021329321));
#194120=CARTESIAN_POINT('',(119.049875110318,9.05,49.9602902344618));
#194121=CARTESIAN_POINT('',(119.107118084187,9.05,49.6658021329321));
#194122=CARTESIAN_POINT('',(118.559061607768,9.05,49.8648852780125));
#194123=CARTESIAN_POINT('',(118.559061607768,9.05,49.8648852780125));
#194124=CARTESIAN_POINT('',(118.616304581638,9.05,49.5703971764828));
#194125=CARTESIAN_POINT('',(118.616304581638,9.05,49.5703971764828));
#194126=CARTESIAN_POINT('',(118.616304581638,9.05,49.5703971764828));
#194127=CARTESIAN_POINT('Origin',(119.107118084187,9.05,49.6658021329321));
#194128=CARTESIAN_POINT('',(119.107118084187,8.55,49.6658021329321));
#194129=CARTESIAN_POINT('',(119.049875110318,8.55,49.9602902344618));
#194130=CARTESIAN_POINT('',(119.107118084187,8.55,49.6658021329321));
#194131=CARTESIAN_POINT('',(119.049875110318,9.05,49.9602902344618));
#194132=CARTESIAN_POINT('',(119.107118084187,9.05,49.6658021329321));
#194133=CARTESIAN_POINT('Origin',(119.107118084187,8.55,49.6658021329321));
#194134=CARTESIAN_POINT('',(118.616304581638,8.55,49.5703971764828));
#194135=CARTESIAN_POINT('',(118.559061607768,8.55,49.8648852780125));
#194136=CARTESIAN_POINT('',(118.616304581638,8.55,49.5703971764828));
#194137=CARTESIAN_POINT('',(119.049875110318,8.55,49.9602902344618));
#194138=CARTESIAN_POINT('',(119.107118084187,8.55,49.6658021329321));
#194139=CARTESIAN_POINT('Origin',(118.616304581638,8.55,49.5703971764828));
#194140=CARTESIAN_POINT('',(118.559061607768,8.55,49.8648852780125));
#194141=CARTESIAN_POINT('',(118.616304581638,8.55,49.5703971764828));
#194142=CARTESIAN_POINT('Origin',(117.831002977559,9.05,49.417749246164));
#194143=CARTESIAN_POINT('',(118.321816480108,9.05,49.5131542026133));
#194144=CARTESIAN_POINT('',(118.264573506239,9.05,49.807642304143));
#194145=CARTESIAN_POINT('',(118.321816480108,9.05,49.5131542026133));
#194146=CARTESIAN_POINT('',(117.773760003689,9.05,49.7122373476937));
#194147=CARTESIAN_POINT('',(117.773760003689,9.05,49.7122373476937));
#194148=CARTESIAN_POINT('',(117.831002977559,9.05,49.417749246164));
#194149=CARTESIAN_POINT('',(117.831002977559,9.05,49.417749246164));
#194150=CARTESIAN_POINT('',(117.831002977559,9.05,49.417749246164));
#194151=CARTESIAN_POINT('Origin',(118.321816480108,9.05,49.5131542026133));
#194152=CARTESIAN_POINT('',(118.321816480108,8.55,49.5131542026133));
#194153=CARTESIAN_POINT('',(118.264573506239,8.55,49.807642304143));
#194154=CARTESIAN_POINT('',(118.321816480108,8.55,49.5131542026133));
#194155=CARTESIAN_POINT('',(118.264573506239,9.05,49.807642304143));
#194156=CARTESIAN_POINT('',(118.321816480108,9.05,49.5131542026133));
#194157=CARTESIAN_POINT('Origin',(118.321816480108,8.55,49.5131542026133));
#194158=CARTESIAN_POINT('',(117.831002977559,8.55,49.417749246164));
#194159=CARTESIAN_POINT('',(117.773760003689,8.55,49.7122373476937));
#194160=CARTESIAN_POINT('',(117.831002977559,8.55,49.417749246164));
#194161=CARTESIAN_POINT('',(118.264573506239,8.55,49.807642304143));
#194162=CARTESIAN_POINT('',(118.321816480108,8.55,49.5131542026133));
#194163=CARTESIAN_POINT('Origin',(117.831002977559,8.55,49.417749246164));
#194164=CARTESIAN_POINT('',(117.773760003689,8.55,49.7122373476937));
#194165=CARTESIAN_POINT('',(117.831002977559,8.55,49.417749246164));
#194166=CARTESIAN_POINT('Origin',(117.045701373479,9.05,49.2651013158452));
#194167=CARTESIAN_POINT('',(117.536514876029,9.05,49.3605062722945));
#194168=CARTESIAN_POINT('',(117.479271902159,9.05,49.6549943738242));
#194169=CARTESIAN_POINT('',(117.536514876029,9.05,49.3605062722945));
#194170=CARTESIAN_POINT('',(116.98845839961,9.05,49.5595894173749));
#194171=CARTESIAN_POINT('',(116.98845839961,9.05,49.5595894173749));
#194172=CARTESIAN_POINT('',(117.045701373479,9.05,49.2651013158452));
#194173=CARTESIAN_POINT('',(117.045701373479,9.05,49.2651013158452));
#194174=CARTESIAN_POINT('',(117.045701373479,9.05,49.2651013158452));
#194175=CARTESIAN_POINT('Origin',(117.536514876029,9.05,49.3605062722945));
#194176=CARTESIAN_POINT('',(117.536514876029,8.55,49.3605062722945));
#194177=CARTESIAN_POINT('',(117.479271902159,8.55,49.6549943738242));
#194178=CARTESIAN_POINT('',(117.536514876029,8.55,49.3605062722945));
#194179=CARTESIAN_POINT('',(117.479271902159,9.05,49.6549943738242));
#194180=CARTESIAN_POINT('',(117.536514876029,9.05,49.3605062722945));
#194181=CARTESIAN_POINT('Origin',(117.536514876029,8.55,49.3605062722945));
#194182=CARTESIAN_POINT('',(117.045701373479,8.55,49.2651013158452));
#194183=CARTESIAN_POINT('',(116.98845839961,8.55,49.5595894173749));
#194184=CARTESIAN_POINT('',(117.045701373479,8.55,49.2651013158452));
#194185=CARTESIAN_POINT('',(117.479271902159,8.55,49.6549943738242));
#194186=CARTESIAN_POINT('',(117.536514876029,8.55,49.3605062722945));
#194187=CARTESIAN_POINT('Origin',(117.045701373479,8.55,49.2651013158452));
#194188=CARTESIAN_POINT('',(116.98845839961,8.55,49.5595894173749));
#194189=CARTESIAN_POINT('',(117.045701373479,8.55,49.2651013158452));
#194190=CARTESIAN_POINT('Origin',(116.2603997694,9.05,49.1124533855264));
#194191=CARTESIAN_POINT('',(116.75121327195,9.05,49.2078583419757));
#194192=CARTESIAN_POINT('',(116.69397029808,9.05,49.5023464435054));
#194193=CARTESIAN_POINT('',(116.75121327195,9.05,49.2078583419757));
#194194=CARTESIAN_POINT('',(116.203156795531,9.05,49.4069414870561));
#194195=CARTESIAN_POINT('',(116.203156795531,9.05,49.4069414870561));
#194196=CARTESIAN_POINT('',(116.2603997694,9.05,49.1124533855264));
#194197=CARTESIAN_POINT('',(116.2603997694,9.05,49.1124533855264));
#194198=CARTESIAN_POINT('',(116.2603997694,9.05,49.1124533855264));
#194199=CARTESIAN_POINT('Origin',(116.75121327195,9.05,49.2078583419757));
#194200=CARTESIAN_POINT('',(116.75121327195,8.55,49.2078583419757));
#194201=CARTESIAN_POINT('',(116.69397029808,8.55,49.5023464435054));
#194202=CARTESIAN_POINT('',(116.75121327195,8.55,49.2078583419757));
#194203=CARTESIAN_POINT('',(116.69397029808,9.05,49.5023464435054));
#194204=CARTESIAN_POINT('',(116.75121327195,9.05,49.2078583419757));
#194205=CARTESIAN_POINT('Origin',(116.75121327195,8.55,49.2078583419757));
#194206=CARTESIAN_POINT('',(116.2603997694,8.55,49.1124533855264));
#194207=CARTESIAN_POINT('',(116.203156795531,8.55,49.4069414870561));
#194208=CARTESIAN_POINT('',(116.2603997694,8.55,49.1124533855264));
#194209=CARTESIAN_POINT('',(116.69397029808,8.55,49.5023464435054));
#194210=CARTESIAN_POINT('',(116.75121327195,8.55,49.2078583419757));
#194211=CARTESIAN_POINT('Origin',(116.2603997694,8.55,49.1124533855264));
#194212=CARTESIAN_POINT('',(116.203156795531,8.55,49.4069414870561));
#194213=CARTESIAN_POINT('',(116.2603997694,8.55,49.1124533855264));
#194214=CARTESIAN_POINT('Origin',(115.475098165321,9.05,48.9598054552076));
#194215=CARTESIAN_POINT('',(115.96591166787,9.05,49.0552104116569));
#194216=CARTESIAN_POINT('',(115.908668694001,9.05,49.3496985131866));
#194217=CARTESIAN_POINT('',(115.96591166787,9.05,49.0552104116569));
#194218=CARTESIAN_POINT('',(115.417855191451,9.05,49.2542935567373));
#194219=CARTESIAN_POINT('',(115.417855191451,9.05,49.2542935567373));
#194220=CARTESIAN_POINT('',(115.475098165321,9.05,48.9598054552076));
#194221=CARTESIAN_POINT('',(115.475098165321,9.05,48.9598054552076));
#194222=CARTESIAN_POINT('',(115.475098165321,9.05,48.9598054552076));
#194223=CARTESIAN_POINT('Origin',(115.96591166787,9.05,49.0552104116569));
#194224=CARTESIAN_POINT('',(115.96591166787,8.55,49.0552104116569));
#194225=CARTESIAN_POINT('',(115.908668694001,8.55,49.3496985131866));
#194226=CARTESIAN_POINT('',(115.96591166787,8.55,49.0552104116569));
#194227=CARTESIAN_POINT('',(115.908668694001,9.05,49.3496985131866));
#194228=CARTESIAN_POINT('',(115.96591166787,9.05,49.0552104116569));
#194229=CARTESIAN_POINT('Origin',(115.96591166787,8.55,49.0552104116569));
#194230=CARTESIAN_POINT('',(115.475098165321,8.55,48.9598054552076));
#194231=CARTESIAN_POINT('',(115.417855191451,8.55,49.2542935567373));
#194232=CARTESIAN_POINT('',(115.475098165321,8.55,48.9598054552076));
#194233=CARTESIAN_POINT('',(115.908668694001,8.55,49.3496985131866));
#194234=CARTESIAN_POINT('',(115.96591166787,8.55,49.0552104116569));
#194235=CARTESIAN_POINT('Origin',(115.475098165321,8.55,48.9598054552076));
#194236=CARTESIAN_POINT('',(115.417855191451,8.55,49.2542935567373));
#194237=CARTESIAN_POINT('',(115.475098165321,8.55,48.9598054552076));
#194238=CARTESIAN_POINT('Origin',(114.689796561242,9.05,48.8071575248888));
#194239=CARTESIAN_POINT('',(115.180610063791,9.05,48.9025624813381));
#194240=CARTESIAN_POINT('',(115.123367089922,9.05,49.1970505828678));
#194241=CARTESIAN_POINT('',(115.180610063791,9.05,48.9025624813381));
#194242=CARTESIAN_POINT('',(114.632553587372,9.05,49.1016456264185));
#194243=CARTESIAN_POINT('',(114.632553587372,9.05,49.1016456264185));
#194244=CARTESIAN_POINT('',(114.689796561242,9.05,48.8071575248888));
#194245=CARTESIAN_POINT('',(114.689796561242,9.05,48.8071575248888));
#194246=CARTESIAN_POINT('',(114.689796561242,9.05,48.8071575248888));
#194247=CARTESIAN_POINT('Origin',(115.180610063791,9.05,48.9025624813381));
#194248=CARTESIAN_POINT('',(115.180610063791,8.55,48.9025624813381));
#194249=CARTESIAN_POINT('',(115.123367089922,8.55,49.1970505828678));
#194250=CARTESIAN_POINT('',(115.180610063791,8.55,48.9025624813381));
#194251=CARTESIAN_POINT('',(115.123367089922,9.05,49.1970505828678));
#194252=CARTESIAN_POINT('',(115.180610063791,9.05,48.9025624813381));
#194253=CARTESIAN_POINT('Origin',(115.180610063791,8.55,48.9025624813381));
#194254=CARTESIAN_POINT('',(114.689796561242,8.55,48.8071575248888));
#194255=CARTESIAN_POINT('',(114.632553587372,8.55,49.1016456264185));
#194256=CARTESIAN_POINT('',(114.689796561242,8.55,48.8071575248888));
#194257=CARTESIAN_POINT('',(115.123367089922,8.55,49.1970505828678));
#194258=CARTESIAN_POINT('',(115.180610063791,8.55,48.9025624813381));
#194259=CARTESIAN_POINT('Origin',(114.689796561242,8.55,48.8071575248888));
#194260=CARTESIAN_POINT('',(114.632553587372,8.55,49.1016456264185));
#194261=CARTESIAN_POINT('',(114.689796561242,8.55,48.8071575248888));
#194262=CARTESIAN_POINT('Origin',(113.904494957163,9.05,48.65450959457));
#194263=CARTESIAN_POINT('',(114.395308459712,9.05,48.7499145510193));
#194264=CARTESIAN_POINT('',(114.338065485842,9.05,49.044402652549));
#194265=CARTESIAN_POINT('',(114.395308459712,9.05,48.7499145510193));
#194266=CARTESIAN_POINT('',(113.847251983293,9.05,48.9489976960997));
#194267=CARTESIAN_POINT('',(113.847251983293,9.05,48.9489976960997));
#194268=CARTESIAN_POINT('',(113.904494957163,9.05,48.65450959457));
#194269=CARTESIAN_POINT('',(113.904494957163,9.05,48.65450959457));
#194270=CARTESIAN_POINT('',(113.904494957163,9.05,48.65450959457));
#194271=CARTESIAN_POINT('Origin',(114.395308459712,9.05,48.7499145510193));
#194272=CARTESIAN_POINT('',(114.395308459712,8.55,48.7499145510193));
#194273=CARTESIAN_POINT('',(114.338065485842,8.55,49.044402652549));
#194274=CARTESIAN_POINT('',(114.395308459712,8.55,48.7499145510193));
#194275=CARTESIAN_POINT('',(114.338065485842,9.05,49.044402652549));
#194276=CARTESIAN_POINT('',(114.395308459712,9.05,48.7499145510193));
#194277=CARTESIAN_POINT('Origin',(114.395308459712,8.55,48.7499145510193));
#194278=CARTESIAN_POINT('',(113.904494957163,8.55,48.65450959457));
#194279=CARTESIAN_POINT('',(113.847251983293,8.55,48.9489976960997));
#194280=CARTESIAN_POINT('',(113.904494957163,8.55,48.65450959457));
#194281=CARTESIAN_POINT('',(114.338065485842,8.55,49.044402652549));
#194282=CARTESIAN_POINT('',(114.395308459712,8.55,48.7499145510193));
#194283=CARTESIAN_POINT('Origin',(113.904494957163,8.55,48.65450959457));
#194284=CARTESIAN_POINT('',(113.847251983293,8.55,48.9489976960997));
#194285=CARTESIAN_POINT('',(113.904494957163,8.55,48.65450959457));
#194286=CARTESIAN_POINT('Origin',(109.192685332687,5.05,47.7386220126572));
#194287=CARTESIAN_POINT('',(109.683498835237,5.05,47.8340269691064));
#194288=CARTESIAN_POINT('',(109.626255861367,5.05,48.1285150706361));
#194289=CARTESIAN_POINT('',(109.683498835237,5.05,47.8340269691064));
#194290=CARTESIAN_POINT('',(109.135442358818,5.05,48.0331101141869));
#194291=CARTESIAN_POINT('',(109.135442358818,5.05,48.0331101141869));
#194292=CARTESIAN_POINT('',(109.192685332687,5.05,47.7386220126572));
#194293=CARTESIAN_POINT('',(109.192685332687,5.05,47.7386220126572));
#194294=CARTESIAN_POINT('',(109.192685332687,5.05,47.7386220126572));
#194295=CARTESIAN_POINT('Origin',(109.683498835237,5.05,47.8340269691064));
#194296=CARTESIAN_POINT('',(109.683498835237,4.55,47.8340269691064));
#194297=CARTESIAN_POINT('',(109.626255861367,4.55,48.1285150706361));
#194298=CARTESIAN_POINT('',(109.683498835237,4.55,47.8340269691064));
#194299=CARTESIAN_POINT('',(109.626255861367,5.05,48.1285150706361));
#194300=CARTESIAN_POINT('',(109.683498835237,5.05,47.8340269691064));
#194301=CARTESIAN_POINT('Origin',(109.683498835237,4.55,47.8340269691064));
#194302=CARTESIAN_POINT('',(109.192685332687,4.55,47.7386220126572));
#194303=CARTESIAN_POINT('',(109.135442358818,4.55,48.0331101141869));
#194304=CARTESIAN_POINT('',(109.192685332687,4.55,47.7386220126572));
#194305=CARTESIAN_POINT('',(109.626255861367,4.55,48.1285150706361));
#194306=CARTESIAN_POINT('',(109.683498835237,4.55,47.8340269691064));
#194307=CARTESIAN_POINT('Origin',(109.192685332687,4.55,47.7386220126572));
#194308=CARTESIAN_POINT('',(109.135442358818,4.55,48.0331101141869));
#194309=CARTESIAN_POINT('',(109.192685332687,4.55,47.7386220126572));
#194310=CARTESIAN_POINT('Origin',(109.192685332687,4.25,47.7386220126572));
#194311=CARTESIAN_POINT('',(109.683498835237,4.25,47.8340269691064));
#194312=CARTESIAN_POINT('',(109.626255861367,4.25,48.1285150706361));
#194313=CARTESIAN_POINT('',(109.683498835237,4.25,47.8340269691064));
#194314=CARTESIAN_POINT('',(109.135442358818,4.25,48.0331101141869));
#194315=CARTESIAN_POINT('',(109.135442358818,4.25,48.0331101141869));
#194316=CARTESIAN_POINT('',(109.192685332687,4.25,47.7386220126572));
#194317=CARTESIAN_POINT('',(109.192685332687,4.25,47.7386220126572));
#194318=CARTESIAN_POINT('',(109.192685332687,4.25,47.7386220126572));
#194319=CARTESIAN_POINT('Origin',(109.683498835237,4.25,47.8340269691064));
#194320=CARTESIAN_POINT('',(109.683498835237,3.75,47.8340269691064));
#194321=CARTESIAN_POINT('',(109.626255861367,3.75,48.1285150706361));
#194322=CARTESIAN_POINT('',(109.683498835237,3.75,47.8340269691064));
#194323=CARTESIAN_POINT('',(109.626255861367,4.25,48.1285150706361));
#194324=CARTESIAN_POINT('',(109.683498835237,4.25,47.8340269691064));
#194325=CARTESIAN_POINT('Origin',(109.683498835237,3.75,47.8340269691064));
#194326=CARTESIAN_POINT('',(109.192685332687,3.75,47.7386220126572));
#194327=CARTESIAN_POINT('',(109.135442358818,3.75,48.0331101141869));
#194328=CARTESIAN_POINT('',(109.192685332687,3.75,47.7386220126572));
#194329=CARTESIAN_POINT('',(109.626255861367,3.75,48.1285150706361));
#194330=CARTESIAN_POINT('',(109.683498835237,3.75,47.8340269691064));
#194331=CARTESIAN_POINT('Origin',(109.192685332687,3.75,47.7386220126572));
#194332=CARTESIAN_POINT('',(109.135442358818,3.75,48.0331101141869));
#194333=CARTESIAN_POINT('',(109.192685332687,3.75,47.7386220126572));
#194334=CARTESIAN_POINT('Origin',(109.192685332687,3.45,47.7386220126572));
#194335=CARTESIAN_POINT('',(109.683498835237,3.45,47.8340269691064));
#194336=CARTESIAN_POINT('',(109.626255861367,3.45,48.1285150706361));
#194337=CARTESIAN_POINT('',(109.683498835237,3.45,47.8340269691064));
#194338=CARTESIAN_POINT('',(109.135442358818,3.45,48.0331101141869));
#194339=CARTESIAN_POINT('',(109.135442358818,3.45,48.0331101141869));
#194340=CARTESIAN_POINT('',(109.192685332687,3.45,47.7386220126572));
#194341=CARTESIAN_POINT('',(109.192685332687,3.45,47.7386220126572));
#194342=CARTESIAN_POINT('',(109.192685332687,3.45,47.7386220126572));
#194343=CARTESIAN_POINT('Origin',(109.683498835237,3.45,47.8340269691064));
#194344=CARTESIAN_POINT('',(109.683498835237,2.95,47.8340269691064));
#194345=CARTESIAN_POINT('',(109.626255861367,2.95,48.1285150706361));
#194346=CARTESIAN_POINT('',(109.683498835237,2.95,47.8340269691064));
#194347=CARTESIAN_POINT('',(109.626255861367,3.45,48.1285150706361));
#194348=CARTESIAN_POINT('',(109.683498835237,3.45,47.8340269691064));
#194349=CARTESIAN_POINT('Origin',(109.683498835237,2.95,47.8340269691064));
#194350=CARTESIAN_POINT('',(109.192685332687,2.95,47.7386220126572));
#194351=CARTESIAN_POINT('',(109.135442358818,2.95,48.0331101141869));
#194352=CARTESIAN_POINT('',(109.192685332687,2.95,47.7386220126572));
#194353=CARTESIAN_POINT('',(109.626255861367,2.95,48.1285150706361));
#194354=CARTESIAN_POINT('',(109.683498835237,2.95,47.8340269691064));
#194355=CARTESIAN_POINT('Origin',(109.192685332687,2.95,47.7386220126572));
#194356=CARTESIAN_POINT('',(109.135442358818,2.95,48.0331101141869));
#194357=CARTESIAN_POINT('',(109.192685332687,2.95,47.7386220126572));
#194358=CARTESIAN_POINT('Origin',(109.192685332687,2.65,47.7386220126572));
#194359=CARTESIAN_POINT('',(109.683498835237,2.65,47.8340269691064));
#194360=CARTESIAN_POINT('',(109.626255861367,2.65,48.1285150706361));
#194361=CARTESIAN_POINT('',(109.683498835237,2.65,47.8340269691064));
#194362=CARTESIAN_POINT('',(109.135442358818,2.65,48.0331101141869));
#194363=CARTESIAN_POINT('',(109.135442358818,2.65,48.0331101141869));
#194364=CARTESIAN_POINT('',(109.192685332687,2.65,47.7386220126572));
#194365=CARTESIAN_POINT('',(109.192685332687,2.65,47.7386220126572));
#194366=CARTESIAN_POINT('',(109.192685332687,2.65,47.7386220126572));
#194367=CARTESIAN_POINT('Origin',(109.683498835237,2.65,47.8340269691064));
#194368=CARTESIAN_POINT('',(109.683498835237,2.15,47.8340269691064));
#194369=CARTESIAN_POINT('',(109.626255861367,2.15,48.1285150706361));
#194370=CARTESIAN_POINT('',(109.683498835237,2.15,47.8340269691064));
#194371=CARTESIAN_POINT('',(109.626255861367,2.65,48.1285150706361));
#194372=CARTESIAN_POINT('',(109.683498835237,2.65,47.8340269691064));
#194373=CARTESIAN_POINT('Origin',(109.683498835237,2.15,47.8340269691064));
#194374=CARTESIAN_POINT('',(109.192685332687,2.15,47.7386220126572));
#194375=CARTESIAN_POINT('',(109.135442358818,2.15,48.0331101141869));
#194376=CARTESIAN_POINT('',(109.192685332687,2.15,47.7386220126572));
#194377=CARTESIAN_POINT('',(109.626255861367,2.15,48.1285150706361));
#194378=CARTESIAN_POINT('',(109.683498835237,2.15,47.8340269691064));
#194379=CARTESIAN_POINT('Origin',(109.192685332687,2.15,47.7386220126572));
#194380=CARTESIAN_POINT('',(109.135442358818,2.15,48.0331101141869));
#194381=CARTESIAN_POINT('',(109.192685332687,2.15,47.7386220126572));
#194382=CARTESIAN_POINT('Origin',(109.192685332687,1.85,47.7386220126572));
#194383=CARTESIAN_POINT('',(109.683498835237,1.85,47.8340269691064));
#194384=CARTESIAN_POINT('',(109.626255861367,1.85,48.1285150706361));
#194385=CARTESIAN_POINT('',(109.683498835237,1.85,47.8340269691064));
#194386=CARTESIAN_POINT('',(109.135442358818,1.85,48.0331101141869));
#194387=CARTESIAN_POINT('',(109.135442358818,1.85,48.0331101141869));
#194388=CARTESIAN_POINT('',(109.192685332687,1.85,47.7386220126572));
#194389=CARTESIAN_POINT('',(109.192685332687,1.85,47.7386220126572));
#194390=CARTESIAN_POINT('',(109.192685332687,1.85,47.7386220126572));
#194391=CARTESIAN_POINT('Origin',(109.683498835237,1.85,47.8340269691064));
#194392=CARTESIAN_POINT('',(109.683498835237,1.35,47.8340269691064));
#194393=CARTESIAN_POINT('',(109.626255861367,1.35,48.1285150706361));
#194394=CARTESIAN_POINT('',(109.683498835237,1.35,47.8340269691064));
#194395=CARTESIAN_POINT('',(109.626255861367,1.85,48.1285150706361));
#194396=CARTESIAN_POINT('',(109.683498835237,1.85,47.8340269691064));
#194397=CARTESIAN_POINT('Origin',(109.683498835237,1.35,47.8340269691064));
#194398=CARTESIAN_POINT('',(109.192685332687,1.35,47.7386220126572));
#194399=CARTESIAN_POINT('',(109.135442358818,1.35,48.0331101141869));
#194400=CARTESIAN_POINT('',(109.192685332687,1.35,47.7386220126572));
#194401=CARTESIAN_POINT('',(109.626255861367,1.35,48.1285150706361));
#194402=CARTESIAN_POINT('',(109.683498835237,1.35,47.8340269691064));
#194403=CARTESIAN_POINT('Origin',(109.192685332687,1.35,47.7386220126572));
#194404=CARTESIAN_POINT('',(109.135442358818,1.35,48.0331101141869));
#194405=CARTESIAN_POINT('',(109.192685332687,1.35,47.7386220126572));
#194406=CARTESIAN_POINT('Origin',(109.192685332687,1.05,47.7386220126572));
#194407=CARTESIAN_POINT('',(109.683498835237,1.05,47.8340269691064));
#194408=CARTESIAN_POINT('',(109.626255861367,1.05,48.1285150706361));
#194409=CARTESIAN_POINT('',(109.683498835237,1.05,47.8340269691064));
#194410=CARTESIAN_POINT('',(109.135442358818,1.05,48.0331101141869));
#194411=CARTESIAN_POINT('',(109.135442358818,1.05,48.0331101141869));
#194412=CARTESIAN_POINT('',(109.192685332687,1.05,47.7386220126572));
#194413=CARTESIAN_POINT('',(109.192685332687,1.05,47.7386220126572));
#194414=CARTESIAN_POINT('',(109.192685332687,1.05,47.7386220126572));
#194415=CARTESIAN_POINT('Origin',(109.683498835237,1.05,47.8340269691064));
#194416=CARTESIAN_POINT('',(109.683498835237,0.550000000000015,47.8340269691064));
#194417=CARTESIAN_POINT('',(109.626255861367,0.550000000000015,48.1285150706361));
#194418=CARTESIAN_POINT('',(109.683498835237,0.550000000000015,47.8340269691064));
#194419=CARTESIAN_POINT('',(109.626255861367,1.05,48.1285150706361));
#194420=CARTESIAN_POINT('',(109.683498835237,1.05,47.8340269691064));
#194421=CARTESIAN_POINT('Origin',(109.683498835237,0.550000000000015,47.8340269691064));
#194422=CARTESIAN_POINT('',(109.192685332687,0.550000000000015,47.7386220126572));
#194423=CARTESIAN_POINT('',(109.135442358818,0.550000000000015,48.0331101141869));
#194424=CARTESIAN_POINT('',(109.192685332687,0.550000000000015,47.7386220126572));
#194425=CARTESIAN_POINT('',(109.626255861367,0.550000000000015,48.1285150706361));
#194426=CARTESIAN_POINT('',(109.683498835237,0.550000000000015,47.8340269691064));
#194427=CARTESIAN_POINT('Origin',(109.192685332687,0.550000000000015,47.7386220126572));
#194428=CARTESIAN_POINT('',(109.135442358818,0.550000000000015,48.0331101141869));
#194429=CARTESIAN_POINT('',(109.192685332687,0.550000000000015,47.7386220126572));
#194430=CARTESIAN_POINT('Origin',(109.192685332687,0.250000000000015,47.7386220126572));
#194431=CARTESIAN_POINT('',(109.683498835237,0.250000000000015,47.8340269691064));
#194432=CARTESIAN_POINT('',(109.626255861367,0.250000000000015,48.1285150706361));
#194433=CARTESIAN_POINT('',(109.683498835237,0.250000000000015,47.8340269691064));
#194434=CARTESIAN_POINT('',(109.135442358818,0.250000000000015,48.0331101141869));
#194435=CARTESIAN_POINT('',(109.135442358818,0.250000000000015,48.0331101141869));
#194436=CARTESIAN_POINT('',(109.192685332687,0.250000000000015,47.7386220126572));
#194437=CARTESIAN_POINT('',(109.192685332687,0.250000000000015,47.7386220126572));
#194438=CARTESIAN_POINT('',(109.192685332687,0.250000000000015,47.7386220126572));
#194439=CARTESIAN_POINT('Origin',(109.683498835237,0.250000000000015,47.8340269691064));
#194440=CARTESIAN_POINT('',(109.683498835237,-0.249999999999985,47.8340269691064));
#194441=CARTESIAN_POINT('',(109.626255861367,-0.249999999999985,48.1285150706361));
#194442=CARTESIAN_POINT('',(109.683498835237,-0.249999999999985,47.8340269691064));
#194443=CARTESIAN_POINT('',(109.626255861367,0.250000000000015,48.1285150706361));
#194444=CARTESIAN_POINT('',(109.683498835237,0.250000000000015,47.8340269691064));
#194445=CARTESIAN_POINT('Origin',(109.683498835237,-0.249999999999985,47.8340269691064));
#194446=CARTESIAN_POINT('',(109.192685332687,-0.249999999999985,47.7386220126572));
#194447=CARTESIAN_POINT('',(109.135442358818,-0.249999999999985,48.0331101141869));
#194448=CARTESIAN_POINT('',(109.192685332687,-0.249999999999985,47.7386220126572));
#194449=CARTESIAN_POINT('',(109.626255861367,-0.249999999999985,48.1285150706361));
#194450=CARTESIAN_POINT('',(109.683498835237,-0.249999999999985,47.8340269691064));
#194451=CARTESIAN_POINT('Origin',(109.192685332687,-0.249999999999985,47.7386220126572));
#194452=CARTESIAN_POINT('',(109.135442358818,-0.249999999999985,48.0331101141869));
#194453=CARTESIAN_POINT('',(109.192685332687,-0.249999999999985,47.7386220126572));
#194454=CARTESIAN_POINT('Origin',(109.192685332687,-0.549999999999986,47.7386220126572));
#194455=CARTESIAN_POINT('',(109.683498835237,-0.549999999999986,47.8340269691064));
#194456=CARTESIAN_POINT('',(109.626255861367,-0.549999999999986,48.1285150706361));
#194457=CARTESIAN_POINT('',(109.683498835237,-0.549999999999986,47.8340269691064));
#194458=CARTESIAN_POINT('',(109.135442358818,-0.549999999999986,48.0331101141869));
#194459=CARTESIAN_POINT('',(109.135442358818,-0.549999999999986,48.0331101141869));
#194460=CARTESIAN_POINT('',(109.192685332687,-0.549999999999986,47.7386220126572));
#194461=CARTESIAN_POINT('',(109.192685332687,-0.549999999999986,47.7386220126572));
#194462=CARTESIAN_POINT('',(109.192685332687,-0.549999999999986,47.7386220126572));
#194463=CARTESIAN_POINT('Origin',(109.683498835237,-0.549999999999986,47.8340269691064));
#194464=CARTESIAN_POINT('',(109.683498835237,-1.05,47.8340269691064));
#194465=CARTESIAN_POINT('',(109.626255861367,-1.05,48.1285150706361));
#194466=CARTESIAN_POINT('',(109.683498835237,-1.05,47.8340269691064));
#194467=CARTESIAN_POINT('',(109.626255861367,-0.549999999999986,48.1285150706361));
#194468=CARTESIAN_POINT('',(109.683498835237,-0.549999999999986,47.8340269691064));
#194469=CARTESIAN_POINT('Origin',(109.683498835237,-1.05,47.8340269691064));
#194470=CARTESIAN_POINT('',(109.192685332687,-1.05,47.7386220126572));
#194471=CARTESIAN_POINT('',(109.135442358818,-1.05,48.0331101141869));
#194472=CARTESIAN_POINT('',(109.192685332687,-1.05,47.7386220126572));
#194473=CARTESIAN_POINT('',(109.626255861367,-1.05,48.1285150706361));
#194474=CARTESIAN_POINT('',(109.683498835237,-1.05,47.8340269691064));
#194475=CARTESIAN_POINT('Origin',(109.192685332687,-1.05,47.7386220126572));
#194476=CARTESIAN_POINT('',(109.135442358818,-1.05,48.0331101141869));
#194477=CARTESIAN_POINT('',(109.192685332687,-1.05,47.7386220126572));
#194478=CARTESIAN_POINT('Origin',(109.192685332687,-1.35,47.7386220126572));
#194479=CARTESIAN_POINT('',(109.683498835237,-1.35,47.8340269691064));
#194480=CARTESIAN_POINT('',(109.626255861367,-1.35,48.1285150706361));
#194481=CARTESIAN_POINT('',(109.683498835237,-1.35,47.8340269691064));
#194482=CARTESIAN_POINT('',(109.135442358818,-1.35,48.0331101141869));
#194483=CARTESIAN_POINT('',(109.135442358818,-1.35,48.0331101141869));
#194484=CARTESIAN_POINT('',(109.192685332687,-1.35,47.7386220126572));
#194485=CARTESIAN_POINT('',(109.192685332687,-1.35,47.7386220126572));
#194486=CARTESIAN_POINT('',(109.192685332687,-1.35,47.7386220126572));
#194487=CARTESIAN_POINT('Origin',(109.683498835237,-1.35,47.8340269691064));
#194488=CARTESIAN_POINT('',(109.683498835237,-1.85,47.8340269691064));
#194489=CARTESIAN_POINT('',(109.626255861367,-1.85,48.1285150706361));
#194490=CARTESIAN_POINT('',(109.683498835237,-1.85,47.8340269691064));
#194491=CARTESIAN_POINT('',(109.626255861367,-1.35,48.1285150706361));
#194492=CARTESIAN_POINT('',(109.683498835237,-1.35,47.8340269691064));
#194493=CARTESIAN_POINT('Origin',(109.683498835237,-1.85,47.8340269691064));
#194494=CARTESIAN_POINT('',(109.192685332687,-1.85,47.7386220126572));
#194495=CARTESIAN_POINT('',(109.135442358818,-1.85,48.0331101141869));
#194496=CARTESIAN_POINT('',(109.192685332687,-1.85,47.7386220126572));
#194497=CARTESIAN_POINT('',(109.626255861367,-1.85,48.1285150706361));
#194498=CARTESIAN_POINT('',(109.683498835237,-1.85,47.8340269691064));
#194499=CARTESIAN_POINT('Origin',(109.192685332687,-1.85,47.7386220126572));
#194500=CARTESIAN_POINT('',(109.135442358818,-1.85,48.0331101141869));
#194501=CARTESIAN_POINT('',(109.192685332687,-1.85,47.7386220126572));
#194502=CARTESIAN_POINT('Origin',(109.192685332687,-2.15,47.7386220126572));
#194503=CARTESIAN_POINT('',(109.683498835237,-2.15,47.8340269691064));
#194504=CARTESIAN_POINT('',(109.626255861367,-2.15,48.1285150706361));
#194505=CARTESIAN_POINT('',(109.683498835237,-2.15,47.8340269691064));
#194506=CARTESIAN_POINT('',(109.135442358818,-2.15,48.0331101141869));
#194507=CARTESIAN_POINT('',(109.135442358818,-2.15,48.0331101141869));
#194508=CARTESIAN_POINT('',(109.192685332687,-2.15,47.7386220126572));
#194509=CARTESIAN_POINT('',(109.192685332687,-2.15,47.7386220126572));
#194510=CARTESIAN_POINT('',(109.192685332687,-2.15,47.7386220126572));
#194511=CARTESIAN_POINT('Origin',(109.683498835237,-2.15,47.8340269691064));
#194512=CARTESIAN_POINT('',(109.683498835237,-2.65,47.8340269691064));
#194513=CARTESIAN_POINT('',(109.626255861367,-2.65,48.1285150706361));
#194514=CARTESIAN_POINT('',(109.683498835237,-2.65,47.8340269691064));
#194515=CARTESIAN_POINT('',(109.626255861367,-2.15,48.1285150706361));
#194516=CARTESIAN_POINT('',(109.683498835237,-2.15,47.8340269691064));
#194517=CARTESIAN_POINT('Origin',(109.683498835237,-2.65,47.8340269691064));
#194518=CARTESIAN_POINT('',(109.192685332687,-2.65,47.7386220126572));
#194519=CARTESIAN_POINT('',(109.135442358818,-2.65,48.0331101141869));
#194520=CARTESIAN_POINT('',(109.192685332687,-2.65,47.7386220126572));
#194521=CARTESIAN_POINT('',(109.626255861367,-2.65,48.1285150706361));
#194522=CARTESIAN_POINT('',(109.683498835237,-2.65,47.8340269691064));
#194523=CARTESIAN_POINT('Origin',(109.192685332687,-2.65,47.7386220126572));
#194524=CARTESIAN_POINT('',(109.135442358818,-2.65,48.0331101141869));
#194525=CARTESIAN_POINT('',(109.192685332687,-2.65,47.7386220126572));
#194526=CARTESIAN_POINT('Origin',(109.192685332687,-2.95,47.7386220126572));
#194527=CARTESIAN_POINT('',(109.683498835237,-2.95,47.8340269691064));
#194528=CARTESIAN_POINT('',(109.626255861367,-2.95,48.1285150706361));
#194529=CARTESIAN_POINT('',(109.683498835237,-2.95,47.8340269691064));
#194530=CARTESIAN_POINT('',(109.135442358818,-2.95,48.0331101141869));
#194531=CARTESIAN_POINT('',(109.135442358818,-2.95,48.0331101141869));
#194532=CARTESIAN_POINT('',(109.192685332687,-2.95,47.7386220126572));
#194533=CARTESIAN_POINT('',(109.192685332687,-2.95,47.7386220126572));
#194534=CARTESIAN_POINT('',(109.192685332687,-2.95,47.7386220126572));
#194535=CARTESIAN_POINT('Origin',(109.683498835237,-2.95,47.8340269691064));
#194536=CARTESIAN_POINT('',(109.683498835237,-3.45,47.8340269691064));
#194537=CARTESIAN_POINT('',(109.626255861367,-3.45,48.1285150706361));
#194538=CARTESIAN_POINT('',(109.683498835237,-3.45,47.8340269691064));
#194539=CARTESIAN_POINT('',(109.626255861367,-2.95,48.1285150706361));
#194540=CARTESIAN_POINT('',(109.683498835237,-2.95,47.8340269691064));
#194541=CARTESIAN_POINT('Origin',(109.683498835237,-3.45,47.8340269691064));
#194542=CARTESIAN_POINT('',(109.192685332687,-3.45,47.7386220126572));
#194543=CARTESIAN_POINT('',(109.135442358818,-3.45,48.0331101141869));
#194544=CARTESIAN_POINT('',(109.192685332687,-3.45,47.7386220126572));
#194545=CARTESIAN_POINT('',(109.626255861367,-3.45,48.1285150706361));
#194546=CARTESIAN_POINT('',(109.683498835237,-3.45,47.8340269691064));
#194547=CARTESIAN_POINT('Origin',(109.192685332687,-3.45,47.7386220126572));
#194548=CARTESIAN_POINT('',(109.135442358818,-3.45,48.0331101141869));
#194549=CARTESIAN_POINT('',(109.192685332687,-3.45,47.7386220126572));
#194550=CARTESIAN_POINT('Origin',(109.192685332687,-3.75,47.7386220126572));
#194551=CARTESIAN_POINT('',(109.683498835237,-3.75,47.8340269691064));
#194552=CARTESIAN_POINT('',(109.626255861367,-3.75,48.1285150706361));
#194553=CARTESIAN_POINT('',(109.683498835237,-3.75,47.8340269691064));
#194554=CARTESIAN_POINT('',(109.135442358818,-3.75,48.0331101141869));
#194555=CARTESIAN_POINT('',(109.135442358818,-3.75,48.0331101141869));
#194556=CARTESIAN_POINT('',(109.192685332687,-3.75,47.7386220126572));
#194557=CARTESIAN_POINT('',(109.192685332687,-3.75,47.7386220126572));
#194558=CARTESIAN_POINT('',(109.192685332687,-3.75,47.7386220126572));
#194559=CARTESIAN_POINT('Origin',(109.683498835237,-3.75,47.8340269691064));
#194560=CARTESIAN_POINT('',(109.683498835237,-4.25,47.8340269691064));
#194561=CARTESIAN_POINT('',(109.626255861367,-4.25,48.1285150706361));
#194562=CARTESIAN_POINT('',(109.683498835237,-4.25,47.8340269691064));
#194563=CARTESIAN_POINT('',(109.626255861367,-3.75,48.1285150706361));
#194564=CARTESIAN_POINT('',(109.683498835237,-3.75,47.8340269691064));
#194565=CARTESIAN_POINT('Origin',(109.683498835237,-4.25,47.8340269691064));
#194566=CARTESIAN_POINT('',(109.192685332687,-4.25,47.7386220126572));
#194567=CARTESIAN_POINT('',(109.135442358818,-4.25,48.0331101141869));
#194568=CARTESIAN_POINT('',(109.192685332687,-4.25,47.7386220126572));
#194569=CARTESIAN_POINT('',(109.626255861367,-4.25,48.1285150706361));
#194570=CARTESIAN_POINT('',(109.683498835237,-4.25,47.8340269691064));
#194571=CARTESIAN_POINT('Origin',(109.192685332687,-4.25,47.7386220126572));
#194572=CARTESIAN_POINT('',(109.135442358818,-4.25,48.0331101141869));
#194573=CARTESIAN_POINT('',(109.192685332687,-4.25,47.7386220126572));
#194574=CARTESIAN_POINT('Origin',(109.192685332687,-4.55,47.7386220126572));
#194575=CARTESIAN_POINT('',(109.683498835237,-4.55,47.8340269691064));
#194576=CARTESIAN_POINT('',(109.626255861367,-4.55,48.1285150706361));
#194577=CARTESIAN_POINT('',(109.683498835237,-4.55,47.8340269691064));
#194578=CARTESIAN_POINT('',(109.135442358818,-4.55,48.0331101141869));
#194579=CARTESIAN_POINT('',(109.135442358818,-4.55,48.0331101141869));
#194580=CARTESIAN_POINT('',(109.192685332687,-4.55,47.7386220126572));
#194581=CARTESIAN_POINT('',(109.192685332687,-4.55,47.7386220126572));
#194582=CARTESIAN_POINT('',(109.192685332687,-4.55,47.7386220126572));
#194583=CARTESIAN_POINT('Origin',(109.683498835237,-4.55,47.8340269691064));
#194584=CARTESIAN_POINT('',(109.683498835237,-5.05,47.8340269691064));
#194585=CARTESIAN_POINT('',(109.626255861367,-5.05,48.1285150706361));
#194586=CARTESIAN_POINT('',(109.683498835237,-5.05,47.8340269691064));
#194587=CARTESIAN_POINT('',(109.626255861367,-4.55,48.1285150706361));
#194588=CARTESIAN_POINT('',(109.683498835237,-4.55,47.8340269691064));
#194589=CARTESIAN_POINT('Origin',(109.683498835237,-5.05,47.8340269691064));
#194590=CARTESIAN_POINT('',(109.192685332687,-5.05,47.7386220126572));
#194591=CARTESIAN_POINT('',(109.135442358818,-5.05,48.0331101141869));
#194592=CARTESIAN_POINT('',(109.192685332687,-5.05,47.7386220126572));
#194593=CARTESIAN_POINT('',(109.626255861367,-5.05,48.1285150706361));
#194594=CARTESIAN_POINT('',(109.683498835237,-5.05,47.8340269691064));
#194595=CARTESIAN_POINT('Origin',(109.192685332687,-5.05,47.7386220126572));
#194596=CARTESIAN_POINT('',(109.135442358818,-5.05,48.0331101141869));
#194597=CARTESIAN_POINT('',(109.192685332687,-5.05,47.7386220126572));
#194598=CARTESIAN_POINT('Origin',(112.333891749004,-7.75,48.3492137339324));
#194599=CARTESIAN_POINT('',(112.824705251554,-7.75,48.4446186903817));
#194600=CARTESIAN_POINT('',(112.767462277684,-7.75,48.7391067919114));
#194601=CARTESIAN_POINT('',(112.824705251554,-7.75,48.4446186903817));
#194602=CARTESIAN_POINT('',(112.276648775135,-7.75,48.6437018354621));
#194603=CARTESIAN_POINT('',(112.276648775135,-7.75,48.6437018354621));
#194604=CARTESIAN_POINT('',(112.333891749004,-7.75,48.3492137339324));
#194605=CARTESIAN_POINT('',(112.333891749004,-7.75,48.3492137339324));
#194606=CARTESIAN_POINT('',(112.333891749004,-7.75,48.3492137339324));
#194607=CARTESIAN_POINT('Origin',(112.824705251554,-7.75,48.4446186903817));
#194608=CARTESIAN_POINT('',(112.824705251554,-8.25,48.4446186903817));
#194609=CARTESIAN_POINT('',(112.767462277684,-8.25,48.7391067919114));
#194610=CARTESIAN_POINT('',(112.824705251554,-8.25,48.4446186903817));
#194611=CARTESIAN_POINT('',(112.767462277684,-7.75,48.7391067919114));
#194612=CARTESIAN_POINT('',(112.824705251554,-7.75,48.4446186903817));
#194613=CARTESIAN_POINT('Origin',(112.824705251554,-8.25,48.4446186903817));
#194614=CARTESIAN_POINT('',(112.333891749004,-8.25,48.3492137339324));
#194615=CARTESIAN_POINT('',(112.276648775135,-8.25,48.6437018354621));
#194616=CARTESIAN_POINT('',(112.333891749004,-8.25,48.3492137339324));
#194617=CARTESIAN_POINT('',(112.767462277684,-8.25,48.7391067919114));
#194618=CARTESIAN_POINT('',(112.824705251554,-8.25,48.4446186903817));
#194619=CARTESIAN_POINT('Origin',(112.333891749004,-8.25,48.3492137339324));
#194620=CARTESIAN_POINT('',(112.276648775135,-8.25,48.6437018354621));
#194621=CARTESIAN_POINT('',(112.333891749004,-8.25,48.3492137339324));
#194622=CARTESIAN_POINT('Origin',(113.119193353083,-7.75,48.5018616642512));
#194623=CARTESIAN_POINT('',(113.610006855633,-7.75,48.5972666207005));
#194624=CARTESIAN_POINT('',(113.552763881763,-7.75,48.8917547222302));
#194625=CARTESIAN_POINT('',(113.610006855633,-7.75,48.5972666207005));
#194626=CARTESIAN_POINT('',(113.061950379214,-7.75,48.7963497657809));
#194627=CARTESIAN_POINT('',(113.061950379214,-7.75,48.7963497657809));
#194628=CARTESIAN_POINT('',(113.119193353083,-7.75,48.5018616642512));
#194629=CARTESIAN_POINT('',(113.119193353083,-7.75,48.5018616642512));
#194630=CARTESIAN_POINT('',(113.119193353083,-7.75,48.5018616642512));
#194631=CARTESIAN_POINT('Origin',(113.610006855633,-7.75,48.5972666207005));
#194632=CARTESIAN_POINT('',(113.610006855633,-8.25,48.5972666207005));
#194633=CARTESIAN_POINT('',(113.552763881763,-8.25,48.8917547222302));
#194634=CARTESIAN_POINT('',(113.610006855633,-8.25,48.5972666207005));
#194635=CARTESIAN_POINT('',(113.552763881763,-7.75,48.8917547222302));
#194636=CARTESIAN_POINT('',(113.610006855633,-7.75,48.5972666207005));
#194637=CARTESIAN_POINT('Origin',(113.610006855633,-8.25,48.5972666207005));
#194638=CARTESIAN_POINT('',(113.119193353083,-8.25,48.5018616642512));
#194639=CARTESIAN_POINT('',(113.061950379214,-8.25,48.7963497657809));
#194640=CARTESIAN_POINT('',(113.119193353083,-8.25,48.5018616642512));
#194641=CARTESIAN_POINT('',(113.552763881763,-8.25,48.8917547222302));
#194642=CARTESIAN_POINT('',(113.610006855633,-8.25,48.5972666207005));
#194643=CARTESIAN_POINT('Origin',(113.119193353083,-8.25,48.5018616642512));
#194644=CARTESIAN_POINT('',(113.061950379214,-8.25,48.7963497657809));
#194645=CARTESIAN_POINT('',(113.119193353083,-8.25,48.5018616642512));
#194646=CARTESIAN_POINT('Origin',(113.904494957163,-7.75,48.65450959457));
#194647=CARTESIAN_POINT('',(114.395308459712,-7.75,48.7499145510193));
#194648=CARTESIAN_POINT('',(114.338065485842,-7.75,49.044402652549));
#194649=CARTESIAN_POINT('',(114.395308459712,-7.75,48.7499145510193));
#194650=CARTESIAN_POINT('',(113.847251983293,-7.75,48.9489976960997));
#194651=CARTESIAN_POINT('',(113.847251983293,-7.75,48.9489976960997));
#194652=CARTESIAN_POINT('',(113.904494957163,-7.75,48.65450959457));
#194653=CARTESIAN_POINT('',(113.904494957163,-7.75,48.65450959457));
#194654=CARTESIAN_POINT('',(113.904494957163,-7.75,48.65450959457));
#194655=CARTESIAN_POINT('Origin',(114.395308459712,-7.75,48.7499145510193));
#194656=CARTESIAN_POINT('',(114.395308459712,-8.25,48.7499145510193));
#194657=CARTESIAN_POINT('',(114.338065485842,-8.25,49.044402652549));
#194658=CARTESIAN_POINT('',(114.395308459712,-8.25,48.7499145510193));
#194659=CARTESIAN_POINT('',(114.338065485842,-7.75,49.044402652549));
#194660=CARTESIAN_POINT('',(114.395308459712,-7.75,48.7499145510193));
#194661=CARTESIAN_POINT('Origin',(114.395308459712,-8.25,48.7499145510193));
#194662=CARTESIAN_POINT('',(113.904494957163,-8.25,48.65450959457));
#194663=CARTESIAN_POINT('',(113.847251983293,-8.25,48.9489976960997));
#194664=CARTESIAN_POINT('',(113.904494957163,-8.25,48.65450959457));
#194665=CARTESIAN_POINT('',(114.338065485842,-8.25,49.044402652549));
#194666=CARTESIAN_POINT('',(114.395308459712,-8.25,48.7499145510193));
#194667=CARTESIAN_POINT('Origin',(113.904494957163,-8.25,48.65450959457));
#194668=CARTESIAN_POINT('',(113.847251983293,-8.25,48.9489976960997));
#194669=CARTESIAN_POINT('',(113.904494957163,-8.25,48.65450959457));
#194670=CARTESIAN_POINT('Origin',(114.689796561242,-7.75,48.8071575248888));
#194671=CARTESIAN_POINT('',(115.180610063791,-7.75,48.9025624813381));
#194672=CARTESIAN_POINT('',(115.123367089922,-7.75,49.1970505828678));
#194673=CARTESIAN_POINT('',(115.180610063791,-7.75,48.9025624813381));
#194674=CARTESIAN_POINT('',(114.632553587372,-7.75,49.1016456264185));
#194675=CARTESIAN_POINT('',(114.632553587372,-7.75,49.1016456264185));
#194676=CARTESIAN_POINT('',(114.689796561242,-7.75,48.8071575248888));
#194677=CARTESIAN_POINT('',(114.689796561242,-7.75,48.8071575248888));
#194678=CARTESIAN_POINT('',(114.689796561242,-7.75,48.8071575248888));
#194679=CARTESIAN_POINT('Origin',(115.180610063791,-7.75,48.9025624813381));
#194680=CARTESIAN_POINT('',(115.180610063791,-8.25,48.9025624813381));
#194681=CARTESIAN_POINT('',(115.123367089922,-8.25,49.1970505828678));
#194682=CARTESIAN_POINT('',(115.180610063791,-8.25,48.9025624813381));
#194683=CARTESIAN_POINT('',(115.123367089922,-7.75,49.1970505828678));
#194684=CARTESIAN_POINT('',(115.180610063791,-7.75,48.9025624813381));
#194685=CARTESIAN_POINT('Origin',(115.180610063791,-8.25,48.9025624813381));
#194686=CARTESIAN_POINT('',(114.689796561242,-8.25,48.8071575248888));
#194687=CARTESIAN_POINT('',(114.632553587372,-8.25,49.1016456264185));
#194688=CARTESIAN_POINT('',(114.689796561242,-8.25,48.8071575248888));
#194689=CARTESIAN_POINT('',(115.123367089922,-8.25,49.1970505828678));
#194690=CARTESIAN_POINT('',(115.180610063791,-8.25,48.9025624813381));
#194691=CARTESIAN_POINT('Origin',(114.689796561242,-8.25,48.8071575248888));
#194692=CARTESIAN_POINT('',(114.632553587372,-8.25,49.1016456264185));
#194693=CARTESIAN_POINT('',(114.689796561242,-8.25,48.8071575248888));
#194694=CARTESIAN_POINT('Origin',(115.475098165321,-7.75,48.9598054552076));
#194695=CARTESIAN_POINT('',(115.96591166787,-7.75,49.0552104116569));
#194696=CARTESIAN_POINT('',(115.908668694001,-7.75,49.3496985131866));
#194697=CARTESIAN_POINT('',(115.96591166787,-7.75,49.0552104116569));
#194698=CARTESIAN_POINT('',(115.417855191451,-7.75,49.2542935567373));
#194699=CARTESIAN_POINT('',(115.417855191451,-7.75,49.2542935567373));
#194700=CARTESIAN_POINT('',(115.475098165321,-7.75,48.9598054552076));
#194701=CARTESIAN_POINT('',(115.475098165321,-7.75,48.9598054552076));
#194702=CARTESIAN_POINT('',(115.475098165321,-7.75,48.9598054552076));
#194703=CARTESIAN_POINT('Origin',(115.96591166787,-7.75,49.0552104116569));
#194704=CARTESIAN_POINT('',(115.96591166787,-8.25,49.0552104116569));
#194705=CARTESIAN_POINT('',(115.908668694001,-8.25,49.3496985131866));
#194706=CARTESIAN_POINT('',(115.96591166787,-8.25,49.0552104116569));
#194707=CARTESIAN_POINT('',(115.908668694001,-7.75,49.3496985131866));
#194708=CARTESIAN_POINT('',(115.96591166787,-7.75,49.0552104116569));
#194709=CARTESIAN_POINT('Origin',(115.96591166787,-8.25,49.0552104116569));
#194710=CARTESIAN_POINT('',(115.475098165321,-8.25,48.9598054552076));
#194711=CARTESIAN_POINT('',(115.417855191451,-8.25,49.2542935567373));
#194712=CARTESIAN_POINT('',(115.475098165321,-8.25,48.9598054552076));
#194713=CARTESIAN_POINT('',(115.908668694001,-8.25,49.3496985131866));
#194714=CARTESIAN_POINT('',(115.96591166787,-8.25,49.0552104116569));
#194715=CARTESIAN_POINT('Origin',(115.475098165321,-8.25,48.9598054552076));
#194716=CARTESIAN_POINT('',(115.417855191451,-8.25,49.2542935567373));
#194717=CARTESIAN_POINT('',(115.475098165321,-8.25,48.9598054552076));
#194718=CARTESIAN_POINT('Origin',(116.2603997694,-7.75,49.1124533855264));
#194719=CARTESIAN_POINT('',(116.75121327195,-7.75,49.2078583419757));
#194720=CARTESIAN_POINT('',(116.69397029808,-7.75,49.5023464435054));
#194721=CARTESIAN_POINT('',(116.75121327195,-7.75,49.2078583419757));
#194722=CARTESIAN_POINT('',(116.203156795531,-7.75,49.4069414870561));
#194723=CARTESIAN_POINT('',(116.203156795531,-7.75,49.4069414870561));
#194724=CARTESIAN_POINT('',(116.2603997694,-7.75,49.1124533855264));
#194725=CARTESIAN_POINT('',(116.2603997694,-7.75,49.1124533855264));
#194726=CARTESIAN_POINT('',(116.2603997694,-7.75,49.1124533855264));
#194727=CARTESIAN_POINT('Origin',(116.75121327195,-7.75,49.2078583419757));
#194728=CARTESIAN_POINT('',(116.75121327195,-8.25,49.2078583419757));
#194729=CARTESIAN_POINT('',(116.69397029808,-8.25,49.5023464435054));
#194730=CARTESIAN_POINT('',(116.75121327195,-8.25,49.2078583419757));
#194731=CARTESIAN_POINT('',(116.69397029808,-7.75,49.5023464435054));
#194732=CARTESIAN_POINT('',(116.75121327195,-7.75,49.2078583419757));
#194733=CARTESIAN_POINT('Origin',(116.75121327195,-8.25,49.2078583419757));
#194734=CARTESIAN_POINT('',(116.2603997694,-8.25,49.1124533855264));
#194735=CARTESIAN_POINT('',(116.203156795531,-8.25,49.4069414870561));
#194736=CARTESIAN_POINT('',(116.2603997694,-8.25,49.1124533855264));
#194737=CARTESIAN_POINT('',(116.69397029808,-8.25,49.5023464435054));
#194738=CARTESIAN_POINT('',(116.75121327195,-8.25,49.2078583419757));
#194739=CARTESIAN_POINT('Origin',(116.2603997694,-8.25,49.1124533855264));
#194740=CARTESIAN_POINT('',(116.203156795531,-8.25,49.4069414870561));
#194741=CARTESIAN_POINT('',(116.2603997694,-8.25,49.1124533855264));
#194742=CARTESIAN_POINT('Origin',(117.045701373479,-7.75,49.2651013158452));
#194743=CARTESIAN_POINT('',(117.536514876029,-7.75,49.3605062722945));
#194744=CARTESIAN_POINT('',(117.479271902159,-7.75,49.6549943738242));
#194745=CARTESIAN_POINT('',(117.536514876029,-7.75,49.3605062722945));
#194746=CARTESIAN_POINT('',(116.98845839961,-7.75,49.5595894173749));
#194747=CARTESIAN_POINT('',(116.98845839961,-7.75,49.5595894173749));
#194748=CARTESIAN_POINT('',(117.045701373479,-7.75,49.2651013158452));
#194749=CARTESIAN_POINT('',(117.045701373479,-7.75,49.2651013158452));
#194750=CARTESIAN_POINT('',(117.045701373479,-7.75,49.2651013158452));
#194751=CARTESIAN_POINT('Origin',(117.536514876029,-7.75,49.3605062722945));
#194752=CARTESIAN_POINT('',(117.536514876029,-8.25,49.3605062722945));
#194753=CARTESIAN_POINT('',(117.479271902159,-8.25,49.6549943738242));
#194754=CARTESIAN_POINT('',(117.536514876029,-8.25,49.3605062722945));
#194755=CARTESIAN_POINT('',(117.479271902159,-7.75,49.6549943738242));
#194756=CARTESIAN_POINT('',(117.536514876029,-7.75,49.3605062722945));
#194757=CARTESIAN_POINT('Origin',(117.536514876029,-8.25,49.3605062722945));
#194758=CARTESIAN_POINT('',(117.045701373479,-8.25,49.2651013158452));
#194759=CARTESIAN_POINT('',(116.98845839961,-8.25,49.5595894173749));
#194760=CARTESIAN_POINT('',(117.045701373479,-8.25,49.2651013158452));
#194761=CARTESIAN_POINT('',(117.479271902159,-8.25,49.6549943738242));
#194762=CARTESIAN_POINT('',(117.536514876029,-8.25,49.3605062722945));
#194763=CARTESIAN_POINT('Origin',(117.045701373479,-8.25,49.2651013158452));
#194764=CARTESIAN_POINT('',(116.98845839961,-8.25,49.5595894173749));
#194765=CARTESIAN_POINT('',(117.045701373479,-8.25,49.2651013158452));
#194766=CARTESIAN_POINT('Origin',(117.831002977559,-7.75,49.417749246164));
#194767=CARTESIAN_POINT('',(118.321816480108,-7.75,49.5131542026133));
#194768=CARTESIAN_POINT('',(118.264573506239,-7.75,49.807642304143));
#194769=CARTESIAN_POINT('',(118.321816480108,-7.75,49.5131542026133));
#194770=CARTESIAN_POINT('',(117.773760003689,-7.75,49.7122373476937));
#194771=CARTESIAN_POINT('',(117.773760003689,-7.75,49.7122373476937));
#194772=CARTESIAN_POINT('',(117.831002977559,-7.75,49.417749246164));
#194773=CARTESIAN_POINT('',(117.831002977559,-7.75,49.417749246164));
#194774=CARTESIAN_POINT('',(117.831002977559,-7.75,49.417749246164));
#194775=CARTESIAN_POINT('Origin',(118.321816480108,-7.75,49.5131542026133));
#194776=CARTESIAN_POINT('',(118.321816480108,-8.25,49.5131542026133));
#194777=CARTESIAN_POINT('',(118.264573506239,-8.25,49.807642304143));
#194778=CARTESIAN_POINT('',(118.321816480108,-8.25,49.5131542026133));
#194779=CARTESIAN_POINT('',(118.264573506239,-7.75,49.807642304143));
#194780=CARTESIAN_POINT('',(118.321816480108,-7.75,49.5131542026133));
#194781=CARTESIAN_POINT('Origin',(118.321816480108,-8.25,49.5131542026133));
#194782=CARTESIAN_POINT('',(117.831002977559,-8.25,49.417749246164));
#194783=CARTESIAN_POINT('',(117.773760003689,-8.25,49.7122373476937));
#194784=CARTESIAN_POINT('',(117.831002977559,-8.25,49.417749246164));
#194785=CARTESIAN_POINT('',(118.264573506239,-8.25,49.807642304143));
#194786=CARTESIAN_POINT('',(118.321816480108,-8.25,49.5131542026133));
#194787=CARTESIAN_POINT('Origin',(117.831002977559,-8.25,49.417749246164));
#194788=CARTESIAN_POINT('',(117.773760003689,-8.25,49.7122373476937));
#194789=CARTESIAN_POINT('',(117.831002977559,-8.25,49.417749246164));
#194790=CARTESIAN_POINT('Origin',(118.616304581638,-7.75,49.5703971764828));
#194791=CARTESIAN_POINT('',(119.107118084187,-7.75,49.6658021329321));
#194792=CARTESIAN_POINT('',(119.049875110318,-7.75,49.9602902344618));
#194793=CARTESIAN_POINT('',(119.107118084187,-7.75,49.6658021329321));
#194794=CARTESIAN_POINT('',(118.559061607768,-7.75,49.8648852780125));
#194795=CARTESIAN_POINT('',(118.559061607768,-7.75,49.8648852780125));
#194796=CARTESIAN_POINT('',(118.616304581638,-7.75,49.5703971764828));
#194797=CARTESIAN_POINT('',(118.616304581638,-7.75,49.5703971764828));
#194798=CARTESIAN_POINT('',(118.616304581638,-7.75,49.5703971764828));
#194799=CARTESIAN_POINT('Origin',(119.107118084187,-7.75,49.6658021329321));
#194800=CARTESIAN_POINT('',(119.107118084187,-8.25,49.6658021329321));
#194801=CARTESIAN_POINT('',(119.049875110318,-8.25,49.9602902344618));
#194802=CARTESIAN_POINT('',(119.107118084187,-8.25,49.6658021329321));
#194803=CARTESIAN_POINT('',(119.049875110318,-7.75,49.9602902344618));
#194804=CARTESIAN_POINT('',(119.107118084187,-7.75,49.6658021329321));
#194805=CARTESIAN_POINT('Origin',(119.107118084187,-8.25,49.6658021329321));
#194806=CARTESIAN_POINT('',(118.616304581638,-8.25,49.5703971764828));
#194807=CARTESIAN_POINT('',(118.559061607768,-8.25,49.8648852780125));
#194808=CARTESIAN_POINT('',(118.616304581638,-8.25,49.5703971764828));
#194809=CARTESIAN_POINT('',(119.049875110318,-8.25,49.9602902344618));
#194810=CARTESIAN_POINT('',(119.107118084187,-8.25,49.6658021329321));
#194811=CARTESIAN_POINT('Origin',(118.616304581638,-8.25,49.5703971764828));
#194812=CARTESIAN_POINT('',(118.559061607768,-8.25,49.8648852780125));
#194813=CARTESIAN_POINT('',(118.616304581638,-8.25,49.5703971764828));
#194814=CARTESIAN_POINT('Origin',(119.401606185717,-7.75,49.7230451068016));
#194815=CARTESIAN_POINT('',(119.892419688267,-7.75,49.8184500632509));
#194816=CARTESIAN_POINT('',(119.835176714397,-7.75,50.1129381647806));
#194817=CARTESIAN_POINT('',(119.892419688267,-7.75,49.8184500632509));
#194818=CARTESIAN_POINT('',(119.344363211847,-7.75,50.0175332083313));
#194819=CARTESIAN_POINT('',(119.344363211847,-7.75,50.0175332083313));
#194820=CARTESIAN_POINT('',(119.401606185717,-7.75,49.7230451068016));
#194821=CARTESIAN_POINT('',(119.401606185717,-7.75,49.7230451068016));
#194822=CARTESIAN_POINT('',(119.401606185717,-7.75,49.7230451068016));
#194823=CARTESIAN_POINT('Origin',(119.892419688267,-7.75,49.8184500632509));
#194824=CARTESIAN_POINT('',(119.892419688267,-8.25,49.8184500632509));
#194825=CARTESIAN_POINT('',(119.835176714397,-8.25,50.1129381647806));
#194826=CARTESIAN_POINT('',(119.892419688267,-8.25,49.8184500632509));
#194827=CARTESIAN_POINT('',(119.835176714397,-7.75,50.1129381647806));
#194828=CARTESIAN_POINT('',(119.892419688267,-7.75,49.8184500632509));
#194829=CARTESIAN_POINT('Origin',(119.892419688267,-8.25,49.8184500632509));
#194830=CARTESIAN_POINT('',(119.401606185717,-8.25,49.7230451068016));
#194831=CARTESIAN_POINT('',(119.344363211847,-8.25,50.0175332083313));
#194832=CARTESIAN_POINT('',(119.401606185717,-8.25,49.7230451068016));
#194833=CARTESIAN_POINT('',(119.835176714397,-8.25,50.1129381647806));
#194834=CARTESIAN_POINT('',(119.892419688267,-8.25,49.8184500632509));
#194835=CARTESIAN_POINT('Origin',(119.401606185717,-8.25,49.7230451068016));
#194836=CARTESIAN_POINT('',(119.344363211847,-8.25,50.0175332083313));
#194837=CARTESIAN_POINT('',(119.401606185717,-8.25,49.7230451068016));
#194838=CARTESIAN_POINT('Origin',(120.186907789796,-7.75,49.8756930371204));
#194839=CARTESIAN_POINT('',(120.677721292346,-7.75,49.9710979935697));
#194840=CARTESIAN_POINT('',(120.620478318476,-7.75,50.2655860950994));
#194841=CARTESIAN_POINT('',(120.677721292346,-7.75,49.9710979935697));
#194842=CARTESIAN_POINT('',(120.129664815927,-7.75,50.1701811386501));
#194843=CARTESIAN_POINT('',(120.129664815927,-7.75,50.1701811386501));
#194844=CARTESIAN_POINT('',(120.186907789796,-7.75,49.8756930371204));
#194845=CARTESIAN_POINT('',(120.186907789796,-7.75,49.8756930371204));
#194846=CARTESIAN_POINT('',(120.186907789796,-7.75,49.8756930371204));
#194847=CARTESIAN_POINT('Origin',(120.677721292346,-7.75,49.9710979935697));
#194848=CARTESIAN_POINT('',(120.677721292346,-8.25,49.9710979935697));
#194849=CARTESIAN_POINT('',(120.620478318476,-8.25,50.2655860950994));
#194850=CARTESIAN_POINT('',(120.677721292346,-8.25,49.9710979935697));
#194851=CARTESIAN_POINT('',(120.620478318476,-7.75,50.2655860950994));
#194852=CARTESIAN_POINT('',(120.677721292346,-7.75,49.9710979935697));
#194853=CARTESIAN_POINT('Origin',(120.677721292346,-8.25,49.9710979935697));
#194854=CARTESIAN_POINT('',(120.186907789796,-8.25,49.8756930371204));
#194855=CARTESIAN_POINT('',(120.129664815927,-8.25,50.1701811386501));
#194856=CARTESIAN_POINT('',(120.186907789796,-8.25,49.8756930371204));
#194857=CARTESIAN_POINT('',(120.620478318476,-8.25,50.2655860950994));
#194858=CARTESIAN_POINT('',(120.677721292346,-8.25,49.9710979935697));
#194859=CARTESIAN_POINT('Origin',(120.186907789796,-8.25,49.8756930371204));
#194860=CARTESIAN_POINT('',(120.129664815927,-8.25,50.1701811386501));
#194861=CARTESIAN_POINT('',(120.186907789796,-8.25,49.8756930371204));
#194862=CARTESIAN_POINT('Origin',(120.972209393875,-7.75,50.0283409674392));
#194863=CARTESIAN_POINT('',(121.463022896425,-7.75,50.1237459238885));
#194864=CARTESIAN_POINT('',(121.405779922555,-7.75,50.4182340254182));
#194865=CARTESIAN_POINT('',(121.463022896425,-7.75,50.1237459238885));
#194866=CARTESIAN_POINT('',(120.914966420006,-7.75,50.3228290689689));
#194867=CARTESIAN_POINT('',(120.914966420006,-7.75,50.3228290689689));
#194868=CARTESIAN_POINT('',(120.972209393875,-7.75,50.0283409674392));
#194869=CARTESIAN_POINT('',(120.972209393875,-7.75,50.0283409674392));
#194870=CARTESIAN_POINT('',(120.972209393875,-7.75,50.0283409674392));
#194871=CARTESIAN_POINT('Origin',(121.463022896425,-7.75,50.1237459238885));
#194872=CARTESIAN_POINT('',(121.463022896425,-8.25,50.1237459238885));
#194873=CARTESIAN_POINT('',(121.405779922555,-8.25,50.4182340254182));
#194874=CARTESIAN_POINT('',(121.463022896425,-8.25,50.1237459238885));
#194875=CARTESIAN_POINT('',(121.405779922555,-7.75,50.4182340254182));
#194876=CARTESIAN_POINT('',(121.463022896425,-7.75,50.1237459238885));
#194877=CARTESIAN_POINT('Origin',(121.463022896425,-8.25,50.1237459238885));
#194878=CARTESIAN_POINT('',(120.972209393875,-8.25,50.0283409674392));
#194879=CARTESIAN_POINT('',(120.914966420006,-8.25,50.3228290689689));
#194880=CARTESIAN_POINT('',(120.972209393875,-8.25,50.0283409674392));
#194881=CARTESIAN_POINT('',(121.405779922555,-8.25,50.4182340254182));
#194882=CARTESIAN_POINT('',(121.463022896425,-8.25,50.1237459238885));
#194883=CARTESIAN_POINT('Origin',(120.972209393875,-8.25,50.0283409674392));
#194884=CARTESIAN_POINT('',(120.914966420006,-8.25,50.3228290689689));
#194885=CARTESIAN_POINT('',(120.972209393875,-8.25,50.0283409674392));
#194886=CARTESIAN_POINT('Origin',(121.757510997955,-7.75,50.180988897758));
#194887=CARTESIAN_POINT('',(122.248324500504,-7.75,50.2763938542073));
#194888=CARTESIAN_POINT('',(122.191081526635,-7.75,50.570881955737));
#194889=CARTESIAN_POINT('',(122.248324500504,-7.75,50.2763938542073));
#194890=CARTESIAN_POINT('',(121.700268024085,-7.75,50.4754769992877));
#194891=CARTESIAN_POINT('',(121.700268024085,-7.75,50.4754769992877));
#194892=CARTESIAN_POINT('',(121.757510997955,-7.75,50.180988897758));
#194893=CARTESIAN_POINT('',(121.757510997955,-7.75,50.180988897758));
#194894=CARTESIAN_POINT('',(121.757510997955,-7.75,50.180988897758));
#194895=CARTESIAN_POINT('Origin',(122.248324500504,-7.75,50.2763938542073));
#194896=CARTESIAN_POINT('',(122.248324500504,-8.25,50.2763938542073));
#194897=CARTESIAN_POINT('',(122.191081526635,-8.25,50.570881955737));
#194898=CARTESIAN_POINT('',(122.248324500504,-8.25,50.2763938542073));
#194899=CARTESIAN_POINT('',(122.191081526635,-7.75,50.570881955737));
#194900=CARTESIAN_POINT('',(122.248324500504,-7.75,50.2763938542073));
#194901=CARTESIAN_POINT('Origin',(122.248324500504,-8.25,50.2763938542073));
#194902=CARTESIAN_POINT('',(121.757510997955,-8.25,50.180988897758));
#194903=CARTESIAN_POINT('',(121.700268024085,-8.25,50.4754769992877));
#194904=CARTESIAN_POINT('',(121.757510997955,-8.25,50.180988897758));
#194905=CARTESIAN_POINT('',(122.191081526635,-8.25,50.570881955737));
#194906=CARTESIAN_POINT('',(122.248324500504,-8.25,50.2763938542073));
#194907=CARTESIAN_POINT('Origin',(121.757510997955,-8.25,50.180988897758));
#194908=CARTESIAN_POINT('',(121.700268024085,-8.25,50.4754769992877));
#194909=CARTESIAN_POINT('',(121.757510997955,-8.25,50.180988897758));
#194910=CARTESIAN_POINT('Origin',(124.898717414272,-4.55,50.7915806190332));
#194911=CARTESIAN_POINT('',(125.389530916821,-4.55,50.8869855754825));
#194912=CARTESIAN_POINT('',(125.332287942951,-4.55,51.1814736770122));
#194913=CARTESIAN_POINT('',(125.389530916821,-4.55,50.8869855754825));
#194914=CARTESIAN_POINT('',(124.841474440402,-4.55,51.0860687205629));
#194915=CARTESIAN_POINT('',(124.841474440402,-4.55,51.0860687205629));
#194916=CARTESIAN_POINT('',(124.898717414272,-4.55,50.7915806190332));
#194917=CARTESIAN_POINT('',(124.898717414272,-4.55,50.7915806190332));
#194918=CARTESIAN_POINT('',(124.898717414272,-4.55,50.7915806190332));
#194919=CARTESIAN_POINT('Origin',(125.389530916821,-4.55,50.8869855754825));
#194920=CARTESIAN_POINT('',(125.389530916821,-5.05,50.8869855754825));
#194921=CARTESIAN_POINT('',(125.332287942951,-5.05,51.1814736770122));
#194922=CARTESIAN_POINT('',(125.389530916821,-5.05,50.8869855754825));
#194923=CARTESIAN_POINT('',(125.332287942951,-4.55,51.1814736770122));
#194924=CARTESIAN_POINT('',(125.389530916821,-4.55,50.8869855754825));
#194925=CARTESIAN_POINT('Origin',(125.389530916821,-5.05,50.8869855754825));
#194926=CARTESIAN_POINT('',(124.898717414272,-5.05,50.7915806190332));
#194927=CARTESIAN_POINT('',(124.841474440402,-5.05,51.0860687205629));
#194928=CARTESIAN_POINT('',(124.898717414272,-5.05,50.7915806190332));
#194929=CARTESIAN_POINT('',(125.332287942951,-5.05,51.1814736770122));
#194930=CARTESIAN_POINT('',(125.389530916821,-5.05,50.8869855754825));
#194931=CARTESIAN_POINT('Origin',(124.898717414272,-5.05,50.7915806190332));
#194932=CARTESIAN_POINT('',(124.841474440402,-5.05,51.0860687205629));
#194933=CARTESIAN_POINT('',(124.898717414272,-5.05,50.7915806190332));
#194934=CARTESIAN_POINT('Origin',(124.898717414272,-3.75,50.7915806190332));
#194935=CARTESIAN_POINT('',(125.389530916821,-3.75,50.8869855754825));
#194936=CARTESIAN_POINT('',(125.332287942951,-3.75,51.1814736770122));
#194937=CARTESIAN_POINT('',(125.389530916821,-3.75,50.8869855754825));
#194938=CARTESIAN_POINT('',(124.841474440402,-3.75,51.0860687205629));
#194939=CARTESIAN_POINT('',(124.841474440402,-3.75,51.0860687205629));
#194940=CARTESIAN_POINT('',(124.898717414272,-3.75,50.7915806190332));
#194941=CARTESIAN_POINT('',(124.898717414272,-3.75,50.7915806190332));
#194942=CARTESIAN_POINT('',(124.898717414272,-3.75,50.7915806190332));
#194943=CARTESIAN_POINT('Origin',(125.389530916821,-3.75,50.8869855754825));
#194944=CARTESIAN_POINT('',(125.389530916821,-4.25,50.8869855754825));
#194945=CARTESIAN_POINT('',(125.332287942951,-4.25,51.1814736770122));
#194946=CARTESIAN_POINT('',(125.389530916821,-4.25,50.8869855754825));
#194947=CARTESIAN_POINT('',(125.332287942951,-3.75,51.1814736770122));
#194948=CARTESIAN_POINT('',(125.389530916821,-3.75,50.8869855754825));
#194949=CARTESIAN_POINT('Origin',(125.389530916821,-4.25,50.8869855754825));
#194950=CARTESIAN_POINT('',(124.898717414272,-4.25,50.7915806190332));
#194951=CARTESIAN_POINT('',(124.841474440402,-4.25,51.0860687205629));
#194952=CARTESIAN_POINT('',(124.898717414272,-4.25,50.7915806190332));
#194953=CARTESIAN_POINT('',(125.332287942951,-4.25,51.1814736770122));
#194954=CARTESIAN_POINT('',(125.389530916821,-4.25,50.8869855754825));
#194955=CARTESIAN_POINT('Origin',(124.898717414272,-4.25,50.7915806190332));
#194956=CARTESIAN_POINT('',(124.841474440402,-4.25,51.0860687205629));
#194957=CARTESIAN_POINT('',(124.898717414272,-4.25,50.7915806190332));
#194958=CARTESIAN_POINT('Origin',(124.898717414272,-2.95,50.7915806190332));
#194959=CARTESIAN_POINT('',(125.389530916821,-2.95,50.8869855754825));
#194960=CARTESIAN_POINT('',(125.332287942951,-2.95,51.1814736770122));
#194961=CARTESIAN_POINT('',(125.389530916821,-2.95,50.8869855754825));
#194962=CARTESIAN_POINT('',(124.841474440402,-2.95,51.0860687205629));
#194963=CARTESIAN_POINT('',(124.841474440402,-2.95,51.0860687205629));
#194964=CARTESIAN_POINT('',(124.898717414272,-2.95,50.7915806190332));
#194965=CARTESIAN_POINT('',(124.898717414272,-2.95,50.7915806190332));
#194966=CARTESIAN_POINT('',(124.898717414272,-2.95,50.7915806190332));
#194967=CARTESIAN_POINT('Origin',(125.389530916821,-2.95,50.8869855754825));
#194968=CARTESIAN_POINT('',(125.389530916821,-3.45,50.8869855754825));
#194969=CARTESIAN_POINT('',(125.332287942951,-3.45,51.1814736770122));
#194970=CARTESIAN_POINT('',(125.389530916821,-3.45,50.8869855754825));
#194971=CARTESIAN_POINT('',(125.332287942951,-2.95,51.1814736770122));
#194972=CARTESIAN_POINT('',(125.389530916821,-2.95,50.8869855754825));
#194973=CARTESIAN_POINT('Origin',(125.389530916821,-3.45,50.8869855754825));
#194974=CARTESIAN_POINT('',(124.898717414272,-3.45,50.7915806190332));
#194975=CARTESIAN_POINT('',(124.841474440402,-3.45,51.0860687205629));
#194976=CARTESIAN_POINT('',(124.898717414272,-3.45,50.7915806190332));
#194977=CARTESIAN_POINT('',(125.332287942951,-3.45,51.1814736770122));
#194978=CARTESIAN_POINT('',(125.389530916821,-3.45,50.8869855754825));
#194979=CARTESIAN_POINT('Origin',(124.898717414272,-3.45,50.7915806190332));
#194980=CARTESIAN_POINT('',(124.841474440402,-3.45,51.0860687205629));
#194981=CARTESIAN_POINT('',(124.898717414272,-3.45,50.7915806190332));
#194982=CARTESIAN_POINT('Origin',(124.898717414272,-2.15,50.7915806190332));
#194983=CARTESIAN_POINT('',(125.389530916821,-2.15,50.8869855754825));
#194984=CARTESIAN_POINT('',(125.332287942951,-2.15,51.1814736770122));
#194985=CARTESIAN_POINT('',(125.389530916821,-2.15,50.8869855754825));
#194986=CARTESIAN_POINT('',(124.841474440402,-2.15,51.0860687205629));
#194987=CARTESIAN_POINT('',(124.841474440402,-2.15,51.0860687205629));
#194988=CARTESIAN_POINT('',(124.898717414272,-2.15,50.7915806190332));
#194989=CARTESIAN_POINT('',(124.898717414272,-2.15,50.7915806190332));
#194990=CARTESIAN_POINT('',(124.898717414272,-2.15,50.7915806190332));
#194991=CARTESIAN_POINT('Origin',(125.389530916821,-2.15,50.8869855754825));
#194992=CARTESIAN_POINT('',(125.389530916821,-2.65,50.8869855754825));
#194993=CARTESIAN_POINT('',(125.332287942951,-2.65,51.1814736770122));
#194994=CARTESIAN_POINT('',(125.389530916821,-2.65,50.8869855754825));
#194995=CARTESIAN_POINT('',(125.332287942951,-2.15,51.1814736770122));
#194996=CARTESIAN_POINT('',(125.389530916821,-2.15,50.8869855754825));
#194997=CARTESIAN_POINT('Origin',(125.389530916821,-2.65,50.8869855754825));
#194998=CARTESIAN_POINT('',(124.898717414272,-2.65,50.7915806190332));
#194999=CARTESIAN_POINT('',(124.841474440402,-2.65,51.0860687205629));
#195000=CARTESIAN_POINT('',(124.898717414272,-2.65,50.7915806190332));
#195001=CARTESIAN_POINT('',(125.332287942951,-2.65,51.1814736770122));
#195002=CARTESIAN_POINT('',(125.389530916821,-2.65,50.8869855754825));
#195003=CARTESIAN_POINT('Origin',(124.898717414272,-2.65,50.7915806190332));
#195004=CARTESIAN_POINT('',(124.841474440402,-2.65,51.0860687205629));
#195005=CARTESIAN_POINT('',(124.898717414272,-2.65,50.7915806190332));
#195006=CARTESIAN_POINT('Origin',(124.898717414272,-1.35,50.7915806190332));
#195007=CARTESIAN_POINT('',(125.389530916821,-1.35,50.8869855754825));
#195008=CARTESIAN_POINT('',(125.332287942951,-1.35,51.1814736770122));
#195009=CARTESIAN_POINT('',(125.389530916821,-1.35,50.8869855754825));
#195010=CARTESIAN_POINT('',(124.841474440402,-1.35,51.0860687205629));
#195011=CARTESIAN_POINT('',(124.841474440402,-1.35,51.0860687205629));
#195012=CARTESIAN_POINT('',(124.898717414272,-1.35,50.7915806190332));
#195013=CARTESIAN_POINT('',(124.898717414272,-1.35,50.7915806190332));
#195014=CARTESIAN_POINT('',(124.898717414272,-1.35,50.7915806190332));
#195015=CARTESIAN_POINT('Origin',(125.389530916821,-1.35,50.8869855754825));
#195016=CARTESIAN_POINT('',(125.389530916821,-1.85,50.8869855754825));
#195017=CARTESIAN_POINT('',(125.332287942951,-1.85,51.1814736770122));
#195018=CARTESIAN_POINT('',(125.389530916821,-1.85,50.8869855754825));
#195019=CARTESIAN_POINT('',(125.332287942951,-1.35,51.1814736770122));
#195020=CARTESIAN_POINT('',(125.389530916821,-1.35,50.8869855754825));
#195021=CARTESIAN_POINT('Origin',(125.389530916821,-1.85,50.8869855754825));
#195022=CARTESIAN_POINT('',(124.898717414272,-1.85,50.7915806190332));
#195023=CARTESIAN_POINT('',(124.841474440402,-1.85,51.0860687205629));
#195024=CARTESIAN_POINT('',(124.898717414272,-1.85,50.7915806190332));
#195025=CARTESIAN_POINT('',(125.332287942951,-1.85,51.1814736770122));
#195026=CARTESIAN_POINT('',(125.389530916821,-1.85,50.8869855754825));
#195027=CARTESIAN_POINT('Origin',(124.898717414272,-1.85,50.7915806190332));
#195028=CARTESIAN_POINT('',(124.841474440402,-1.85,51.0860687205629));
#195029=CARTESIAN_POINT('',(124.898717414272,-1.85,50.7915806190332));
#195030=CARTESIAN_POINT('Origin',(124.898717414272,-0.549999999999986,50.7915806190332));
#195031=CARTESIAN_POINT('',(125.389530916821,-0.549999999999986,50.8869855754825));
#195032=CARTESIAN_POINT('',(125.332287942951,-0.549999999999986,51.1814736770122));
#195033=CARTESIAN_POINT('',(125.389530916821,-0.549999999999986,50.8869855754825));
#195034=CARTESIAN_POINT('',(124.841474440402,-0.549999999999986,51.0860687205629));
#195035=CARTESIAN_POINT('',(124.841474440402,-0.549999999999986,51.0860687205629));
#195036=CARTESIAN_POINT('',(124.898717414272,-0.549999999999986,50.7915806190332));
#195037=CARTESIAN_POINT('',(124.898717414272,-0.549999999999986,50.7915806190332));
#195038=CARTESIAN_POINT('',(124.898717414272,-0.549999999999986,50.7915806190332));
#195039=CARTESIAN_POINT('Origin',(125.389530916821,-0.549999999999986,50.8869855754825));
#195040=CARTESIAN_POINT('',(125.389530916821,-1.05,50.8869855754825));
#195041=CARTESIAN_POINT('',(125.332287942951,-1.05,51.1814736770122));
#195042=CARTESIAN_POINT('',(125.389530916821,-1.05,50.8869855754825));
#195043=CARTESIAN_POINT('',(125.332287942951,-0.549999999999986,51.1814736770122));
#195044=CARTESIAN_POINT('',(125.389530916821,-0.549999999999986,50.8869855754825));
#195045=CARTESIAN_POINT('Origin',(125.389530916821,-1.05,50.8869855754825));
#195046=CARTESIAN_POINT('',(124.898717414272,-1.05,50.7915806190332));
#195047=CARTESIAN_POINT('',(124.841474440402,-1.05,51.0860687205629));
#195048=CARTESIAN_POINT('',(124.898717414272,-1.05,50.7915806190332));
#195049=CARTESIAN_POINT('',(125.332287942951,-1.05,51.1814736770122));
#195050=CARTESIAN_POINT('',(125.389530916821,-1.05,50.8869855754825));
#195051=CARTESIAN_POINT('Origin',(124.898717414272,-1.05,50.7915806190332));
#195052=CARTESIAN_POINT('',(124.841474440402,-1.05,51.0860687205629));
#195053=CARTESIAN_POINT('',(124.898717414272,-1.05,50.7915806190332));
#195054=CARTESIAN_POINT('Origin',(124.898717414272,0.250000000000015,50.7915806190332));
#195055=CARTESIAN_POINT('',(125.389530916821,0.250000000000015,50.8869855754825));
#195056=CARTESIAN_POINT('',(125.332287942951,0.250000000000015,51.1814736770122));
#195057=CARTESIAN_POINT('',(125.389530916821,0.250000000000015,50.8869855754825));
#195058=CARTESIAN_POINT('',(124.841474440402,0.250000000000015,51.0860687205629));
#195059=CARTESIAN_POINT('',(124.841474440402,0.250000000000015,51.0860687205629));
#195060=CARTESIAN_POINT('',(124.898717414272,0.250000000000015,50.7915806190332));
#195061=CARTESIAN_POINT('',(124.898717414272,0.250000000000015,50.7915806190332));
#195062=CARTESIAN_POINT('',(124.898717414272,0.250000000000015,50.7915806190332));
#195063=CARTESIAN_POINT('Origin',(125.389530916821,0.250000000000015,50.8869855754825));
#195064=CARTESIAN_POINT('',(125.389530916821,-0.249999999999985,50.8869855754825));
#195065=CARTESIAN_POINT('',(125.332287942951,-0.249999999999985,51.1814736770122));
#195066=CARTESIAN_POINT('',(125.389530916821,-0.249999999999985,50.8869855754825));
#195067=CARTESIAN_POINT('',(125.332287942951,0.250000000000015,51.1814736770122));
#195068=CARTESIAN_POINT('',(125.389530916821,0.250000000000015,50.8869855754825));
#195069=CARTESIAN_POINT('Origin',(125.389530916821,-0.249999999999985,50.8869855754825));
#195070=CARTESIAN_POINT('',(124.898717414272,-0.249999999999985,50.7915806190332));
#195071=CARTESIAN_POINT('',(124.841474440402,-0.249999999999985,51.0860687205629));
#195072=CARTESIAN_POINT('',(124.898717414272,-0.249999999999985,50.7915806190332));
#195073=CARTESIAN_POINT('',(125.332287942951,-0.249999999999985,51.1814736770122));
#195074=CARTESIAN_POINT('',(125.389530916821,-0.249999999999985,50.8869855754825));
#195075=CARTESIAN_POINT('Origin',(124.898717414272,-0.249999999999985,50.7915806190332));
#195076=CARTESIAN_POINT('',(124.841474440402,-0.249999999999985,51.0860687205629));
#195077=CARTESIAN_POINT('',(124.898717414272,-0.249999999999985,50.7915806190332));
#195078=CARTESIAN_POINT('Origin',(124.898717414272,1.05,50.7915806190332));
#195079=CARTESIAN_POINT('',(125.389530916821,1.05,50.8869855754825));
#195080=CARTESIAN_POINT('',(125.332287942951,1.05,51.1814736770122));
#195081=CARTESIAN_POINT('',(125.389530916821,1.05,50.8869855754825));
#195082=CARTESIAN_POINT('',(124.841474440402,1.05,51.0860687205629));
#195083=CARTESIAN_POINT('',(124.841474440402,1.05,51.0860687205629));
#195084=CARTESIAN_POINT('',(124.898717414272,1.05,50.7915806190332));
#195085=CARTESIAN_POINT('',(124.898717414272,1.05,50.7915806190332));
#195086=CARTESIAN_POINT('',(124.898717414272,1.05,50.7915806190332));
#195087=CARTESIAN_POINT('Origin',(125.389530916821,1.05,50.8869855754825));
#195088=CARTESIAN_POINT('',(125.389530916821,0.550000000000015,50.8869855754825));
#195089=CARTESIAN_POINT('',(125.332287942951,0.550000000000015,51.1814736770122));
#195090=CARTESIAN_POINT('',(125.389530916821,0.550000000000015,50.8869855754825));
#195091=CARTESIAN_POINT('',(125.332287942951,1.05,51.1814736770122));
#195092=CARTESIAN_POINT('',(125.389530916821,1.05,50.8869855754825));
#195093=CARTESIAN_POINT('Origin',(125.389530916821,0.550000000000015,50.8869855754825));
#195094=CARTESIAN_POINT('',(124.898717414272,0.550000000000015,50.7915806190332));
#195095=CARTESIAN_POINT('',(124.841474440402,0.550000000000015,51.0860687205629));
#195096=CARTESIAN_POINT('',(124.898717414272,0.550000000000015,50.7915806190332));
#195097=CARTESIAN_POINT('',(125.332287942951,0.550000000000015,51.1814736770122));
#195098=CARTESIAN_POINT('',(125.389530916821,0.550000000000015,50.8869855754825));
#195099=CARTESIAN_POINT('Origin',(124.898717414272,0.550000000000015,50.7915806190332));
#195100=CARTESIAN_POINT('',(124.841474440402,0.550000000000015,51.0860687205629));
#195101=CARTESIAN_POINT('',(124.898717414272,0.550000000000015,50.7915806190332));
#195102=CARTESIAN_POINT('Origin',(124.898717414272,1.85,50.7915806190332));
#195103=CARTESIAN_POINT('',(125.389530916821,1.85,50.8869855754825));
#195104=CARTESIAN_POINT('',(125.332287942951,1.85,51.1814736770122));
#195105=CARTESIAN_POINT('',(125.389530916821,1.85,50.8869855754825));
#195106=CARTESIAN_POINT('',(124.841474440402,1.85,51.0860687205629));
#195107=CARTESIAN_POINT('',(124.841474440402,1.85,51.0860687205629));
#195108=CARTESIAN_POINT('',(124.898717414272,1.85,50.7915806190332));
#195109=CARTESIAN_POINT('',(124.898717414272,1.85,50.7915806190332));
#195110=CARTESIAN_POINT('',(124.898717414272,1.85,50.7915806190332));
#195111=CARTESIAN_POINT('Origin',(125.389530916821,1.85,50.8869855754825));
#195112=CARTESIAN_POINT('',(125.389530916821,1.35,50.8869855754825));
#195113=CARTESIAN_POINT('',(125.332287942951,1.35,51.1814736770122));
#195114=CARTESIAN_POINT('',(125.389530916821,1.35,50.8869855754825));
#195115=CARTESIAN_POINT('',(125.332287942951,1.85,51.1814736770122));
#195116=CARTESIAN_POINT('',(125.389530916821,1.85,50.8869855754825));
#195117=CARTESIAN_POINT('Origin',(125.389530916821,1.35,50.8869855754825));
#195118=CARTESIAN_POINT('',(124.898717414272,1.35,50.7915806190332));
#195119=CARTESIAN_POINT('',(124.841474440402,1.35,51.0860687205629));
#195120=CARTESIAN_POINT('',(124.898717414272,1.35,50.7915806190332));
#195121=CARTESIAN_POINT('',(125.332287942951,1.35,51.1814736770122));
#195122=CARTESIAN_POINT('',(125.389530916821,1.35,50.8869855754825));
#195123=CARTESIAN_POINT('Origin',(124.898717414272,1.35,50.7915806190332));
#195124=CARTESIAN_POINT('',(124.841474440402,1.35,51.0860687205629));
#195125=CARTESIAN_POINT('',(124.898717414272,1.35,50.7915806190332));
#195126=CARTESIAN_POINT('Origin',(124.898717414272,2.65,50.7915806190332));
#195127=CARTESIAN_POINT('',(125.389530916821,2.65,50.8869855754825));
#195128=CARTESIAN_POINT('',(125.332287942951,2.65,51.1814736770122));
#195129=CARTESIAN_POINT('',(125.389530916821,2.65,50.8869855754825));
#195130=CARTESIAN_POINT('',(124.841474440402,2.65,51.0860687205629));
#195131=CARTESIAN_POINT('',(124.841474440402,2.65,51.0860687205629));
#195132=CARTESIAN_POINT('',(124.898717414272,2.65,50.7915806190332));
#195133=CARTESIAN_POINT('',(124.898717414272,2.65,50.7915806190332));
#195134=CARTESIAN_POINT('',(124.898717414272,2.65,50.7915806190332));
#195135=CARTESIAN_POINT('Origin',(125.389530916821,2.65,50.8869855754825));
#195136=CARTESIAN_POINT('',(125.389530916821,2.15,50.8869855754825));
#195137=CARTESIAN_POINT('',(125.332287942951,2.15,51.1814736770122));
#195138=CARTESIAN_POINT('',(125.389530916821,2.15,50.8869855754825));
#195139=CARTESIAN_POINT('',(125.332287942951,2.65,51.1814736770122));
#195140=CARTESIAN_POINT('',(125.389530916821,2.65,50.8869855754825));
#195141=CARTESIAN_POINT('Origin',(125.389530916821,2.15,50.8869855754825));
#195142=CARTESIAN_POINT('',(124.898717414272,2.15,50.7915806190332));
#195143=CARTESIAN_POINT('',(124.841474440402,2.15,51.0860687205629));
#195144=CARTESIAN_POINT('',(124.898717414272,2.15,50.7915806190332));
#195145=CARTESIAN_POINT('',(125.332287942951,2.15,51.1814736770122));
#195146=CARTESIAN_POINT('',(125.389530916821,2.15,50.8869855754825));
#195147=CARTESIAN_POINT('Origin',(124.898717414272,2.15,50.7915806190332));
#195148=CARTESIAN_POINT('',(124.841474440402,2.15,51.0860687205629));
#195149=CARTESIAN_POINT('',(124.898717414272,2.15,50.7915806190332));
#195150=CARTESIAN_POINT('Origin',(124.898717414272,3.45,50.7915806190332));
#195151=CARTESIAN_POINT('',(125.389530916821,3.45,50.8869855754825));
#195152=CARTESIAN_POINT('',(125.332287942951,3.45,51.1814736770122));
#195153=CARTESIAN_POINT('',(125.389530916821,3.45,50.8869855754825));
#195154=CARTESIAN_POINT('',(124.841474440402,3.45,51.0860687205629));
#195155=CARTESIAN_POINT('',(124.841474440402,3.45,51.0860687205629));
#195156=CARTESIAN_POINT('',(124.898717414272,3.45,50.7915806190332));
#195157=CARTESIAN_POINT('',(124.898717414272,3.45,50.7915806190332));
#195158=CARTESIAN_POINT('',(124.898717414272,3.45,50.7915806190332));
#195159=CARTESIAN_POINT('Origin',(125.389530916821,3.45,50.8869855754825));
#195160=CARTESIAN_POINT('',(125.389530916821,2.95,50.8869855754825));
#195161=CARTESIAN_POINT('',(125.332287942951,2.95,51.1814736770122));
#195162=CARTESIAN_POINT('',(125.389530916821,2.95,50.8869855754825));
#195163=CARTESIAN_POINT('',(125.332287942951,3.45,51.1814736770122));
#195164=CARTESIAN_POINT('',(125.389530916821,3.45,50.8869855754825));
#195165=CARTESIAN_POINT('Origin',(125.389530916821,2.95,50.8869855754825));
#195166=CARTESIAN_POINT('',(124.898717414272,2.95,50.7915806190332));
#195167=CARTESIAN_POINT('',(124.841474440402,2.95,51.0860687205629));
#195168=CARTESIAN_POINT('',(124.898717414272,2.95,50.7915806190332));
#195169=CARTESIAN_POINT('',(125.332287942951,2.95,51.1814736770122));
#195170=CARTESIAN_POINT('',(125.389530916821,2.95,50.8869855754825));
#195171=CARTESIAN_POINT('Origin',(124.898717414272,2.95,50.7915806190332));
#195172=CARTESIAN_POINT('',(124.841474440402,2.95,51.0860687205629));
#195173=CARTESIAN_POINT('',(124.898717414272,2.95,50.7915806190332));
#195174=CARTESIAN_POINT('Origin',(124.898717414272,4.25,50.7915806190332));
#195175=CARTESIAN_POINT('',(125.389530916821,4.25,50.8869855754825));
#195176=CARTESIAN_POINT('',(125.332287942951,4.25,51.1814736770122));
#195177=CARTESIAN_POINT('',(125.389530916821,4.25,50.8869855754825));
#195178=CARTESIAN_POINT('',(124.841474440402,4.25,51.0860687205629));
#195179=CARTESIAN_POINT('',(124.841474440402,4.25,51.0860687205629));
#195180=CARTESIAN_POINT('',(124.898717414272,4.25,50.7915806190332));
#195181=CARTESIAN_POINT('',(124.898717414272,4.25,50.7915806190332));
#195182=CARTESIAN_POINT('',(124.898717414272,4.25,50.7915806190332));
#195183=CARTESIAN_POINT('Origin',(125.389530916821,4.25,50.8869855754825));
#195184=CARTESIAN_POINT('',(125.389530916821,3.75,50.8869855754825));
#195185=CARTESIAN_POINT('',(125.332287942951,3.75,51.1814736770122));
#195186=CARTESIAN_POINT('',(125.389530916821,3.75,50.8869855754825));
#195187=CARTESIAN_POINT('',(125.332287942951,4.25,51.1814736770122));
#195188=CARTESIAN_POINT('',(125.389530916821,4.25,50.8869855754825));
#195189=CARTESIAN_POINT('Origin',(125.389530916821,3.75,50.8869855754825));
#195190=CARTESIAN_POINT('',(124.898717414272,3.75,50.7915806190332));
#195191=CARTESIAN_POINT('',(124.841474440402,3.75,51.0860687205629));
#195192=CARTESIAN_POINT('',(124.898717414272,3.75,50.7915806190332));
#195193=CARTESIAN_POINT('',(125.332287942951,3.75,51.1814736770122));
#195194=CARTESIAN_POINT('',(125.389530916821,3.75,50.8869855754825));
#195195=CARTESIAN_POINT('Origin',(124.898717414272,3.75,50.7915806190332));
#195196=CARTESIAN_POINT('',(124.841474440402,3.75,51.0860687205629));
#195197=CARTESIAN_POINT('',(124.898717414272,3.75,50.7915806190332));
#195198=CARTESIAN_POINT('Origin',(124.898717414272,5.05,50.7915806190332));
#195199=CARTESIAN_POINT('',(125.389530916821,5.05,50.8869855754825));
#195200=CARTESIAN_POINT('',(125.332287942951,5.05,51.1814736770122));
#195201=CARTESIAN_POINT('',(125.389530916821,5.05,50.8869855754825));
#195202=CARTESIAN_POINT('',(124.841474440402,5.05,51.0860687205629));
#195203=CARTESIAN_POINT('',(124.841474440402,5.05,51.0860687205629));
#195204=CARTESIAN_POINT('',(124.898717414272,5.05,50.7915806190332));
#195205=CARTESIAN_POINT('',(124.898717414272,5.05,50.7915806190332));
#195206=CARTESIAN_POINT('',(124.898717414272,5.05,50.7915806190332));
#195207=CARTESIAN_POINT('Origin',(125.389530916821,5.05,50.8869855754825));
#195208=CARTESIAN_POINT('',(125.389530916821,4.55,50.8869855754825));
#195209=CARTESIAN_POINT('',(125.332287942951,4.55,51.1814736770122));
#195210=CARTESIAN_POINT('',(125.389530916821,4.55,50.8869855754825));
#195211=CARTESIAN_POINT('',(125.332287942951,5.05,51.1814736770122));
#195212=CARTESIAN_POINT('',(125.389530916821,5.05,50.8869855754825));
#195213=CARTESIAN_POINT('Origin',(125.389530916821,4.55,50.8869855754825));
#195214=CARTESIAN_POINT('',(124.898717414272,4.55,50.7915806190332));
#195215=CARTESIAN_POINT('',(124.841474440402,4.55,51.0860687205629));
#195216=CARTESIAN_POINT('',(124.898717414272,4.55,50.7915806190332));
#195217=CARTESIAN_POINT('',(125.332287942951,4.55,51.1814736770122));
#195218=CARTESIAN_POINT('',(125.389530916821,4.55,50.8869855754825));
#195219=CARTESIAN_POINT('Origin',(124.898717414272,4.55,50.7915806190332));
#195220=CARTESIAN_POINT('',(124.841474440402,4.55,51.0860687205629));
#195221=CARTESIAN_POINT('',(124.898717414272,4.55,50.7915806190332));
#195222=CARTESIAN_POINT('Origin',(121.757510997955,8.25,50.180988897758));
#195223=CARTESIAN_POINT('',(122.248324500504,8.25,50.2763938542073));
#195224=CARTESIAN_POINT('',(122.191081526635,8.25,50.570881955737));
#195225=CARTESIAN_POINT('',(122.248324500504,8.25,50.2763938542073));
#195226=CARTESIAN_POINT('',(121.700268024085,8.25,50.4754769992877));
#195227=CARTESIAN_POINT('',(121.700268024085,8.25,50.4754769992877));
#195228=CARTESIAN_POINT('',(121.757510997955,8.25,50.180988897758));
#195229=CARTESIAN_POINT('',(121.757510997955,8.25,50.180988897758));
#195230=CARTESIAN_POINT('',(121.757510997955,8.25,50.180988897758));
#195231=CARTESIAN_POINT('Origin',(122.248324500504,8.25,50.2763938542073));
#195232=CARTESIAN_POINT('',(122.248324500504,7.75,50.2763938542073));
#195233=CARTESIAN_POINT('',(122.191081526635,7.75,50.570881955737));
#195234=CARTESIAN_POINT('',(122.248324500504,7.75,50.2763938542073));
#195235=CARTESIAN_POINT('',(122.191081526635,8.25,50.570881955737));
#195236=CARTESIAN_POINT('',(122.248324500504,8.25,50.2763938542073));
#195237=CARTESIAN_POINT('Origin',(122.248324500504,7.75,50.2763938542073));
#195238=CARTESIAN_POINT('',(121.757510997955,7.75,50.180988897758));
#195239=CARTESIAN_POINT('',(121.700268024085,7.75,50.4754769992877));
#195240=CARTESIAN_POINT('',(121.757510997955,7.75,50.180988897758));
#195241=CARTESIAN_POINT('',(122.191081526635,7.75,50.570881955737));
#195242=CARTESIAN_POINT('',(122.248324500504,7.75,50.2763938542073));
#195243=CARTESIAN_POINT('Origin',(121.757510997955,7.75,50.180988897758));
#195244=CARTESIAN_POINT('',(121.700268024085,7.75,50.4754769992877));
#195245=CARTESIAN_POINT('',(121.757510997955,7.75,50.180988897758));
#195246=CARTESIAN_POINT('Origin',(120.972209393875,8.25,50.0283409674392));
#195247=CARTESIAN_POINT('',(121.463022896425,8.25,50.1237459238885));
#195248=CARTESIAN_POINT('',(121.405779922555,8.25,50.4182340254182));
#195249=CARTESIAN_POINT('',(121.463022896425,8.25,50.1237459238885));
#195250=CARTESIAN_POINT('',(120.914966420006,8.25,50.3228290689689));
#195251=CARTESIAN_POINT('',(120.914966420006,8.25,50.3228290689689));
#195252=CARTESIAN_POINT('',(120.972209393875,8.25,50.0283409674392));
#195253=CARTESIAN_POINT('',(120.972209393875,8.25,50.0283409674392));
#195254=CARTESIAN_POINT('',(120.972209393875,8.25,50.0283409674392));
#195255=CARTESIAN_POINT('Origin',(121.463022896425,8.25,50.1237459238885));
#195256=CARTESIAN_POINT('',(121.463022896425,7.75,50.1237459238885));
#195257=CARTESIAN_POINT('',(121.405779922555,7.75,50.4182340254182));
#195258=CARTESIAN_POINT('',(121.463022896425,7.75,50.1237459238885));
#195259=CARTESIAN_POINT('',(121.405779922555,8.25,50.4182340254182));
#195260=CARTESIAN_POINT('',(121.463022896425,8.25,50.1237459238885));
#195261=CARTESIAN_POINT('Origin',(121.463022896425,7.75,50.1237459238885));
#195262=CARTESIAN_POINT('',(120.972209393875,7.75,50.0283409674392));
#195263=CARTESIAN_POINT('',(120.914966420006,7.75,50.3228290689689));
#195264=CARTESIAN_POINT('',(120.972209393875,7.75,50.0283409674392));
#195265=CARTESIAN_POINT('',(121.405779922555,7.75,50.4182340254182));
#195266=CARTESIAN_POINT('',(121.463022896425,7.75,50.1237459238885));
#195267=CARTESIAN_POINT('Origin',(120.972209393875,7.75,50.0283409674392));
#195268=CARTESIAN_POINT('',(120.914966420006,7.75,50.3228290689689));
#195269=CARTESIAN_POINT('',(120.972209393875,7.75,50.0283409674392));
#195270=CARTESIAN_POINT('Origin',(120.186907789796,8.25,49.8756930371204));
#195271=CARTESIAN_POINT('',(120.677721292346,8.25,49.9710979935697));
#195272=CARTESIAN_POINT('',(120.620478318476,8.25,50.2655860950994));
#195273=CARTESIAN_POINT('',(120.677721292346,8.25,49.9710979935697));
#195274=CARTESIAN_POINT('',(120.129664815927,8.25,50.1701811386501));
#195275=CARTESIAN_POINT('',(120.129664815927,8.25,50.1701811386501));
#195276=CARTESIAN_POINT('',(120.186907789796,8.25,49.8756930371204));
#195277=CARTESIAN_POINT('',(120.186907789796,8.25,49.8756930371204));
#195278=CARTESIAN_POINT('',(120.186907789796,8.25,49.8756930371204));
#195279=CARTESIAN_POINT('Origin',(120.677721292346,8.25,49.9710979935697));
#195280=CARTESIAN_POINT('',(120.677721292346,7.75,49.9710979935697));
#195281=CARTESIAN_POINT('',(120.620478318476,7.75,50.2655860950994));
#195282=CARTESIAN_POINT('',(120.677721292346,7.75,49.9710979935697));
#195283=CARTESIAN_POINT('',(120.620478318476,8.25,50.2655860950994));
#195284=CARTESIAN_POINT('',(120.677721292346,8.25,49.9710979935697));
#195285=CARTESIAN_POINT('Origin',(120.677721292346,7.75,49.9710979935697));
#195286=CARTESIAN_POINT('',(120.186907789796,7.75,49.8756930371204));
#195287=CARTESIAN_POINT('',(120.129664815927,7.75,50.1701811386501));
#195288=CARTESIAN_POINT('',(120.186907789796,7.75,49.8756930371204));
#195289=CARTESIAN_POINT('',(120.620478318476,7.75,50.2655860950994));
#195290=CARTESIAN_POINT('',(120.677721292346,7.75,49.9710979935697));
#195291=CARTESIAN_POINT('Origin',(120.186907789796,7.75,49.8756930371204));
#195292=CARTESIAN_POINT('',(120.129664815927,7.75,50.1701811386501));
#195293=CARTESIAN_POINT('',(120.186907789796,7.75,49.8756930371204));
#195294=CARTESIAN_POINT('Origin',(119.401606185717,8.25,49.7230451068016));
#195295=CARTESIAN_POINT('',(119.892419688267,8.25,49.8184500632509));
#195296=CARTESIAN_POINT('',(119.835176714397,8.25,50.1129381647806));
#195297=CARTESIAN_POINT('',(119.892419688267,8.25,49.8184500632509));
#195298=CARTESIAN_POINT('',(119.344363211847,8.25,50.0175332083313));
#195299=CARTESIAN_POINT('',(119.344363211847,8.25,50.0175332083313));
#195300=CARTESIAN_POINT('',(119.401606185717,8.25,49.7230451068016));
#195301=CARTESIAN_POINT('',(119.401606185717,8.25,49.7230451068016));
#195302=CARTESIAN_POINT('',(119.401606185717,8.25,49.7230451068016));
#195303=CARTESIAN_POINT('Origin',(119.892419688267,8.25,49.8184500632509));
#195304=CARTESIAN_POINT('',(119.892419688267,7.75,49.8184500632509));
#195305=CARTESIAN_POINT('',(119.835176714397,7.75,50.1129381647806));
#195306=CARTESIAN_POINT('',(119.892419688267,7.75,49.8184500632509));
#195307=CARTESIAN_POINT('',(119.835176714397,8.25,50.1129381647806));
#195308=CARTESIAN_POINT('',(119.892419688267,8.25,49.8184500632509));
#195309=CARTESIAN_POINT('Origin',(119.892419688267,7.75,49.8184500632509));
#195310=CARTESIAN_POINT('',(119.401606185717,7.75,49.7230451068016));
#195311=CARTESIAN_POINT('',(119.344363211847,7.75,50.0175332083313));
#195312=CARTESIAN_POINT('',(119.401606185717,7.75,49.7230451068016));
#195313=CARTESIAN_POINT('',(119.835176714397,7.75,50.1129381647806));
#195314=CARTESIAN_POINT('',(119.892419688267,7.75,49.8184500632509));
#195315=CARTESIAN_POINT('Origin',(119.401606185717,7.75,49.7230451068016));
#195316=CARTESIAN_POINT('',(119.344363211847,7.75,50.0175332083313));
#195317=CARTESIAN_POINT('',(119.401606185717,7.75,49.7230451068016));
#195318=CARTESIAN_POINT('Origin',(118.616304581638,8.25,49.5703971764828));
#195319=CARTESIAN_POINT('',(119.107118084187,8.25,49.6658021329321));
#195320=CARTESIAN_POINT('',(119.049875110318,8.25,49.9602902344618));
#195321=CARTESIAN_POINT('',(119.107118084187,8.25,49.6658021329321));
#195322=CARTESIAN_POINT('',(118.559061607768,8.25,49.8648852780125));
#195323=CARTESIAN_POINT('',(118.559061607768,8.25,49.8648852780125));
#195324=CARTESIAN_POINT('',(118.616304581638,8.25,49.5703971764828));
#195325=CARTESIAN_POINT('',(118.616304581638,8.25,49.5703971764828));
#195326=CARTESIAN_POINT('',(118.616304581638,8.25,49.5703971764828));
#195327=CARTESIAN_POINT('Origin',(119.107118084187,8.25,49.6658021329321));
#195328=CARTESIAN_POINT('',(119.107118084187,7.75,49.6658021329321));
#195329=CARTESIAN_POINT('',(119.049875110318,7.75,49.9602902344618));
#195330=CARTESIAN_POINT('',(119.107118084187,7.75,49.6658021329321));
#195331=CARTESIAN_POINT('',(119.049875110318,8.25,49.9602902344618));
#195332=CARTESIAN_POINT('',(119.107118084187,8.25,49.6658021329321));
#195333=CARTESIAN_POINT('Origin',(119.107118084187,7.75,49.6658021329321));
#195334=CARTESIAN_POINT('',(118.616304581638,7.75,49.5703971764828));
#195335=CARTESIAN_POINT('',(118.559061607768,7.75,49.8648852780125));
#195336=CARTESIAN_POINT('',(118.616304581638,7.75,49.5703971764828));
#195337=CARTESIAN_POINT('',(119.049875110318,7.75,49.9602902344618));
#195338=CARTESIAN_POINT('',(119.107118084187,7.75,49.6658021329321));
#195339=CARTESIAN_POINT('Origin',(118.616304581638,7.75,49.5703971764828));
#195340=CARTESIAN_POINT('',(118.559061607768,7.75,49.8648852780125));
#195341=CARTESIAN_POINT('',(118.616304581638,7.75,49.5703971764828));
#195342=CARTESIAN_POINT('Origin',(117.831002977559,8.25,49.417749246164));
#195343=CARTESIAN_POINT('',(118.321816480108,8.25,49.5131542026133));
#195344=CARTESIAN_POINT('',(118.264573506239,8.25,49.807642304143));
#195345=CARTESIAN_POINT('',(118.321816480108,8.25,49.5131542026133));
#195346=CARTESIAN_POINT('',(117.773760003689,8.25,49.7122373476937));
#195347=CARTESIAN_POINT('',(117.773760003689,8.25,49.7122373476937));
#195348=CARTESIAN_POINT('',(117.831002977559,8.25,49.417749246164));
#195349=CARTESIAN_POINT('',(117.831002977559,8.25,49.417749246164));
#195350=CARTESIAN_POINT('',(117.831002977559,8.25,49.417749246164));
#195351=CARTESIAN_POINT('Origin',(118.321816480108,8.25,49.5131542026133));
#195352=CARTESIAN_POINT('',(118.321816480108,7.75,49.5131542026133));
#195353=CARTESIAN_POINT('',(118.264573506239,7.75,49.807642304143));
#195354=CARTESIAN_POINT('',(118.321816480108,7.75,49.5131542026133));
#195355=CARTESIAN_POINT('',(118.264573506239,8.25,49.807642304143));
#195356=CARTESIAN_POINT('',(118.321816480108,8.25,49.5131542026133));
#195357=CARTESIAN_POINT('Origin',(118.321816480108,7.75,49.5131542026133));
#195358=CARTESIAN_POINT('',(117.831002977559,7.75,49.417749246164));
#195359=CARTESIAN_POINT('',(117.773760003689,7.75,49.7122373476937));
#195360=CARTESIAN_POINT('',(117.831002977559,7.75,49.417749246164));
#195361=CARTESIAN_POINT('',(118.264573506239,7.75,49.807642304143));
#195362=CARTESIAN_POINT('',(118.321816480108,7.75,49.5131542026133));
#195363=CARTESIAN_POINT('Origin',(117.831002977559,7.75,49.417749246164));
#195364=CARTESIAN_POINT('',(117.773760003689,7.75,49.7122373476937));
#195365=CARTESIAN_POINT('',(117.831002977559,7.75,49.417749246164));
#195366=CARTESIAN_POINT('Origin',(117.045701373479,8.25,49.2651013158452));
#195367=CARTESIAN_POINT('',(117.536514876029,8.25,49.3605062722945));
#195368=CARTESIAN_POINT('',(117.479271902159,8.25,49.6549943738242));
#195369=CARTESIAN_POINT('',(117.536514876029,8.25,49.3605062722945));
#195370=CARTESIAN_POINT('',(116.98845839961,8.25,49.5595894173749));
#195371=CARTESIAN_POINT('',(116.98845839961,8.25,49.5595894173749));
#195372=CARTESIAN_POINT('',(117.045701373479,8.25,49.2651013158452));
#195373=CARTESIAN_POINT('',(117.045701373479,8.25,49.2651013158452));
#195374=CARTESIAN_POINT('',(117.045701373479,8.25,49.2651013158452));
#195375=CARTESIAN_POINT('Origin',(117.536514876029,8.25,49.3605062722945));
#195376=CARTESIAN_POINT('',(117.536514876029,7.75,49.3605062722945));
#195377=CARTESIAN_POINT('',(117.479271902159,7.75,49.6549943738242));
#195378=CARTESIAN_POINT('',(117.536514876029,7.75,49.3605062722945));
#195379=CARTESIAN_POINT('',(117.479271902159,8.25,49.6549943738242));
#195380=CARTESIAN_POINT('',(117.536514876029,8.25,49.3605062722945));
#195381=CARTESIAN_POINT('Origin',(117.536514876029,7.75,49.3605062722945));
#195382=CARTESIAN_POINT('',(117.045701373479,7.75,49.2651013158452));
#195383=CARTESIAN_POINT('',(116.98845839961,7.75,49.5595894173749));
#195384=CARTESIAN_POINT('',(117.045701373479,7.75,49.2651013158452));
#195385=CARTESIAN_POINT('',(117.479271902159,7.75,49.6549943738242));
#195386=CARTESIAN_POINT('',(117.536514876029,7.75,49.3605062722945));
#195387=CARTESIAN_POINT('Origin',(117.045701373479,7.75,49.2651013158452));
#195388=CARTESIAN_POINT('',(116.98845839961,7.75,49.5595894173749));
#195389=CARTESIAN_POINT('',(117.045701373479,7.75,49.2651013158452));
#195390=CARTESIAN_POINT('Origin',(116.2603997694,8.25,49.1124533855264));
#195391=CARTESIAN_POINT('',(116.75121327195,8.25,49.2078583419757));
#195392=CARTESIAN_POINT('',(116.69397029808,8.25,49.5023464435054));
#195393=CARTESIAN_POINT('',(116.75121327195,8.25,49.2078583419757));
#195394=CARTESIAN_POINT('',(116.203156795531,8.25,49.4069414870561));
#195395=CARTESIAN_POINT('',(116.203156795531,8.25,49.4069414870561));
#195396=CARTESIAN_POINT('',(116.2603997694,8.25,49.1124533855264));
#195397=CARTESIAN_POINT('',(116.2603997694,8.25,49.1124533855264));
#195398=CARTESIAN_POINT('',(116.2603997694,8.25,49.1124533855264));
#195399=CARTESIAN_POINT('Origin',(116.75121327195,8.25,49.2078583419757));
#195400=CARTESIAN_POINT('',(116.75121327195,7.75,49.2078583419757));
#195401=CARTESIAN_POINT('',(116.69397029808,7.75,49.5023464435054));
#195402=CARTESIAN_POINT('',(116.75121327195,7.75,49.2078583419757));
#195403=CARTESIAN_POINT('',(116.69397029808,8.25,49.5023464435054));
#195404=CARTESIAN_POINT('',(116.75121327195,8.25,49.2078583419757));
#195405=CARTESIAN_POINT('Origin',(116.75121327195,7.75,49.2078583419757));
#195406=CARTESIAN_POINT('',(116.2603997694,7.75,49.1124533855264));
#195407=CARTESIAN_POINT('',(116.203156795531,7.75,49.4069414870561));
#195408=CARTESIAN_POINT('',(116.2603997694,7.75,49.1124533855264));
#195409=CARTESIAN_POINT('',(116.69397029808,7.75,49.5023464435054));
#195410=CARTESIAN_POINT('',(116.75121327195,7.75,49.2078583419757));
#195411=CARTESIAN_POINT('Origin',(116.2603997694,7.75,49.1124533855264));
#195412=CARTESIAN_POINT('',(116.203156795531,7.75,49.4069414870561));
#195413=CARTESIAN_POINT('',(116.2603997694,7.75,49.1124533855264));
#195414=CARTESIAN_POINT('Origin',(115.475098165321,8.25,48.9598054552076));
#195415=CARTESIAN_POINT('',(115.96591166787,8.25,49.0552104116569));
#195416=CARTESIAN_POINT('',(115.908668694001,8.25,49.3496985131866));
#195417=CARTESIAN_POINT('',(115.96591166787,8.25,49.0552104116569));
#195418=CARTESIAN_POINT('',(115.417855191451,8.25,49.2542935567373));
#195419=CARTESIAN_POINT('',(115.417855191451,8.25,49.2542935567373));
#195420=CARTESIAN_POINT('',(115.475098165321,8.25,48.9598054552076));
#195421=CARTESIAN_POINT('',(115.475098165321,8.25,48.9598054552076));
#195422=CARTESIAN_POINT('',(115.475098165321,8.25,48.9598054552076));
#195423=CARTESIAN_POINT('Origin',(115.96591166787,8.25,49.0552104116569));
#195424=CARTESIAN_POINT('',(115.96591166787,7.75,49.0552104116569));
#195425=CARTESIAN_POINT('',(115.908668694001,7.75,49.3496985131866));
#195426=CARTESIAN_POINT('',(115.96591166787,7.75,49.0552104116569));
#195427=CARTESIAN_POINT('',(115.908668694001,8.25,49.3496985131866));
#195428=CARTESIAN_POINT('',(115.96591166787,8.25,49.0552104116569));
#195429=CARTESIAN_POINT('Origin',(115.96591166787,7.75,49.0552104116569));
#195430=CARTESIAN_POINT('',(115.475098165321,7.75,48.9598054552076));
#195431=CARTESIAN_POINT('',(115.417855191451,7.75,49.2542935567373));
#195432=CARTESIAN_POINT('',(115.475098165321,7.75,48.9598054552076));
#195433=CARTESIAN_POINT('',(115.908668694001,7.75,49.3496985131866));
#195434=CARTESIAN_POINT('',(115.96591166787,7.75,49.0552104116569));
#195435=CARTESIAN_POINT('Origin',(115.475098165321,7.75,48.9598054552076));
#195436=CARTESIAN_POINT('',(115.417855191451,7.75,49.2542935567373));
#195437=CARTESIAN_POINT('',(115.475098165321,7.75,48.9598054552076));
#195438=CARTESIAN_POINT('Origin',(114.689796561242,8.25,48.8071575248888));
#195439=CARTESIAN_POINT('',(115.180610063791,8.25,48.9025624813381));
#195440=CARTESIAN_POINT('',(115.123367089922,8.25,49.1970505828678));
#195441=CARTESIAN_POINT('',(115.180610063791,8.25,48.9025624813381));
#195442=CARTESIAN_POINT('',(114.632553587372,8.25,49.1016456264185));
#195443=CARTESIAN_POINT('',(114.632553587372,8.25,49.1016456264185));
#195444=CARTESIAN_POINT('',(114.689796561242,8.25,48.8071575248888));
#195445=CARTESIAN_POINT('',(114.689796561242,8.25,48.8071575248888));
#195446=CARTESIAN_POINT('',(114.689796561242,8.25,48.8071575248888));
#195447=CARTESIAN_POINT('Origin',(115.180610063791,8.25,48.9025624813381));
#195448=CARTESIAN_POINT('',(115.180610063791,7.75,48.9025624813381));
#195449=CARTESIAN_POINT('',(115.123367089922,7.75,49.1970505828678));
#195450=CARTESIAN_POINT('',(115.180610063791,7.75,48.9025624813381));
#195451=CARTESIAN_POINT('',(115.123367089922,8.25,49.1970505828678));
#195452=CARTESIAN_POINT('',(115.180610063791,8.25,48.9025624813381));
#195453=CARTESIAN_POINT('Origin',(115.180610063791,7.75,48.9025624813381));
#195454=CARTESIAN_POINT('',(114.689796561242,7.75,48.8071575248888));
#195455=CARTESIAN_POINT('',(114.632553587372,7.75,49.1016456264185));
#195456=CARTESIAN_POINT('',(114.689796561242,7.75,48.8071575248888));
#195457=CARTESIAN_POINT('',(115.123367089922,7.75,49.1970505828678));
#195458=CARTESIAN_POINT('',(115.180610063791,7.75,48.9025624813381));
#195459=CARTESIAN_POINT('Origin',(114.689796561242,7.75,48.8071575248888));
#195460=CARTESIAN_POINT('',(114.632553587372,7.75,49.1016456264185));
#195461=CARTESIAN_POINT('',(114.689796561242,7.75,48.8071575248888));
#195462=CARTESIAN_POINT('Origin',(113.904494957163,8.25,48.65450959457));
#195463=CARTESIAN_POINT('',(114.395308459712,8.25,48.7499145510193));
#195464=CARTESIAN_POINT('',(114.338065485842,8.25,49.044402652549));
#195465=CARTESIAN_POINT('',(114.395308459712,8.25,48.7499145510193));
#195466=CARTESIAN_POINT('',(113.847251983293,8.25,48.9489976960997));
#195467=CARTESIAN_POINT('',(113.847251983293,8.25,48.9489976960997));
#195468=CARTESIAN_POINT('',(113.904494957163,8.25,48.65450959457));
#195469=CARTESIAN_POINT('',(113.904494957163,8.25,48.65450959457));
#195470=CARTESIAN_POINT('',(113.904494957163,8.25,48.65450959457));
#195471=CARTESIAN_POINT('Origin',(114.395308459712,8.25,48.7499145510193));
#195472=CARTESIAN_POINT('',(114.395308459712,7.75,48.7499145510193));
#195473=CARTESIAN_POINT('',(114.338065485842,7.75,49.044402652549));
#195474=CARTESIAN_POINT('',(114.395308459712,7.75,48.7499145510193));
#195475=CARTESIAN_POINT('',(114.338065485842,8.25,49.044402652549));
#195476=CARTESIAN_POINT('',(114.395308459712,8.25,48.7499145510193));
#195477=CARTESIAN_POINT('Origin',(114.395308459712,7.75,48.7499145510193));
#195478=CARTESIAN_POINT('',(113.904494957163,7.75,48.65450959457));
#195479=CARTESIAN_POINT('',(113.847251983293,7.75,48.9489976960997));
#195480=CARTESIAN_POINT('',(113.904494957163,7.75,48.65450959457));
#195481=CARTESIAN_POINT('',(114.338065485842,7.75,49.044402652549));
#195482=CARTESIAN_POINT('',(114.395308459712,7.75,48.7499145510193));
#195483=CARTESIAN_POINT('Origin',(113.904494957163,7.75,48.65450959457));
#195484=CARTESIAN_POINT('',(113.847251983293,7.75,48.9489976960997));
#195485=CARTESIAN_POINT('',(113.904494957163,7.75,48.65450959457));
#195486=CARTESIAN_POINT('Origin',(113.119193353083,8.25,48.5018616642512));
#195487=CARTESIAN_POINT('',(113.610006855633,8.25,48.5972666207005));
#195488=CARTESIAN_POINT('',(113.552763881763,8.25,48.8917547222302));
#195489=CARTESIAN_POINT('',(113.610006855633,8.25,48.5972666207005));
#195490=CARTESIAN_POINT('',(113.061950379214,8.25,48.7963497657809));
#195491=CARTESIAN_POINT('',(113.061950379214,8.25,48.7963497657809));
#195492=CARTESIAN_POINT('',(113.119193353083,8.25,48.5018616642512));
#195493=CARTESIAN_POINT('',(113.119193353083,8.25,48.5018616642512));
#195494=CARTESIAN_POINT('',(113.119193353083,8.25,48.5018616642512));
#195495=CARTESIAN_POINT('Origin',(113.610006855633,8.25,48.5972666207005));
#195496=CARTESIAN_POINT('',(113.610006855633,7.75,48.5972666207005));
#195497=CARTESIAN_POINT('',(113.552763881763,7.75,48.8917547222302));
#195498=CARTESIAN_POINT('',(113.610006855633,7.75,48.5972666207005));
#195499=CARTESIAN_POINT('',(113.552763881763,8.25,48.8917547222302));
#195500=CARTESIAN_POINT('',(113.610006855633,8.25,48.5972666207005));
#195501=CARTESIAN_POINT('Origin',(113.610006855633,7.75,48.5972666207005));
#195502=CARTESIAN_POINT('',(113.119193353083,7.75,48.5018616642512));
#195503=CARTESIAN_POINT('',(113.061950379214,7.75,48.7963497657809));
#195504=CARTESIAN_POINT('',(113.119193353083,7.75,48.5018616642512));
#195505=CARTESIAN_POINT('',(113.552763881763,7.75,48.8917547222302));
#195506=CARTESIAN_POINT('',(113.610006855633,7.75,48.5972666207005));
#195507=CARTESIAN_POINT('Origin',(113.119193353083,7.75,48.5018616642512));
#195508=CARTESIAN_POINT('',(113.061950379214,7.75,48.7963497657809));
#195509=CARTESIAN_POINT('',(113.119193353083,7.75,48.5018616642512));
#195510=CARTESIAN_POINT('Origin',(112.333891749004,8.25,48.3492137339324));
#195511=CARTESIAN_POINT('',(112.824705251554,8.25,48.4446186903817));
#195512=CARTESIAN_POINT('',(112.767462277684,8.25,48.7391067919114));
#195513=CARTESIAN_POINT('',(112.824705251554,8.25,48.4446186903817));
#195514=CARTESIAN_POINT('',(112.276648775135,8.25,48.6437018354621));
#195515=CARTESIAN_POINT('',(112.276648775135,8.25,48.6437018354621));
#195516=CARTESIAN_POINT('',(112.333891749004,8.25,48.3492137339324));
#195517=CARTESIAN_POINT('',(112.333891749004,8.25,48.3492137339324));
#195518=CARTESIAN_POINT('',(112.333891749004,8.25,48.3492137339324));
#195519=CARTESIAN_POINT('Origin',(112.824705251554,8.25,48.4446186903817));
#195520=CARTESIAN_POINT('',(112.824705251554,7.75,48.4446186903817));
#195521=CARTESIAN_POINT('',(112.767462277684,7.75,48.7391067919114));
#195522=CARTESIAN_POINT('',(112.824705251554,7.75,48.4446186903817));
#195523=CARTESIAN_POINT('',(112.767462277684,8.25,48.7391067919114));
#195524=CARTESIAN_POINT('',(112.824705251554,8.25,48.4446186903817));
#195525=CARTESIAN_POINT('Origin',(112.824705251554,7.75,48.4446186903817));
#195526=CARTESIAN_POINT('',(112.333891749004,7.75,48.3492137339324));
#195527=CARTESIAN_POINT('',(112.276648775135,7.75,48.6437018354621));
#195528=CARTESIAN_POINT('',(112.333891749004,7.75,48.3492137339324));
#195529=CARTESIAN_POINT('',(112.767462277684,7.75,48.7391067919114));
#195530=CARTESIAN_POINT('',(112.824705251554,7.75,48.4446186903817));
#195531=CARTESIAN_POINT('Origin',(112.333891749004,7.75,48.3492137339324));
#195532=CARTESIAN_POINT('',(112.276648775135,7.75,48.6437018354621));
#195533=CARTESIAN_POINT('',(112.333891749004,7.75,48.3492137339324));
#195534=CARTESIAN_POINT('Origin',(109.977986936766,5.85,47.891269942976));
#195535=CARTESIAN_POINT('',(110.468800439316,5.85,47.9866748994252));
#195536=CARTESIAN_POINT('',(110.411557465446,5.85,48.2811630009549));
#195537=CARTESIAN_POINT('',(110.468800439316,5.85,47.9866748994252));
#195538=CARTESIAN_POINT('',(109.920743962897,5.85,48.1857580445057));
#195539=CARTESIAN_POINT('',(109.920743962897,5.85,48.1857580445057));
#195540=CARTESIAN_POINT('',(109.977986936766,5.85,47.891269942976));
#195541=CARTESIAN_POINT('',(109.977986936766,5.85,47.891269942976));
#195542=CARTESIAN_POINT('',(109.977986936766,5.85,47.891269942976));
#195543=CARTESIAN_POINT('Origin',(110.468800439316,5.85,47.9866748994252));
#195544=CARTESIAN_POINT('',(110.468800439316,5.35,47.9866748994252));
#195545=CARTESIAN_POINT('',(110.411557465446,5.35,48.2811630009549));
#195546=CARTESIAN_POINT('',(110.468800439316,5.35,47.9866748994252));
#195547=CARTESIAN_POINT('',(110.411557465446,5.85,48.2811630009549));
#195548=CARTESIAN_POINT('',(110.468800439316,5.85,47.9866748994252));
#195549=CARTESIAN_POINT('Origin',(110.468800439316,5.35,47.9866748994252));
#195550=CARTESIAN_POINT('',(109.977986936766,5.35,47.891269942976));
#195551=CARTESIAN_POINT('',(109.920743962897,5.35,48.1857580445057));
#195552=CARTESIAN_POINT('',(109.977986936766,5.35,47.891269942976));
#195553=CARTESIAN_POINT('',(110.411557465446,5.35,48.2811630009549));
#195554=CARTESIAN_POINT('',(110.468800439316,5.35,47.9866748994252));
#195555=CARTESIAN_POINT('Origin',(109.977986936766,5.35,47.891269942976));
#195556=CARTESIAN_POINT('',(109.920743962897,5.35,48.1857580445057));
#195557=CARTESIAN_POINT('',(109.977986936766,5.35,47.891269942976));
#195558=CARTESIAN_POINT('Origin',(109.977986936766,5.05,47.891269942976));
#195559=CARTESIAN_POINT('',(110.468800439316,5.05,47.9866748994252));
#195560=CARTESIAN_POINT('',(110.411557465446,5.05,48.2811630009549));
#195561=CARTESIAN_POINT('',(110.468800439316,5.05,47.9866748994252));
#195562=CARTESIAN_POINT('',(109.920743962897,5.05,48.1857580445057));
#195563=CARTESIAN_POINT('',(109.920743962897,5.05,48.1857580445057));
#195564=CARTESIAN_POINT('',(109.977986936766,5.05,47.891269942976));
#195565=CARTESIAN_POINT('',(109.977986936766,5.05,47.891269942976));
#195566=CARTESIAN_POINT('',(109.977986936766,5.05,47.891269942976));
#195567=CARTESIAN_POINT('Origin',(110.468800439316,5.05,47.9866748994252));
#195568=CARTESIAN_POINT('',(110.468800439316,4.55,47.9866748994252));
#195569=CARTESIAN_POINT('',(110.411557465446,4.55,48.2811630009549));
#195570=CARTESIAN_POINT('',(110.468800439316,4.55,47.9866748994252));
#195571=CARTESIAN_POINT('',(110.411557465446,5.05,48.2811630009549));
#195572=CARTESIAN_POINT('',(110.468800439316,5.05,47.9866748994252));
#195573=CARTESIAN_POINT('Origin',(110.468800439316,4.55,47.9866748994252));
#195574=CARTESIAN_POINT('',(109.977986936766,4.55,47.891269942976));
#195575=CARTESIAN_POINT('',(109.920743962897,4.55,48.1857580445057));
#195576=CARTESIAN_POINT('',(109.977986936766,4.55,47.891269942976));
#195577=CARTESIAN_POINT('',(110.411557465446,4.55,48.2811630009549));
#195578=CARTESIAN_POINT('',(110.468800439316,4.55,47.9866748994252));
#195579=CARTESIAN_POINT('Origin',(109.977986936766,4.55,47.891269942976));
#195580=CARTESIAN_POINT('',(109.920743962897,4.55,48.1857580445057));
#195581=CARTESIAN_POINT('',(109.977986936766,4.55,47.891269942976));
#195582=CARTESIAN_POINT('Origin',(109.977986936766,4.25,47.891269942976));
#195583=CARTESIAN_POINT('',(110.468800439316,4.25,47.9866748994252));
#195584=CARTESIAN_POINT('',(110.411557465446,4.25,48.2811630009549));
#195585=CARTESIAN_POINT('',(110.468800439316,4.25,47.9866748994252));
#195586=CARTESIAN_POINT('',(109.920743962897,4.25,48.1857580445057));
#195587=CARTESIAN_POINT('',(109.920743962897,4.25,48.1857580445057));
#195588=CARTESIAN_POINT('',(109.977986936766,4.25,47.891269942976));
#195589=CARTESIAN_POINT('',(109.977986936766,4.25,47.891269942976));
#195590=CARTESIAN_POINT('',(109.977986936766,4.25,47.891269942976));
#195591=CARTESIAN_POINT('Origin',(110.468800439316,4.25,47.9866748994252));
#195592=CARTESIAN_POINT('',(110.468800439316,3.75,47.9866748994252));
#195593=CARTESIAN_POINT('',(110.411557465446,3.75,48.2811630009549));
#195594=CARTESIAN_POINT('',(110.468800439316,3.75,47.9866748994252));
#195595=CARTESIAN_POINT('',(110.411557465446,4.25,48.2811630009549));
#195596=CARTESIAN_POINT('',(110.468800439316,4.25,47.9866748994252));
#195597=CARTESIAN_POINT('Origin',(110.468800439316,3.75,47.9866748994252));
#195598=CARTESIAN_POINT('',(109.977986936766,3.75,47.891269942976));
#195599=CARTESIAN_POINT('',(109.920743962897,3.75,48.1857580445057));
#195600=CARTESIAN_POINT('',(109.977986936766,3.75,47.891269942976));
#195601=CARTESIAN_POINT('',(110.411557465446,3.75,48.2811630009549));
#195602=CARTESIAN_POINT('',(110.468800439316,3.75,47.9866748994252));
#195603=CARTESIAN_POINT('Origin',(109.977986936766,3.75,47.891269942976));
#195604=CARTESIAN_POINT('',(109.920743962897,3.75,48.1857580445057));
#195605=CARTESIAN_POINT('',(109.977986936766,3.75,47.891269942976));
#195606=CARTESIAN_POINT('Origin',(109.977986936766,3.45,47.891269942976));
#195607=CARTESIAN_POINT('',(110.468800439316,3.45,47.9866748994252));
#195608=CARTESIAN_POINT('',(110.411557465446,3.45,48.2811630009549));
#195609=CARTESIAN_POINT('',(110.468800439316,3.45,47.9866748994252));
#195610=CARTESIAN_POINT('',(109.920743962897,3.45,48.1857580445057));
#195611=CARTESIAN_POINT('',(109.920743962897,3.45,48.1857580445057));
#195612=CARTESIAN_POINT('',(109.977986936766,3.45,47.891269942976));
#195613=CARTESIAN_POINT('',(109.977986936766,3.45,47.891269942976));
#195614=CARTESIAN_POINT('',(109.977986936766,3.45,47.891269942976));
#195615=CARTESIAN_POINT('Origin',(110.468800439316,3.45,47.9866748994252));
#195616=CARTESIAN_POINT('',(110.468800439316,2.95,47.9866748994252));
#195617=CARTESIAN_POINT('',(110.411557465446,2.95,48.2811630009549));
#195618=CARTESIAN_POINT('',(110.468800439316,2.95,47.9866748994252));
#195619=CARTESIAN_POINT('',(110.411557465446,3.45,48.2811630009549));
#195620=CARTESIAN_POINT('',(110.468800439316,3.45,47.9866748994252));
#195621=CARTESIAN_POINT('Origin',(110.468800439316,2.95,47.9866748994252));
#195622=CARTESIAN_POINT('',(109.977986936766,2.95,47.891269942976));
#195623=CARTESIAN_POINT('',(109.920743962897,2.95,48.1857580445057));
#195624=CARTESIAN_POINT('',(109.977986936766,2.95,47.891269942976));
#195625=CARTESIAN_POINT('',(110.411557465446,2.95,48.2811630009549));
#195626=CARTESIAN_POINT('',(110.468800439316,2.95,47.9866748994252));
#195627=CARTESIAN_POINT('Origin',(109.977986936766,2.95,47.891269942976));
#195628=CARTESIAN_POINT('',(109.920743962897,2.95,48.1857580445057));
#195629=CARTESIAN_POINT('',(109.977986936766,2.95,47.891269942976));
#195630=CARTESIAN_POINT('Origin',(109.977986936766,2.65,47.891269942976));
#195631=CARTESIAN_POINT('',(110.468800439316,2.65,47.9866748994252));
#195632=CARTESIAN_POINT('',(110.411557465446,2.65,48.2811630009549));
#195633=CARTESIAN_POINT('',(110.468800439316,2.65,47.9866748994252));
#195634=CARTESIAN_POINT('',(109.920743962897,2.65,48.1857580445057));
#195635=CARTESIAN_POINT('',(109.920743962897,2.65,48.1857580445057));
#195636=CARTESIAN_POINT('',(109.977986936766,2.65,47.891269942976));
#195637=CARTESIAN_POINT('',(109.977986936766,2.65,47.891269942976));
#195638=CARTESIAN_POINT('',(109.977986936766,2.65,47.891269942976));
#195639=CARTESIAN_POINT('Origin',(110.468800439316,2.65,47.9866748994252));
#195640=CARTESIAN_POINT('',(110.468800439316,2.15,47.9866748994252));
#195641=CARTESIAN_POINT('',(110.411557465446,2.15,48.2811630009549));
#195642=CARTESIAN_POINT('',(110.468800439316,2.15,47.9866748994252));
#195643=CARTESIAN_POINT('',(110.411557465446,2.65,48.2811630009549));
#195644=CARTESIAN_POINT('',(110.468800439316,2.65,47.9866748994252));
#195645=CARTESIAN_POINT('Origin',(110.468800439316,2.15,47.9866748994252));
#195646=CARTESIAN_POINT('',(109.977986936766,2.15,47.891269942976));
#195647=CARTESIAN_POINT('',(109.920743962897,2.15,48.1857580445057));
#195648=CARTESIAN_POINT('',(109.977986936766,2.15,47.891269942976));
#195649=CARTESIAN_POINT('',(110.411557465446,2.15,48.2811630009549));
#195650=CARTESIAN_POINT('',(110.468800439316,2.15,47.9866748994252));
#195651=CARTESIAN_POINT('Origin',(109.977986936766,2.15,47.891269942976));
#195652=CARTESIAN_POINT('',(109.920743962897,2.15,48.1857580445057));
#195653=CARTESIAN_POINT('',(109.977986936766,2.15,47.891269942976));
#195654=CARTESIAN_POINT('Origin',(109.977986936766,1.85,47.891269942976));
#195655=CARTESIAN_POINT('',(110.468800439316,1.85,47.9866748994252));
#195656=CARTESIAN_POINT('',(110.411557465446,1.85,48.2811630009549));
#195657=CARTESIAN_POINT('',(110.468800439316,1.85,47.9866748994252));
#195658=CARTESIAN_POINT('',(109.920743962897,1.85,48.1857580445057));
#195659=CARTESIAN_POINT('',(109.920743962897,1.85,48.1857580445057));
#195660=CARTESIAN_POINT('',(109.977986936766,1.85,47.891269942976));
#195661=CARTESIAN_POINT('',(109.977986936766,1.85,47.891269942976));
#195662=CARTESIAN_POINT('',(109.977986936766,1.85,47.891269942976));
#195663=CARTESIAN_POINT('Origin',(110.468800439316,1.85,47.9866748994252));
#195664=CARTESIAN_POINT('',(110.468800439316,1.35,47.9866748994252));
#195665=CARTESIAN_POINT('',(110.411557465446,1.35,48.2811630009549));
#195666=CARTESIAN_POINT('',(110.468800439316,1.35,47.9866748994252));
#195667=CARTESIAN_POINT('',(110.411557465446,1.85,48.2811630009549));
#195668=CARTESIAN_POINT('',(110.468800439316,1.85,47.9866748994252));
#195669=CARTESIAN_POINT('Origin',(110.468800439316,1.35,47.9866748994252));
#195670=CARTESIAN_POINT('',(109.977986936766,1.35,47.891269942976));
#195671=CARTESIAN_POINT('',(109.920743962897,1.35,48.1857580445057));
#195672=CARTESIAN_POINT('',(109.977986936766,1.35,47.891269942976));
#195673=CARTESIAN_POINT('',(110.411557465446,1.35,48.2811630009549));
#195674=CARTESIAN_POINT('',(110.468800439316,1.35,47.9866748994252));
#195675=CARTESIAN_POINT('Origin',(109.977986936766,1.35,47.891269942976));
#195676=CARTESIAN_POINT('',(109.920743962897,1.35,48.1857580445057));
#195677=CARTESIAN_POINT('',(109.977986936766,1.35,47.891269942976));
#195678=CARTESIAN_POINT('Origin',(109.977986936766,1.05,47.891269942976));
#195679=CARTESIAN_POINT('',(110.468800439316,1.05,47.9866748994252));
#195680=CARTESIAN_POINT('',(110.411557465446,1.05,48.2811630009549));
#195681=CARTESIAN_POINT('',(110.468800439316,1.05,47.9866748994252));
#195682=CARTESIAN_POINT('',(109.920743962897,1.05,48.1857580445057));
#195683=CARTESIAN_POINT('',(109.920743962897,1.05,48.1857580445057));
#195684=CARTESIAN_POINT('',(109.977986936766,1.05,47.891269942976));
#195685=CARTESIAN_POINT('',(109.977986936766,1.05,47.891269942976));
#195686=CARTESIAN_POINT('',(109.977986936766,1.05,47.891269942976));
#195687=CARTESIAN_POINT('Origin',(110.468800439316,1.05,47.9866748994252));
#195688=CARTESIAN_POINT('',(110.468800439316,0.550000000000015,47.9866748994252));
#195689=CARTESIAN_POINT('',(110.411557465446,0.550000000000015,48.2811630009549));
#195690=CARTESIAN_POINT('',(110.468800439316,0.550000000000015,47.9866748994252));
#195691=CARTESIAN_POINT('',(110.411557465446,1.05,48.2811630009549));
#195692=CARTESIAN_POINT('',(110.468800439316,1.05,47.9866748994252));
#195693=CARTESIAN_POINT('Origin',(110.468800439316,0.550000000000015,47.9866748994252));
#195694=CARTESIAN_POINT('',(109.977986936766,0.550000000000015,47.891269942976));
#195695=CARTESIAN_POINT('',(109.920743962897,0.550000000000015,48.1857580445057));
#195696=CARTESIAN_POINT('',(109.977986936766,0.550000000000015,47.891269942976));
#195697=CARTESIAN_POINT('',(110.411557465446,0.550000000000015,48.2811630009549));
#195698=CARTESIAN_POINT('',(110.468800439316,0.550000000000015,47.9866748994252));
#195699=CARTESIAN_POINT('Origin',(109.977986936766,0.550000000000015,47.891269942976));
#195700=CARTESIAN_POINT('',(109.920743962897,0.550000000000015,48.1857580445057));
#195701=CARTESIAN_POINT('',(109.977986936766,0.550000000000015,47.891269942976));
#195702=CARTESIAN_POINT('Origin',(109.977986936766,0.250000000000015,47.891269942976));
#195703=CARTESIAN_POINT('',(110.468800439316,0.250000000000015,47.9866748994252));
#195704=CARTESIAN_POINT('',(110.411557465446,0.250000000000015,48.2811630009549));
#195705=CARTESIAN_POINT('',(110.468800439316,0.250000000000015,47.9866748994252));
#195706=CARTESIAN_POINT('',(109.920743962897,0.250000000000015,48.1857580445057));
#195707=CARTESIAN_POINT('',(109.920743962897,0.250000000000015,48.1857580445057));
#195708=CARTESIAN_POINT('',(109.977986936766,0.250000000000015,47.891269942976));
#195709=CARTESIAN_POINT('',(109.977986936766,0.250000000000015,47.891269942976));
#195710=CARTESIAN_POINT('',(109.977986936766,0.250000000000015,47.891269942976));
#195711=CARTESIAN_POINT('Origin',(110.468800439316,0.250000000000015,47.9866748994252));
#195712=CARTESIAN_POINT('',(110.468800439316,-0.249999999999985,47.9866748994252));
#195713=CARTESIAN_POINT('',(110.411557465446,-0.249999999999985,48.2811630009549));
#195714=CARTESIAN_POINT('',(110.468800439316,-0.249999999999985,47.9866748994252));
#195715=CARTESIAN_POINT('',(110.411557465446,0.250000000000015,48.2811630009549));
#195716=CARTESIAN_POINT('',(110.468800439316,0.250000000000015,47.9866748994252));
#195717=CARTESIAN_POINT('Origin',(110.468800439316,-0.249999999999985,47.9866748994252));
#195718=CARTESIAN_POINT('',(109.977986936766,-0.249999999999985,47.891269942976));
#195719=CARTESIAN_POINT('',(109.920743962897,-0.249999999999985,48.1857580445057));
#195720=CARTESIAN_POINT('',(109.977986936766,-0.249999999999985,47.891269942976));
#195721=CARTESIAN_POINT('',(110.411557465446,-0.249999999999985,48.2811630009549));
#195722=CARTESIAN_POINT('',(110.468800439316,-0.249999999999985,47.9866748994252));
#195723=CARTESIAN_POINT('Origin',(109.977986936766,-0.249999999999985,47.891269942976));
#195724=CARTESIAN_POINT('',(109.920743962897,-0.249999999999985,48.1857580445057));
#195725=CARTESIAN_POINT('',(109.977986936766,-0.249999999999985,47.891269942976));
#195726=CARTESIAN_POINT('Origin',(109.977986936766,-0.549999999999986,47.891269942976));
#195727=CARTESIAN_POINT('',(110.468800439316,-0.549999999999986,47.9866748994252));
#195728=CARTESIAN_POINT('',(110.411557465446,-0.549999999999986,48.2811630009549));
#195729=CARTESIAN_POINT('',(110.468800439316,-0.549999999999986,47.9866748994252));
#195730=CARTESIAN_POINT('',(109.920743962897,-0.549999999999986,48.1857580445057));
#195731=CARTESIAN_POINT('',(109.920743962897,-0.549999999999986,48.1857580445057));
#195732=CARTESIAN_POINT('',(109.977986936766,-0.549999999999986,47.891269942976));
#195733=CARTESIAN_POINT('',(109.977986936766,-0.549999999999986,47.891269942976));
#195734=CARTESIAN_POINT('',(109.977986936766,-0.549999999999986,47.891269942976));
#195735=CARTESIAN_POINT('Origin',(110.468800439316,-0.549999999999986,47.9866748994252));
#195736=CARTESIAN_POINT('',(110.468800439316,-1.05,47.9866748994252));
#195737=CARTESIAN_POINT('',(110.411557465446,-1.05,48.2811630009549));
#195738=CARTESIAN_POINT('',(110.468800439316,-1.05,47.9866748994252));
#195739=CARTESIAN_POINT('',(110.411557465446,-0.549999999999986,48.2811630009549));
#195740=CARTESIAN_POINT('',(110.468800439316,-0.549999999999986,47.9866748994252));
#195741=CARTESIAN_POINT('Origin',(110.468800439316,-1.05,47.9866748994252));
#195742=CARTESIAN_POINT('',(109.977986936766,-1.05,47.891269942976));
#195743=CARTESIAN_POINT('',(109.920743962897,-1.05,48.1857580445057));
#195744=CARTESIAN_POINT('',(109.977986936766,-1.05,47.891269942976));
#195745=CARTESIAN_POINT('',(110.411557465446,-1.05,48.2811630009549));
#195746=CARTESIAN_POINT('',(110.468800439316,-1.05,47.9866748994252));
#195747=CARTESIAN_POINT('Origin',(109.977986936766,-1.05,47.891269942976));
#195748=CARTESIAN_POINT('',(109.920743962897,-1.05,48.1857580445057));
#195749=CARTESIAN_POINT('',(109.977986936766,-1.05,47.891269942976));
#195750=CARTESIAN_POINT('Origin',(109.977986936766,-1.35,47.891269942976));
#195751=CARTESIAN_POINT('',(110.468800439316,-1.35,47.9866748994252));
#195752=CARTESIAN_POINT('',(110.411557465446,-1.35,48.2811630009549));
#195753=CARTESIAN_POINT('',(110.468800439316,-1.35,47.9866748994252));
#195754=CARTESIAN_POINT('',(109.920743962897,-1.35,48.1857580445057));
#195755=CARTESIAN_POINT('',(109.920743962897,-1.35,48.1857580445057));
#195756=CARTESIAN_POINT('',(109.977986936766,-1.35,47.891269942976));
#195757=CARTESIAN_POINT('',(109.977986936766,-1.35,47.891269942976));
#195758=CARTESIAN_POINT('',(109.977986936766,-1.35,47.891269942976));
#195759=CARTESIAN_POINT('Origin',(110.468800439316,-1.35,47.9866748994252));
#195760=CARTESIAN_POINT('',(110.468800439316,-1.85,47.9866748994252));
#195761=CARTESIAN_POINT('',(110.411557465446,-1.85,48.2811630009549));
#195762=CARTESIAN_POINT('',(110.468800439316,-1.85,47.9866748994252));
#195763=CARTESIAN_POINT('',(110.411557465446,-1.35,48.2811630009549));
#195764=CARTESIAN_POINT('',(110.468800439316,-1.35,47.9866748994252));
#195765=CARTESIAN_POINT('Origin',(110.468800439316,-1.85,47.9866748994252));
#195766=CARTESIAN_POINT('',(109.977986936766,-1.85,47.891269942976));
#195767=CARTESIAN_POINT('',(109.920743962897,-1.85,48.1857580445057));
#195768=CARTESIAN_POINT('',(109.977986936766,-1.85,47.891269942976));
#195769=CARTESIAN_POINT('',(110.411557465446,-1.85,48.2811630009549));
#195770=CARTESIAN_POINT('',(110.468800439316,-1.85,47.9866748994252));
#195771=CARTESIAN_POINT('Origin',(109.977986936766,-1.85,47.891269942976));
#195772=CARTESIAN_POINT('',(109.920743962897,-1.85,48.1857580445057));
#195773=CARTESIAN_POINT('',(109.977986936766,-1.85,47.891269942976));
#195774=CARTESIAN_POINT('Origin',(109.977986936766,-2.15,47.891269942976));
#195775=CARTESIAN_POINT('',(110.468800439316,-2.15,47.9866748994252));
#195776=CARTESIAN_POINT('',(110.411557465446,-2.15,48.2811630009549));
#195777=CARTESIAN_POINT('',(110.468800439316,-2.15,47.9866748994252));
#195778=CARTESIAN_POINT('',(109.920743962897,-2.15,48.1857580445057));
#195779=CARTESIAN_POINT('',(109.920743962897,-2.15,48.1857580445057));
#195780=CARTESIAN_POINT('',(109.977986936766,-2.15,47.891269942976));
#195781=CARTESIAN_POINT('',(109.977986936766,-2.15,47.891269942976));
#195782=CARTESIAN_POINT('',(109.977986936766,-2.15,47.891269942976));
#195783=CARTESIAN_POINT('Origin',(110.468800439316,-2.15,47.9866748994252));
#195784=CARTESIAN_POINT('',(110.468800439316,-2.65,47.9866748994252));
#195785=CARTESIAN_POINT('',(110.411557465446,-2.65,48.2811630009549));
#195786=CARTESIAN_POINT('',(110.468800439316,-2.65,47.9866748994252));
#195787=CARTESIAN_POINT('',(110.411557465446,-2.15,48.2811630009549));
#195788=CARTESIAN_POINT('',(110.468800439316,-2.15,47.9866748994252));
#195789=CARTESIAN_POINT('Origin',(110.468800439316,-2.65,47.9866748994252));
#195790=CARTESIAN_POINT('',(109.977986936766,-2.65,47.891269942976));
#195791=CARTESIAN_POINT('',(109.920743962897,-2.65,48.1857580445057));
#195792=CARTESIAN_POINT('',(109.977986936766,-2.65,47.891269942976));
#195793=CARTESIAN_POINT('',(110.411557465446,-2.65,48.2811630009549));
#195794=CARTESIAN_POINT('',(110.468800439316,-2.65,47.9866748994252));
#195795=CARTESIAN_POINT('Origin',(109.977986936766,-2.65,47.891269942976));
#195796=CARTESIAN_POINT('',(109.920743962897,-2.65,48.1857580445057));
#195797=CARTESIAN_POINT('',(109.977986936766,-2.65,47.891269942976));
#195798=CARTESIAN_POINT('Origin',(109.977986936766,-2.95,47.891269942976));
#195799=CARTESIAN_POINT('',(110.468800439316,-2.95,47.9866748994252));
#195800=CARTESIAN_POINT('',(110.411557465446,-2.95,48.2811630009549));
#195801=CARTESIAN_POINT('',(110.468800439316,-2.95,47.9866748994252));
#195802=CARTESIAN_POINT('',(109.920743962897,-2.95,48.1857580445057));
#195803=CARTESIAN_POINT('',(109.920743962897,-2.95,48.1857580445057));
#195804=CARTESIAN_POINT('',(109.977986936766,-2.95,47.891269942976));
#195805=CARTESIAN_POINT('',(109.977986936766,-2.95,47.891269942976));
#195806=CARTESIAN_POINT('',(109.977986936766,-2.95,47.891269942976));
#195807=CARTESIAN_POINT('Origin',(110.468800439316,-2.95,47.9866748994252));
#195808=CARTESIAN_POINT('',(110.468800439316,-3.45,47.9866748994252));
#195809=CARTESIAN_POINT('',(110.411557465446,-3.45,48.2811630009549));
#195810=CARTESIAN_POINT('',(110.468800439316,-3.45,47.9866748994252));
#195811=CARTESIAN_POINT('',(110.411557465446,-2.95,48.2811630009549));
#195812=CARTESIAN_POINT('',(110.468800439316,-2.95,47.9866748994252));
#195813=CARTESIAN_POINT('Origin',(110.468800439316,-3.45,47.9866748994252));
#195814=CARTESIAN_POINT('',(109.977986936766,-3.45,47.891269942976));
#195815=CARTESIAN_POINT('',(109.920743962897,-3.45,48.1857580445057));
#195816=CARTESIAN_POINT('',(109.977986936766,-3.45,47.891269942976));
#195817=CARTESIAN_POINT('',(110.411557465446,-3.45,48.2811630009549));
#195818=CARTESIAN_POINT('',(110.468800439316,-3.45,47.9866748994252));
#195819=CARTESIAN_POINT('Origin',(109.977986936766,-3.45,47.891269942976));
#195820=CARTESIAN_POINT('',(109.920743962897,-3.45,48.1857580445057));
#195821=CARTESIAN_POINT('',(109.977986936766,-3.45,47.891269942976));
#195822=CARTESIAN_POINT('Origin',(109.977986936766,-3.75,47.891269942976));
#195823=CARTESIAN_POINT('',(110.468800439316,-3.75,47.9866748994252));
#195824=CARTESIAN_POINT('',(110.411557465446,-3.75,48.2811630009549));
#195825=CARTESIAN_POINT('',(110.468800439316,-3.75,47.9866748994252));
#195826=CARTESIAN_POINT('',(109.920743962897,-3.75,48.1857580445057));
#195827=CARTESIAN_POINT('',(109.920743962897,-3.75,48.1857580445057));
#195828=CARTESIAN_POINT('',(109.977986936766,-3.75,47.891269942976));
#195829=CARTESIAN_POINT('',(109.977986936766,-3.75,47.891269942976));
#195830=CARTESIAN_POINT('',(109.977986936766,-3.75,47.891269942976));
#195831=CARTESIAN_POINT('Origin',(110.468800439316,-3.75,47.9866748994252));
#195832=CARTESIAN_POINT('',(110.468800439316,-4.25,47.9866748994252));
#195833=CARTESIAN_POINT('',(110.411557465446,-4.25,48.2811630009549));
#195834=CARTESIAN_POINT('',(110.468800439316,-4.25,47.9866748994252));
#195835=CARTESIAN_POINT('',(110.411557465446,-3.75,48.2811630009549));
#195836=CARTESIAN_POINT('',(110.468800439316,-3.75,47.9866748994252));
#195837=CARTESIAN_POINT('Origin',(110.468800439316,-4.25,47.9866748994252));
#195838=CARTESIAN_POINT('',(109.977986936766,-4.25,47.891269942976));
#195839=CARTESIAN_POINT('',(109.920743962897,-4.25,48.1857580445057));
#195840=CARTESIAN_POINT('',(109.977986936766,-4.25,47.891269942976));
#195841=CARTESIAN_POINT('',(110.411557465446,-4.25,48.2811630009549));
#195842=CARTESIAN_POINT('',(110.468800439316,-4.25,47.9866748994252));
#195843=CARTESIAN_POINT('Origin',(109.977986936766,-4.25,47.891269942976));
#195844=CARTESIAN_POINT('',(109.920743962897,-4.25,48.1857580445057));
#195845=CARTESIAN_POINT('',(109.977986936766,-4.25,47.891269942976));
#195846=CARTESIAN_POINT('Origin',(109.977986936766,-4.55,47.891269942976));
#195847=CARTESIAN_POINT('',(110.468800439316,-4.55,47.9866748994252));
#195848=CARTESIAN_POINT('',(110.411557465446,-4.55,48.2811630009549));
#195849=CARTESIAN_POINT('',(110.468800439316,-4.55,47.9866748994252));
#195850=CARTESIAN_POINT('',(109.920743962897,-4.55,48.1857580445057));
#195851=CARTESIAN_POINT('',(109.920743962897,-4.55,48.1857580445057));
#195852=CARTESIAN_POINT('',(109.977986936766,-4.55,47.891269942976));
#195853=CARTESIAN_POINT('',(109.977986936766,-4.55,47.891269942976));
#195854=CARTESIAN_POINT('',(109.977986936766,-4.55,47.891269942976));
#195855=CARTESIAN_POINT('Origin',(110.468800439316,-4.55,47.9866748994252));
#195856=CARTESIAN_POINT('',(110.468800439316,-5.05,47.9866748994252));
#195857=CARTESIAN_POINT('',(110.411557465446,-5.05,48.2811630009549));
#195858=CARTESIAN_POINT('',(110.468800439316,-5.05,47.9866748994252));
#195859=CARTESIAN_POINT('',(110.411557465446,-4.55,48.2811630009549));
#195860=CARTESIAN_POINT('',(110.468800439316,-4.55,47.9866748994252));
#195861=CARTESIAN_POINT('Origin',(110.468800439316,-5.05,47.9866748994252));
#195862=CARTESIAN_POINT('',(109.977986936766,-5.05,47.891269942976));
#195863=CARTESIAN_POINT('',(109.920743962897,-5.05,48.1857580445057));
#195864=CARTESIAN_POINT('',(109.977986936766,-5.05,47.891269942976));
#195865=CARTESIAN_POINT('',(110.411557465446,-5.05,48.2811630009549));
#195866=CARTESIAN_POINT('',(110.468800439316,-5.05,47.9866748994252));
#195867=CARTESIAN_POINT('Origin',(109.977986936766,-5.05,47.891269942976));
#195868=CARTESIAN_POINT('',(109.920743962897,-5.05,48.1857580445057));
#195869=CARTESIAN_POINT('',(109.977986936766,-5.05,47.891269942976));
#195870=CARTESIAN_POINT('Origin',(109.977986936766,-5.35,47.891269942976));
#195871=CARTESIAN_POINT('',(110.468800439316,-5.35,47.9866748994252));
#195872=CARTESIAN_POINT('',(110.411557465446,-5.35,48.2811630009549));
#195873=CARTESIAN_POINT('',(110.468800439316,-5.35,47.9866748994252));
#195874=CARTESIAN_POINT('',(109.920743962897,-5.35,48.1857580445057));
#195875=CARTESIAN_POINT('',(109.920743962897,-5.35,48.1857580445057));
#195876=CARTESIAN_POINT('',(109.977986936766,-5.35,47.891269942976));
#195877=CARTESIAN_POINT('',(109.977986936766,-5.35,47.891269942976));
#195878=CARTESIAN_POINT('',(109.977986936766,-5.35,47.891269942976));
#195879=CARTESIAN_POINT('Origin',(110.468800439316,-5.35,47.9866748994252));
#195880=CARTESIAN_POINT('',(110.468800439316,-5.85,47.9866748994252));
#195881=CARTESIAN_POINT('',(110.411557465446,-5.85,48.2811630009549));
#195882=CARTESIAN_POINT('',(110.468800439316,-5.85,47.9866748994252));
#195883=CARTESIAN_POINT('',(110.411557465446,-5.35,48.2811630009549));
#195884=CARTESIAN_POINT('',(110.468800439316,-5.35,47.9866748994252));
#195885=CARTESIAN_POINT('Origin',(110.468800439316,-5.85,47.9866748994252));
#195886=CARTESIAN_POINT('',(109.977986936766,-5.85,47.891269942976));
#195887=CARTESIAN_POINT('',(109.920743962897,-5.85,48.1857580445057));
#195888=CARTESIAN_POINT('',(109.977986936766,-5.85,47.891269942976));
#195889=CARTESIAN_POINT('',(110.411557465446,-5.85,48.2811630009549));
#195890=CARTESIAN_POINT('',(110.468800439316,-5.85,47.9866748994252));
#195891=CARTESIAN_POINT('Origin',(109.977986936766,-5.85,47.891269942976));
#195892=CARTESIAN_POINT('',(109.920743962897,-5.85,48.1857580445057));
#195893=CARTESIAN_POINT('',(109.977986936766,-5.85,47.891269942976));
#195894=CARTESIAN_POINT('Origin',(111.548590144925,-6.95,48.1965658036136));
#195895=CARTESIAN_POINT('',(112.039403647474,-6.95,48.2919707600629));
#195896=CARTESIAN_POINT('',(111.982160673605,-6.95,48.5864588615926));
#195897=CARTESIAN_POINT('',(112.039403647474,-6.95,48.2919707600629));
#195898=CARTESIAN_POINT('',(111.491347171055,-6.95,48.4910539051433));
#195899=CARTESIAN_POINT('',(111.491347171055,-6.95,48.4910539051433));
#195900=CARTESIAN_POINT('',(111.548590144925,-6.95,48.1965658036136));
#195901=CARTESIAN_POINT('',(111.548590144925,-6.95,48.1965658036136));
#195902=CARTESIAN_POINT('',(111.548590144925,-6.95,48.1965658036136));
#195903=CARTESIAN_POINT('Origin',(112.039403647474,-6.95,48.2919707600629));
#195904=CARTESIAN_POINT('',(112.039403647474,-7.45,48.2919707600629));
#195905=CARTESIAN_POINT('',(111.982160673605,-7.45,48.5864588615926));
#195906=CARTESIAN_POINT('',(112.039403647474,-7.45,48.2919707600629));
#195907=CARTESIAN_POINT('',(111.982160673605,-6.95,48.5864588615926));
#195908=CARTESIAN_POINT('',(112.039403647474,-6.95,48.2919707600629));
#195909=CARTESIAN_POINT('Origin',(112.039403647474,-7.45,48.2919707600629));
#195910=CARTESIAN_POINT('',(111.548590144925,-7.45,48.1965658036136));
#195911=CARTESIAN_POINT('',(111.491347171055,-7.45,48.4910539051433));
#195912=CARTESIAN_POINT('',(111.548590144925,-7.45,48.1965658036136));
#195913=CARTESIAN_POINT('',(111.982160673605,-7.45,48.5864588615926));
#195914=CARTESIAN_POINT('',(112.039403647474,-7.45,48.2919707600629));
#195915=CARTESIAN_POINT('Origin',(111.548590144925,-7.45,48.1965658036136));
#195916=CARTESIAN_POINT('',(111.491347171055,-7.45,48.4910539051433));
#195917=CARTESIAN_POINT('',(111.548590144925,-7.45,48.1965658036136));
#195918=CARTESIAN_POINT('Origin',(112.333891749004,-6.95,48.3492137339324));
#195919=CARTESIAN_POINT('',(112.824705251554,-6.95,48.4446186903817));
#195920=CARTESIAN_POINT('',(112.767462277684,-6.95,48.7391067919114));
#195921=CARTESIAN_POINT('',(112.824705251554,-6.95,48.4446186903817));
#195922=CARTESIAN_POINT('',(112.276648775135,-6.95,48.6437018354621));
#195923=CARTESIAN_POINT('',(112.276648775135,-6.95,48.6437018354621));
#195924=CARTESIAN_POINT('',(112.333891749004,-6.95,48.3492137339324));
#195925=CARTESIAN_POINT('',(112.333891749004,-6.95,48.3492137339324));
#195926=CARTESIAN_POINT('',(112.333891749004,-6.95,48.3492137339324));
#195927=CARTESIAN_POINT('Origin',(112.824705251554,-6.95,48.4446186903817));
#195928=CARTESIAN_POINT('',(112.824705251554,-7.45,48.4446186903817));
#195929=CARTESIAN_POINT('',(112.767462277684,-7.45,48.7391067919114));
#195930=CARTESIAN_POINT('',(112.824705251554,-7.45,48.4446186903817));
#195931=CARTESIAN_POINT('',(112.767462277684,-6.95,48.7391067919114));
#195932=CARTESIAN_POINT('',(112.824705251554,-6.95,48.4446186903817));
#195933=CARTESIAN_POINT('Origin',(112.824705251554,-7.45,48.4446186903817));
#195934=CARTESIAN_POINT('',(112.333891749004,-7.45,48.3492137339324));
#195935=CARTESIAN_POINT('',(112.276648775135,-7.45,48.6437018354621));
#195936=CARTESIAN_POINT('',(112.333891749004,-7.45,48.3492137339324));
#195937=CARTESIAN_POINT('',(112.767462277684,-7.45,48.7391067919114));
#195938=CARTESIAN_POINT('',(112.824705251554,-7.45,48.4446186903817));
#195939=CARTESIAN_POINT('Origin',(112.333891749004,-7.45,48.3492137339324));
#195940=CARTESIAN_POINT('',(112.276648775135,-7.45,48.6437018354621));
#195941=CARTESIAN_POINT('',(112.333891749004,-7.45,48.3492137339324));
#195942=CARTESIAN_POINT('Origin',(113.119193353083,-6.95,48.5018616642512));
#195943=CARTESIAN_POINT('',(113.610006855633,-6.95,48.5972666207005));
#195944=CARTESIAN_POINT('',(113.552763881763,-6.95,48.8917547222302));
#195945=CARTESIAN_POINT('',(113.610006855633,-6.95,48.5972666207005));
#195946=CARTESIAN_POINT('',(113.061950379214,-6.95,48.7963497657809));
#195947=CARTESIAN_POINT('',(113.061950379214,-6.95,48.7963497657809));
#195948=CARTESIAN_POINT('',(113.119193353083,-6.95,48.5018616642512));
#195949=CARTESIAN_POINT('',(113.119193353083,-6.95,48.5018616642512));
#195950=CARTESIAN_POINT('',(113.119193353083,-6.95,48.5018616642512));
#195951=CARTESIAN_POINT('Origin',(113.610006855633,-6.95,48.5972666207005));
#195952=CARTESIAN_POINT('',(113.610006855633,-7.45,48.5972666207005));
#195953=CARTESIAN_POINT('',(113.552763881763,-7.45,48.8917547222302));
#195954=CARTESIAN_POINT('',(113.610006855633,-7.45,48.5972666207005));
#195955=CARTESIAN_POINT('',(113.552763881763,-6.95,48.8917547222302));
#195956=CARTESIAN_POINT('',(113.610006855633,-6.95,48.5972666207005));
#195957=CARTESIAN_POINT('Origin',(113.610006855633,-7.45,48.5972666207005));
#195958=CARTESIAN_POINT('',(113.119193353083,-7.45,48.5018616642512));
#195959=CARTESIAN_POINT('',(113.061950379214,-7.45,48.7963497657809));
#195960=CARTESIAN_POINT('',(113.119193353083,-7.45,48.5018616642512));
#195961=CARTESIAN_POINT('',(113.552763881763,-7.45,48.8917547222302));
#195962=CARTESIAN_POINT('',(113.610006855633,-7.45,48.5972666207005));
#195963=CARTESIAN_POINT('Origin',(113.119193353083,-7.45,48.5018616642512));
#195964=CARTESIAN_POINT('',(113.061950379214,-7.45,48.7963497657809));
#195965=CARTESIAN_POINT('',(113.119193353083,-7.45,48.5018616642512));
#195966=CARTESIAN_POINT('Origin',(113.904494957163,-6.95,48.65450959457));
#195967=CARTESIAN_POINT('',(114.395308459712,-6.95,48.7499145510193));
#195968=CARTESIAN_POINT('',(114.338065485842,-6.95,49.044402652549));
#195969=CARTESIAN_POINT('',(114.395308459712,-6.95,48.7499145510193));
#195970=CARTESIAN_POINT('',(113.847251983293,-6.95,48.9489976960997));
#195971=CARTESIAN_POINT('',(113.847251983293,-6.95,48.9489976960997));
#195972=CARTESIAN_POINT('',(113.904494957163,-6.95,48.65450959457));
#195973=CARTESIAN_POINT('',(113.904494957163,-6.95,48.65450959457));
#195974=CARTESIAN_POINT('',(113.904494957163,-6.95,48.65450959457));
#195975=CARTESIAN_POINT('Origin',(114.395308459712,-6.95,48.7499145510193));
#195976=CARTESIAN_POINT('',(114.395308459712,-7.45,48.7499145510193));
#195977=CARTESIAN_POINT('',(114.338065485842,-7.45,49.044402652549));
#195978=CARTESIAN_POINT('',(114.395308459712,-7.45,48.7499145510193));
#195979=CARTESIAN_POINT('',(114.338065485842,-6.95,49.044402652549));
#195980=CARTESIAN_POINT('',(114.395308459712,-6.95,48.7499145510193));
#195981=CARTESIAN_POINT('Origin',(114.395308459712,-7.45,48.7499145510193));
#195982=CARTESIAN_POINT('',(113.904494957163,-7.45,48.65450959457));
#195983=CARTESIAN_POINT('',(113.847251983293,-7.45,48.9489976960997));
#195984=CARTESIAN_POINT('',(113.904494957163,-7.45,48.65450959457));
#195985=CARTESIAN_POINT('',(114.338065485842,-7.45,49.044402652549));
#195986=CARTESIAN_POINT('',(114.395308459712,-7.45,48.7499145510193));
#195987=CARTESIAN_POINT('Origin',(113.904494957163,-7.45,48.65450959457));
#195988=CARTESIAN_POINT('',(113.847251983293,-7.45,48.9489976960997));
#195989=CARTESIAN_POINT('',(113.904494957163,-7.45,48.65450959457));
#195990=CARTESIAN_POINT('Origin',(114.689796561242,-6.95,48.8071575248888));
#195991=CARTESIAN_POINT('',(115.180610063791,-6.95,48.9025624813381));
#195992=CARTESIAN_POINT('',(115.123367089922,-6.95,49.1970505828678));
#195993=CARTESIAN_POINT('',(115.180610063791,-6.95,48.9025624813381));
#195994=CARTESIAN_POINT('',(114.632553587372,-6.95,49.1016456264185));
#195995=CARTESIAN_POINT('',(114.632553587372,-6.95,49.1016456264185));
#195996=CARTESIAN_POINT('',(114.689796561242,-6.95,48.8071575248888));
#195997=CARTESIAN_POINT('',(114.689796561242,-6.95,48.8071575248888));
#195998=CARTESIAN_POINT('',(114.689796561242,-6.95,48.8071575248888));
#195999=CARTESIAN_POINT('Origin',(115.180610063791,-6.95,48.9025624813381));
#196000=CARTESIAN_POINT('',(115.180610063791,-7.45,48.9025624813381));
#196001=CARTESIAN_POINT('',(115.123367089922,-7.45,49.1970505828678));
#196002=CARTESIAN_POINT('',(115.180610063791,-7.45,48.9025624813381));
#196003=CARTESIAN_POINT('',(115.123367089922,-6.95,49.1970505828678));
#196004=CARTESIAN_POINT('',(115.180610063791,-6.95,48.9025624813381));
#196005=CARTESIAN_POINT('Origin',(115.180610063791,-7.45,48.9025624813381));
#196006=CARTESIAN_POINT('',(114.689796561242,-7.45,48.8071575248888));
#196007=CARTESIAN_POINT('',(114.632553587372,-7.45,49.1016456264185));
#196008=CARTESIAN_POINT('',(114.689796561242,-7.45,48.8071575248888));
#196009=CARTESIAN_POINT('',(115.123367089922,-7.45,49.1970505828678));
#196010=CARTESIAN_POINT('',(115.180610063791,-7.45,48.9025624813381));
#196011=CARTESIAN_POINT('Origin',(114.689796561242,-7.45,48.8071575248888));
#196012=CARTESIAN_POINT('',(114.632553587372,-7.45,49.1016456264185));
#196013=CARTESIAN_POINT('',(114.689796561242,-7.45,48.8071575248888));
#196014=CARTESIAN_POINT('Origin',(115.475098165321,-6.95,48.9598054552076));
#196015=CARTESIAN_POINT('',(115.96591166787,-6.95,49.0552104116569));
#196016=CARTESIAN_POINT('',(115.908668694001,-6.95,49.3496985131866));
#196017=CARTESIAN_POINT('',(115.96591166787,-6.95,49.0552104116569));
#196018=CARTESIAN_POINT('',(115.417855191451,-6.95,49.2542935567373));
#196019=CARTESIAN_POINT('',(115.417855191451,-6.95,49.2542935567373));
#196020=CARTESIAN_POINT('',(115.475098165321,-6.95,48.9598054552076));
#196021=CARTESIAN_POINT('',(115.475098165321,-6.95,48.9598054552076));
#196022=CARTESIAN_POINT('',(115.475098165321,-6.95,48.9598054552076));
#196023=CARTESIAN_POINT('Origin',(115.96591166787,-6.95,49.0552104116569));
#196024=CARTESIAN_POINT('',(115.96591166787,-7.45,49.0552104116569));
#196025=CARTESIAN_POINT('',(115.908668694001,-7.45,49.3496985131866));
#196026=CARTESIAN_POINT('',(115.96591166787,-7.45,49.0552104116569));
#196027=CARTESIAN_POINT('',(115.908668694001,-6.95,49.3496985131866));
#196028=CARTESIAN_POINT('',(115.96591166787,-6.95,49.0552104116569));
#196029=CARTESIAN_POINT('Origin',(115.96591166787,-7.45,49.0552104116569));
#196030=CARTESIAN_POINT('',(115.475098165321,-7.45,48.9598054552076));
#196031=CARTESIAN_POINT('',(115.417855191451,-7.45,49.2542935567373));
#196032=CARTESIAN_POINT('',(115.475098165321,-7.45,48.9598054552076));
#196033=CARTESIAN_POINT('',(115.908668694001,-7.45,49.3496985131866));
#196034=CARTESIAN_POINT('',(115.96591166787,-7.45,49.0552104116569));
#196035=CARTESIAN_POINT('Origin',(115.475098165321,-7.45,48.9598054552076));
#196036=CARTESIAN_POINT('',(115.417855191451,-7.45,49.2542935567373));
#196037=CARTESIAN_POINT('',(115.475098165321,-7.45,48.9598054552076));
#196038=CARTESIAN_POINT('Origin',(116.2603997694,-6.95,49.1124533855264));
#196039=CARTESIAN_POINT('',(116.75121327195,-6.95,49.2078583419757));
#196040=CARTESIAN_POINT('',(116.69397029808,-6.95,49.5023464435054));
#196041=CARTESIAN_POINT('',(116.75121327195,-6.95,49.2078583419757));
#196042=CARTESIAN_POINT('',(116.203156795531,-6.95,49.4069414870561));
#196043=CARTESIAN_POINT('',(116.203156795531,-6.95,49.4069414870561));
#196044=CARTESIAN_POINT('',(116.2603997694,-6.95,49.1124533855264));
#196045=CARTESIAN_POINT('',(116.2603997694,-6.95,49.1124533855264));
#196046=CARTESIAN_POINT('',(116.2603997694,-6.95,49.1124533855264));
#196047=CARTESIAN_POINT('Origin',(116.75121327195,-6.95,49.2078583419757));
#196048=CARTESIAN_POINT('',(116.75121327195,-7.45,49.2078583419757));
#196049=CARTESIAN_POINT('',(116.69397029808,-7.45,49.5023464435054));
#196050=CARTESIAN_POINT('',(116.75121327195,-7.45,49.2078583419757));
#196051=CARTESIAN_POINT('',(116.69397029808,-6.95,49.5023464435054));
#196052=CARTESIAN_POINT('',(116.75121327195,-6.95,49.2078583419757));
#196053=CARTESIAN_POINT('Origin',(116.75121327195,-7.45,49.2078583419757));
#196054=CARTESIAN_POINT('',(116.2603997694,-7.45,49.1124533855264));
#196055=CARTESIAN_POINT('',(116.203156795531,-7.45,49.4069414870561));
#196056=CARTESIAN_POINT('',(116.2603997694,-7.45,49.1124533855264));
#196057=CARTESIAN_POINT('',(116.69397029808,-7.45,49.5023464435054));
#196058=CARTESIAN_POINT('',(116.75121327195,-7.45,49.2078583419757));
#196059=CARTESIAN_POINT('Origin',(116.2603997694,-7.45,49.1124533855264));
#196060=CARTESIAN_POINT('',(116.203156795531,-7.45,49.4069414870561));
#196061=CARTESIAN_POINT('',(116.2603997694,-7.45,49.1124533855264));
#196062=CARTESIAN_POINT('Origin',(117.045701373479,-6.95,49.2651013158452));
#196063=CARTESIAN_POINT('',(117.536514876029,-6.95,49.3605062722945));
#196064=CARTESIAN_POINT('',(117.479271902159,-6.95,49.6549943738242));
#196065=CARTESIAN_POINT('',(117.536514876029,-6.95,49.3605062722945));
#196066=CARTESIAN_POINT('',(116.98845839961,-6.95,49.5595894173749));
#196067=CARTESIAN_POINT('',(116.98845839961,-6.95,49.5595894173749));
#196068=CARTESIAN_POINT('',(117.045701373479,-6.95,49.2651013158452));
#196069=CARTESIAN_POINT('',(117.045701373479,-6.95,49.2651013158452));
#196070=CARTESIAN_POINT('',(117.045701373479,-6.95,49.2651013158452));
#196071=CARTESIAN_POINT('Origin',(117.536514876029,-6.95,49.3605062722945));
#196072=CARTESIAN_POINT('',(117.536514876029,-7.45,49.3605062722945));
#196073=CARTESIAN_POINT('',(117.479271902159,-7.45,49.6549943738242));
#196074=CARTESIAN_POINT('',(117.536514876029,-7.45,49.3605062722945));
#196075=CARTESIAN_POINT('',(117.479271902159,-6.95,49.6549943738242));
#196076=CARTESIAN_POINT('',(117.536514876029,-6.95,49.3605062722945));
#196077=CARTESIAN_POINT('Origin',(117.536514876029,-7.45,49.3605062722945));
#196078=CARTESIAN_POINT('',(117.045701373479,-7.45,49.2651013158452));
#196079=CARTESIAN_POINT('',(116.98845839961,-7.45,49.5595894173749));
#196080=CARTESIAN_POINT('',(117.045701373479,-7.45,49.2651013158452));
#196081=CARTESIAN_POINT('',(117.479271902159,-7.45,49.6549943738242));
#196082=CARTESIAN_POINT('',(117.536514876029,-7.45,49.3605062722945));
#196083=CARTESIAN_POINT('Origin',(117.045701373479,-7.45,49.2651013158452));
#196084=CARTESIAN_POINT('',(116.98845839961,-7.45,49.5595894173749));
#196085=CARTESIAN_POINT('',(117.045701373479,-7.45,49.2651013158452));
#196086=CARTESIAN_POINT('Origin',(117.831002977559,-6.95,49.417749246164));
#196087=CARTESIAN_POINT('',(118.321816480108,-6.95,49.5131542026133));
#196088=CARTESIAN_POINT('',(118.264573506239,-6.95,49.807642304143));
#196089=CARTESIAN_POINT('',(118.321816480108,-6.95,49.5131542026133));
#196090=CARTESIAN_POINT('',(117.773760003689,-6.95,49.7122373476937));
#196091=CARTESIAN_POINT('',(117.773760003689,-6.95,49.7122373476937));
#196092=CARTESIAN_POINT('',(117.831002977559,-6.95,49.417749246164));
#196093=CARTESIAN_POINT('',(117.831002977559,-6.95,49.417749246164));
#196094=CARTESIAN_POINT('',(117.831002977559,-6.95,49.417749246164));
#196095=CARTESIAN_POINT('Origin',(118.321816480108,-6.95,49.5131542026133));
#196096=CARTESIAN_POINT('',(118.321816480108,-7.45,49.5131542026133));
#196097=CARTESIAN_POINT('',(118.264573506239,-7.45,49.807642304143));
#196098=CARTESIAN_POINT('',(118.321816480108,-7.45,49.5131542026133));
#196099=CARTESIAN_POINT('',(118.264573506239,-6.95,49.807642304143));
#196100=CARTESIAN_POINT('',(118.321816480108,-6.95,49.5131542026133));
#196101=CARTESIAN_POINT('Origin',(118.321816480108,-7.45,49.5131542026133));
#196102=CARTESIAN_POINT('',(117.831002977559,-7.45,49.417749246164));
#196103=CARTESIAN_POINT('',(117.773760003689,-7.45,49.7122373476937));
#196104=CARTESIAN_POINT('',(117.831002977559,-7.45,49.417749246164));
#196105=CARTESIAN_POINT('',(118.264573506239,-7.45,49.807642304143));
#196106=CARTESIAN_POINT('',(118.321816480108,-7.45,49.5131542026133));
#196107=CARTESIAN_POINT('Origin',(117.831002977559,-7.45,49.417749246164));
#196108=CARTESIAN_POINT('',(117.773760003689,-7.45,49.7122373476937));
#196109=CARTESIAN_POINT('',(117.831002977559,-7.45,49.417749246164));
#196110=CARTESIAN_POINT('Origin',(118.616304581638,-6.95,49.5703971764828));
#196111=CARTESIAN_POINT('',(119.107118084187,-6.95,49.6658021329321));
#196112=CARTESIAN_POINT('',(119.049875110318,-6.95,49.9602902344618));
#196113=CARTESIAN_POINT('',(119.107118084187,-6.95,49.6658021329321));
#196114=CARTESIAN_POINT('',(118.559061607768,-6.95,49.8648852780125));
#196115=CARTESIAN_POINT('',(118.559061607768,-6.95,49.8648852780125));
#196116=CARTESIAN_POINT('',(118.616304581638,-6.95,49.5703971764828));
#196117=CARTESIAN_POINT('',(118.616304581638,-6.95,49.5703971764828));
#196118=CARTESIAN_POINT('',(118.616304581638,-6.95,49.5703971764828));
#196119=CARTESIAN_POINT('Origin',(119.107118084187,-6.95,49.6658021329321));
#196120=CARTESIAN_POINT('',(119.107118084187,-7.45,49.6658021329321));
#196121=CARTESIAN_POINT('',(119.049875110318,-7.45,49.9602902344618));
#196122=CARTESIAN_POINT('',(119.107118084187,-7.45,49.6658021329321));
#196123=CARTESIAN_POINT('',(119.049875110318,-6.95,49.9602902344618));
#196124=CARTESIAN_POINT('',(119.107118084187,-6.95,49.6658021329321));
#196125=CARTESIAN_POINT('Origin',(119.107118084187,-7.45,49.6658021329321));
#196126=CARTESIAN_POINT('',(118.616304581638,-7.45,49.5703971764828));
#196127=CARTESIAN_POINT('',(118.559061607768,-7.45,49.8648852780125));
#196128=CARTESIAN_POINT('',(118.616304581638,-7.45,49.5703971764828));
#196129=CARTESIAN_POINT('',(119.049875110318,-7.45,49.9602902344618));
#196130=CARTESIAN_POINT('',(119.107118084187,-7.45,49.6658021329321));
#196131=CARTESIAN_POINT('Origin',(118.616304581638,-7.45,49.5703971764828));
#196132=CARTESIAN_POINT('',(118.559061607768,-7.45,49.8648852780125));
#196133=CARTESIAN_POINT('',(118.616304581638,-7.45,49.5703971764828));
#196134=CARTESIAN_POINT('Origin',(119.401606185717,-6.95,49.7230451068016));
#196135=CARTESIAN_POINT('',(119.892419688267,-6.95,49.8184500632509));
#196136=CARTESIAN_POINT('',(119.835176714397,-6.95,50.1129381647806));
#196137=CARTESIAN_POINT('',(119.892419688267,-6.95,49.8184500632509));
#196138=CARTESIAN_POINT('',(119.344363211847,-6.95,50.0175332083313));
#196139=CARTESIAN_POINT('',(119.344363211847,-6.95,50.0175332083313));
#196140=CARTESIAN_POINT('',(119.401606185717,-6.95,49.7230451068016));
#196141=CARTESIAN_POINT('',(119.401606185717,-6.95,49.7230451068016));
#196142=CARTESIAN_POINT('',(119.401606185717,-6.95,49.7230451068016));
#196143=CARTESIAN_POINT('Origin',(119.892419688267,-6.95,49.8184500632509));
#196144=CARTESIAN_POINT('',(119.892419688267,-7.45,49.8184500632509));
#196145=CARTESIAN_POINT('',(119.835176714397,-7.45,50.1129381647806));
#196146=CARTESIAN_POINT('',(119.892419688267,-7.45,49.8184500632509));
#196147=CARTESIAN_POINT('',(119.835176714397,-6.95,50.1129381647806));
#196148=CARTESIAN_POINT('',(119.892419688267,-6.95,49.8184500632509));
#196149=CARTESIAN_POINT('Origin',(119.892419688267,-7.45,49.8184500632509));
#196150=CARTESIAN_POINT('',(119.401606185717,-7.45,49.7230451068016));
#196151=CARTESIAN_POINT('',(119.344363211847,-7.45,50.0175332083313));
#196152=CARTESIAN_POINT('',(119.401606185717,-7.45,49.7230451068016));
#196153=CARTESIAN_POINT('',(119.835176714397,-7.45,50.1129381647806));
#196154=CARTESIAN_POINT('',(119.892419688267,-7.45,49.8184500632509));
#196155=CARTESIAN_POINT('Origin',(119.401606185717,-7.45,49.7230451068016));
#196156=CARTESIAN_POINT('',(119.344363211847,-7.45,50.0175332083313));
#196157=CARTESIAN_POINT('',(119.401606185717,-7.45,49.7230451068016));
#196158=CARTESIAN_POINT('Origin',(120.186907789796,-6.95,49.8756930371204));
#196159=CARTESIAN_POINT('',(120.677721292346,-6.95,49.9710979935697));
#196160=CARTESIAN_POINT('',(120.620478318476,-6.95,50.2655860950994));
#196161=CARTESIAN_POINT('',(120.677721292346,-6.95,49.9710979935697));
#196162=CARTESIAN_POINT('',(120.129664815927,-6.95,50.1701811386501));
#196163=CARTESIAN_POINT('',(120.129664815927,-6.95,50.1701811386501));
#196164=CARTESIAN_POINT('',(120.186907789796,-6.95,49.8756930371204));
#196165=CARTESIAN_POINT('',(120.186907789796,-6.95,49.8756930371204));
#196166=CARTESIAN_POINT('',(120.186907789796,-6.95,49.8756930371204));
#196167=CARTESIAN_POINT('Origin',(120.677721292346,-6.95,49.9710979935697));
#196168=CARTESIAN_POINT('',(120.677721292346,-7.45,49.9710979935697));
#196169=CARTESIAN_POINT('',(120.620478318476,-7.45,50.2655860950994));
#196170=CARTESIAN_POINT('',(120.677721292346,-7.45,49.9710979935697));
#196171=CARTESIAN_POINT('',(120.620478318476,-6.95,50.2655860950994));
#196172=CARTESIAN_POINT('',(120.677721292346,-6.95,49.9710979935697));
#196173=CARTESIAN_POINT('Origin',(120.677721292346,-7.45,49.9710979935697));
#196174=CARTESIAN_POINT('',(120.186907789796,-7.45,49.8756930371204));
#196175=CARTESIAN_POINT('',(120.129664815927,-7.45,50.1701811386501));
#196176=CARTESIAN_POINT('',(120.186907789796,-7.45,49.8756930371204));
#196177=CARTESIAN_POINT('',(120.620478318476,-7.45,50.2655860950994));
#196178=CARTESIAN_POINT('',(120.677721292346,-7.45,49.9710979935697));
#196179=CARTESIAN_POINT('Origin',(120.186907789796,-7.45,49.8756930371204));
#196180=CARTESIAN_POINT('',(120.129664815927,-7.45,50.1701811386501));
#196181=CARTESIAN_POINT('',(120.186907789796,-7.45,49.8756930371204));
#196182=CARTESIAN_POINT('Origin',(120.972209393875,-6.95,50.0283409674392));
#196183=CARTESIAN_POINT('',(121.463022896425,-6.95,50.1237459238885));
#196184=CARTESIAN_POINT('',(121.405779922555,-6.95,50.4182340254182));
#196185=CARTESIAN_POINT('',(121.463022896425,-6.95,50.1237459238885));
#196186=CARTESIAN_POINT('',(120.914966420006,-6.95,50.3228290689689));
#196187=CARTESIAN_POINT('',(120.914966420006,-6.95,50.3228290689689));
#196188=CARTESIAN_POINT('',(120.972209393875,-6.95,50.0283409674392));
#196189=CARTESIAN_POINT('',(120.972209393875,-6.95,50.0283409674392));
#196190=CARTESIAN_POINT('',(120.972209393875,-6.95,50.0283409674392));
#196191=CARTESIAN_POINT('Origin',(121.463022896425,-6.95,50.1237459238885));
#196192=CARTESIAN_POINT('',(121.463022896425,-7.45,50.1237459238885));
#196193=CARTESIAN_POINT('',(121.405779922555,-7.45,50.4182340254182));
#196194=CARTESIAN_POINT('',(121.463022896425,-7.45,50.1237459238885));
#196195=CARTESIAN_POINT('',(121.405779922555,-6.95,50.4182340254182));
#196196=CARTESIAN_POINT('',(121.463022896425,-6.95,50.1237459238885));
#196197=CARTESIAN_POINT('Origin',(121.463022896425,-7.45,50.1237459238885));
#196198=CARTESIAN_POINT('',(120.972209393875,-7.45,50.0283409674392));
#196199=CARTESIAN_POINT('',(120.914966420006,-7.45,50.3228290689689));
#196200=CARTESIAN_POINT('',(120.972209393875,-7.45,50.0283409674392));
#196201=CARTESIAN_POINT('',(121.405779922555,-7.45,50.4182340254182));
#196202=CARTESIAN_POINT('',(121.463022896425,-7.45,50.1237459238885));
#196203=CARTESIAN_POINT('Origin',(120.972209393875,-7.45,50.0283409674392));
#196204=CARTESIAN_POINT('',(120.914966420006,-7.45,50.3228290689689));
#196205=CARTESIAN_POINT('',(120.972209393875,-7.45,50.0283409674392));
#196206=CARTESIAN_POINT('Origin',(121.757510997955,-6.95,50.180988897758));
#196207=CARTESIAN_POINT('',(122.248324500504,-6.95,50.2763938542073));
#196208=CARTESIAN_POINT('',(122.191081526635,-6.95,50.570881955737));
#196209=CARTESIAN_POINT('',(122.248324500504,-6.95,50.2763938542073));
#196210=CARTESIAN_POINT('',(121.700268024085,-6.95,50.4754769992877));
#196211=CARTESIAN_POINT('',(121.700268024085,-6.95,50.4754769992877));
#196212=CARTESIAN_POINT('',(121.757510997955,-6.95,50.180988897758));
#196213=CARTESIAN_POINT('',(121.757510997955,-6.95,50.180988897758));
#196214=CARTESIAN_POINT('',(121.757510997955,-6.95,50.180988897758));
#196215=CARTESIAN_POINT('Origin',(122.248324500504,-6.95,50.2763938542073));
#196216=CARTESIAN_POINT('',(122.248324500504,-7.45,50.2763938542073));
#196217=CARTESIAN_POINT('',(122.191081526635,-7.45,50.570881955737));
#196218=CARTESIAN_POINT('',(122.248324500504,-7.45,50.2763938542073));
#196219=CARTESIAN_POINT('',(122.191081526635,-6.95,50.570881955737));
#196220=CARTESIAN_POINT('',(122.248324500504,-6.95,50.2763938542073));
#196221=CARTESIAN_POINT('Origin',(122.248324500504,-7.45,50.2763938542073));
#196222=CARTESIAN_POINT('',(121.757510997955,-7.45,50.180988897758));
#196223=CARTESIAN_POINT('',(121.700268024085,-7.45,50.4754769992877));
#196224=CARTESIAN_POINT('',(121.757510997955,-7.45,50.180988897758));
#196225=CARTESIAN_POINT('',(122.191081526635,-7.45,50.570881955737));
#196226=CARTESIAN_POINT('',(122.248324500504,-7.45,50.2763938542073));
#196227=CARTESIAN_POINT('Origin',(121.757510997955,-7.45,50.180988897758));
#196228=CARTESIAN_POINT('',(121.700268024085,-7.45,50.4754769992877));
#196229=CARTESIAN_POINT('',(121.757510997955,-7.45,50.180988897758));
#196230=CARTESIAN_POINT('Origin',(122.542812602034,-6.95,50.3336368280768));
#196231=CARTESIAN_POINT('',(123.033626104583,-6.95,50.4290417845261));
#196232=CARTESIAN_POINT('',(122.976383130714,-6.95,50.7235298860558));
#196233=CARTESIAN_POINT('',(123.033626104583,-6.95,50.4290417845261));
#196234=CARTESIAN_POINT('',(122.485569628164,-6.95,50.6281249296065));
#196235=CARTESIAN_POINT('',(122.485569628164,-6.95,50.6281249296065));
#196236=CARTESIAN_POINT('',(122.542812602034,-6.95,50.3336368280768));
#196237=CARTESIAN_POINT('',(122.542812602034,-6.95,50.3336368280768));
#196238=CARTESIAN_POINT('',(122.542812602034,-6.95,50.3336368280768));
#196239=CARTESIAN_POINT('Origin',(123.033626104583,-6.95,50.4290417845261));
#196240=CARTESIAN_POINT('',(123.033626104583,-7.45,50.4290417845261));
#196241=CARTESIAN_POINT('',(122.976383130714,-7.45,50.7235298860558));
#196242=CARTESIAN_POINT('',(123.033626104583,-7.45,50.4290417845261));
#196243=CARTESIAN_POINT('',(122.976383130714,-6.95,50.7235298860558));
#196244=CARTESIAN_POINT('',(123.033626104583,-6.95,50.4290417845261));
#196245=CARTESIAN_POINT('Origin',(123.033626104583,-7.45,50.4290417845261));
#196246=CARTESIAN_POINT('',(122.542812602034,-7.45,50.3336368280768));
#196247=CARTESIAN_POINT('',(122.485569628164,-7.45,50.6281249296065));
#196248=CARTESIAN_POINT('',(122.542812602034,-7.45,50.3336368280768));
#196249=CARTESIAN_POINT('',(122.976383130714,-7.45,50.7235298860558));
#196250=CARTESIAN_POINT('',(123.033626104583,-7.45,50.4290417845261));
#196251=CARTESIAN_POINT('Origin',(122.542812602034,-7.45,50.3336368280768));
#196252=CARTESIAN_POINT('',(122.485569628164,-7.45,50.6281249296065));
#196253=CARTESIAN_POINT('',(122.542812602034,-7.45,50.3336368280768));
#196254=CARTESIAN_POINT('Origin',(124.113415810192,-5.35,50.6389326887144));
#196255=CARTESIAN_POINT('',(124.604229312742,-5.35,50.7343376451637));
#196256=CARTESIAN_POINT('',(124.546986338872,-5.35,51.0288257466934));
#196257=CARTESIAN_POINT('',(124.604229312742,-5.35,50.7343376451637));
#196258=CARTESIAN_POINT('',(124.056172836323,-5.35,50.9334207902441));
#196259=CARTESIAN_POINT('',(124.056172836323,-5.35,50.9334207902441));
#196260=CARTESIAN_POINT('',(124.113415810192,-5.35,50.6389326887144));
#196261=CARTESIAN_POINT('',(124.113415810192,-5.35,50.6389326887144));
#196262=CARTESIAN_POINT('',(124.113415810192,-5.35,50.6389326887144));
#196263=CARTESIAN_POINT('Origin',(124.604229312742,-5.35,50.7343376451637));
#196264=CARTESIAN_POINT('',(124.604229312742,-5.85,50.7343376451637));
#196265=CARTESIAN_POINT('',(124.546986338872,-5.85,51.0288257466934));
#196266=CARTESIAN_POINT('',(124.604229312742,-5.85,50.7343376451637));
#196267=CARTESIAN_POINT('',(124.546986338872,-5.35,51.0288257466934));
#196268=CARTESIAN_POINT('',(124.604229312742,-5.35,50.7343376451637));
#196269=CARTESIAN_POINT('Origin',(124.604229312742,-5.85,50.7343376451637));
#196270=CARTESIAN_POINT('',(124.113415810192,-5.85,50.6389326887144));
#196271=CARTESIAN_POINT('',(124.056172836323,-5.85,50.9334207902441));
#196272=CARTESIAN_POINT('',(124.113415810192,-5.85,50.6389326887144));
#196273=CARTESIAN_POINT('',(124.546986338872,-5.85,51.0288257466934));
#196274=CARTESIAN_POINT('',(124.604229312742,-5.85,50.7343376451637));
#196275=CARTESIAN_POINT('Origin',(124.113415810192,-5.85,50.6389326887144));
#196276=CARTESIAN_POINT('',(124.056172836323,-5.85,50.9334207902441));
#196277=CARTESIAN_POINT('',(124.113415810192,-5.85,50.6389326887144));
#196278=CARTESIAN_POINT('Origin',(124.113415810192,-4.55,50.6389326887144));
#196279=CARTESIAN_POINT('',(124.604229312742,-4.55,50.7343376451637));
#196280=CARTESIAN_POINT('',(124.546986338872,-4.55,51.0288257466934));
#196281=CARTESIAN_POINT('',(124.604229312742,-4.55,50.7343376451637));
#196282=CARTESIAN_POINT('',(124.056172836323,-4.55,50.9334207902441));
#196283=CARTESIAN_POINT('',(124.056172836323,-4.55,50.9334207902441));
#196284=CARTESIAN_POINT('',(124.113415810192,-4.55,50.6389326887144));
#196285=CARTESIAN_POINT('',(124.113415810192,-4.55,50.6389326887144));
#196286=CARTESIAN_POINT('',(124.113415810192,-4.55,50.6389326887144));
#196287=CARTESIAN_POINT('Origin',(124.604229312742,-4.55,50.7343376451637));
#196288=CARTESIAN_POINT('',(124.604229312742,-5.05,50.7343376451637));
#196289=CARTESIAN_POINT('',(124.546986338872,-5.05,51.0288257466934));
#196290=CARTESIAN_POINT('',(124.604229312742,-5.05,50.7343376451637));
#196291=CARTESIAN_POINT('',(124.546986338872,-4.55,51.0288257466934));
#196292=CARTESIAN_POINT('',(124.604229312742,-4.55,50.7343376451637));
#196293=CARTESIAN_POINT('Origin',(124.604229312742,-5.05,50.7343376451637));
#196294=CARTESIAN_POINT('',(124.113415810192,-5.05,50.6389326887144));
#196295=CARTESIAN_POINT('',(124.056172836323,-5.05,50.9334207902441));
#196296=CARTESIAN_POINT('',(124.113415810192,-5.05,50.6389326887144));
#196297=CARTESIAN_POINT('',(124.546986338872,-5.05,51.0288257466934));
#196298=CARTESIAN_POINT('',(124.604229312742,-5.05,50.7343376451637));
#196299=CARTESIAN_POINT('Origin',(124.113415810192,-5.05,50.6389326887144));
#196300=CARTESIAN_POINT('',(124.056172836323,-5.05,50.9334207902441));
#196301=CARTESIAN_POINT('',(124.113415810192,-5.05,50.6389326887144));
#196302=CARTESIAN_POINT('Origin',(124.113415810192,-3.75,50.6389326887144));
#196303=CARTESIAN_POINT('',(124.604229312742,-3.75,50.7343376451637));
#196304=CARTESIAN_POINT('',(124.546986338872,-3.75,51.0288257466934));
#196305=CARTESIAN_POINT('',(124.604229312742,-3.75,50.7343376451637));
#196306=CARTESIAN_POINT('',(124.056172836323,-3.75,50.9334207902441));
#196307=CARTESIAN_POINT('',(124.056172836323,-3.75,50.9334207902441));
#196308=CARTESIAN_POINT('',(124.113415810192,-3.75,50.6389326887144));
#196309=CARTESIAN_POINT('',(124.113415810192,-3.75,50.6389326887144));
#196310=CARTESIAN_POINT('',(124.113415810192,-3.75,50.6389326887144));
#196311=CARTESIAN_POINT('Origin',(124.604229312742,-3.75,50.7343376451637));
#196312=CARTESIAN_POINT('',(124.604229312742,-4.25,50.7343376451637));
#196313=CARTESIAN_POINT('',(124.546986338872,-4.25,51.0288257466934));
#196314=CARTESIAN_POINT('',(124.604229312742,-4.25,50.7343376451637));
#196315=CARTESIAN_POINT('',(124.546986338872,-3.75,51.0288257466934));
#196316=CARTESIAN_POINT('',(124.604229312742,-3.75,50.7343376451637));
#196317=CARTESIAN_POINT('Origin',(124.604229312742,-4.25,50.7343376451637));
#196318=CARTESIAN_POINT('',(124.113415810192,-4.25,50.6389326887144));
#196319=CARTESIAN_POINT('',(124.056172836323,-4.25,50.9334207902441));
#196320=CARTESIAN_POINT('',(124.113415810192,-4.25,50.6389326887144));
#196321=CARTESIAN_POINT('',(124.546986338872,-4.25,51.0288257466934));
#196322=CARTESIAN_POINT('',(124.604229312742,-4.25,50.7343376451637));
#196323=CARTESIAN_POINT('Origin',(124.113415810192,-4.25,50.6389326887144));
#196324=CARTESIAN_POINT('',(124.056172836323,-4.25,50.9334207902441));
#196325=CARTESIAN_POINT('',(124.113415810192,-4.25,50.6389326887144));
#196326=CARTESIAN_POINT('Origin',(124.113415810192,-2.95,50.6389326887144));
#196327=CARTESIAN_POINT('',(124.604229312742,-2.95,50.7343376451637));
#196328=CARTESIAN_POINT('',(124.546986338872,-2.95,51.0288257466934));
#196329=CARTESIAN_POINT('',(124.604229312742,-2.95,50.7343376451637));
#196330=CARTESIAN_POINT('',(124.056172836323,-2.95,50.9334207902441));
#196331=CARTESIAN_POINT('',(124.056172836323,-2.95,50.9334207902441));
#196332=CARTESIAN_POINT('',(124.113415810192,-2.95,50.6389326887144));
#196333=CARTESIAN_POINT('',(124.113415810192,-2.95,50.6389326887144));
#196334=CARTESIAN_POINT('',(124.113415810192,-2.95,50.6389326887144));
#196335=CARTESIAN_POINT('Origin',(124.604229312742,-2.95,50.7343376451637));
#196336=CARTESIAN_POINT('',(124.604229312742,-3.45,50.7343376451637));
#196337=CARTESIAN_POINT('',(124.546986338872,-3.45,51.0288257466934));
#196338=CARTESIAN_POINT('',(124.604229312742,-3.45,50.7343376451637));
#196339=CARTESIAN_POINT('',(124.546986338872,-2.95,51.0288257466934));
#196340=CARTESIAN_POINT('',(124.604229312742,-2.95,50.7343376451637));
#196341=CARTESIAN_POINT('Origin',(124.604229312742,-3.45,50.7343376451637));
#196342=CARTESIAN_POINT('',(124.113415810192,-3.45,50.6389326887144));
#196343=CARTESIAN_POINT('',(124.056172836323,-3.45,50.9334207902441));
#196344=CARTESIAN_POINT('',(124.113415810192,-3.45,50.6389326887144));
#196345=CARTESIAN_POINT('',(124.546986338872,-3.45,51.0288257466934));
#196346=CARTESIAN_POINT('',(124.604229312742,-3.45,50.7343376451637));
#196347=CARTESIAN_POINT('Origin',(124.113415810192,-3.45,50.6389326887144));
#196348=CARTESIAN_POINT('',(124.056172836323,-3.45,50.9334207902441));
#196349=CARTESIAN_POINT('',(124.113415810192,-3.45,50.6389326887144));
#196350=CARTESIAN_POINT('Origin',(124.113415810192,-2.15,50.6389326887144));
#196351=CARTESIAN_POINT('',(124.604229312742,-2.15,50.7343376451637));
#196352=CARTESIAN_POINT('',(124.546986338872,-2.15,51.0288257466934));
#196353=CARTESIAN_POINT('',(124.604229312742,-2.15,50.7343376451637));
#196354=CARTESIAN_POINT('',(124.056172836323,-2.15,50.9334207902441));
#196355=CARTESIAN_POINT('',(124.056172836323,-2.15,50.9334207902441));
#196356=CARTESIAN_POINT('',(124.113415810192,-2.15,50.6389326887144));
#196357=CARTESIAN_POINT('',(124.113415810192,-2.15,50.6389326887144));
#196358=CARTESIAN_POINT('',(124.113415810192,-2.15,50.6389326887144));
#196359=CARTESIAN_POINT('Origin',(124.604229312742,-2.15,50.7343376451637));
#196360=CARTESIAN_POINT('',(124.604229312742,-2.65,50.7343376451637));
#196361=CARTESIAN_POINT('',(124.546986338872,-2.65,51.0288257466934));
#196362=CARTESIAN_POINT('',(124.604229312742,-2.65,50.7343376451637));
#196363=CARTESIAN_POINT('',(124.546986338872,-2.15,51.0288257466934));
#196364=CARTESIAN_POINT('',(124.604229312742,-2.15,50.7343376451637));
#196365=CARTESIAN_POINT('Origin',(124.604229312742,-2.65,50.7343376451637));
#196366=CARTESIAN_POINT('',(124.113415810192,-2.65,50.6389326887144));
#196367=CARTESIAN_POINT('',(124.056172836323,-2.65,50.9334207902441));
#196368=CARTESIAN_POINT('',(124.113415810192,-2.65,50.6389326887144));
#196369=CARTESIAN_POINT('',(124.546986338872,-2.65,51.0288257466934));
#196370=CARTESIAN_POINT('',(124.604229312742,-2.65,50.7343376451637));
#196371=CARTESIAN_POINT('Origin',(124.113415810192,-2.65,50.6389326887144));
#196372=CARTESIAN_POINT('',(124.056172836323,-2.65,50.9334207902441));
#196373=CARTESIAN_POINT('',(124.113415810192,-2.65,50.6389326887144));
#196374=CARTESIAN_POINT('Origin',(124.113415810192,-1.35,50.6389326887144));
#196375=CARTESIAN_POINT('',(124.604229312742,-1.35,50.7343376451637));
#196376=CARTESIAN_POINT('',(124.546986338872,-1.35,51.0288257466934));
#196377=CARTESIAN_POINT('',(124.604229312742,-1.35,50.7343376451637));
#196378=CARTESIAN_POINT('',(124.056172836323,-1.35,50.9334207902441));
#196379=CARTESIAN_POINT('',(124.056172836323,-1.35,50.9334207902441));
#196380=CARTESIAN_POINT('',(124.113415810192,-1.35,50.6389326887144));
#196381=CARTESIAN_POINT('',(124.113415810192,-1.35,50.6389326887144));
#196382=CARTESIAN_POINT('',(124.113415810192,-1.35,50.6389326887144));
#196383=CARTESIAN_POINT('Origin',(124.604229312742,-1.35,50.7343376451637));
#196384=CARTESIAN_POINT('',(124.604229312742,-1.85,50.7343376451637));
#196385=CARTESIAN_POINT('',(124.546986338872,-1.85,51.0288257466934));
#196386=CARTESIAN_POINT('',(124.604229312742,-1.85,50.7343376451637));
#196387=CARTESIAN_POINT('',(124.546986338872,-1.35,51.0288257466934));
#196388=CARTESIAN_POINT('',(124.604229312742,-1.35,50.7343376451637));
#196389=CARTESIAN_POINT('Origin',(124.604229312742,-1.85,50.7343376451637));
#196390=CARTESIAN_POINT('',(124.113415810192,-1.85,50.6389326887144));
#196391=CARTESIAN_POINT('',(124.056172836323,-1.85,50.9334207902441));
#196392=CARTESIAN_POINT('',(124.113415810192,-1.85,50.6389326887144));
#196393=CARTESIAN_POINT('',(124.546986338872,-1.85,51.0288257466934));
#196394=CARTESIAN_POINT('',(124.604229312742,-1.85,50.7343376451637));
#196395=CARTESIAN_POINT('Origin',(124.113415810192,-1.85,50.6389326887144));
#196396=CARTESIAN_POINT('',(124.056172836323,-1.85,50.9334207902441));
#196397=CARTESIAN_POINT('',(124.113415810192,-1.85,50.6389326887144));
#196398=CARTESIAN_POINT('Origin',(124.113415810192,-0.549999999999986,50.6389326887144));
#196399=CARTESIAN_POINT('',(124.604229312742,-0.549999999999986,50.7343376451637));
#196400=CARTESIAN_POINT('',(124.546986338872,-0.549999999999986,51.0288257466934));
#196401=CARTESIAN_POINT('',(124.604229312742,-0.549999999999986,50.7343376451637));
#196402=CARTESIAN_POINT('',(124.056172836323,-0.549999999999986,50.9334207902441));
#196403=CARTESIAN_POINT('',(124.056172836323,-0.549999999999986,50.9334207902441));
#196404=CARTESIAN_POINT('',(124.113415810192,-0.549999999999986,50.6389326887144));
#196405=CARTESIAN_POINT('',(124.113415810192,-0.549999999999986,50.6389326887144));
#196406=CARTESIAN_POINT('',(124.113415810192,-0.549999999999986,50.6389326887144));
#196407=CARTESIAN_POINT('Origin',(124.604229312742,-0.549999999999986,50.7343376451637));
#196408=CARTESIAN_POINT('',(124.604229312742,-1.05,50.7343376451637));
#196409=CARTESIAN_POINT('',(124.546986338872,-1.05,51.0288257466934));
#196410=CARTESIAN_POINT('',(124.604229312742,-1.05,50.7343376451637));
#196411=CARTESIAN_POINT('',(124.546986338872,-0.549999999999986,51.0288257466934));
#196412=CARTESIAN_POINT('',(124.604229312742,-0.549999999999986,50.7343376451637));
#196413=CARTESIAN_POINT('Origin',(124.604229312742,-1.05,50.7343376451637));
#196414=CARTESIAN_POINT('',(124.113415810192,-1.05,50.6389326887144));
#196415=CARTESIAN_POINT('',(124.056172836323,-1.05,50.9334207902441));
#196416=CARTESIAN_POINT('',(124.113415810192,-1.05,50.6389326887144));
#196417=CARTESIAN_POINT('',(124.546986338872,-1.05,51.0288257466934));
#196418=CARTESIAN_POINT('',(124.604229312742,-1.05,50.7343376451637));
#196419=CARTESIAN_POINT('Origin',(124.113415810192,-1.05,50.6389326887144));
#196420=CARTESIAN_POINT('',(124.056172836323,-1.05,50.9334207902441));
#196421=CARTESIAN_POINT('',(124.113415810192,-1.05,50.6389326887144));
#196422=CARTESIAN_POINT('Origin',(124.113415810192,0.250000000000015,50.6389326887144));
#196423=CARTESIAN_POINT('',(124.604229312742,0.250000000000015,50.7343376451637));
#196424=CARTESIAN_POINT('',(124.546986338872,0.250000000000015,51.0288257466934));
#196425=CARTESIAN_POINT('',(124.604229312742,0.250000000000015,50.7343376451637));
#196426=CARTESIAN_POINT('',(124.056172836323,0.250000000000015,50.9334207902441));
#196427=CARTESIAN_POINT('',(124.056172836323,0.250000000000015,50.9334207902441));
#196428=CARTESIAN_POINT('',(124.113415810192,0.250000000000015,50.6389326887144));
#196429=CARTESIAN_POINT('',(124.113415810192,0.250000000000015,50.6389326887144));
#196430=CARTESIAN_POINT('',(124.113415810192,0.250000000000015,50.6389326887144));
#196431=CARTESIAN_POINT('Origin',(124.604229312742,0.250000000000015,50.7343376451637));
#196432=CARTESIAN_POINT('',(124.604229312742,-0.249999999999985,50.7343376451637));
#196433=CARTESIAN_POINT('',(124.546986338872,-0.249999999999985,51.0288257466934));
#196434=CARTESIAN_POINT('',(124.604229312742,-0.249999999999985,50.7343376451637));
#196435=CARTESIAN_POINT('',(124.546986338872,0.250000000000015,51.0288257466934));
#196436=CARTESIAN_POINT('',(124.604229312742,0.250000000000015,50.7343376451637));
#196437=CARTESIAN_POINT('Origin',(124.604229312742,-0.249999999999985,50.7343376451637));
#196438=CARTESIAN_POINT('',(124.113415810192,-0.249999999999985,50.6389326887144));
#196439=CARTESIAN_POINT('',(124.056172836323,-0.249999999999985,50.9334207902441));
#196440=CARTESIAN_POINT('',(124.113415810192,-0.249999999999985,50.6389326887144));
#196441=CARTESIAN_POINT('',(124.546986338872,-0.249999999999985,51.0288257466934));
#196442=CARTESIAN_POINT('',(124.604229312742,-0.249999999999985,50.7343376451637));
#196443=CARTESIAN_POINT('Origin',(124.113415810192,-0.249999999999985,50.6389326887144));
#196444=CARTESIAN_POINT('',(124.056172836323,-0.249999999999985,50.9334207902441));
#196445=CARTESIAN_POINT('',(124.113415810192,-0.249999999999985,50.6389326887144));
#196446=CARTESIAN_POINT('Origin',(124.113415810192,1.05,50.6389326887144));
#196447=CARTESIAN_POINT('',(124.604229312742,1.05,50.7343376451637));
#196448=CARTESIAN_POINT('',(124.546986338872,1.05,51.0288257466934));
#196449=CARTESIAN_POINT('',(124.604229312742,1.05,50.7343376451637));
#196450=CARTESIAN_POINT('',(124.056172836323,1.05,50.9334207902441));
#196451=CARTESIAN_POINT('',(124.056172836323,1.05,50.9334207902441));
#196452=CARTESIAN_POINT('',(124.113415810192,1.05,50.6389326887144));
#196453=CARTESIAN_POINT('',(124.113415810192,1.05,50.6389326887144));
#196454=CARTESIAN_POINT('',(124.113415810192,1.05,50.6389326887144));
#196455=CARTESIAN_POINT('Origin',(124.604229312742,1.05,50.7343376451637));
#196456=CARTESIAN_POINT('',(124.604229312742,0.550000000000015,50.7343376451637));
#196457=CARTESIAN_POINT('',(124.546986338872,0.550000000000015,51.0288257466934));
#196458=CARTESIAN_POINT('',(124.604229312742,0.550000000000015,50.7343376451637));
#196459=CARTESIAN_POINT('',(124.546986338872,1.05,51.0288257466934));
#196460=CARTESIAN_POINT('',(124.604229312742,1.05,50.7343376451637));
#196461=CARTESIAN_POINT('Origin',(124.604229312742,0.550000000000015,50.7343376451637));
#196462=CARTESIAN_POINT('',(124.113415810192,0.550000000000015,50.6389326887144));
#196463=CARTESIAN_POINT('',(124.056172836323,0.550000000000015,50.9334207902441));
#196464=CARTESIAN_POINT('',(124.113415810192,0.550000000000015,50.6389326887144));
#196465=CARTESIAN_POINT('',(124.546986338872,0.550000000000015,51.0288257466934));
#196466=CARTESIAN_POINT('',(124.604229312742,0.550000000000015,50.7343376451637));
#196467=CARTESIAN_POINT('Origin',(124.113415810192,0.550000000000015,50.6389326887144));
#196468=CARTESIAN_POINT('',(124.056172836323,0.550000000000015,50.9334207902441));
#196469=CARTESIAN_POINT('',(124.113415810192,0.550000000000015,50.6389326887144));
#196470=CARTESIAN_POINT('Origin',(124.113415810192,1.85,50.6389326887144));
#196471=CARTESIAN_POINT('',(124.604229312742,1.85,50.7343376451637));
#196472=CARTESIAN_POINT('',(124.546986338872,1.85,51.0288257466934));
#196473=CARTESIAN_POINT('',(124.604229312742,1.85,50.7343376451637));
#196474=CARTESIAN_POINT('',(124.056172836323,1.85,50.9334207902441));
#196475=CARTESIAN_POINT('',(124.056172836323,1.85,50.9334207902441));
#196476=CARTESIAN_POINT('',(124.113415810192,1.85,50.6389326887144));
#196477=CARTESIAN_POINT('',(124.113415810192,1.85,50.6389326887144));
#196478=CARTESIAN_POINT('',(124.113415810192,1.85,50.6389326887144));
#196479=CARTESIAN_POINT('Origin',(124.604229312742,1.85,50.7343376451637));
#196480=CARTESIAN_POINT('',(124.604229312742,1.35,50.7343376451637));
#196481=CARTESIAN_POINT('',(124.546986338872,1.35,51.0288257466934));
#196482=CARTESIAN_POINT('',(124.604229312742,1.35,50.7343376451637));
#196483=CARTESIAN_POINT('',(124.546986338872,1.85,51.0288257466934));
#196484=CARTESIAN_POINT('',(124.604229312742,1.85,50.7343376451637));
#196485=CARTESIAN_POINT('Origin',(124.604229312742,1.35,50.7343376451637));
#196486=CARTESIAN_POINT('',(124.113415810192,1.35,50.6389326887144));
#196487=CARTESIAN_POINT('',(124.056172836323,1.35,50.9334207902441));
#196488=CARTESIAN_POINT('',(124.113415810192,1.35,50.6389326887144));
#196489=CARTESIAN_POINT('',(124.546986338872,1.35,51.0288257466934));
#196490=CARTESIAN_POINT('',(124.604229312742,1.35,50.7343376451637));
#196491=CARTESIAN_POINT('Origin',(124.113415810192,1.35,50.6389326887144));
#196492=CARTESIAN_POINT('',(124.056172836323,1.35,50.9334207902441));
#196493=CARTESIAN_POINT('',(124.113415810192,1.35,50.6389326887144));
#196494=CARTESIAN_POINT('Origin',(124.113415810192,2.65,50.6389326887144));
#196495=CARTESIAN_POINT('',(124.604229312742,2.65,50.7343376451637));
#196496=CARTESIAN_POINT('',(124.546986338872,2.65,51.0288257466934));
#196497=CARTESIAN_POINT('',(124.604229312742,2.65,50.7343376451637));
#196498=CARTESIAN_POINT('',(124.056172836323,2.65,50.9334207902441));
#196499=CARTESIAN_POINT('',(124.056172836323,2.65,50.9334207902441));
#196500=CARTESIAN_POINT('',(124.113415810192,2.65,50.6389326887144));
#196501=CARTESIAN_POINT('',(124.113415810192,2.65,50.6389326887144));
#196502=CARTESIAN_POINT('',(124.113415810192,2.65,50.6389326887144));
#196503=CARTESIAN_POINT('Origin',(124.604229312742,2.65,50.7343376451637));
#196504=CARTESIAN_POINT('',(124.604229312742,2.15,50.7343376451637));
#196505=CARTESIAN_POINT('',(124.546986338872,2.15,51.0288257466934));
#196506=CARTESIAN_POINT('',(124.604229312742,2.15,50.7343376451637));
#196507=CARTESIAN_POINT('',(124.546986338872,2.65,51.0288257466934));
#196508=CARTESIAN_POINT('',(124.604229312742,2.65,50.7343376451637));
#196509=CARTESIAN_POINT('Origin',(124.604229312742,2.15,50.7343376451637));
#196510=CARTESIAN_POINT('',(124.113415810192,2.15,50.6389326887144));
#196511=CARTESIAN_POINT('',(124.056172836323,2.15,50.9334207902441));
#196512=CARTESIAN_POINT('',(124.113415810192,2.15,50.6389326887144));
#196513=CARTESIAN_POINT('',(124.546986338872,2.15,51.0288257466934));
#196514=CARTESIAN_POINT('',(124.604229312742,2.15,50.7343376451637));
#196515=CARTESIAN_POINT('Origin',(124.113415810192,2.15,50.6389326887144));
#196516=CARTESIAN_POINT('',(124.056172836323,2.15,50.9334207902441));
#196517=CARTESIAN_POINT('',(124.113415810192,2.15,50.6389326887144));
#196518=CARTESIAN_POINT('Origin',(124.113415810192,3.45,50.6389326887144));
#196519=CARTESIAN_POINT('',(124.604229312742,3.45,50.7343376451637));
#196520=CARTESIAN_POINT('',(124.546986338872,3.45,51.0288257466934));
#196521=CARTESIAN_POINT('',(124.604229312742,3.45,50.7343376451637));
#196522=CARTESIAN_POINT('',(124.056172836323,3.45,50.9334207902441));
#196523=CARTESIAN_POINT('',(124.056172836323,3.45,50.9334207902441));
#196524=CARTESIAN_POINT('',(124.113415810192,3.45,50.6389326887144));
#196525=CARTESIAN_POINT('',(124.113415810192,3.45,50.6389326887144));
#196526=CARTESIAN_POINT('',(124.113415810192,3.45,50.6389326887144));
#196527=CARTESIAN_POINT('Origin',(124.604229312742,3.45,50.7343376451637));
#196528=CARTESIAN_POINT('',(124.604229312742,2.95,50.7343376451637));
#196529=CARTESIAN_POINT('',(124.546986338872,2.95,51.0288257466934));
#196530=CARTESIAN_POINT('',(124.604229312742,2.95,50.7343376451637));
#196531=CARTESIAN_POINT('',(124.546986338872,3.45,51.0288257466934));
#196532=CARTESIAN_POINT('',(124.604229312742,3.45,50.7343376451637));
#196533=CARTESIAN_POINT('Origin',(124.604229312742,2.95,50.7343376451637));
#196534=CARTESIAN_POINT('',(124.113415810192,2.95,50.6389326887144));
#196535=CARTESIAN_POINT('',(124.056172836323,2.95,50.9334207902441));
#196536=CARTESIAN_POINT('',(124.113415810192,2.95,50.6389326887144));
#196537=CARTESIAN_POINT('',(124.546986338872,2.95,51.0288257466934));
#196538=CARTESIAN_POINT('',(124.604229312742,2.95,50.7343376451637));
#196539=CARTESIAN_POINT('Origin',(124.113415810192,2.95,50.6389326887144));
#196540=CARTESIAN_POINT('',(124.056172836323,2.95,50.9334207902441));
#196541=CARTESIAN_POINT('',(124.113415810192,2.95,50.6389326887144));
#196542=CARTESIAN_POINT('Origin',(124.113415810192,4.25,50.6389326887144));
#196543=CARTESIAN_POINT('',(124.604229312742,4.25,50.7343376451637));
#196544=CARTESIAN_POINT('',(124.546986338872,4.25,51.0288257466934));
#196545=CARTESIAN_POINT('',(124.604229312742,4.25,50.7343376451637));
#196546=CARTESIAN_POINT('',(124.056172836323,4.25,50.9334207902441));
#196547=CARTESIAN_POINT('',(124.056172836323,4.25,50.9334207902441));
#196548=CARTESIAN_POINT('',(124.113415810192,4.25,50.6389326887144));
#196549=CARTESIAN_POINT('',(124.113415810192,4.25,50.6389326887144));
#196550=CARTESIAN_POINT('',(124.113415810192,4.25,50.6389326887144));
#196551=CARTESIAN_POINT('Origin',(124.604229312742,4.25,50.7343376451637));
#196552=CARTESIAN_POINT('',(124.604229312742,3.75,50.7343376451637));
#196553=CARTESIAN_POINT('',(124.546986338872,3.75,51.0288257466934));
#196554=CARTESIAN_POINT('',(124.604229312742,3.75,50.7343376451637));
#196555=CARTESIAN_POINT('',(124.546986338872,4.25,51.0288257466934));
#196556=CARTESIAN_POINT('',(124.604229312742,4.25,50.7343376451637));
#196557=CARTESIAN_POINT('Origin',(124.604229312742,3.75,50.7343376451637));
#196558=CARTESIAN_POINT('',(124.113415810192,3.75,50.6389326887144));
#196559=CARTESIAN_POINT('',(124.056172836323,3.75,50.9334207902441));
#196560=CARTESIAN_POINT('',(124.113415810192,3.75,50.6389326887144));
#196561=CARTESIAN_POINT('',(124.546986338872,3.75,51.0288257466934));
#196562=CARTESIAN_POINT('',(124.604229312742,3.75,50.7343376451637));
#196563=CARTESIAN_POINT('Origin',(124.113415810192,3.75,50.6389326887144));
#196564=CARTESIAN_POINT('',(124.056172836323,3.75,50.9334207902441));
#196565=CARTESIAN_POINT('',(124.113415810192,3.75,50.6389326887144));
#196566=CARTESIAN_POINT('Origin',(124.113415810192,5.05,50.6389326887144));
#196567=CARTESIAN_POINT('',(124.604229312742,5.05,50.7343376451637));
#196568=CARTESIAN_POINT('',(124.546986338872,5.05,51.0288257466934));
#196569=CARTESIAN_POINT('',(124.604229312742,5.05,50.7343376451637));
#196570=CARTESIAN_POINT('',(124.056172836323,5.05,50.9334207902441));
#196571=CARTESIAN_POINT('',(124.056172836323,5.05,50.9334207902441));
#196572=CARTESIAN_POINT('',(124.113415810192,5.05,50.6389326887144));
#196573=CARTESIAN_POINT('',(124.113415810192,5.05,50.6389326887144));
#196574=CARTESIAN_POINT('',(124.113415810192,5.05,50.6389326887144));
#196575=CARTESIAN_POINT('Origin',(124.604229312742,5.05,50.7343376451637));
#196576=CARTESIAN_POINT('',(124.604229312742,4.55,50.7343376451637));
#196577=CARTESIAN_POINT('',(124.546986338872,4.55,51.0288257466934));
#196578=CARTESIAN_POINT('',(124.604229312742,4.55,50.7343376451637));
#196579=CARTESIAN_POINT('',(124.546986338872,5.05,51.0288257466934));
#196580=CARTESIAN_POINT('',(124.604229312742,5.05,50.7343376451637));
#196581=CARTESIAN_POINT('Origin',(124.604229312742,4.55,50.7343376451637));
#196582=CARTESIAN_POINT('',(124.113415810192,4.55,50.6389326887144));
#196583=CARTESIAN_POINT('',(124.056172836323,4.55,50.9334207902441));
#196584=CARTESIAN_POINT('',(124.113415810192,4.55,50.6389326887144));
#196585=CARTESIAN_POINT('',(124.546986338872,4.55,51.0288257466934));
#196586=CARTESIAN_POINT('',(124.604229312742,4.55,50.7343376451637));
#196587=CARTESIAN_POINT('Origin',(124.113415810192,4.55,50.6389326887144));
#196588=CARTESIAN_POINT('',(124.056172836323,4.55,50.9334207902441));
#196589=CARTESIAN_POINT('',(124.113415810192,4.55,50.6389326887144));
#196590=CARTESIAN_POINT('Origin',(124.113415810192,5.85,50.6389326887144));
#196591=CARTESIAN_POINT('',(124.604229312742,5.85,50.7343376451637));
#196592=CARTESIAN_POINT('',(124.546986338872,5.85,51.0288257466934));
#196593=CARTESIAN_POINT('',(124.604229312742,5.85,50.7343376451637));
#196594=CARTESIAN_POINT('',(124.056172836323,5.85,50.9334207902441));
#196595=CARTESIAN_POINT('',(124.056172836323,5.85,50.9334207902441));
#196596=CARTESIAN_POINT('',(124.113415810192,5.85,50.6389326887144));
#196597=CARTESIAN_POINT('',(124.113415810192,5.85,50.6389326887144));
#196598=CARTESIAN_POINT('',(124.113415810192,5.85,50.6389326887144));
#196599=CARTESIAN_POINT('Origin',(124.604229312742,5.85,50.7343376451637));
#196600=CARTESIAN_POINT('',(124.604229312742,5.35,50.7343376451637));
#196601=CARTESIAN_POINT('',(124.546986338872,5.35,51.0288257466934));
#196602=CARTESIAN_POINT('',(124.604229312742,5.35,50.7343376451637));
#196603=CARTESIAN_POINT('',(124.546986338872,5.85,51.0288257466934));
#196604=CARTESIAN_POINT('',(124.604229312742,5.85,50.7343376451637));
#196605=CARTESIAN_POINT('Origin',(124.604229312742,5.35,50.7343376451637));
#196606=CARTESIAN_POINT('',(124.113415810192,5.35,50.6389326887144));
#196607=CARTESIAN_POINT('',(124.056172836323,5.35,50.9334207902441));
#196608=CARTESIAN_POINT('',(124.113415810192,5.35,50.6389326887144));
#196609=CARTESIAN_POINT('',(124.546986338872,5.35,51.0288257466934));
#196610=CARTESIAN_POINT('',(124.604229312742,5.35,50.7343376451637));
#196611=CARTESIAN_POINT('Origin',(124.113415810192,5.35,50.6389326887144));
#196612=CARTESIAN_POINT('',(124.056172836323,5.35,50.9334207902441));
#196613=CARTESIAN_POINT('',(124.113415810192,5.35,50.6389326887144));
#196614=CARTESIAN_POINT('Origin',(122.542812602034,7.45,50.3336368280768));
#196615=CARTESIAN_POINT('',(123.033626104583,7.45,50.4290417845261));
#196616=CARTESIAN_POINT('',(122.976383130714,7.45,50.7235298860558));
#196617=CARTESIAN_POINT('',(123.033626104583,7.45,50.4290417845261));
#196618=CARTESIAN_POINT('',(122.485569628164,7.45,50.6281249296065));
#196619=CARTESIAN_POINT('',(122.485569628164,7.45,50.6281249296065));
#196620=CARTESIAN_POINT('',(122.542812602034,7.45,50.3336368280768));
#196621=CARTESIAN_POINT('',(122.542812602034,7.45,50.3336368280768));
#196622=CARTESIAN_POINT('',(122.542812602034,7.45,50.3336368280768));
#196623=CARTESIAN_POINT('Origin',(123.033626104583,7.45,50.4290417845261));
#196624=CARTESIAN_POINT('',(123.033626104583,6.95,50.4290417845261));
#196625=CARTESIAN_POINT('',(122.976383130714,6.95,50.7235298860558));
#196626=CARTESIAN_POINT('',(123.033626104583,6.95,50.4290417845261));
#196627=CARTESIAN_POINT('',(122.976383130714,7.45,50.7235298860558));
#196628=CARTESIAN_POINT('',(123.033626104583,7.45,50.4290417845261));
#196629=CARTESIAN_POINT('Origin',(123.033626104583,6.95,50.4290417845261));
#196630=CARTESIAN_POINT('',(122.542812602034,6.95,50.3336368280768));
#196631=CARTESIAN_POINT('',(122.485569628164,6.95,50.6281249296065));
#196632=CARTESIAN_POINT('',(122.542812602034,6.95,50.3336368280768));
#196633=CARTESIAN_POINT('',(122.976383130714,6.95,50.7235298860558));
#196634=CARTESIAN_POINT('',(123.033626104583,6.95,50.4290417845261));
#196635=CARTESIAN_POINT('Origin',(122.542812602034,6.95,50.3336368280768));
#196636=CARTESIAN_POINT('',(122.485569628164,6.95,50.6281249296065));
#196637=CARTESIAN_POINT('',(122.542812602034,6.95,50.3336368280768));
#196638=CARTESIAN_POINT('Origin',(121.757510997955,7.45,50.180988897758));
#196639=CARTESIAN_POINT('',(122.248324500504,7.45,50.2763938542073));
#196640=CARTESIAN_POINT('',(122.191081526635,7.45,50.570881955737));
#196641=CARTESIAN_POINT('',(122.248324500504,7.45,50.2763938542073));
#196642=CARTESIAN_POINT('',(121.700268024085,7.45,50.4754769992877));
#196643=CARTESIAN_POINT('',(121.700268024085,7.45,50.4754769992877));
#196644=CARTESIAN_POINT('',(121.757510997955,7.45,50.180988897758));
#196645=CARTESIAN_POINT('',(121.757510997955,7.45,50.180988897758));
#196646=CARTESIAN_POINT('',(121.757510997955,7.45,50.180988897758));
#196647=CARTESIAN_POINT('Origin',(122.248324500504,7.45,50.2763938542073));
#196648=CARTESIAN_POINT('',(122.248324500504,6.95,50.2763938542073));
#196649=CARTESIAN_POINT('',(122.191081526635,6.95,50.570881955737));
#196650=CARTESIAN_POINT('',(122.248324500504,6.95,50.2763938542073));
#196651=CARTESIAN_POINT('',(122.191081526635,7.45,50.570881955737));
#196652=CARTESIAN_POINT('',(122.248324500504,7.45,50.2763938542073));
#196653=CARTESIAN_POINT('Origin',(122.248324500504,6.95,50.2763938542073));
#196654=CARTESIAN_POINT('',(121.757510997955,6.95,50.180988897758));
#196655=CARTESIAN_POINT('',(121.700268024085,6.95,50.4754769992877));
#196656=CARTESIAN_POINT('',(121.757510997955,6.95,50.180988897758));
#196657=CARTESIAN_POINT('',(122.191081526635,6.95,50.570881955737));
#196658=CARTESIAN_POINT('',(122.248324500504,6.95,50.2763938542073));
#196659=CARTESIAN_POINT('Origin',(121.757510997955,6.95,50.180988897758));
#196660=CARTESIAN_POINT('',(121.700268024085,6.95,50.4754769992877));
#196661=CARTESIAN_POINT('',(121.757510997955,6.95,50.180988897758));
#196662=CARTESIAN_POINT('Origin',(120.972209393875,7.45,50.0283409674392));
#196663=CARTESIAN_POINT('',(121.463022896425,7.45,50.1237459238885));
#196664=CARTESIAN_POINT('',(121.405779922555,7.45,50.4182340254182));
#196665=CARTESIAN_POINT('',(121.463022896425,7.45,50.1237459238885));
#196666=CARTESIAN_POINT('',(120.914966420006,7.45,50.3228290689689));
#196667=CARTESIAN_POINT('',(120.914966420006,7.45,50.3228290689689));
#196668=CARTESIAN_POINT('',(120.972209393875,7.45,50.0283409674392));
#196669=CARTESIAN_POINT('',(120.972209393875,7.45,50.0283409674392));
#196670=CARTESIAN_POINT('',(120.972209393875,7.45,50.0283409674392));
#196671=CARTESIAN_POINT('Origin',(121.463022896425,7.45,50.1237459238885));
#196672=CARTESIAN_POINT('',(121.463022896425,6.95,50.1237459238885));
#196673=CARTESIAN_POINT('',(121.405779922555,6.95,50.4182340254182));
#196674=CARTESIAN_POINT('',(121.463022896425,6.95,50.1237459238885));
#196675=CARTESIAN_POINT('',(121.405779922555,7.45,50.4182340254182));
#196676=CARTESIAN_POINT('',(121.463022896425,7.45,50.1237459238885));
#196677=CARTESIAN_POINT('Origin',(121.463022896425,6.95,50.1237459238885));
#196678=CARTESIAN_POINT('',(120.972209393875,6.95,50.0283409674392));
#196679=CARTESIAN_POINT('',(120.914966420006,6.95,50.3228290689689));
#196680=CARTESIAN_POINT('',(120.972209393875,6.95,50.0283409674392));
#196681=CARTESIAN_POINT('',(121.405779922555,6.95,50.4182340254182));
#196682=CARTESIAN_POINT('',(121.463022896425,6.95,50.1237459238885));
#196683=CARTESIAN_POINT('Origin',(120.972209393875,6.95,50.0283409674392));
#196684=CARTESIAN_POINT('',(120.914966420006,6.95,50.3228290689689));
#196685=CARTESIAN_POINT('',(120.972209393875,6.95,50.0283409674392));
#196686=CARTESIAN_POINT('Origin',(120.186907789796,7.45,49.8756930371204));
#196687=CARTESIAN_POINT('',(120.677721292346,7.45,49.9710979935697));
#196688=CARTESIAN_POINT('',(120.620478318476,7.45,50.2655860950994));
#196689=CARTESIAN_POINT('',(120.677721292346,7.45,49.9710979935697));
#196690=CARTESIAN_POINT('',(120.129664815927,7.45,50.1701811386501));
#196691=CARTESIAN_POINT('',(120.129664815927,7.45,50.1701811386501));
#196692=CARTESIAN_POINT('',(120.186907789796,7.45,49.8756930371204));
#196693=CARTESIAN_POINT('',(120.186907789796,7.45,49.8756930371204));
#196694=CARTESIAN_POINT('',(120.186907789796,7.45,49.8756930371204));
#196695=CARTESIAN_POINT('Origin',(120.677721292346,7.45,49.9710979935697));
#196696=CARTESIAN_POINT('',(120.677721292346,6.95,49.9710979935697));
#196697=CARTESIAN_POINT('',(120.620478318476,6.95,50.2655860950994));
#196698=CARTESIAN_POINT('',(120.677721292346,6.95,49.9710979935697));
#196699=CARTESIAN_POINT('',(120.620478318476,7.45,50.2655860950994));
#196700=CARTESIAN_POINT('',(120.677721292346,7.45,49.9710979935697));
#196701=CARTESIAN_POINT('Origin',(120.677721292346,6.95,49.9710979935697));
#196702=CARTESIAN_POINT('',(120.186907789796,6.95,49.8756930371204));
#196703=CARTESIAN_POINT('',(120.129664815927,6.95,50.1701811386501));
#196704=CARTESIAN_POINT('',(120.186907789796,6.95,49.8756930371204));
#196705=CARTESIAN_POINT('',(120.620478318476,6.95,50.2655860950994));
#196706=CARTESIAN_POINT('',(120.677721292346,6.95,49.9710979935697));
#196707=CARTESIAN_POINT('Origin',(120.186907789796,6.95,49.8756930371204));
#196708=CARTESIAN_POINT('',(120.129664815927,6.95,50.1701811386501));
#196709=CARTESIAN_POINT('',(120.186907789796,6.95,49.8756930371204));
#196710=CARTESIAN_POINT('Origin',(119.401606185717,7.45,49.7230451068016));
#196711=CARTESIAN_POINT('',(119.892419688267,7.45,49.8184500632509));
#196712=CARTESIAN_POINT('',(119.835176714397,7.45,50.1129381647806));
#196713=CARTESIAN_POINT('',(119.892419688267,7.45,49.8184500632509));
#196714=CARTESIAN_POINT('',(119.344363211847,7.45,50.0175332083313));
#196715=CARTESIAN_POINT('',(119.344363211847,7.45,50.0175332083313));
#196716=CARTESIAN_POINT('',(119.401606185717,7.45,49.7230451068016));
#196717=CARTESIAN_POINT('',(119.401606185717,7.45,49.7230451068016));
#196718=CARTESIAN_POINT('',(119.401606185717,7.45,49.7230451068016));
#196719=CARTESIAN_POINT('Origin',(119.892419688267,7.45,49.8184500632509));
#196720=CARTESIAN_POINT('',(119.892419688267,6.95,49.8184500632509));
#196721=CARTESIAN_POINT('',(119.835176714397,6.95,50.1129381647806));
#196722=CARTESIAN_POINT('',(119.892419688267,6.95,49.8184500632509));
#196723=CARTESIAN_POINT('',(119.835176714397,7.45,50.1129381647806));
#196724=CARTESIAN_POINT('',(119.892419688267,7.45,49.8184500632509));
#196725=CARTESIAN_POINT('Origin',(119.892419688267,6.95,49.8184500632509));
#196726=CARTESIAN_POINT('',(119.401606185717,6.95,49.7230451068016));
#196727=CARTESIAN_POINT('',(119.344363211847,6.95,50.0175332083313));
#196728=CARTESIAN_POINT('',(119.401606185717,6.95,49.7230451068016));
#196729=CARTESIAN_POINT('',(119.835176714397,6.95,50.1129381647806));
#196730=CARTESIAN_POINT('',(119.892419688267,6.95,49.8184500632509));
#196731=CARTESIAN_POINT('Origin',(119.401606185717,6.95,49.7230451068016));
#196732=CARTESIAN_POINT('',(119.344363211847,6.95,50.0175332083313));
#196733=CARTESIAN_POINT('',(119.401606185717,6.95,49.7230451068016));
#196734=CARTESIAN_POINT('Origin',(118.616304581638,7.45,49.5703971764828));
#196735=CARTESIAN_POINT('',(119.107118084187,7.45,49.6658021329321));
#196736=CARTESIAN_POINT('',(119.049875110318,7.45,49.9602902344618));
#196737=CARTESIAN_POINT('',(119.107118084187,7.45,49.6658021329321));
#196738=CARTESIAN_POINT('',(118.559061607768,7.45,49.8648852780125));
#196739=CARTESIAN_POINT('',(118.559061607768,7.45,49.8648852780125));
#196740=CARTESIAN_POINT('',(118.616304581638,7.45,49.5703971764828));
#196741=CARTESIAN_POINT('',(118.616304581638,7.45,49.5703971764828));
#196742=CARTESIAN_POINT('',(118.616304581638,7.45,49.5703971764828));
#196743=CARTESIAN_POINT('Origin',(119.107118084187,7.45,49.6658021329321));
#196744=CARTESIAN_POINT('',(119.107118084187,6.95,49.6658021329321));
#196745=CARTESIAN_POINT('',(119.049875110318,6.95,49.9602902344618));
#196746=CARTESIAN_POINT('',(119.107118084187,6.95,49.6658021329321));
#196747=CARTESIAN_POINT('',(119.049875110318,7.45,49.9602902344618));
#196748=CARTESIAN_POINT('',(119.107118084187,7.45,49.6658021329321));
#196749=CARTESIAN_POINT('Origin',(119.107118084187,6.95,49.6658021329321));
#196750=CARTESIAN_POINT('',(118.616304581638,6.95,49.5703971764828));
#196751=CARTESIAN_POINT('',(118.559061607768,6.95,49.8648852780125));
#196752=CARTESIAN_POINT('',(118.616304581638,6.95,49.5703971764828));
#196753=CARTESIAN_POINT('',(119.049875110318,6.95,49.9602902344618));
#196754=CARTESIAN_POINT('',(119.107118084187,6.95,49.6658021329321));
#196755=CARTESIAN_POINT('Origin',(118.616304581638,6.95,49.5703971764828));
#196756=CARTESIAN_POINT('',(118.559061607768,6.95,49.8648852780125));
#196757=CARTESIAN_POINT('',(118.616304581638,6.95,49.5703971764828));
#196758=CARTESIAN_POINT('Origin',(117.831002977559,7.45,49.417749246164));
#196759=CARTESIAN_POINT('',(118.321816480108,7.45,49.5131542026133));
#196760=CARTESIAN_POINT('',(118.264573506239,7.45,49.807642304143));
#196761=CARTESIAN_POINT('',(118.321816480108,7.45,49.5131542026133));
#196762=CARTESIAN_POINT('',(117.773760003689,7.45,49.7122373476937));
#196763=CARTESIAN_POINT('',(117.773760003689,7.45,49.7122373476937));
#196764=CARTESIAN_POINT('',(117.831002977559,7.45,49.417749246164));
#196765=CARTESIAN_POINT('',(117.831002977559,7.45,49.417749246164));
#196766=CARTESIAN_POINT('',(117.831002977559,7.45,49.417749246164));
#196767=CARTESIAN_POINT('Origin',(118.321816480108,7.45,49.5131542026133));
#196768=CARTESIAN_POINT('',(118.321816480108,6.95,49.5131542026133));
#196769=CARTESIAN_POINT('',(118.264573506239,6.95,49.807642304143));
#196770=CARTESIAN_POINT('',(118.321816480108,6.95,49.5131542026133));
#196771=CARTESIAN_POINT('',(118.264573506239,7.45,49.807642304143));
#196772=CARTESIAN_POINT('',(118.321816480108,7.45,49.5131542026133));
#196773=CARTESIAN_POINT('Origin',(118.321816480108,6.95,49.5131542026133));
#196774=CARTESIAN_POINT('',(117.831002977559,6.95,49.417749246164));
#196775=CARTESIAN_POINT('',(117.773760003689,6.95,49.7122373476937));
#196776=CARTESIAN_POINT('',(117.831002977559,6.95,49.417749246164));
#196777=CARTESIAN_POINT('',(118.264573506239,6.95,49.807642304143));
#196778=CARTESIAN_POINT('',(118.321816480108,6.95,49.5131542026133));
#196779=CARTESIAN_POINT('Origin',(117.831002977559,6.95,49.417749246164));
#196780=CARTESIAN_POINT('',(117.773760003689,6.95,49.7122373476937));
#196781=CARTESIAN_POINT('',(117.831002977559,6.95,49.417749246164));
#196782=CARTESIAN_POINT('Origin',(117.045701373479,7.45,49.2651013158452));
#196783=CARTESIAN_POINT('',(117.536514876029,7.45,49.3605062722945));
#196784=CARTESIAN_POINT('',(117.479271902159,7.45,49.6549943738242));
#196785=CARTESIAN_POINT('',(117.536514876029,7.45,49.3605062722945));
#196786=CARTESIAN_POINT('',(116.98845839961,7.45,49.5595894173749));
#196787=CARTESIAN_POINT('',(116.98845839961,7.45,49.5595894173749));
#196788=CARTESIAN_POINT('',(117.045701373479,7.45,49.2651013158452));
#196789=CARTESIAN_POINT('',(117.045701373479,7.45,49.2651013158452));
#196790=CARTESIAN_POINT('',(117.045701373479,7.45,49.2651013158452));
#196791=CARTESIAN_POINT('Origin',(117.536514876029,7.45,49.3605062722945));
#196792=CARTESIAN_POINT('',(117.536514876029,6.95,49.3605062722945));
#196793=CARTESIAN_POINT('',(117.479271902159,6.95,49.6549943738242));
#196794=CARTESIAN_POINT('',(117.536514876029,6.95,49.3605062722945));
#196795=CARTESIAN_POINT('',(117.479271902159,7.45,49.6549943738242));
#196796=CARTESIAN_POINT('',(117.536514876029,7.45,49.3605062722945));
#196797=CARTESIAN_POINT('Origin',(117.536514876029,6.95,49.3605062722945));
#196798=CARTESIAN_POINT('',(117.045701373479,6.95,49.2651013158452));
#196799=CARTESIAN_POINT('',(116.98845839961,6.95,49.5595894173749));
#196800=CARTESIAN_POINT('',(117.045701373479,6.95,49.2651013158452));
#196801=CARTESIAN_POINT('',(117.479271902159,6.95,49.6549943738242));
#196802=CARTESIAN_POINT('',(117.536514876029,6.95,49.3605062722945));
#196803=CARTESIAN_POINT('Origin',(117.045701373479,6.95,49.2651013158452));
#196804=CARTESIAN_POINT('',(116.98845839961,6.95,49.5595894173749));
#196805=CARTESIAN_POINT('',(117.045701373479,6.95,49.2651013158452));
#196806=CARTESIAN_POINT('Origin',(116.2603997694,7.45,49.1124533855264));
#196807=CARTESIAN_POINT('',(116.75121327195,7.45,49.2078583419757));
#196808=CARTESIAN_POINT('',(116.69397029808,7.45,49.5023464435054));
#196809=CARTESIAN_POINT('',(116.75121327195,7.45,49.2078583419757));
#196810=CARTESIAN_POINT('',(116.203156795531,7.45,49.4069414870561));
#196811=CARTESIAN_POINT('',(116.203156795531,7.45,49.4069414870561));
#196812=CARTESIAN_POINT('',(116.2603997694,7.45,49.1124533855264));
#196813=CARTESIAN_POINT('',(116.2603997694,7.45,49.1124533855264));
#196814=CARTESIAN_POINT('',(116.2603997694,7.45,49.1124533855264));
#196815=CARTESIAN_POINT('Origin',(116.75121327195,7.45,49.2078583419757));
#196816=CARTESIAN_POINT('',(116.75121327195,6.95,49.2078583419757));
#196817=CARTESIAN_POINT('',(116.69397029808,6.95,49.5023464435054));
#196818=CARTESIAN_POINT('',(116.75121327195,6.95,49.2078583419757));
#196819=CARTESIAN_POINT('',(116.69397029808,7.45,49.5023464435054));
#196820=CARTESIAN_POINT('',(116.75121327195,7.45,49.2078583419757));
#196821=CARTESIAN_POINT('Origin',(116.75121327195,6.95,49.2078583419757));
#196822=CARTESIAN_POINT('',(116.2603997694,6.95,49.1124533855264));
#196823=CARTESIAN_POINT('',(116.203156795531,6.95,49.4069414870561));
#196824=CARTESIAN_POINT('',(116.2603997694,6.95,49.1124533855264));
#196825=CARTESIAN_POINT('',(116.69397029808,6.95,49.5023464435054));
#196826=CARTESIAN_POINT('',(116.75121327195,6.95,49.2078583419757));
#196827=CARTESIAN_POINT('Origin',(116.2603997694,6.95,49.1124533855264));
#196828=CARTESIAN_POINT('',(116.203156795531,6.95,49.4069414870561));
#196829=CARTESIAN_POINT('',(116.2603997694,6.95,49.1124533855264));
#196830=CARTESIAN_POINT('Origin',(115.475098165321,7.45,48.9598054552076));
#196831=CARTESIAN_POINT('',(115.96591166787,7.45,49.0552104116569));
#196832=CARTESIAN_POINT('',(115.908668694001,7.45,49.3496985131866));
#196833=CARTESIAN_POINT('',(115.96591166787,7.45,49.0552104116569));
#196834=CARTESIAN_POINT('',(115.417855191451,7.45,49.2542935567373));
#196835=CARTESIAN_POINT('',(115.417855191451,7.45,49.2542935567373));
#196836=CARTESIAN_POINT('',(115.475098165321,7.45,48.9598054552076));
#196837=CARTESIAN_POINT('',(115.475098165321,7.45,48.9598054552076));
#196838=CARTESIAN_POINT('',(115.475098165321,7.45,48.9598054552076));
#196839=CARTESIAN_POINT('Origin',(115.96591166787,7.45,49.0552104116569));
#196840=CARTESIAN_POINT('',(115.96591166787,6.95,49.0552104116569));
#196841=CARTESIAN_POINT('',(115.908668694001,6.95,49.3496985131866));
#196842=CARTESIAN_POINT('',(115.96591166787,6.95,49.0552104116569));
#196843=CARTESIAN_POINT('',(115.908668694001,7.45,49.3496985131866));
#196844=CARTESIAN_POINT('',(115.96591166787,7.45,49.0552104116569));
#196845=CARTESIAN_POINT('Origin',(115.96591166787,6.95,49.0552104116569));
#196846=CARTESIAN_POINT('',(115.475098165321,6.95,48.9598054552076));
#196847=CARTESIAN_POINT('',(115.417855191451,6.95,49.2542935567373));
#196848=CARTESIAN_POINT('',(115.475098165321,6.95,48.9598054552076));
#196849=CARTESIAN_POINT('',(115.908668694001,6.95,49.3496985131866));
#196850=CARTESIAN_POINT('',(115.96591166787,6.95,49.0552104116569));
#196851=CARTESIAN_POINT('Origin',(115.475098165321,6.95,48.9598054552076));
#196852=CARTESIAN_POINT('',(115.417855191451,6.95,49.2542935567373));
#196853=CARTESIAN_POINT('',(115.475098165321,6.95,48.9598054552076));
#196854=CARTESIAN_POINT('Origin',(114.689796561242,7.45,48.8071575248888));
#196855=CARTESIAN_POINT('',(115.180610063791,7.45,48.9025624813381));
#196856=CARTESIAN_POINT('',(115.123367089922,7.45,49.1970505828678));
#196857=CARTESIAN_POINT('',(115.180610063791,7.45,48.9025624813381));
#196858=CARTESIAN_POINT('',(114.632553587372,7.45,49.1016456264185));
#196859=CARTESIAN_POINT('',(114.632553587372,7.45,49.1016456264185));
#196860=CARTESIAN_POINT('',(114.689796561242,7.45,48.8071575248888));
#196861=CARTESIAN_POINT('',(114.689796561242,7.45,48.8071575248888));
#196862=CARTESIAN_POINT('',(114.689796561242,7.45,48.8071575248888));
#196863=CARTESIAN_POINT('Origin',(115.180610063791,7.45,48.9025624813381));
#196864=CARTESIAN_POINT('',(115.180610063791,6.95,48.9025624813381));
#196865=CARTESIAN_POINT('',(115.123367089922,6.95,49.1970505828678));
#196866=CARTESIAN_POINT('',(115.180610063791,6.95,48.9025624813381));
#196867=CARTESIAN_POINT('',(115.123367089922,7.45,49.1970505828678));
#196868=CARTESIAN_POINT('',(115.180610063791,7.45,48.9025624813381));
#196869=CARTESIAN_POINT('Origin',(115.180610063791,6.95,48.9025624813381));
#196870=CARTESIAN_POINT('',(114.689796561242,6.95,48.8071575248888));
#196871=CARTESIAN_POINT('',(114.632553587372,6.95,49.1016456264185));
#196872=CARTESIAN_POINT('',(114.689796561242,6.95,48.8071575248888));
#196873=CARTESIAN_POINT('',(115.123367089922,6.95,49.1970505828678));
#196874=CARTESIAN_POINT('',(115.180610063791,6.95,48.9025624813381));
#196875=CARTESIAN_POINT('Origin',(114.689796561242,6.95,48.8071575248888));
#196876=CARTESIAN_POINT('',(114.632553587372,6.95,49.1016456264185));
#196877=CARTESIAN_POINT('',(114.689796561242,6.95,48.8071575248888));
#196878=CARTESIAN_POINT('Origin',(113.904494957163,7.45,48.65450959457));
#196879=CARTESIAN_POINT('',(114.395308459712,7.45,48.7499145510193));
#196880=CARTESIAN_POINT('',(114.338065485842,7.45,49.044402652549));
#196881=CARTESIAN_POINT('',(114.395308459712,7.45,48.7499145510193));
#196882=CARTESIAN_POINT('',(113.847251983293,7.45,48.9489976960997));
#196883=CARTESIAN_POINT('',(113.847251983293,7.45,48.9489976960997));
#196884=CARTESIAN_POINT('',(113.904494957163,7.45,48.65450959457));
#196885=CARTESIAN_POINT('',(113.904494957163,7.45,48.65450959457));
#196886=CARTESIAN_POINT('',(113.904494957163,7.45,48.65450959457));
#196887=CARTESIAN_POINT('Origin',(114.395308459712,7.45,48.7499145510193));
#196888=CARTESIAN_POINT('',(114.395308459712,6.95,48.7499145510193));
#196889=CARTESIAN_POINT('',(114.338065485842,6.95,49.044402652549));
#196890=CARTESIAN_POINT('',(114.395308459712,6.95,48.7499145510193));
#196891=CARTESIAN_POINT('',(114.338065485842,7.45,49.044402652549));
#196892=CARTESIAN_POINT('',(114.395308459712,7.45,48.7499145510193));
#196893=CARTESIAN_POINT('Origin',(114.395308459712,6.95,48.7499145510193));
#196894=CARTESIAN_POINT('',(113.904494957163,6.95,48.65450959457));
#196895=CARTESIAN_POINT('',(113.847251983293,6.95,48.9489976960997));
#196896=CARTESIAN_POINT('',(113.904494957163,6.95,48.65450959457));
#196897=CARTESIAN_POINT('',(114.338065485842,6.95,49.044402652549));
#196898=CARTESIAN_POINT('',(114.395308459712,6.95,48.7499145510193));
#196899=CARTESIAN_POINT('Origin',(113.904494957163,6.95,48.65450959457));
#196900=CARTESIAN_POINT('',(113.847251983293,6.95,48.9489976960997));
#196901=CARTESIAN_POINT('',(113.904494957163,6.95,48.65450959457));
#196902=CARTESIAN_POINT('Origin',(113.119193353083,7.45,48.5018616642512));
#196903=CARTESIAN_POINT('',(113.610006855633,7.45,48.5972666207005));
#196904=CARTESIAN_POINT('',(113.552763881763,7.45,48.8917547222302));
#196905=CARTESIAN_POINT('',(113.610006855633,7.45,48.5972666207005));
#196906=CARTESIAN_POINT('',(113.061950379214,7.45,48.7963497657809));
#196907=CARTESIAN_POINT('',(113.061950379214,7.45,48.7963497657809));
#196908=CARTESIAN_POINT('',(113.119193353083,7.45,48.5018616642512));
#196909=CARTESIAN_POINT('',(113.119193353083,7.45,48.5018616642512));
#196910=CARTESIAN_POINT('',(113.119193353083,7.45,48.5018616642512));
#196911=CARTESIAN_POINT('Origin',(113.610006855633,7.45,48.5972666207005));
#196912=CARTESIAN_POINT('',(113.610006855633,6.95,48.5972666207005));
#196913=CARTESIAN_POINT('',(113.552763881763,6.95,48.8917547222302));
#196914=CARTESIAN_POINT('',(113.610006855633,6.95,48.5972666207005));
#196915=CARTESIAN_POINT('',(113.552763881763,7.45,48.8917547222302));
#196916=CARTESIAN_POINT('',(113.610006855633,7.45,48.5972666207005));
#196917=CARTESIAN_POINT('Origin',(113.610006855633,6.95,48.5972666207005));
#196918=CARTESIAN_POINT('',(113.119193353083,6.95,48.5018616642512));
#196919=CARTESIAN_POINT('',(113.061950379214,6.95,48.7963497657809));
#196920=CARTESIAN_POINT('',(113.119193353083,6.95,48.5018616642512));
#196921=CARTESIAN_POINT('',(113.552763881763,6.95,48.8917547222302));
#196922=CARTESIAN_POINT('',(113.610006855633,6.95,48.5972666207005));
#196923=CARTESIAN_POINT('Origin',(113.119193353083,6.95,48.5018616642512));
#196924=CARTESIAN_POINT('',(113.061950379214,6.95,48.7963497657809));
#196925=CARTESIAN_POINT('',(113.119193353083,6.95,48.5018616642512));
#196926=CARTESIAN_POINT('Origin',(112.333891749004,7.45,48.3492137339324));
#196927=CARTESIAN_POINT('',(112.824705251554,7.45,48.4446186903817));
#196928=CARTESIAN_POINT('',(112.767462277684,7.45,48.7391067919114));
#196929=CARTESIAN_POINT('',(112.824705251554,7.45,48.4446186903817));
#196930=CARTESIAN_POINT('',(112.276648775135,7.45,48.6437018354621));
#196931=CARTESIAN_POINT('',(112.276648775135,7.45,48.6437018354621));
#196932=CARTESIAN_POINT('',(112.333891749004,7.45,48.3492137339324));
#196933=CARTESIAN_POINT('',(112.333891749004,7.45,48.3492137339324));
#196934=CARTESIAN_POINT('',(112.333891749004,7.45,48.3492137339324));
#196935=CARTESIAN_POINT('Origin',(112.824705251554,7.45,48.4446186903817));
#196936=CARTESIAN_POINT('',(112.824705251554,6.95,48.4446186903817));
#196937=CARTESIAN_POINT('',(112.767462277684,6.95,48.7391067919114));
#196938=CARTESIAN_POINT('',(112.824705251554,6.95,48.4446186903817));
#196939=CARTESIAN_POINT('',(112.767462277684,7.45,48.7391067919114));
#196940=CARTESIAN_POINT('',(112.824705251554,7.45,48.4446186903817));
#196941=CARTESIAN_POINT('Origin',(112.824705251554,6.95,48.4446186903817));
#196942=CARTESIAN_POINT('',(112.333891749004,6.95,48.3492137339324));
#196943=CARTESIAN_POINT('',(112.276648775135,6.95,48.6437018354621));
#196944=CARTESIAN_POINT('',(112.333891749004,6.95,48.3492137339324));
#196945=CARTESIAN_POINT('',(112.767462277684,6.95,48.7391067919114));
#196946=CARTESIAN_POINT('',(112.824705251554,6.95,48.4446186903817));
#196947=CARTESIAN_POINT('Origin',(112.333891749004,6.95,48.3492137339324));
#196948=CARTESIAN_POINT('',(112.276648775135,6.95,48.6437018354621));
#196949=CARTESIAN_POINT('',(112.333891749004,6.95,48.3492137339324));
#196950=CARTESIAN_POINT('Origin',(111.548590144925,7.45,48.1965658036136));
#196951=CARTESIAN_POINT('',(112.039403647474,7.45,48.2919707600629));
#196952=CARTESIAN_POINT('',(111.982160673605,7.45,48.5864588615926));
#196953=CARTESIAN_POINT('',(112.039403647474,7.45,48.2919707600629));
#196954=CARTESIAN_POINT('',(111.491347171055,7.45,48.4910539051433));
#196955=CARTESIAN_POINT('',(111.491347171055,7.45,48.4910539051433));
#196956=CARTESIAN_POINT('',(111.548590144925,7.45,48.1965658036136));
#196957=CARTESIAN_POINT('',(111.548590144925,7.45,48.1965658036136));
#196958=CARTESIAN_POINT('',(111.548590144925,7.45,48.1965658036136));
#196959=CARTESIAN_POINT('Origin',(112.039403647474,7.45,48.2919707600629));
#196960=CARTESIAN_POINT('',(112.039403647474,6.95,48.2919707600629));
#196961=CARTESIAN_POINT('',(111.982160673605,6.95,48.5864588615926));
#196962=CARTESIAN_POINT('',(112.039403647474,6.95,48.2919707600629));
#196963=CARTESIAN_POINT('',(111.982160673605,7.45,48.5864588615926));
#196964=CARTESIAN_POINT('',(112.039403647474,7.45,48.2919707600629));
#196965=CARTESIAN_POINT('Origin',(112.039403647474,6.95,48.2919707600629));
#196966=CARTESIAN_POINT('',(111.548590144925,6.95,48.1965658036136));
#196967=CARTESIAN_POINT('',(111.491347171055,6.95,48.4910539051433));
#196968=CARTESIAN_POINT('',(111.548590144925,6.95,48.1965658036136));
#196969=CARTESIAN_POINT('',(111.982160673605,6.95,48.5864588615926));
#196970=CARTESIAN_POINT('',(112.039403647474,6.95,48.2919707600629));
#196971=CARTESIAN_POINT('Origin',(111.548590144925,6.95,48.1965658036136));
#196972=CARTESIAN_POINT('',(111.491347171055,6.95,48.4910539051433));
#196973=CARTESIAN_POINT('',(111.548590144925,6.95,48.1965658036136));
#196974=CARTESIAN_POINT('Origin',(110.763288540846,6.65,48.0439178732948));
#196975=CARTESIAN_POINT('',(111.254102043395,6.65,48.139322829744));
#196976=CARTESIAN_POINT('',(111.196859069526,6.65,48.4338109312737));
#196977=CARTESIAN_POINT('',(111.254102043395,6.65,48.139322829744));
#196978=CARTESIAN_POINT('',(110.706045566976,6.65,48.3384059748245));
#196979=CARTESIAN_POINT('',(110.706045566976,6.65,48.3384059748245));
#196980=CARTESIAN_POINT('',(110.763288540846,6.65,48.0439178732948));
#196981=CARTESIAN_POINT('',(110.763288540846,6.65,48.0439178732948));
#196982=CARTESIAN_POINT('',(110.763288540846,6.65,48.0439178732948));
#196983=CARTESIAN_POINT('Origin',(111.254102043395,6.65,48.139322829744));
#196984=CARTESIAN_POINT('',(111.254102043395,6.15,48.139322829744));
#196985=CARTESIAN_POINT('',(111.196859069526,6.15,48.4338109312737));
#196986=CARTESIAN_POINT('',(111.254102043395,6.15,48.139322829744));
#196987=CARTESIAN_POINT('',(111.196859069526,6.65,48.4338109312737));
#196988=CARTESIAN_POINT('',(111.254102043395,6.65,48.139322829744));
#196989=CARTESIAN_POINT('Origin',(111.254102043395,6.15,48.139322829744));
#196990=CARTESIAN_POINT('',(110.763288540846,6.15,48.0439178732948));
#196991=CARTESIAN_POINT('',(110.706045566976,6.15,48.3384059748245));
#196992=CARTESIAN_POINT('',(110.763288540846,6.15,48.0439178732948));
#196993=CARTESIAN_POINT('',(111.196859069526,6.15,48.4338109312737));
#196994=CARTESIAN_POINT('',(111.254102043395,6.15,48.139322829744));
#196995=CARTESIAN_POINT('Origin',(110.763288540846,6.15,48.0439178732948));
#196996=CARTESIAN_POINT('',(110.706045566976,6.15,48.3384059748245));
#196997=CARTESIAN_POINT('',(110.763288540846,6.15,48.0439178732948));
#196998=CARTESIAN_POINT('Origin',(110.763288540846,5.85,48.0439178732948));
#196999=CARTESIAN_POINT('',(111.254102043395,5.85,48.139322829744));
#197000=CARTESIAN_POINT('',(111.196859069526,5.85,48.4338109312737));
#197001=CARTESIAN_POINT('',(111.254102043395,5.85,48.139322829744));
#197002=CARTESIAN_POINT('',(110.706045566976,5.85,48.3384059748245));
#197003=CARTESIAN_POINT('',(110.706045566976,5.85,48.3384059748245));
#197004=CARTESIAN_POINT('',(110.763288540846,5.85,48.0439178732948));
#197005=CARTESIAN_POINT('',(110.763288540846,5.85,48.0439178732948));
#197006=CARTESIAN_POINT('',(110.763288540846,5.85,48.0439178732948));
#197007=CARTESIAN_POINT('Origin',(111.254102043395,5.85,48.139322829744));
#197008=CARTESIAN_POINT('',(111.254102043395,5.35,48.139322829744));
#197009=CARTESIAN_POINT('',(111.196859069526,5.35,48.4338109312737));
#197010=CARTESIAN_POINT('',(111.254102043395,5.35,48.139322829744));
#197011=CARTESIAN_POINT('',(111.196859069526,5.85,48.4338109312737));
#197012=CARTESIAN_POINT('',(111.254102043395,5.85,48.139322829744));
#197013=CARTESIAN_POINT('Origin',(111.254102043395,5.35,48.139322829744));
#197014=CARTESIAN_POINT('',(110.763288540846,5.35,48.0439178732948));
#197015=CARTESIAN_POINT('',(110.706045566976,5.35,48.3384059748245));
#197016=CARTESIAN_POINT('',(110.763288540846,5.35,48.0439178732948));
#197017=CARTESIAN_POINT('',(111.196859069526,5.35,48.4338109312737));
#197018=CARTESIAN_POINT('',(111.254102043395,5.35,48.139322829744));
#197019=CARTESIAN_POINT('Origin',(110.763288540846,5.35,48.0439178732948));
#197020=CARTESIAN_POINT('',(110.706045566976,5.35,48.3384059748245));
#197021=CARTESIAN_POINT('',(110.763288540846,5.35,48.0439178732948));
#197022=CARTESIAN_POINT('Origin',(110.763288540846,5.05,48.0439178732948));
#197023=CARTESIAN_POINT('',(111.254102043395,5.05,48.139322829744));
#197024=CARTESIAN_POINT('',(111.196859069526,5.05,48.4338109312737));
#197025=CARTESIAN_POINT('',(111.254102043395,5.05,48.139322829744));
#197026=CARTESIAN_POINT('',(110.706045566976,5.05,48.3384059748245));
#197027=CARTESIAN_POINT('',(110.706045566976,5.05,48.3384059748245));
#197028=CARTESIAN_POINT('',(110.763288540846,5.05,48.0439178732948));
#197029=CARTESIAN_POINT('',(110.763288540846,5.05,48.0439178732948));
#197030=CARTESIAN_POINT('',(110.763288540846,5.05,48.0439178732948));
#197031=CARTESIAN_POINT('Origin',(111.254102043395,5.05,48.139322829744));
#197032=CARTESIAN_POINT('',(111.254102043395,4.55,48.139322829744));
#197033=CARTESIAN_POINT('',(111.196859069526,4.55,48.4338109312737));
#197034=CARTESIAN_POINT('',(111.254102043395,4.55,48.139322829744));
#197035=CARTESIAN_POINT('',(111.196859069526,5.05,48.4338109312737));
#197036=CARTESIAN_POINT('',(111.254102043395,5.05,48.139322829744));
#197037=CARTESIAN_POINT('Origin',(111.254102043395,4.55,48.139322829744));
#197038=CARTESIAN_POINT('',(110.763288540846,4.55,48.0439178732948));
#197039=CARTESIAN_POINT('',(110.706045566976,4.55,48.3384059748245));
#197040=CARTESIAN_POINT('',(110.763288540846,4.55,48.0439178732948));
#197041=CARTESIAN_POINT('',(111.196859069526,4.55,48.4338109312737));
#197042=CARTESIAN_POINT('',(111.254102043395,4.55,48.139322829744));
#197043=CARTESIAN_POINT('Origin',(110.763288540846,4.55,48.0439178732948));
#197044=CARTESIAN_POINT('',(110.706045566976,4.55,48.3384059748245));
#197045=CARTESIAN_POINT('',(110.763288540846,4.55,48.0439178732948));
#197046=CARTESIAN_POINT('Origin',(110.763288540846,4.25,48.0439178732948));
#197047=CARTESIAN_POINT('',(111.254102043395,4.25,48.139322829744));
#197048=CARTESIAN_POINT('',(111.196859069526,4.25,48.4338109312737));
#197049=CARTESIAN_POINT('',(111.254102043395,4.25,48.139322829744));
#197050=CARTESIAN_POINT('',(110.706045566976,4.25,48.3384059748245));
#197051=CARTESIAN_POINT('',(110.706045566976,4.25,48.3384059748245));
#197052=CARTESIAN_POINT('',(110.763288540846,4.25,48.0439178732948));
#197053=CARTESIAN_POINT('',(110.763288540846,4.25,48.0439178732948));
#197054=CARTESIAN_POINT('',(110.763288540846,4.25,48.0439178732948));
#197055=CARTESIAN_POINT('Origin',(111.254102043395,4.25,48.139322829744));
#197056=CARTESIAN_POINT('',(111.254102043395,3.75,48.139322829744));
#197057=CARTESIAN_POINT('',(111.196859069526,3.75,48.4338109312737));
#197058=CARTESIAN_POINT('',(111.254102043395,3.75,48.139322829744));
#197059=CARTESIAN_POINT('',(111.196859069526,4.25,48.4338109312737));
#197060=CARTESIAN_POINT('',(111.254102043395,4.25,48.139322829744));
#197061=CARTESIAN_POINT('Origin',(111.254102043395,3.75,48.139322829744));
#197062=CARTESIAN_POINT('',(110.763288540846,3.75,48.0439178732948));
#197063=CARTESIAN_POINT('',(110.706045566976,3.75,48.3384059748245));
#197064=CARTESIAN_POINT('',(110.763288540846,3.75,48.0439178732948));
#197065=CARTESIAN_POINT('',(111.196859069526,3.75,48.4338109312737));
#197066=CARTESIAN_POINT('',(111.254102043395,3.75,48.139322829744));
#197067=CARTESIAN_POINT('Origin',(110.763288540846,3.75,48.0439178732948));
#197068=CARTESIAN_POINT('',(110.706045566976,3.75,48.3384059748245));
#197069=CARTESIAN_POINT('',(110.763288540846,3.75,48.0439178732948));
#197070=CARTESIAN_POINT('Origin',(110.763288540846,3.45,48.0439178732948));
#197071=CARTESIAN_POINT('',(111.254102043395,3.45,48.139322829744));
#197072=CARTESIAN_POINT('',(111.196859069526,3.45,48.4338109312737));
#197073=CARTESIAN_POINT('',(111.254102043395,3.45,48.139322829744));
#197074=CARTESIAN_POINT('',(110.706045566976,3.45,48.3384059748245));
#197075=CARTESIAN_POINT('',(110.706045566976,3.45,48.3384059748245));
#197076=CARTESIAN_POINT('',(110.763288540846,3.45,48.0439178732948));
#197077=CARTESIAN_POINT('',(110.763288540846,3.45,48.0439178732948));
#197078=CARTESIAN_POINT('',(110.763288540846,3.45,48.0439178732948));
#197079=CARTESIAN_POINT('Origin',(111.254102043395,3.45,48.139322829744));
#197080=CARTESIAN_POINT('',(111.254102043395,2.95,48.139322829744));
#197081=CARTESIAN_POINT('',(111.196859069526,2.95,48.4338109312737));
#197082=CARTESIAN_POINT('',(111.254102043395,2.95,48.139322829744));
#197083=CARTESIAN_POINT('',(111.196859069526,3.45,48.4338109312737));
#197084=CARTESIAN_POINT('',(111.254102043395,3.45,48.139322829744));
#197085=CARTESIAN_POINT('Origin',(111.254102043395,2.95,48.139322829744));
#197086=CARTESIAN_POINT('',(110.763288540846,2.95,48.0439178732948));
#197087=CARTESIAN_POINT('',(110.706045566976,2.95,48.3384059748245));
#197088=CARTESIAN_POINT('',(110.763288540846,2.95,48.0439178732948));
#197089=CARTESIAN_POINT('',(111.196859069526,2.95,48.4338109312737));
#197090=CARTESIAN_POINT('',(111.254102043395,2.95,48.139322829744));
#197091=CARTESIAN_POINT('Origin',(110.763288540846,2.95,48.0439178732948));
#197092=CARTESIAN_POINT('',(110.706045566976,2.95,48.3384059748245));
#197093=CARTESIAN_POINT('',(110.763288540846,2.95,48.0439178732948));
#197094=CARTESIAN_POINT('Origin',(110.763288540846,2.65,48.0439178732948));
#197095=CARTESIAN_POINT('',(111.254102043395,2.65,48.139322829744));
#197096=CARTESIAN_POINT('',(111.196859069526,2.65,48.4338109312737));
#197097=CARTESIAN_POINT('',(111.254102043395,2.65,48.139322829744));
#197098=CARTESIAN_POINT('',(110.706045566976,2.65,48.3384059748245));
#197099=CARTESIAN_POINT('',(110.706045566976,2.65,48.3384059748245));
#197100=CARTESIAN_POINT('',(110.763288540846,2.65,48.0439178732948));
#197101=CARTESIAN_POINT('',(110.763288540846,2.65,48.0439178732948));
#197102=CARTESIAN_POINT('',(110.763288540846,2.65,48.0439178732948));
#197103=CARTESIAN_POINT('Origin',(111.254102043395,2.65,48.139322829744));
#197104=CARTESIAN_POINT('',(111.254102043395,2.15,48.139322829744));
#197105=CARTESIAN_POINT('',(111.196859069526,2.15,48.4338109312737));
#197106=CARTESIAN_POINT('',(111.254102043395,2.15,48.139322829744));
#197107=CARTESIAN_POINT('',(111.196859069526,2.65,48.4338109312737));
#197108=CARTESIAN_POINT('',(111.254102043395,2.65,48.139322829744));
#197109=CARTESIAN_POINT('Origin',(111.254102043395,2.15,48.139322829744));
#197110=CARTESIAN_POINT('',(110.763288540846,2.15,48.0439178732948));
#197111=CARTESIAN_POINT('',(110.706045566976,2.15,48.3384059748245));
#197112=CARTESIAN_POINT('',(110.763288540846,2.15,48.0439178732948));
#197113=CARTESIAN_POINT('',(111.196859069526,2.15,48.4338109312737));
#197114=CARTESIAN_POINT('',(111.254102043395,2.15,48.139322829744));
#197115=CARTESIAN_POINT('Origin',(110.763288540846,2.15,48.0439178732948));
#197116=CARTESIAN_POINT('',(110.706045566976,2.15,48.3384059748245));
#197117=CARTESIAN_POINT('',(110.763288540846,2.15,48.0439178732948));
#197118=CARTESIAN_POINT('Origin',(110.763288540846,1.85,48.0439178732948));
#197119=CARTESIAN_POINT('',(111.254102043395,1.85,48.139322829744));
#197120=CARTESIAN_POINT('',(111.196859069526,1.85,48.4338109312737));
#197121=CARTESIAN_POINT('',(111.254102043395,1.85,48.139322829744));
#197122=CARTESIAN_POINT('',(110.706045566976,1.85,48.3384059748245));
#197123=CARTESIAN_POINT('',(110.706045566976,1.85,48.3384059748245));
#197124=CARTESIAN_POINT('',(110.763288540846,1.85,48.0439178732948));
#197125=CARTESIAN_POINT('',(110.763288540846,1.85,48.0439178732948));
#197126=CARTESIAN_POINT('',(110.763288540846,1.85,48.0439178732948));
#197127=CARTESIAN_POINT('Origin',(111.254102043395,1.85,48.139322829744));
#197128=CARTESIAN_POINT('',(111.254102043395,1.35,48.139322829744));
#197129=CARTESIAN_POINT('',(111.196859069526,1.35,48.4338109312737));
#197130=CARTESIAN_POINT('',(111.254102043395,1.35,48.139322829744));
#197131=CARTESIAN_POINT('',(111.196859069526,1.85,48.4338109312737));
#197132=CARTESIAN_POINT('',(111.254102043395,1.85,48.139322829744));
#197133=CARTESIAN_POINT('Origin',(111.254102043395,1.35,48.139322829744));
#197134=CARTESIAN_POINT('',(110.763288540846,1.35,48.0439178732948));
#197135=CARTESIAN_POINT('',(110.706045566976,1.35,48.3384059748245));
#197136=CARTESIAN_POINT('',(110.763288540846,1.35,48.0439178732948));
#197137=CARTESIAN_POINT('',(111.196859069526,1.35,48.4338109312737));
#197138=CARTESIAN_POINT('',(111.254102043395,1.35,48.139322829744));
#197139=CARTESIAN_POINT('Origin',(110.763288540846,1.35,48.0439178732948));
#197140=CARTESIAN_POINT('',(110.706045566976,1.35,48.3384059748245));
#197141=CARTESIAN_POINT('',(110.763288540846,1.35,48.0439178732948));
#197142=CARTESIAN_POINT('Origin',(110.763288540846,1.05,48.0439178732948));
#197143=CARTESIAN_POINT('',(111.254102043395,1.05,48.139322829744));
#197144=CARTESIAN_POINT('',(111.196859069526,1.05,48.4338109312737));
#197145=CARTESIAN_POINT('',(111.254102043395,1.05,48.139322829744));
#197146=CARTESIAN_POINT('',(110.706045566976,1.05,48.3384059748245));
#197147=CARTESIAN_POINT('',(110.706045566976,1.05,48.3384059748245));
#197148=CARTESIAN_POINT('',(110.763288540846,1.05,48.0439178732948));
#197149=CARTESIAN_POINT('',(110.763288540846,1.05,48.0439178732948));
#197150=CARTESIAN_POINT('',(110.763288540846,1.05,48.0439178732948));
#197151=CARTESIAN_POINT('Origin',(111.254102043395,1.05,48.139322829744));
#197152=CARTESIAN_POINT('',(111.254102043395,0.550000000000015,48.139322829744));
#197153=CARTESIAN_POINT('',(111.196859069526,0.550000000000015,48.4338109312737));
#197154=CARTESIAN_POINT('',(111.254102043395,0.550000000000015,48.139322829744));
#197155=CARTESIAN_POINT('',(111.196859069526,1.05,48.4338109312737));
#197156=CARTESIAN_POINT('',(111.254102043395,1.05,48.139322829744));
#197157=CARTESIAN_POINT('Origin',(111.254102043395,0.550000000000015,48.139322829744));
#197158=CARTESIAN_POINT('',(110.763288540846,0.550000000000015,48.0439178732948));
#197159=CARTESIAN_POINT('',(110.706045566976,0.550000000000015,48.3384059748245));
#197160=CARTESIAN_POINT('',(110.763288540846,0.550000000000015,48.0439178732948));
#197161=CARTESIAN_POINT('',(111.196859069526,0.550000000000015,48.4338109312737));
#197162=CARTESIAN_POINT('',(111.254102043395,0.550000000000015,48.139322829744));
#197163=CARTESIAN_POINT('Origin',(110.763288540846,0.550000000000015,48.0439178732948));
#197164=CARTESIAN_POINT('',(110.706045566976,0.550000000000015,48.3384059748245));
#197165=CARTESIAN_POINT('',(110.763288540846,0.550000000000015,48.0439178732948));
#197166=CARTESIAN_POINT('Origin',(110.763288540846,0.250000000000015,48.0439178732948));
#197167=CARTESIAN_POINT('',(111.254102043395,0.250000000000015,48.139322829744));
#197168=CARTESIAN_POINT('',(111.196859069526,0.250000000000015,48.4338109312737));
#197169=CARTESIAN_POINT('',(111.254102043395,0.250000000000015,48.139322829744));
#197170=CARTESIAN_POINT('',(110.706045566976,0.250000000000015,48.3384059748245));
#197171=CARTESIAN_POINT('',(110.706045566976,0.250000000000015,48.3384059748245));
#197172=CARTESIAN_POINT('',(110.763288540846,0.250000000000015,48.0439178732948));
#197173=CARTESIAN_POINT('',(110.763288540846,0.250000000000015,48.0439178732948));
#197174=CARTESIAN_POINT('',(110.763288540846,0.250000000000015,48.0439178732948));
#197175=CARTESIAN_POINT('Origin',(111.254102043395,0.250000000000015,48.139322829744));
#197176=CARTESIAN_POINT('',(111.254102043395,-0.249999999999985,48.139322829744));
#197177=CARTESIAN_POINT('',(111.196859069526,-0.249999999999985,48.4338109312737));
#197178=CARTESIAN_POINT('',(111.254102043395,-0.249999999999985,48.139322829744));
#197179=CARTESIAN_POINT('',(111.196859069526,0.250000000000015,48.4338109312737));
#197180=CARTESIAN_POINT('',(111.254102043395,0.250000000000015,48.139322829744));
#197181=CARTESIAN_POINT('Origin',(111.254102043395,-0.249999999999985,48.139322829744));
#197182=CARTESIAN_POINT('',(110.763288540846,-0.249999999999985,48.0439178732948));
#197183=CARTESIAN_POINT('',(110.706045566976,-0.249999999999985,48.3384059748245));
#197184=CARTESIAN_POINT('',(110.763288540846,-0.249999999999985,48.0439178732948));
#197185=CARTESIAN_POINT('',(111.196859069526,-0.249999999999985,48.4338109312737));
#197186=CARTESIAN_POINT('',(111.254102043395,-0.249999999999985,48.139322829744));
#197187=CARTESIAN_POINT('Origin',(110.763288540846,-0.249999999999985,48.0439178732948));
#197188=CARTESIAN_POINT('',(110.706045566976,-0.249999999999985,48.3384059748245));
#197189=CARTESIAN_POINT('',(110.763288540846,-0.249999999999985,48.0439178732948));
#197190=CARTESIAN_POINT('Origin',(110.763288540846,-0.549999999999986,48.0439178732948));
#197191=CARTESIAN_POINT('',(111.254102043395,-0.549999999999986,48.139322829744));
#197192=CARTESIAN_POINT('',(111.196859069526,-0.549999999999986,48.4338109312737));
#197193=CARTESIAN_POINT('',(111.254102043395,-0.549999999999986,48.139322829744));
#197194=CARTESIAN_POINT('',(110.706045566976,-0.549999999999986,48.3384059748245));
#197195=CARTESIAN_POINT('',(110.706045566976,-0.549999999999986,48.3384059748245));
#197196=CARTESIAN_POINT('',(110.763288540846,-0.549999999999986,48.0439178732948));
#197197=CARTESIAN_POINT('',(110.763288540846,-0.549999999999986,48.0439178732948));
#197198=CARTESIAN_POINT('',(110.763288540846,-0.549999999999986,48.0439178732948));
#197199=CARTESIAN_POINT('Origin',(111.254102043395,-0.549999999999986,48.139322829744));
#197200=CARTESIAN_POINT('',(111.254102043395,-1.05,48.139322829744));
#197201=CARTESIAN_POINT('',(111.196859069526,-1.05,48.4338109312737));
#197202=CARTESIAN_POINT('',(111.254102043395,-1.05,48.139322829744));
#197203=CARTESIAN_POINT('',(111.196859069526,-0.549999999999986,48.4338109312737));
#197204=CARTESIAN_POINT('',(111.254102043395,-0.549999999999986,48.139322829744));
#197205=CARTESIAN_POINT('Origin',(111.254102043395,-1.05,48.139322829744));
#197206=CARTESIAN_POINT('',(110.763288540846,-1.05,48.0439178732948));
#197207=CARTESIAN_POINT('',(110.706045566976,-1.05,48.3384059748245));
#197208=CARTESIAN_POINT('',(110.763288540846,-1.05,48.0439178732948));
#197209=CARTESIAN_POINT('',(111.196859069526,-1.05,48.4338109312737));
#197210=CARTESIAN_POINT('',(111.254102043395,-1.05,48.139322829744));
#197211=CARTESIAN_POINT('Origin',(110.763288540846,-1.05,48.0439178732948));
#197212=CARTESIAN_POINT('',(110.706045566976,-1.05,48.3384059748245));
#197213=CARTESIAN_POINT('',(110.763288540846,-1.05,48.0439178732948));
#197214=CARTESIAN_POINT('Origin',(110.763288540846,-1.35,48.0439178732948));
#197215=CARTESIAN_POINT('',(111.254102043395,-1.35,48.139322829744));
#197216=CARTESIAN_POINT('',(111.196859069526,-1.35,48.4338109312737));
#197217=CARTESIAN_POINT('',(111.254102043395,-1.35,48.139322829744));
#197218=CARTESIAN_POINT('',(110.706045566976,-1.35,48.3384059748245));
#197219=CARTESIAN_POINT('',(110.706045566976,-1.35,48.3384059748245));
#197220=CARTESIAN_POINT('',(110.763288540846,-1.35,48.0439178732948));
#197221=CARTESIAN_POINT('',(110.763288540846,-1.35,48.0439178732948));
#197222=CARTESIAN_POINT('',(110.763288540846,-1.35,48.0439178732948));
#197223=CARTESIAN_POINT('Origin',(111.254102043395,-1.35,48.139322829744));
#197224=CARTESIAN_POINT('',(111.254102043395,-1.85,48.139322829744));
#197225=CARTESIAN_POINT('',(111.196859069526,-1.85,48.4338109312737));
#197226=CARTESIAN_POINT('',(111.254102043395,-1.85,48.139322829744));
#197227=CARTESIAN_POINT('',(111.196859069526,-1.35,48.4338109312737));
#197228=CARTESIAN_POINT('',(111.254102043395,-1.35,48.139322829744));
#197229=CARTESIAN_POINT('Origin',(111.254102043395,-1.85,48.139322829744));
#197230=CARTESIAN_POINT('',(110.763288540846,-1.85,48.0439178732948));
#197231=CARTESIAN_POINT('',(110.706045566976,-1.85,48.3384059748245));
#197232=CARTESIAN_POINT('',(110.763288540846,-1.85,48.0439178732948));
#197233=CARTESIAN_POINT('',(111.196859069526,-1.85,48.4338109312737));
#197234=CARTESIAN_POINT('',(111.254102043395,-1.85,48.139322829744));
#197235=CARTESIAN_POINT('Origin',(110.763288540846,-1.85,48.0439178732948));
#197236=CARTESIAN_POINT('',(110.706045566976,-1.85,48.3384059748245));
#197237=CARTESIAN_POINT('',(110.763288540846,-1.85,48.0439178732948));
#197238=CARTESIAN_POINT('Origin',(110.763288540846,-2.15,48.0439178732948));
#197239=CARTESIAN_POINT('',(111.254102043395,-2.15,48.139322829744));
#197240=CARTESIAN_POINT('',(111.196859069526,-2.15,48.4338109312737));
#197241=CARTESIAN_POINT('',(111.254102043395,-2.15,48.139322829744));
#197242=CARTESIAN_POINT('',(110.706045566976,-2.15,48.3384059748245));
#197243=CARTESIAN_POINT('',(110.706045566976,-2.15,48.3384059748245));
#197244=CARTESIAN_POINT('',(110.763288540846,-2.15,48.0439178732948));
#197245=CARTESIAN_POINT('',(110.763288540846,-2.15,48.0439178732948));
#197246=CARTESIAN_POINT('',(110.763288540846,-2.15,48.0439178732948));
#197247=CARTESIAN_POINT('Origin',(111.254102043395,-2.15,48.139322829744));
#197248=CARTESIAN_POINT('',(111.254102043395,-2.65,48.139322829744));
#197249=CARTESIAN_POINT('',(111.196859069526,-2.65,48.4338109312737));
#197250=CARTESIAN_POINT('',(111.254102043395,-2.65,48.139322829744));
#197251=CARTESIAN_POINT('',(111.196859069526,-2.15,48.4338109312737));
#197252=CARTESIAN_POINT('',(111.254102043395,-2.15,48.139322829744));
#197253=CARTESIAN_POINT('Origin',(111.254102043395,-2.65,48.139322829744));
#197254=CARTESIAN_POINT('',(110.763288540846,-2.65,48.0439178732948));
#197255=CARTESIAN_POINT('',(110.706045566976,-2.65,48.3384059748245));
#197256=CARTESIAN_POINT('',(110.763288540846,-2.65,48.0439178732948));
#197257=CARTESIAN_POINT('',(111.196859069526,-2.65,48.4338109312737));
#197258=CARTESIAN_POINT('',(111.254102043395,-2.65,48.139322829744));
#197259=CARTESIAN_POINT('Origin',(110.763288540846,-2.65,48.0439178732948));
#197260=CARTESIAN_POINT('',(110.706045566976,-2.65,48.3384059748245));
#197261=CARTESIAN_POINT('',(110.763288540846,-2.65,48.0439178732948));
#197262=CARTESIAN_POINT('Origin',(110.763288540846,-2.95,48.0439178732948));
#197263=CARTESIAN_POINT('',(111.254102043395,-2.95,48.139322829744));
#197264=CARTESIAN_POINT('',(111.196859069526,-2.95,48.4338109312737));
#197265=CARTESIAN_POINT('',(111.254102043395,-2.95,48.139322829744));
#197266=CARTESIAN_POINT('',(110.706045566976,-2.95,48.3384059748245));
#197267=CARTESIAN_POINT('',(110.706045566976,-2.95,48.3384059748245));
#197268=CARTESIAN_POINT('',(110.763288540846,-2.95,48.0439178732948));
#197269=CARTESIAN_POINT('',(110.763288540846,-2.95,48.0439178732948));
#197270=CARTESIAN_POINT('',(110.763288540846,-2.95,48.0439178732948));
#197271=CARTESIAN_POINT('Origin',(111.254102043395,-2.95,48.139322829744));
#197272=CARTESIAN_POINT('',(111.254102043395,-3.45,48.139322829744));
#197273=CARTESIAN_POINT('',(111.196859069526,-3.45,48.4338109312737));
#197274=CARTESIAN_POINT('',(111.254102043395,-3.45,48.139322829744));
#197275=CARTESIAN_POINT('',(111.196859069526,-2.95,48.4338109312737));
#197276=CARTESIAN_POINT('',(111.254102043395,-2.95,48.139322829744));
#197277=CARTESIAN_POINT('Origin',(111.254102043395,-3.45,48.139322829744));
#197278=CARTESIAN_POINT('',(110.763288540846,-3.45,48.0439178732948));
#197279=CARTESIAN_POINT('',(110.706045566976,-3.45,48.3384059748245));
#197280=CARTESIAN_POINT('',(110.763288540846,-3.45,48.0439178732948));
#197281=CARTESIAN_POINT('',(111.196859069526,-3.45,48.4338109312737));
#197282=CARTESIAN_POINT('',(111.254102043395,-3.45,48.139322829744));
#197283=CARTESIAN_POINT('Origin',(110.763288540846,-3.45,48.0439178732948));
#197284=CARTESIAN_POINT('',(110.706045566976,-3.45,48.3384059748245));
#197285=CARTESIAN_POINT('',(110.763288540846,-3.45,48.0439178732948));
#197286=CARTESIAN_POINT('Origin',(110.763288540846,-3.75,48.0439178732948));
#197287=CARTESIAN_POINT('',(111.254102043395,-3.75,48.139322829744));
#197288=CARTESIAN_POINT('',(111.196859069526,-3.75,48.4338109312737));
#197289=CARTESIAN_POINT('',(111.254102043395,-3.75,48.139322829744));
#197290=CARTESIAN_POINT('',(110.706045566976,-3.75,48.3384059748245));
#197291=CARTESIAN_POINT('',(110.706045566976,-3.75,48.3384059748245));
#197292=CARTESIAN_POINT('',(110.763288540846,-3.75,48.0439178732948));
#197293=CARTESIAN_POINT('',(110.763288540846,-3.75,48.0439178732948));
#197294=CARTESIAN_POINT('',(110.763288540846,-3.75,48.0439178732948));
#197295=CARTESIAN_POINT('Origin',(111.254102043395,-3.75,48.139322829744));
#197296=CARTESIAN_POINT('',(111.254102043395,-4.25,48.139322829744));
#197297=CARTESIAN_POINT('',(111.196859069526,-4.25,48.4338109312737));
#197298=CARTESIAN_POINT('',(111.254102043395,-4.25,48.139322829744));
#197299=CARTESIAN_POINT('',(111.196859069526,-3.75,48.4338109312737));
#197300=CARTESIAN_POINT('',(111.254102043395,-3.75,48.139322829744));
#197301=CARTESIAN_POINT('Origin',(111.254102043395,-4.25,48.139322829744));
#197302=CARTESIAN_POINT('',(110.763288540846,-4.25,48.0439178732948));
#197303=CARTESIAN_POINT('',(110.706045566976,-4.25,48.3384059748245));
#197304=CARTESIAN_POINT('',(110.763288540846,-4.25,48.0439178732948));
#197305=CARTESIAN_POINT('',(111.196859069526,-4.25,48.4338109312737));
#197306=CARTESIAN_POINT('',(111.254102043395,-4.25,48.139322829744));
#197307=CARTESIAN_POINT('Origin',(110.763288540846,-4.25,48.0439178732948));
#197308=CARTESIAN_POINT('',(110.706045566976,-4.25,48.3384059748245));
#197309=CARTESIAN_POINT('',(110.763288540846,-4.25,48.0439178732948));
#197310=CARTESIAN_POINT('Origin',(110.763288540846,-4.55,48.0439178732948));
#197311=CARTESIAN_POINT('',(111.254102043395,-4.55,48.139322829744));
#197312=CARTESIAN_POINT('',(111.196859069526,-4.55,48.4338109312737));
#197313=CARTESIAN_POINT('',(111.254102043395,-4.55,48.139322829744));
#197314=CARTESIAN_POINT('',(110.706045566976,-4.55,48.3384059748245));
#197315=CARTESIAN_POINT('',(110.706045566976,-4.55,48.3384059748245));
#197316=CARTESIAN_POINT('',(110.763288540846,-4.55,48.0439178732948));
#197317=CARTESIAN_POINT('',(110.763288540846,-4.55,48.0439178732948));
#197318=CARTESIAN_POINT('',(110.763288540846,-4.55,48.0439178732948));
#197319=CARTESIAN_POINT('Origin',(111.254102043395,-4.55,48.139322829744));
#197320=CARTESIAN_POINT('',(111.254102043395,-5.05,48.139322829744));
#197321=CARTESIAN_POINT('',(111.196859069526,-5.05,48.4338109312737));
#197322=CARTESIAN_POINT('',(111.254102043395,-5.05,48.139322829744));
#197323=CARTESIAN_POINT('',(111.196859069526,-4.55,48.4338109312737));
#197324=CARTESIAN_POINT('',(111.254102043395,-4.55,48.139322829744));
#197325=CARTESIAN_POINT('Origin',(111.254102043395,-5.05,48.139322829744));
#197326=CARTESIAN_POINT('',(110.763288540846,-5.05,48.0439178732948));
#197327=CARTESIAN_POINT('',(110.706045566976,-5.05,48.3384059748245));
#197328=CARTESIAN_POINT('',(110.763288540846,-5.05,48.0439178732948));
#197329=CARTESIAN_POINT('',(111.196859069526,-5.05,48.4338109312737));
#197330=CARTESIAN_POINT('',(111.254102043395,-5.05,48.139322829744));
#197331=CARTESIAN_POINT('Origin',(110.763288540846,-5.05,48.0439178732948));
#197332=CARTESIAN_POINT('',(110.706045566976,-5.05,48.3384059748245));
#197333=CARTESIAN_POINT('',(110.763288540846,-5.05,48.0439178732948));
#197334=CARTESIAN_POINT('Origin',(110.763288540846,-5.35,48.0439178732948));
#197335=CARTESIAN_POINT('',(111.254102043395,-5.35,48.139322829744));
#197336=CARTESIAN_POINT('',(111.196859069526,-5.35,48.4338109312737));
#197337=CARTESIAN_POINT('',(111.254102043395,-5.35,48.139322829744));
#197338=CARTESIAN_POINT('',(110.706045566976,-5.35,48.3384059748245));
#197339=CARTESIAN_POINT('',(110.706045566976,-5.35,48.3384059748245));
#197340=CARTESIAN_POINT('',(110.763288540846,-5.35,48.0439178732948));
#197341=CARTESIAN_POINT('',(110.763288540846,-5.35,48.0439178732948));
#197342=CARTESIAN_POINT('',(110.763288540846,-5.35,48.0439178732948));
#197343=CARTESIAN_POINT('Origin',(111.254102043395,-5.35,48.139322829744));
#197344=CARTESIAN_POINT('',(111.254102043395,-5.85,48.139322829744));
#197345=CARTESIAN_POINT('',(111.196859069526,-5.85,48.4338109312737));
#197346=CARTESIAN_POINT('',(111.254102043395,-5.85,48.139322829744));
#197347=CARTESIAN_POINT('',(111.196859069526,-5.35,48.4338109312737));
#197348=CARTESIAN_POINT('',(111.254102043395,-5.35,48.139322829744));
#197349=CARTESIAN_POINT('Origin',(111.254102043395,-5.85,48.139322829744));
#197350=CARTESIAN_POINT('',(110.763288540846,-5.85,48.0439178732948));
#197351=CARTESIAN_POINT('',(110.706045566976,-5.85,48.3384059748245));
#197352=CARTESIAN_POINT('',(110.763288540846,-5.85,48.0439178732948));
#197353=CARTESIAN_POINT('',(111.196859069526,-5.85,48.4338109312737));
#197354=CARTESIAN_POINT('',(111.254102043395,-5.85,48.139322829744));
#197355=CARTESIAN_POINT('Origin',(110.763288540846,-5.85,48.0439178732948));
#197356=CARTESIAN_POINT('',(110.706045566976,-5.85,48.3384059748245));
#197357=CARTESIAN_POINT('',(110.763288540846,-5.85,48.0439178732948));
#197358=CARTESIAN_POINT('Origin',(110.763288540846,-6.15,48.0439178732948));
#197359=CARTESIAN_POINT('',(111.254102043395,-6.15,48.139322829744));
#197360=CARTESIAN_POINT('',(111.196859069526,-6.15,48.4338109312737));
#197361=CARTESIAN_POINT('',(111.254102043395,-6.15,48.139322829744));
#197362=CARTESIAN_POINT('',(110.706045566976,-6.15,48.3384059748245));
#197363=CARTESIAN_POINT('',(110.706045566976,-6.15,48.3384059748245));
#197364=CARTESIAN_POINT('',(110.763288540846,-6.15,48.0439178732948));
#197365=CARTESIAN_POINT('',(110.763288540846,-6.15,48.0439178732948));
#197366=CARTESIAN_POINT('',(110.763288540846,-6.15,48.0439178732948));
#197367=CARTESIAN_POINT('Origin',(111.254102043395,-6.15,48.139322829744));
#197368=CARTESIAN_POINT('',(111.254102043395,-6.65,48.139322829744));
#197369=CARTESIAN_POINT('',(111.196859069526,-6.65,48.4338109312737));
#197370=CARTESIAN_POINT('',(111.254102043395,-6.65,48.139322829744));
#197371=CARTESIAN_POINT('',(111.196859069526,-6.15,48.4338109312737));
#197372=CARTESIAN_POINT('',(111.254102043395,-6.15,48.139322829744));
#197373=CARTESIAN_POINT('Origin',(111.254102043395,-6.65,48.139322829744));
#197374=CARTESIAN_POINT('',(110.763288540846,-6.65,48.0439178732948));
#197375=CARTESIAN_POINT('',(110.706045566976,-6.65,48.3384059748245));
#197376=CARTESIAN_POINT('',(110.763288540846,-6.65,48.0439178732948));
#197377=CARTESIAN_POINT('',(111.196859069526,-6.65,48.4338109312737));
#197378=CARTESIAN_POINT('',(111.254102043395,-6.65,48.139322829744));
#197379=CARTESIAN_POINT('Origin',(110.763288540846,-6.65,48.0439178732948));
#197380=CARTESIAN_POINT('',(110.706045566976,-6.65,48.3384059748245));
#197381=CARTESIAN_POINT('',(110.763288540846,-6.65,48.0439178732948));
#197382=CARTESIAN_POINT('Origin',(111.548590144925,-6.15,48.1965658036136));
#197383=CARTESIAN_POINT('',(112.039403647474,-6.15,48.2919707600629));
#197384=CARTESIAN_POINT('',(111.982160673605,-6.15,48.5864588615926));
#197385=CARTESIAN_POINT('',(112.039403647474,-6.15,48.2919707600629));
#197386=CARTESIAN_POINT('',(111.491347171055,-6.15,48.4910539051433));
#197387=CARTESIAN_POINT('',(111.491347171055,-6.15,48.4910539051433));
#197388=CARTESIAN_POINT('',(111.548590144925,-6.15,48.1965658036136));
#197389=CARTESIAN_POINT('',(111.548590144925,-6.15,48.1965658036136));
#197390=CARTESIAN_POINT('',(111.548590144925,-6.15,48.1965658036136));
#197391=CARTESIAN_POINT('Origin',(112.039403647474,-6.15,48.2919707600629));
#197392=CARTESIAN_POINT('',(112.039403647474,-6.65,48.2919707600629));
#197393=CARTESIAN_POINT('',(111.982160673605,-6.65,48.5864588615926));
#197394=CARTESIAN_POINT('',(112.039403647474,-6.65,48.2919707600629));
#197395=CARTESIAN_POINT('',(111.982160673605,-6.15,48.5864588615926));
#197396=CARTESIAN_POINT('',(112.039403647474,-6.15,48.2919707600629));
#197397=CARTESIAN_POINT('Origin',(112.039403647474,-6.65,48.2919707600629));
#197398=CARTESIAN_POINT('',(111.548590144925,-6.65,48.1965658036136));
#197399=CARTESIAN_POINT('',(111.491347171055,-6.65,48.4910539051433));
#197400=CARTESIAN_POINT('',(111.548590144925,-6.65,48.1965658036136));
#197401=CARTESIAN_POINT('',(111.982160673605,-6.65,48.5864588615926));
#197402=CARTESIAN_POINT('',(112.039403647474,-6.65,48.2919707600629));
#197403=CARTESIAN_POINT('Origin',(111.548590144925,-6.65,48.1965658036136));
#197404=CARTESIAN_POINT('',(111.491347171055,-6.65,48.4910539051433));
#197405=CARTESIAN_POINT('',(111.548590144925,-6.65,48.1965658036136));
#197406=CARTESIAN_POINT('Origin',(112.333891749004,-6.15,48.3492137339324));
#197407=CARTESIAN_POINT('',(112.824705251554,-6.15,48.4446186903817));
#197408=CARTESIAN_POINT('',(112.767462277684,-6.15,48.7391067919114));
#197409=CARTESIAN_POINT('',(112.824705251554,-6.15,48.4446186903817));
#197410=CARTESIAN_POINT('',(112.276648775135,-6.15,48.6437018354621));
#197411=CARTESIAN_POINT('',(112.276648775135,-6.15,48.6437018354621));
#197412=CARTESIAN_POINT('',(112.333891749004,-6.15,48.3492137339324));
#197413=CARTESIAN_POINT('',(112.333891749004,-6.15,48.3492137339324));
#197414=CARTESIAN_POINT('',(112.333891749004,-6.15,48.3492137339324));
#197415=CARTESIAN_POINT('Origin',(112.824705251554,-6.15,48.4446186903817));
#197416=CARTESIAN_POINT('',(112.824705251554,-6.65,48.4446186903817));
#197417=CARTESIAN_POINT('',(112.767462277684,-6.65,48.7391067919114));
#197418=CARTESIAN_POINT('',(112.824705251554,-6.65,48.4446186903817));
#197419=CARTESIAN_POINT('',(112.767462277684,-6.15,48.7391067919114));
#197420=CARTESIAN_POINT('',(112.824705251554,-6.15,48.4446186903817));
#197421=CARTESIAN_POINT('Origin',(112.824705251554,-6.65,48.4446186903817));
#197422=CARTESIAN_POINT('',(112.333891749004,-6.65,48.3492137339324));
#197423=CARTESIAN_POINT('',(112.276648775135,-6.65,48.6437018354621));
#197424=CARTESIAN_POINT('',(112.333891749004,-6.65,48.3492137339324));
#197425=CARTESIAN_POINT('',(112.767462277684,-6.65,48.7391067919114));
#197426=CARTESIAN_POINT('',(112.824705251554,-6.65,48.4446186903817));
#197427=CARTESIAN_POINT('Origin',(112.333891749004,-6.65,48.3492137339324));
#197428=CARTESIAN_POINT('',(112.276648775135,-6.65,48.6437018354621));
#197429=CARTESIAN_POINT('',(112.333891749004,-6.65,48.3492137339324));
#197430=CARTESIAN_POINT('Origin',(113.119193353083,-6.15,48.5018616642512));
#197431=CARTESIAN_POINT('',(113.610006855633,-6.15,48.5972666207005));
#197432=CARTESIAN_POINT('',(113.552763881763,-6.15,48.8917547222302));
#197433=CARTESIAN_POINT('',(113.610006855633,-6.15,48.5972666207005));
#197434=CARTESIAN_POINT('',(113.061950379214,-6.15,48.7963497657809));
#197435=CARTESIAN_POINT('',(113.061950379214,-6.15,48.7963497657809));
#197436=CARTESIAN_POINT('',(113.119193353083,-6.15,48.5018616642512));
#197437=CARTESIAN_POINT('',(113.119193353083,-6.15,48.5018616642512));
#197438=CARTESIAN_POINT('',(113.119193353083,-6.15,48.5018616642512));
#197439=CARTESIAN_POINT('Origin',(113.610006855633,-6.15,48.5972666207005));
#197440=CARTESIAN_POINT('',(113.610006855633,-6.65,48.5972666207005));
#197441=CARTESIAN_POINT('',(113.552763881763,-6.65,48.8917547222302));
#197442=CARTESIAN_POINT('',(113.610006855633,-6.65,48.5972666207005));
#197443=CARTESIAN_POINT('',(113.552763881763,-6.15,48.8917547222302));
#197444=CARTESIAN_POINT('',(113.610006855633,-6.15,48.5972666207005));
#197445=CARTESIAN_POINT('Origin',(113.610006855633,-6.65,48.5972666207005));
#197446=CARTESIAN_POINT('',(113.119193353083,-6.65,48.5018616642512));
#197447=CARTESIAN_POINT('',(113.061950379214,-6.65,48.7963497657809));
#197448=CARTESIAN_POINT('',(113.119193353083,-6.65,48.5018616642512));
#197449=CARTESIAN_POINT('',(113.552763881763,-6.65,48.8917547222302));
#197450=CARTESIAN_POINT('',(113.610006855633,-6.65,48.5972666207005));
#197451=CARTESIAN_POINT('Origin',(113.119193353083,-6.65,48.5018616642512));
#197452=CARTESIAN_POINT('',(113.061950379214,-6.65,48.7963497657809));
#197453=CARTESIAN_POINT('',(113.119193353083,-6.65,48.5018616642512));
#197454=CARTESIAN_POINT('Origin',(113.904494957163,-6.15,48.65450959457));
#197455=CARTESIAN_POINT('',(114.395308459712,-6.15,48.7499145510193));
#197456=CARTESIAN_POINT('',(114.338065485842,-6.15,49.044402652549));
#197457=CARTESIAN_POINT('',(114.395308459712,-6.15,48.7499145510193));
#197458=CARTESIAN_POINT('',(113.847251983293,-6.15,48.9489976960997));
#197459=CARTESIAN_POINT('',(113.847251983293,-6.15,48.9489976960997));
#197460=CARTESIAN_POINT('',(113.904494957163,-6.15,48.65450959457));
#197461=CARTESIAN_POINT('',(113.904494957163,-6.15,48.65450959457));
#197462=CARTESIAN_POINT('',(113.904494957163,-6.15,48.65450959457));
#197463=CARTESIAN_POINT('Origin',(114.395308459712,-6.15,48.7499145510193));
#197464=CARTESIAN_POINT('',(114.395308459712,-6.65,48.7499145510193));
#197465=CARTESIAN_POINT('',(114.338065485842,-6.65,49.044402652549));
#197466=CARTESIAN_POINT('',(114.395308459712,-6.65,48.7499145510193));
#197467=CARTESIAN_POINT('',(114.338065485842,-6.15,49.044402652549));
#197468=CARTESIAN_POINT('',(114.395308459712,-6.15,48.7499145510193));
#197469=CARTESIAN_POINT('Origin',(114.395308459712,-6.65,48.7499145510193));
#197470=CARTESIAN_POINT('',(113.904494957163,-6.65,48.65450959457));
#197471=CARTESIAN_POINT('',(113.847251983293,-6.65,48.9489976960997));
#197472=CARTESIAN_POINT('',(113.904494957163,-6.65,48.65450959457));
#197473=CARTESIAN_POINT('',(114.338065485842,-6.65,49.044402652549));
#197474=CARTESIAN_POINT('',(114.395308459712,-6.65,48.7499145510193));
#197475=CARTESIAN_POINT('Origin',(113.904494957163,-6.65,48.65450959457));
#197476=CARTESIAN_POINT('',(113.847251983293,-6.65,48.9489976960997));
#197477=CARTESIAN_POINT('',(113.904494957163,-6.65,48.65450959457));
#197478=CARTESIAN_POINT('Origin',(114.689796561242,-6.15,48.8071575248888));
#197479=CARTESIAN_POINT('',(115.180610063791,-6.15,48.9025624813381));
#197480=CARTESIAN_POINT('',(115.123367089922,-6.15,49.1970505828678));
#197481=CARTESIAN_POINT('',(115.180610063791,-6.15,48.9025624813381));
#197482=CARTESIAN_POINT('',(114.632553587372,-6.15,49.1016456264185));
#197483=CARTESIAN_POINT('',(114.632553587372,-6.15,49.1016456264185));
#197484=CARTESIAN_POINT('',(114.689796561242,-6.15,48.8071575248888));
#197485=CARTESIAN_POINT('',(114.689796561242,-6.15,48.8071575248888));
#197486=CARTESIAN_POINT('',(114.689796561242,-6.15,48.8071575248888));
#197487=CARTESIAN_POINT('Origin',(115.180610063791,-6.15,48.9025624813381));
#197488=CARTESIAN_POINT('',(115.180610063791,-6.65,48.9025624813381));
#197489=CARTESIAN_POINT('',(115.123367089922,-6.65,49.1970505828678));
#197490=CARTESIAN_POINT('',(115.180610063791,-6.65,48.9025624813381));
#197491=CARTESIAN_POINT('',(115.123367089922,-6.15,49.1970505828678));
#197492=CARTESIAN_POINT('',(115.180610063791,-6.15,48.9025624813381));
#197493=CARTESIAN_POINT('Origin',(115.180610063791,-6.65,48.9025624813381));
#197494=CARTESIAN_POINT('',(114.689796561242,-6.65,48.8071575248888));
#197495=CARTESIAN_POINT('',(114.632553587372,-6.65,49.1016456264185));
#197496=CARTESIAN_POINT('',(114.689796561242,-6.65,48.8071575248888));
#197497=CARTESIAN_POINT('',(115.123367089922,-6.65,49.1970505828678));
#197498=CARTESIAN_POINT('',(115.180610063791,-6.65,48.9025624813381));
#197499=CARTESIAN_POINT('Origin',(114.689796561242,-6.65,48.8071575248888));
#197500=CARTESIAN_POINT('',(114.632553587372,-6.65,49.1016456264185));
#197501=CARTESIAN_POINT('',(114.689796561242,-6.65,48.8071575248888));
#197502=CARTESIAN_POINT('Origin',(115.475098165321,-6.15,48.9598054552076));
#197503=CARTESIAN_POINT('',(115.96591166787,-6.15,49.0552104116569));
#197504=CARTESIAN_POINT('',(115.908668694001,-6.15,49.3496985131866));
#197505=CARTESIAN_POINT('',(115.96591166787,-6.15,49.0552104116569));
#197506=CARTESIAN_POINT('',(115.417855191451,-6.15,49.2542935567373));
#197507=CARTESIAN_POINT('',(115.417855191451,-6.15,49.2542935567373));
#197508=CARTESIAN_POINT('',(115.475098165321,-6.15,48.9598054552076));
#197509=CARTESIAN_POINT('',(115.475098165321,-6.15,48.9598054552076));
#197510=CARTESIAN_POINT('',(115.475098165321,-6.15,48.9598054552076));
#197511=CARTESIAN_POINT('Origin',(115.96591166787,-6.15,49.0552104116569));
#197512=CARTESIAN_POINT('',(115.96591166787,-6.65,49.0552104116569));
#197513=CARTESIAN_POINT('',(115.908668694001,-6.65,49.3496985131866));
#197514=CARTESIAN_POINT('',(115.96591166787,-6.65,49.0552104116569));
#197515=CARTESIAN_POINT('',(115.908668694001,-6.15,49.3496985131866));
#197516=CARTESIAN_POINT('',(115.96591166787,-6.15,49.0552104116569));
#197517=CARTESIAN_POINT('Origin',(115.96591166787,-6.65,49.0552104116569));
#197518=CARTESIAN_POINT('',(115.475098165321,-6.65,48.9598054552076));
#197519=CARTESIAN_POINT('',(115.417855191451,-6.65,49.2542935567373));
#197520=CARTESIAN_POINT('',(115.475098165321,-6.65,48.9598054552076));
#197521=CARTESIAN_POINT('',(115.908668694001,-6.65,49.3496985131866));
#197522=CARTESIAN_POINT('',(115.96591166787,-6.65,49.0552104116569));
#197523=CARTESIAN_POINT('Origin',(115.475098165321,-6.65,48.9598054552076));
#197524=CARTESIAN_POINT('',(115.417855191451,-6.65,49.2542935567373));
#197525=CARTESIAN_POINT('',(115.475098165321,-6.65,48.9598054552076));
#197526=CARTESIAN_POINT('Origin',(116.2603997694,-6.15,49.1124533855264));
#197527=CARTESIAN_POINT('',(116.75121327195,-6.15,49.2078583419757));
#197528=CARTESIAN_POINT('',(116.69397029808,-6.15,49.5023464435054));
#197529=CARTESIAN_POINT('',(116.75121327195,-6.15,49.2078583419757));
#197530=CARTESIAN_POINT('',(116.203156795531,-6.15,49.4069414870561));
#197531=CARTESIAN_POINT('',(116.203156795531,-6.15,49.4069414870561));
#197532=CARTESIAN_POINT('',(116.2603997694,-6.15,49.1124533855264));
#197533=CARTESIAN_POINT('',(116.2603997694,-6.15,49.1124533855264));
#197534=CARTESIAN_POINT('',(116.2603997694,-6.15,49.1124533855264));
#197535=CARTESIAN_POINT('Origin',(116.75121327195,-6.15,49.2078583419757));
#197536=CARTESIAN_POINT('',(116.75121327195,-6.65,49.2078583419757));
#197537=CARTESIAN_POINT('',(116.69397029808,-6.65,49.5023464435054));
#197538=CARTESIAN_POINT('',(116.75121327195,-6.65,49.2078583419757));
#197539=CARTESIAN_POINT('',(116.69397029808,-6.15,49.5023464435054));
#197540=CARTESIAN_POINT('',(116.75121327195,-6.15,49.2078583419757));
#197541=CARTESIAN_POINT('Origin',(116.75121327195,-6.65,49.2078583419757));
#197542=CARTESIAN_POINT('',(116.2603997694,-6.65,49.1124533855264));
#197543=CARTESIAN_POINT('',(116.203156795531,-6.65,49.4069414870561));
#197544=CARTESIAN_POINT('',(116.2603997694,-6.65,49.1124533855264));
#197545=CARTESIAN_POINT('',(116.69397029808,-6.65,49.5023464435054));
#197546=CARTESIAN_POINT('',(116.75121327195,-6.65,49.2078583419757));
#197547=CARTESIAN_POINT('Origin',(116.2603997694,-6.65,49.1124533855264));
#197548=CARTESIAN_POINT('',(116.203156795531,-6.65,49.4069414870561));
#197549=CARTESIAN_POINT('',(116.2603997694,-6.65,49.1124533855264));
#197550=CARTESIAN_POINT('Origin',(117.045701373479,-6.15,49.2651013158452));
#197551=CARTESIAN_POINT('',(117.536514876029,-6.15,49.3605062722945));
#197552=CARTESIAN_POINT('',(117.479271902159,-6.15,49.6549943738242));
#197553=CARTESIAN_POINT('',(117.536514876029,-6.15,49.3605062722945));
#197554=CARTESIAN_POINT('',(116.98845839961,-6.15,49.5595894173749));
#197555=CARTESIAN_POINT('',(116.98845839961,-6.15,49.5595894173749));
#197556=CARTESIAN_POINT('',(117.045701373479,-6.15,49.2651013158452));
#197557=CARTESIAN_POINT('',(117.045701373479,-6.15,49.2651013158452));
#197558=CARTESIAN_POINT('',(117.045701373479,-6.15,49.2651013158452));
#197559=CARTESIAN_POINT('Origin',(117.536514876029,-6.15,49.3605062722945));
#197560=CARTESIAN_POINT('',(117.536514876029,-6.65,49.3605062722945));
#197561=CARTESIAN_POINT('',(117.479271902159,-6.65,49.6549943738242));
#197562=CARTESIAN_POINT('',(117.536514876029,-6.65,49.3605062722945));
#197563=CARTESIAN_POINT('',(117.479271902159,-6.15,49.6549943738242));
#197564=CARTESIAN_POINT('',(117.536514876029,-6.15,49.3605062722945));
#197565=CARTESIAN_POINT('Origin',(117.536514876029,-6.65,49.3605062722945));
#197566=CARTESIAN_POINT('',(117.045701373479,-6.65,49.2651013158452));
#197567=CARTESIAN_POINT('',(116.98845839961,-6.65,49.5595894173749));
#197568=CARTESIAN_POINT('',(117.045701373479,-6.65,49.2651013158452));
#197569=CARTESIAN_POINT('',(117.479271902159,-6.65,49.6549943738242));
#197570=CARTESIAN_POINT('',(117.536514876029,-6.65,49.3605062722945));
#197571=CARTESIAN_POINT('Origin',(117.045701373479,-6.65,49.2651013158452));
#197572=CARTESIAN_POINT('',(116.98845839961,-6.65,49.5595894173749));
#197573=CARTESIAN_POINT('',(117.045701373479,-6.65,49.2651013158452));
#197574=CARTESIAN_POINT('Origin',(117.831002977559,-6.15,49.417749246164));
#197575=CARTESIAN_POINT('',(118.321816480108,-6.15,49.5131542026133));
#197576=CARTESIAN_POINT('',(118.264573506239,-6.15,49.807642304143));
#197577=CARTESIAN_POINT('',(118.321816480108,-6.15,49.5131542026133));
#197578=CARTESIAN_POINT('',(117.773760003689,-6.15,49.7122373476937));
#197579=CARTESIAN_POINT('',(117.773760003689,-6.15,49.7122373476937));
#197580=CARTESIAN_POINT('',(117.831002977559,-6.15,49.417749246164));
#197581=CARTESIAN_POINT('',(117.831002977559,-6.15,49.417749246164));
#197582=CARTESIAN_POINT('',(117.831002977559,-6.15,49.417749246164));
#197583=CARTESIAN_POINT('Origin',(118.321816480108,-6.15,49.5131542026133));
#197584=CARTESIAN_POINT('',(118.321816480108,-6.65,49.5131542026133));
#197585=CARTESIAN_POINT('',(118.264573506239,-6.65,49.807642304143));
#197586=CARTESIAN_POINT('',(118.321816480108,-6.65,49.5131542026133));
#197587=CARTESIAN_POINT('',(118.264573506239,-6.15,49.807642304143));
#197588=CARTESIAN_POINT('',(118.321816480108,-6.15,49.5131542026133));
#197589=CARTESIAN_POINT('Origin',(118.321816480108,-6.65,49.5131542026133));
#197590=CARTESIAN_POINT('',(117.831002977559,-6.65,49.417749246164));
#197591=CARTESIAN_POINT('',(117.773760003689,-6.65,49.7122373476937));
#197592=CARTESIAN_POINT('',(117.831002977559,-6.65,49.417749246164));
#197593=CARTESIAN_POINT('',(118.264573506239,-6.65,49.807642304143));
#197594=CARTESIAN_POINT('',(118.321816480108,-6.65,49.5131542026133));
#197595=CARTESIAN_POINT('Origin',(117.831002977559,-6.65,49.417749246164));
#197596=CARTESIAN_POINT('',(117.773760003689,-6.65,49.7122373476937));
#197597=CARTESIAN_POINT('',(117.831002977559,-6.65,49.417749246164));
#197598=CARTESIAN_POINT('Origin',(118.616304581638,-6.15,49.5703971764828));
#197599=CARTESIAN_POINT('',(119.107118084187,-6.15,49.6658021329321));
#197600=CARTESIAN_POINT('',(119.049875110318,-6.15,49.9602902344618));
#197601=CARTESIAN_POINT('',(119.107118084187,-6.15,49.6658021329321));
#197602=CARTESIAN_POINT('',(118.559061607768,-6.15,49.8648852780125));
#197603=CARTESIAN_POINT('',(118.559061607768,-6.15,49.8648852780125));
#197604=CARTESIAN_POINT('',(118.616304581638,-6.15,49.5703971764828));
#197605=CARTESIAN_POINT('',(118.616304581638,-6.15,49.5703971764828));
#197606=CARTESIAN_POINT('',(118.616304581638,-6.15,49.5703971764828));
#197607=CARTESIAN_POINT('Origin',(119.107118084187,-6.15,49.6658021329321));
#197608=CARTESIAN_POINT('',(119.107118084187,-6.65,49.6658021329321));
#197609=CARTESIAN_POINT('',(119.049875110318,-6.65,49.9602902344618));
#197610=CARTESIAN_POINT('',(119.107118084187,-6.65,49.6658021329321));
#197611=CARTESIAN_POINT('',(119.049875110318,-6.15,49.9602902344618));
#197612=CARTESIAN_POINT('',(119.107118084187,-6.15,49.6658021329321));
#197613=CARTESIAN_POINT('Origin',(119.107118084187,-6.65,49.6658021329321));
#197614=CARTESIAN_POINT('',(118.616304581638,-6.65,49.5703971764828));
#197615=CARTESIAN_POINT('',(118.559061607768,-6.65,49.8648852780125));
#197616=CARTESIAN_POINT('',(118.616304581638,-6.65,49.5703971764828));
#197617=CARTESIAN_POINT('',(119.049875110318,-6.65,49.9602902344618));
#197618=CARTESIAN_POINT('',(119.107118084187,-6.65,49.6658021329321));
#197619=CARTESIAN_POINT('Origin',(118.616304581638,-6.65,49.5703971764828));
#197620=CARTESIAN_POINT('',(118.559061607768,-6.65,49.8648852780125));
#197621=CARTESIAN_POINT('',(118.616304581638,-6.65,49.5703971764828));
#197622=CARTESIAN_POINT('Origin',(119.401606185717,-6.15,49.7230451068016));
#197623=CARTESIAN_POINT('',(119.892419688267,-6.15,49.8184500632509));
#197624=CARTESIAN_POINT('',(119.835176714397,-6.15,50.1129381647806));
#197625=CARTESIAN_POINT('',(119.892419688267,-6.15,49.8184500632509));
#197626=CARTESIAN_POINT('',(119.344363211847,-6.15,50.0175332083313));
#197627=CARTESIAN_POINT('',(119.344363211847,-6.15,50.0175332083313));
#197628=CARTESIAN_POINT('',(119.401606185717,-6.15,49.7230451068016));
#197629=CARTESIAN_POINT('',(119.401606185717,-6.15,49.7230451068016));
#197630=CARTESIAN_POINT('',(119.401606185717,-6.15,49.7230451068016));
#197631=CARTESIAN_POINT('Origin',(119.892419688267,-6.15,49.8184500632509));
#197632=CARTESIAN_POINT('',(119.892419688267,-6.65,49.8184500632509));
#197633=CARTESIAN_POINT('',(119.835176714397,-6.65,50.1129381647806));
#197634=CARTESIAN_POINT('',(119.892419688267,-6.65,49.8184500632509));
#197635=CARTESIAN_POINT('',(119.835176714397,-6.15,50.1129381647806));
#197636=CARTESIAN_POINT('',(119.892419688267,-6.15,49.8184500632509));
#197637=CARTESIAN_POINT('Origin',(119.892419688267,-6.65,49.8184500632509));
#197638=CARTESIAN_POINT('',(119.401606185717,-6.65,49.7230451068016));
#197639=CARTESIAN_POINT('',(119.344363211847,-6.65,50.0175332083313));
#197640=CARTESIAN_POINT('',(119.401606185717,-6.65,49.7230451068016));
#197641=CARTESIAN_POINT('',(119.835176714397,-6.65,50.1129381647806));
#197642=CARTESIAN_POINT('',(119.892419688267,-6.65,49.8184500632509));
#197643=CARTESIAN_POINT('Origin',(119.401606185717,-6.65,49.7230451068016));
#197644=CARTESIAN_POINT('',(119.344363211847,-6.65,50.0175332083313));
#197645=CARTESIAN_POINT('',(119.401606185717,-6.65,49.7230451068016));
#197646=CARTESIAN_POINT('Origin',(120.186907789796,-6.15,49.8756930371204));
#197647=CARTESIAN_POINT('',(120.677721292346,-6.15,49.9710979935697));
#197648=CARTESIAN_POINT('',(120.620478318476,-6.15,50.2655860950994));
#197649=CARTESIAN_POINT('',(120.677721292346,-6.15,49.9710979935697));
#197650=CARTESIAN_POINT('',(120.129664815927,-6.15,50.1701811386501));
#197651=CARTESIAN_POINT('',(120.129664815927,-6.15,50.1701811386501));
#197652=CARTESIAN_POINT('',(120.186907789796,-6.15,49.8756930371204));
#197653=CARTESIAN_POINT('',(120.186907789796,-6.15,49.8756930371204));
#197654=CARTESIAN_POINT('',(120.186907789796,-6.15,49.8756930371204));
#197655=CARTESIAN_POINT('Origin',(120.677721292346,-6.15,49.9710979935697));
#197656=CARTESIAN_POINT('',(120.677721292346,-6.65,49.9710979935697));
#197657=CARTESIAN_POINT('',(120.620478318476,-6.65,50.2655860950994));
#197658=CARTESIAN_POINT('',(120.677721292346,-6.65,49.9710979935697));
#197659=CARTESIAN_POINT('',(120.620478318476,-6.15,50.2655860950994));
#197660=CARTESIAN_POINT('',(120.677721292346,-6.15,49.9710979935697));
#197661=CARTESIAN_POINT('Origin',(120.677721292346,-6.65,49.9710979935697));
#197662=CARTESIAN_POINT('',(120.186907789796,-6.65,49.8756930371204));
#197663=CARTESIAN_POINT('',(120.129664815927,-6.65,50.1701811386501));
#197664=CARTESIAN_POINT('',(120.186907789796,-6.65,49.8756930371204));
#197665=CARTESIAN_POINT('',(120.620478318476,-6.65,50.2655860950994));
#197666=CARTESIAN_POINT('',(120.677721292346,-6.65,49.9710979935697));
#197667=CARTESIAN_POINT('Origin',(120.186907789796,-6.65,49.8756930371204));
#197668=CARTESIAN_POINT('',(120.129664815927,-6.65,50.1701811386501));
#197669=CARTESIAN_POINT('',(120.186907789796,-6.65,49.8756930371204));
#197670=CARTESIAN_POINT('Origin',(120.972209393875,-6.15,50.0283409674392));
#197671=CARTESIAN_POINT('',(121.463022896425,-6.15,50.1237459238885));
#197672=CARTESIAN_POINT('',(121.405779922555,-6.15,50.4182340254182));
#197673=CARTESIAN_POINT('',(121.463022896425,-6.15,50.1237459238885));
#197674=CARTESIAN_POINT('',(120.914966420006,-6.15,50.3228290689689));
#197675=CARTESIAN_POINT('',(120.914966420006,-6.15,50.3228290689689));
#197676=CARTESIAN_POINT('',(120.972209393875,-6.15,50.0283409674392));
#197677=CARTESIAN_POINT('',(120.972209393875,-6.15,50.0283409674392));
#197678=CARTESIAN_POINT('',(120.972209393875,-6.15,50.0283409674392));
#197679=CARTESIAN_POINT('Origin',(121.463022896425,-6.15,50.1237459238885));
#197680=CARTESIAN_POINT('',(121.463022896425,-6.65,50.1237459238885));
#197681=CARTESIAN_POINT('',(121.405779922555,-6.65,50.4182340254182));
#197682=CARTESIAN_POINT('',(121.463022896425,-6.65,50.1237459238885));
#197683=CARTESIAN_POINT('',(121.405779922555,-6.15,50.4182340254182));
#197684=CARTESIAN_POINT('',(121.463022896425,-6.15,50.1237459238885));
#197685=CARTESIAN_POINT('Origin',(121.463022896425,-6.65,50.1237459238885));
#197686=CARTESIAN_POINT('',(120.972209393875,-6.65,50.0283409674392));
#197687=CARTESIAN_POINT('',(120.914966420006,-6.65,50.3228290689689));
#197688=CARTESIAN_POINT('',(120.972209393875,-6.65,50.0283409674392));
#197689=CARTESIAN_POINT('',(121.405779922555,-6.65,50.4182340254182));
#197690=CARTESIAN_POINT('',(121.463022896425,-6.65,50.1237459238885));
#197691=CARTESIAN_POINT('Origin',(120.972209393875,-6.65,50.0283409674392));
#197692=CARTESIAN_POINT('',(120.914966420006,-6.65,50.3228290689689));
#197693=CARTESIAN_POINT('',(120.972209393875,-6.65,50.0283409674392));
#197694=CARTESIAN_POINT('Origin',(121.757510997955,-6.15,50.180988897758));
#197695=CARTESIAN_POINT('',(122.248324500504,-6.15,50.2763938542073));
#197696=CARTESIAN_POINT('',(122.191081526635,-6.15,50.570881955737));
#197697=CARTESIAN_POINT('',(122.248324500504,-6.15,50.2763938542073));
#197698=CARTESIAN_POINT('',(121.700268024085,-6.15,50.4754769992877));
#197699=CARTESIAN_POINT('',(121.700268024085,-6.15,50.4754769992877));
#197700=CARTESIAN_POINT('',(121.757510997955,-6.15,50.180988897758));
#197701=CARTESIAN_POINT('',(121.757510997955,-6.15,50.180988897758));
#197702=CARTESIAN_POINT('',(121.757510997955,-6.15,50.180988897758));
#197703=CARTESIAN_POINT('Origin',(122.248324500504,-6.15,50.2763938542073));
#197704=CARTESIAN_POINT('',(122.248324500504,-6.65,50.2763938542073));
#197705=CARTESIAN_POINT('',(122.191081526635,-6.65,50.570881955737));
#197706=CARTESIAN_POINT('',(122.248324500504,-6.65,50.2763938542073));
#197707=CARTESIAN_POINT('',(122.191081526635,-6.15,50.570881955737));
#197708=CARTESIAN_POINT('',(122.248324500504,-6.15,50.2763938542073));
#197709=CARTESIAN_POINT('Origin',(122.248324500504,-6.65,50.2763938542073));
#197710=CARTESIAN_POINT('',(121.757510997955,-6.65,50.180988897758));
#197711=CARTESIAN_POINT('',(121.700268024085,-6.65,50.4754769992877));
#197712=CARTESIAN_POINT('',(121.757510997955,-6.65,50.180988897758));
#197713=CARTESIAN_POINT('',(122.191081526635,-6.65,50.570881955737));
#197714=CARTESIAN_POINT('',(122.248324500504,-6.65,50.2763938542073));
#197715=CARTESIAN_POINT('Origin',(121.757510997955,-6.65,50.180988897758));
#197716=CARTESIAN_POINT('',(121.700268024085,-6.65,50.4754769992877));
#197717=CARTESIAN_POINT('',(121.757510997955,-6.65,50.180988897758));
#197718=CARTESIAN_POINT('Origin',(122.542812602034,-6.15,50.3336368280768));
#197719=CARTESIAN_POINT('',(123.033626104583,-6.15,50.4290417845261));
#197720=CARTESIAN_POINT('',(122.976383130714,-6.15,50.7235298860558));
#197721=CARTESIAN_POINT('',(123.033626104583,-6.15,50.4290417845261));
#197722=CARTESIAN_POINT('',(122.485569628164,-6.15,50.6281249296065));
#197723=CARTESIAN_POINT('',(122.485569628164,-6.15,50.6281249296065));
#197724=CARTESIAN_POINT('',(122.542812602034,-6.15,50.3336368280768));
#197725=CARTESIAN_POINT('',(122.542812602034,-6.15,50.3336368280768));
#197726=CARTESIAN_POINT('',(122.542812602034,-6.15,50.3336368280768));
#197727=CARTESIAN_POINT('Origin',(123.033626104583,-6.15,50.4290417845261));
#197728=CARTESIAN_POINT('',(123.033626104583,-6.65,50.4290417845261));
#197729=CARTESIAN_POINT('',(122.976383130714,-6.65,50.7235298860558));
#197730=CARTESIAN_POINT('',(123.033626104583,-6.65,50.4290417845261));
#197731=CARTESIAN_POINT('',(122.976383130714,-6.15,50.7235298860558));
#197732=CARTESIAN_POINT('',(123.033626104583,-6.15,50.4290417845261));
#197733=CARTESIAN_POINT('Origin',(123.033626104583,-6.65,50.4290417845261));
#197734=CARTESIAN_POINT('',(122.542812602034,-6.65,50.3336368280768));
#197735=CARTESIAN_POINT('',(122.485569628164,-6.65,50.6281249296065));
#197736=CARTESIAN_POINT('',(122.542812602034,-6.65,50.3336368280768));
#197737=CARTESIAN_POINT('',(122.976383130714,-6.65,50.7235298860558));
#197738=CARTESIAN_POINT('',(123.033626104583,-6.65,50.4290417845261));
#197739=CARTESIAN_POINT('Origin',(122.542812602034,-6.65,50.3336368280768));
#197740=CARTESIAN_POINT('',(122.485569628164,-6.65,50.6281249296065));
#197741=CARTESIAN_POINT('',(122.542812602034,-6.65,50.3336368280768));
#197742=CARTESIAN_POINT('Origin',(123.328114206113,-6.15,50.4862847583956));
#197743=CARTESIAN_POINT('',(123.818927708663,-6.15,50.5816897148449));
#197744=CARTESIAN_POINT('',(123.761684734793,-6.15,50.8761778163746));
#197745=CARTESIAN_POINT('',(123.818927708663,-6.15,50.5816897148449));
#197746=CARTESIAN_POINT('',(123.270871232244,-6.15,50.7807728599253));
#197747=CARTESIAN_POINT('',(123.270871232244,-6.15,50.7807728599253));
#197748=CARTESIAN_POINT('',(123.328114206113,-6.15,50.4862847583956));
#197749=CARTESIAN_POINT('',(123.328114206113,-6.15,50.4862847583956));
#197750=CARTESIAN_POINT('',(123.328114206113,-6.15,50.4862847583956));
#197751=CARTESIAN_POINT('Origin',(123.818927708663,-6.15,50.5816897148449));
#197752=CARTESIAN_POINT('',(123.818927708663,-6.65,50.5816897148449));
#197753=CARTESIAN_POINT('',(123.761684734793,-6.65,50.8761778163746));
#197754=CARTESIAN_POINT('',(123.818927708663,-6.65,50.5816897148449));
#197755=CARTESIAN_POINT('',(123.761684734793,-6.15,50.8761778163746));
#197756=CARTESIAN_POINT('',(123.818927708663,-6.15,50.5816897148449));
#197757=CARTESIAN_POINT('Origin',(123.818927708663,-6.65,50.5816897148449));
#197758=CARTESIAN_POINT('',(123.328114206113,-6.65,50.4862847583956));
#197759=CARTESIAN_POINT('',(123.270871232244,-6.65,50.7807728599253));
#197760=CARTESIAN_POINT('',(123.328114206113,-6.65,50.4862847583956));
#197761=CARTESIAN_POINT('',(123.761684734793,-6.65,50.8761778163746));
#197762=CARTESIAN_POINT('',(123.818927708663,-6.65,50.5816897148449));
#197763=CARTESIAN_POINT('Origin',(123.328114206113,-6.65,50.4862847583956));
#197764=CARTESIAN_POINT('',(123.270871232244,-6.65,50.7807728599253));
#197765=CARTESIAN_POINT('',(123.328114206113,-6.65,50.4862847583956));
#197766=CARTESIAN_POINT('Origin',(123.328114206113,-5.35,50.4862847583956));
#197767=CARTESIAN_POINT('',(123.818927708663,-5.35,50.5816897148449));
#197768=CARTESIAN_POINT('',(123.761684734793,-5.35,50.8761778163746));
#197769=CARTESIAN_POINT('',(123.818927708663,-5.35,50.5816897148449));
#197770=CARTESIAN_POINT('',(123.270871232244,-5.35,50.7807728599253));
#197771=CARTESIAN_POINT('',(123.270871232244,-5.35,50.7807728599253));
#197772=CARTESIAN_POINT('',(123.328114206113,-5.35,50.4862847583956));
#197773=CARTESIAN_POINT('',(123.328114206113,-5.35,50.4862847583956));
#197774=CARTESIAN_POINT('',(123.328114206113,-5.35,50.4862847583956));
#197775=CARTESIAN_POINT('Origin',(123.818927708663,-5.35,50.5816897148449));
#197776=CARTESIAN_POINT('',(123.818927708663,-5.85,50.5816897148449));
#197777=CARTESIAN_POINT('',(123.761684734793,-5.85,50.8761778163746));
#197778=CARTESIAN_POINT('',(123.818927708663,-5.85,50.5816897148449));
#197779=CARTESIAN_POINT('',(123.761684734793,-5.35,50.8761778163746));
#197780=CARTESIAN_POINT('',(123.818927708663,-5.35,50.5816897148449));
#197781=CARTESIAN_POINT('Origin',(123.818927708663,-5.85,50.5816897148449));
#197782=CARTESIAN_POINT('',(123.328114206113,-5.85,50.4862847583956));
#197783=CARTESIAN_POINT('',(123.270871232244,-5.85,50.7807728599253));
#197784=CARTESIAN_POINT('',(123.328114206113,-5.85,50.4862847583956));
#197785=CARTESIAN_POINT('',(123.761684734793,-5.85,50.8761778163746));
#197786=CARTESIAN_POINT('',(123.818927708663,-5.85,50.5816897148449));
#197787=CARTESIAN_POINT('Origin',(123.328114206113,-5.85,50.4862847583956));
#197788=CARTESIAN_POINT('',(123.270871232244,-5.85,50.7807728599253));
#197789=CARTESIAN_POINT('',(123.328114206113,-5.85,50.4862847583956));
#197790=CARTESIAN_POINT('Origin',(123.328114206113,-4.55,50.4862847583956));
#197791=CARTESIAN_POINT('',(123.818927708663,-4.55,50.5816897148449));
#197792=CARTESIAN_POINT('',(123.761684734793,-4.55,50.8761778163746));
#197793=CARTESIAN_POINT('',(123.818927708663,-4.55,50.5816897148449));
#197794=CARTESIAN_POINT('',(123.270871232244,-4.55,50.7807728599253));
#197795=CARTESIAN_POINT('',(123.270871232244,-4.55,50.7807728599253));
#197796=CARTESIAN_POINT('',(123.328114206113,-4.55,50.4862847583956));
#197797=CARTESIAN_POINT('',(123.328114206113,-4.55,50.4862847583956));
#197798=CARTESIAN_POINT('',(123.328114206113,-4.55,50.4862847583956));
#197799=CARTESIAN_POINT('Origin',(123.818927708663,-4.55,50.5816897148449));
#197800=CARTESIAN_POINT('',(123.818927708663,-5.05,50.5816897148449));
#197801=CARTESIAN_POINT('',(123.761684734793,-5.05,50.8761778163746));
#197802=CARTESIAN_POINT('',(123.818927708663,-5.05,50.5816897148449));
#197803=CARTESIAN_POINT('',(123.761684734793,-4.55,50.8761778163746));
#197804=CARTESIAN_POINT('',(123.818927708663,-4.55,50.5816897148449));
#197805=CARTESIAN_POINT('Origin',(123.818927708663,-5.05,50.5816897148449));
#197806=CARTESIAN_POINT('',(123.328114206113,-5.05,50.4862847583956));
#197807=CARTESIAN_POINT('',(123.270871232244,-5.05,50.7807728599253));
#197808=CARTESIAN_POINT('',(123.328114206113,-5.05,50.4862847583956));
#197809=CARTESIAN_POINT('',(123.761684734793,-5.05,50.8761778163746));
#197810=CARTESIAN_POINT('',(123.818927708663,-5.05,50.5816897148449));
#197811=CARTESIAN_POINT('Origin',(123.328114206113,-5.05,50.4862847583956));
#197812=CARTESIAN_POINT('',(123.270871232244,-5.05,50.7807728599253));
#197813=CARTESIAN_POINT('',(123.328114206113,-5.05,50.4862847583956));
#197814=CARTESIAN_POINT('Origin',(123.328114206113,-3.75,50.4862847583956));
#197815=CARTESIAN_POINT('',(123.818927708663,-3.75,50.5816897148449));
#197816=CARTESIAN_POINT('',(123.761684734793,-3.75,50.8761778163746));
#197817=CARTESIAN_POINT('',(123.818927708663,-3.75,50.5816897148449));
#197818=CARTESIAN_POINT('',(123.270871232244,-3.75,50.7807728599253));
#197819=CARTESIAN_POINT('',(123.270871232244,-3.75,50.7807728599253));
#197820=CARTESIAN_POINT('',(123.328114206113,-3.75,50.4862847583956));
#197821=CARTESIAN_POINT('',(123.328114206113,-3.75,50.4862847583956));
#197822=CARTESIAN_POINT('',(123.328114206113,-3.75,50.4862847583956));
#197823=CARTESIAN_POINT('Origin',(123.818927708663,-3.75,50.5816897148449));
#197824=CARTESIAN_POINT('',(123.818927708663,-4.25,50.5816897148449));
#197825=CARTESIAN_POINT('',(123.761684734793,-4.25,50.8761778163746));
#197826=CARTESIAN_POINT('',(123.818927708663,-4.25,50.5816897148449));
#197827=CARTESIAN_POINT('',(123.761684734793,-3.75,50.8761778163746));
#197828=CARTESIAN_POINT('',(123.818927708663,-3.75,50.5816897148449));
#197829=CARTESIAN_POINT('Origin',(123.818927708663,-4.25,50.5816897148449));
#197830=CARTESIAN_POINT('',(123.328114206113,-4.25,50.4862847583956));
#197831=CARTESIAN_POINT('',(123.270871232244,-4.25,50.7807728599253));
#197832=CARTESIAN_POINT('',(123.328114206113,-4.25,50.4862847583956));
#197833=CARTESIAN_POINT('',(123.761684734793,-4.25,50.8761778163746));
#197834=CARTESIAN_POINT('',(123.818927708663,-4.25,50.5816897148449));
#197835=CARTESIAN_POINT('Origin',(123.328114206113,-4.25,50.4862847583956));
#197836=CARTESIAN_POINT('',(123.270871232244,-4.25,50.7807728599253));
#197837=CARTESIAN_POINT('',(123.328114206113,-4.25,50.4862847583956));
#197838=CARTESIAN_POINT('Origin',(123.328114206113,-2.95,50.4862847583956));
#197839=CARTESIAN_POINT('',(123.818927708663,-2.95,50.5816897148449));
#197840=CARTESIAN_POINT('',(123.761684734793,-2.95,50.8761778163746));
#197841=CARTESIAN_POINT('',(123.818927708663,-2.95,50.5816897148449));
#197842=CARTESIAN_POINT('',(123.270871232244,-2.95,50.7807728599253));
#197843=CARTESIAN_POINT('',(123.270871232244,-2.95,50.7807728599253));
#197844=CARTESIAN_POINT('',(123.328114206113,-2.95,50.4862847583956));
#197845=CARTESIAN_POINT('',(123.328114206113,-2.95,50.4862847583956));
#197846=CARTESIAN_POINT('',(123.328114206113,-2.95,50.4862847583956));
#197847=CARTESIAN_POINT('Origin',(123.818927708663,-2.95,50.5816897148449));
#197848=CARTESIAN_POINT('',(123.818927708663,-3.45,50.5816897148449));
#197849=CARTESIAN_POINT('',(123.761684734793,-3.45,50.8761778163746));
#197850=CARTESIAN_POINT('',(123.818927708663,-3.45,50.5816897148449));
#197851=CARTESIAN_POINT('',(123.761684734793,-2.95,50.8761778163746));
#197852=CARTESIAN_POINT('',(123.818927708663,-2.95,50.5816897148449));
#197853=CARTESIAN_POINT('Origin',(123.818927708663,-3.45,50.5816897148449));
#197854=CARTESIAN_POINT('',(123.328114206113,-3.45,50.4862847583956));
#197855=CARTESIAN_POINT('',(123.270871232244,-3.45,50.7807728599253));
#197856=CARTESIAN_POINT('',(123.328114206113,-3.45,50.4862847583956));
#197857=CARTESIAN_POINT('',(123.761684734793,-3.45,50.8761778163746));
#197858=CARTESIAN_POINT('',(123.818927708663,-3.45,50.5816897148449));
#197859=CARTESIAN_POINT('Origin',(123.328114206113,-3.45,50.4862847583956));
#197860=CARTESIAN_POINT('',(123.270871232244,-3.45,50.7807728599253));
#197861=CARTESIAN_POINT('',(123.328114206113,-3.45,50.4862847583956));
#197862=CARTESIAN_POINT('Origin',(123.328114206113,-2.15,50.4862847583956));
#197863=CARTESIAN_POINT('',(123.818927708663,-2.15,50.5816897148449));
#197864=CARTESIAN_POINT('',(123.761684734793,-2.15,50.8761778163746));
#197865=CARTESIAN_POINT('',(123.818927708663,-2.15,50.5816897148449));
#197866=CARTESIAN_POINT('',(123.270871232244,-2.15,50.7807728599253));
#197867=CARTESIAN_POINT('',(123.270871232244,-2.15,50.7807728599253));
#197868=CARTESIAN_POINT('',(123.328114206113,-2.15,50.4862847583956));
#197869=CARTESIAN_POINT('',(123.328114206113,-2.15,50.4862847583956));
#197870=CARTESIAN_POINT('',(123.328114206113,-2.15,50.4862847583956));
#197871=CARTESIAN_POINT('Origin',(123.818927708663,-2.15,50.5816897148449));
#197872=CARTESIAN_POINT('',(123.818927708663,-2.65,50.5816897148449));
#197873=CARTESIAN_POINT('',(123.761684734793,-2.65,50.8761778163746));
#197874=CARTESIAN_POINT('',(123.818927708663,-2.65,50.5816897148449));
#197875=CARTESIAN_POINT('',(123.761684734793,-2.15,50.8761778163746));
#197876=CARTESIAN_POINT('',(123.818927708663,-2.15,50.5816897148449));
#197877=CARTESIAN_POINT('Origin',(123.818927708663,-2.65,50.5816897148449));
#197878=CARTESIAN_POINT('',(123.328114206113,-2.65,50.4862847583956));
#197879=CARTESIAN_POINT('',(123.270871232244,-2.65,50.7807728599253));
#197880=CARTESIAN_POINT('',(123.328114206113,-2.65,50.4862847583956));
#197881=CARTESIAN_POINT('',(123.761684734793,-2.65,50.8761778163746));
#197882=CARTESIAN_POINT('',(123.818927708663,-2.65,50.5816897148449));
#197883=CARTESIAN_POINT('Origin',(123.328114206113,-2.65,50.4862847583956));
#197884=CARTESIAN_POINT('',(123.270871232244,-2.65,50.7807728599253));
#197885=CARTESIAN_POINT('',(123.328114206113,-2.65,50.4862847583956));
#197886=CARTESIAN_POINT('Origin',(123.328114206113,-1.35,50.4862847583956));
#197887=CARTESIAN_POINT('',(123.818927708663,-1.35,50.5816897148449));
#197888=CARTESIAN_POINT('',(123.761684734793,-1.35,50.8761778163746));
#197889=CARTESIAN_POINT('',(123.818927708663,-1.35,50.5816897148449));
#197890=CARTESIAN_POINT('',(123.270871232244,-1.35,50.7807728599253));
#197891=CARTESIAN_POINT('',(123.270871232244,-1.35,50.7807728599253));
#197892=CARTESIAN_POINT('',(123.328114206113,-1.35,50.4862847583956));
#197893=CARTESIAN_POINT('',(123.328114206113,-1.35,50.4862847583956));
#197894=CARTESIAN_POINT('',(123.328114206113,-1.35,50.4862847583956));
#197895=CARTESIAN_POINT('Origin',(123.818927708663,-1.35,50.5816897148449));
#197896=CARTESIAN_POINT('',(123.818927708663,-1.85,50.5816897148449));
#197897=CARTESIAN_POINT('',(123.761684734793,-1.85,50.8761778163746));
#197898=CARTESIAN_POINT('',(123.818927708663,-1.85,50.5816897148449));
#197899=CARTESIAN_POINT('',(123.761684734793,-1.35,50.8761778163746));
#197900=CARTESIAN_POINT('',(123.818927708663,-1.35,50.5816897148449));
#197901=CARTESIAN_POINT('Origin',(123.818927708663,-1.85,50.5816897148449));
#197902=CARTESIAN_POINT('',(123.328114206113,-1.85,50.4862847583956));
#197903=CARTESIAN_POINT('',(123.270871232244,-1.85,50.7807728599253));
#197904=CARTESIAN_POINT('',(123.328114206113,-1.85,50.4862847583956));
#197905=CARTESIAN_POINT('',(123.761684734793,-1.85,50.8761778163746));
#197906=CARTESIAN_POINT('',(123.818927708663,-1.85,50.5816897148449));
#197907=CARTESIAN_POINT('Origin',(123.328114206113,-1.85,50.4862847583956));
#197908=CARTESIAN_POINT('',(123.270871232244,-1.85,50.7807728599253));
#197909=CARTESIAN_POINT('',(123.328114206113,-1.85,50.4862847583956));
#197910=CARTESIAN_POINT('Origin',(123.328114206113,-0.549999999999986,50.4862847583956));
#197911=CARTESIAN_POINT('',(123.818927708663,-0.549999999999986,50.5816897148449));
#197912=CARTESIAN_POINT('',(123.761684734793,-0.549999999999986,50.8761778163746));
#197913=CARTESIAN_POINT('',(123.818927708663,-0.549999999999986,50.5816897148449));
#197914=CARTESIAN_POINT('',(123.270871232244,-0.549999999999986,50.7807728599253));
#197915=CARTESIAN_POINT('',(123.270871232244,-0.549999999999986,50.7807728599253));
#197916=CARTESIAN_POINT('',(123.328114206113,-0.549999999999986,50.4862847583956));
#197917=CARTESIAN_POINT('',(123.328114206113,-0.549999999999986,50.4862847583956));
#197918=CARTESIAN_POINT('',(123.328114206113,-0.549999999999986,50.4862847583956));
#197919=CARTESIAN_POINT('Origin',(123.818927708663,-0.549999999999986,50.5816897148449));
#197920=CARTESIAN_POINT('',(123.818927708663,-1.05,50.5816897148449));
#197921=CARTESIAN_POINT('',(123.761684734793,-1.05,50.8761778163746));
#197922=CARTESIAN_POINT('',(123.818927708663,-1.05,50.5816897148449));
#197923=CARTESIAN_POINT('',(123.761684734793,-0.549999999999986,50.8761778163746));
#197924=CARTESIAN_POINT('',(123.818927708663,-0.549999999999986,50.5816897148449));
#197925=CARTESIAN_POINT('Origin',(123.818927708663,-1.05,50.5816897148449));
#197926=CARTESIAN_POINT('',(123.328114206113,-1.05,50.4862847583956));
#197927=CARTESIAN_POINT('',(123.270871232244,-1.05,50.7807728599253));
#197928=CARTESIAN_POINT('',(123.328114206113,-1.05,50.4862847583956));
#197929=CARTESIAN_POINT('',(123.761684734793,-1.05,50.8761778163746));
#197930=CARTESIAN_POINT('',(123.818927708663,-1.05,50.5816897148449));
#197931=CARTESIAN_POINT('Origin',(123.328114206113,-1.05,50.4862847583956));
#197932=CARTESIAN_POINT('',(123.270871232244,-1.05,50.7807728599253));
#197933=CARTESIAN_POINT('',(123.328114206113,-1.05,50.4862847583956));
#197934=CARTESIAN_POINT('Origin',(123.328114206113,0.250000000000015,50.4862847583956));
#197935=CARTESIAN_POINT('',(123.818927708663,0.250000000000015,50.5816897148449));
#197936=CARTESIAN_POINT('',(123.761684734793,0.250000000000015,50.8761778163746));
#197937=CARTESIAN_POINT('',(123.818927708663,0.250000000000015,50.5816897148449));
#197938=CARTESIAN_POINT('',(123.270871232244,0.250000000000015,50.7807728599253));
#197939=CARTESIAN_POINT('',(123.270871232244,0.250000000000015,50.7807728599253));
#197940=CARTESIAN_POINT('',(123.328114206113,0.250000000000015,50.4862847583956));
#197941=CARTESIAN_POINT('',(123.328114206113,0.250000000000015,50.4862847583956));
#197942=CARTESIAN_POINT('',(123.328114206113,0.250000000000015,50.4862847583956));
#197943=CARTESIAN_POINT('Origin',(123.818927708663,0.250000000000015,50.5816897148449));
#197944=CARTESIAN_POINT('',(123.818927708663,-0.249999999999985,50.5816897148449));
#197945=CARTESIAN_POINT('',(123.761684734793,-0.249999999999985,50.8761778163746));
#197946=CARTESIAN_POINT('',(123.818927708663,-0.249999999999985,50.5816897148449));
#197947=CARTESIAN_POINT('',(123.761684734793,0.250000000000015,50.8761778163746));
#197948=CARTESIAN_POINT('',(123.818927708663,0.250000000000015,50.5816897148449));
#197949=CARTESIAN_POINT('Origin',(123.818927708663,-0.249999999999985,50.5816897148449));
#197950=CARTESIAN_POINT('',(123.328114206113,-0.249999999999985,50.4862847583956));
#197951=CARTESIAN_POINT('',(123.270871232244,-0.249999999999985,50.7807728599253));
#197952=CARTESIAN_POINT('',(123.328114206113,-0.249999999999985,50.4862847583956));
#197953=CARTESIAN_POINT('',(123.761684734793,-0.249999999999985,50.8761778163746));
#197954=CARTESIAN_POINT('',(123.818927708663,-0.249999999999985,50.5816897148449));
#197955=CARTESIAN_POINT('Origin',(123.328114206113,-0.249999999999985,50.4862847583956));
#197956=CARTESIAN_POINT('',(123.270871232244,-0.249999999999985,50.7807728599253));
#197957=CARTESIAN_POINT('',(123.328114206113,-0.249999999999985,50.4862847583956));
#197958=CARTESIAN_POINT('Origin',(123.328114206113,1.05,50.4862847583956));
#197959=CARTESIAN_POINT('',(123.818927708663,1.05,50.5816897148449));
#197960=CARTESIAN_POINT('',(123.761684734793,1.05,50.8761778163746));
#197961=CARTESIAN_POINT('',(123.818927708663,1.05,50.5816897148449));
#197962=CARTESIAN_POINT('',(123.270871232244,1.05,50.7807728599253));
#197963=CARTESIAN_POINT('',(123.270871232244,1.05,50.7807728599253));
#197964=CARTESIAN_POINT('',(123.328114206113,1.05,50.4862847583956));
#197965=CARTESIAN_POINT('',(123.328114206113,1.05,50.4862847583956));
#197966=CARTESIAN_POINT('',(123.328114206113,1.05,50.4862847583956));
#197967=CARTESIAN_POINT('Origin',(123.818927708663,1.05,50.5816897148449));
#197968=CARTESIAN_POINT('',(123.818927708663,0.550000000000015,50.5816897148449));
#197969=CARTESIAN_POINT('',(123.761684734793,0.550000000000015,50.8761778163746));
#197970=CARTESIAN_POINT('',(123.818927708663,0.550000000000015,50.5816897148449));
#197971=CARTESIAN_POINT('',(123.761684734793,1.05,50.8761778163746));
#197972=CARTESIAN_POINT('',(123.818927708663,1.05,50.5816897148449));
#197973=CARTESIAN_POINT('Origin',(123.818927708663,0.550000000000015,50.5816897148449));
#197974=CARTESIAN_POINT('',(123.328114206113,0.550000000000015,50.4862847583956));
#197975=CARTESIAN_POINT('',(123.270871232244,0.550000000000015,50.7807728599253));
#197976=CARTESIAN_POINT('',(123.328114206113,0.550000000000015,50.4862847583956));
#197977=CARTESIAN_POINT('',(123.761684734793,0.550000000000015,50.8761778163746));
#197978=CARTESIAN_POINT('',(123.818927708663,0.550000000000015,50.5816897148449));
#197979=CARTESIAN_POINT('Origin',(123.328114206113,0.550000000000015,50.4862847583956));
#197980=CARTESIAN_POINT('',(123.270871232244,0.550000000000015,50.7807728599253));
#197981=CARTESIAN_POINT('',(123.328114206113,0.550000000000015,50.4862847583956));
#197982=CARTESIAN_POINT('Origin',(123.328114206113,1.85,50.4862847583956));
#197983=CARTESIAN_POINT('',(123.818927708663,1.85,50.5816897148449));
#197984=CARTESIAN_POINT('',(123.761684734793,1.85,50.8761778163746));
#197985=CARTESIAN_POINT('',(123.818927708663,1.85,50.5816897148449));
#197986=CARTESIAN_POINT('',(123.270871232244,1.85,50.7807728599253));
#197987=CARTESIAN_POINT('',(123.270871232244,1.85,50.7807728599253));
#197988=CARTESIAN_POINT('',(123.328114206113,1.85,50.4862847583956));
#197989=CARTESIAN_POINT('',(123.328114206113,1.85,50.4862847583956));
#197990=CARTESIAN_POINT('',(123.328114206113,1.85,50.4862847583956));
#197991=CARTESIAN_POINT('Origin',(123.818927708663,1.85,50.5816897148449));
#197992=CARTESIAN_POINT('',(123.818927708663,1.35,50.5816897148449));
#197993=CARTESIAN_POINT('',(123.761684734793,1.35,50.8761778163746));
#197994=CARTESIAN_POINT('',(123.818927708663,1.35,50.5816897148449));
#197995=CARTESIAN_POINT('',(123.761684734793,1.85,50.8761778163746));
#197996=CARTESIAN_POINT('',(123.818927708663,1.85,50.5816897148449));
#197997=CARTESIAN_POINT('Origin',(123.818927708663,1.35,50.5816897148449));
#197998=CARTESIAN_POINT('',(123.328114206113,1.35,50.4862847583956));
#197999=CARTESIAN_POINT('',(123.270871232244,1.35,50.7807728599253));
#198000=CARTESIAN_POINT('',(123.328114206113,1.35,50.4862847583956));
#198001=CARTESIAN_POINT('',(123.761684734793,1.35,50.8761778163746));
#198002=CARTESIAN_POINT('',(123.818927708663,1.35,50.5816897148449));
#198003=CARTESIAN_POINT('Origin',(123.328114206113,1.35,50.4862847583956));
#198004=CARTESIAN_POINT('',(123.270871232244,1.35,50.7807728599253));
#198005=CARTESIAN_POINT('',(123.328114206113,1.35,50.4862847583956));
#198006=CARTESIAN_POINT('Origin',(123.328114206113,2.65,50.4862847583956));
#198007=CARTESIAN_POINT('',(123.818927708663,2.65,50.5816897148449));
#198008=CARTESIAN_POINT('',(123.761684734793,2.65,50.8761778163746));
#198009=CARTESIAN_POINT('',(123.818927708663,2.65,50.5816897148449));
#198010=CARTESIAN_POINT('',(123.270871232244,2.65,50.7807728599253));
#198011=CARTESIAN_POINT('',(123.270871232244,2.65,50.7807728599253));
#198012=CARTESIAN_POINT('',(123.328114206113,2.65,50.4862847583956));
#198013=CARTESIAN_POINT('',(123.328114206113,2.65,50.4862847583956));
#198014=CARTESIAN_POINT('',(123.328114206113,2.65,50.4862847583956));
#198015=CARTESIAN_POINT('Origin',(123.818927708663,2.65,50.5816897148449));
#198016=CARTESIAN_POINT('',(123.818927708663,2.15,50.5816897148449));
#198017=CARTESIAN_POINT('',(123.761684734793,2.15,50.8761778163746));
#198018=CARTESIAN_POINT('',(123.818927708663,2.15,50.5816897148449));
#198019=CARTESIAN_POINT('',(123.761684734793,2.65,50.8761778163746));
#198020=CARTESIAN_POINT('',(123.818927708663,2.65,50.5816897148449));
#198021=CARTESIAN_POINT('Origin',(123.818927708663,2.15,50.5816897148449));
#198022=CARTESIAN_POINT('',(123.328114206113,2.15,50.4862847583956));
#198023=CARTESIAN_POINT('',(123.270871232244,2.15,50.7807728599253));
#198024=CARTESIAN_POINT('',(123.328114206113,2.15,50.4862847583956));
#198025=CARTESIAN_POINT('',(123.761684734793,2.15,50.8761778163746));
#198026=CARTESIAN_POINT('',(123.818927708663,2.15,50.5816897148449));
#198027=CARTESIAN_POINT('Origin',(123.328114206113,2.15,50.4862847583956));
#198028=CARTESIAN_POINT('',(123.270871232244,2.15,50.7807728599253));
#198029=CARTESIAN_POINT('',(123.328114206113,2.15,50.4862847583956));
#198030=CARTESIAN_POINT('Origin',(123.328114206113,3.45,50.4862847583956));
#198031=CARTESIAN_POINT('',(123.818927708663,3.45,50.5816897148449));
#198032=CARTESIAN_POINT('',(123.761684734793,3.45,50.8761778163746));
#198033=CARTESIAN_POINT('',(123.818927708663,3.45,50.5816897148449));
#198034=CARTESIAN_POINT('',(123.270871232244,3.45,50.7807728599253));
#198035=CARTESIAN_POINT('',(123.270871232244,3.45,50.7807728599253));
#198036=CARTESIAN_POINT('',(123.328114206113,3.45,50.4862847583956));
#198037=CARTESIAN_POINT('',(123.328114206113,3.45,50.4862847583956));
#198038=CARTESIAN_POINT('',(123.328114206113,3.45,50.4862847583956));
#198039=CARTESIAN_POINT('Origin',(123.818927708663,3.45,50.5816897148449));
#198040=CARTESIAN_POINT('',(123.818927708663,2.95,50.5816897148449));
#198041=CARTESIAN_POINT('',(123.761684734793,2.95,50.8761778163746));
#198042=CARTESIAN_POINT('',(123.818927708663,2.95,50.5816897148449));
#198043=CARTESIAN_POINT('',(123.761684734793,3.45,50.8761778163746));
#198044=CARTESIAN_POINT('',(123.818927708663,3.45,50.5816897148449));
#198045=CARTESIAN_POINT('Origin',(123.818927708663,2.95,50.5816897148449));
#198046=CARTESIAN_POINT('',(123.328114206113,2.95,50.4862847583956));
#198047=CARTESIAN_POINT('',(123.270871232244,2.95,50.7807728599253));
#198048=CARTESIAN_POINT('',(123.328114206113,2.95,50.4862847583956));
#198049=CARTESIAN_POINT('',(123.761684734793,2.95,50.8761778163746));
#198050=CARTESIAN_POINT('',(123.818927708663,2.95,50.5816897148449));
#198051=CARTESIAN_POINT('Origin',(123.328114206113,2.95,50.4862847583956));
#198052=CARTESIAN_POINT('',(123.270871232244,2.95,50.7807728599253));
#198053=CARTESIAN_POINT('',(123.328114206113,2.95,50.4862847583956));
#198054=CARTESIAN_POINT('Origin',(123.328114206113,4.25,50.4862847583956));
#198055=CARTESIAN_POINT('',(123.818927708663,4.25,50.5816897148449));
#198056=CARTESIAN_POINT('',(123.761684734793,4.25,50.8761778163746));
#198057=CARTESIAN_POINT('',(123.818927708663,4.25,50.5816897148449));
#198058=CARTESIAN_POINT('',(123.270871232244,4.25,50.7807728599253));
#198059=CARTESIAN_POINT('',(123.270871232244,4.25,50.7807728599253));
#198060=CARTESIAN_POINT('',(123.328114206113,4.25,50.4862847583956));
#198061=CARTESIAN_POINT('',(123.328114206113,4.25,50.4862847583956));
#198062=CARTESIAN_POINT('',(123.328114206113,4.25,50.4862847583956));
#198063=CARTESIAN_POINT('Origin',(123.818927708663,4.25,50.5816897148449));
#198064=CARTESIAN_POINT('',(123.818927708663,3.75,50.5816897148449));
#198065=CARTESIAN_POINT('',(123.761684734793,3.75,50.8761778163746));
#198066=CARTESIAN_POINT('',(123.818927708663,3.75,50.5816897148449));
#198067=CARTESIAN_POINT('',(123.761684734793,4.25,50.8761778163746));
#198068=CARTESIAN_POINT('',(123.818927708663,4.25,50.5816897148449));
#198069=CARTESIAN_POINT('Origin',(123.818927708663,3.75,50.5816897148449));
#198070=CARTESIAN_POINT('',(123.328114206113,3.75,50.4862847583956));
#198071=CARTESIAN_POINT('',(123.270871232244,3.75,50.7807728599253));
#198072=CARTESIAN_POINT('',(123.328114206113,3.75,50.4862847583956));
#198073=CARTESIAN_POINT('',(123.761684734793,3.75,50.8761778163746));
#198074=CARTESIAN_POINT('',(123.818927708663,3.75,50.5816897148449));
#198075=CARTESIAN_POINT('Origin',(123.328114206113,3.75,50.4862847583956));
#198076=CARTESIAN_POINT('',(123.270871232244,3.75,50.7807728599253));
#198077=CARTESIAN_POINT('',(123.328114206113,3.75,50.4862847583956));
#198078=CARTESIAN_POINT('Origin',(123.328114206113,5.05,50.4862847583956));
#198079=CARTESIAN_POINT('',(123.818927708663,5.05,50.5816897148449));
#198080=CARTESIAN_POINT('',(123.761684734793,5.05,50.8761778163746));
#198081=CARTESIAN_POINT('',(123.818927708663,5.05,50.5816897148449));
#198082=CARTESIAN_POINT('',(123.270871232244,5.05,50.7807728599253));
#198083=CARTESIAN_POINT('',(123.270871232244,5.05,50.7807728599253));
#198084=CARTESIAN_POINT('',(123.328114206113,5.05,50.4862847583956));
#198085=CARTESIAN_POINT('',(123.328114206113,5.05,50.4862847583956));
#198086=CARTESIAN_POINT('',(123.328114206113,5.05,50.4862847583956));
#198087=CARTESIAN_POINT('Origin',(123.818927708663,5.05,50.5816897148449));
#198088=CARTESIAN_POINT('',(123.818927708663,4.55,50.5816897148449));
#198089=CARTESIAN_POINT('',(123.761684734793,4.55,50.8761778163746));
#198090=CARTESIAN_POINT('',(123.818927708663,4.55,50.5816897148449));
#198091=CARTESIAN_POINT('',(123.761684734793,5.05,50.8761778163746));
#198092=CARTESIAN_POINT('',(123.818927708663,5.05,50.5816897148449));
#198093=CARTESIAN_POINT('Origin',(123.818927708663,4.55,50.5816897148449));
#198094=CARTESIAN_POINT('',(123.328114206113,4.55,50.4862847583956));
#198095=CARTESIAN_POINT('',(123.270871232244,4.55,50.7807728599253));
#198096=CARTESIAN_POINT('',(123.328114206113,4.55,50.4862847583956));
#198097=CARTESIAN_POINT('',(123.761684734793,4.55,50.8761778163746));
#198098=CARTESIAN_POINT('',(123.818927708663,4.55,50.5816897148449));
#198099=CARTESIAN_POINT('Origin',(123.328114206113,4.55,50.4862847583956));
#198100=CARTESIAN_POINT('',(123.270871232244,4.55,50.7807728599253));
#198101=CARTESIAN_POINT('',(123.328114206113,4.55,50.4862847583956));
#198102=CARTESIAN_POINT('Origin',(123.328114206113,5.85,50.4862847583956));
#198103=CARTESIAN_POINT('',(123.818927708663,5.85,50.5816897148449));
#198104=CARTESIAN_POINT('',(123.761684734793,5.85,50.8761778163746));
#198105=CARTESIAN_POINT('',(123.818927708663,5.85,50.5816897148449));
#198106=CARTESIAN_POINT('',(123.270871232244,5.85,50.7807728599253));
#198107=CARTESIAN_POINT('',(123.270871232244,5.85,50.7807728599253));
#198108=CARTESIAN_POINT('',(123.328114206113,5.85,50.4862847583956));
#198109=CARTESIAN_POINT('',(123.328114206113,5.85,50.4862847583956));
#198110=CARTESIAN_POINT('',(123.328114206113,5.85,50.4862847583956));
#198111=CARTESIAN_POINT('Origin',(123.818927708663,5.85,50.5816897148449));
#198112=CARTESIAN_POINT('',(123.818927708663,5.35,50.5816897148449));
#198113=CARTESIAN_POINT('',(123.761684734793,5.35,50.8761778163746));
#198114=CARTESIAN_POINT('',(123.818927708663,5.35,50.5816897148449));
#198115=CARTESIAN_POINT('',(123.761684734793,5.85,50.8761778163746));
#198116=CARTESIAN_POINT('',(123.818927708663,5.85,50.5816897148449));
#198117=CARTESIAN_POINT('Origin',(123.818927708663,5.35,50.5816897148449));
#198118=CARTESIAN_POINT('',(123.328114206113,5.35,50.4862847583956));
#198119=CARTESIAN_POINT('',(123.270871232244,5.35,50.7807728599253));
#198120=CARTESIAN_POINT('',(123.328114206113,5.35,50.4862847583956));
#198121=CARTESIAN_POINT('',(123.761684734793,5.35,50.8761778163746));
#198122=CARTESIAN_POINT('',(123.818927708663,5.35,50.5816897148449));
#198123=CARTESIAN_POINT('Origin',(123.328114206113,5.35,50.4862847583956));
#198124=CARTESIAN_POINT('',(123.270871232244,5.35,50.7807728599253));
#198125=CARTESIAN_POINT('',(123.328114206113,5.35,50.4862847583956));
#198126=CARTESIAN_POINT('Origin',(123.328114206113,6.65,50.4862847583956));
#198127=CARTESIAN_POINT('',(123.818927708663,6.65,50.5816897148449));
#198128=CARTESIAN_POINT('',(123.761684734793,6.65,50.8761778163746));
#198129=CARTESIAN_POINT('',(123.818927708663,6.65,50.5816897148449));
#198130=CARTESIAN_POINT('',(123.270871232244,6.65,50.7807728599253));
#198131=CARTESIAN_POINT('',(123.270871232244,6.65,50.7807728599253));
#198132=CARTESIAN_POINT('',(123.328114206113,6.65,50.4862847583956));
#198133=CARTESIAN_POINT('',(123.328114206113,6.65,50.4862847583956));
#198134=CARTESIAN_POINT('',(123.328114206113,6.65,50.4862847583956));
#198135=CARTESIAN_POINT('Origin',(123.818927708663,6.65,50.5816897148449));
#198136=CARTESIAN_POINT('',(123.818927708663,6.15,50.5816897148449));
#198137=CARTESIAN_POINT('',(123.761684734793,6.15,50.8761778163746));
#198138=CARTESIAN_POINT('',(123.818927708663,6.15,50.5816897148449));
#198139=CARTESIAN_POINT('',(123.761684734793,6.65,50.8761778163746));
#198140=CARTESIAN_POINT('',(123.818927708663,6.65,50.5816897148449));
#198141=CARTESIAN_POINT('Origin',(123.818927708663,6.15,50.5816897148449));
#198142=CARTESIAN_POINT('',(123.328114206113,6.15,50.4862847583956));
#198143=CARTESIAN_POINT('',(123.270871232244,6.15,50.7807728599253));
#198144=CARTESIAN_POINT('',(123.328114206113,6.15,50.4862847583956));
#198145=CARTESIAN_POINT('',(123.761684734793,6.15,50.8761778163746));
#198146=CARTESIAN_POINT('',(123.818927708663,6.15,50.5816897148449));
#198147=CARTESIAN_POINT('Origin',(123.328114206113,6.15,50.4862847583956));
#198148=CARTESIAN_POINT('',(123.270871232244,6.15,50.7807728599253));
#198149=CARTESIAN_POINT('',(123.328114206113,6.15,50.4862847583956));
#198150=CARTESIAN_POINT('Origin',(122.542812602034,6.65,50.3336368280768));
#198151=CARTESIAN_POINT('',(123.033626104583,6.65,50.4290417845261));
#198152=CARTESIAN_POINT('',(122.976383130714,6.65,50.7235298860558));
#198153=CARTESIAN_POINT('',(123.033626104583,6.65,50.4290417845261));
#198154=CARTESIAN_POINT('',(122.485569628164,6.65,50.6281249296065));
#198155=CARTESIAN_POINT('',(122.485569628164,6.65,50.6281249296065));
#198156=CARTESIAN_POINT('',(122.542812602034,6.65,50.3336368280768));
#198157=CARTESIAN_POINT('',(122.542812602034,6.65,50.3336368280768));
#198158=CARTESIAN_POINT('',(122.542812602034,6.65,50.3336368280768));
#198159=CARTESIAN_POINT('Origin',(123.033626104583,6.65,50.4290417845261));
#198160=CARTESIAN_POINT('',(123.033626104583,6.15,50.4290417845261));
#198161=CARTESIAN_POINT('',(122.976383130714,6.15,50.7235298860558));
#198162=CARTESIAN_POINT('',(123.033626104583,6.15,50.4290417845261));
#198163=CARTESIAN_POINT('',(122.976383130714,6.65,50.7235298860558));
#198164=CARTESIAN_POINT('',(123.033626104583,6.65,50.4290417845261));
#198165=CARTESIAN_POINT('Origin',(123.033626104583,6.15,50.4290417845261));
#198166=CARTESIAN_POINT('',(122.542812602034,6.15,50.3336368280768));
#198167=CARTESIAN_POINT('',(122.485569628164,6.15,50.6281249296065));
#198168=CARTESIAN_POINT('',(122.542812602034,6.15,50.3336368280768));
#198169=CARTESIAN_POINT('',(122.976383130714,6.15,50.7235298860558));
#198170=CARTESIAN_POINT('',(123.033626104583,6.15,50.4290417845261));
#198171=CARTESIAN_POINT('Origin',(122.542812602034,6.15,50.3336368280768));
#198172=CARTESIAN_POINT('',(122.485569628164,6.15,50.6281249296065));
#198173=CARTESIAN_POINT('',(122.542812602034,6.15,50.3336368280768));
#198174=CARTESIAN_POINT('Origin',(121.757510997955,6.65,50.180988897758));
#198175=CARTESIAN_POINT('',(122.248324500504,6.65,50.2763938542073));
#198176=CARTESIAN_POINT('',(122.191081526635,6.65,50.570881955737));
#198177=CARTESIAN_POINT('',(122.248324500504,6.65,50.2763938542073));
#198178=CARTESIAN_POINT('',(121.700268024085,6.65,50.4754769992877));
#198179=CARTESIAN_POINT('',(121.700268024085,6.65,50.4754769992877));
#198180=CARTESIAN_POINT('',(121.757510997955,6.65,50.180988897758));
#198181=CARTESIAN_POINT('',(121.757510997955,6.65,50.180988897758));
#198182=CARTESIAN_POINT('',(121.757510997955,6.65,50.180988897758));
#198183=CARTESIAN_POINT('Origin',(122.248324500504,6.65,50.2763938542073));
#198184=CARTESIAN_POINT('',(122.248324500504,6.15,50.2763938542073));
#198185=CARTESIAN_POINT('',(122.191081526635,6.15,50.570881955737));
#198186=CARTESIAN_POINT('',(122.248324500504,6.15,50.2763938542073));
#198187=CARTESIAN_POINT('',(122.191081526635,6.65,50.570881955737));
#198188=CARTESIAN_POINT('',(122.248324500504,6.65,50.2763938542073));
#198189=CARTESIAN_POINT('Origin',(122.248324500504,6.15,50.2763938542073));
#198190=CARTESIAN_POINT('',(121.757510997955,6.15,50.180988897758));
#198191=CARTESIAN_POINT('',(121.700268024085,6.15,50.4754769992877));
#198192=CARTESIAN_POINT('',(121.757510997955,6.15,50.180988897758));
#198193=CARTESIAN_POINT('',(122.191081526635,6.15,50.570881955737));
#198194=CARTESIAN_POINT('',(122.248324500504,6.15,50.2763938542073));
#198195=CARTESIAN_POINT('Origin',(121.757510997955,6.15,50.180988897758));
#198196=CARTESIAN_POINT('',(121.700268024085,6.15,50.4754769992877));
#198197=CARTESIAN_POINT('',(121.757510997955,6.15,50.180988897758));
#198198=CARTESIAN_POINT('Origin',(120.972209393875,6.65,50.0283409674392));
#198199=CARTESIAN_POINT('',(121.463022896425,6.65,50.1237459238885));
#198200=CARTESIAN_POINT('',(121.405779922555,6.65,50.4182340254182));
#198201=CARTESIAN_POINT('',(121.463022896425,6.65,50.1237459238885));
#198202=CARTESIAN_POINT('',(120.914966420006,6.65,50.3228290689689));
#198203=CARTESIAN_POINT('',(120.914966420006,6.65,50.3228290689689));
#198204=CARTESIAN_POINT('',(120.972209393875,6.65,50.0283409674392));
#198205=CARTESIAN_POINT('',(120.972209393875,6.65,50.0283409674392));
#198206=CARTESIAN_POINT('',(120.972209393875,6.65,50.0283409674392));
#198207=CARTESIAN_POINT('Origin',(121.463022896425,6.65,50.1237459238885));
#198208=CARTESIAN_POINT('',(121.463022896425,6.15,50.1237459238885));
#198209=CARTESIAN_POINT('',(121.405779922555,6.15,50.4182340254182));
#198210=CARTESIAN_POINT('',(121.463022896425,6.15,50.1237459238885));
#198211=CARTESIAN_POINT('',(121.405779922555,6.65,50.4182340254182));
#198212=CARTESIAN_POINT('',(121.463022896425,6.65,50.1237459238885));
#198213=CARTESIAN_POINT('Origin',(121.463022896425,6.15,50.1237459238885));
#198214=CARTESIAN_POINT('',(120.972209393875,6.15,50.0283409674392));
#198215=CARTESIAN_POINT('',(120.914966420006,6.15,50.3228290689689));
#198216=CARTESIAN_POINT('',(120.972209393875,6.15,50.0283409674392));
#198217=CARTESIAN_POINT('',(121.405779922555,6.15,50.4182340254182));
#198218=CARTESIAN_POINT('',(121.463022896425,6.15,50.1237459238885));
#198219=CARTESIAN_POINT('Origin',(120.972209393875,6.15,50.0283409674392));
#198220=CARTESIAN_POINT('',(120.914966420006,6.15,50.3228290689689));
#198221=CARTESIAN_POINT('',(120.972209393875,6.15,50.0283409674392));
#198222=CARTESIAN_POINT('Origin',(120.186907789796,6.65,49.8756930371204));
#198223=CARTESIAN_POINT('',(120.677721292346,6.65,49.9710979935697));
#198224=CARTESIAN_POINT('',(120.620478318476,6.65,50.2655860950994));
#198225=CARTESIAN_POINT('',(120.677721292346,6.65,49.9710979935697));
#198226=CARTESIAN_POINT('',(120.129664815927,6.65,50.1701811386501));
#198227=CARTESIAN_POINT('',(120.129664815927,6.65,50.1701811386501));
#198228=CARTESIAN_POINT('',(120.186907789796,6.65,49.8756930371204));
#198229=CARTESIAN_POINT('',(120.186907789796,6.65,49.8756930371204));
#198230=CARTESIAN_POINT('',(120.186907789796,6.65,49.8756930371204));
#198231=CARTESIAN_POINT('Origin',(120.677721292346,6.65,49.9710979935697));
#198232=CARTESIAN_POINT('',(120.677721292346,6.15,49.9710979935697));
#198233=CARTESIAN_POINT('',(120.620478318476,6.15,50.2655860950994));
#198234=CARTESIAN_POINT('',(120.677721292346,6.15,49.9710979935697));
#198235=CARTESIAN_POINT('',(120.620478318476,6.65,50.2655860950994));
#198236=CARTESIAN_POINT('',(120.677721292346,6.65,49.9710979935697));
#198237=CARTESIAN_POINT('Origin',(120.677721292346,6.15,49.9710979935697));
#198238=CARTESIAN_POINT('',(120.186907789796,6.15,49.8756930371204));
#198239=CARTESIAN_POINT('',(120.129664815927,6.15,50.1701811386501));
#198240=CARTESIAN_POINT('',(120.186907789796,6.15,49.8756930371204));
#198241=CARTESIAN_POINT('',(120.620478318476,6.15,50.2655860950994));
#198242=CARTESIAN_POINT('',(120.677721292346,6.15,49.9710979935697));
#198243=CARTESIAN_POINT('Origin',(120.186907789796,6.15,49.8756930371204));
#198244=CARTESIAN_POINT('',(120.129664815927,6.15,50.1701811386501));
#198245=CARTESIAN_POINT('',(120.186907789796,6.15,49.8756930371204));
#198246=CARTESIAN_POINT('Origin',(119.401606185717,6.65,49.7230451068016));
#198247=CARTESIAN_POINT('',(119.892419688267,6.65,49.8184500632509));
#198248=CARTESIAN_POINT('',(119.835176714397,6.65,50.1129381647806));
#198249=CARTESIAN_POINT('',(119.892419688267,6.65,49.8184500632509));
#198250=CARTESIAN_POINT('',(119.344363211847,6.65,50.0175332083313));
#198251=CARTESIAN_POINT('',(119.344363211847,6.65,50.0175332083313));
#198252=CARTESIAN_POINT('',(119.401606185717,6.65,49.7230451068016));
#198253=CARTESIAN_POINT('',(119.401606185717,6.65,49.7230451068016));
#198254=CARTESIAN_POINT('',(119.401606185717,6.65,49.7230451068016));
#198255=CARTESIAN_POINT('Origin',(119.892419688267,6.65,49.8184500632509));
#198256=CARTESIAN_POINT('',(119.892419688267,6.15,49.8184500632509));
#198257=CARTESIAN_POINT('',(119.835176714397,6.15,50.1129381647806));
#198258=CARTESIAN_POINT('',(119.892419688267,6.15,49.8184500632509));
#198259=CARTESIAN_POINT('',(119.835176714397,6.65,50.1129381647806));
#198260=CARTESIAN_POINT('',(119.892419688267,6.65,49.8184500632509));
#198261=CARTESIAN_POINT('Origin',(119.892419688267,6.15,49.8184500632509));
#198262=CARTESIAN_POINT('',(119.401606185717,6.15,49.7230451068016));
#198263=CARTESIAN_POINT('',(119.344363211847,6.15,50.0175332083313));
#198264=CARTESIAN_POINT('',(119.401606185717,6.15,49.7230451068016));
#198265=CARTESIAN_POINT('',(119.835176714397,6.15,50.1129381647806));
#198266=CARTESIAN_POINT('',(119.892419688267,6.15,49.8184500632509));
#198267=CARTESIAN_POINT('Origin',(119.401606185717,6.15,49.7230451068016));
#198268=CARTESIAN_POINT('',(119.344363211847,6.15,50.0175332083313));
#198269=CARTESIAN_POINT('',(119.401606185717,6.15,49.7230451068016));
#198270=CARTESIAN_POINT('Origin',(118.616304581638,6.65,49.5703971764828));
#198271=CARTESIAN_POINT('',(119.107118084187,6.65,49.6658021329321));
#198272=CARTESIAN_POINT('',(119.049875110318,6.65,49.9602902344618));
#198273=CARTESIAN_POINT('',(119.107118084187,6.65,49.6658021329321));
#198274=CARTESIAN_POINT('',(118.559061607768,6.65,49.8648852780125));
#198275=CARTESIAN_POINT('',(118.559061607768,6.65,49.8648852780125));
#198276=CARTESIAN_POINT('',(118.616304581638,6.65,49.5703971764828));
#198277=CARTESIAN_POINT('',(118.616304581638,6.65,49.5703971764828));
#198278=CARTESIAN_POINT('',(118.616304581638,6.65,49.5703971764828));
#198279=CARTESIAN_POINT('Origin',(119.107118084187,6.65,49.6658021329321));
#198280=CARTESIAN_POINT('',(119.107118084187,6.15,49.6658021329321));
#198281=CARTESIAN_POINT('',(119.049875110318,6.15,49.9602902344618));
#198282=CARTESIAN_POINT('',(119.107118084187,6.15,49.6658021329321));
#198283=CARTESIAN_POINT('',(119.049875110318,6.65,49.9602902344618));
#198284=CARTESIAN_POINT('',(119.107118084187,6.65,49.6658021329321));
#198285=CARTESIAN_POINT('Origin',(119.107118084187,6.15,49.6658021329321));
#198286=CARTESIAN_POINT('',(118.616304581638,6.15,49.5703971764828));
#198287=CARTESIAN_POINT('',(118.559061607768,6.15,49.8648852780125));
#198288=CARTESIAN_POINT('',(118.616304581638,6.15,49.5703971764828));
#198289=CARTESIAN_POINT('',(119.049875110318,6.15,49.9602902344618));
#198290=CARTESIAN_POINT('',(119.107118084187,6.15,49.6658021329321));
#198291=CARTESIAN_POINT('Origin',(118.616304581638,6.15,49.5703971764828));
#198292=CARTESIAN_POINT('',(118.559061607768,6.15,49.8648852780125));
#198293=CARTESIAN_POINT('',(118.616304581638,6.15,49.5703971764828));
#198294=CARTESIAN_POINT('Origin',(117.831002977559,6.65,49.417749246164));
#198295=CARTESIAN_POINT('',(118.321816480108,6.65,49.5131542026133));
#198296=CARTESIAN_POINT('',(118.264573506239,6.65,49.807642304143));
#198297=CARTESIAN_POINT('',(118.321816480108,6.65,49.5131542026133));
#198298=CARTESIAN_POINT('',(117.773760003689,6.65,49.7122373476937));
#198299=CARTESIAN_POINT('',(117.773760003689,6.65,49.7122373476937));
#198300=CARTESIAN_POINT('',(117.831002977559,6.65,49.417749246164));
#198301=CARTESIAN_POINT('',(117.831002977559,6.65,49.417749246164));
#198302=CARTESIAN_POINT('',(117.831002977559,6.65,49.417749246164));
#198303=CARTESIAN_POINT('Origin',(118.321816480108,6.65,49.5131542026133));
#198304=CARTESIAN_POINT('',(118.321816480108,6.15,49.5131542026133));
#198305=CARTESIAN_POINT('',(118.264573506239,6.15,49.807642304143));
#198306=CARTESIAN_POINT('',(118.321816480108,6.15,49.5131542026133));
#198307=CARTESIAN_POINT('',(118.264573506239,6.65,49.807642304143));
#198308=CARTESIAN_POINT('',(118.321816480108,6.65,49.5131542026133));
#198309=CARTESIAN_POINT('Origin',(118.321816480108,6.15,49.5131542026133));
#198310=CARTESIAN_POINT('',(117.831002977559,6.15,49.417749246164));
#198311=CARTESIAN_POINT('',(117.773760003689,6.15,49.7122373476937));
#198312=CARTESIAN_POINT('',(117.831002977559,6.15,49.417749246164));
#198313=CARTESIAN_POINT('',(118.264573506239,6.15,49.807642304143));
#198314=CARTESIAN_POINT('',(118.321816480108,6.15,49.5131542026133));
#198315=CARTESIAN_POINT('Origin',(117.831002977559,6.15,49.417749246164));
#198316=CARTESIAN_POINT('',(117.773760003689,6.15,49.7122373476937));
#198317=CARTESIAN_POINT('',(117.831002977559,6.15,49.417749246164));
#198318=CARTESIAN_POINT('Origin',(117.045701373479,6.65,49.2651013158452));
#198319=CARTESIAN_POINT('',(117.536514876029,6.65,49.3605062722945));
#198320=CARTESIAN_POINT('',(117.479271902159,6.65,49.6549943738242));
#198321=CARTESIAN_POINT('',(117.536514876029,6.65,49.3605062722945));
#198322=CARTESIAN_POINT('',(116.98845839961,6.65,49.5595894173749));
#198323=CARTESIAN_POINT('',(116.98845839961,6.65,49.5595894173749));
#198324=CARTESIAN_POINT('',(117.045701373479,6.65,49.2651013158452));
#198325=CARTESIAN_POINT('',(117.045701373479,6.65,49.2651013158452));
#198326=CARTESIAN_POINT('',(117.045701373479,6.65,49.2651013158452));
#198327=CARTESIAN_POINT('Origin',(117.536514876029,6.65,49.3605062722945));
#198328=CARTESIAN_POINT('',(117.536514876029,6.15,49.3605062722945));
#198329=CARTESIAN_POINT('',(117.479271902159,6.15,49.6549943738242));
#198330=CARTESIAN_POINT('',(117.536514876029,6.15,49.3605062722945));
#198331=CARTESIAN_POINT('',(117.479271902159,6.65,49.6549943738242));
#198332=CARTESIAN_POINT('',(117.536514876029,6.65,49.3605062722945));
#198333=CARTESIAN_POINT('Origin',(117.536514876029,6.15,49.3605062722945));
#198334=CARTESIAN_POINT('',(117.045701373479,6.15,49.2651013158452));
#198335=CARTESIAN_POINT('',(116.98845839961,6.15,49.5595894173749));
#198336=CARTESIAN_POINT('',(117.045701373479,6.15,49.2651013158452));
#198337=CARTESIAN_POINT('',(117.479271902159,6.15,49.6549943738242));
#198338=CARTESIAN_POINT('',(117.536514876029,6.15,49.3605062722945));
#198339=CARTESIAN_POINT('Origin',(117.045701373479,6.15,49.2651013158452));
#198340=CARTESIAN_POINT('',(116.98845839961,6.15,49.5595894173749));
#198341=CARTESIAN_POINT('',(117.045701373479,6.15,49.2651013158452));
#198342=CARTESIAN_POINT('Origin',(116.2603997694,6.65,49.1124533855264));
#198343=CARTESIAN_POINT('',(116.75121327195,6.65,49.2078583419757));
#198344=CARTESIAN_POINT('',(116.69397029808,6.65,49.5023464435054));
#198345=CARTESIAN_POINT('',(116.75121327195,6.65,49.2078583419757));
#198346=CARTESIAN_POINT('',(116.203156795531,6.65,49.4069414870561));
#198347=CARTESIAN_POINT('',(116.203156795531,6.65,49.4069414870561));
#198348=CARTESIAN_POINT('',(116.2603997694,6.65,49.1124533855264));
#198349=CARTESIAN_POINT('',(116.2603997694,6.65,49.1124533855264));
#198350=CARTESIAN_POINT('',(116.2603997694,6.65,49.1124533855264));
#198351=CARTESIAN_POINT('Origin',(116.75121327195,6.65,49.2078583419757));
#198352=CARTESIAN_POINT('',(116.75121327195,6.15,49.2078583419757));
#198353=CARTESIAN_POINT('',(116.69397029808,6.15,49.5023464435054));
#198354=CARTESIAN_POINT('',(116.75121327195,6.15,49.2078583419757));
#198355=CARTESIAN_POINT('',(116.69397029808,6.65,49.5023464435054));
#198356=CARTESIAN_POINT('',(116.75121327195,6.65,49.2078583419757));
#198357=CARTESIAN_POINT('Origin',(116.75121327195,6.15,49.2078583419757));
#198358=CARTESIAN_POINT('',(116.2603997694,6.15,49.1124533855264));
#198359=CARTESIAN_POINT('',(116.203156795531,6.15,49.4069414870561));
#198360=CARTESIAN_POINT('',(116.2603997694,6.15,49.1124533855264));
#198361=CARTESIAN_POINT('',(116.69397029808,6.15,49.5023464435054));
#198362=CARTESIAN_POINT('',(116.75121327195,6.15,49.2078583419757));
#198363=CARTESIAN_POINT('Origin',(116.2603997694,6.15,49.1124533855264));
#198364=CARTESIAN_POINT('',(116.203156795531,6.15,49.4069414870561));
#198365=CARTESIAN_POINT('',(116.2603997694,6.15,49.1124533855264));
#198366=CARTESIAN_POINT('Origin',(115.475098165321,6.65,48.9598054552076));
#198367=CARTESIAN_POINT('',(115.96591166787,6.65,49.0552104116569));
#198368=CARTESIAN_POINT('',(115.908668694001,6.65,49.3496985131866));
#198369=CARTESIAN_POINT('',(115.96591166787,6.65,49.0552104116569));
#198370=CARTESIAN_POINT('',(115.417855191451,6.65,49.2542935567373));
#198371=CARTESIAN_POINT('',(115.417855191451,6.65,49.2542935567373));
#198372=CARTESIAN_POINT('',(115.475098165321,6.65,48.9598054552076));
#198373=CARTESIAN_POINT('',(115.475098165321,6.65,48.9598054552076));
#198374=CARTESIAN_POINT('',(115.475098165321,6.65,48.9598054552076));
#198375=CARTESIAN_POINT('Origin',(115.96591166787,6.65,49.0552104116569));
#198376=CARTESIAN_POINT('',(115.96591166787,6.15,49.0552104116569));
#198377=CARTESIAN_POINT('',(115.908668694001,6.15,49.3496985131866));
#198378=CARTESIAN_POINT('',(115.96591166787,6.15,49.0552104116569));
#198379=CARTESIAN_POINT('',(115.908668694001,6.65,49.3496985131866));
#198380=CARTESIAN_POINT('',(115.96591166787,6.65,49.0552104116569));
#198381=CARTESIAN_POINT('Origin',(115.96591166787,6.15,49.0552104116569));
#198382=CARTESIAN_POINT('',(115.475098165321,6.15,48.9598054552076));
#198383=CARTESIAN_POINT('',(115.417855191451,6.15,49.2542935567373));
#198384=CARTESIAN_POINT('',(115.475098165321,6.15,48.9598054552076));
#198385=CARTESIAN_POINT('',(115.908668694001,6.15,49.3496985131866));
#198386=CARTESIAN_POINT('',(115.96591166787,6.15,49.0552104116569));
#198387=CARTESIAN_POINT('Origin',(115.475098165321,6.15,48.9598054552076));
#198388=CARTESIAN_POINT('',(115.417855191451,6.15,49.2542935567373));
#198389=CARTESIAN_POINT('',(115.475098165321,6.15,48.9598054552076));
#198390=CARTESIAN_POINT('Origin',(114.689796561242,6.65,48.8071575248888));
#198391=CARTESIAN_POINT('',(115.180610063791,6.65,48.9025624813381));
#198392=CARTESIAN_POINT('',(115.123367089922,6.65,49.1970505828678));
#198393=CARTESIAN_POINT('',(115.180610063791,6.65,48.9025624813381));
#198394=CARTESIAN_POINT('',(114.632553587372,6.65,49.1016456264185));
#198395=CARTESIAN_POINT('',(114.632553587372,6.65,49.1016456264185));
#198396=CARTESIAN_POINT('',(114.689796561242,6.65,48.8071575248888));
#198397=CARTESIAN_POINT('',(114.689796561242,6.65,48.8071575248888));
#198398=CARTESIAN_POINT('',(114.689796561242,6.65,48.8071575248888));
#198399=CARTESIAN_POINT('Origin',(115.180610063791,6.65,48.9025624813381));
#198400=CARTESIAN_POINT('',(115.180610063791,6.15,48.9025624813381));
#198401=CARTESIAN_POINT('',(115.123367089922,6.15,49.1970505828678));
#198402=CARTESIAN_POINT('',(115.180610063791,6.15,48.9025624813381));
#198403=CARTESIAN_POINT('',(115.123367089922,6.65,49.1970505828678));
#198404=CARTESIAN_POINT('',(115.180610063791,6.65,48.9025624813381));
#198405=CARTESIAN_POINT('Origin',(115.180610063791,6.15,48.9025624813381));
#198406=CARTESIAN_POINT('',(114.689796561242,6.15,48.8071575248888));
#198407=CARTESIAN_POINT('',(114.632553587372,6.15,49.1016456264185));
#198408=CARTESIAN_POINT('',(114.689796561242,6.15,48.8071575248888));
#198409=CARTESIAN_POINT('',(115.123367089922,6.15,49.1970505828678));
#198410=CARTESIAN_POINT('',(115.180610063791,6.15,48.9025624813381));
#198411=CARTESIAN_POINT('Origin',(114.689796561242,6.15,48.8071575248888));
#198412=CARTESIAN_POINT('',(114.632553587372,6.15,49.1016456264185));
#198413=CARTESIAN_POINT('',(114.689796561242,6.15,48.8071575248888));
#198414=CARTESIAN_POINT('Origin',(113.904494957163,6.65,48.65450959457));
#198415=CARTESIAN_POINT('',(114.395308459712,6.65,48.7499145510193));
#198416=CARTESIAN_POINT('',(114.338065485842,6.65,49.044402652549));
#198417=CARTESIAN_POINT('',(114.395308459712,6.65,48.7499145510193));
#198418=CARTESIAN_POINT('',(113.847251983293,6.65,48.9489976960997));
#198419=CARTESIAN_POINT('',(113.847251983293,6.65,48.9489976960997));
#198420=CARTESIAN_POINT('',(113.904494957163,6.65,48.65450959457));
#198421=CARTESIAN_POINT('',(113.904494957163,6.65,48.65450959457));
#198422=CARTESIAN_POINT('',(113.904494957163,6.65,48.65450959457));
#198423=CARTESIAN_POINT('Origin',(114.395308459712,6.65,48.7499145510193));
#198424=CARTESIAN_POINT('',(114.395308459712,6.15,48.7499145510193));
#198425=CARTESIAN_POINT('',(114.338065485842,6.15,49.044402652549));
#198426=CARTESIAN_POINT('',(114.395308459712,6.15,48.7499145510193));
#198427=CARTESIAN_POINT('',(114.338065485842,6.65,49.044402652549));
#198428=CARTESIAN_POINT('',(114.395308459712,6.65,48.7499145510193));
#198429=CARTESIAN_POINT('Origin',(114.395308459712,6.15,48.7499145510193));
#198430=CARTESIAN_POINT('',(113.904494957163,6.15,48.65450959457));
#198431=CARTESIAN_POINT('',(113.847251983293,6.15,48.9489976960997));
#198432=CARTESIAN_POINT('',(113.904494957163,6.15,48.65450959457));
#198433=CARTESIAN_POINT('',(114.338065485842,6.15,49.044402652549));
#198434=CARTESIAN_POINT('',(114.395308459712,6.15,48.7499145510193));
#198435=CARTESIAN_POINT('Origin',(113.904494957163,6.15,48.65450959457));
#198436=CARTESIAN_POINT('',(113.847251983293,6.15,48.9489976960997));
#198437=CARTESIAN_POINT('',(113.904494957163,6.15,48.65450959457));
#198438=CARTESIAN_POINT('Origin',(113.119193353083,6.65,48.5018616642512));
#198439=CARTESIAN_POINT('',(113.610006855633,6.65,48.5972666207005));
#198440=CARTESIAN_POINT('',(113.552763881763,6.65,48.8917547222302));
#198441=CARTESIAN_POINT('',(113.610006855633,6.65,48.5972666207005));
#198442=CARTESIAN_POINT('',(113.061950379214,6.65,48.7963497657809));
#198443=CARTESIAN_POINT('',(113.061950379214,6.65,48.7963497657809));
#198444=CARTESIAN_POINT('',(113.119193353083,6.65,48.5018616642512));
#198445=CARTESIAN_POINT('',(113.119193353083,6.65,48.5018616642512));
#198446=CARTESIAN_POINT('',(113.119193353083,6.65,48.5018616642512));
#198447=CARTESIAN_POINT('Origin',(113.610006855633,6.65,48.5972666207005));
#198448=CARTESIAN_POINT('',(113.610006855633,6.15,48.5972666207005));
#198449=CARTESIAN_POINT('',(113.552763881763,6.15,48.8917547222302));
#198450=CARTESIAN_POINT('',(113.610006855633,6.15,48.5972666207005));
#198451=CARTESIAN_POINT('',(113.552763881763,6.65,48.8917547222302));
#198452=CARTESIAN_POINT('',(113.610006855633,6.65,48.5972666207005));
#198453=CARTESIAN_POINT('Origin',(113.610006855633,6.15,48.5972666207005));
#198454=CARTESIAN_POINT('',(113.119193353083,6.15,48.5018616642512));
#198455=CARTESIAN_POINT('',(113.061950379214,6.15,48.7963497657809));
#198456=CARTESIAN_POINT('',(113.119193353083,6.15,48.5018616642512));
#198457=CARTESIAN_POINT('',(113.552763881763,6.15,48.8917547222302));
#198458=CARTESIAN_POINT('',(113.610006855633,6.15,48.5972666207005));
#198459=CARTESIAN_POINT('Origin',(113.119193353083,6.15,48.5018616642512));
#198460=CARTESIAN_POINT('',(113.061950379214,6.15,48.7963497657809));
#198461=CARTESIAN_POINT('',(113.119193353083,6.15,48.5018616642512));
#198462=CARTESIAN_POINT('Origin',(112.333891749004,6.65,48.3492137339324));
#198463=CARTESIAN_POINT('',(112.824705251554,6.65,48.4446186903817));
#198464=CARTESIAN_POINT('',(112.767462277684,6.65,48.7391067919114));
#198465=CARTESIAN_POINT('',(112.824705251554,6.65,48.4446186903817));
#198466=CARTESIAN_POINT('',(112.276648775135,6.65,48.6437018354621));
#198467=CARTESIAN_POINT('',(112.276648775135,6.65,48.6437018354621));
#198468=CARTESIAN_POINT('',(112.333891749004,6.65,48.3492137339324));
#198469=CARTESIAN_POINT('',(112.333891749004,6.65,48.3492137339324));
#198470=CARTESIAN_POINT('',(112.333891749004,6.65,48.3492137339324));
#198471=CARTESIAN_POINT('Origin',(112.824705251554,6.65,48.4446186903817));
#198472=CARTESIAN_POINT('',(112.824705251554,6.15,48.4446186903817));
#198473=CARTESIAN_POINT('',(112.767462277684,6.15,48.7391067919114));
#198474=CARTESIAN_POINT('',(112.824705251554,6.15,48.4446186903817));
#198475=CARTESIAN_POINT('',(112.767462277684,6.65,48.7391067919114));
#198476=CARTESIAN_POINT('',(112.824705251554,6.65,48.4446186903817));
#198477=CARTESIAN_POINT('Origin',(112.824705251554,6.15,48.4446186903817));
#198478=CARTESIAN_POINT('',(112.333891749004,6.15,48.3492137339324));
#198479=CARTESIAN_POINT('',(112.276648775135,6.15,48.6437018354621));
#198480=CARTESIAN_POINT('',(112.333891749004,6.15,48.3492137339324));
#198481=CARTESIAN_POINT('',(112.767462277684,6.15,48.7391067919114));
#198482=CARTESIAN_POINT('',(112.824705251554,6.15,48.4446186903817));
#198483=CARTESIAN_POINT('Origin',(112.333891749004,6.15,48.3492137339324));
#198484=CARTESIAN_POINT('',(112.276648775135,6.15,48.6437018354621));
#198485=CARTESIAN_POINT('',(112.333891749004,6.15,48.3492137339324));
#198486=CARTESIAN_POINT('Origin',(111.548590144925,6.65,48.1965658036136));
#198487=CARTESIAN_POINT('',(112.039403647474,6.65,48.2919707600629));
#198488=CARTESIAN_POINT('',(111.982160673605,6.65,48.5864588615926));
#198489=CARTESIAN_POINT('',(112.039403647474,6.65,48.2919707600629));
#198490=CARTESIAN_POINT('',(111.491347171055,6.65,48.4910539051433));
#198491=CARTESIAN_POINT('',(111.491347171055,6.65,48.4910539051433));
#198492=CARTESIAN_POINT('',(111.548590144925,6.65,48.1965658036136));
#198493=CARTESIAN_POINT('',(111.548590144925,6.65,48.1965658036136));
#198494=CARTESIAN_POINT('',(111.548590144925,6.65,48.1965658036136));
#198495=CARTESIAN_POINT('Origin',(112.039403647474,6.65,48.2919707600629));
#198496=CARTESIAN_POINT('',(112.039403647474,6.15,48.2919707600629));
#198497=CARTESIAN_POINT('',(111.982160673605,6.15,48.5864588615926));
#198498=CARTESIAN_POINT('',(112.039403647474,6.15,48.2919707600629));
#198499=CARTESIAN_POINT('',(111.982160673605,6.65,48.5864588615926));
#198500=CARTESIAN_POINT('',(112.039403647474,6.65,48.2919707600629));
#198501=CARTESIAN_POINT('Origin',(112.039403647474,6.15,48.2919707600629));
#198502=CARTESIAN_POINT('',(111.548590144925,6.15,48.1965658036136));
#198503=CARTESIAN_POINT('',(111.491347171055,6.15,48.4910539051433));
#198504=CARTESIAN_POINT('',(111.548590144925,6.15,48.1965658036136));
#198505=CARTESIAN_POINT('',(111.982160673605,6.15,48.5864588615926));
#198506=CARTESIAN_POINT('',(112.039403647474,6.15,48.2919707600629));
#198507=CARTESIAN_POINT('Origin',(111.548590144925,6.15,48.1965658036136));
#198508=CARTESIAN_POINT('',(111.491347171055,6.15,48.4910539051433));
#198509=CARTESIAN_POINT('',(111.548590144925,6.15,48.1965658036136));
#198510=CARTESIAN_POINT('Origin',(111.548590144925,5.85,48.1965658036136));
#198511=CARTESIAN_POINT('',(112.039403647474,5.85,48.2919707600629));
#198512=CARTESIAN_POINT('',(111.982160673605,5.85,48.5864588615926));
#198513=CARTESIAN_POINT('',(112.039403647474,5.85,48.2919707600629));
#198514=CARTESIAN_POINT('',(111.491347171055,5.85,48.4910539051433));
#198515=CARTESIAN_POINT('',(111.491347171055,5.85,48.4910539051433));
#198516=CARTESIAN_POINT('',(111.548590144925,5.85,48.1965658036136));
#198517=CARTESIAN_POINT('',(111.548590144925,5.85,48.1965658036136));
#198518=CARTESIAN_POINT('',(111.548590144925,5.85,48.1965658036136));
#198519=CARTESIAN_POINT('Origin',(112.039403647474,5.85,48.2919707600629));
#198520=CARTESIAN_POINT('',(112.039403647474,5.35,48.2919707600629));
#198521=CARTESIAN_POINT('',(111.982160673605,5.35,48.5864588615926));
#198522=CARTESIAN_POINT('',(112.039403647474,5.35,48.2919707600629));
#198523=CARTESIAN_POINT('',(111.982160673605,5.85,48.5864588615926));
#198524=CARTESIAN_POINT('',(112.039403647474,5.85,48.2919707600629));
#198525=CARTESIAN_POINT('Origin',(112.039403647474,5.35,48.2919707600629));
#198526=CARTESIAN_POINT('',(111.548590144925,5.35,48.1965658036136));
#198527=CARTESIAN_POINT('',(111.491347171055,5.35,48.4910539051433));
#198528=CARTESIAN_POINT('',(111.548590144925,5.35,48.1965658036136));
#198529=CARTESIAN_POINT('',(111.982160673605,5.35,48.5864588615926));
#198530=CARTESIAN_POINT('',(112.039403647474,5.35,48.2919707600629));
#198531=CARTESIAN_POINT('Origin',(111.548590144925,5.35,48.1965658036136));
#198532=CARTESIAN_POINT('',(111.491347171055,5.35,48.4910539051433));
#198533=CARTESIAN_POINT('',(111.548590144925,5.35,48.1965658036136));
#198534=CARTESIAN_POINT('Origin',(111.548590144925,5.05,48.1965658036136));
#198535=CARTESIAN_POINT('',(112.039403647474,5.05,48.2919707600629));
#198536=CARTESIAN_POINT('',(111.982160673605,5.05,48.5864588615926));
#198537=CARTESIAN_POINT('',(112.039403647474,5.05,48.2919707600629));
#198538=CARTESIAN_POINT('',(111.491347171055,5.05,48.4910539051433));
#198539=CARTESIAN_POINT('',(111.491347171055,5.05,48.4910539051433));
#198540=CARTESIAN_POINT('',(111.548590144925,5.05,48.1965658036136));
#198541=CARTESIAN_POINT('',(111.548590144925,5.05,48.1965658036136));
#198542=CARTESIAN_POINT('',(111.548590144925,5.05,48.1965658036136));
#198543=CARTESIAN_POINT('Origin',(112.039403647474,5.05,48.2919707600629));
#198544=CARTESIAN_POINT('',(112.039403647474,4.55,48.2919707600629));
#198545=CARTESIAN_POINT('',(111.982160673605,4.55,48.5864588615926));
#198546=CARTESIAN_POINT('',(112.039403647474,4.55,48.2919707600629));
#198547=CARTESIAN_POINT('',(111.982160673605,5.05,48.5864588615926));
#198548=CARTESIAN_POINT('',(112.039403647474,5.05,48.2919707600629));
#198549=CARTESIAN_POINT('Origin',(112.039403647474,4.55,48.2919707600629));
#198550=CARTESIAN_POINT('',(111.548590144925,4.55,48.1965658036136));
#198551=CARTESIAN_POINT('',(111.491347171055,4.55,48.4910539051433));
#198552=CARTESIAN_POINT('',(111.548590144925,4.55,48.1965658036136));
#198553=CARTESIAN_POINT('',(111.982160673605,4.55,48.5864588615926));
#198554=CARTESIAN_POINT('',(112.039403647474,4.55,48.2919707600629));
#198555=CARTESIAN_POINT('Origin',(111.548590144925,4.55,48.1965658036136));
#198556=CARTESIAN_POINT('',(111.491347171055,4.55,48.4910539051433));
#198557=CARTESIAN_POINT('',(111.548590144925,4.55,48.1965658036136));
#198558=CARTESIAN_POINT('Origin',(111.548590144925,4.25,48.1965658036136));
#198559=CARTESIAN_POINT('',(112.039403647474,4.25,48.2919707600629));
#198560=CARTESIAN_POINT('',(111.982160673605,4.25,48.5864588615926));
#198561=CARTESIAN_POINT('',(112.039403647474,4.25,48.2919707600629));
#198562=CARTESIAN_POINT('',(111.491347171055,4.25,48.4910539051433));
#198563=CARTESIAN_POINT('',(111.491347171055,4.25,48.4910539051433));
#198564=CARTESIAN_POINT('',(111.548590144925,4.25,48.1965658036136));
#198565=CARTESIAN_POINT('',(111.548590144925,4.25,48.1965658036136));
#198566=CARTESIAN_POINT('',(111.548590144925,4.25,48.1965658036136));
#198567=CARTESIAN_POINT('Origin',(112.039403647474,4.25,48.2919707600629));
#198568=CARTESIAN_POINT('',(112.039403647474,3.75,48.2919707600629));
#198569=CARTESIAN_POINT('',(111.982160673605,3.75,48.5864588615926));
#198570=CARTESIAN_POINT('',(112.039403647474,3.75,48.2919707600629));
#198571=CARTESIAN_POINT('',(111.982160673605,4.25,48.5864588615926));
#198572=CARTESIAN_POINT('',(112.039403647474,4.25,48.2919707600629));
#198573=CARTESIAN_POINT('Origin',(112.039403647474,3.75,48.2919707600629));
#198574=CARTESIAN_POINT('',(111.548590144925,3.75,48.1965658036136));
#198575=CARTESIAN_POINT('',(111.491347171055,3.75,48.4910539051433));
#198576=CARTESIAN_POINT('',(111.548590144925,3.75,48.1965658036136));
#198577=CARTESIAN_POINT('',(111.982160673605,3.75,48.5864588615926));
#198578=CARTESIAN_POINT('',(112.039403647474,3.75,48.2919707600629));
#198579=CARTESIAN_POINT('Origin',(111.548590144925,3.75,48.1965658036136));
#198580=CARTESIAN_POINT('',(111.491347171055,3.75,48.4910539051433));
#198581=CARTESIAN_POINT('',(111.548590144925,3.75,48.1965658036136));
#198582=CARTESIAN_POINT('Origin',(111.548590144925,3.45,48.1965658036136));
#198583=CARTESIAN_POINT('',(112.039403647474,3.45,48.2919707600629));
#198584=CARTESIAN_POINT('',(111.982160673605,3.45,48.5864588615926));
#198585=CARTESIAN_POINT('',(112.039403647474,3.45,48.2919707600629));
#198586=CARTESIAN_POINT('',(111.491347171055,3.45,48.4910539051433));
#198587=CARTESIAN_POINT('',(111.491347171055,3.45,48.4910539051433));
#198588=CARTESIAN_POINT('',(111.548590144925,3.45,48.1965658036136));
#198589=CARTESIAN_POINT('',(111.548590144925,3.45,48.1965658036136));
#198590=CARTESIAN_POINT('',(111.548590144925,3.45,48.1965658036136));
#198591=CARTESIAN_POINT('Origin',(112.039403647474,3.45,48.2919707600629));
#198592=CARTESIAN_POINT('',(112.039403647474,2.95,48.2919707600629));
#198593=CARTESIAN_POINT('',(111.982160673605,2.95,48.5864588615926));
#198594=CARTESIAN_POINT('',(112.039403647474,2.95,48.2919707600629));
#198595=CARTESIAN_POINT('',(111.982160673605,3.45,48.5864588615926));
#198596=CARTESIAN_POINT('',(112.039403647474,3.45,48.2919707600629));
#198597=CARTESIAN_POINT('Origin',(112.039403647474,2.95,48.2919707600629));
#198598=CARTESIAN_POINT('',(111.548590144925,2.95,48.1965658036136));
#198599=CARTESIAN_POINT('',(111.491347171055,2.95,48.4910539051433));
#198600=CARTESIAN_POINT('',(111.548590144925,2.95,48.1965658036136));
#198601=CARTESIAN_POINT('',(111.982160673605,2.95,48.5864588615926));
#198602=CARTESIAN_POINT('',(112.039403647474,2.95,48.2919707600629));
#198603=CARTESIAN_POINT('Origin',(111.548590144925,2.95,48.1965658036136));
#198604=CARTESIAN_POINT('',(111.491347171055,2.95,48.4910539051433));
#198605=CARTESIAN_POINT('',(111.548590144925,2.95,48.1965658036136));
#198606=CARTESIAN_POINT('Origin',(111.548590144925,2.65,48.1965658036136));
#198607=CARTESIAN_POINT('',(112.039403647474,2.65,48.2919707600629));
#198608=CARTESIAN_POINT('',(111.982160673605,2.65,48.5864588615926));
#198609=CARTESIAN_POINT('',(112.039403647474,2.65,48.2919707600629));
#198610=CARTESIAN_POINT('',(111.491347171055,2.65,48.4910539051433));
#198611=CARTESIAN_POINT('',(111.491347171055,2.65,48.4910539051433));
#198612=CARTESIAN_POINT('',(111.548590144925,2.65,48.1965658036136));
#198613=CARTESIAN_POINT('',(111.548590144925,2.65,48.1965658036136));
#198614=CARTESIAN_POINT('',(111.548590144925,2.65,48.1965658036136));
#198615=CARTESIAN_POINT('Origin',(112.039403647474,2.65,48.2919707600629));
#198616=CARTESIAN_POINT('',(112.039403647474,2.15,48.2919707600629));
#198617=CARTESIAN_POINT('',(111.982160673605,2.15,48.5864588615926));
#198618=CARTESIAN_POINT('',(112.039403647474,2.15,48.2919707600629));
#198619=CARTESIAN_POINT('',(111.982160673605,2.65,48.5864588615926));
#198620=CARTESIAN_POINT('',(112.039403647474,2.65,48.2919707600629));
#198621=CARTESIAN_POINT('Origin',(112.039403647474,2.15,48.2919707600629));
#198622=CARTESIAN_POINT('',(111.548590144925,2.15,48.1965658036136));
#198623=CARTESIAN_POINT('',(111.491347171055,2.15,48.4910539051433));
#198624=CARTESIAN_POINT('',(111.548590144925,2.15,48.1965658036136));
#198625=CARTESIAN_POINT('',(111.982160673605,2.15,48.5864588615926));
#198626=CARTESIAN_POINT('',(112.039403647474,2.15,48.2919707600629));
#198627=CARTESIAN_POINT('Origin',(111.548590144925,2.15,48.1965658036136));
#198628=CARTESIAN_POINT('',(111.491347171055,2.15,48.4910539051433));
#198629=CARTESIAN_POINT('',(111.548590144925,2.15,48.1965658036136));
#198630=CARTESIAN_POINT('Origin',(111.548590144925,1.85,48.1965658036136));
#198631=CARTESIAN_POINT('',(112.039403647474,1.85,48.2919707600629));
#198632=CARTESIAN_POINT('',(111.982160673605,1.85,48.5864588615926));
#198633=CARTESIAN_POINT('',(112.039403647474,1.85,48.2919707600629));
#198634=CARTESIAN_POINT('',(111.491347171055,1.85,48.4910539051433));
#198635=CARTESIAN_POINT('',(111.491347171055,1.85,48.4910539051433));
#198636=CARTESIAN_POINT('',(111.548590144925,1.85,48.1965658036136));
#198637=CARTESIAN_POINT('',(111.548590144925,1.85,48.1965658036136));
#198638=CARTESIAN_POINT('',(111.548590144925,1.85,48.1965658036136));
#198639=CARTESIAN_POINT('Origin',(112.039403647474,1.85,48.2919707600629));
#198640=CARTESIAN_POINT('',(112.039403647474,1.35,48.2919707600629));
#198641=CARTESIAN_POINT('',(111.982160673605,1.35,48.5864588615926));
#198642=CARTESIAN_POINT('',(112.039403647474,1.35,48.2919707600629));
#198643=CARTESIAN_POINT('',(111.982160673605,1.85,48.5864588615926));
#198644=CARTESIAN_POINT('',(112.039403647474,1.85,48.2919707600629));
#198645=CARTESIAN_POINT('Origin',(112.039403647474,1.35,48.2919707600629));
#198646=CARTESIAN_POINT('',(111.548590144925,1.35,48.1965658036136));
#198647=CARTESIAN_POINT('',(111.491347171055,1.35,48.4910539051433));
#198648=CARTESIAN_POINT('',(111.548590144925,1.35,48.1965658036136));
#198649=CARTESIAN_POINT('',(111.982160673605,1.35,48.5864588615926));
#198650=CARTESIAN_POINT('',(112.039403647474,1.35,48.2919707600629));
#198651=CARTESIAN_POINT('Origin',(111.548590144925,1.35,48.1965658036136));
#198652=CARTESIAN_POINT('',(111.491347171055,1.35,48.4910539051433));
#198653=CARTESIAN_POINT('',(111.548590144925,1.35,48.1965658036136));
#198654=CARTESIAN_POINT('Origin',(111.548590144925,1.05,48.1965658036136));
#198655=CARTESIAN_POINT('',(112.039403647474,1.05,48.2919707600629));
#198656=CARTESIAN_POINT('',(111.982160673605,1.05,48.5864588615926));
#198657=CARTESIAN_POINT('',(112.039403647474,1.05,48.2919707600629));
#198658=CARTESIAN_POINT('',(111.491347171055,1.05,48.4910539051433));
#198659=CARTESIAN_POINT('',(111.491347171055,1.05,48.4910539051433));
#198660=CARTESIAN_POINT('',(111.548590144925,1.05,48.1965658036136));
#198661=CARTESIAN_POINT('',(111.548590144925,1.05,48.1965658036136));
#198662=CARTESIAN_POINT('',(111.548590144925,1.05,48.1965658036136));
#198663=CARTESIAN_POINT('Origin',(112.039403647474,1.05,48.2919707600629));
#198664=CARTESIAN_POINT('',(112.039403647474,0.550000000000015,48.2919707600629));
#198665=CARTESIAN_POINT('',(111.982160673605,0.550000000000015,48.5864588615926));
#198666=CARTESIAN_POINT('',(112.039403647474,0.550000000000015,48.2919707600629));
#198667=CARTESIAN_POINT('',(111.982160673605,1.05,48.5864588615926));
#198668=CARTESIAN_POINT('',(112.039403647474,1.05,48.2919707600629));
#198669=CARTESIAN_POINT('Origin',(112.039403647474,0.550000000000015,48.2919707600629));
#198670=CARTESIAN_POINT('',(111.548590144925,0.550000000000015,48.1965658036136));
#198671=CARTESIAN_POINT('',(111.491347171055,0.550000000000015,48.4910539051433));
#198672=CARTESIAN_POINT('',(111.548590144925,0.550000000000015,48.1965658036136));
#198673=CARTESIAN_POINT('',(111.982160673605,0.550000000000015,48.5864588615926));
#198674=CARTESIAN_POINT('',(112.039403647474,0.550000000000015,48.2919707600629));
#198675=CARTESIAN_POINT('Origin',(111.548590144925,0.550000000000015,48.1965658036136));
#198676=CARTESIAN_POINT('',(111.491347171055,0.550000000000015,48.4910539051433));
#198677=CARTESIAN_POINT('',(111.548590144925,0.550000000000015,48.1965658036136));
#198678=CARTESIAN_POINT('Origin',(111.548590144925,0.250000000000015,48.1965658036136));
#198679=CARTESIAN_POINT('',(112.039403647474,0.250000000000015,48.2919707600629));
#198680=CARTESIAN_POINT('',(111.982160673605,0.250000000000015,48.5864588615926));
#198681=CARTESIAN_POINT('',(112.039403647474,0.250000000000015,48.2919707600629));
#198682=CARTESIAN_POINT('',(111.491347171055,0.250000000000015,48.4910539051433));
#198683=CARTESIAN_POINT('',(111.491347171055,0.250000000000015,48.4910539051433));
#198684=CARTESIAN_POINT('',(111.548590144925,0.250000000000015,48.1965658036136));
#198685=CARTESIAN_POINT('',(111.548590144925,0.250000000000015,48.1965658036136));
#198686=CARTESIAN_POINT('',(111.548590144925,0.250000000000015,48.1965658036136));
#198687=CARTESIAN_POINT('Origin',(112.039403647474,0.250000000000015,48.2919707600629));
#198688=CARTESIAN_POINT('',(112.039403647474,-0.249999999999985,48.2919707600629));
#198689=CARTESIAN_POINT('',(111.982160673605,-0.249999999999985,48.5864588615926));
#198690=CARTESIAN_POINT('',(112.039403647474,-0.249999999999985,48.2919707600629));
#198691=CARTESIAN_POINT('',(111.982160673605,0.250000000000015,48.5864588615926));
#198692=CARTESIAN_POINT('',(112.039403647474,0.250000000000015,48.2919707600629));
#198693=CARTESIAN_POINT('Origin',(112.039403647474,-0.249999999999985,48.2919707600629));
#198694=CARTESIAN_POINT('',(111.548590144925,-0.249999999999985,48.1965658036136));
#198695=CARTESIAN_POINT('',(111.491347171055,-0.249999999999985,48.4910539051433));
#198696=CARTESIAN_POINT('',(111.548590144925,-0.249999999999985,48.1965658036136));
#198697=CARTESIAN_POINT('',(111.982160673605,-0.249999999999985,48.5864588615926));
#198698=CARTESIAN_POINT('',(112.039403647474,-0.249999999999985,48.2919707600629));
#198699=CARTESIAN_POINT('Origin',(111.548590144925,-0.249999999999985,48.1965658036136));
#198700=CARTESIAN_POINT('',(111.491347171055,-0.249999999999985,48.4910539051433));
#198701=CARTESIAN_POINT('',(111.548590144925,-0.249999999999985,48.1965658036136));
#198702=CARTESIAN_POINT('Origin',(111.548590144925,-0.549999999999986,48.1965658036136));
#198703=CARTESIAN_POINT('',(112.039403647474,-0.549999999999986,48.2919707600629));
#198704=CARTESIAN_POINT('',(111.982160673605,-0.549999999999986,48.5864588615926));
#198705=CARTESIAN_POINT('',(112.039403647474,-0.549999999999986,48.2919707600629));
#198706=CARTESIAN_POINT('',(111.491347171055,-0.549999999999986,48.4910539051433));
#198707=CARTESIAN_POINT('',(111.491347171055,-0.549999999999986,48.4910539051433));
#198708=CARTESIAN_POINT('',(111.548590144925,-0.549999999999986,48.1965658036136));
#198709=CARTESIAN_POINT('',(111.548590144925,-0.549999999999986,48.1965658036136));
#198710=CARTESIAN_POINT('',(111.548590144925,-0.549999999999986,48.1965658036136));
#198711=CARTESIAN_POINT('Origin',(112.039403647474,-0.549999999999986,48.2919707600629));
#198712=CARTESIAN_POINT('',(112.039403647474,-1.05,48.2919707600629));
#198713=CARTESIAN_POINT('',(111.982160673605,-1.05,48.5864588615926));
#198714=CARTESIAN_POINT('',(112.039403647474,-1.05,48.2919707600629));
#198715=CARTESIAN_POINT('',(111.982160673605,-0.549999999999986,48.5864588615926));
#198716=CARTESIAN_POINT('',(112.039403647474,-0.549999999999986,48.2919707600629));
#198717=CARTESIAN_POINT('Origin',(112.039403647474,-1.05,48.2919707600629));
#198718=CARTESIAN_POINT('',(111.548590144925,-1.05,48.1965658036136));
#198719=CARTESIAN_POINT('',(111.491347171055,-1.05,48.4910539051433));
#198720=CARTESIAN_POINT('',(111.548590144925,-1.05,48.1965658036136));
#198721=CARTESIAN_POINT('',(111.982160673605,-1.05,48.5864588615926));
#198722=CARTESIAN_POINT('',(112.039403647474,-1.05,48.2919707600629));
#198723=CARTESIAN_POINT('Origin',(111.548590144925,-1.05,48.1965658036136));
#198724=CARTESIAN_POINT('',(111.491347171055,-1.05,48.4910539051433));
#198725=CARTESIAN_POINT('',(111.548590144925,-1.05,48.1965658036136));
#198726=CARTESIAN_POINT('Origin',(111.548590144925,-1.35,48.1965658036136));
#198727=CARTESIAN_POINT('',(112.039403647474,-1.35,48.2919707600629));
#198728=CARTESIAN_POINT('',(111.982160673605,-1.35,48.5864588615926));
#198729=CARTESIAN_POINT('',(112.039403647474,-1.35,48.2919707600629));
#198730=CARTESIAN_POINT('',(111.491347171055,-1.35,48.4910539051433));
#198731=CARTESIAN_POINT('',(111.491347171055,-1.35,48.4910539051433));
#198732=CARTESIAN_POINT('',(111.548590144925,-1.35,48.1965658036136));
#198733=CARTESIAN_POINT('',(111.548590144925,-1.35,48.1965658036136));
#198734=CARTESIAN_POINT('',(111.548590144925,-1.35,48.1965658036136));
#198735=CARTESIAN_POINT('Origin',(112.039403647474,-1.35,48.2919707600629));
#198736=CARTESIAN_POINT('',(112.039403647474,-1.85,48.2919707600629));
#198737=CARTESIAN_POINT('',(111.982160673605,-1.85,48.5864588615926));
#198738=CARTESIAN_POINT('',(112.039403647474,-1.85,48.2919707600629));
#198739=CARTESIAN_POINT('',(111.982160673605,-1.35,48.5864588615926));
#198740=CARTESIAN_POINT('',(112.039403647474,-1.35,48.2919707600629));
#198741=CARTESIAN_POINT('Origin',(112.039403647474,-1.85,48.2919707600629));
#198742=CARTESIAN_POINT('',(111.548590144925,-1.85,48.1965658036136));
#198743=CARTESIAN_POINT('',(111.491347171055,-1.85,48.4910539051433));
#198744=CARTESIAN_POINT('',(111.548590144925,-1.85,48.1965658036136));
#198745=CARTESIAN_POINT('',(111.982160673605,-1.85,48.5864588615926));
#198746=CARTESIAN_POINT('',(112.039403647474,-1.85,48.2919707600629));
#198747=CARTESIAN_POINT('Origin',(111.548590144925,-1.85,48.1965658036136));
#198748=CARTESIAN_POINT('',(111.491347171055,-1.85,48.4910539051433));
#198749=CARTESIAN_POINT('',(111.548590144925,-1.85,48.1965658036136));
#198750=CARTESIAN_POINT('Origin',(111.548590144925,-2.15,48.1965658036136));
#198751=CARTESIAN_POINT('',(112.039403647474,-2.15,48.2919707600629));
#198752=CARTESIAN_POINT('',(111.982160673605,-2.15,48.5864588615926));
#198753=CARTESIAN_POINT('',(112.039403647474,-2.15,48.2919707600629));
#198754=CARTESIAN_POINT('',(111.491347171055,-2.15,48.4910539051433));
#198755=CARTESIAN_POINT('',(111.491347171055,-2.15,48.4910539051433));
#198756=CARTESIAN_POINT('',(111.548590144925,-2.15,48.1965658036136));
#198757=CARTESIAN_POINT('',(111.548590144925,-2.15,48.1965658036136));
#198758=CARTESIAN_POINT('',(111.548590144925,-2.15,48.1965658036136));
#198759=CARTESIAN_POINT('Origin',(112.039403647474,-2.15,48.2919707600629));
#198760=CARTESIAN_POINT('',(112.039403647474,-2.65,48.2919707600629));
#198761=CARTESIAN_POINT('',(111.982160673605,-2.65,48.5864588615926));
#198762=CARTESIAN_POINT('',(112.039403647474,-2.65,48.2919707600629));
#198763=CARTESIAN_POINT('',(111.982160673605,-2.15,48.5864588615926));
#198764=CARTESIAN_POINT('',(112.039403647474,-2.15,48.2919707600629));
#198765=CARTESIAN_POINT('Origin',(112.039403647474,-2.65,48.2919707600629));
#198766=CARTESIAN_POINT('',(111.548590144925,-2.65,48.1965658036136));
#198767=CARTESIAN_POINT('',(111.491347171055,-2.65,48.4910539051433));
#198768=CARTESIAN_POINT('',(111.548590144925,-2.65,48.1965658036136));
#198769=CARTESIAN_POINT('',(111.982160673605,-2.65,48.5864588615926));
#198770=CARTESIAN_POINT('',(112.039403647474,-2.65,48.2919707600629));
#198771=CARTESIAN_POINT('Origin',(111.548590144925,-2.65,48.1965658036136));
#198772=CARTESIAN_POINT('',(111.491347171055,-2.65,48.4910539051433));
#198773=CARTESIAN_POINT('',(111.548590144925,-2.65,48.1965658036136));
#198774=CARTESIAN_POINT('Origin',(111.548590144925,-2.95,48.1965658036136));
#198775=CARTESIAN_POINT('',(112.039403647474,-2.95,48.2919707600629));
#198776=CARTESIAN_POINT('',(111.982160673605,-2.95,48.5864588615926));
#198777=CARTESIAN_POINT('',(112.039403647474,-2.95,48.2919707600629));
#198778=CARTESIAN_POINT('',(111.491347171055,-2.95,48.4910539051433));
#198779=CARTESIAN_POINT('',(111.491347171055,-2.95,48.4910539051433));
#198780=CARTESIAN_POINT('',(111.548590144925,-2.95,48.1965658036136));
#198781=CARTESIAN_POINT('',(111.548590144925,-2.95,48.1965658036136));
#198782=CARTESIAN_POINT('',(111.548590144925,-2.95,48.1965658036136));
#198783=CARTESIAN_POINT('Origin',(112.039403647474,-2.95,48.2919707600629));
#198784=CARTESIAN_POINT('',(112.039403647474,-3.45,48.2919707600629));
#198785=CARTESIAN_POINT('',(111.982160673605,-3.45,48.5864588615926));
#198786=CARTESIAN_POINT('',(112.039403647474,-3.45,48.2919707600629));
#198787=CARTESIAN_POINT('',(111.982160673605,-2.95,48.5864588615926));
#198788=CARTESIAN_POINT('',(112.039403647474,-2.95,48.2919707600629));
#198789=CARTESIAN_POINT('Origin',(112.039403647474,-3.45,48.2919707600629));
#198790=CARTESIAN_POINT('',(111.548590144925,-3.45,48.1965658036136));
#198791=CARTESIAN_POINT('',(111.491347171055,-3.45,48.4910539051433));
#198792=CARTESIAN_POINT('',(111.548590144925,-3.45,48.1965658036136));
#198793=CARTESIAN_POINT('',(111.982160673605,-3.45,48.5864588615926));
#198794=CARTESIAN_POINT('',(112.039403647474,-3.45,48.2919707600629));
#198795=CARTESIAN_POINT('Origin',(111.548590144925,-3.45,48.1965658036136));
#198796=CARTESIAN_POINT('',(111.491347171055,-3.45,48.4910539051433));
#198797=CARTESIAN_POINT('',(111.548590144925,-3.45,48.1965658036136));
#198798=CARTESIAN_POINT('Origin',(111.548590144925,-3.75,48.1965658036136));
#198799=CARTESIAN_POINT('',(112.039403647474,-3.75,48.2919707600629));
#198800=CARTESIAN_POINT('',(111.982160673605,-3.75,48.5864588615926));
#198801=CARTESIAN_POINT('',(112.039403647474,-3.75,48.2919707600629));
#198802=CARTESIAN_POINT('',(111.491347171055,-3.75,48.4910539051433));
#198803=CARTESIAN_POINT('',(111.491347171055,-3.75,48.4910539051433));
#198804=CARTESIAN_POINT('',(111.548590144925,-3.75,48.1965658036136));
#198805=CARTESIAN_POINT('',(111.548590144925,-3.75,48.1965658036136));
#198806=CARTESIAN_POINT('',(111.548590144925,-3.75,48.1965658036136));
#198807=CARTESIAN_POINT('Origin',(112.039403647474,-3.75,48.2919707600629));
#198808=CARTESIAN_POINT('',(112.039403647474,-4.25,48.2919707600629));
#198809=CARTESIAN_POINT('',(111.982160673605,-4.25,48.5864588615926));
#198810=CARTESIAN_POINT('',(112.039403647474,-4.25,48.2919707600629));
#198811=CARTESIAN_POINT('',(111.982160673605,-3.75,48.5864588615926));
#198812=CARTESIAN_POINT('',(112.039403647474,-3.75,48.2919707600629));
#198813=CARTESIAN_POINT('Origin',(112.039403647474,-4.25,48.2919707600629));
#198814=CARTESIAN_POINT('',(111.548590144925,-4.25,48.1965658036136));
#198815=CARTESIAN_POINT('',(111.491347171055,-4.25,48.4910539051433));
#198816=CARTESIAN_POINT('',(111.548590144925,-4.25,48.1965658036136));
#198817=CARTESIAN_POINT('',(111.982160673605,-4.25,48.5864588615926));
#198818=CARTESIAN_POINT('',(112.039403647474,-4.25,48.2919707600629));
#198819=CARTESIAN_POINT('Origin',(111.548590144925,-4.25,48.1965658036136));
#198820=CARTESIAN_POINT('',(111.491347171055,-4.25,48.4910539051433));
#198821=CARTESIAN_POINT('',(111.548590144925,-4.25,48.1965658036136));
#198822=CARTESIAN_POINT('Origin',(111.548590144925,-4.55,48.1965658036136));
#198823=CARTESIAN_POINT('',(112.039403647474,-4.55,48.2919707600629));
#198824=CARTESIAN_POINT('',(111.982160673605,-4.55,48.5864588615926));
#198825=CARTESIAN_POINT('',(112.039403647474,-4.55,48.2919707600629));
#198826=CARTESIAN_POINT('',(111.491347171055,-4.55,48.4910539051433));
#198827=CARTESIAN_POINT('',(111.491347171055,-4.55,48.4910539051433));
#198828=CARTESIAN_POINT('',(111.548590144925,-4.55,48.1965658036136));
#198829=CARTESIAN_POINT('',(111.548590144925,-4.55,48.1965658036136));
#198830=CARTESIAN_POINT('',(111.548590144925,-4.55,48.1965658036136));
#198831=CARTESIAN_POINT('Origin',(112.039403647474,-4.55,48.2919707600629));
#198832=CARTESIAN_POINT('',(112.039403647474,-5.05,48.2919707600629));
#198833=CARTESIAN_POINT('',(111.982160673605,-5.05,48.5864588615926));
#198834=CARTESIAN_POINT('',(112.039403647474,-5.05,48.2919707600629));
#198835=CARTESIAN_POINT('',(111.982160673605,-4.55,48.5864588615926));
#198836=CARTESIAN_POINT('',(112.039403647474,-4.55,48.2919707600629));
#198837=CARTESIAN_POINT('Origin',(112.039403647474,-5.05,48.2919707600629));
#198838=CARTESIAN_POINT('',(111.548590144925,-5.05,48.1965658036136));
#198839=CARTESIAN_POINT('',(111.491347171055,-5.05,48.4910539051433));
#198840=CARTESIAN_POINT('',(111.548590144925,-5.05,48.1965658036136));
#198841=CARTESIAN_POINT('',(111.982160673605,-5.05,48.5864588615926));
#198842=CARTESIAN_POINT('',(112.039403647474,-5.05,48.2919707600629));
#198843=CARTESIAN_POINT('Origin',(111.548590144925,-5.05,48.1965658036136));
#198844=CARTESIAN_POINT('',(111.491347171055,-5.05,48.4910539051433));
#198845=CARTESIAN_POINT('',(111.548590144925,-5.05,48.1965658036136));
#198846=CARTESIAN_POINT('Origin',(111.548590144925,-5.35,48.1965658036136));
#198847=CARTESIAN_POINT('',(112.039403647474,-5.35,48.2919707600629));
#198848=CARTESIAN_POINT('',(111.982160673605,-5.35,48.5864588615926));
#198849=CARTESIAN_POINT('',(112.039403647474,-5.35,48.2919707600629));
#198850=CARTESIAN_POINT('',(111.491347171055,-5.35,48.4910539051433));
#198851=CARTESIAN_POINT('',(111.491347171055,-5.35,48.4910539051433));
#198852=CARTESIAN_POINT('',(111.548590144925,-5.35,48.1965658036136));
#198853=CARTESIAN_POINT('',(111.548590144925,-5.35,48.1965658036136));
#198854=CARTESIAN_POINT('',(111.548590144925,-5.35,48.1965658036136));
#198855=CARTESIAN_POINT('Origin',(112.039403647474,-5.35,48.2919707600629));
#198856=CARTESIAN_POINT('',(112.039403647474,-5.85,48.2919707600629));
#198857=CARTESIAN_POINT('',(111.982160673605,-5.85,48.5864588615926));
#198858=CARTESIAN_POINT('',(112.039403647474,-5.85,48.2919707600629));
#198859=CARTESIAN_POINT('',(111.982160673605,-5.35,48.5864588615926));
#198860=CARTESIAN_POINT('',(112.039403647474,-5.35,48.2919707600629));
#198861=CARTESIAN_POINT('Origin',(112.039403647474,-5.85,48.2919707600629));
#198862=CARTESIAN_POINT('',(111.548590144925,-5.85,48.1965658036136));
#198863=CARTESIAN_POINT('',(111.491347171055,-5.85,48.4910539051433));
#198864=CARTESIAN_POINT('',(111.548590144925,-5.85,48.1965658036136));
#198865=CARTESIAN_POINT('',(111.982160673605,-5.85,48.5864588615926));
#198866=CARTESIAN_POINT('',(112.039403647474,-5.85,48.2919707600629));
#198867=CARTESIAN_POINT('Origin',(111.548590144925,-5.85,48.1965658036136));
#198868=CARTESIAN_POINT('',(111.491347171055,-5.85,48.4910539051433));
#198869=CARTESIAN_POINT('',(111.548590144925,-5.85,48.1965658036136));
#198870=CARTESIAN_POINT('Origin',(112.333891749004,-5.35,48.3492137339324));
#198871=CARTESIAN_POINT('',(112.824705251554,-5.35,48.4446186903817));
#198872=CARTESIAN_POINT('',(112.767462277684,-5.35,48.7391067919114));
#198873=CARTESIAN_POINT('',(112.824705251554,-5.35,48.4446186903817));
#198874=CARTESIAN_POINT('',(112.276648775135,-5.35,48.6437018354621));
#198875=CARTESIAN_POINT('',(112.276648775135,-5.35,48.6437018354621));
#198876=CARTESIAN_POINT('',(112.333891749004,-5.35,48.3492137339324));
#198877=CARTESIAN_POINT('',(112.333891749004,-5.35,48.3492137339324));
#198878=CARTESIAN_POINT('',(112.333891749004,-5.35,48.3492137339324));
#198879=CARTESIAN_POINT('Origin',(112.824705251554,-5.35,48.4446186903817));
#198880=CARTESIAN_POINT('',(112.824705251554,-5.85,48.4446186903817));
#198881=CARTESIAN_POINT('',(112.767462277684,-5.85,48.7391067919114));
#198882=CARTESIAN_POINT('',(112.824705251554,-5.85,48.4446186903817));
#198883=CARTESIAN_POINT('',(112.767462277684,-5.35,48.7391067919114));
#198884=CARTESIAN_POINT('',(112.824705251554,-5.35,48.4446186903817));
#198885=CARTESIAN_POINT('Origin',(112.824705251554,-5.85,48.4446186903817));
#198886=CARTESIAN_POINT('',(112.333891749004,-5.85,48.3492137339324));
#198887=CARTESIAN_POINT('',(112.276648775135,-5.85,48.6437018354621));
#198888=CARTESIAN_POINT('',(112.333891749004,-5.85,48.3492137339324));
#198889=CARTESIAN_POINT('',(112.767462277684,-5.85,48.7391067919114));
#198890=CARTESIAN_POINT('',(112.824705251554,-5.85,48.4446186903817));
#198891=CARTESIAN_POINT('Origin',(112.333891749004,-5.85,48.3492137339324));
#198892=CARTESIAN_POINT('',(112.276648775135,-5.85,48.6437018354621));
#198893=CARTESIAN_POINT('',(112.333891749004,-5.85,48.3492137339324));
#198894=CARTESIAN_POINT('Origin',(113.119193353083,-5.35,48.5018616642512));
#198895=CARTESIAN_POINT('',(113.610006855633,-5.35,48.5972666207005));
#198896=CARTESIAN_POINT('',(113.552763881763,-5.35,48.8917547222302));
#198897=CARTESIAN_POINT('',(113.610006855633,-5.35,48.5972666207005));
#198898=CARTESIAN_POINT('',(113.061950379214,-5.35,48.7963497657809));
#198899=CARTESIAN_POINT('',(113.061950379214,-5.35,48.7963497657809));
#198900=CARTESIAN_POINT('',(113.119193353083,-5.35,48.5018616642512));
#198901=CARTESIAN_POINT('',(113.119193353083,-5.35,48.5018616642512));
#198902=CARTESIAN_POINT('',(113.119193353083,-5.35,48.5018616642512));
#198903=CARTESIAN_POINT('Origin',(113.610006855633,-5.35,48.5972666207005));
#198904=CARTESIAN_POINT('',(113.610006855633,-5.85,48.5972666207005));
#198905=CARTESIAN_POINT('',(113.552763881763,-5.85,48.8917547222302));
#198906=CARTESIAN_POINT('',(113.610006855633,-5.85,48.5972666207005));
#198907=CARTESIAN_POINT('',(113.552763881763,-5.35,48.8917547222302));
#198908=CARTESIAN_POINT('',(113.610006855633,-5.35,48.5972666207005));
#198909=CARTESIAN_POINT('Origin',(113.610006855633,-5.85,48.5972666207005));
#198910=CARTESIAN_POINT('',(113.119193353083,-5.85,48.5018616642512));
#198911=CARTESIAN_POINT('',(113.061950379214,-5.85,48.7963497657809));
#198912=CARTESIAN_POINT('',(113.119193353083,-5.85,48.5018616642512));
#198913=CARTESIAN_POINT('',(113.552763881763,-5.85,48.8917547222302));
#198914=CARTESIAN_POINT('',(113.610006855633,-5.85,48.5972666207005));
#198915=CARTESIAN_POINT('Origin',(113.119193353083,-5.85,48.5018616642512));
#198916=CARTESIAN_POINT('',(113.061950379214,-5.85,48.7963497657809));
#198917=CARTESIAN_POINT('',(113.119193353083,-5.85,48.5018616642512));
#198918=CARTESIAN_POINT('Origin',(113.904494957163,-5.35,48.65450959457));
#198919=CARTESIAN_POINT('',(114.395308459712,-5.35,48.7499145510193));
#198920=CARTESIAN_POINT('',(114.338065485842,-5.35,49.044402652549));
#198921=CARTESIAN_POINT('',(114.395308459712,-5.35,48.7499145510193));
#198922=CARTESIAN_POINT('',(113.847251983293,-5.35,48.9489976960997));
#198923=CARTESIAN_POINT('',(113.847251983293,-5.35,48.9489976960997));
#198924=CARTESIAN_POINT('',(113.904494957163,-5.35,48.65450959457));
#198925=CARTESIAN_POINT('',(113.904494957163,-5.35,48.65450959457));
#198926=CARTESIAN_POINT('',(113.904494957163,-5.35,48.65450959457));
#198927=CARTESIAN_POINT('Origin',(114.395308459712,-5.35,48.7499145510193));
#198928=CARTESIAN_POINT('',(114.395308459712,-5.85,48.7499145510193));
#198929=CARTESIAN_POINT('',(114.338065485842,-5.85,49.044402652549));
#198930=CARTESIAN_POINT('',(114.395308459712,-5.85,48.7499145510193));
#198931=CARTESIAN_POINT('',(114.338065485842,-5.35,49.044402652549));
#198932=CARTESIAN_POINT('',(114.395308459712,-5.35,48.7499145510193));
#198933=CARTESIAN_POINT('Origin',(114.395308459712,-5.85,48.7499145510193));
#198934=CARTESIAN_POINT('',(113.904494957163,-5.85,48.65450959457));
#198935=CARTESIAN_POINT('',(113.847251983293,-5.85,48.9489976960997));
#198936=CARTESIAN_POINT('',(113.904494957163,-5.85,48.65450959457));
#198937=CARTESIAN_POINT('',(114.338065485842,-5.85,49.044402652549));
#198938=CARTESIAN_POINT('',(114.395308459712,-5.85,48.7499145510193));
#198939=CARTESIAN_POINT('Origin',(113.904494957163,-5.85,48.65450959457));
#198940=CARTESIAN_POINT('',(113.847251983293,-5.85,48.9489976960997));
#198941=CARTESIAN_POINT('',(113.904494957163,-5.85,48.65450959457));
#198942=CARTESIAN_POINT('Origin',(114.689796561242,-5.35,48.8071575248888));
#198943=CARTESIAN_POINT('',(115.180610063791,-5.35,48.9025624813381));
#198944=CARTESIAN_POINT('',(115.123367089922,-5.35,49.1970505828678));
#198945=CARTESIAN_POINT('',(115.180610063791,-5.35,48.9025624813381));
#198946=CARTESIAN_POINT('',(114.632553587372,-5.35,49.1016456264185));
#198947=CARTESIAN_POINT('',(114.632553587372,-5.35,49.1016456264185));
#198948=CARTESIAN_POINT('',(114.689796561242,-5.35,48.8071575248888));
#198949=CARTESIAN_POINT('',(114.689796561242,-5.35,48.8071575248888));
#198950=CARTESIAN_POINT('',(114.689796561242,-5.35,48.8071575248888));
#198951=CARTESIAN_POINT('Origin',(115.180610063791,-5.35,48.9025624813381));
#198952=CARTESIAN_POINT('',(115.180610063791,-5.85,48.9025624813381));
#198953=CARTESIAN_POINT('',(115.123367089922,-5.85,49.1970505828678));
#198954=CARTESIAN_POINT('',(115.180610063791,-5.85,48.9025624813381));
#198955=CARTESIAN_POINT('',(115.123367089922,-5.35,49.1970505828678));
#198956=CARTESIAN_POINT('',(115.180610063791,-5.35,48.9025624813381));
#198957=CARTESIAN_POINT('Origin',(115.180610063791,-5.85,48.9025624813381));
#198958=CARTESIAN_POINT('',(114.689796561242,-5.85,48.8071575248888));
#198959=CARTESIAN_POINT('',(114.632553587372,-5.85,49.1016456264185));
#198960=CARTESIAN_POINT('',(114.689796561242,-5.85,48.8071575248888));
#198961=CARTESIAN_POINT('',(115.123367089922,-5.85,49.1970505828678));
#198962=CARTESIAN_POINT('',(115.180610063791,-5.85,48.9025624813381));
#198963=CARTESIAN_POINT('Origin',(114.689796561242,-5.85,48.8071575248888));
#198964=CARTESIAN_POINT('',(114.632553587372,-5.85,49.1016456264185));
#198965=CARTESIAN_POINT('',(114.689796561242,-5.85,48.8071575248888));
#198966=CARTESIAN_POINT('Origin',(115.475098165321,-5.35,48.9598054552076));
#198967=CARTESIAN_POINT('',(115.96591166787,-5.35,49.0552104116569));
#198968=CARTESIAN_POINT('',(115.908668694001,-5.35,49.3496985131866));
#198969=CARTESIAN_POINT('',(115.96591166787,-5.35,49.0552104116569));
#198970=CARTESIAN_POINT('',(115.417855191451,-5.35,49.2542935567373));
#198971=CARTESIAN_POINT('',(115.417855191451,-5.35,49.2542935567373));
#198972=CARTESIAN_POINT('',(115.475098165321,-5.35,48.9598054552076));
#198973=CARTESIAN_POINT('',(115.475098165321,-5.35,48.9598054552076));
#198974=CARTESIAN_POINT('',(115.475098165321,-5.35,48.9598054552076));
#198975=CARTESIAN_POINT('Origin',(115.96591166787,-5.35,49.0552104116569));
#198976=CARTESIAN_POINT('',(115.96591166787,-5.85,49.0552104116569));
#198977=CARTESIAN_POINT('',(115.908668694001,-5.85,49.3496985131866));
#198978=CARTESIAN_POINT('',(115.96591166787,-5.85,49.0552104116569));
#198979=CARTESIAN_POINT('',(115.908668694001,-5.35,49.3496985131866));
#198980=CARTESIAN_POINT('',(115.96591166787,-5.35,49.0552104116569));
#198981=CARTESIAN_POINT('Origin',(115.96591166787,-5.85,49.0552104116569));
#198982=CARTESIAN_POINT('',(115.475098165321,-5.85,48.9598054552076));
#198983=CARTESIAN_POINT('',(115.417855191451,-5.85,49.2542935567373));
#198984=CARTESIAN_POINT('',(115.475098165321,-5.85,48.9598054552076));
#198985=CARTESIAN_POINT('',(115.908668694001,-5.85,49.3496985131866));
#198986=CARTESIAN_POINT('',(115.96591166787,-5.85,49.0552104116569));
#198987=CARTESIAN_POINT('Origin',(115.475098165321,-5.85,48.9598054552076));
#198988=CARTESIAN_POINT('',(115.417855191451,-5.85,49.2542935567373));
#198989=CARTESIAN_POINT('',(115.475098165321,-5.85,48.9598054552076));
#198990=CARTESIAN_POINT('Origin',(116.2603997694,-5.35,49.1124533855264));
#198991=CARTESIAN_POINT('',(116.75121327195,-5.35,49.2078583419757));
#198992=CARTESIAN_POINT('',(116.69397029808,-5.35,49.5023464435054));
#198993=CARTESIAN_POINT('',(116.75121327195,-5.35,49.2078583419757));
#198994=CARTESIAN_POINT('',(116.203156795531,-5.35,49.4069414870561));
#198995=CARTESIAN_POINT('',(116.203156795531,-5.35,49.4069414870561));
#198996=CARTESIAN_POINT('',(116.2603997694,-5.35,49.1124533855264));
#198997=CARTESIAN_POINT('',(116.2603997694,-5.35,49.1124533855264));
#198998=CARTESIAN_POINT('',(116.2603997694,-5.35,49.1124533855264));
#198999=CARTESIAN_POINT('Origin',(116.75121327195,-5.35,49.2078583419757));
#199000=CARTESIAN_POINT('',(116.75121327195,-5.85,49.2078583419757));
#199001=CARTESIAN_POINT('',(116.69397029808,-5.85,49.5023464435054));
#199002=CARTESIAN_POINT('',(116.75121327195,-5.85,49.2078583419757));
#199003=CARTESIAN_POINT('',(116.69397029808,-5.35,49.5023464435054));
#199004=CARTESIAN_POINT('',(116.75121327195,-5.35,49.2078583419757));
#199005=CARTESIAN_POINT('Origin',(116.75121327195,-5.85,49.2078583419757));
#199006=CARTESIAN_POINT('',(116.2603997694,-5.85,49.1124533855264));
#199007=CARTESIAN_POINT('',(116.203156795531,-5.85,49.4069414870561));
#199008=CARTESIAN_POINT('',(116.2603997694,-5.85,49.1124533855264));
#199009=CARTESIAN_POINT('',(116.69397029808,-5.85,49.5023464435054));
#199010=CARTESIAN_POINT('',(116.75121327195,-5.85,49.2078583419757));
#199011=CARTESIAN_POINT('Origin',(116.2603997694,-5.85,49.1124533855264));
#199012=CARTESIAN_POINT('',(116.203156795531,-5.85,49.4069414870561));
#199013=CARTESIAN_POINT('',(116.2603997694,-5.85,49.1124533855264));
#199014=CARTESIAN_POINT('Origin',(117.045701373479,-5.35,49.2651013158452));
#199015=CARTESIAN_POINT('',(117.536514876029,-5.35,49.3605062722945));
#199016=CARTESIAN_POINT('',(117.479271902159,-5.35,49.6549943738242));
#199017=CARTESIAN_POINT('',(117.536514876029,-5.35,49.3605062722945));
#199018=CARTESIAN_POINT('',(116.98845839961,-5.35,49.5595894173749));
#199019=CARTESIAN_POINT('',(116.98845839961,-5.35,49.5595894173749));
#199020=CARTESIAN_POINT('',(117.045701373479,-5.35,49.2651013158452));
#199021=CARTESIAN_POINT('',(117.045701373479,-5.35,49.2651013158452));
#199022=CARTESIAN_POINT('',(117.045701373479,-5.35,49.2651013158452));
#199023=CARTESIAN_POINT('Origin',(117.536514876029,-5.35,49.3605062722945));
#199024=CARTESIAN_POINT('',(117.536514876029,-5.85,49.3605062722945));
#199025=CARTESIAN_POINT('',(117.479271902159,-5.85,49.6549943738242));
#199026=CARTESIAN_POINT('',(117.536514876029,-5.85,49.3605062722945));
#199027=CARTESIAN_POINT('',(117.479271902159,-5.35,49.6549943738242));
#199028=CARTESIAN_POINT('',(117.536514876029,-5.35,49.3605062722945));
#199029=CARTESIAN_POINT('Origin',(117.536514876029,-5.85,49.3605062722945));
#199030=CARTESIAN_POINT('',(117.045701373479,-5.85,49.2651013158452));
#199031=CARTESIAN_POINT('',(116.98845839961,-5.85,49.5595894173749));
#199032=CARTESIAN_POINT('',(117.045701373479,-5.85,49.2651013158452));
#199033=CARTESIAN_POINT('',(117.479271902159,-5.85,49.6549943738242));
#199034=CARTESIAN_POINT('',(117.536514876029,-5.85,49.3605062722945));
#199035=CARTESIAN_POINT('Origin',(117.045701373479,-5.85,49.2651013158452));
#199036=CARTESIAN_POINT('',(116.98845839961,-5.85,49.5595894173749));
#199037=CARTESIAN_POINT('',(117.045701373479,-5.85,49.2651013158452));
#199038=CARTESIAN_POINT('Origin',(117.831002977559,-5.35,49.417749246164));
#199039=CARTESIAN_POINT('',(118.321816480108,-5.35,49.5131542026133));
#199040=CARTESIAN_POINT('',(118.264573506239,-5.35,49.807642304143));
#199041=CARTESIAN_POINT('',(118.321816480108,-5.35,49.5131542026133));
#199042=CARTESIAN_POINT('',(117.773760003689,-5.35,49.7122373476937));
#199043=CARTESIAN_POINT('',(117.773760003689,-5.35,49.7122373476937));
#199044=CARTESIAN_POINT('',(117.831002977559,-5.35,49.417749246164));
#199045=CARTESIAN_POINT('',(117.831002977559,-5.35,49.417749246164));
#199046=CARTESIAN_POINT('',(117.831002977559,-5.35,49.417749246164));
#199047=CARTESIAN_POINT('Origin',(118.321816480108,-5.35,49.5131542026133));
#199048=CARTESIAN_POINT('',(118.321816480108,-5.85,49.5131542026133));
#199049=CARTESIAN_POINT('',(118.264573506239,-5.85,49.807642304143));
#199050=CARTESIAN_POINT('',(118.321816480108,-5.85,49.5131542026133));
#199051=CARTESIAN_POINT('',(118.264573506239,-5.35,49.807642304143));
#199052=CARTESIAN_POINT('',(118.321816480108,-5.35,49.5131542026133));
#199053=CARTESIAN_POINT('Origin',(118.321816480108,-5.85,49.5131542026133));
#199054=CARTESIAN_POINT('',(117.831002977559,-5.85,49.417749246164));
#199055=CARTESIAN_POINT('',(117.773760003689,-5.85,49.7122373476937));
#199056=CARTESIAN_POINT('',(117.831002977559,-5.85,49.417749246164));
#199057=CARTESIAN_POINT('',(118.264573506239,-5.85,49.807642304143));
#199058=CARTESIAN_POINT('',(118.321816480108,-5.85,49.5131542026133));
#199059=CARTESIAN_POINT('Origin',(117.831002977559,-5.85,49.417749246164));
#199060=CARTESIAN_POINT('',(117.773760003689,-5.85,49.7122373476937));
#199061=CARTESIAN_POINT('',(117.831002977559,-5.85,49.417749246164));
#199062=CARTESIAN_POINT('Origin',(118.616304581638,-5.35,49.5703971764828));
#199063=CARTESIAN_POINT('',(119.107118084187,-5.35,49.6658021329321));
#199064=CARTESIAN_POINT('',(119.049875110318,-5.35,49.9602902344618));
#199065=CARTESIAN_POINT('',(119.107118084187,-5.35,49.6658021329321));
#199066=CARTESIAN_POINT('',(118.559061607768,-5.35,49.8648852780125));
#199067=CARTESIAN_POINT('',(118.559061607768,-5.35,49.8648852780125));
#199068=CARTESIAN_POINT('',(118.616304581638,-5.35,49.5703971764828));
#199069=CARTESIAN_POINT('',(118.616304581638,-5.35,49.5703971764828));
#199070=CARTESIAN_POINT('',(118.616304581638,-5.35,49.5703971764828));
#199071=CARTESIAN_POINT('Origin',(119.107118084187,-5.35,49.6658021329321));
#199072=CARTESIAN_POINT('',(119.107118084187,-5.85,49.6658021329321));
#199073=CARTESIAN_POINT('',(119.049875110318,-5.85,49.9602902344618));
#199074=CARTESIAN_POINT('',(119.107118084187,-5.85,49.6658021329321));
#199075=CARTESIAN_POINT('',(119.049875110318,-5.35,49.9602902344618));
#199076=CARTESIAN_POINT('',(119.107118084187,-5.35,49.6658021329321));
#199077=CARTESIAN_POINT('Origin',(119.107118084187,-5.85,49.6658021329321));
#199078=CARTESIAN_POINT('',(118.616304581638,-5.85,49.5703971764828));
#199079=CARTESIAN_POINT('',(118.559061607768,-5.85,49.8648852780125));
#199080=CARTESIAN_POINT('',(118.616304581638,-5.85,49.5703971764828));
#199081=CARTESIAN_POINT('',(119.049875110318,-5.85,49.9602902344618));
#199082=CARTESIAN_POINT('',(119.107118084187,-5.85,49.6658021329321));
#199083=CARTESIAN_POINT('Origin',(118.616304581638,-5.85,49.5703971764828));
#199084=CARTESIAN_POINT('',(118.559061607768,-5.85,49.8648852780125));
#199085=CARTESIAN_POINT('',(118.616304581638,-5.85,49.5703971764828));
#199086=CARTESIAN_POINT('Origin',(119.401606185717,-5.35,49.7230451068016));
#199087=CARTESIAN_POINT('',(119.892419688267,-5.35,49.8184500632509));
#199088=CARTESIAN_POINT('',(119.835176714397,-5.35,50.1129381647806));
#199089=CARTESIAN_POINT('',(119.892419688267,-5.35,49.8184500632509));
#199090=CARTESIAN_POINT('',(119.344363211847,-5.35,50.0175332083313));
#199091=CARTESIAN_POINT('',(119.344363211847,-5.35,50.0175332083313));
#199092=CARTESIAN_POINT('',(119.401606185717,-5.35,49.7230451068016));
#199093=CARTESIAN_POINT('',(119.401606185717,-5.35,49.7230451068016));
#199094=CARTESIAN_POINT('',(119.401606185717,-5.35,49.7230451068016));
#199095=CARTESIAN_POINT('Origin',(119.892419688267,-5.35,49.8184500632509));
#199096=CARTESIAN_POINT('',(119.892419688267,-5.85,49.8184500632509));
#199097=CARTESIAN_POINT('',(119.835176714397,-5.85,50.1129381647806));
#199098=CARTESIAN_POINT('',(119.892419688267,-5.85,49.8184500632509));
#199099=CARTESIAN_POINT('',(119.835176714397,-5.35,50.1129381647806));
#199100=CARTESIAN_POINT('',(119.892419688267,-5.35,49.8184500632509));
#199101=CARTESIAN_POINT('Origin',(119.892419688267,-5.85,49.8184500632509));
#199102=CARTESIAN_POINT('',(119.401606185717,-5.85,49.7230451068016));
#199103=CARTESIAN_POINT('',(119.344363211847,-5.85,50.0175332083313));
#199104=CARTESIAN_POINT('',(119.401606185717,-5.85,49.7230451068016));
#199105=CARTESIAN_POINT('',(119.835176714397,-5.85,50.1129381647806));
#199106=CARTESIAN_POINT('',(119.892419688267,-5.85,49.8184500632509));
#199107=CARTESIAN_POINT('Origin',(119.401606185717,-5.85,49.7230451068016));
#199108=CARTESIAN_POINT('',(119.344363211847,-5.85,50.0175332083313));
#199109=CARTESIAN_POINT('',(119.401606185717,-5.85,49.7230451068016));
#199110=CARTESIAN_POINT('Origin',(120.186907789796,-5.35,49.8756930371204));
#199111=CARTESIAN_POINT('',(120.677721292346,-5.35,49.9710979935697));
#199112=CARTESIAN_POINT('',(120.620478318476,-5.35,50.2655860950994));
#199113=CARTESIAN_POINT('',(120.677721292346,-5.35,49.9710979935697));
#199114=CARTESIAN_POINT('',(120.129664815927,-5.35,50.1701811386501));
#199115=CARTESIAN_POINT('',(120.129664815927,-5.35,50.1701811386501));
#199116=CARTESIAN_POINT('',(120.186907789796,-5.35,49.8756930371204));
#199117=CARTESIAN_POINT('',(120.186907789796,-5.35,49.8756930371204));
#199118=CARTESIAN_POINT('',(120.186907789796,-5.35,49.8756930371204));
#199119=CARTESIAN_POINT('Origin',(120.677721292346,-5.35,49.9710979935697));
#199120=CARTESIAN_POINT('',(120.677721292346,-5.85,49.9710979935697));
#199121=CARTESIAN_POINT('',(120.620478318476,-5.85,50.2655860950994));
#199122=CARTESIAN_POINT('',(120.677721292346,-5.85,49.9710979935697));
#199123=CARTESIAN_POINT('',(120.620478318476,-5.35,50.2655860950994));
#199124=CARTESIAN_POINT('',(120.677721292346,-5.35,49.9710979935697));
#199125=CARTESIAN_POINT('Origin',(120.677721292346,-5.85,49.9710979935697));
#199126=CARTESIAN_POINT('',(120.186907789796,-5.85,49.8756930371204));
#199127=CARTESIAN_POINT('',(120.129664815927,-5.85,50.1701811386501));
#199128=CARTESIAN_POINT('',(120.186907789796,-5.85,49.8756930371204));
#199129=CARTESIAN_POINT('',(120.620478318476,-5.85,50.2655860950994));
#199130=CARTESIAN_POINT('',(120.677721292346,-5.85,49.9710979935697));
#199131=CARTESIAN_POINT('Origin',(120.186907789796,-5.85,49.8756930371204));
#199132=CARTESIAN_POINT('',(120.129664815927,-5.85,50.1701811386501));
#199133=CARTESIAN_POINT('',(120.186907789796,-5.85,49.8756930371204));
#199134=CARTESIAN_POINT('Origin',(120.972209393875,-5.35,50.0283409674392));
#199135=CARTESIAN_POINT('',(121.463022896425,-5.35,50.1237459238885));
#199136=CARTESIAN_POINT('',(121.405779922555,-5.35,50.4182340254182));
#199137=CARTESIAN_POINT('',(121.463022896425,-5.35,50.1237459238885));
#199138=CARTESIAN_POINT('',(120.914966420006,-5.35,50.3228290689689));
#199139=CARTESIAN_POINT('',(120.914966420006,-5.35,50.3228290689689));
#199140=CARTESIAN_POINT('',(120.972209393875,-5.35,50.0283409674392));
#199141=CARTESIAN_POINT('',(120.972209393875,-5.35,50.0283409674392));
#199142=CARTESIAN_POINT('',(120.972209393875,-5.35,50.0283409674392));
#199143=CARTESIAN_POINT('Origin',(121.463022896425,-5.35,50.1237459238885));
#199144=CARTESIAN_POINT('',(121.463022896425,-5.85,50.1237459238885));
#199145=CARTESIAN_POINT('',(121.405779922555,-5.85,50.4182340254182));
#199146=CARTESIAN_POINT('',(121.463022896425,-5.85,50.1237459238885));
#199147=CARTESIAN_POINT('',(121.405779922555,-5.35,50.4182340254182));
#199148=CARTESIAN_POINT('',(121.463022896425,-5.35,50.1237459238885));
#199149=CARTESIAN_POINT('Origin',(121.463022896425,-5.85,50.1237459238885));
#199150=CARTESIAN_POINT('',(120.972209393875,-5.85,50.0283409674392));
#199151=CARTESIAN_POINT('',(120.914966420006,-5.85,50.3228290689689));
#199152=CARTESIAN_POINT('',(120.972209393875,-5.85,50.0283409674392));
#199153=CARTESIAN_POINT('',(121.405779922555,-5.85,50.4182340254182));
#199154=CARTESIAN_POINT('',(121.463022896425,-5.85,50.1237459238885));
#199155=CARTESIAN_POINT('Origin',(120.972209393875,-5.85,50.0283409674392));
#199156=CARTESIAN_POINT('',(120.914966420006,-5.85,50.3228290689689));
#199157=CARTESIAN_POINT('',(120.972209393875,-5.85,50.0283409674392));
#199158=CARTESIAN_POINT('Origin',(121.757510997955,-5.35,50.180988897758));
#199159=CARTESIAN_POINT('',(122.248324500504,-5.35,50.2763938542073));
#199160=CARTESIAN_POINT('',(122.191081526635,-5.35,50.570881955737));
#199161=CARTESIAN_POINT('',(122.248324500504,-5.35,50.2763938542073));
#199162=CARTESIAN_POINT('',(121.700268024085,-5.35,50.4754769992877));
#199163=CARTESIAN_POINT('',(121.700268024085,-5.35,50.4754769992877));
#199164=CARTESIAN_POINT('',(121.757510997955,-5.35,50.180988897758));
#199165=CARTESIAN_POINT('',(121.757510997955,-5.35,50.180988897758));
#199166=CARTESIAN_POINT('',(121.757510997955,-5.35,50.180988897758));
#199167=CARTESIAN_POINT('Origin',(122.248324500504,-5.35,50.2763938542073));
#199168=CARTESIAN_POINT('',(122.248324500504,-5.85,50.2763938542073));
#199169=CARTESIAN_POINT('',(122.191081526635,-5.85,50.570881955737));
#199170=CARTESIAN_POINT('',(122.248324500504,-5.85,50.2763938542073));
#199171=CARTESIAN_POINT('',(122.191081526635,-5.35,50.570881955737));
#199172=CARTESIAN_POINT('',(122.248324500504,-5.35,50.2763938542073));
#199173=CARTESIAN_POINT('Origin',(122.248324500504,-5.85,50.2763938542073));
#199174=CARTESIAN_POINT('',(121.757510997955,-5.85,50.180988897758));
#199175=CARTESIAN_POINT('',(121.700268024085,-5.85,50.4754769992877));
#199176=CARTESIAN_POINT('',(121.757510997955,-5.85,50.180988897758));
#199177=CARTESIAN_POINT('',(122.191081526635,-5.85,50.570881955737));
#199178=CARTESIAN_POINT('',(122.248324500504,-5.85,50.2763938542073));
#199179=CARTESIAN_POINT('Origin',(121.757510997955,-5.85,50.180988897758));
#199180=CARTESIAN_POINT('',(121.700268024085,-5.85,50.4754769992877));
#199181=CARTESIAN_POINT('',(121.757510997955,-5.85,50.180988897758));
#199182=CARTESIAN_POINT('Origin',(122.542812602034,-5.35,50.3336368280768));
#199183=CARTESIAN_POINT('',(123.033626104583,-5.35,50.4290417845261));
#199184=CARTESIAN_POINT('',(122.976383130714,-5.35,50.7235298860558));
#199185=CARTESIAN_POINT('',(123.033626104583,-5.35,50.4290417845261));
#199186=CARTESIAN_POINT('',(122.485569628164,-5.35,50.6281249296065));
#199187=CARTESIAN_POINT('',(122.485569628164,-5.35,50.6281249296065));
#199188=CARTESIAN_POINT('',(122.542812602034,-5.35,50.3336368280768));
#199189=CARTESIAN_POINT('',(122.542812602034,-5.35,50.3336368280768));
#199190=CARTESIAN_POINT('',(122.542812602034,-5.35,50.3336368280768));
#199191=CARTESIAN_POINT('Origin',(123.033626104583,-5.35,50.4290417845261));
#199192=CARTESIAN_POINT('',(123.033626104583,-5.85,50.4290417845261));
#199193=CARTESIAN_POINT('',(122.976383130714,-5.85,50.7235298860558));
#199194=CARTESIAN_POINT('',(123.033626104583,-5.85,50.4290417845261));
#199195=CARTESIAN_POINT('',(122.976383130714,-5.35,50.7235298860558));
#199196=CARTESIAN_POINT('',(123.033626104583,-5.35,50.4290417845261));
#199197=CARTESIAN_POINT('Origin',(123.033626104583,-5.85,50.4290417845261));
#199198=CARTESIAN_POINT('',(122.542812602034,-5.85,50.3336368280768));
#199199=CARTESIAN_POINT('',(122.485569628164,-5.85,50.6281249296065));
#199200=CARTESIAN_POINT('',(122.542812602034,-5.85,50.3336368280768));
#199201=CARTESIAN_POINT('',(122.976383130714,-5.85,50.7235298860558));
#199202=CARTESIAN_POINT('',(123.033626104583,-5.85,50.4290417845261));
#199203=CARTESIAN_POINT('Origin',(122.542812602034,-5.85,50.3336368280768));
#199204=CARTESIAN_POINT('',(122.485569628164,-5.85,50.6281249296065));
#199205=CARTESIAN_POINT('',(122.542812602034,-5.85,50.3336368280768));
#199206=CARTESIAN_POINT('Origin',(122.542812602034,-4.55,50.3336368280768));
#199207=CARTESIAN_POINT('',(123.033626104583,-4.55,50.4290417845261));
#199208=CARTESIAN_POINT('',(122.976383130714,-4.55,50.7235298860558));
#199209=CARTESIAN_POINT('',(123.033626104583,-4.55,50.4290417845261));
#199210=CARTESIAN_POINT('',(122.485569628164,-4.55,50.6281249296065));
#199211=CARTESIAN_POINT('',(122.485569628164,-4.55,50.6281249296065));
#199212=CARTESIAN_POINT('',(122.542812602034,-4.55,50.3336368280768));
#199213=CARTESIAN_POINT('',(122.542812602034,-4.55,50.3336368280768));
#199214=CARTESIAN_POINT('',(122.542812602034,-4.55,50.3336368280768));
#199215=CARTESIAN_POINT('Origin',(123.033626104583,-4.55,50.4290417845261));
#199216=CARTESIAN_POINT('',(123.033626104583,-5.05,50.4290417845261));
#199217=CARTESIAN_POINT('',(122.976383130714,-5.05,50.7235298860558));
#199218=CARTESIAN_POINT('',(123.033626104583,-5.05,50.4290417845261));
#199219=CARTESIAN_POINT('',(122.976383130714,-4.55,50.7235298860558));
#199220=CARTESIAN_POINT('',(123.033626104583,-4.55,50.4290417845261));
#199221=CARTESIAN_POINT('Origin',(123.033626104583,-5.05,50.4290417845261));
#199222=CARTESIAN_POINT('',(122.542812602034,-5.05,50.3336368280768));
#199223=CARTESIAN_POINT('',(122.485569628164,-5.05,50.6281249296065));
#199224=CARTESIAN_POINT('',(122.542812602034,-5.05,50.3336368280768));
#199225=CARTESIAN_POINT('',(122.976383130714,-5.05,50.7235298860558));
#199226=CARTESIAN_POINT('',(123.033626104583,-5.05,50.4290417845261));
#199227=CARTESIAN_POINT('Origin',(122.542812602034,-5.05,50.3336368280768));
#199228=CARTESIAN_POINT('',(122.485569628164,-5.05,50.6281249296065));
#199229=CARTESIAN_POINT('',(122.542812602034,-5.05,50.3336368280768));
#199230=CARTESIAN_POINT('Origin',(122.542812602034,-3.75,50.3336368280768));
#199231=CARTESIAN_POINT('',(123.033626104583,-3.75,50.4290417845261));
#199232=CARTESIAN_POINT('',(122.976383130714,-3.75,50.7235298860558));
#199233=CARTESIAN_POINT('',(123.033626104583,-3.75,50.4290417845261));
#199234=CARTESIAN_POINT('',(122.485569628164,-3.75,50.6281249296065));
#199235=CARTESIAN_POINT('',(122.485569628164,-3.75,50.6281249296065));
#199236=CARTESIAN_POINT('',(122.542812602034,-3.75,50.3336368280768));
#199237=CARTESIAN_POINT('',(122.542812602034,-3.75,50.3336368280768));
#199238=CARTESIAN_POINT('',(122.542812602034,-3.75,50.3336368280768));
#199239=CARTESIAN_POINT('Origin',(123.033626104583,-3.75,50.4290417845261));
#199240=CARTESIAN_POINT('',(123.033626104583,-4.25,50.4290417845261));
#199241=CARTESIAN_POINT('',(122.976383130714,-4.25,50.7235298860558));
#199242=CARTESIAN_POINT('',(123.033626104583,-4.25,50.4290417845261));
#199243=CARTESIAN_POINT('',(122.976383130714,-3.75,50.7235298860558));
#199244=CARTESIAN_POINT('',(123.033626104583,-3.75,50.4290417845261));
#199245=CARTESIAN_POINT('Origin',(123.033626104583,-4.25,50.4290417845261));
#199246=CARTESIAN_POINT('',(122.542812602034,-4.25,50.3336368280768));
#199247=CARTESIAN_POINT('',(122.485569628164,-4.25,50.6281249296065));
#199248=CARTESIAN_POINT('',(122.542812602034,-4.25,50.3336368280768));
#199249=CARTESIAN_POINT('',(122.976383130714,-4.25,50.7235298860558));
#199250=CARTESIAN_POINT('',(123.033626104583,-4.25,50.4290417845261));
#199251=CARTESIAN_POINT('Origin',(122.542812602034,-4.25,50.3336368280768));
#199252=CARTESIAN_POINT('',(122.485569628164,-4.25,50.6281249296065));
#199253=CARTESIAN_POINT('',(122.542812602034,-4.25,50.3336368280768));
#199254=CARTESIAN_POINT('Origin',(122.542812602034,-2.95,50.3336368280768));
#199255=CARTESIAN_POINT('',(123.033626104583,-2.95,50.4290417845261));
#199256=CARTESIAN_POINT('',(122.976383130714,-2.95,50.7235298860558));
#199257=CARTESIAN_POINT('',(123.033626104583,-2.95,50.4290417845261));
#199258=CARTESIAN_POINT('',(122.485569628164,-2.95,50.6281249296065));
#199259=CARTESIAN_POINT('',(122.485569628164,-2.95,50.6281249296065));
#199260=CARTESIAN_POINT('',(122.542812602034,-2.95,50.3336368280768));
#199261=CARTESIAN_POINT('',(122.542812602034,-2.95,50.3336368280768));
#199262=CARTESIAN_POINT('',(122.542812602034,-2.95,50.3336368280768));
#199263=CARTESIAN_POINT('Origin',(123.033626104583,-2.95,50.4290417845261));
#199264=CARTESIAN_POINT('',(123.033626104583,-3.45,50.4290417845261));
#199265=CARTESIAN_POINT('',(122.976383130714,-3.45,50.7235298860558));
#199266=CARTESIAN_POINT('',(123.033626104583,-3.45,50.4290417845261));
#199267=CARTESIAN_POINT('',(122.976383130714,-2.95,50.7235298860558));
#199268=CARTESIAN_POINT('',(123.033626104583,-2.95,50.4290417845261));
#199269=CARTESIAN_POINT('Origin',(123.033626104583,-3.45,50.4290417845261));
#199270=CARTESIAN_POINT('',(122.542812602034,-3.45,50.3336368280768));
#199271=CARTESIAN_POINT('',(122.485569628164,-3.45,50.6281249296065));
#199272=CARTESIAN_POINT('',(122.542812602034,-3.45,50.3336368280768));
#199273=CARTESIAN_POINT('',(122.976383130714,-3.45,50.7235298860558));
#199274=CARTESIAN_POINT('',(123.033626104583,-3.45,50.4290417845261));
#199275=CARTESIAN_POINT('Origin',(122.542812602034,-3.45,50.3336368280768));
#199276=CARTESIAN_POINT('',(122.485569628164,-3.45,50.6281249296065));
#199277=CARTESIAN_POINT('',(122.542812602034,-3.45,50.3336368280768));
#199278=CARTESIAN_POINT('Origin',(122.542812602034,-2.15,50.3336368280768));
#199279=CARTESIAN_POINT('',(123.033626104583,-2.15,50.4290417845261));
#199280=CARTESIAN_POINT('',(122.976383130714,-2.15,50.7235298860558));
#199281=CARTESIAN_POINT('',(123.033626104583,-2.15,50.4290417845261));
#199282=CARTESIAN_POINT('',(122.485569628164,-2.15,50.6281249296065));
#199283=CARTESIAN_POINT('',(122.485569628164,-2.15,50.6281249296065));
#199284=CARTESIAN_POINT('',(122.542812602034,-2.15,50.3336368280768));
#199285=CARTESIAN_POINT('',(122.542812602034,-2.15,50.3336368280768));
#199286=CARTESIAN_POINT('',(122.542812602034,-2.15,50.3336368280768));
#199287=CARTESIAN_POINT('Origin',(123.033626104583,-2.15,50.4290417845261));
#199288=CARTESIAN_POINT('',(123.033626104583,-2.65,50.4290417845261));
#199289=CARTESIAN_POINT('',(122.976383130714,-2.65,50.7235298860558));
#199290=CARTESIAN_POINT('',(123.033626104583,-2.65,50.4290417845261));
#199291=CARTESIAN_POINT('',(122.976383130714,-2.15,50.7235298860558));
#199292=CARTESIAN_POINT('',(123.033626104583,-2.15,50.4290417845261));
#199293=CARTESIAN_POINT('Origin',(123.033626104583,-2.65,50.4290417845261));
#199294=CARTESIAN_POINT('',(122.542812602034,-2.65,50.3336368280768));
#199295=CARTESIAN_POINT('',(122.485569628164,-2.65,50.6281249296065));
#199296=CARTESIAN_POINT('',(122.542812602034,-2.65,50.3336368280768));
#199297=CARTESIAN_POINT('',(122.976383130714,-2.65,50.7235298860558));
#199298=CARTESIAN_POINT('',(123.033626104583,-2.65,50.4290417845261));
#199299=CARTESIAN_POINT('Origin',(122.542812602034,-2.65,50.3336368280768));
#199300=CARTESIAN_POINT('',(122.485569628164,-2.65,50.6281249296065));
#199301=CARTESIAN_POINT('',(122.542812602034,-2.65,50.3336368280768));
#199302=CARTESIAN_POINT('Origin',(122.542812602034,-1.35,50.3336368280768));
#199303=CARTESIAN_POINT('',(123.033626104583,-1.35,50.4290417845261));
#199304=CARTESIAN_POINT('',(122.976383130714,-1.35,50.7235298860558));
#199305=CARTESIAN_POINT('',(123.033626104583,-1.35,50.4290417845261));
#199306=CARTESIAN_POINT('',(122.485569628164,-1.35,50.6281249296065));
#199307=CARTESIAN_POINT('',(122.485569628164,-1.35,50.6281249296065));
#199308=CARTESIAN_POINT('',(122.542812602034,-1.35,50.3336368280768));
#199309=CARTESIAN_POINT('',(122.542812602034,-1.35,50.3336368280768));
#199310=CARTESIAN_POINT('',(122.542812602034,-1.35,50.3336368280768));
#199311=CARTESIAN_POINT('Origin',(123.033626104583,-1.35,50.4290417845261));
#199312=CARTESIAN_POINT('',(123.033626104583,-1.85,50.4290417845261));
#199313=CARTESIAN_POINT('',(122.976383130714,-1.85,50.7235298860558));
#199314=CARTESIAN_POINT('',(123.033626104583,-1.85,50.4290417845261));
#199315=CARTESIAN_POINT('',(122.976383130714,-1.35,50.7235298860558));
#199316=CARTESIAN_POINT('',(123.033626104583,-1.35,50.4290417845261));
#199317=CARTESIAN_POINT('Origin',(123.033626104583,-1.85,50.4290417845261));
#199318=CARTESIAN_POINT('',(122.542812602034,-1.85,50.3336368280768));
#199319=CARTESIAN_POINT('',(122.485569628164,-1.85,50.6281249296065));
#199320=CARTESIAN_POINT('',(122.542812602034,-1.85,50.3336368280768));
#199321=CARTESIAN_POINT('',(122.976383130714,-1.85,50.7235298860558));
#199322=CARTESIAN_POINT('',(123.033626104583,-1.85,50.4290417845261));
#199323=CARTESIAN_POINT('Origin',(122.542812602034,-1.85,50.3336368280768));
#199324=CARTESIAN_POINT('',(122.485569628164,-1.85,50.6281249296065));
#199325=CARTESIAN_POINT('',(122.542812602034,-1.85,50.3336368280768));
#199326=CARTESIAN_POINT('Origin',(122.542812602034,-0.549999999999986,50.3336368280768));
#199327=CARTESIAN_POINT('',(123.033626104583,-0.549999999999986,50.4290417845261));
#199328=CARTESIAN_POINT('',(122.976383130714,-0.549999999999986,50.7235298860558));
#199329=CARTESIAN_POINT('',(123.033626104583,-0.549999999999986,50.4290417845261));
#199330=CARTESIAN_POINT('',(122.485569628164,-0.549999999999986,50.6281249296065));
#199331=CARTESIAN_POINT('',(122.485569628164,-0.549999999999986,50.6281249296065));
#199332=CARTESIAN_POINT('',(122.542812602034,-0.549999999999986,50.3336368280768));
#199333=CARTESIAN_POINT('',(122.542812602034,-0.549999999999986,50.3336368280768));
#199334=CARTESIAN_POINT('',(122.542812602034,-0.549999999999986,50.3336368280768));
#199335=CARTESIAN_POINT('Origin',(123.033626104583,-0.549999999999986,50.4290417845261));
#199336=CARTESIAN_POINT('',(123.033626104583,-1.05,50.4290417845261));
#199337=CARTESIAN_POINT('',(122.976383130714,-1.05,50.7235298860558));
#199338=CARTESIAN_POINT('',(123.033626104583,-1.05,50.4290417845261));
#199339=CARTESIAN_POINT('',(122.976383130714,-0.549999999999986,50.7235298860558));
#199340=CARTESIAN_POINT('',(123.033626104583,-0.549999999999986,50.4290417845261));
#199341=CARTESIAN_POINT('Origin',(123.033626104583,-1.05,50.4290417845261));
#199342=CARTESIAN_POINT('',(122.542812602034,-1.05,50.3336368280768));
#199343=CARTESIAN_POINT('',(122.485569628164,-1.05,50.6281249296065));
#199344=CARTESIAN_POINT('',(122.542812602034,-1.05,50.3336368280768));
#199345=CARTESIAN_POINT('',(122.976383130714,-1.05,50.7235298860558));
#199346=CARTESIAN_POINT('',(123.033626104583,-1.05,50.4290417845261));
#199347=CARTESIAN_POINT('Origin',(122.542812602034,-1.05,50.3336368280768));
#199348=CARTESIAN_POINT('',(122.485569628164,-1.05,50.6281249296065));
#199349=CARTESIAN_POINT('',(122.542812602034,-1.05,50.3336368280768));
#199350=CARTESIAN_POINT('Origin',(122.542812602034,0.250000000000015,50.3336368280768));
#199351=CARTESIAN_POINT('',(123.033626104583,0.250000000000015,50.4290417845261));
#199352=CARTESIAN_POINT('',(122.976383130714,0.250000000000015,50.7235298860558));
#199353=CARTESIAN_POINT('',(123.033626104583,0.250000000000015,50.4290417845261));
#199354=CARTESIAN_POINT('',(122.485569628164,0.250000000000015,50.6281249296065));
#199355=CARTESIAN_POINT('',(122.485569628164,0.250000000000015,50.6281249296065));
#199356=CARTESIAN_POINT('',(122.542812602034,0.250000000000015,50.3336368280768));
#199357=CARTESIAN_POINT('',(122.542812602034,0.250000000000015,50.3336368280768));
#199358=CARTESIAN_POINT('',(122.542812602034,0.250000000000015,50.3336368280768));
#199359=CARTESIAN_POINT('Origin',(123.033626104583,0.250000000000015,50.4290417845261));
#199360=CARTESIAN_POINT('',(123.033626104583,-0.249999999999985,50.4290417845261));
#199361=CARTESIAN_POINT('',(122.976383130714,-0.249999999999985,50.7235298860558));
#199362=CARTESIAN_POINT('',(123.033626104583,-0.249999999999985,50.4290417845261));
#199363=CARTESIAN_POINT('',(122.976383130714,0.250000000000015,50.7235298860558));
#199364=CARTESIAN_POINT('',(123.033626104583,0.250000000000015,50.4290417845261));
#199365=CARTESIAN_POINT('Origin',(123.033626104583,-0.249999999999985,50.4290417845261));
#199366=CARTESIAN_POINT('',(122.542812602034,-0.249999999999985,50.3336368280768));
#199367=CARTESIAN_POINT('',(122.485569628164,-0.249999999999985,50.6281249296065));
#199368=CARTESIAN_POINT('',(122.542812602034,-0.249999999999985,50.3336368280768));
#199369=CARTESIAN_POINT('',(122.976383130714,-0.249999999999985,50.7235298860558));
#199370=CARTESIAN_POINT('',(123.033626104583,-0.249999999999985,50.4290417845261));
#199371=CARTESIAN_POINT('Origin',(122.542812602034,-0.249999999999985,50.3336368280768));
#199372=CARTESIAN_POINT('',(122.485569628164,-0.249999999999985,50.6281249296065));
#199373=CARTESIAN_POINT('',(122.542812602034,-0.249999999999985,50.3336368280768));
#199374=CARTESIAN_POINT('Origin',(122.542812602034,1.05,50.3336368280768));
#199375=CARTESIAN_POINT('',(123.033626104583,1.05,50.4290417845261));
#199376=CARTESIAN_POINT('',(122.976383130714,1.05,50.7235298860558));
#199377=CARTESIAN_POINT('',(123.033626104583,1.05,50.4290417845261));
#199378=CARTESIAN_POINT('',(122.485569628164,1.05,50.6281249296065));
#199379=CARTESIAN_POINT('',(122.485569628164,1.05,50.6281249296065));
#199380=CARTESIAN_POINT('',(122.542812602034,1.05,50.3336368280768));
#199381=CARTESIAN_POINT('',(122.542812602034,1.05,50.3336368280768));
#199382=CARTESIAN_POINT('',(122.542812602034,1.05,50.3336368280768));
#199383=CARTESIAN_POINT('Origin',(123.033626104583,1.05,50.4290417845261));
#199384=CARTESIAN_POINT('',(123.033626104583,0.550000000000015,50.4290417845261));
#199385=CARTESIAN_POINT('',(122.976383130714,0.550000000000015,50.7235298860558));
#199386=CARTESIAN_POINT('',(123.033626104583,0.550000000000015,50.4290417845261));
#199387=CARTESIAN_POINT('',(122.976383130714,1.05,50.7235298860558));
#199388=CARTESIAN_POINT('',(123.033626104583,1.05,50.4290417845261));
#199389=CARTESIAN_POINT('Origin',(123.033626104583,0.550000000000015,50.4290417845261));
#199390=CARTESIAN_POINT('',(122.542812602034,0.550000000000015,50.3336368280768));
#199391=CARTESIAN_POINT('',(122.485569628164,0.550000000000015,50.6281249296065));
#199392=CARTESIAN_POINT('',(122.542812602034,0.550000000000015,50.3336368280768));
#199393=CARTESIAN_POINT('',(122.976383130714,0.550000000000015,50.7235298860558));
#199394=CARTESIAN_POINT('',(123.033626104583,0.550000000000015,50.4290417845261));
#199395=CARTESIAN_POINT('Origin',(122.542812602034,0.550000000000015,50.3336368280768));
#199396=CARTESIAN_POINT('',(122.485569628164,0.550000000000015,50.6281249296065));
#199397=CARTESIAN_POINT('',(122.542812602034,0.550000000000015,50.3336368280768));
#199398=CARTESIAN_POINT('Origin',(122.542812602034,1.85,50.3336368280768));
#199399=CARTESIAN_POINT('',(123.033626104583,1.85,50.4290417845261));
#199400=CARTESIAN_POINT('',(122.976383130714,1.85,50.7235298860558));
#199401=CARTESIAN_POINT('',(123.033626104583,1.85,50.4290417845261));
#199402=CARTESIAN_POINT('',(122.485569628164,1.85,50.6281249296065));
#199403=CARTESIAN_POINT('',(122.485569628164,1.85,50.6281249296065));
#199404=CARTESIAN_POINT('',(122.542812602034,1.85,50.3336368280768));
#199405=CARTESIAN_POINT('',(122.542812602034,1.85,50.3336368280768));
#199406=CARTESIAN_POINT('',(122.542812602034,1.85,50.3336368280768));
#199407=CARTESIAN_POINT('Origin',(123.033626104583,1.85,50.4290417845261));
#199408=CARTESIAN_POINT('',(123.033626104583,1.35,50.4290417845261));
#199409=CARTESIAN_POINT('',(122.976383130714,1.35,50.7235298860558));
#199410=CARTESIAN_POINT('',(123.033626104583,1.35,50.4290417845261));
#199411=CARTESIAN_POINT('',(122.976383130714,1.85,50.7235298860558));
#199412=CARTESIAN_POINT('',(123.033626104583,1.85,50.4290417845261));
#199413=CARTESIAN_POINT('Origin',(123.033626104583,1.35,50.4290417845261));
#199414=CARTESIAN_POINT('',(122.542812602034,1.35,50.3336368280768));
#199415=CARTESIAN_POINT('',(122.485569628164,1.35,50.6281249296065));
#199416=CARTESIAN_POINT('',(122.542812602034,1.35,50.3336368280768));
#199417=CARTESIAN_POINT('',(122.976383130714,1.35,50.7235298860558));
#199418=CARTESIAN_POINT('',(123.033626104583,1.35,50.4290417845261));
#199419=CARTESIAN_POINT('Origin',(122.542812602034,1.35,50.3336368280768));
#199420=CARTESIAN_POINT('',(122.485569628164,1.35,50.6281249296065));
#199421=CARTESIAN_POINT('',(122.542812602034,1.35,50.3336368280768));
#199422=CARTESIAN_POINT('Origin',(122.542812602034,2.65,50.3336368280768));
#199423=CARTESIAN_POINT('',(123.033626104583,2.65,50.4290417845261));
#199424=CARTESIAN_POINT('',(122.976383130714,2.65,50.7235298860558));
#199425=CARTESIAN_POINT('',(123.033626104583,2.65,50.4290417845261));
#199426=CARTESIAN_POINT('',(122.485569628164,2.65,50.6281249296065));
#199427=CARTESIAN_POINT('',(122.485569628164,2.65,50.6281249296065));
#199428=CARTESIAN_POINT('',(122.542812602034,2.65,50.3336368280768));
#199429=CARTESIAN_POINT('',(122.542812602034,2.65,50.3336368280768));
#199430=CARTESIAN_POINT('',(122.542812602034,2.65,50.3336368280768));
#199431=CARTESIAN_POINT('Origin',(123.033626104583,2.65,50.4290417845261));
#199432=CARTESIAN_POINT('',(123.033626104583,2.15,50.4290417845261));
#199433=CARTESIAN_POINT('',(122.976383130714,2.15,50.7235298860558));
#199434=CARTESIAN_POINT('',(123.033626104583,2.15,50.4290417845261));
#199435=CARTESIAN_POINT('',(122.976383130714,2.65,50.7235298860558));
#199436=CARTESIAN_POINT('',(123.033626104583,2.65,50.4290417845261));
#199437=CARTESIAN_POINT('Origin',(123.033626104583,2.15,50.4290417845261));
#199438=CARTESIAN_POINT('',(122.542812602034,2.15,50.3336368280768));
#199439=CARTESIAN_POINT('',(122.485569628164,2.15,50.6281249296065));
#199440=CARTESIAN_POINT('',(122.542812602034,2.15,50.3336368280768));
#199441=CARTESIAN_POINT('',(122.976383130714,2.15,50.7235298860558));
#199442=CARTESIAN_POINT('',(123.033626104583,2.15,50.4290417845261));
#199443=CARTESIAN_POINT('Origin',(122.542812602034,2.15,50.3336368280768));
#199444=CARTESIAN_POINT('',(122.485569628164,2.15,50.6281249296065));
#199445=CARTESIAN_POINT('',(122.542812602034,2.15,50.3336368280768));
#199446=CARTESIAN_POINT('Origin',(122.542812602034,3.45,50.3336368280768));
#199447=CARTESIAN_POINT('',(123.033626104583,3.45,50.4290417845261));
#199448=CARTESIAN_POINT('',(122.976383130714,3.45,50.7235298860558));
#199449=CARTESIAN_POINT('',(123.033626104583,3.45,50.4290417845261));
#199450=CARTESIAN_POINT('',(122.485569628164,3.45,50.6281249296065));
#199451=CARTESIAN_POINT('',(122.485569628164,3.45,50.6281249296065));
#199452=CARTESIAN_POINT('',(122.542812602034,3.45,50.3336368280768));
#199453=CARTESIAN_POINT('',(122.542812602034,3.45,50.3336368280768));
#199454=CARTESIAN_POINT('',(122.542812602034,3.45,50.3336368280768));
#199455=CARTESIAN_POINT('Origin',(123.033626104583,3.45,50.4290417845261));
#199456=CARTESIAN_POINT('',(123.033626104583,2.95,50.4290417845261));
#199457=CARTESIAN_POINT('',(122.976383130714,2.95,50.7235298860558));
#199458=CARTESIAN_POINT('',(123.033626104583,2.95,50.4290417845261));
#199459=CARTESIAN_POINT('',(122.976383130714,3.45,50.7235298860558));
#199460=CARTESIAN_POINT('',(123.033626104583,3.45,50.4290417845261));
#199461=CARTESIAN_POINT('Origin',(123.033626104583,2.95,50.4290417845261));
#199462=CARTESIAN_POINT('',(122.542812602034,2.95,50.3336368280768));
#199463=CARTESIAN_POINT('',(122.485569628164,2.95,50.6281249296065));
#199464=CARTESIAN_POINT('',(122.542812602034,2.95,50.3336368280768));
#199465=CARTESIAN_POINT('',(122.976383130714,2.95,50.7235298860558));
#199466=CARTESIAN_POINT('',(123.033626104583,2.95,50.4290417845261));
#199467=CARTESIAN_POINT('Origin',(122.542812602034,2.95,50.3336368280768));
#199468=CARTESIAN_POINT('',(122.485569628164,2.95,50.6281249296065));
#199469=CARTESIAN_POINT('',(122.542812602034,2.95,50.3336368280768));
#199470=CARTESIAN_POINT('Origin',(122.542812602034,4.25,50.3336368280768));
#199471=CARTESIAN_POINT('',(123.033626104583,4.25,50.4290417845261));
#199472=CARTESIAN_POINT('',(122.976383130714,4.25,50.7235298860558));
#199473=CARTESIAN_POINT('',(123.033626104583,4.25,50.4290417845261));
#199474=CARTESIAN_POINT('',(122.485569628164,4.25,50.6281249296065));
#199475=CARTESIAN_POINT('',(122.485569628164,4.25,50.6281249296065));
#199476=CARTESIAN_POINT('',(122.542812602034,4.25,50.3336368280768));
#199477=CARTESIAN_POINT('',(122.542812602034,4.25,50.3336368280768));
#199478=CARTESIAN_POINT('',(122.542812602034,4.25,50.3336368280768));
#199479=CARTESIAN_POINT('Origin',(123.033626104583,4.25,50.4290417845261));
#199480=CARTESIAN_POINT('',(123.033626104583,3.75,50.4290417845261));
#199481=CARTESIAN_POINT('',(122.976383130714,3.75,50.7235298860558));
#199482=CARTESIAN_POINT('',(123.033626104583,3.75,50.4290417845261));
#199483=CARTESIAN_POINT('',(122.976383130714,4.25,50.7235298860558));
#199484=CARTESIAN_POINT('',(123.033626104583,4.25,50.4290417845261));
#199485=CARTESIAN_POINT('Origin',(123.033626104583,3.75,50.4290417845261));
#199486=CARTESIAN_POINT('',(122.542812602034,3.75,50.3336368280768));
#199487=CARTESIAN_POINT('',(122.485569628164,3.75,50.6281249296065));
#199488=CARTESIAN_POINT('',(122.542812602034,3.75,50.3336368280768));
#199489=CARTESIAN_POINT('',(122.976383130714,3.75,50.7235298860558));
#199490=CARTESIAN_POINT('',(123.033626104583,3.75,50.4290417845261));
#199491=CARTESIAN_POINT('Origin',(122.542812602034,3.75,50.3336368280768));
#199492=CARTESIAN_POINT('',(122.485569628164,3.75,50.6281249296065));
#199493=CARTESIAN_POINT('',(122.542812602034,3.75,50.3336368280768));
#199494=CARTESIAN_POINT('Origin',(122.542812602034,5.05,50.3336368280768));
#199495=CARTESIAN_POINT('',(123.033626104583,5.05,50.4290417845261));
#199496=CARTESIAN_POINT('',(122.976383130714,5.05,50.7235298860558));
#199497=CARTESIAN_POINT('',(123.033626104583,5.05,50.4290417845261));
#199498=CARTESIAN_POINT('',(122.485569628164,5.05,50.6281249296065));
#199499=CARTESIAN_POINT('',(122.485569628164,5.05,50.6281249296065));
#199500=CARTESIAN_POINT('',(122.542812602034,5.05,50.3336368280768));
#199501=CARTESIAN_POINT('',(122.542812602034,5.05,50.3336368280768));
#199502=CARTESIAN_POINT('',(122.542812602034,5.05,50.3336368280768));
#199503=CARTESIAN_POINT('Origin',(123.033626104583,5.05,50.4290417845261));
#199504=CARTESIAN_POINT('',(123.033626104583,4.55,50.4290417845261));
#199505=CARTESIAN_POINT('',(122.976383130714,4.55,50.7235298860558));
#199506=CARTESIAN_POINT('',(123.033626104583,4.55,50.4290417845261));
#199507=CARTESIAN_POINT('',(122.976383130714,5.05,50.7235298860558));
#199508=CARTESIAN_POINT('',(123.033626104583,5.05,50.4290417845261));
#199509=CARTESIAN_POINT('Origin',(123.033626104583,4.55,50.4290417845261));
#199510=CARTESIAN_POINT('',(122.542812602034,4.55,50.3336368280768));
#199511=CARTESIAN_POINT('',(122.485569628164,4.55,50.6281249296065));
#199512=CARTESIAN_POINT('',(122.542812602034,4.55,50.3336368280768));
#199513=CARTESIAN_POINT('',(122.976383130714,4.55,50.7235298860558));
#199514=CARTESIAN_POINT('',(123.033626104583,4.55,50.4290417845261));
#199515=CARTESIAN_POINT('Origin',(122.542812602034,4.55,50.3336368280768));
#199516=CARTESIAN_POINT('',(122.485569628164,4.55,50.6281249296065));
#199517=CARTESIAN_POINT('',(122.542812602034,4.55,50.3336368280768));
#199518=CARTESIAN_POINT('Origin',(122.542812602034,5.85,50.3336368280768));
#199519=CARTESIAN_POINT('',(123.033626104583,5.85,50.4290417845261));
#199520=CARTESIAN_POINT('',(122.976383130714,5.85,50.7235298860558));
#199521=CARTESIAN_POINT('',(123.033626104583,5.85,50.4290417845261));
#199522=CARTESIAN_POINT('',(122.485569628164,5.85,50.6281249296065));
#199523=CARTESIAN_POINT('',(122.485569628164,5.85,50.6281249296065));
#199524=CARTESIAN_POINT('',(122.542812602034,5.85,50.3336368280768));
#199525=CARTESIAN_POINT('',(122.542812602034,5.85,50.3336368280768));
#199526=CARTESIAN_POINT('',(122.542812602034,5.85,50.3336368280768));
#199527=CARTESIAN_POINT('Origin',(123.033626104583,5.85,50.4290417845261));
#199528=CARTESIAN_POINT('',(123.033626104583,5.35,50.4290417845261));
#199529=CARTESIAN_POINT('',(122.976383130714,5.35,50.7235298860558));
#199530=CARTESIAN_POINT('',(123.033626104583,5.35,50.4290417845261));
#199531=CARTESIAN_POINT('',(122.976383130714,5.85,50.7235298860558));
#199532=CARTESIAN_POINT('',(123.033626104583,5.85,50.4290417845261));
#199533=CARTESIAN_POINT('Origin',(123.033626104583,5.35,50.4290417845261));
#199534=CARTESIAN_POINT('',(122.542812602034,5.35,50.3336368280768));
#199535=CARTESIAN_POINT('',(122.485569628164,5.35,50.6281249296065));
#199536=CARTESIAN_POINT('',(122.542812602034,5.35,50.3336368280768));
#199537=CARTESIAN_POINT('',(122.976383130714,5.35,50.7235298860558));
#199538=CARTESIAN_POINT('',(123.033626104583,5.35,50.4290417845261));
#199539=CARTESIAN_POINT('Origin',(122.542812602034,5.35,50.3336368280768));
#199540=CARTESIAN_POINT('',(122.485569628164,5.35,50.6281249296065));
#199541=CARTESIAN_POINT('',(122.542812602034,5.35,50.3336368280768));
#199542=CARTESIAN_POINT('Origin',(121.757510997955,5.85,50.180988897758));
#199543=CARTESIAN_POINT('',(122.248324500504,5.85,50.2763938542073));
#199544=CARTESIAN_POINT('',(122.191081526635,5.85,50.570881955737));
#199545=CARTESIAN_POINT('',(122.248324500504,5.85,50.2763938542073));
#199546=CARTESIAN_POINT('',(121.700268024085,5.85,50.4754769992877));
#199547=CARTESIAN_POINT('',(121.700268024085,5.85,50.4754769992877));
#199548=CARTESIAN_POINT('',(121.757510997955,5.85,50.180988897758));
#199549=CARTESIAN_POINT('',(121.757510997955,5.85,50.180988897758));
#199550=CARTESIAN_POINT('',(121.757510997955,5.85,50.180988897758));
#199551=CARTESIAN_POINT('Origin',(122.248324500504,5.85,50.2763938542073));
#199552=CARTESIAN_POINT('',(122.248324500504,5.35,50.2763938542073));
#199553=CARTESIAN_POINT('',(122.191081526635,5.35,50.570881955737));
#199554=CARTESIAN_POINT('',(122.248324500504,5.35,50.2763938542073));
#199555=CARTESIAN_POINT('',(122.191081526635,5.85,50.570881955737));
#199556=CARTESIAN_POINT('',(122.248324500504,5.85,50.2763938542073));
#199557=CARTESIAN_POINT('Origin',(122.248324500504,5.35,50.2763938542073));
#199558=CARTESIAN_POINT('',(121.757510997955,5.35,50.180988897758));
#199559=CARTESIAN_POINT('',(121.700268024085,5.35,50.4754769992877));
#199560=CARTESIAN_POINT('',(121.757510997955,5.35,50.180988897758));
#199561=CARTESIAN_POINT('',(122.191081526635,5.35,50.570881955737));
#199562=CARTESIAN_POINT('',(122.248324500504,5.35,50.2763938542073));
#199563=CARTESIAN_POINT('Origin',(121.757510997955,5.35,50.180988897758));
#199564=CARTESIAN_POINT('',(121.700268024085,5.35,50.4754769992877));
#199565=CARTESIAN_POINT('',(121.757510997955,5.35,50.180988897758));
#199566=CARTESIAN_POINT('Origin',(120.972209393875,5.85,50.0283409674392));
#199567=CARTESIAN_POINT('',(121.463022896425,5.85,50.1237459238885));
#199568=CARTESIAN_POINT('',(121.405779922555,5.85,50.4182340254182));
#199569=CARTESIAN_POINT('',(121.463022896425,5.85,50.1237459238885));
#199570=CARTESIAN_POINT('',(120.914966420006,5.85,50.3228290689689));
#199571=CARTESIAN_POINT('',(120.914966420006,5.85,50.3228290689689));
#199572=CARTESIAN_POINT('',(120.972209393875,5.85,50.0283409674392));
#199573=CARTESIAN_POINT('',(120.972209393875,5.85,50.0283409674392));
#199574=CARTESIAN_POINT('',(120.972209393875,5.85,50.0283409674392));
#199575=CARTESIAN_POINT('Origin',(121.463022896425,5.85,50.1237459238885));
#199576=CARTESIAN_POINT('',(121.463022896425,5.35,50.1237459238885));
#199577=CARTESIAN_POINT('',(121.405779922555,5.35,50.4182340254182));
#199578=CARTESIAN_POINT('',(121.463022896425,5.35,50.1237459238885));
#199579=CARTESIAN_POINT('',(121.405779922555,5.85,50.4182340254182));
#199580=CARTESIAN_POINT('',(121.463022896425,5.85,50.1237459238885));
#199581=CARTESIAN_POINT('Origin',(121.463022896425,5.35,50.1237459238885));
#199582=CARTESIAN_POINT('',(120.972209393875,5.35,50.0283409674392));
#199583=CARTESIAN_POINT('',(120.914966420006,5.35,50.3228290689689));
#199584=CARTESIAN_POINT('',(120.972209393875,5.35,50.0283409674392));
#199585=CARTESIAN_POINT('',(121.405779922555,5.35,50.4182340254182));
#199586=CARTESIAN_POINT('',(121.463022896425,5.35,50.1237459238885));
#199587=CARTESIAN_POINT('Origin',(120.972209393875,5.35,50.0283409674392));
#199588=CARTESIAN_POINT('',(120.914966420006,5.35,50.3228290689689));
#199589=CARTESIAN_POINT('',(120.972209393875,5.35,50.0283409674392));
#199590=CARTESIAN_POINT('Origin',(120.186907789796,5.85,49.8756930371204));
#199591=CARTESIAN_POINT('',(120.677721292346,5.85,49.9710979935697));
#199592=CARTESIAN_POINT('',(120.620478318476,5.85,50.2655860950994));
#199593=CARTESIAN_POINT('',(120.677721292346,5.85,49.9710979935697));
#199594=CARTESIAN_POINT('',(120.129664815927,5.85,50.1701811386501));
#199595=CARTESIAN_POINT('',(120.129664815927,5.85,50.1701811386501));
#199596=CARTESIAN_POINT('',(120.186907789796,5.85,49.8756930371204));
#199597=CARTESIAN_POINT('',(120.186907789796,5.85,49.8756930371204));
#199598=CARTESIAN_POINT('',(120.186907789796,5.85,49.8756930371204));
#199599=CARTESIAN_POINT('Origin',(120.677721292346,5.85,49.9710979935697));
#199600=CARTESIAN_POINT('',(120.677721292346,5.35,49.9710979935697));
#199601=CARTESIAN_POINT('',(120.620478318476,5.35,50.2655860950994));
#199602=CARTESIAN_POINT('',(120.677721292346,5.35,49.9710979935697));
#199603=CARTESIAN_POINT('',(120.620478318476,5.85,50.2655860950994));
#199604=CARTESIAN_POINT('',(120.677721292346,5.85,49.9710979935697));
#199605=CARTESIAN_POINT('Origin',(120.677721292346,5.35,49.9710979935697));
#199606=CARTESIAN_POINT('',(120.186907789796,5.35,49.8756930371204));
#199607=CARTESIAN_POINT('',(120.129664815927,5.35,50.1701811386501));
#199608=CARTESIAN_POINT('',(120.186907789796,5.35,49.8756930371204));
#199609=CARTESIAN_POINT('',(120.620478318476,5.35,50.2655860950994));
#199610=CARTESIAN_POINT('',(120.677721292346,5.35,49.9710979935697));
#199611=CARTESIAN_POINT('Origin',(120.186907789796,5.35,49.8756930371204));
#199612=CARTESIAN_POINT('',(120.129664815927,5.35,50.1701811386501));
#199613=CARTESIAN_POINT('',(120.186907789796,5.35,49.8756930371204));
#199614=CARTESIAN_POINT('Origin',(119.401606185717,5.85,49.7230451068016));
#199615=CARTESIAN_POINT('',(119.892419688267,5.85,49.8184500632509));
#199616=CARTESIAN_POINT('',(119.835176714397,5.85,50.1129381647806));
#199617=CARTESIAN_POINT('',(119.892419688267,5.85,49.8184500632509));
#199618=CARTESIAN_POINT('',(119.344363211847,5.85,50.0175332083313));
#199619=CARTESIAN_POINT('',(119.344363211847,5.85,50.0175332083313));
#199620=CARTESIAN_POINT('',(119.401606185717,5.85,49.7230451068016));
#199621=CARTESIAN_POINT('',(119.401606185717,5.85,49.7230451068016));
#199622=CARTESIAN_POINT('',(119.401606185717,5.85,49.7230451068016));
#199623=CARTESIAN_POINT('Origin',(119.892419688267,5.85,49.8184500632509));
#199624=CARTESIAN_POINT('',(119.892419688267,5.35,49.8184500632509));
#199625=CARTESIAN_POINT('',(119.835176714397,5.35,50.1129381647806));
#199626=CARTESIAN_POINT('',(119.892419688267,5.35,49.8184500632509));
#199627=CARTESIAN_POINT('',(119.835176714397,5.85,50.1129381647806));
#199628=CARTESIAN_POINT('',(119.892419688267,5.85,49.8184500632509));
#199629=CARTESIAN_POINT('Origin',(119.892419688267,5.35,49.8184500632509));
#199630=CARTESIAN_POINT('',(119.401606185717,5.35,49.7230451068016));
#199631=CARTESIAN_POINT('',(119.344363211847,5.35,50.0175332083313));
#199632=CARTESIAN_POINT('',(119.401606185717,5.35,49.7230451068016));
#199633=CARTESIAN_POINT('',(119.835176714397,5.35,50.1129381647806));
#199634=CARTESIAN_POINT('',(119.892419688267,5.35,49.8184500632509));
#199635=CARTESIAN_POINT('Origin',(119.401606185717,5.35,49.7230451068016));
#199636=CARTESIAN_POINT('',(119.344363211847,5.35,50.0175332083313));
#199637=CARTESIAN_POINT('',(119.401606185717,5.35,49.7230451068016));
#199638=CARTESIAN_POINT('Origin',(118.616304581638,5.85,49.5703971764828));
#199639=CARTESIAN_POINT('',(119.107118084187,5.85,49.6658021329321));
#199640=CARTESIAN_POINT('',(119.049875110318,5.85,49.9602902344618));
#199641=CARTESIAN_POINT('',(119.107118084187,5.85,49.6658021329321));
#199642=CARTESIAN_POINT('',(118.559061607768,5.85,49.8648852780125));
#199643=CARTESIAN_POINT('',(118.559061607768,5.85,49.8648852780125));
#199644=CARTESIAN_POINT('',(118.616304581638,5.85,49.5703971764828));
#199645=CARTESIAN_POINT('',(118.616304581638,5.85,49.5703971764828));
#199646=CARTESIAN_POINT('',(118.616304581638,5.85,49.5703971764828));
#199647=CARTESIAN_POINT('Origin',(119.107118084187,5.85,49.6658021329321));
#199648=CARTESIAN_POINT('',(119.107118084187,5.35,49.6658021329321));
#199649=CARTESIAN_POINT('',(119.049875110318,5.35,49.9602902344618));
#199650=CARTESIAN_POINT('',(119.107118084187,5.35,49.6658021329321));
#199651=CARTESIAN_POINT('',(119.049875110318,5.85,49.9602902344618));
#199652=CARTESIAN_POINT('',(119.107118084187,5.85,49.6658021329321));
#199653=CARTESIAN_POINT('Origin',(119.107118084187,5.35,49.6658021329321));
#199654=CARTESIAN_POINT('',(118.616304581638,5.35,49.5703971764828));
#199655=CARTESIAN_POINT('',(118.559061607768,5.35,49.8648852780125));
#199656=CARTESIAN_POINT('',(118.616304581638,5.35,49.5703971764828));
#199657=CARTESIAN_POINT('',(119.049875110318,5.35,49.9602902344618));
#199658=CARTESIAN_POINT('',(119.107118084187,5.35,49.6658021329321));
#199659=CARTESIAN_POINT('Origin',(118.616304581638,5.35,49.5703971764828));
#199660=CARTESIAN_POINT('',(118.559061607768,5.35,49.8648852780125));
#199661=CARTESIAN_POINT('',(118.616304581638,5.35,49.5703971764828));
#199662=CARTESIAN_POINT('Origin',(117.831002977559,5.85,49.417749246164));
#199663=CARTESIAN_POINT('',(118.321816480108,5.85,49.5131542026133));
#199664=CARTESIAN_POINT('',(118.264573506239,5.85,49.807642304143));
#199665=CARTESIAN_POINT('',(118.321816480108,5.85,49.5131542026133));
#199666=CARTESIAN_POINT('',(117.773760003689,5.85,49.7122373476937));
#199667=CARTESIAN_POINT('',(117.773760003689,5.85,49.7122373476937));
#199668=CARTESIAN_POINT('',(117.831002977559,5.85,49.417749246164));
#199669=CARTESIAN_POINT('',(117.831002977559,5.85,49.417749246164));
#199670=CARTESIAN_POINT('',(117.831002977559,5.85,49.417749246164));
#199671=CARTESIAN_POINT('Origin',(118.321816480108,5.85,49.5131542026133));
#199672=CARTESIAN_POINT('',(118.321816480108,5.35,49.5131542026133));
#199673=CARTESIAN_POINT('',(118.264573506239,5.35,49.807642304143));
#199674=CARTESIAN_POINT('',(118.321816480108,5.35,49.5131542026133));
#199675=CARTESIAN_POINT('',(118.264573506239,5.85,49.807642304143));
#199676=CARTESIAN_POINT('',(118.321816480108,5.85,49.5131542026133));
#199677=CARTESIAN_POINT('Origin',(118.321816480108,5.35,49.5131542026133));
#199678=CARTESIAN_POINT('',(117.831002977559,5.35,49.417749246164));
#199679=CARTESIAN_POINT('',(117.773760003689,5.35,49.7122373476937));
#199680=CARTESIAN_POINT('',(117.831002977559,5.35,49.417749246164));
#199681=CARTESIAN_POINT('',(118.264573506239,5.35,49.807642304143));
#199682=CARTESIAN_POINT('',(118.321816480108,5.35,49.5131542026133));
#199683=CARTESIAN_POINT('Origin',(117.831002977559,5.35,49.417749246164));
#199684=CARTESIAN_POINT('',(117.773760003689,5.35,49.7122373476937));
#199685=CARTESIAN_POINT('',(117.831002977559,5.35,49.417749246164));
#199686=CARTESIAN_POINT('Origin',(117.045701373479,5.85,49.2651013158452));
#199687=CARTESIAN_POINT('',(117.536514876029,5.85,49.3605062722945));
#199688=CARTESIAN_POINT('',(117.479271902159,5.85,49.6549943738242));
#199689=CARTESIAN_POINT('',(117.536514876029,5.85,49.3605062722945));
#199690=CARTESIAN_POINT('',(116.98845839961,5.85,49.5595894173749));
#199691=CARTESIAN_POINT('',(116.98845839961,5.85,49.5595894173749));
#199692=CARTESIAN_POINT('',(117.045701373479,5.85,49.2651013158452));
#199693=CARTESIAN_POINT('',(117.045701373479,5.85,49.2651013158452));
#199694=CARTESIAN_POINT('',(117.045701373479,5.85,49.2651013158452));
#199695=CARTESIAN_POINT('Origin',(117.536514876029,5.85,49.3605062722945));
#199696=CARTESIAN_POINT('',(117.536514876029,5.35,49.3605062722945));
#199697=CARTESIAN_POINT('',(117.479271902159,5.35,49.6549943738242));
#199698=CARTESIAN_POINT('',(117.536514876029,5.35,49.3605062722945));
#199699=CARTESIAN_POINT('',(117.479271902159,5.85,49.6549943738242));
#199700=CARTESIAN_POINT('',(117.536514876029,5.85,49.3605062722945));
#199701=CARTESIAN_POINT('Origin',(117.536514876029,5.35,49.3605062722945));
#199702=CARTESIAN_POINT('',(117.045701373479,5.35,49.2651013158452));
#199703=CARTESIAN_POINT('',(116.98845839961,5.35,49.5595894173749));
#199704=CARTESIAN_POINT('',(117.045701373479,5.35,49.2651013158452));
#199705=CARTESIAN_POINT('',(117.479271902159,5.35,49.6549943738242));
#199706=CARTESIAN_POINT('',(117.536514876029,5.35,49.3605062722945));
#199707=CARTESIAN_POINT('Origin',(117.045701373479,5.35,49.2651013158452));
#199708=CARTESIAN_POINT('',(116.98845839961,5.35,49.5595894173749));
#199709=CARTESIAN_POINT('',(117.045701373479,5.35,49.2651013158452));
#199710=CARTESIAN_POINT('Origin',(116.2603997694,5.85,49.1124533855264));
#199711=CARTESIAN_POINT('',(116.75121327195,5.85,49.2078583419757));
#199712=CARTESIAN_POINT('',(116.69397029808,5.85,49.5023464435054));
#199713=CARTESIAN_POINT('',(116.75121327195,5.85,49.2078583419757));
#199714=CARTESIAN_POINT('',(116.203156795531,5.85,49.4069414870561));
#199715=CARTESIAN_POINT('',(116.203156795531,5.85,49.4069414870561));
#199716=CARTESIAN_POINT('',(116.2603997694,5.85,49.1124533855264));
#199717=CARTESIAN_POINT('',(116.2603997694,5.85,49.1124533855264));
#199718=CARTESIAN_POINT('',(116.2603997694,5.85,49.1124533855264));
#199719=CARTESIAN_POINT('Origin',(116.75121327195,5.85,49.2078583419757));
#199720=CARTESIAN_POINT('',(116.75121327195,5.35,49.2078583419757));
#199721=CARTESIAN_POINT('',(116.69397029808,5.35,49.5023464435054));
#199722=CARTESIAN_POINT('',(116.75121327195,5.35,49.2078583419757));
#199723=CARTESIAN_POINT('',(116.69397029808,5.85,49.5023464435054));
#199724=CARTESIAN_POINT('',(116.75121327195,5.85,49.2078583419757));
#199725=CARTESIAN_POINT('Origin',(116.75121327195,5.35,49.2078583419757));
#199726=CARTESIAN_POINT('',(116.2603997694,5.35,49.1124533855264));
#199727=CARTESIAN_POINT('',(116.203156795531,5.35,49.4069414870561));
#199728=CARTESIAN_POINT('',(116.2603997694,5.35,49.1124533855264));
#199729=CARTESIAN_POINT('',(116.69397029808,5.35,49.5023464435054));
#199730=CARTESIAN_POINT('',(116.75121327195,5.35,49.2078583419757));
#199731=CARTESIAN_POINT('Origin',(116.2603997694,5.35,49.1124533855264));
#199732=CARTESIAN_POINT('',(116.203156795531,5.35,49.4069414870561));
#199733=CARTESIAN_POINT('',(116.2603997694,5.35,49.1124533855264));
#199734=CARTESIAN_POINT('Origin',(115.475098165321,5.85,48.9598054552076));
#199735=CARTESIAN_POINT('',(115.96591166787,5.85,49.0552104116569));
#199736=CARTESIAN_POINT('',(115.908668694001,5.85,49.3496985131866));
#199737=CARTESIAN_POINT('',(115.96591166787,5.85,49.0552104116569));
#199738=CARTESIAN_POINT('',(115.417855191451,5.85,49.2542935567373));
#199739=CARTESIAN_POINT('',(115.417855191451,5.85,49.2542935567373));
#199740=CARTESIAN_POINT('',(115.475098165321,5.85,48.9598054552076));
#199741=CARTESIAN_POINT('',(115.475098165321,5.85,48.9598054552076));
#199742=CARTESIAN_POINT('',(115.475098165321,5.85,48.9598054552076));
#199743=CARTESIAN_POINT('Origin',(115.96591166787,5.85,49.0552104116569));
#199744=CARTESIAN_POINT('',(115.96591166787,5.35,49.0552104116569));
#199745=CARTESIAN_POINT('',(115.908668694001,5.35,49.3496985131866));
#199746=CARTESIAN_POINT('',(115.96591166787,5.35,49.0552104116569));
#199747=CARTESIAN_POINT('',(115.908668694001,5.85,49.3496985131866));
#199748=CARTESIAN_POINT('',(115.96591166787,5.85,49.0552104116569));
#199749=CARTESIAN_POINT('Origin',(115.96591166787,5.35,49.0552104116569));
#199750=CARTESIAN_POINT('',(115.475098165321,5.35,48.9598054552076));
#199751=CARTESIAN_POINT('',(115.417855191451,5.35,49.2542935567373));
#199752=CARTESIAN_POINT('',(115.475098165321,5.35,48.9598054552076));
#199753=CARTESIAN_POINT('',(115.908668694001,5.35,49.3496985131866));
#199754=CARTESIAN_POINT('',(115.96591166787,5.35,49.0552104116569));
#199755=CARTESIAN_POINT('Origin',(115.475098165321,5.35,48.9598054552076));
#199756=CARTESIAN_POINT('',(115.417855191451,5.35,49.2542935567373));
#199757=CARTESIAN_POINT('',(115.475098165321,5.35,48.9598054552076));
#199758=CARTESIAN_POINT('Origin',(114.689796561242,5.85,48.8071575248888));
#199759=CARTESIAN_POINT('',(115.180610063791,5.85,48.9025624813381));
#199760=CARTESIAN_POINT('',(115.123367089922,5.85,49.1970505828678));
#199761=CARTESIAN_POINT('',(115.180610063791,5.85,48.9025624813381));
#199762=CARTESIAN_POINT('',(114.632553587372,5.85,49.1016456264185));
#199763=CARTESIAN_POINT('',(114.632553587372,5.85,49.1016456264185));
#199764=CARTESIAN_POINT('',(114.689796561242,5.85,48.8071575248888));
#199765=CARTESIAN_POINT('',(114.689796561242,5.85,48.8071575248888));
#199766=CARTESIAN_POINT('',(114.689796561242,5.85,48.8071575248888));
#199767=CARTESIAN_POINT('Origin',(115.180610063791,5.85,48.9025624813381));
#199768=CARTESIAN_POINT('',(115.180610063791,5.35,48.9025624813381));
#199769=CARTESIAN_POINT('',(115.123367089922,5.35,49.1970505828678));
#199770=CARTESIAN_POINT('',(115.180610063791,5.35,48.9025624813381));
#199771=CARTESIAN_POINT('',(115.123367089922,5.85,49.1970505828678));
#199772=CARTESIAN_POINT('',(115.180610063791,5.85,48.9025624813381));
#199773=CARTESIAN_POINT('Origin',(115.180610063791,5.35,48.9025624813381));
#199774=CARTESIAN_POINT('',(114.689796561242,5.35,48.8071575248888));
#199775=CARTESIAN_POINT('',(114.632553587372,5.35,49.1016456264185));
#199776=CARTESIAN_POINT('',(114.689796561242,5.35,48.8071575248888));
#199777=CARTESIAN_POINT('',(115.123367089922,5.35,49.1970505828678));
#199778=CARTESIAN_POINT('',(115.180610063791,5.35,48.9025624813381));
#199779=CARTESIAN_POINT('Origin',(114.689796561242,5.35,48.8071575248888));
#199780=CARTESIAN_POINT('',(114.632553587372,5.35,49.1016456264185));
#199781=CARTESIAN_POINT('',(114.689796561242,5.35,48.8071575248888));
#199782=CARTESIAN_POINT('Origin',(113.904494957163,5.85,48.65450959457));
#199783=CARTESIAN_POINT('',(114.395308459712,5.85,48.7499145510193));
#199784=CARTESIAN_POINT('',(114.338065485842,5.85,49.044402652549));
#199785=CARTESIAN_POINT('',(114.395308459712,5.85,48.7499145510193));
#199786=CARTESIAN_POINT('',(113.847251983293,5.85,48.9489976960997));
#199787=CARTESIAN_POINT('',(113.847251983293,5.85,48.9489976960997));
#199788=CARTESIAN_POINT('',(113.904494957163,5.85,48.65450959457));
#199789=CARTESIAN_POINT('',(113.904494957163,5.85,48.65450959457));
#199790=CARTESIAN_POINT('',(113.904494957163,5.85,48.65450959457));
#199791=CARTESIAN_POINT('Origin',(114.395308459712,5.85,48.7499145510193));
#199792=CARTESIAN_POINT('',(114.395308459712,5.35,48.7499145510193));
#199793=CARTESIAN_POINT('',(114.338065485842,5.35,49.044402652549));
#199794=CARTESIAN_POINT('',(114.395308459712,5.35,48.7499145510193));
#199795=CARTESIAN_POINT('',(114.338065485842,5.85,49.044402652549));
#199796=CARTESIAN_POINT('',(114.395308459712,5.85,48.7499145510193));
#199797=CARTESIAN_POINT('Origin',(114.395308459712,5.35,48.7499145510193));
#199798=CARTESIAN_POINT('',(113.904494957163,5.35,48.65450959457));
#199799=CARTESIAN_POINT('',(113.847251983293,5.35,48.9489976960997));
#199800=CARTESIAN_POINT('',(113.904494957163,5.35,48.65450959457));
#199801=CARTESIAN_POINT('',(114.338065485842,5.35,49.044402652549));
#199802=CARTESIAN_POINT('',(114.395308459712,5.35,48.7499145510193));
#199803=CARTESIAN_POINT('Origin',(113.904494957163,5.35,48.65450959457));
#199804=CARTESIAN_POINT('',(113.847251983293,5.35,48.9489976960997));
#199805=CARTESIAN_POINT('',(113.904494957163,5.35,48.65450959457));
#199806=CARTESIAN_POINT('Origin',(113.119193353083,5.85,48.5018616642512));
#199807=CARTESIAN_POINT('',(113.610006855633,5.85,48.5972666207005));
#199808=CARTESIAN_POINT('',(113.552763881763,5.85,48.8917547222302));
#199809=CARTESIAN_POINT('',(113.610006855633,5.85,48.5972666207005));
#199810=CARTESIAN_POINT('',(113.061950379214,5.85,48.7963497657809));
#199811=CARTESIAN_POINT('',(113.061950379214,5.85,48.7963497657809));
#199812=CARTESIAN_POINT('',(113.119193353083,5.85,48.5018616642512));
#199813=CARTESIAN_POINT('',(113.119193353083,5.85,48.5018616642512));
#199814=CARTESIAN_POINT('',(113.119193353083,5.85,48.5018616642512));
#199815=CARTESIAN_POINT('Origin',(113.610006855633,5.85,48.5972666207005));
#199816=CARTESIAN_POINT('',(113.610006855633,5.35,48.5972666207005));
#199817=CARTESIAN_POINT('',(113.552763881763,5.35,48.8917547222302));
#199818=CARTESIAN_POINT('',(113.610006855633,5.35,48.5972666207005));
#199819=CARTESIAN_POINT('',(113.552763881763,5.85,48.8917547222302));
#199820=CARTESIAN_POINT('',(113.610006855633,5.85,48.5972666207005));
#199821=CARTESIAN_POINT('Origin',(113.610006855633,5.35,48.5972666207005));
#199822=CARTESIAN_POINT('',(113.119193353083,5.35,48.5018616642512));
#199823=CARTESIAN_POINT('',(113.061950379214,5.35,48.7963497657809));
#199824=CARTESIAN_POINT('',(113.119193353083,5.35,48.5018616642512));
#199825=CARTESIAN_POINT('',(113.552763881763,5.35,48.8917547222302));
#199826=CARTESIAN_POINT('',(113.610006855633,5.35,48.5972666207005));
#199827=CARTESIAN_POINT('Origin',(113.119193353083,5.35,48.5018616642512));
#199828=CARTESIAN_POINT('',(113.061950379214,5.35,48.7963497657809));
#199829=CARTESIAN_POINT('',(113.119193353083,5.35,48.5018616642512));
#199830=CARTESIAN_POINT('Origin',(112.333891749004,5.85,48.3492137339324));
#199831=CARTESIAN_POINT('',(112.824705251554,5.85,48.4446186903817));
#199832=CARTESIAN_POINT('',(112.767462277684,5.85,48.7391067919114));
#199833=CARTESIAN_POINT('',(112.824705251554,5.85,48.4446186903817));
#199834=CARTESIAN_POINT('',(112.276648775135,5.85,48.6437018354621));
#199835=CARTESIAN_POINT('',(112.276648775135,5.85,48.6437018354621));
#199836=CARTESIAN_POINT('',(112.333891749004,5.85,48.3492137339324));
#199837=CARTESIAN_POINT('',(112.333891749004,5.85,48.3492137339324));
#199838=CARTESIAN_POINT('',(112.333891749004,5.85,48.3492137339324));
#199839=CARTESIAN_POINT('Origin',(112.824705251554,5.85,48.4446186903817));
#199840=CARTESIAN_POINT('',(112.824705251554,5.35,48.4446186903817));
#199841=CARTESIAN_POINT('',(112.767462277684,5.35,48.7391067919114));
#199842=CARTESIAN_POINT('',(112.824705251554,5.35,48.4446186903817));
#199843=CARTESIAN_POINT('',(112.767462277684,5.85,48.7391067919114));
#199844=CARTESIAN_POINT('',(112.824705251554,5.85,48.4446186903817));
#199845=CARTESIAN_POINT('Origin',(112.824705251554,5.35,48.4446186903817));
#199846=CARTESIAN_POINT('',(112.333891749004,5.35,48.3492137339324));
#199847=CARTESIAN_POINT('',(112.276648775135,5.35,48.6437018354621));
#199848=CARTESIAN_POINT('',(112.333891749004,5.35,48.3492137339324));
#199849=CARTESIAN_POINT('',(112.767462277684,5.35,48.7391067919114));
#199850=CARTESIAN_POINT('',(112.824705251554,5.35,48.4446186903817));
#199851=CARTESIAN_POINT('Origin',(112.333891749004,5.35,48.3492137339324));
#199852=CARTESIAN_POINT('',(112.276648775135,5.35,48.6437018354621));
#199853=CARTESIAN_POINT('',(112.333891749004,5.35,48.3492137339324));
#199854=CARTESIAN_POINT('Origin',(112.333891749004,5.05,48.3492137339324));
#199855=CARTESIAN_POINT('',(112.824705251554,5.05,48.4446186903817));
#199856=CARTESIAN_POINT('',(112.767462277684,5.05,48.7391067919114));
#199857=CARTESIAN_POINT('',(112.824705251554,5.05,48.4446186903817));
#199858=CARTESIAN_POINT('',(112.276648775135,5.05,48.6437018354621));
#199859=CARTESIAN_POINT('',(112.276648775135,5.05,48.6437018354621));
#199860=CARTESIAN_POINT('',(112.333891749004,5.05,48.3492137339324));
#199861=CARTESIAN_POINT('',(112.333891749004,5.05,48.3492137339324));
#199862=CARTESIAN_POINT('',(112.333891749004,5.05,48.3492137339324));
#199863=CARTESIAN_POINT('Origin',(112.824705251554,5.05,48.4446186903817));
#199864=CARTESIAN_POINT('',(112.824705251554,4.55,48.4446186903817));
#199865=CARTESIAN_POINT('',(112.767462277684,4.55,48.7391067919114));
#199866=CARTESIAN_POINT('',(112.824705251554,4.55,48.4446186903817));
#199867=CARTESIAN_POINT('',(112.767462277684,5.05,48.7391067919114));
#199868=CARTESIAN_POINT('',(112.824705251554,5.05,48.4446186903817));
#199869=CARTESIAN_POINT('Origin',(112.824705251554,4.55,48.4446186903817));
#199870=CARTESIAN_POINT('',(112.333891749004,4.55,48.3492137339324));
#199871=CARTESIAN_POINT('',(112.276648775135,4.55,48.6437018354621));
#199872=CARTESIAN_POINT('',(112.333891749004,4.55,48.3492137339324));
#199873=CARTESIAN_POINT('',(112.767462277684,4.55,48.7391067919114));
#199874=CARTESIAN_POINT('',(112.824705251554,4.55,48.4446186903817));
#199875=CARTESIAN_POINT('Origin',(112.333891749004,4.55,48.3492137339324));
#199876=CARTESIAN_POINT('',(112.276648775135,4.55,48.6437018354621));
#199877=CARTESIAN_POINT('',(112.333891749004,4.55,48.3492137339324));
#199878=CARTESIAN_POINT('Origin',(112.333891749004,4.25,48.3492137339324));
#199879=CARTESIAN_POINT('',(112.824705251554,4.25,48.4446186903817));
#199880=CARTESIAN_POINT('',(112.767462277684,4.25,48.7391067919114));
#199881=CARTESIAN_POINT('',(112.824705251554,4.25,48.4446186903817));
#199882=CARTESIAN_POINT('',(112.276648775135,4.25,48.6437018354621));
#199883=CARTESIAN_POINT('',(112.276648775135,4.25,48.6437018354621));
#199884=CARTESIAN_POINT('',(112.333891749004,4.25,48.3492137339324));
#199885=CARTESIAN_POINT('',(112.333891749004,4.25,48.3492137339324));
#199886=CARTESIAN_POINT('',(112.333891749004,4.25,48.3492137339324));
#199887=CARTESIAN_POINT('Origin',(112.824705251554,4.25,48.4446186903817));
#199888=CARTESIAN_POINT('',(112.824705251554,3.75,48.4446186903817));
#199889=CARTESIAN_POINT('',(112.767462277684,3.75,48.7391067919114));
#199890=CARTESIAN_POINT('',(112.824705251554,3.75,48.4446186903817));
#199891=CARTESIAN_POINT('',(112.767462277684,4.25,48.7391067919114));
#199892=CARTESIAN_POINT('',(112.824705251554,4.25,48.4446186903817));
#199893=CARTESIAN_POINT('Origin',(112.824705251554,3.75,48.4446186903817));
#199894=CARTESIAN_POINT('',(112.333891749004,3.75,48.3492137339324));
#199895=CARTESIAN_POINT('',(112.276648775135,3.75,48.6437018354621));
#199896=CARTESIAN_POINT('',(112.333891749004,3.75,48.3492137339324));
#199897=CARTESIAN_POINT('',(112.767462277684,3.75,48.7391067919114));
#199898=CARTESIAN_POINT('',(112.824705251554,3.75,48.4446186903817));
#199899=CARTESIAN_POINT('Origin',(112.333891749004,3.75,48.3492137339324));
#199900=CARTESIAN_POINT('',(112.276648775135,3.75,48.6437018354621));
#199901=CARTESIAN_POINT('',(112.333891749004,3.75,48.3492137339324));
#199902=CARTESIAN_POINT('Origin',(112.333891749004,3.45,48.3492137339324));
#199903=CARTESIAN_POINT('',(112.824705251554,3.45,48.4446186903817));
#199904=CARTESIAN_POINT('',(112.767462277684,3.45,48.7391067919114));
#199905=CARTESIAN_POINT('',(112.824705251554,3.45,48.4446186903817));
#199906=CARTESIAN_POINT('',(112.276648775135,3.45,48.6437018354621));
#199907=CARTESIAN_POINT('',(112.276648775135,3.45,48.6437018354621));
#199908=CARTESIAN_POINT('',(112.333891749004,3.45,48.3492137339324));
#199909=CARTESIAN_POINT('',(112.333891749004,3.45,48.3492137339324));
#199910=CARTESIAN_POINT('',(112.333891749004,3.45,48.3492137339324));
#199911=CARTESIAN_POINT('Origin',(112.824705251554,3.45,48.4446186903817));
#199912=CARTESIAN_POINT('',(112.824705251554,2.95,48.4446186903817));
#199913=CARTESIAN_POINT('',(112.767462277684,2.95,48.7391067919114));
#199914=CARTESIAN_POINT('',(112.824705251554,2.95,48.4446186903817));
#199915=CARTESIAN_POINT('',(112.767462277684,3.45,48.7391067919114));
#199916=CARTESIAN_POINT('',(112.824705251554,3.45,48.4446186903817));
#199917=CARTESIAN_POINT('Origin',(112.824705251554,2.95,48.4446186903817));
#199918=CARTESIAN_POINT('',(112.333891749004,2.95,48.3492137339324));
#199919=CARTESIAN_POINT('',(112.276648775135,2.95,48.6437018354621));
#199920=CARTESIAN_POINT('',(112.333891749004,2.95,48.3492137339324));
#199921=CARTESIAN_POINT('',(112.767462277684,2.95,48.7391067919114));
#199922=CARTESIAN_POINT('',(112.824705251554,2.95,48.4446186903817));
#199923=CARTESIAN_POINT('Origin',(112.333891749004,2.95,48.3492137339324));
#199924=CARTESIAN_POINT('',(112.276648775135,2.95,48.6437018354621));
#199925=CARTESIAN_POINT('',(112.333891749004,2.95,48.3492137339324));
#199926=CARTESIAN_POINT('Origin',(112.333891749004,2.65,48.3492137339324));
#199927=CARTESIAN_POINT('',(112.824705251554,2.65,48.4446186903817));
#199928=CARTESIAN_POINT('',(112.767462277684,2.65,48.7391067919114));
#199929=CARTESIAN_POINT('',(112.824705251554,2.65,48.4446186903817));
#199930=CARTESIAN_POINT('',(112.276648775135,2.65,48.6437018354621));
#199931=CARTESIAN_POINT('',(112.276648775135,2.65,48.6437018354621));
#199932=CARTESIAN_POINT('',(112.333891749004,2.65,48.3492137339324));
#199933=CARTESIAN_POINT('',(112.333891749004,2.65,48.3492137339324));
#199934=CARTESIAN_POINT('',(112.333891749004,2.65,48.3492137339324));
#199935=CARTESIAN_POINT('Origin',(112.824705251554,2.65,48.4446186903817));
#199936=CARTESIAN_POINT('',(112.824705251554,2.15,48.4446186903817));
#199937=CARTESIAN_POINT('',(112.767462277684,2.15,48.7391067919114));
#199938=CARTESIAN_POINT('',(112.824705251554,2.15,48.4446186903817));
#199939=CARTESIAN_POINT('',(112.767462277684,2.65,48.7391067919114));
#199940=CARTESIAN_POINT('',(112.824705251554,2.65,48.4446186903817));
#199941=CARTESIAN_POINT('Origin',(112.824705251554,2.15,48.4446186903817));
#199942=CARTESIAN_POINT('',(112.333891749004,2.15,48.3492137339324));
#199943=CARTESIAN_POINT('',(112.276648775135,2.15,48.6437018354621));
#199944=CARTESIAN_POINT('',(112.333891749004,2.15,48.3492137339324));
#199945=CARTESIAN_POINT('',(112.767462277684,2.15,48.7391067919114));
#199946=CARTESIAN_POINT('',(112.824705251554,2.15,48.4446186903817));
#199947=CARTESIAN_POINT('Origin',(112.333891749004,2.15,48.3492137339324));
#199948=CARTESIAN_POINT('',(112.276648775135,2.15,48.6437018354621));
#199949=CARTESIAN_POINT('',(112.333891749004,2.15,48.3492137339324));
#199950=CARTESIAN_POINT('Origin',(112.333891749004,1.85,48.3492137339324));
#199951=CARTESIAN_POINT('',(112.824705251554,1.85,48.4446186903817));
#199952=CARTESIAN_POINT('',(112.767462277684,1.85,48.7391067919114));
#199953=CARTESIAN_POINT('',(112.824705251554,1.85,48.4446186903817));
#199954=CARTESIAN_POINT('',(112.276648775135,1.85,48.6437018354621));
#199955=CARTESIAN_POINT('',(112.276648775135,1.85,48.6437018354621));
#199956=CARTESIAN_POINT('',(112.333891749004,1.85,48.3492137339324));
#199957=CARTESIAN_POINT('',(112.333891749004,1.85,48.3492137339324));
#199958=CARTESIAN_POINT('',(112.333891749004,1.85,48.3492137339324));
#199959=CARTESIAN_POINT('Origin',(112.824705251554,1.85,48.4446186903817));
#199960=CARTESIAN_POINT('',(112.824705251554,1.35,48.4446186903817));
#199961=CARTESIAN_POINT('',(112.767462277684,1.35,48.7391067919114));
#199962=CARTESIAN_POINT('',(112.824705251554,1.35,48.4446186903817));
#199963=CARTESIAN_POINT('',(112.767462277684,1.85,48.7391067919114));
#199964=CARTESIAN_POINT('',(112.824705251554,1.85,48.4446186903817));
#199965=CARTESIAN_POINT('Origin',(112.824705251554,1.35,48.4446186903817));
#199966=CARTESIAN_POINT('',(112.333891749004,1.35,48.3492137339324));
#199967=CARTESIAN_POINT('',(112.276648775135,1.35,48.6437018354621));
#199968=CARTESIAN_POINT('',(112.333891749004,1.35,48.3492137339324));
#199969=CARTESIAN_POINT('',(112.767462277684,1.35,48.7391067919114));
#199970=CARTESIAN_POINT('',(112.824705251554,1.35,48.4446186903817));
#199971=CARTESIAN_POINT('Origin',(112.333891749004,1.35,48.3492137339324));
#199972=CARTESIAN_POINT('',(112.276648775135,1.35,48.6437018354621));
#199973=CARTESIAN_POINT('',(112.333891749004,1.35,48.3492137339324));
#199974=CARTESIAN_POINT('Origin',(112.333891749004,1.05,48.3492137339324));
#199975=CARTESIAN_POINT('',(112.824705251554,1.05,48.4446186903817));
#199976=CARTESIAN_POINT('',(112.767462277684,1.05,48.7391067919114));
#199977=CARTESIAN_POINT('',(112.824705251554,1.05,48.4446186903817));
#199978=CARTESIAN_POINT('',(112.276648775135,1.05,48.6437018354621));
#199979=CARTESIAN_POINT('',(112.276648775135,1.05,48.6437018354621));
#199980=CARTESIAN_POINT('',(112.333891749004,1.05,48.3492137339324));
#199981=CARTESIAN_POINT('',(112.333891749004,1.05,48.3492137339324));
#199982=CARTESIAN_POINT('',(112.333891749004,1.05,48.3492137339324));
#199983=CARTESIAN_POINT('Origin',(112.824705251554,1.05,48.4446186903817));
#199984=CARTESIAN_POINT('',(112.824705251554,0.550000000000015,48.4446186903817));
#199985=CARTESIAN_POINT('',(112.767462277684,0.550000000000015,48.7391067919114));
#199986=CARTESIAN_POINT('',(112.824705251554,0.550000000000015,48.4446186903817));
#199987=CARTESIAN_POINT('',(112.767462277684,1.05,48.7391067919114));
#199988=CARTESIAN_POINT('',(112.824705251554,1.05,48.4446186903817));
#199989=CARTESIAN_POINT('Origin',(112.824705251554,0.550000000000015,48.4446186903817));
#199990=CARTESIAN_POINT('',(112.333891749004,0.550000000000015,48.3492137339324));
#199991=CARTESIAN_POINT('',(112.276648775135,0.550000000000015,48.6437018354621));
#199992=CARTESIAN_POINT('',(112.333891749004,0.550000000000015,48.3492137339324));
#199993=CARTESIAN_POINT('',(112.767462277684,0.550000000000015,48.7391067919114));
#199994=CARTESIAN_POINT('',(112.824705251554,0.550000000000015,48.4446186903817));
#199995=CARTESIAN_POINT('Origin',(112.333891749004,0.550000000000015,48.3492137339324));
#199996=CARTESIAN_POINT('',(112.276648775135,0.550000000000015,48.6437018354621));
#199997=CARTESIAN_POINT('',(112.333891749004,0.550000000000015,48.3492137339324));
#199998=CARTESIAN_POINT('Origin',(112.333891749004,0.250000000000015,48.3492137339324));
#199999=CARTESIAN_POINT('',(112.824705251554,0.250000000000015,48.4446186903817));
#200000=CARTESIAN_POINT('',(112.767462277684,0.250000000000015,48.7391067919114));
#200001=CARTESIAN_POINT('',(112.824705251554,0.250000000000015,48.4446186903817));
#200002=CARTESIAN_POINT('',(112.276648775135,0.250000000000015,48.6437018354621));
#200003=CARTESIAN_POINT('',(112.276648775135,0.250000000000015,48.6437018354621));
#200004=CARTESIAN_POINT('',(112.333891749004,0.250000000000015,48.3492137339324));
#200005=CARTESIAN_POINT('',(112.333891749004,0.250000000000015,48.3492137339324));
#200006=CARTESIAN_POINT('',(112.333891749004,0.250000000000015,48.3492137339324));
#200007=CARTESIAN_POINT('Origin',(112.824705251554,0.250000000000015,48.4446186903817));
#200008=CARTESIAN_POINT('',(112.824705251554,-0.249999999999985,48.4446186903817));
#200009=CARTESIAN_POINT('',(112.767462277684,-0.249999999999985,48.7391067919114));
#200010=CARTESIAN_POINT('',(112.824705251554,-0.249999999999985,48.4446186903817));
#200011=CARTESIAN_POINT('',(112.767462277684,0.250000000000015,48.7391067919114));
#200012=CARTESIAN_POINT('',(112.824705251554,0.250000000000015,48.4446186903817));
#200013=CARTESIAN_POINT('Origin',(112.824705251554,-0.249999999999985,48.4446186903817));
#200014=CARTESIAN_POINT('',(112.333891749004,-0.249999999999985,48.3492137339324));
#200015=CARTESIAN_POINT('',(112.276648775135,-0.249999999999985,48.6437018354621));
#200016=CARTESIAN_POINT('',(112.333891749004,-0.249999999999985,48.3492137339324));
#200017=CARTESIAN_POINT('',(112.767462277684,-0.249999999999985,48.7391067919114));
#200018=CARTESIAN_POINT('',(112.824705251554,-0.249999999999985,48.4446186903817));
#200019=CARTESIAN_POINT('Origin',(112.333891749004,-0.249999999999985,48.3492137339324));
#200020=CARTESIAN_POINT('',(112.276648775135,-0.249999999999985,48.6437018354621));
#200021=CARTESIAN_POINT('',(112.333891749004,-0.249999999999985,48.3492137339324));
#200022=CARTESIAN_POINT('Origin',(112.333891749004,-0.549999999999986,48.3492137339324));
#200023=CARTESIAN_POINT('',(112.824705251554,-0.549999999999986,48.4446186903817));
#200024=CARTESIAN_POINT('',(112.767462277684,-0.549999999999986,48.7391067919114));
#200025=CARTESIAN_POINT('',(112.824705251554,-0.549999999999986,48.4446186903817));
#200026=CARTESIAN_POINT('',(112.276648775135,-0.549999999999986,48.6437018354621));
#200027=CARTESIAN_POINT('',(112.276648775135,-0.549999999999986,48.6437018354621));
#200028=CARTESIAN_POINT('',(112.333891749004,-0.549999999999986,48.3492137339324));
#200029=CARTESIAN_POINT('',(112.333891749004,-0.549999999999986,48.3492137339324));
#200030=CARTESIAN_POINT('',(112.333891749004,-0.549999999999986,48.3492137339324));
#200031=CARTESIAN_POINT('Origin',(112.824705251554,-0.549999999999986,48.4446186903817));
#200032=CARTESIAN_POINT('',(112.824705251554,-1.05,48.4446186903817));
#200033=CARTESIAN_POINT('',(112.767462277684,-1.05,48.7391067919114));
#200034=CARTESIAN_POINT('',(112.824705251554,-1.05,48.4446186903817));
#200035=CARTESIAN_POINT('',(112.767462277684,-0.549999999999986,48.7391067919114));
#200036=CARTESIAN_POINT('',(112.824705251554,-0.549999999999986,48.4446186903817));
#200037=CARTESIAN_POINT('Origin',(112.824705251554,-1.05,48.4446186903817));
#200038=CARTESIAN_POINT('',(112.333891749004,-1.05,48.3492137339324));
#200039=CARTESIAN_POINT('',(112.276648775135,-1.05,48.6437018354621));
#200040=CARTESIAN_POINT('',(112.333891749004,-1.05,48.3492137339324));
#200041=CARTESIAN_POINT('',(112.767462277684,-1.05,48.7391067919114));
#200042=CARTESIAN_POINT('',(112.824705251554,-1.05,48.4446186903817));
#200043=CARTESIAN_POINT('Origin',(112.333891749004,-1.05,48.3492137339324));
#200044=CARTESIAN_POINT('',(112.276648775135,-1.05,48.6437018354621));
#200045=CARTESIAN_POINT('',(112.333891749004,-1.05,48.3492137339324));
#200046=CARTESIAN_POINT('Origin',(112.333891749004,-1.35,48.3492137339324));
#200047=CARTESIAN_POINT('',(112.824705251554,-1.35,48.4446186903817));
#200048=CARTESIAN_POINT('',(112.767462277684,-1.35,48.7391067919114));
#200049=CARTESIAN_POINT('',(112.824705251554,-1.35,48.4446186903817));
#200050=CARTESIAN_POINT('',(112.276648775135,-1.35,48.6437018354621));
#200051=CARTESIAN_POINT('',(112.276648775135,-1.35,48.6437018354621));
#200052=CARTESIAN_POINT('',(112.333891749004,-1.35,48.3492137339324));
#200053=CARTESIAN_POINT('',(112.333891749004,-1.35,48.3492137339324));
#200054=CARTESIAN_POINT('',(112.333891749004,-1.35,48.3492137339324));
#200055=CARTESIAN_POINT('Origin',(112.824705251554,-1.35,48.4446186903817));
#200056=CARTESIAN_POINT('',(112.824705251554,-1.85,48.4446186903817));
#200057=CARTESIAN_POINT('',(112.767462277684,-1.85,48.7391067919114));
#200058=CARTESIAN_POINT('',(112.824705251554,-1.85,48.4446186903817));
#200059=CARTESIAN_POINT('',(112.767462277684,-1.35,48.7391067919114));
#200060=CARTESIAN_POINT('',(112.824705251554,-1.35,48.4446186903817));
#200061=CARTESIAN_POINT('Origin',(112.824705251554,-1.85,48.4446186903817));
#200062=CARTESIAN_POINT('',(112.333891749004,-1.85,48.3492137339324));
#200063=CARTESIAN_POINT('',(112.276648775135,-1.85,48.6437018354621));
#200064=CARTESIAN_POINT('',(112.333891749004,-1.85,48.3492137339324));
#200065=CARTESIAN_POINT('',(112.767462277684,-1.85,48.7391067919114));
#200066=CARTESIAN_POINT('',(112.824705251554,-1.85,48.4446186903817));
#200067=CARTESIAN_POINT('Origin',(112.333891749004,-1.85,48.3492137339324));
#200068=CARTESIAN_POINT('',(112.276648775135,-1.85,48.6437018354621));
#200069=CARTESIAN_POINT('',(112.333891749004,-1.85,48.3492137339324));
#200070=CARTESIAN_POINT('Origin',(112.333891749004,-2.15,48.3492137339324));
#200071=CARTESIAN_POINT('',(112.824705251554,-2.15,48.4446186903817));
#200072=CARTESIAN_POINT('',(112.767462277684,-2.15,48.7391067919114));
#200073=CARTESIAN_POINT('',(112.824705251554,-2.15,48.4446186903817));
#200074=CARTESIAN_POINT('',(112.276648775135,-2.15,48.6437018354621));
#200075=CARTESIAN_POINT('',(112.276648775135,-2.15,48.6437018354621));
#200076=CARTESIAN_POINT('',(112.333891749004,-2.15,48.3492137339324));
#200077=CARTESIAN_POINT('',(112.333891749004,-2.15,48.3492137339324));
#200078=CARTESIAN_POINT('',(112.333891749004,-2.15,48.3492137339324));
#200079=CARTESIAN_POINT('Origin',(112.824705251554,-2.15,48.4446186903817));
#200080=CARTESIAN_POINT('',(112.824705251554,-2.65,48.4446186903817));
#200081=CARTESIAN_POINT('',(112.767462277684,-2.65,48.7391067919114));
#200082=CARTESIAN_POINT('',(112.824705251554,-2.65,48.4446186903817));
#200083=CARTESIAN_POINT('',(112.767462277684,-2.15,48.7391067919114));
#200084=CARTESIAN_POINT('',(112.824705251554,-2.15,48.4446186903817));
#200085=CARTESIAN_POINT('Origin',(112.824705251554,-2.65,48.4446186903817));
#200086=CARTESIAN_POINT('',(112.333891749004,-2.65,48.3492137339324));
#200087=CARTESIAN_POINT('',(112.276648775135,-2.65,48.6437018354621));
#200088=CARTESIAN_POINT('',(112.333891749004,-2.65,48.3492137339324));
#200089=CARTESIAN_POINT('',(112.767462277684,-2.65,48.7391067919114));
#200090=CARTESIAN_POINT('',(112.824705251554,-2.65,48.4446186903817));
#200091=CARTESIAN_POINT('Origin',(112.333891749004,-2.65,48.3492137339324));
#200092=CARTESIAN_POINT('',(112.276648775135,-2.65,48.6437018354621));
#200093=CARTESIAN_POINT('',(112.333891749004,-2.65,48.3492137339324));
#200094=CARTESIAN_POINT('Origin',(112.333891749004,-2.95,48.3492137339324));
#200095=CARTESIAN_POINT('',(112.824705251554,-2.95,48.4446186903817));
#200096=CARTESIAN_POINT('',(112.767462277684,-2.95,48.7391067919114));
#200097=CARTESIAN_POINT('',(112.824705251554,-2.95,48.4446186903817));
#200098=CARTESIAN_POINT('',(112.276648775135,-2.95,48.6437018354621));
#200099=CARTESIAN_POINT('',(112.276648775135,-2.95,48.6437018354621));
#200100=CARTESIAN_POINT('',(112.333891749004,-2.95,48.3492137339324));
#200101=CARTESIAN_POINT('',(112.333891749004,-2.95,48.3492137339324));
#200102=CARTESIAN_POINT('',(112.333891749004,-2.95,48.3492137339324));
#200103=CARTESIAN_POINT('Origin',(112.824705251554,-2.95,48.4446186903817));
#200104=CARTESIAN_POINT('',(112.824705251554,-3.45,48.4446186903817));
#200105=CARTESIAN_POINT('',(112.767462277684,-3.45,48.7391067919114));
#200106=CARTESIAN_POINT('',(112.824705251554,-3.45,48.4446186903817));
#200107=CARTESIAN_POINT('',(112.767462277684,-2.95,48.7391067919114));
#200108=CARTESIAN_POINT('',(112.824705251554,-2.95,48.4446186903817));
#200109=CARTESIAN_POINT('Origin',(112.824705251554,-3.45,48.4446186903817));
#200110=CARTESIAN_POINT('',(112.333891749004,-3.45,48.3492137339324));
#200111=CARTESIAN_POINT('',(112.276648775135,-3.45,48.6437018354621));
#200112=CARTESIAN_POINT('',(112.333891749004,-3.45,48.3492137339324));
#200113=CARTESIAN_POINT('',(112.767462277684,-3.45,48.7391067919114));
#200114=CARTESIAN_POINT('',(112.824705251554,-3.45,48.4446186903817));
#200115=CARTESIAN_POINT('Origin',(112.333891749004,-3.45,48.3492137339324));
#200116=CARTESIAN_POINT('',(112.276648775135,-3.45,48.6437018354621));
#200117=CARTESIAN_POINT('',(112.333891749004,-3.45,48.3492137339324));
#200118=CARTESIAN_POINT('Origin',(112.333891749004,-3.75,48.3492137339324));
#200119=CARTESIAN_POINT('',(112.824705251554,-3.75,48.4446186903817));
#200120=CARTESIAN_POINT('',(112.767462277684,-3.75,48.7391067919114));
#200121=CARTESIAN_POINT('',(112.824705251554,-3.75,48.4446186903817));
#200122=CARTESIAN_POINT('',(112.276648775135,-3.75,48.6437018354621));
#200123=CARTESIAN_POINT('',(112.276648775135,-3.75,48.6437018354621));
#200124=CARTESIAN_POINT('',(112.333891749004,-3.75,48.3492137339324));
#200125=CARTESIAN_POINT('',(112.333891749004,-3.75,48.3492137339324));
#200126=CARTESIAN_POINT('',(112.333891749004,-3.75,48.3492137339324));
#200127=CARTESIAN_POINT('Origin',(112.824705251554,-3.75,48.4446186903817));
#200128=CARTESIAN_POINT('',(112.824705251554,-4.25,48.4446186903817));
#200129=CARTESIAN_POINT('',(112.767462277684,-4.25,48.7391067919114));
#200130=CARTESIAN_POINT('',(112.824705251554,-4.25,48.4446186903817));
#200131=CARTESIAN_POINT('',(112.767462277684,-3.75,48.7391067919114));
#200132=CARTESIAN_POINT('',(112.824705251554,-3.75,48.4446186903817));
#200133=CARTESIAN_POINT('Origin',(112.824705251554,-4.25,48.4446186903817));
#200134=CARTESIAN_POINT('',(112.333891749004,-4.25,48.3492137339324));
#200135=CARTESIAN_POINT('',(112.276648775135,-4.25,48.6437018354621));
#200136=CARTESIAN_POINT('',(112.333891749004,-4.25,48.3492137339324));
#200137=CARTESIAN_POINT('',(112.767462277684,-4.25,48.7391067919114));
#200138=CARTESIAN_POINT('',(112.824705251554,-4.25,48.4446186903817));
#200139=CARTESIAN_POINT('Origin',(112.333891749004,-4.25,48.3492137339324));
#200140=CARTESIAN_POINT('',(112.276648775135,-4.25,48.6437018354621));
#200141=CARTESIAN_POINT('',(112.333891749004,-4.25,48.3492137339324));
#200142=CARTESIAN_POINT('Origin',(112.333891749004,-4.55,48.3492137339324));
#200143=CARTESIAN_POINT('',(112.824705251554,-4.55,48.4446186903817));
#200144=CARTESIAN_POINT('',(112.767462277684,-4.55,48.7391067919114));
#200145=CARTESIAN_POINT('',(112.824705251554,-4.55,48.4446186903817));
#200146=CARTESIAN_POINT('',(112.276648775135,-4.55,48.6437018354621));
#200147=CARTESIAN_POINT('',(112.276648775135,-4.55,48.6437018354621));
#200148=CARTESIAN_POINT('',(112.333891749004,-4.55,48.3492137339324));
#200149=CARTESIAN_POINT('',(112.333891749004,-4.55,48.3492137339324));
#200150=CARTESIAN_POINT('',(112.333891749004,-4.55,48.3492137339324));
#200151=CARTESIAN_POINT('Origin',(112.824705251554,-4.55,48.4446186903817));
#200152=CARTESIAN_POINT('',(112.824705251554,-5.05,48.4446186903817));
#200153=CARTESIAN_POINT('',(112.767462277684,-5.05,48.7391067919114));
#200154=CARTESIAN_POINT('',(112.824705251554,-5.05,48.4446186903817));
#200155=CARTESIAN_POINT('',(112.767462277684,-4.55,48.7391067919114));
#200156=CARTESIAN_POINT('',(112.824705251554,-4.55,48.4446186903817));
#200157=CARTESIAN_POINT('Origin',(112.824705251554,-5.05,48.4446186903817));
#200158=CARTESIAN_POINT('',(112.333891749004,-5.05,48.3492137339324));
#200159=CARTESIAN_POINT('',(112.276648775135,-5.05,48.6437018354621));
#200160=CARTESIAN_POINT('',(112.333891749004,-5.05,48.3492137339324));
#200161=CARTESIAN_POINT('',(112.767462277684,-5.05,48.7391067919114));
#200162=CARTESIAN_POINT('',(112.824705251554,-5.05,48.4446186903817));
#200163=CARTESIAN_POINT('Origin',(112.333891749004,-5.05,48.3492137339324));
#200164=CARTESIAN_POINT('',(112.276648775135,-5.05,48.6437018354621));
#200165=CARTESIAN_POINT('',(112.333891749004,-5.05,48.3492137339324));
#200166=CARTESIAN_POINT('Origin',(113.119193353083,-4.55,48.5018616642512));
#200167=CARTESIAN_POINT('',(113.610006855633,-4.55,48.5972666207005));
#200168=CARTESIAN_POINT('',(113.552763881763,-4.55,48.8917547222302));
#200169=CARTESIAN_POINT('',(113.610006855633,-4.55,48.5972666207005));
#200170=CARTESIAN_POINT('',(113.061950379214,-4.55,48.7963497657809));
#200171=CARTESIAN_POINT('',(113.061950379214,-4.55,48.7963497657809));
#200172=CARTESIAN_POINT('',(113.119193353083,-4.55,48.5018616642512));
#200173=CARTESIAN_POINT('',(113.119193353083,-4.55,48.5018616642512));
#200174=CARTESIAN_POINT('',(113.119193353083,-4.55,48.5018616642512));
#200175=CARTESIAN_POINT('Origin',(113.610006855633,-4.55,48.5972666207005));
#200176=CARTESIAN_POINT('',(113.610006855633,-5.05,48.5972666207005));
#200177=CARTESIAN_POINT('',(113.552763881763,-5.05,48.8917547222302));
#200178=CARTESIAN_POINT('',(113.610006855633,-5.05,48.5972666207005));
#200179=CARTESIAN_POINT('',(113.552763881763,-4.55,48.8917547222302));
#200180=CARTESIAN_POINT('',(113.610006855633,-4.55,48.5972666207005));
#200181=CARTESIAN_POINT('Origin',(113.610006855633,-5.05,48.5972666207005));
#200182=CARTESIAN_POINT('',(113.119193353083,-5.05,48.5018616642512));
#200183=CARTESIAN_POINT('',(113.061950379214,-5.05,48.7963497657809));
#200184=CARTESIAN_POINT('',(113.119193353083,-5.05,48.5018616642512));
#200185=CARTESIAN_POINT('',(113.552763881763,-5.05,48.8917547222302));
#200186=CARTESIAN_POINT('',(113.610006855633,-5.05,48.5972666207005));
#200187=CARTESIAN_POINT('Origin',(113.119193353083,-5.05,48.5018616642512));
#200188=CARTESIAN_POINT('',(113.061950379214,-5.05,48.7963497657809));
#200189=CARTESIAN_POINT('',(113.119193353083,-5.05,48.5018616642512));
#200190=CARTESIAN_POINT('Origin',(113.904494957163,-4.55,48.65450959457));
#200191=CARTESIAN_POINT('',(114.395308459712,-4.55,48.7499145510193));
#200192=CARTESIAN_POINT('',(114.338065485842,-4.55,49.044402652549));
#200193=CARTESIAN_POINT('',(114.395308459712,-4.55,48.7499145510193));
#200194=CARTESIAN_POINT('',(113.847251983293,-4.55,48.9489976960997));
#200195=CARTESIAN_POINT('',(113.847251983293,-4.55,48.9489976960997));
#200196=CARTESIAN_POINT('',(113.904494957163,-4.55,48.65450959457));
#200197=CARTESIAN_POINT('',(113.904494957163,-4.55,48.65450959457));
#200198=CARTESIAN_POINT('',(113.904494957163,-4.55,48.65450959457));
#200199=CARTESIAN_POINT('Origin',(114.395308459712,-4.55,48.7499145510193));
#200200=CARTESIAN_POINT('',(114.395308459712,-5.05,48.7499145510193));
#200201=CARTESIAN_POINT('',(114.338065485842,-5.05,49.044402652549));
#200202=CARTESIAN_POINT('',(114.395308459712,-5.05,48.7499145510193));
#200203=CARTESIAN_POINT('',(114.338065485842,-4.55,49.044402652549));
#200204=CARTESIAN_POINT('',(114.395308459712,-4.55,48.7499145510193));
#200205=CARTESIAN_POINT('Origin',(114.395308459712,-5.05,48.7499145510193));
#200206=CARTESIAN_POINT('',(113.904494957163,-5.05,48.65450959457));
#200207=CARTESIAN_POINT('',(113.847251983293,-5.05,48.9489976960997));
#200208=CARTESIAN_POINT('',(113.904494957163,-5.05,48.65450959457));
#200209=CARTESIAN_POINT('',(114.338065485842,-5.05,49.044402652549));
#200210=CARTESIAN_POINT('',(114.395308459712,-5.05,48.7499145510193));
#200211=CARTESIAN_POINT('Origin',(113.904494957163,-5.05,48.65450959457));
#200212=CARTESIAN_POINT('',(113.847251983293,-5.05,48.9489976960997));
#200213=CARTESIAN_POINT('',(113.904494957163,-5.05,48.65450959457));
#200214=CARTESIAN_POINT('Origin',(114.689796561242,-4.55,48.8071575248888));
#200215=CARTESIAN_POINT('',(115.180610063791,-4.55,48.9025624813381));
#200216=CARTESIAN_POINT('',(115.123367089922,-4.55,49.1970505828678));
#200217=CARTESIAN_POINT('',(115.180610063791,-4.55,48.9025624813381));
#200218=CARTESIAN_POINT('',(114.632553587372,-4.55,49.1016456264185));
#200219=CARTESIAN_POINT('',(114.632553587372,-4.55,49.1016456264185));
#200220=CARTESIAN_POINT('',(114.689796561242,-4.55,48.8071575248888));
#200221=CARTESIAN_POINT('',(114.689796561242,-4.55,48.8071575248888));
#200222=CARTESIAN_POINT('',(114.689796561242,-4.55,48.8071575248888));
#200223=CARTESIAN_POINT('Origin',(115.180610063791,-4.55,48.9025624813381));
#200224=CARTESIAN_POINT('',(115.180610063791,-5.05,48.9025624813381));
#200225=CARTESIAN_POINT('',(115.123367089922,-5.05,49.1970505828678));
#200226=CARTESIAN_POINT('',(115.180610063791,-5.05,48.9025624813381));
#200227=CARTESIAN_POINT('',(115.123367089922,-4.55,49.1970505828678));
#200228=CARTESIAN_POINT('',(115.180610063791,-4.55,48.9025624813381));
#200229=CARTESIAN_POINT('Origin',(115.180610063791,-5.05,48.9025624813381));
#200230=CARTESIAN_POINT('',(114.689796561242,-5.05,48.8071575248888));
#200231=CARTESIAN_POINT('',(114.632553587372,-5.05,49.1016456264185));
#200232=CARTESIAN_POINT('',(114.689796561242,-5.05,48.8071575248888));
#200233=CARTESIAN_POINT('',(115.123367089922,-5.05,49.1970505828678));
#200234=CARTESIAN_POINT('',(115.180610063791,-5.05,48.9025624813381));
#200235=CARTESIAN_POINT('Origin',(114.689796561242,-5.05,48.8071575248888));
#200236=CARTESIAN_POINT('',(114.632553587372,-5.05,49.1016456264185));
#200237=CARTESIAN_POINT('',(114.689796561242,-5.05,48.8071575248888));
#200238=CARTESIAN_POINT('Origin',(115.475098165321,-4.55,48.9598054552076));
#200239=CARTESIAN_POINT('',(115.96591166787,-4.55,49.0552104116569));
#200240=CARTESIAN_POINT('',(115.908668694001,-4.55,49.3496985131866));
#200241=CARTESIAN_POINT('',(115.96591166787,-4.55,49.0552104116569));
#200242=CARTESIAN_POINT('',(115.417855191451,-4.55,49.2542935567373));
#200243=CARTESIAN_POINT('',(115.417855191451,-4.55,49.2542935567373));
#200244=CARTESIAN_POINT('',(115.475098165321,-4.55,48.9598054552076));
#200245=CARTESIAN_POINT('',(115.475098165321,-4.55,48.9598054552076));
#200246=CARTESIAN_POINT('',(115.475098165321,-4.55,48.9598054552076));
#200247=CARTESIAN_POINT('Origin',(115.96591166787,-4.55,49.0552104116569));
#200248=CARTESIAN_POINT('',(115.96591166787,-5.05,49.0552104116569));
#200249=CARTESIAN_POINT('',(115.908668694001,-5.05,49.3496985131866));
#200250=CARTESIAN_POINT('',(115.96591166787,-5.05,49.0552104116569));
#200251=CARTESIAN_POINT('',(115.908668694001,-4.55,49.3496985131866));
#200252=CARTESIAN_POINT('',(115.96591166787,-4.55,49.0552104116569));
#200253=CARTESIAN_POINT('Origin',(115.96591166787,-5.05,49.0552104116569));
#200254=CARTESIAN_POINT('',(115.475098165321,-5.05,48.9598054552076));
#200255=CARTESIAN_POINT('',(115.417855191451,-5.05,49.2542935567373));
#200256=CARTESIAN_POINT('',(115.475098165321,-5.05,48.9598054552076));
#200257=CARTESIAN_POINT('',(115.908668694001,-5.05,49.3496985131866));
#200258=CARTESIAN_POINT('',(115.96591166787,-5.05,49.0552104116569));
#200259=CARTESIAN_POINT('Origin',(115.475098165321,-5.05,48.9598054552076));
#200260=CARTESIAN_POINT('',(115.417855191451,-5.05,49.2542935567373));
#200261=CARTESIAN_POINT('',(115.475098165321,-5.05,48.9598054552076));
#200262=CARTESIAN_POINT('Origin',(116.2603997694,-4.55,49.1124533855264));
#200263=CARTESIAN_POINT('',(116.75121327195,-4.55,49.2078583419757));
#200264=CARTESIAN_POINT('',(116.69397029808,-4.55,49.5023464435054));
#200265=CARTESIAN_POINT('',(116.75121327195,-4.55,49.2078583419757));
#200266=CARTESIAN_POINT('',(116.203156795531,-4.55,49.4069414870561));
#200267=CARTESIAN_POINT('',(116.203156795531,-4.55,49.4069414870561));
#200268=CARTESIAN_POINT('',(116.2603997694,-4.55,49.1124533855264));
#200269=CARTESIAN_POINT('',(116.2603997694,-4.55,49.1124533855264));
#200270=CARTESIAN_POINT('',(116.2603997694,-4.55,49.1124533855264));
#200271=CARTESIAN_POINT('Origin',(116.75121327195,-4.55,49.2078583419757));
#200272=CARTESIAN_POINT('',(116.75121327195,-5.05,49.2078583419757));
#200273=CARTESIAN_POINT('',(116.69397029808,-5.05,49.5023464435054));
#200274=CARTESIAN_POINT('',(116.75121327195,-5.05,49.2078583419757));
#200275=CARTESIAN_POINT('',(116.69397029808,-4.55,49.5023464435054));
#200276=CARTESIAN_POINT('',(116.75121327195,-4.55,49.2078583419757));
#200277=CARTESIAN_POINT('Origin',(116.75121327195,-5.05,49.2078583419757));
#200278=CARTESIAN_POINT('',(116.2603997694,-5.05,49.1124533855264));
#200279=CARTESIAN_POINT('',(116.203156795531,-5.05,49.4069414870561));
#200280=CARTESIAN_POINT('',(116.2603997694,-5.05,49.1124533855264));
#200281=CARTESIAN_POINT('',(116.69397029808,-5.05,49.5023464435054));
#200282=CARTESIAN_POINT('',(116.75121327195,-5.05,49.2078583419757));
#200283=CARTESIAN_POINT('Origin',(116.2603997694,-5.05,49.1124533855264));
#200284=CARTESIAN_POINT('',(116.203156795531,-5.05,49.4069414870561));
#200285=CARTESIAN_POINT('',(116.2603997694,-5.05,49.1124533855264));
#200286=CARTESIAN_POINT('Origin',(117.045701373479,-4.55,49.2651013158452));
#200287=CARTESIAN_POINT('',(117.536514876029,-4.55,49.3605062722945));
#200288=CARTESIAN_POINT('',(117.479271902159,-4.55,49.6549943738242));
#200289=CARTESIAN_POINT('',(117.536514876029,-4.55,49.3605062722945));
#200290=CARTESIAN_POINT('',(116.98845839961,-4.55,49.5595894173749));
#200291=CARTESIAN_POINT('',(116.98845839961,-4.55,49.5595894173749));
#200292=CARTESIAN_POINT('',(117.045701373479,-4.55,49.2651013158452));
#200293=CARTESIAN_POINT('',(117.045701373479,-4.55,49.2651013158452));
#200294=CARTESIAN_POINT('',(117.045701373479,-4.55,49.2651013158452));
#200295=CARTESIAN_POINT('Origin',(117.536514876029,-4.55,49.3605062722945));
#200296=CARTESIAN_POINT('',(117.536514876029,-5.05,49.3605062722945));
#200297=CARTESIAN_POINT('',(117.479271902159,-5.05,49.6549943738242));
#200298=CARTESIAN_POINT('',(117.536514876029,-5.05,49.3605062722945));
#200299=CARTESIAN_POINT('',(117.479271902159,-4.55,49.6549943738242));
#200300=CARTESIAN_POINT('',(117.536514876029,-4.55,49.3605062722945));
#200301=CARTESIAN_POINT('Origin',(117.536514876029,-5.05,49.3605062722945));
#200302=CARTESIAN_POINT('',(117.045701373479,-5.05,49.2651013158452));
#200303=CARTESIAN_POINT('',(116.98845839961,-5.05,49.5595894173749));
#200304=CARTESIAN_POINT('',(117.045701373479,-5.05,49.2651013158452));
#200305=CARTESIAN_POINT('',(117.479271902159,-5.05,49.6549943738242));
#200306=CARTESIAN_POINT('',(117.536514876029,-5.05,49.3605062722945));
#200307=CARTESIAN_POINT('Origin',(117.045701373479,-5.05,49.2651013158452));
#200308=CARTESIAN_POINT('',(116.98845839961,-5.05,49.5595894173749));
#200309=CARTESIAN_POINT('',(117.045701373479,-5.05,49.2651013158452));
#200310=CARTESIAN_POINT('Origin',(117.831002977559,-4.55,49.417749246164));
#200311=CARTESIAN_POINT('',(118.321816480108,-4.55,49.5131542026133));
#200312=CARTESIAN_POINT('',(118.264573506239,-4.55,49.807642304143));
#200313=CARTESIAN_POINT('',(118.321816480108,-4.55,49.5131542026133));
#200314=CARTESIAN_POINT('',(117.773760003689,-4.55,49.7122373476937));
#200315=CARTESIAN_POINT('',(117.773760003689,-4.55,49.7122373476937));
#200316=CARTESIAN_POINT('',(117.831002977559,-4.55,49.417749246164));
#200317=CARTESIAN_POINT('',(117.831002977559,-4.55,49.417749246164));
#200318=CARTESIAN_POINT('',(117.831002977559,-4.55,49.417749246164));
#200319=CARTESIAN_POINT('Origin',(118.321816480108,-4.55,49.5131542026133));
#200320=CARTESIAN_POINT('',(118.321816480108,-5.05,49.5131542026133));
#200321=CARTESIAN_POINT('',(118.264573506239,-5.05,49.807642304143));
#200322=CARTESIAN_POINT('',(118.321816480108,-5.05,49.5131542026133));
#200323=CARTESIAN_POINT('',(118.264573506239,-4.55,49.807642304143));
#200324=CARTESIAN_POINT('',(118.321816480108,-4.55,49.5131542026133));
#200325=CARTESIAN_POINT('Origin',(118.321816480108,-5.05,49.5131542026133));
#200326=CARTESIAN_POINT('',(117.831002977559,-5.05,49.417749246164));
#200327=CARTESIAN_POINT('',(117.773760003689,-5.05,49.7122373476937));
#200328=CARTESIAN_POINT('',(117.831002977559,-5.05,49.417749246164));
#200329=CARTESIAN_POINT('',(118.264573506239,-5.05,49.807642304143));
#200330=CARTESIAN_POINT('',(118.321816480108,-5.05,49.5131542026133));
#200331=CARTESIAN_POINT('Origin',(117.831002977559,-5.05,49.417749246164));
#200332=CARTESIAN_POINT('',(117.773760003689,-5.05,49.7122373476937));
#200333=CARTESIAN_POINT('',(117.831002977559,-5.05,49.417749246164));
#200334=CARTESIAN_POINT('Origin',(118.616304581638,-4.55,49.5703971764828));
#200335=CARTESIAN_POINT('',(119.107118084187,-4.55,49.6658021329321));
#200336=CARTESIAN_POINT('',(119.049875110318,-4.55,49.9602902344618));
#200337=CARTESIAN_POINT('',(119.107118084187,-4.55,49.6658021329321));
#200338=CARTESIAN_POINT('',(118.559061607768,-4.55,49.8648852780125));
#200339=CARTESIAN_POINT('',(118.559061607768,-4.55,49.8648852780125));
#200340=CARTESIAN_POINT('',(118.616304581638,-4.55,49.5703971764828));
#200341=CARTESIAN_POINT('',(118.616304581638,-4.55,49.5703971764828));
#200342=CARTESIAN_POINT('',(118.616304581638,-4.55,49.5703971764828));
#200343=CARTESIAN_POINT('Origin',(119.107118084187,-4.55,49.6658021329321));
#200344=CARTESIAN_POINT('',(119.107118084187,-5.05,49.6658021329321));
#200345=CARTESIAN_POINT('',(119.049875110318,-5.05,49.9602902344618));
#200346=CARTESIAN_POINT('',(119.107118084187,-5.05,49.6658021329321));
#200347=CARTESIAN_POINT('',(119.049875110318,-4.55,49.9602902344618));
#200348=CARTESIAN_POINT('',(119.107118084187,-4.55,49.6658021329321));
#200349=CARTESIAN_POINT('Origin',(119.107118084187,-5.05,49.6658021329321));
#200350=CARTESIAN_POINT('',(118.616304581638,-5.05,49.5703971764828));
#200351=CARTESIAN_POINT('',(118.559061607768,-5.05,49.8648852780125));
#200352=CARTESIAN_POINT('',(118.616304581638,-5.05,49.5703971764828));
#200353=CARTESIAN_POINT('',(119.049875110318,-5.05,49.9602902344618));
#200354=CARTESIAN_POINT('',(119.107118084187,-5.05,49.6658021329321));
#200355=CARTESIAN_POINT('Origin',(118.616304581638,-5.05,49.5703971764828));
#200356=CARTESIAN_POINT('',(118.559061607768,-5.05,49.8648852780125));
#200357=CARTESIAN_POINT('',(118.616304581638,-5.05,49.5703971764828));
#200358=CARTESIAN_POINT('Origin',(119.401606185717,-4.55,49.7230451068016));
#200359=CARTESIAN_POINT('',(119.892419688267,-4.55,49.8184500632509));
#200360=CARTESIAN_POINT('',(119.835176714397,-4.55,50.1129381647806));
#200361=CARTESIAN_POINT('',(119.892419688267,-4.55,49.8184500632509));
#200362=CARTESIAN_POINT('',(119.344363211847,-4.55,50.0175332083313));
#200363=CARTESIAN_POINT('',(119.344363211847,-4.55,50.0175332083313));
#200364=CARTESIAN_POINT('',(119.401606185717,-4.55,49.7230451068016));
#200365=CARTESIAN_POINT('',(119.401606185717,-4.55,49.7230451068016));
#200366=CARTESIAN_POINT('',(119.401606185717,-4.55,49.7230451068016));
#200367=CARTESIAN_POINT('Origin',(119.892419688267,-4.55,49.8184500632509));
#200368=CARTESIAN_POINT('',(119.892419688267,-5.05,49.8184500632509));
#200369=CARTESIAN_POINT('',(119.835176714397,-5.05,50.1129381647806));
#200370=CARTESIAN_POINT('',(119.892419688267,-5.05,49.8184500632509));
#200371=CARTESIAN_POINT('',(119.835176714397,-4.55,50.1129381647806));
#200372=CARTESIAN_POINT('',(119.892419688267,-4.55,49.8184500632509));
#200373=CARTESIAN_POINT('Origin',(119.892419688267,-5.05,49.8184500632509));
#200374=CARTESIAN_POINT('',(119.401606185717,-5.05,49.7230451068016));
#200375=CARTESIAN_POINT('',(119.344363211847,-5.05,50.0175332083313));
#200376=CARTESIAN_POINT('',(119.401606185717,-5.05,49.7230451068016));
#200377=CARTESIAN_POINT('',(119.835176714397,-5.05,50.1129381647806));
#200378=CARTESIAN_POINT('',(119.892419688267,-5.05,49.8184500632509));
#200379=CARTESIAN_POINT('Origin',(119.401606185717,-5.05,49.7230451068016));
#200380=CARTESIAN_POINT('',(119.344363211847,-5.05,50.0175332083313));
#200381=CARTESIAN_POINT('',(119.401606185717,-5.05,49.7230451068016));
#200382=CARTESIAN_POINT('Origin',(120.186907789796,-4.55,49.8756930371204));
#200383=CARTESIAN_POINT('',(120.677721292346,-4.55,49.9710979935697));
#200384=CARTESIAN_POINT('',(120.620478318476,-4.55,50.2655860950994));
#200385=CARTESIAN_POINT('',(120.677721292346,-4.55,49.9710979935697));
#200386=CARTESIAN_POINT('',(120.129664815927,-4.55,50.1701811386501));
#200387=CARTESIAN_POINT('',(120.129664815927,-4.55,50.1701811386501));
#200388=CARTESIAN_POINT('',(120.186907789796,-4.55,49.8756930371204));
#200389=CARTESIAN_POINT('',(120.186907789796,-4.55,49.8756930371204));
#200390=CARTESIAN_POINT('',(120.186907789796,-4.55,49.8756930371204));
#200391=CARTESIAN_POINT('Origin',(120.677721292346,-4.55,49.9710979935697));
#200392=CARTESIAN_POINT('',(120.677721292346,-5.05,49.9710979935697));
#200393=CARTESIAN_POINT('',(120.620478318476,-5.05,50.2655860950994));
#200394=CARTESIAN_POINT('',(120.677721292346,-5.05,49.9710979935697));
#200395=CARTESIAN_POINT('',(120.620478318476,-4.55,50.2655860950994));
#200396=CARTESIAN_POINT('',(120.677721292346,-4.55,49.9710979935697));
#200397=CARTESIAN_POINT('Origin',(120.677721292346,-5.05,49.9710979935697));
#200398=CARTESIAN_POINT('',(120.186907789796,-5.05,49.8756930371204));
#200399=CARTESIAN_POINT('',(120.129664815927,-5.05,50.1701811386501));
#200400=CARTESIAN_POINT('',(120.186907789796,-5.05,49.8756930371204));
#200401=CARTESIAN_POINT('',(120.620478318476,-5.05,50.2655860950994));
#200402=CARTESIAN_POINT('',(120.677721292346,-5.05,49.9710979935697));
#200403=CARTESIAN_POINT('Origin',(120.186907789796,-5.05,49.8756930371204));
#200404=CARTESIAN_POINT('',(120.129664815927,-5.05,50.1701811386501));
#200405=CARTESIAN_POINT('',(120.186907789796,-5.05,49.8756930371204));
#200406=CARTESIAN_POINT('Origin',(120.972209393875,-4.55,50.0283409674392));
#200407=CARTESIAN_POINT('',(121.463022896425,-4.55,50.1237459238885));
#200408=CARTESIAN_POINT('',(121.405779922555,-4.55,50.4182340254182));
#200409=CARTESIAN_POINT('',(121.463022896425,-4.55,50.1237459238885));
#200410=CARTESIAN_POINT('',(120.914966420006,-4.55,50.3228290689689));
#200411=CARTESIAN_POINT('',(120.914966420006,-4.55,50.3228290689689));
#200412=CARTESIAN_POINT('',(120.972209393875,-4.55,50.0283409674392));
#200413=CARTESIAN_POINT('',(120.972209393875,-4.55,50.0283409674392));
#200414=CARTESIAN_POINT('',(120.972209393875,-4.55,50.0283409674392));
#200415=CARTESIAN_POINT('Origin',(121.463022896425,-4.55,50.1237459238885));
#200416=CARTESIAN_POINT('',(121.463022896425,-5.05,50.1237459238885));
#200417=CARTESIAN_POINT('',(121.405779922555,-5.05,50.4182340254182));
#200418=CARTESIAN_POINT('',(121.463022896425,-5.05,50.1237459238885));
#200419=CARTESIAN_POINT('',(121.405779922555,-4.55,50.4182340254182));
#200420=CARTESIAN_POINT('',(121.463022896425,-4.55,50.1237459238885));
#200421=CARTESIAN_POINT('Origin',(121.463022896425,-5.05,50.1237459238885));
#200422=CARTESIAN_POINT('',(120.972209393875,-5.05,50.0283409674392));
#200423=CARTESIAN_POINT('',(120.914966420006,-5.05,50.3228290689689));
#200424=CARTESIAN_POINT('',(120.972209393875,-5.05,50.0283409674392));
#200425=CARTESIAN_POINT('',(121.405779922555,-5.05,50.4182340254182));
#200426=CARTESIAN_POINT('',(121.463022896425,-5.05,50.1237459238885));
#200427=CARTESIAN_POINT('Origin',(120.972209393875,-5.05,50.0283409674392));
#200428=CARTESIAN_POINT('',(120.914966420006,-5.05,50.3228290689689));
#200429=CARTESIAN_POINT('',(120.972209393875,-5.05,50.0283409674392));
#200430=CARTESIAN_POINT('Origin',(121.757510997955,-4.55,50.180988897758));
#200431=CARTESIAN_POINT('',(122.248324500504,-4.55,50.2763938542073));
#200432=CARTESIAN_POINT('',(122.191081526635,-4.55,50.570881955737));
#200433=CARTESIAN_POINT('',(122.248324500504,-4.55,50.2763938542073));
#200434=CARTESIAN_POINT('',(121.700268024085,-4.55,50.4754769992877));
#200435=CARTESIAN_POINT('',(121.700268024085,-4.55,50.4754769992877));
#200436=CARTESIAN_POINT('',(121.757510997955,-4.55,50.180988897758));
#200437=CARTESIAN_POINT('',(121.757510997955,-4.55,50.180988897758));
#200438=CARTESIAN_POINT('',(121.757510997955,-4.55,50.180988897758));
#200439=CARTESIAN_POINT('Origin',(122.248324500504,-4.55,50.2763938542073));
#200440=CARTESIAN_POINT('',(122.248324500504,-5.05,50.2763938542073));
#200441=CARTESIAN_POINT('',(122.191081526635,-5.05,50.570881955737));
#200442=CARTESIAN_POINT('',(122.248324500504,-5.05,50.2763938542073));
#200443=CARTESIAN_POINT('',(122.191081526635,-4.55,50.570881955737));
#200444=CARTESIAN_POINT('',(122.248324500504,-4.55,50.2763938542073));
#200445=CARTESIAN_POINT('Origin',(122.248324500504,-5.05,50.2763938542073));
#200446=CARTESIAN_POINT('',(121.757510997955,-5.05,50.180988897758));
#200447=CARTESIAN_POINT('',(121.700268024085,-5.05,50.4754769992877));
#200448=CARTESIAN_POINT('',(121.757510997955,-5.05,50.180988897758));
#200449=CARTESIAN_POINT('',(122.191081526635,-5.05,50.570881955737));
#200450=CARTESIAN_POINT('',(122.248324500504,-5.05,50.2763938542073));
#200451=CARTESIAN_POINT('Origin',(121.757510997955,-5.05,50.180988897758));
#200452=CARTESIAN_POINT('',(121.700268024085,-5.05,50.4754769992877));
#200453=CARTESIAN_POINT('',(121.757510997955,-5.05,50.180988897758));
#200454=CARTESIAN_POINT('Origin',(121.757510997955,-3.75,50.180988897758));
#200455=CARTESIAN_POINT('',(122.248324500504,-3.75,50.2763938542073));
#200456=CARTESIAN_POINT('',(122.191081526635,-3.75,50.570881955737));
#200457=CARTESIAN_POINT('',(122.248324500504,-3.75,50.2763938542073));
#200458=CARTESIAN_POINT('',(121.700268024085,-3.75,50.4754769992877));
#200459=CARTESIAN_POINT('',(121.700268024085,-3.75,50.4754769992877));
#200460=CARTESIAN_POINT('',(121.757510997955,-3.75,50.180988897758));
#200461=CARTESIAN_POINT('',(121.757510997955,-3.75,50.180988897758));
#200462=CARTESIAN_POINT('',(121.757510997955,-3.75,50.180988897758));
#200463=CARTESIAN_POINT('Origin',(122.248324500504,-3.75,50.2763938542073));
#200464=CARTESIAN_POINT('',(122.248324500504,-4.25,50.2763938542073));
#200465=CARTESIAN_POINT('',(122.191081526635,-4.25,50.570881955737));
#200466=CARTESIAN_POINT('',(122.248324500504,-4.25,50.2763938542073));
#200467=CARTESIAN_POINT('',(122.191081526635,-3.75,50.570881955737));
#200468=CARTESIAN_POINT('',(122.248324500504,-3.75,50.2763938542073));
#200469=CARTESIAN_POINT('Origin',(122.248324500504,-4.25,50.2763938542073));
#200470=CARTESIAN_POINT('',(121.757510997955,-4.25,50.180988897758));
#200471=CARTESIAN_POINT('',(121.700268024085,-4.25,50.4754769992877));
#200472=CARTESIAN_POINT('',(121.757510997955,-4.25,50.180988897758));
#200473=CARTESIAN_POINT('',(122.191081526635,-4.25,50.570881955737));
#200474=CARTESIAN_POINT('',(122.248324500504,-4.25,50.2763938542073));
#200475=CARTESIAN_POINT('Origin',(121.757510997955,-4.25,50.180988897758));
#200476=CARTESIAN_POINT('',(121.700268024085,-4.25,50.4754769992877));
#200477=CARTESIAN_POINT('',(121.757510997955,-4.25,50.180988897758));
#200478=CARTESIAN_POINT('Origin',(121.757510997955,-2.95,50.180988897758));
#200479=CARTESIAN_POINT('',(122.248324500504,-2.95,50.2763938542073));
#200480=CARTESIAN_POINT('',(122.191081526635,-2.95,50.570881955737));
#200481=CARTESIAN_POINT('',(122.248324500504,-2.95,50.2763938542073));
#200482=CARTESIAN_POINT('',(121.700268024085,-2.95,50.4754769992877));
#200483=CARTESIAN_POINT('',(121.700268024085,-2.95,50.4754769992877));
#200484=CARTESIAN_POINT('',(121.757510997955,-2.95,50.180988897758));
#200485=CARTESIAN_POINT('',(121.757510997955,-2.95,50.180988897758));
#200486=CARTESIAN_POINT('',(121.757510997955,-2.95,50.180988897758));
#200487=CARTESIAN_POINT('Origin',(122.248324500504,-2.95,50.2763938542073));
#200488=CARTESIAN_POINT('',(122.248324500504,-3.45,50.2763938542073));
#200489=CARTESIAN_POINT('',(122.191081526635,-3.45,50.570881955737));
#200490=CARTESIAN_POINT('',(122.248324500504,-3.45,50.2763938542073));
#200491=CARTESIAN_POINT('',(122.191081526635,-2.95,50.570881955737));
#200492=CARTESIAN_POINT('',(122.248324500504,-2.95,50.2763938542073));
#200493=CARTESIAN_POINT('Origin',(122.248324500504,-3.45,50.2763938542073));
#200494=CARTESIAN_POINT('',(121.757510997955,-3.45,50.180988897758));
#200495=CARTESIAN_POINT('',(121.700268024085,-3.45,50.4754769992877));
#200496=CARTESIAN_POINT('',(121.757510997955,-3.45,50.180988897758));
#200497=CARTESIAN_POINT('',(122.191081526635,-3.45,50.570881955737));
#200498=CARTESIAN_POINT('',(122.248324500504,-3.45,50.2763938542073));
#200499=CARTESIAN_POINT('Origin',(121.757510997955,-3.45,50.180988897758));
#200500=CARTESIAN_POINT('',(121.700268024085,-3.45,50.4754769992877));
#200501=CARTESIAN_POINT('',(121.757510997955,-3.45,50.180988897758));
#200502=CARTESIAN_POINT('Origin',(121.757510997955,-2.15,50.180988897758));
#200503=CARTESIAN_POINT('',(122.248324500504,-2.15,50.2763938542073));
#200504=CARTESIAN_POINT('',(122.191081526635,-2.15,50.570881955737));
#200505=CARTESIAN_POINT('',(122.248324500504,-2.15,50.2763938542073));
#200506=CARTESIAN_POINT('',(121.700268024085,-2.15,50.4754769992877));
#200507=CARTESIAN_POINT('',(121.700268024085,-2.15,50.4754769992877));
#200508=CARTESIAN_POINT('',(121.757510997955,-2.15,50.180988897758));
#200509=CARTESIAN_POINT('',(121.757510997955,-2.15,50.180988897758));
#200510=CARTESIAN_POINT('',(121.757510997955,-2.15,50.180988897758));
#200511=CARTESIAN_POINT('Origin',(122.248324500504,-2.15,50.2763938542073));
#200512=CARTESIAN_POINT('',(122.248324500504,-2.65,50.2763938542073));
#200513=CARTESIAN_POINT('',(122.191081526635,-2.65,50.570881955737));
#200514=CARTESIAN_POINT('',(122.248324500504,-2.65,50.2763938542073));
#200515=CARTESIAN_POINT('',(122.191081526635,-2.15,50.570881955737));
#200516=CARTESIAN_POINT('',(122.248324500504,-2.15,50.2763938542073));
#200517=CARTESIAN_POINT('Origin',(122.248324500504,-2.65,50.2763938542073));
#200518=CARTESIAN_POINT('',(121.757510997955,-2.65,50.180988897758));
#200519=CARTESIAN_POINT('',(121.700268024085,-2.65,50.4754769992877));
#200520=CARTESIAN_POINT('',(121.757510997955,-2.65,50.180988897758));
#200521=CARTESIAN_POINT('',(122.191081526635,-2.65,50.570881955737));
#200522=CARTESIAN_POINT('',(122.248324500504,-2.65,50.2763938542073));
#200523=CARTESIAN_POINT('Origin',(121.757510997955,-2.65,50.180988897758));
#200524=CARTESIAN_POINT('',(121.700268024085,-2.65,50.4754769992877));
#200525=CARTESIAN_POINT('',(121.757510997955,-2.65,50.180988897758));
#200526=CARTESIAN_POINT('Origin',(121.757510997955,-1.35,50.180988897758));
#200527=CARTESIAN_POINT('',(122.248324500504,-1.35,50.2763938542073));
#200528=CARTESIAN_POINT('',(122.191081526635,-1.35,50.570881955737));
#200529=CARTESIAN_POINT('',(122.248324500504,-1.35,50.2763938542073));
#200530=CARTESIAN_POINT('',(121.700268024085,-1.35,50.4754769992877));
#200531=CARTESIAN_POINT('',(121.700268024085,-1.35,50.4754769992877));
#200532=CARTESIAN_POINT('',(121.757510997955,-1.35,50.180988897758));
#200533=CARTESIAN_POINT('',(121.757510997955,-1.35,50.180988897758));
#200534=CARTESIAN_POINT('',(121.757510997955,-1.35,50.180988897758));
#200535=CARTESIAN_POINT('Origin',(122.248324500504,-1.35,50.2763938542073));
#200536=CARTESIAN_POINT('',(122.248324500504,-1.85,50.2763938542073));
#200537=CARTESIAN_POINT('',(122.191081526635,-1.85,50.570881955737));
#200538=CARTESIAN_POINT('',(122.248324500504,-1.85,50.2763938542073));
#200539=CARTESIAN_POINT('',(122.191081526635,-1.35,50.570881955737));
#200540=CARTESIAN_POINT('',(122.248324500504,-1.35,50.2763938542073));
#200541=CARTESIAN_POINT('Origin',(122.248324500504,-1.85,50.2763938542073));
#200542=CARTESIAN_POINT('',(121.757510997955,-1.85,50.180988897758));
#200543=CARTESIAN_POINT('',(121.700268024085,-1.85,50.4754769992877));
#200544=CARTESIAN_POINT('',(121.757510997955,-1.85,50.180988897758));
#200545=CARTESIAN_POINT('',(122.191081526635,-1.85,50.570881955737));
#200546=CARTESIAN_POINT('',(122.248324500504,-1.85,50.2763938542073));
#200547=CARTESIAN_POINT('Origin',(121.757510997955,-1.85,50.180988897758));
#200548=CARTESIAN_POINT('',(121.700268024085,-1.85,50.4754769992877));
#200549=CARTESIAN_POINT('',(121.757510997955,-1.85,50.180988897758));
#200550=CARTESIAN_POINT('Origin',(121.757510997955,-0.549999999999986,50.180988897758));
#200551=CARTESIAN_POINT('',(122.248324500504,-0.549999999999986,50.2763938542073));
#200552=CARTESIAN_POINT('',(122.191081526635,-0.549999999999986,50.570881955737));
#200553=CARTESIAN_POINT('',(122.248324500504,-0.549999999999986,50.2763938542073));
#200554=CARTESIAN_POINT('',(121.700268024085,-0.549999999999986,50.4754769992877));
#200555=CARTESIAN_POINT('',(121.700268024085,-0.549999999999986,50.4754769992877));
#200556=CARTESIAN_POINT('',(121.757510997955,-0.549999999999986,50.180988897758));
#200557=CARTESIAN_POINT('',(121.757510997955,-0.549999999999986,50.180988897758));
#200558=CARTESIAN_POINT('',(121.757510997955,-0.549999999999986,50.180988897758));
#200559=CARTESIAN_POINT('Origin',(122.248324500504,-0.549999999999986,50.2763938542073));
#200560=CARTESIAN_POINT('',(122.248324500504,-1.05,50.2763938542073));
#200561=CARTESIAN_POINT('',(122.191081526635,-1.05,50.570881955737));
#200562=CARTESIAN_POINT('',(122.248324500504,-1.05,50.2763938542073));
#200563=CARTESIAN_POINT('',(122.191081526635,-0.549999999999986,50.570881955737));
#200564=CARTESIAN_POINT('',(122.248324500504,-0.549999999999986,50.2763938542073));
#200565=CARTESIAN_POINT('Origin',(122.248324500504,-1.05,50.2763938542073));
#200566=CARTESIAN_POINT('',(121.757510997955,-1.05,50.180988897758));
#200567=CARTESIAN_POINT('',(121.700268024085,-1.05,50.4754769992877));
#200568=CARTESIAN_POINT('',(121.757510997955,-1.05,50.180988897758));
#200569=CARTESIAN_POINT('',(122.191081526635,-1.05,50.570881955737));
#200570=CARTESIAN_POINT('',(122.248324500504,-1.05,50.2763938542073));
#200571=CARTESIAN_POINT('Origin',(121.757510997955,-1.05,50.180988897758));
#200572=CARTESIAN_POINT('',(121.700268024085,-1.05,50.4754769992877));
#200573=CARTESIAN_POINT('',(121.757510997955,-1.05,50.180988897758));
#200574=CARTESIAN_POINT('Origin',(121.757510997955,0.250000000000015,50.180988897758));
#200575=CARTESIAN_POINT('',(122.248324500504,0.250000000000015,50.2763938542073));
#200576=CARTESIAN_POINT('',(122.191081526635,0.250000000000015,50.570881955737));
#200577=CARTESIAN_POINT('',(122.248324500504,0.250000000000015,50.2763938542073));
#200578=CARTESIAN_POINT('',(121.700268024085,0.250000000000015,50.4754769992877));
#200579=CARTESIAN_POINT('',(121.700268024085,0.250000000000015,50.4754769992877));
#200580=CARTESIAN_POINT('',(121.757510997955,0.250000000000015,50.180988897758));
#200581=CARTESIAN_POINT('',(121.757510997955,0.250000000000015,50.180988897758));
#200582=CARTESIAN_POINT('',(121.757510997955,0.250000000000015,50.180988897758));
#200583=CARTESIAN_POINT('Origin',(122.248324500504,0.250000000000015,50.2763938542073));
#200584=CARTESIAN_POINT('',(122.248324500504,-0.249999999999985,50.2763938542073));
#200585=CARTESIAN_POINT('',(122.191081526635,-0.249999999999985,50.570881955737));
#200586=CARTESIAN_POINT('',(122.248324500504,-0.249999999999985,50.2763938542073));
#200587=CARTESIAN_POINT('',(122.191081526635,0.250000000000015,50.570881955737));
#200588=CARTESIAN_POINT('',(122.248324500504,0.250000000000015,50.2763938542073));
#200589=CARTESIAN_POINT('Origin',(122.248324500504,-0.249999999999985,50.2763938542073));
#200590=CARTESIAN_POINT('',(121.757510997955,-0.249999999999985,50.180988897758));
#200591=CARTESIAN_POINT('',(121.700268024085,-0.249999999999985,50.4754769992877));
#200592=CARTESIAN_POINT('',(121.757510997955,-0.249999999999985,50.180988897758));
#200593=CARTESIAN_POINT('',(122.191081526635,-0.249999999999985,50.570881955737));
#200594=CARTESIAN_POINT('',(122.248324500504,-0.249999999999985,50.2763938542073));
#200595=CARTESIAN_POINT('Origin',(121.757510997955,-0.249999999999985,50.180988897758));
#200596=CARTESIAN_POINT('',(121.700268024085,-0.249999999999985,50.4754769992877));
#200597=CARTESIAN_POINT('',(121.757510997955,-0.249999999999985,50.180988897758));
#200598=CARTESIAN_POINT('Origin',(121.757510997955,1.05,50.180988897758));
#200599=CARTESIAN_POINT('',(122.248324500504,1.05,50.2763938542073));
#200600=CARTESIAN_POINT('',(122.191081526635,1.05,50.570881955737));
#200601=CARTESIAN_POINT('',(122.248324500504,1.05,50.2763938542073));
#200602=CARTESIAN_POINT('',(121.700268024085,1.05,50.4754769992877));
#200603=CARTESIAN_POINT('',(121.700268024085,1.05,50.4754769992877));
#200604=CARTESIAN_POINT('',(121.757510997955,1.05,50.180988897758));
#200605=CARTESIAN_POINT('',(121.757510997955,1.05,50.180988897758));
#200606=CARTESIAN_POINT('',(121.757510997955,1.05,50.180988897758));
#200607=CARTESIAN_POINT('Origin',(122.248324500504,1.05,50.2763938542073));
#200608=CARTESIAN_POINT('',(122.248324500504,0.550000000000015,50.2763938542073));
#200609=CARTESIAN_POINT('',(122.191081526635,0.550000000000015,50.570881955737));
#200610=CARTESIAN_POINT('',(122.248324500504,0.550000000000015,50.2763938542073));
#200611=CARTESIAN_POINT('',(122.191081526635,1.05,50.570881955737));
#200612=CARTESIAN_POINT('',(122.248324500504,1.05,50.2763938542073));
#200613=CARTESIAN_POINT('Origin',(122.248324500504,0.550000000000015,50.2763938542073));
#200614=CARTESIAN_POINT('',(121.757510997955,0.550000000000015,50.180988897758));
#200615=CARTESIAN_POINT('',(121.700268024085,0.550000000000015,50.4754769992877));
#200616=CARTESIAN_POINT('',(121.757510997955,0.550000000000015,50.180988897758));
#200617=CARTESIAN_POINT('',(122.191081526635,0.550000000000015,50.570881955737));
#200618=CARTESIAN_POINT('',(122.248324500504,0.550000000000015,50.2763938542073));
#200619=CARTESIAN_POINT('Origin',(121.757510997955,0.550000000000015,50.180988897758));
#200620=CARTESIAN_POINT('',(121.700268024085,0.550000000000015,50.4754769992877));
#200621=CARTESIAN_POINT('',(121.757510997955,0.550000000000015,50.180988897758));
#200622=CARTESIAN_POINT('Origin',(121.757510997955,1.85,50.180988897758));
#200623=CARTESIAN_POINT('',(122.248324500504,1.85,50.2763938542073));
#200624=CARTESIAN_POINT('',(122.191081526635,1.85,50.570881955737));
#200625=CARTESIAN_POINT('',(122.248324500504,1.85,50.2763938542073));
#200626=CARTESIAN_POINT('',(121.700268024085,1.85,50.4754769992877));
#200627=CARTESIAN_POINT('',(121.700268024085,1.85,50.4754769992877));
#200628=CARTESIAN_POINT('',(121.757510997955,1.85,50.180988897758));
#200629=CARTESIAN_POINT('',(121.757510997955,1.85,50.180988897758));
#200630=CARTESIAN_POINT('',(121.757510997955,1.85,50.180988897758));
#200631=CARTESIAN_POINT('Origin',(122.248324500504,1.85,50.2763938542073));
#200632=CARTESIAN_POINT('',(122.248324500504,1.35,50.2763938542073));
#200633=CARTESIAN_POINT('',(122.191081526635,1.35,50.570881955737));
#200634=CARTESIAN_POINT('',(122.248324500504,1.35,50.2763938542073));
#200635=CARTESIAN_POINT('',(122.191081526635,1.85,50.570881955737));
#200636=CARTESIAN_POINT('',(122.248324500504,1.85,50.2763938542073));
#200637=CARTESIAN_POINT('Origin',(122.248324500504,1.35,50.2763938542073));
#200638=CARTESIAN_POINT('',(121.757510997955,1.35,50.180988897758));
#200639=CARTESIAN_POINT('',(121.700268024085,1.35,50.4754769992877));
#200640=CARTESIAN_POINT('',(121.757510997955,1.35,50.180988897758));
#200641=CARTESIAN_POINT('',(122.191081526635,1.35,50.570881955737));
#200642=CARTESIAN_POINT('',(122.248324500504,1.35,50.2763938542073));
#200643=CARTESIAN_POINT('Origin',(121.757510997955,1.35,50.180988897758));
#200644=CARTESIAN_POINT('',(121.700268024085,1.35,50.4754769992877));
#200645=CARTESIAN_POINT('',(121.757510997955,1.35,50.180988897758));
#200646=CARTESIAN_POINT('Origin',(121.757510997955,2.65,50.180988897758));
#200647=CARTESIAN_POINT('',(122.248324500504,2.65,50.2763938542073));
#200648=CARTESIAN_POINT('',(122.191081526635,2.65,50.570881955737));
#200649=CARTESIAN_POINT('',(122.248324500504,2.65,50.2763938542073));
#200650=CARTESIAN_POINT('',(121.700268024085,2.65,50.4754769992877));
#200651=CARTESIAN_POINT('',(121.700268024085,2.65,50.4754769992877));
#200652=CARTESIAN_POINT('',(121.757510997955,2.65,50.180988897758));
#200653=CARTESIAN_POINT('',(121.757510997955,2.65,50.180988897758));
#200654=CARTESIAN_POINT('',(121.757510997955,2.65,50.180988897758));
#200655=CARTESIAN_POINT('Origin',(122.248324500504,2.65,50.2763938542073));
#200656=CARTESIAN_POINT('',(122.248324500504,2.15,50.2763938542073));
#200657=CARTESIAN_POINT('',(122.191081526635,2.15,50.570881955737));
#200658=CARTESIAN_POINT('',(122.248324500504,2.15,50.2763938542073));
#200659=CARTESIAN_POINT('',(122.191081526635,2.65,50.570881955737));
#200660=CARTESIAN_POINT('',(122.248324500504,2.65,50.2763938542073));
#200661=CARTESIAN_POINT('Origin',(122.248324500504,2.15,50.2763938542073));
#200662=CARTESIAN_POINT('',(121.757510997955,2.15,50.180988897758));
#200663=CARTESIAN_POINT('',(121.700268024085,2.15,50.4754769992877));
#200664=CARTESIAN_POINT('',(121.757510997955,2.15,50.180988897758));
#200665=CARTESIAN_POINT('',(122.191081526635,2.15,50.570881955737));
#200666=CARTESIAN_POINT('',(122.248324500504,2.15,50.2763938542073));
#200667=CARTESIAN_POINT('Origin',(121.757510997955,2.15,50.180988897758));
#200668=CARTESIAN_POINT('',(121.700268024085,2.15,50.4754769992877));
#200669=CARTESIAN_POINT('',(121.757510997955,2.15,50.180988897758));
#200670=CARTESIAN_POINT('Origin',(121.757510997955,3.45,50.180988897758));
#200671=CARTESIAN_POINT('',(122.248324500504,3.45,50.2763938542073));
#200672=CARTESIAN_POINT('',(122.191081526635,3.45,50.570881955737));
#200673=CARTESIAN_POINT('',(122.248324500504,3.45,50.2763938542073));
#200674=CARTESIAN_POINT('',(121.700268024085,3.45,50.4754769992877));
#200675=CARTESIAN_POINT('',(121.700268024085,3.45,50.4754769992877));
#200676=CARTESIAN_POINT('',(121.757510997955,3.45,50.180988897758));
#200677=CARTESIAN_POINT('',(121.757510997955,3.45,50.180988897758));
#200678=CARTESIAN_POINT('',(121.757510997955,3.45,50.180988897758));
#200679=CARTESIAN_POINT('Origin',(122.248324500504,3.45,50.2763938542073));
#200680=CARTESIAN_POINT('',(122.248324500504,2.95,50.2763938542073));
#200681=CARTESIAN_POINT('',(122.191081526635,2.95,50.570881955737));
#200682=CARTESIAN_POINT('',(122.248324500504,2.95,50.2763938542073));
#200683=CARTESIAN_POINT('',(122.191081526635,3.45,50.570881955737));
#200684=CARTESIAN_POINT('',(122.248324500504,3.45,50.2763938542073));
#200685=CARTESIAN_POINT('Origin',(122.248324500504,2.95,50.2763938542073));
#200686=CARTESIAN_POINT('',(121.757510997955,2.95,50.180988897758));
#200687=CARTESIAN_POINT('',(121.700268024085,2.95,50.4754769992877));
#200688=CARTESIAN_POINT('',(121.757510997955,2.95,50.180988897758));
#200689=CARTESIAN_POINT('',(122.191081526635,2.95,50.570881955737));
#200690=CARTESIAN_POINT('',(122.248324500504,2.95,50.2763938542073));
#200691=CARTESIAN_POINT('Origin',(121.757510997955,2.95,50.180988897758));
#200692=CARTESIAN_POINT('',(121.700268024085,2.95,50.4754769992877));
#200693=CARTESIAN_POINT('',(121.757510997955,2.95,50.180988897758));
#200694=CARTESIAN_POINT('Origin',(121.757510997955,4.25,50.180988897758));
#200695=CARTESIAN_POINT('',(122.248324500504,4.25,50.2763938542073));
#200696=CARTESIAN_POINT('',(122.191081526635,4.25,50.570881955737));
#200697=CARTESIAN_POINT('',(122.248324500504,4.25,50.2763938542073));
#200698=CARTESIAN_POINT('',(121.700268024085,4.25,50.4754769992877));
#200699=CARTESIAN_POINT('',(121.700268024085,4.25,50.4754769992877));
#200700=CARTESIAN_POINT('',(121.757510997955,4.25,50.180988897758));
#200701=CARTESIAN_POINT('',(121.757510997955,4.25,50.180988897758));
#200702=CARTESIAN_POINT('',(121.757510997955,4.25,50.180988897758));
#200703=CARTESIAN_POINT('Origin',(122.248324500504,4.25,50.2763938542073));
#200704=CARTESIAN_POINT('',(122.248324500504,3.75,50.2763938542073));
#200705=CARTESIAN_POINT('',(122.191081526635,3.75,50.570881955737));
#200706=CARTESIAN_POINT('',(122.248324500504,3.75,50.2763938542073));
#200707=CARTESIAN_POINT('',(122.191081526635,4.25,50.570881955737));
#200708=CARTESIAN_POINT('',(122.248324500504,4.25,50.2763938542073));
#200709=CARTESIAN_POINT('Origin',(122.248324500504,3.75,50.2763938542073));
#200710=CARTESIAN_POINT('',(121.757510997955,3.75,50.180988897758));
#200711=CARTESIAN_POINT('',(121.700268024085,3.75,50.4754769992877));
#200712=CARTESIAN_POINT('',(121.757510997955,3.75,50.180988897758));
#200713=CARTESIAN_POINT('',(122.191081526635,3.75,50.570881955737));
#200714=CARTESIAN_POINT('',(122.248324500504,3.75,50.2763938542073));
#200715=CARTESIAN_POINT('Origin',(121.757510997955,3.75,50.180988897758));
#200716=CARTESIAN_POINT('',(121.700268024085,3.75,50.4754769992877));
#200717=CARTESIAN_POINT('',(121.757510997955,3.75,50.180988897758));
#200718=CARTESIAN_POINT('Origin',(121.757510997955,5.05,50.180988897758));
#200719=CARTESIAN_POINT('',(122.248324500504,5.05,50.2763938542073));
#200720=CARTESIAN_POINT('',(122.191081526635,5.05,50.570881955737));
#200721=CARTESIAN_POINT('',(122.248324500504,5.05,50.2763938542073));
#200722=CARTESIAN_POINT('',(121.700268024085,5.05,50.4754769992877));
#200723=CARTESIAN_POINT('',(121.700268024085,5.05,50.4754769992877));
#200724=CARTESIAN_POINT('',(121.757510997955,5.05,50.180988897758));
#200725=CARTESIAN_POINT('',(121.757510997955,5.05,50.180988897758));
#200726=CARTESIAN_POINT('',(121.757510997955,5.05,50.180988897758));
#200727=CARTESIAN_POINT('Origin',(122.248324500504,5.05,50.2763938542073));
#200728=CARTESIAN_POINT('',(122.248324500504,4.55,50.2763938542073));
#200729=CARTESIAN_POINT('',(122.191081526635,4.55,50.570881955737));
#200730=CARTESIAN_POINT('',(122.248324500504,4.55,50.2763938542073));
#200731=CARTESIAN_POINT('',(122.191081526635,5.05,50.570881955737));
#200732=CARTESIAN_POINT('',(122.248324500504,5.05,50.2763938542073));
#200733=CARTESIAN_POINT('Origin',(122.248324500504,4.55,50.2763938542073));
#200734=CARTESIAN_POINT('',(121.757510997955,4.55,50.180988897758));
#200735=CARTESIAN_POINT('',(121.700268024085,4.55,50.4754769992877));
#200736=CARTESIAN_POINT('',(121.757510997955,4.55,50.180988897758));
#200737=CARTESIAN_POINT('',(122.191081526635,4.55,50.570881955737));
#200738=CARTESIAN_POINT('',(122.248324500504,4.55,50.2763938542073));
#200739=CARTESIAN_POINT('Origin',(121.757510997955,4.55,50.180988897758));
#200740=CARTESIAN_POINT('',(121.700268024085,4.55,50.4754769992877));
#200741=CARTESIAN_POINT('',(121.757510997955,4.55,50.180988897758));
#200742=CARTESIAN_POINT('Origin',(120.972209393875,5.05,50.0283409674392));
#200743=CARTESIAN_POINT('',(121.463022896425,5.05,50.1237459238885));
#200744=CARTESIAN_POINT('',(121.405779922555,5.05,50.4182340254182));
#200745=CARTESIAN_POINT('',(121.463022896425,5.05,50.1237459238885));
#200746=CARTESIAN_POINT('',(120.914966420006,5.05,50.3228290689689));
#200747=CARTESIAN_POINT('',(120.914966420006,5.05,50.3228290689689));
#200748=CARTESIAN_POINT('',(120.972209393875,5.05,50.0283409674392));
#200749=CARTESIAN_POINT('',(120.972209393875,5.05,50.0283409674392));
#200750=CARTESIAN_POINT('',(120.972209393875,5.05,50.0283409674392));
#200751=CARTESIAN_POINT('Origin',(121.463022896425,5.05,50.1237459238885));
#200752=CARTESIAN_POINT('',(121.463022896425,4.55,50.1237459238885));
#200753=CARTESIAN_POINT('',(121.405779922555,4.55,50.4182340254182));
#200754=CARTESIAN_POINT('',(121.463022896425,4.55,50.1237459238885));
#200755=CARTESIAN_POINT('',(121.405779922555,5.05,50.4182340254182));
#200756=CARTESIAN_POINT('',(121.463022896425,5.05,50.1237459238885));
#200757=CARTESIAN_POINT('Origin',(121.463022896425,4.55,50.1237459238885));
#200758=CARTESIAN_POINT('',(120.972209393875,4.55,50.0283409674392));
#200759=CARTESIAN_POINT('',(120.914966420006,4.55,50.3228290689689));
#200760=CARTESIAN_POINT('',(120.972209393875,4.55,50.0283409674392));
#200761=CARTESIAN_POINT('',(121.405779922555,4.55,50.4182340254182));
#200762=CARTESIAN_POINT('',(121.463022896425,4.55,50.1237459238885));
#200763=CARTESIAN_POINT('Origin',(120.972209393875,4.55,50.0283409674392));
#200764=CARTESIAN_POINT('',(120.914966420006,4.55,50.3228290689689));
#200765=CARTESIAN_POINT('',(120.972209393875,4.55,50.0283409674392));
#200766=CARTESIAN_POINT('Origin',(120.186907789796,5.05,49.8756930371204));
#200767=CARTESIAN_POINT('',(120.677721292346,5.05,49.9710979935697));
#200768=CARTESIAN_POINT('',(120.620478318476,5.05,50.2655860950994));
#200769=CARTESIAN_POINT('',(120.677721292346,5.05,49.9710979935697));
#200770=CARTESIAN_POINT('',(120.129664815927,5.05,50.1701811386501));
#200771=CARTESIAN_POINT('',(120.129664815927,5.05,50.1701811386501));
#200772=CARTESIAN_POINT('',(120.186907789796,5.05,49.8756930371204));
#200773=CARTESIAN_POINT('',(120.186907789796,5.05,49.8756930371204));
#200774=CARTESIAN_POINT('',(120.186907789796,5.05,49.8756930371204));
#200775=CARTESIAN_POINT('Origin',(120.677721292346,5.05,49.9710979935697));
#200776=CARTESIAN_POINT('',(120.677721292346,4.55,49.9710979935697));
#200777=CARTESIAN_POINT('',(120.620478318476,4.55,50.2655860950994));
#200778=CARTESIAN_POINT('',(120.677721292346,4.55,49.9710979935697));
#200779=CARTESIAN_POINT('',(120.620478318476,5.05,50.2655860950994));
#200780=CARTESIAN_POINT('',(120.677721292346,5.05,49.9710979935697));
#200781=CARTESIAN_POINT('Origin',(120.677721292346,4.55,49.9710979935697));
#200782=CARTESIAN_POINT('',(120.186907789796,4.55,49.8756930371204));
#200783=CARTESIAN_POINT('',(120.129664815927,4.55,50.1701811386501));
#200784=CARTESIAN_POINT('',(120.186907789796,4.55,49.8756930371204));
#200785=CARTESIAN_POINT('',(120.620478318476,4.55,50.2655860950994));
#200786=CARTESIAN_POINT('',(120.677721292346,4.55,49.9710979935697));
#200787=CARTESIAN_POINT('Origin',(120.186907789796,4.55,49.8756930371204));
#200788=CARTESIAN_POINT('',(120.129664815927,4.55,50.1701811386501));
#200789=CARTESIAN_POINT('',(120.186907789796,4.55,49.8756930371204));
#200790=CARTESIAN_POINT('Origin',(119.401606185717,5.05,49.7230451068016));
#200791=CARTESIAN_POINT('',(119.892419688267,5.05,49.8184500632509));
#200792=CARTESIAN_POINT('',(119.835176714397,5.05,50.1129381647806));
#200793=CARTESIAN_POINT('',(119.892419688267,5.05,49.8184500632509));
#200794=CARTESIAN_POINT('',(119.344363211847,5.05,50.0175332083313));
#200795=CARTESIAN_POINT('',(119.344363211847,5.05,50.0175332083313));
#200796=CARTESIAN_POINT('',(119.401606185717,5.05,49.7230451068016));
#200797=CARTESIAN_POINT('',(119.401606185717,5.05,49.7230451068016));
#200798=CARTESIAN_POINT('',(119.401606185717,5.05,49.7230451068016));
#200799=CARTESIAN_POINT('Origin',(119.892419688267,5.05,49.8184500632509));
#200800=CARTESIAN_POINT('',(119.892419688267,4.55,49.8184500632509));
#200801=CARTESIAN_POINT('',(119.835176714397,4.55,50.1129381647806));
#200802=CARTESIAN_POINT('',(119.892419688267,4.55,49.8184500632509));
#200803=CARTESIAN_POINT('',(119.835176714397,5.05,50.1129381647806));
#200804=CARTESIAN_POINT('',(119.892419688267,5.05,49.8184500632509));
#200805=CARTESIAN_POINT('Origin',(119.892419688267,4.55,49.8184500632509));
#200806=CARTESIAN_POINT('',(119.401606185717,4.55,49.7230451068016));
#200807=CARTESIAN_POINT('',(119.344363211847,4.55,50.0175332083313));
#200808=CARTESIAN_POINT('',(119.401606185717,4.55,49.7230451068016));
#200809=CARTESIAN_POINT('',(119.835176714397,4.55,50.1129381647806));
#200810=CARTESIAN_POINT('',(119.892419688267,4.55,49.8184500632509));
#200811=CARTESIAN_POINT('Origin',(119.401606185717,4.55,49.7230451068016));
#200812=CARTESIAN_POINT('',(119.344363211847,4.55,50.0175332083313));
#200813=CARTESIAN_POINT('',(119.401606185717,4.55,49.7230451068016));
#200814=CARTESIAN_POINT('Origin',(118.616304581638,5.05,49.5703971764828));
#200815=CARTESIAN_POINT('',(119.107118084187,5.05,49.6658021329321));
#200816=CARTESIAN_POINT('',(119.049875110318,5.05,49.9602902344618));
#200817=CARTESIAN_POINT('',(119.107118084187,5.05,49.6658021329321));
#200818=CARTESIAN_POINT('',(118.559061607768,5.05,49.8648852780125));
#200819=CARTESIAN_POINT('',(118.559061607768,5.05,49.8648852780125));
#200820=CARTESIAN_POINT('',(118.616304581638,5.05,49.5703971764828));
#200821=CARTESIAN_POINT('',(118.616304581638,5.05,49.5703971764828));
#200822=CARTESIAN_POINT('',(118.616304581638,5.05,49.5703971764828));
#200823=CARTESIAN_POINT('Origin',(119.107118084187,5.05,49.6658021329321));
#200824=CARTESIAN_POINT('',(119.107118084187,4.55,49.6658021329321));
#200825=CARTESIAN_POINT('',(119.049875110318,4.55,49.9602902344618));
#200826=CARTESIAN_POINT('',(119.107118084187,4.55,49.6658021329321));
#200827=CARTESIAN_POINT('',(119.049875110318,5.05,49.9602902344618));
#200828=CARTESIAN_POINT('',(119.107118084187,5.05,49.6658021329321));
#200829=CARTESIAN_POINT('Origin',(119.107118084187,4.55,49.6658021329321));
#200830=CARTESIAN_POINT('',(118.616304581638,4.55,49.5703971764828));
#200831=CARTESIAN_POINT('',(118.559061607768,4.55,49.8648852780125));
#200832=CARTESIAN_POINT('',(118.616304581638,4.55,49.5703971764828));
#200833=CARTESIAN_POINT('',(119.049875110318,4.55,49.9602902344618));
#200834=CARTESIAN_POINT('',(119.107118084187,4.55,49.6658021329321));
#200835=CARTESIAN_POINT('Origin',(118.616304581638,4.55,49.5703971764828));
#200836=CARTESIAN_POINT('',(118.559061607768,4.55,49.8648852780125));
#200837=CARTESIAN_POINT('',(118.616304581638,4.55,49.5703971764828));
#200838=CARTESIAN_POINT('Origin',(117.831002977559,5.05,49.417749246164));
#200839=CARTESIAN_POINT('',(118.321816480108,5.05,49.5131542026133));
#200840=CARTESIAN_POINT('',(118.264573506239,5.05,49.807642304143));
#200841=CARTESIAN_POINT('',(118.321816480108,5.05,49.5131542026133));
#200842=CARTESIAN_POINT('',(117.773760003689,5.05,49.7122373476937));
#200843=CARTESIAN_POINT('',(117.773760003689,5.05,49.7122373476937));
#200844=CARTESIAN_POINT('',(117.831002977559,5.05,49.417749246164));
#200845=CARTESIAN_POINT('',(117.831002977559,5.05,49.417749246164));
#200846=CARTESIAN_POINT('',(117.831002977559,5.05,49.417749246164));
#200847=CARTESIAN_POINT('Origin',(118.321816480108,5.05,49.5131542026133));
#200848=CARTESIAN_POINT('',(118.321816480108,4.55,49.5131542026133));
#200849=CARTESIAN_POINT('',(118.264573506239,4.55,49.807642304143));
#200850=CARTESIAN_POINT('',(118.321816480108,4.55,49.5131542026133));
#200851=CARTESIAN_POINT('',(118.264573506239,5.05,49.807642304143));
#200852=CARTESIAN_POINT('',(118.321816480108,5.05,49.5131542026133));
#200853=CARTESIAN_POINT('Origin',(118.321816480108,4.55,49.5131542026133));
#200854=CARTESIAN_POINT('',(117.831002977559,4.55,49.417749246164));
#200855=CARTESIAN_POINT('',(117.773760003689,4.55,49.7122373476937));
#200856=CARTESIAN_POINT('',(117.831002977559,4.55,49.417749246164));
#200857=CARTESIAN_POINT('',(118.264573506239,4.55,49.807642304143));
#200858=CARTESIAN_POINT('',(118.321816480108,4.55,49.5131542026133));
#200859=CARTESIAN_POINT('Origin',(117.831002977559,4.55,49.417749246164));
#200860=CARTESIAN_POINT('',(117.773760003689,4.55,49.7122373476937));
#200861=CARTESIAN_POINT('',(117.831002977559,4.55,49.417749246164));
#200862=CARTESIAN_POINT('Origin',(117.045701373479,5.05,49.2651013158452));
#200863=CARTESIAN_POINT('',(117.536514876029,5.05,49.3605062722945));
#200864=CARTESIAN_POINT('',(117.479271902159,5.05,49.6549943738242));
#200865=CARTESIAN_POINT('',(117.536514876029,5.05,49.3605062722945));
#200866=CARTESIAN_POINT('',(116.98845839961,5.05,49.5595894173749));
#200867=CARTESIAN_POINT('',(116.98845839961,5.05,49.5595894173749));
#200868=CARTESIAN_POINT('',(117.045701373479,5.05,49.2651013158452));
#200869=CARTESIAN_POINT('',(117.045701373479,5.05,49.2651013158452));
#200870=CARTESIAN_POINT('',(117.045701373479,5.05,49.2651013158452));
#200871=CARTESIAN_POINT('Origin',(117.536514876029,5.05,49.3605062722945));
#200872=CARTESIAN_POINT('',(117.536514876029,4.55,49.3605062722945));
#200873=CARTESIAN_POINT('',(117.479271902159,4.55,49.6549943738242));
#200874=CARTESIAN_POINT('',(117.536514876029,4.55,49.3605062722945));
#200875=CARTESIAN_POINT('',(117.479271902159,5.05,49.6549943738242));
#200876=CARTESIAN_POINT('',(117.536514876029,5.05,49.3605062722945));
#200877=CARTESIAN_POINT('Origin',(117.536514876029,4.55,49.3605062722945));
#200878=CARTESIAN_POINT('',(117.045701373479,4.55,49.2651013158452));
#200879=CARTESIAN_POINT('',(116.98845839961,4.55,49.5595894173749));
#200880=CARTESIAN_POINT('',(117.045701373479,4.55,49.2651013158452));
#200881=CARTESIAN_POINT('',(117.479271902159,4.55,49.6549943738242));
#200882=CARTESIAN_POINT('',(117.536514876029,4.55,49.3605062722945));
#200883=CARTESIAN_POINT('Origin',(117.045701373479,4.55,49.2651013158452));
#200884=CARTESIAN_POINT('',(116.98845839961,4.55,49.5595894173749));
#200885=CARTESIAN_POINT('',(117.045701373479,4.55,49.2651013158452));
#200886=CARTESIAN_POINT('Origin',(116.2603997694,5.05,49.1124533855264));
#200887=CARTESIAN_POINT('',(116.75121327195,5.05,49.2078583419757));
#200888=CARTESIAN_POINT('',(116.69397029808,5.05,49.5023464435054));
#200889=CARTESIAN_POINT('',(116.75121327195,5.05,49.2078583419757));
#200890=CARTESIAN_POINT('',(116.203156795531,5.05,49.4069414870561));
#200891=CARTESIAN_POINT('',(116.203156795531,5.05,49.4069414870561));
#200892=CARTESIAN_POINT('',(116.2603997694,5.05,49.1124533855264));
#200893=CARTESIAN_POINT('',(116.2603997694,5.05,49.1124533855264));
#200894=CARTESIAN_POINT('',(116.2603997694,5.05,49.1124533855264));
#200895=CARTESIAN_POINT('Origin',(116.75121327195,5.05,49.2078583419757));
#200896=CARTESIAN_POINT('',(116.75121327195,4.55,49.2078583419757));
#200897=CARTESIAN_POINT('',(116.69397029808,4.55,49.5023464435054));
#200898=CARTESIAN_POINT('',(116.75121327195,4.55,49.2078583419757));
#200899=CARTESIAN_POINT('',(116.69397029808,5.05,49.5023464435054));
#200900=CARTESIAN_POINT('',(116.75121327195,5.05,49.2078583419757));
#200901=CARTESIAN_POINT('Origin',(116.75121327195,4.55,49.2078583419757));
#200902=CARTESIAN_POINT('',(116.2603997694,4.55,49.1124533855264));
#200903=CARTESIAN_POINT('',(116.203156795531,4.55,49.4069414870561));
#200904=CARTESIAN_POINT('',(116.2603997694,4.55,49.1124533855264));
#200905=CARTESIAN_POINT('',(116.69397029808,4.55,49.5023464435054));
#200906=CARTESIAN_POINT('',(116.75121327195,4.55,49.2078583419757));
#200907=CARTESIAN_POINT('Origin',(116.2603997694,4.55,49.1124533855264));
#200908=CARTESIAN_POINT('',(116.203156795531,4.55,49.4069414870561));
#200909=CARTESIAN_POINT('',(116.2603997694,4.55,49.1124533855264));
#200910=CARTESIAN_POINT('Origin',(115.475098165321,5.05,48.9598054552076));
#200911=CARTESIAN_POINT('',(115.96591166787,5.05,49.0552104116569));
#200912=CARTESIAN_POINT('',(115.908668694001,5.05,49.3496985131866));
#200913=CARTESIAN_POINT('',(115.96591166787,5.05,49.0552104116569));
#200914=CARTESIAN_POINT('',(115.417855191451,5.05,49.2542935567373));
#200915=CARTESIAN_POINT('',(115.417855191451,5.05,49.2542935567373));
#200916=CARTESIAN_POINT('',(115.475098165321,5.05,48.9598054552076));
#200917=CARTESIAN_POINT('',(115.475098165321,5.05,48.9598054552076));
#200918=CARTESIAN_POINT('',(115.475098165321,5.05,48.9598054552076));
#200919=CARTESIAN_POINT('Origin',(115.96591166787,5.05,49.0552104116569));
#200920=CARTESIAN_POINT('',(115.96591166787,4.55,49.0552104116569));
#200921=CARTESIAN_POINT('',(115.908668694001,4.55,49.3496985131866));
#200922=CARTESIAN_POINT('',(115.96591166787,4.55,49.0552104116569));
#200923=CARTESIAN_POINT('',(115.908668694001,5.05,49.3496985131866));
#200924=CARTESIAN_POINT('',(115.96591166787,5.05,49.0552104116569));
#200925=CARTESIAN_POINT('Origin',(115.96591166787,4.55,49.0552104116569));
#200926=CARTESIAN_POINT('',(115.475098165321,4.55,48.9598054552076));
#200927=CARTESIAN_POINT('',(115.417855191451,4.55,49.2542935567373));
#200928=CARTESIAN_POINT('',(115.475098165321,4.55,48.9598054552076));
#200929=CARTESIAN_POINT('',(115.908668694001,4.55,49.3496985131866));
#200930=CARTESIAN_POINT('',(115.96591166787,4.55,49.0552104116569));
#200931=CARTESIAN_POINT('Origin',(115.475098165321,4.55,48.9598054552076));
#200932=CARTESIAN_POINT('',(115.417855191451,4.55,49.2542935567373));
#200933=CARTESIAN_POINT('',(115.475098165321,4.55,48.9598054552076));
#200934=CARTESIAN_POINT('Origin',(114.689796561242,5.05,48.8071575248888));
#200935=CARTESIAN_POINT('',(115.180610063791,5.05,48.9025624813381));
#200936=CARTESIAN_POINT('',(115.123367089922,5.05,49.1970505828678));
#200937=CARTESIAN_POINT('',(115.180610063791,5.05,48.9025624813381));
#200938=CARTESIAN_POINT('',(114.632553587372,5.05,49.1016456264185));
#200939=CARTESIAN_POINT('',(114.632553587372,5.05,49.1016456264185));
#200940=CARTESIAN_POINT('',(114.689796561242,5.05,48.8071575248888));
#200941=CARTESIAN_POINT('',(114.689796561242,5.05,48.8071575248888));
#200942=CARTESIAN_POINT('',(114.689796561242,5.05,48.8071575248888));
#200943=CARTESIAN_POINT('Origin',(115.180610063791,5.05,48.9025624813381));
#200944=CARTESIAN_POINT('',(115.180610063791,4.55,48.9025624813381));
#200945=CARTESIAN_POINT('',(115.123367089922,4.55,49.1970505828678));
#200946=CARTESIAN_POINT('',(115.180610063791,4.55,48.9025624813381));
#200947=CARTESIAN_POINT('',(115.123367089922,5.05,49.1970505828678));
#200948=CARTESIAN_POINT('',(115.180610063791,5.05,48.9025624813381));
#200949=CARTESIAN_POINT('Origin',(115.180610063791,4.55,48.9025624813381));
#200950=CARTESIAN_POINT('',(114.689796561242,4.55,48.8071575248888));
#200951=CARTESIAN_POINT('',(114.632553587372,4.55,49.1016456264185));
#200952=CARTESIAN_POINT('',(114.689796561242,4.55,48.8071575248888));
#200953=CARTESIAN_POINT('',(115.123367089922,4.55,49.1970505828678));
#200954=CARTESIAN_POINT('',(115.180610063791,4.55,48.9025624813381));
#200955=CARTESIAN_POINT('Origin',(114.689796561242,4.55,48.8071575248888));
#200956=CARTESIAN_POINT('',(114.632553587372,4.55,49.1016456264185));
#200957=CARTESIAN_POINT('',(114.689796561242,4.55,48.8071575248888));
#200958=CARTESIAN_POINT('Origin',(113.904494957163,5.05,48.65450959457));
#200959=CARTESIAN_POINT('',(114.395308459712,5.05,48.7499145510193));
#200960=CARTESIAN_POINT('',(114.338065485842,5.05,49.044402652549));
#200961=CARTESIAN_POINT('',(114.395308459712,5.05,48.7499145510193));
#200962=CARTESIAN_POINT('',(113.847251983293,5.05,48.9489976960997));
#200963=CARTESIAN_POINT('',(113.847251983293,5.05,48.9489976960997));
#200964=CARTESIAN_POINT('',(113.904494957163,5.05,48.65450959457));
#200965=CARTESIAN_POINT('',(113.904494957163,5.05,48.65450959457));
#200966=CARTESIAN_POINT('',(113.904494957163,5.05,48.65450959457));
#200967=CARTESIAN_POINT('Origin',(114.395308459712,5.05,48.7499145510193));
#200968=CARTESIAN_POINT('',(114.395308459712,4.55,48.7499145510193));
#200969=CARTESIAN_POINT('',(114.338065485842,4.55,49.044402652549));
#200970=CARTESIAN_POINT('',(114.395308459712,4.55,48.7499145510193));
#200971=CARTESIAN_POINT('',(114.338065485842,5.05,49.044402652549));
#200972=CARTESIAN_POINT('',(114.395308459712,5.05,48.7499145510193));
#200973=CARTESIAN_POINT('Origin',(114.395308459712,4.55,48.7499145510193));
#200974=CARTESIAN_POINT('',(113.904494957163,4.55,48.65450959457));
#200975=CARTESIAN_POINT('',(113.847251983293,4.55,48.9489976960997));
#200976=CARTESIAN_POINT('',(113.904494957163,4.55,48.65450959457));
#200977=CARTESIAN_POINT('',(114.338065485842,4.55,49.044402652549));
#200978=CARTESIAN_POINT('',(114.395308459712,4.55,48.7499145510193));
#200979=CARTESIAN_POINT('Origin',(113.904494957163,4.55,48.65450959457));
#200980=CARTESIAN_POINT('',(113.847251983293,4.55,48.9489976960997));
#200981=CARTESIAN_POINT('',(113.904494957163,4.55,48.65450959457));
#200982=CARTESIAN_POINT('Origin',(113.119193353083,5.05,48.5018616642512));
#200983=CARTESIAN_POINT('',(113.610006855633,5.05,48.5972666207005));
#200984=CARTESIAN_POINT('',(113.552763881763,5.05,48.8917547222302));
#200985=CARTESIAN_POINT('',(113.610006855633,5.05,48.5972666207005));
#200986=CARTESIAN_POINT('',(113.061950379214,5.05,48.7963497657809));
#200987=CARTESIAN_POINT('',(113.061950379214,5.05,48.7963497657809));
#200988=CARTESIAN_POINT('',(113.119193353083,5.05,48.5018616642512));
#200989=CARTESIAN_POINT('',(113.119193353083,5.05,48.5018616642512));
#200990=CARTESIAN_POINT('',(113.119193353083,5.05,48.5018616642512));
#200991=CARTESIAN_POINT('Origin',(113.610006855633,5.05,48.5972666207005));
#200992=CARTESIAN_POINT('',(113.610006855633,4.55,48.5972666207005));
#200993=CARTESIAN_POINT('',(113.552763881763,4.55,48.8917547222302));
#200994=CARTESIAN_POINT('',(113.610006855633,4.55,48.5972666207005));
#200995=CARTESIAN_POINT('',(113.552763881763,5.05,48.8917547222302));
#200996=CARTESIAN_POINT('',(113.610006855633,5.05,48.5972666207005));
#200997=CARTESIAN_POINT('Origin',(113.610006855633,4.55,48.5972666207005));
#200998=CARTESIAN_POINT('',(113.119193353083,4.55,48.5018616642512));
#200999=CARTESIAN_POINT('',(113.061950379214,4.55,48.7963497657809));
#201000=CARTESIAN_POINT('',(113.119193353083,4.55,48.5018616642512));
#201001=CARTESIAN_POINT('',(113.552763881763,4.55,48.8917547222302));
#201002=CARTESIAN_POINT('',(113.610006855633,4.55,48.5972666207005));
#201003=CARTESIAN_POINT('Origin',(113.119193353083,4.55,48.5018616642512));
#201004=CARTESIAN_POINT('',(113.061950379214,4.55,48.7963497657809));
#201005=CARTESIAN_POINT('',(113.119193353083,4.55,48.5018616642512));
#201006=CARTESIAN_POINT('Origin',(113.119193353083,4.25,48.5018616642512));
#201007=CARTESIAN_POINT('',(113.610006855633,4.25,48.5972666207005));
#201008=CARTESIAN_POINT('',(113.552763881763,4.25,48.8917547222302));
#201009=CARTESIAN_POINT('',(113.610006855633,4.25,48.5972666207005));
#201010=CARTESIAN_POINT('',(113.061950379214,4.25,48.7963497657809));
#201011=CARTESIAN_POINT('',(113.061950379214,4.25,48.7963497657809));
#201012=CARTESIAN_POINT('',(113.119193353083,4.25,48.5018616642512));
#201013=CARTESIAN_POINT('',(113.119193353083,4.25,48.5018616642512));
#201014=CARTESIAN_POINT('',(113.119193353083,4.25,48.5018616642512));
#201015=CARTESIAN_POINT('Origin',(113.610006855633,4.25,48.5972666207005));
#201016=CARTESIAN_POINT('',(113.610006855633,3.75,48.5972666207005));
#201017=CARTESIAN_POINT('',(113.552763881763,3.75,48.8917547222302));
#201018=CARTESIAN_POINT('',(113.610006855633,3.75,48.5972666207005));
#201019=CARTESIAN_POINT('',(113.552763881763,4.25,48.8917547222302));
#201020=CARTESIAN_POINT('',(113.610006855633,4.25,48.5972666207005));
#201021=CARTESIAN_POINT('Origin',(113.610006855633,3.75,48.5972666207005));
#201022=CARTESIAN_POINT('',(113.119193353083,3.75,48.5018616642512));
#201023=CARTESIAN_POINT('',(113.061950379214,3.75,48.7963497657809));
#201024=CARTESIAN_POINT('',(113.119193353083,3.75,48.5018616642512));
#201025=CARTESIAN_POINT('',(113.552763881763,3.75,48.8917547222302));
#201026=CARTESIAN_POINT('',(113.610006855633,3.75,48.5972666207005));
#201027=CARTESIAN_POINT('Origin',(113.119193353083,3.75,48.5018616642512));
#201028=CARTESIAN_POINT('',(113.061950379214,3.75,48.7963497657809));
#201029=CARTESIAN_POINT('',(113.119193353083,3.75,48.5018616642512));
#201030=CARTESIAN_POINT('Origin',(113.119193353083,3.45,48.5018616642512));
#201031=CARTESIAN_POINT('',(113.610006855633,3.45,48.5972666207005));
#201032=CARTESIAN_POINT('',(113.552763881763,3.45,48.8917547222302));
#201033=CARTESIAN_POINT('',(113.610006855633,3.45,48.5972666207005));
#201034=CARTESIAN_POINT('',(113.061950379214,3.45,48.7963497657809));
#201035=CARTESIAN_POINT('',(113.061950379214,3.45,48.7963497657809));
#201036=CARTESIAN_POINT('',(113.119193353083,3.45,48.5018616642512));
#201037=CARTESIAN_POINT('',(113.119193353083,3.45,48.5018616642512));
#201038=CARTESIAN_POINT('',(113.119193353083,3.45,48.5018616642512));
#201039=CARTESIAN_POINT('Origin',(113.610006855633,3.45,48.5972666207005));
#201040=CARTESIAN_POINT('',(113.610006855633,2.95,48.5972666207005));
#201041=CARTESIAN_POINT('',(113.552763881763,2.95,48.8917547222302));
#201042=CARTESIAN_POINT('',(113.610006855633,2.95,48.5972666207005));
#201043=CARTESIAN_POINT('',(113.552763881763,3.45,48.8917547222302));
#201044=CARTESIAN_POINT('',(113.610006855633,3.45,48.5972666207005));
#201045=CARTESIAN_POINT('Origin',(113.610006855633,2.95,48.5972666207005));
#201046=CARTESIAN_POINT('',(113.119193353083,2.95,48.5018616642512));
#201047=CARTESIAN_POINT('',(113.061950379214,2.95,48.7963497657809));
#201048=CARTESIAN_POINT('',(113.119193353083,2.95,48.5018616642512));
#201049=CARTESIAN_POINT('',(113.552763881763,2.95,48.8917547222302));
#201050=CARTESIAN_POINT('',(113.610006855633,2.95,48.5972666207005));
#201051=CARTESIAN_POINT('Origin',(113.119193353083,2.95,48.5018616642512));
#201052=CARTESIAN_POINT('',(113.061950379214,2.95,48.7963497657809));
#201053=CARTESIAN_POINT('',(113.119193353083,2.95,48.5018616642512));
#201054=CARTESIAN_POINT('Origin',(113.119193353083,2.65,48.5018616642512));
#201055=CARTESIAN_POINT('',(113.610006855633,2.65,48.5972666207005));
#201056=CARTESIAN_POINT('',(113.552763881763,2.65,48.8917547222302));
#201057=CARTESIAN_POINT('',(113.610006855633,2.65,48.5972666207005));
#201058=CARTESIAN_POINT('',(113.061950379214,2.65,48.7963497657809));
#201059=CARTESIAN_POINT('',(113.061950379214,2.65,48.7963497657809));
#201060=CARTESIAN_POINT('',(113.119193353083,2.65,48.5018616642512));
#201061=CARTESIAN_POINT('',(113.119193353083,2.65,48.5018616642512));
#201062=CARTESIAN_POINT('',(113.119193353083,2.65,48.5018616642512));
#201063=CARTESIAN_POINT('Origin',(113.610006855633,2.65,48.5972666207005));
#201064=CARTESIAN_POINT('',(113.610006855633,2.15,48.5972666207005));
#201065=CARTESIAN_POINT('',(113.552763881763,2.15,48.8917547222302));
#201066=CARTESIAN_POINT('',(113.610006855633,2.15,48.5972666207005));
#201067=CARTESIAN_POINT('',(113.552763881763,2.65,48.8917547222302));
#201068=CARTESIAN_POINT('',(113.610006855633,2.65,48.5972666207005));
#201069=CARTESIAN_POINT('Origin',(113.610006855633,2.15,48.5972666207005));
#201070=CARTESIAN_POINT('',(113.119193353083,2.15,48.5018616642512));
#201071=CARTESIAN_POINT('',(113.061950379214,2.15,48.7963497657809));
#201072=CARTESIAN_POINT('',(113.119193353083,2.15,48.5018616642512));
#201073=CARTESIAN_POINT('',(113.552763881763,2.15,48.8917547222302));
#201074=CARTESIAN_POINT('',(113.610006855633,2.15,48.5972666207005));
#201075=CARTESIAN_POINT('Origin',(113.119193353083,2.15,48.5018616642512));
#201076=CARTESIAN_POINT('',(113.061950379214,2.15,48.7963497657809));
#201077=CARTESIAN_POINT('',(113.119193353083,2.15,48.5018616642512));
#201078=CARTESIAN_POINT('Origin',(113.119193353083,1.85,48.5018616642512));
#201079=CARTESIAN_POINT('',(113.610006855633,1.85,48.5972666207005));
#201080=CARTESIAN_POINT('',(113.552763881763,1.85,48.8917547222302));
#201081=CARTESIAN_POINT('',(113.610006855633,1.85,48.5972666207005));
#201082=CARTESIAN_POINT('',(113.061950379214,1.85,48.7963497657809));
#201083=CARTESIAN_POINT('',(113.061950379214,1.85,48.7963497657809));
#201084=CARTESIAN_POINT('',(113.119193353083,1.85,48.5018616642512));
#201085=CARTESIAN_POINT('',(113.119193353083,1.85,48.5018616642512));
#201086=CARTESIAN_POINT('',(113.119193353083,1.85,48.5018616642512));
#201087=CARTESIAN_POINT('Origin',(113.610006855633,1.85,48.5972666207005));
#201088=CARTESIAN_POINT('',(113.610006855633,1.35,48.5972666207005));
#201089=CARTESIAN_POINT('',(113.552763881763,1.35,48.8917547222302));
#201090=CARTESIAN_POINT('',(113.610006855633,1.35,48.5972666207005));
#201091=CARTESIAN_POINT('',(113.552763881763,1.85,48.8917547222302));
#201092=CARTESIAN_POINT('',(113.610006855633,1.85,48.5972666207005));
#201093=CARTESIAN_POINT('Origin',(113.610006855633,1.35,48.5972666207005));
#201094=CARTESIAN_POINT('',(113.119193353083,1.35,48.5018616642512));
#201095=CARTESIAN_POINT('',(113.061950379214,1.35,48.7963497657809));
#201096=CARTESIAN_POINT('',(113.119193353083,1.35,48.5018616642512));
#201097=CARTESIAN_POINT('',(113.552763881763,1.35,48.8917547222302));
#201098=CARTESIAN_POINT('',(113.610006855633,1.35,48.5972666207005));
#201099=CARTESIAN_POINT('Origin',(113.119193353083,1.35,48.5018616642512));
#201100=CARTESIAN_POINT('',(113.061950379214,1.35,48.7963497657809));
#201101=CARTESIAN_POINT('',(113.119193353083,1.35,48.5018616642512));
#201102=CARTESIAN_POINT('Origin',(113.119193353083,1.05,48.5018616642512));
#201103=CARTESIAN_POINT('',(113.610006855633,1.05,48.5972666207005));
#201104=CARTESIAN_POINT('',(113.552763881763,1.05,48.8917547222302));
#201105=CARTESIAN_POINT('',(113.610006855633,1.05,48.5972666207005));
#201106=CARTESIAN_POINT('',(113.061950379214,1.05,48.7963497657809));
#201107=CARTESIAN_POINT('',(113.061950379214,1.05,48.7963497657809));
#201108=CARTESIAN_POINT('',(113.119193353083,1.05,48.5018616642512));
#201109=CARTESIAN_POINT('',(113.119193353083,1.05,48.5018616642512));
#201110=CARTESIAN_POINT('',(113.119193353083,1.05,48.5018616642512));
#201111=CARTESIAN_POINT('Origin',(113.610006855633,1.05,48.5972666207005));
#201112=CARTESIAN_POINT('',(113.610006855633,0.550000000000015,48.5972666207005));
#201113=CARTESIAN_POINT('',(113.552763881763,0.550000000000015,48.8917547222302));
#201114=CARTESIAN_POINT('',(113.610006855633,0.550000000000015,48.5972666207005));
#201115=CARTESIAN_POINT('',(113.552763881763,1.05,48.8917547222302));
#201116=CARTESIAN_POINT('',(113.610006855633,1.05,48.5972666207005));
#201117=CARTESIAN_POINT('Origin',(113.610006855633,0.550000000000015,48.5972666207005));
#201118=CARTESIAN_POINT('',(113.119193353083,0.550000000000015,48.5018616642512));
#201119=CARTESIAN_POINT('',(113.061950379214,0.550000000000015,48.7963497657809));
#201120=CARTESIAN_POINT('',(113.119193353083,0.550000000000015,48.5018616642512));
#201121=CARTESIAN_POINT('',(113.552763881763,0.550000000000015,48.8917547222302));
#201122=CARTESIAN_POINT('',(113.610006855633,0.550000000000015,48.5972666207005));
#201123=CARTESIAN_POINT('Origin',(113.119193353083,0.550000000000015,48.5018616642512));
#201124=CARTESIAN_POINT('',(113.061950379214,0.550000000000015,48.7963497657809));
#201125=CARTESIAN_POINT('',(113.119193353083,0.550000000000015,48.5018616642512));
#201126=CARTESIAN_POINT('Origin',(113.119193353083,0.250000000000015,48.5018616642512));
#201127=CARTESIAN_POINT('',(113.610006855633,0.250000000000015,48.5972666207005));
#201128=CARTESIAN_POINT('',(113.552763881763,0.250000000000015,48.8917547222302));
#201129=CARTESIAN_POINT('',(113.610006855633,0.250000000000015,48.5972666207005));
#201130=CARTESIAN_POINT('',(113.061950379214,0.250000000000015,48.7963497657809));
#201131=CARTESIAN_POINT('',(113.061950379214,0.250000000000015,48.7963497657809));
#201132=CARTESIAN_POINT('',(113.119193353083,0.250000000000015,48.5018616642512));
#201133=CARTESIAN_POINT('',(113.119193353083,0.250000000000015,48.5018616642512));
#201134=CARTESIAN_POINT('',(113.119193353083,0.250000000000015,48.5018616642512));
#201135=CARTESIAN_POINT('Origin',(113.610006855633,0.250000000000015,48.5972666207005));
#201136=CARTESIAN_POINT('',(113.610006855633,-0.249999999999985,48.5972666207005));
#201137=CARTESIAN_POINT('',(113.552763881763,-0.249999999999985,48.8917547222302));
#201138=CARTESIAN_POINT('',(113.610006855633,-0.249999999999985,48.5972666207005));
#201139=CARTESIAN_POINT('',(113.552763881763,0.250000000000015,48.8917547222302));
#201140=CARTESIAN_POINT('',(113.610006855633,0.250000000000015,48.5972666207005));
#201141=CARTESIAN_POINT('Origin',(113.610006855633,-0.249999999999985,48.5972666207005));
#201142=CARTESIAN_POINT('',(113.119193353083,-0.249999999999985,48.5018616642512));
#201143=CARTESIAN_POINT('',(113.061950379214,-0.249999999999985,48.7963497657809));
#201144=CARTESIAN_POINT('',(113.119193353083,-0.249999999999985,48.5018616642512));
#201145=CARTESIAN_POINT('',(113.552763881763,-0.249999999999985,48.8917547222302));
#201146=CARTESIAN_POINT('',(113.610006855633,-0.249999999999985,48.5972666207005));
#201147=CARTESIAN_POINT('Origin',(113.119193353083,-0.249999999999985,48.5018616642512));
#201148=CARTESIAN_POINT('',(113.061950379214,-0.249999999999985,48.7963497657809));
#201149=CARTESIAN_POINT('',(113.119193353083,-0.249999999999985,48.5018616642512));
#201150=CARTESIAN_POINT('Origin',(113.119193353083,-0.549999999999986,48.5018616642512));
#201151=CARTESIAN_POINT('',(113.610006855633,-0.549999999999986,48.5972666207005));
#201152=CARTESIAN_POINT('',(113.552763881763,-0.549999999999986,48.8917547222302));
#201153=CARTESIAN_POINT('',(113.610006855633,-0.549999999999986,48.5972666207005));
#201154=CARTESIAN_POINT('',(113.061950379214,-0.549999999999986,48.7963497657809));
#201155=CARTESIAN_POINT('',(113.061950379214,-0.549999999999986,48.7963497657809));
#201156=CARTESIAN_POINT('',(113.119193353083,-0.549999999999986,48.5018616642512));
#201157=CARTESIAN_POINT('',(113.119193353083,-0.549999999999986,48.5018616642512));
#201158=CARTESIAN_POINT('',(113.119193353083,-0.549999999999986,48.5018616642512));
#201159=CARTESIAN_POINT('Origin',(113.610006855633,-0.549999999999986,48.5972666207005));
#201160=CARTESIAN_POINT('',(113.610006855633,-1.05,48.5972666207005));
#201161=CARTESIAN_POINT('',(113.552763881763,-1.05,48.8917547222302));
#201162=CARTESIAN_POINT('',(113.610006855633,-1.05,48.5972666207005));
#201163=CARTESIAN_POINT('',(113.552763881763,-0.549999999999986,48.8917547222302));
#201164=CARTESIAN_POINT('',(113.610006855633,-0.549999999999986,48.5972666207005));
#201165=CARTESIAN_POINT('Origin',(113.610006855633,-1.05,48.5972666207005));
#201166=CARTESIAN_POINT('',(113.119193353083,-1.05,48.5018616642512));
#201167=CARTESIAN_POINT('',(113.061950379214,-1.05,48.7963497657809));
#201168=CARTESIAN_POINT('',(113.119193353083,-1.05,48.5018616642512));
#201169=CARTESIAN_POINT('',(113.552763881763,-1.05,48.8917547222302));
#201170=CARTESIAN_POINT('',(113.610006855633,-1.05,48.5972666207005));
#201171=CARTESIAN_POINT('Origin',(113.119193353083,-1.05,48.5018616642512));
#201172=CARTESIAN_POINT('',(113.061950379214,-1.05,48.7963497657809));
#201173=CARTESIAN_POINT('',(113.119193353083,-1.05,48.5018616642512));
#201174=CARTESIAN_POINT('Origin',(113.119193353083,-1.35,48.5018616642512));
#201175=CARTESIAN_POINT('',(113.610006855633,-1.35,48.5972666207005));
#201176=CARTESIAN_POINT('',(113.552763881763,-1.35,48.8917547222302));
#201177=CARTESIAN_POINT('',(113.610006855633,-1.35,48.5972666207005));
#201178=CARTESIAN_POINT('',(113.061950379214,-1.35,48.7963497657809));
#201179=CARTESIAN_POINT('',(113.061950379214,-1.35,48.7963497657809));
#201180=CARTESIAN_POINT('',(113.119193353083,-1.35,48.5018616642512));
#201181=CARTESIAN_POINT('',(113.119193353083,-1.35,48.5018616642512));
#201182=CARTESIAN_POINT('',(113.119193353083,-1.35,48.5018616642512));
#201183=CARTESIAN_POINT('Origin',(113.610006855633,-1.35,48.5972666207005));
#201184=CARTESIAN_POINT('',(113.610006855633,-1.85,48.5972666207005));
#201185=CARTESIAN_POINT('',(113.552763881763,-1.85,48.8917547222302));
#201186=CARTESIAN_POINT('',(113.610006855633,-1.85,48.5972666207005));
#201187=CARTESIAN_POINT('',(113.552763881763,-1.35,48.8917547222302));
#201188=CARTESIAN_POINT('',(113.610006855633,-1.35,48.5972666207005));
#201189=CARTESIAN_POINT('Origin',(113.610006855633,-1.85,48.5972666207005));
#201190=CARTESIAN_POINT('',(113.119193353083,-1.85,48.5018616642512));
#201191=CARTESIAN_POINT('',(113.061950379214,-1.85,48.7963497657809));
#201192=CARTESIAN_POINT('',(113.119193353083,-1.85,48.5018616642512));
#201193=CARTESIAN_POINT('',(113.552763881763,-1.85,48.8917547222302));
#201194=CARTESIAN_POINT('',(113.610006855633,-1.85,48.5972666207005));
#201195=CARTESIAN_POINT('Origin',(113.119193353083,-1.85,48.5018616642512));
#201196=CARTESIAN_POINT('',(113.061950379214,-1.85,48.7963497657809));
#201197=CARTESIAN_POINT('',(113.119193353083,-1.85,48.5018616642512));
#201198=CARTESIAN_POINT('Origin',(113.119193353083,-2.15,48.5018616642512));
#201199=CARTESIAN_POINT('',(113.610006855633,-2.15,48.5972666207005));
#201200=CARTESIAN_POINT('',(113.552763881763,-2.15,48.8917547222302));
#201201=CARTESIAN_POINT('',(113.610006855633,-2.15,48.5972666207005));
#201202=CARTESIAN_POINT('',(113.061950379214,-2.15,48.7963497657809));
#201203=CARTESIAN_POINT('',(113.061950379214,-2.15,48.7963497657809));
#201204=CARTESIAN_POINT('',(113.119193353083,-2.15,48.5018616642512));
#201205=CARTESIAN_POINT('',(113.119193353083,-2.15,48.5018616642512));
#201206=CARTESIAN_POINT('',(113.119193353083,-2.15,48.5018616642512));
#201207=CARTESIAN_POINT('Origin',(113.610006855633,-2.15,48.5972666207005));
#201208=CARTESIAN_POINT('',(113.610006855633,-2.65,48.5972666207005));
#201209=CARTESIAN_POINT('',(113.552763881763,-2.65,48.8917547222302));
#201210=CARTESIAN_POINT('',(113.610006855633,-2.65,48.5972666207005));
#201211=CARTESIAN_POINT('',(113.552763881763,-2.15,48.8917547222302));
#201212=CARTESIAN_POINT('',(113.610006855633,-2.15,48.5972666207005));
#201213=CARTESIAN_POINT('Origin',(113.610006855633,-2.65,48.5972666207005));
#201214=CARTESIAN_POINT('',(113.119193353083,-2.65,48.5018616642512));
#201215=CARTESIAN_POINT('',(113.061950379214,-2.65,48.7963497657809));
#201216=CARTESIAN_POINT('',(113.119193353083,-2.65,48.5018616642512));
#201217=CARTESIAN_POINT('',(113.552763881763,-2.65,48.8917547222302));
#201218=CARTESIAN_POINT('',(113.610006855633,-2.65,48.5972666207005));
#201219=CARTESIAN_POINT('Origin',(113.119193353083,-2.65,48.5018616642512));
#201220=CARTESIAN_POINT('',(113.061950379214,-2.65,48.7963497657809));
#201221=CARTESIAN_POINT('',(113.119193353083,-2.65,48.5018616642512));
#201222=CARTESIAN_POINT('Origin',(113.119193353083,-2.95,48.5018616642512));
#201223=CARTESIAN_POINT('',(113.610006855633,-2.95,48.5972666207005));
#201224=CARTESIAN_POINT('',(113.552763881763,-2.95,48.8917547222302));
#201225=CARTESIAN_POINT('',(113.610006855633,-2.95,48.5972666207005));
#201226=CARTESIAN_POINT('',(113.061950379214,-2.95,48.7963497657809));
#201227=CARTESIAN_POINT('',(113.061950379214,-2.95,48.7963497657809));
#201228=CARTESIAN_POINT('',(113.119193353083,-2.95,48.5018616642512));
#201229=CARTESIAN_POINT('',(113.119193353083,-2.95,48.5018616642512));
#201230=CARTESIAN_POINT('',(113.119193353083,-2.95,48.5018616642512));
#201231=CARTESIAN_POINT('Origin',(113.610006855633,-2.95,48.5972666207005));
#201232=CARTESIAN_POINT('',(113.610006855633,-3.45,48.5972666207005));
#201233=CARTESIAN_POINT('',(113.552763881763,-3.45,48.8917547222302));
#201234=CARTESIAN_POINT('',(113.610006855633,-3.45,48.5972666207005));
#201235=CARTESIAN_POINT('',(113.552763881763,-2.95,48.8917547222302));
#201236=CARTESIAN_POINT('',(113.610006855633,-2.95,48.5972666207005));
#201237=CARTESIAN_POINT('Origin',(113.610006855633,-3.45,48.5972666207005));
#201238=CARTESIAN_POINT('',(113.119193353083,-3.45,48.5018616642512));
#201239=CARTESIAN_POINT('',(113.061950379214,-3.45,48.7963497657809));
#201240=CARTESIAN_POINT('',(113.119193353083,-3.45,48.5018616642512));
#201241=CARTESIAN_POINT('',(113.552763881763,-3.45,48.8917547222302));
#201242=CARTESIAN_POINT('',(113.610006855633,-3.45,48.5972666207005));
#201243=CARTESIAN_POINT('Origin',(113.119193353083,-3.45,48.5018616642512));
#201244=CARTESIAN_POINT('',(113.061950379214,-3.45,48.7963497657809));
#201245=CARTESIAN_POINT('',(113.119193353083,-3.45,48.5018616642512));
#201246=CARTESIAN_POINT('Origin',(113.119193353083,-3.75,48.5018616642512));
#201247=CARTESIAN_POINT('',(113.610006855633,-3.75,48.5972666207005));
#201248=CARTESIAN_POINT('',(113.552763881763,-3.75,48.8917547222302));
#201249=CARTESIAN_POINT('',(113.610006855633,-3.75,48.5972666207005));
#201250=CARTESIAN_POINT('',(113.061950379214,-3.75,48.7963497657809));
#201251=CARTESIAN_POINT('',(113.061950379214,-3.75,48.7963497657809));
#201252=CARTESIAN_POINT('',(113.119193353083,-3.75,48.5018616642512));
#201253=CARTESIAN_POINT('',(113.119193353083,-3.75,48.5018616642512));
#201254=CARTESIAN_POINT('',(113.119193353083,-3.75,48.5018616642512));
#201255=CARTESIAN_POINT('Origin',(113.610006855633,-3.75,48.5972666207005));
#201256=CARTESIAN_POINT('',(113.610006855633,-4.25,48.5972666207005));
#201257=CARTESIAN_POINT('',(113.552763881763,-4.25,48.8917547222302));
#201258=CARTESIAN_POINT('',(113.610006855633,-4.25,48.5972666207005));
#201259=CARTESIAN_POINT('',(113.552763881763,-3.75,48.8917547222302));
#201260=CARTESIAN_POINT('',(113.610006855633,-3.75,48.5972666207005));
#201261=CARTESIAN_POINT('Origin',(113.610006855633,-4.25,48.5972666207005));
#201262=CARTESIAN_POINT('',(113.119193353083,-4.25,48.5018616642512));
#201263=CARTESIAN_POINT('',(113.061950379214,-4.25,48.7963497657809));
#201264=CARTESIAN_POINT('',(113.119193353083,-4.25,48.5018616642512));
#201265=CARTESIAN_POINT('',(113.552763881763,-4.25,48.8917547222302));
#201266=CARTESIAN_POINT('',(113.610006855633,-4.25,48.5972666207005));
#201267=CARTESIAN_POINT('Origin',(113.119193353083,-4.25,48.5018616642512));
#201268=CARTESIAN_POINT('',(113.061950379214,-4.25,48.7963497657809));
#201269=CARTESIAN_POINT('',(113.119193353083,-4.25,48.5018616642512));
#201270=CARTESIAN_POINT('Origin',(113.904494957163,-3.75,48.65450959457));
#201271=CARTESIAN_POINT('',(114.395308459712,-3.75,48.7499145510193));
#201272=CARTESIAN_POINT('',(114.338065485842,-3.75,49.044402652549));
#201273=CARTESIAN_POINT('',(114.395308459712,-3.75,48.7499145510193));
#201274=CARTESIAN_POINT('',(113.847251983293,-3.75,48.9489976960997));
#201275=CARTESIAN_POINT('',(113.847251983293,-3.75,48.9489976960997));
#201276=CARTESIAN_POINT('',(113.904494957163,-3.75,48.65450959457));
#201277=CARTESIAN_POINT('',(113.904494957163,-3.75,48.65450959457));
#201278=CARTESIAN_POINT('',(113.904494957163,-3.75,48.65450959457));
#201279=CARTESIAN_POINT('Origin',(114.395308459712,-3.75,48.7499145510193));
#201280=CARTESIAN_POINT('',(114.395308459712,-4.25,48.7499145510193));
#201281=CARTESIAN_POINT('',(114.338065485842,-4.25,49.044402652549));
#201282=CARTESIAN_POINT('',(114.395308459712,-4.25,48.7499145510193));
#201283=CARTESIAN_POINT('',(114.338065485842,-3.75,49.044402652549));
#201284=CARTESIAN_POINT('',(114.395308459712,-3.75,48.7499145510193));
#201285=CARTESIAN_POINT('Origin',(114.395308459712,-4.25,48.7499145510193));
#201286=CARTESIAN_POINT('',(113.904494957163,-4.25,48.65450959457));
#201287=CARTESIAN_POINT('',(113.847251983293,-4.25,48.9489976960997));
#201288=CARTESIAN_POINT('',(113.904494957163,-4.25,48.65450959457));
#201289=CARTESIAN_POINT('',(114.338065485842,-4.25,49.044402652549));
#201290=CARTESIAN_POINT('',(114.395308459712,-4.25,48.7499145510193));
#201291=CARTESIAN_POINT('Origin',(113.904494957163,-4.25,48.65450959457));
#201292=CARTESIAN_POINT('',(113.847251983293,-4.25,48.9489976960997));
#201293=CARTESIAN_POINT('',(113.904494957163,-4.25,48.65450959457));
#201294=CARTESIAN_POINT('Origin',(114.689796561242,-3.75,48.8071575248888));
#201295=CARTESIAN_POINT('',(115.180610063791,-3.75,48.9025624813381));
#201296=CARTESIAN_POINT('',(115.123367089922,-3.75,49.1970505828678));
#201297=CARTESIAN_POINT('',(115.180610063791,-3.75,48.9025624813381));
#201298=CARTESIAN_POINT('',(114.632553587372,-3.75,49.1016456264185));
#201299=CARTESIAN_POINT('',(114.632553587372,-3.75,49.1016456264185));
#201300=CARTESIAN_POINT('',(114.689796561242,-3.75,48.8071575248888));
#201301=CARTESIAN_POINT('',(114.689796561242,-3.75,48.8071575248888));
#201302=CARTESIAN_POINT('',(114.689796561242,-3.75,48.8071575248888));
#201303=CARTESIAN_POINT('Origin',(115.180610063791,-3.75,48.9025624813381));
#201304=CARTESIAN_POINT('',(115.180610063791,-4.25,48.9025624813381));
#201305=CARTESIAN_POINT('',(115.123367089922,-4.25,49.1970505828678));
#201306=CARTESIAN_POINT('',(115.180610063791,-4.25,48.9025624813381));
#201307=CARTESIAN_POINT('',(115.123367089922,-3.75,49.1970505828678));
#201308=CARTESIAN_POINT('',(115.180610063791,-3.75,48.9025624813381));
#201309=CARTESIAN_POINT('Origin',(115.180610063791,-4.25,48.9025624813381));
#201310=CARTESIAN_POINT('',(114.689796561242,-4.25,48.8071575248888));
#201311=CARTESIAN_POINT('',(114.632553587372,-4.25,49.1016456264185));
#201312=CARTESIAN_POINT('',(114.689796561242,-4.25,48.8071575248888));
#201313=CARTESIAN_POINT('',(115.123367089922,-4.25,49.1970505828678));
#201314=CARTESIAN_POINT('',(115.180610063791,-4.25,48.9025624813381));
#201315=CARTESIAN_POINT('Origin',(114.689796561242,-4.25,48.8071575248888));
#201316=CARTESIAN_POINT('',(114.632553587372,-4.25,49.1016456264185));
#201317=CARTESIAN_POINT('',(114.689796561242,-4.25,48.8071575248888));
#201318=CARTESIAN_POINT('Origin',(115.475098165321,-3.75,48.9598054552076));
#201319=CARTESIAN_POINT('',(115.96591166787,-3.75,49.0552104116569));
#201320=CARTESIAN_POINT('',(115.908668694001,-3.75,49.3496985131866));
#201321=CARTESIAN_POINT('',(115.96591166787,-3.75,49.0552104116569));
#201322=CARTESIAN_POINT('',(115.417855191451,-3.75,49.2542935567373));
#201323=CARTESIAN_POINT('',(115.417855191451,-3.75,49.2542935567373));
#201324=CARTESIAN_POINT('',(115.475098165321,-3.75,48.9598054552076));
#201325=CARTESIAN_POINT('',(115.475098165321,-3.75,48.9598054552076));
#201326=CARTESIAN_POINT('',(115.475098165321,-3.75,48.9598054552076));
#201327=CARTESIAN_POINT('Origin',(115.96591166787,-3.75,49.0552104116569));
#201328=CARTESIAN_POINT('',(115.96591166787,-4.25,49.0552104116569));
#201329=CARTESIAN_POINT('',(115.908668694001,-4.25,49.3496985131866));
#201330=CARTESIAN_POINT('',(115.96591166787,-4.25,49.0552104116569));
#201331=CARTESIAN_POINT('',(115.908668694001,-3.75,49.3496985131866));
#201332=CARTESIAN_POINT('',(115.96591166787,-3.75,49.0552104116569));
#201333=CARTESIAN_POINT('Origin',(115.96591166787,-4.25,49.0552104116569));
#201334=CARTESIAN_POINT('',(115.475098165321,-4.25,48.9598054552076));
#201335=CARTESIAN_POINT('',(115.417855191451,-4.25,49.2542935567373));
#201336=CARTESIAN_POINT('',(115.475098165321,-4.25,48.9598054552076));
#201337=CARTESIAN_POINT('',(115.908668694001,-4.25,49.3496985131866));
#201338=CARTESIAN_POINT('',(115.96591166787,-4.25,49.0552104116569));
#201339=CARTESIAN_POINT('Origin',(115.475098165321,-4.25,48.9598054552076));
#201340=CARTESIAN_POINT('',(115.417855191451,-4.25,49.2542935567373));
#201341=CARTESIAN_POINT('',(115.475098165321,-4.25,48.9598054552076));
#201342=CARTESIAN_POINT('Origin',(116.2603997694,-3.75,49.1124533855264));
#201343=CARTESIAN_POINT('',(116.75121327195,-3.75,49.2078583419757));
#201344=CARTESIAN_POINT('',(116.69397029808,-3.75,49.5023464435054));
#201345=CARTESIAN_POINT('',(116.75121327195,-3.75,49.2078583419757));
#201346=CARTESIAN_POINT('',(116.203156795531,-3.75,49.4069414870561));
#201347=CARTESIAN_POINT('',(116.203156795531,-3.75,49.4069414870561));
#201348=CARTESIAN_POINT('',(116.2603997694,-3.75,49.1124533855264));
#201349=CARTESIAN_POINT('',(116.2603997694,-3.75,49.1124533855264));
#201350=CARTESIAN_POINT('',(116.2603997694,-3.75,49.1124533855264));
#201351=CARTESIAN_POINT('Origin',(116.75121327195,-3.75,49.2078583419757));
#201352=CARTESIAN_POINT('',(116.75121327195,-4.25,49.2078583419757));
#201353=CARTESIAN_POINT('',(116.69397029808,-4.25,49.5023464435054));
#201354=CARTESIAN_POINT('',(116.75121327195,-4.25,49.2078583419757));
#201355=CARTESIAN_POINT('',(116.69397029808,-3.75,49.5023464435054));
#201356=CARTESIAN_POINT('',(116.75121327195,-3.75,49.2078583419757));
#201357=CARTESIAN_POINT('Origin',(116.75121327195,-4.25,49.2078583419757));
#201358=CARTESIAN_POINT('',(116.2603997694,-4.25,49.1124533855264));
#201359=CARTESIAN_POINT('',(116.203156795531,-4.25,49.4069414870561));
#201360=CARTESIAN_POINT('',(116.2603997694,-4.25,49.1124533855264));
#201361=CARTESIAN_POINT('',(116.69397029808,-4.25,49.5023464435054));
#201362=CARTESIAN_POINT('',(116.75121327195,-4.25,49.2078583419757));
#201363=CARTESIAN_POINT('Origin',(116.2603997694,-4.25,49.1124533855264));
#201364=CARTESIAN_POINT('',(116.203156795531,-4.25,49.4069414870561));
#201365=CARTESIAN_POINT('',(116.2603997694,-4.25,49.1124533855264));
#201366=CARTESIAN_POINT('Origin',(117.045701373479,-3.75,49.2651013158452));
#201367=CARTESIAN_POINT('',(117.536514876029,-3.75,49.3605062722945));
#201368=CARTESIAN_POINT('',(117.479271902159,-3.75,49.6549943738242));
#201369=CARTESIAN_POINT('',(117.536514876029,-3.75,49.3605062722945));
#201370=CARTESIAN_POINT('',(116.98845839961,-3.75,49.5595894173749));
#201371=CARTESIAN_POINT('',(116.98845839961,-3.75,49.5595894173749));
#201372=CARTESIAN_POINT('',(117.045701373479,-3.75,49.2651013158452));
#201373=CARTESIAN_POINT('',(117.045701373479,-3.75,49.2651013158452));
#201374=CARTESIAN_POINT('',(117.045701373479,-3.75,49.2651013158452));
#201375=CARTESIAN_POINT('Origin',(117.536514876029,-3.75,49.3605062722945));
#201376=CARTESIAN_POINT('',(117.536514876029,-4.25,49.3605062722945));
#201377=CARTESIAN_POINT('',(117.479271902159,-4.25,49.6549943738242));
#201378=CARTESIAN_POINT('',(117.536514876029,-4.25,49.3605062722945));
#201379=CARTESIAN_POINT('',(117.479271902159,-3.75,49.6549943738242));
#201380=CARTESIAN_POINT('',(117.536514876029,-3.75,49.3605062722945));
#201381=CARTESIAN_POINT('Origin',(117.536514876029,-4.25,49.3605062722945));
#201382=CARTESIAN_POINT('',(117.045701373479,-4.25,49.2651013158452));
#201383=CARTESIAN_POINT('',(116.98845839961,-4.25,49.5595894173749));
#201384=CARTESIAN_POINT('',(117.045701373479,-4.25,49.2651013158452));
#201385=CARTESIAN_POINT('',(117.479271902159,-4.25,49.6549943738242));
#201386=CARTESIAN_POINT('',(117.536514876029,-4.25,49.3605062722945));
#201387=CARTESIAN_POINT('Origin',(117.045701373479,-4.25,49.2651013158452));
#201388=CARTESIAN_POINT('',(116.98845839961,-4.25,49.5595894173749));
#201389=CARTESIAN_POINT('',(117.045701373479,-4.25,49.2651013158452));
#201390=CARTESIAN_POINT('Origin',(117.831002977559,-3.75,49.417749246164));
#201391=CARTESIAN_POINT('',(118.321816480108,-3.75,49.5131542026133));
#201392=CARTESIAN_POINT('',(118.264573506239,-3.75,49.807642304143));
#201393=CARTESIAN_POINT('',(118.321816480108,-3.75,49.5131542026133));
#201394=CARTESIAN_POINT('',(117.773760003689,-3.75,49.7122373476937));
#201395=CARTESIAN_POINT('',(117.773760003689,-3.75,49.7122373476937));
#201396=CARTESIAN_POINT('',(117.831002977559,-3.75,49.417749246164));
#201397=CARTESIAN_POINT('',(117.831002977559,-3.75,49.417749246164));
#201398=CARTESIAN_POINT('',(117.831002977559,-3.75,49.417749246164));
#201399=CARTESIAN_POINT('Origin',(118.321816480108,-3.75,49.5131542026133));
#201400=CARTESIAN_POINT('',(118.321816480108,-4.25,49.5131542026133));
#201401=CARTESIAN_POINT('',(118.264573506239,-4.25,49.807642304143));
#201402=CARTESIAN_POINT('',(118.321816480108,-4.25,49.5131542026133));
#201403=CARTESIAN_POINT('',(118.264573506239,-3.75,49.807642304143));
#201404=CARTESIAN_POINT('',(118.321816480108,-3.75,49.5131542026133));
#201405=CARTESIAN_POINT('Origin',(118.321816480108,-4.25,49.5131542026133));
#201406=CARTESIAN_POINT('',(117.831002977559,-4.25,49.417749246164));
#201407=CARTESIAN_POINT('',(117.773760003689,-4.25,49.7122373476937));
#201408=CARTESIAN_POINT('',(117.831002977559,-4.25,49.417749246164));
#201409=CARTESIAN_POINT('',(118.264573506239,-4.25,49.807642304143));
#201410=CARTESIAN_POINT('',(118.321816480108,-4.25,49.5131542026133));
#201411=CARTESIAN_POINT('Origin',(117.831002977559,-4.25,49.417749246164));
#201412=CARTESIAN_POINT('',(117.773760003689,-4.25,49.7122373476937));
#201413=CARTESIAN_POINT('',(117.831002977559,-4.25,49.417749246164));
#201414=CARTESIAN_POINT('Origin',(118.616304581638,-3.75,49.5703971764828));
#201415=CARTESIAN_POINT('',(119.107118084187,-3.75,49.6658021329321));
#201416=CARTESIAN_POINT('',(119.049875110318,-3.75,49.9602902344618));
#201417=CARTESIAN_POINT('',(119.107118084187,-3.75,49.6658021329321));
#201418=CARTESIAN_POINT('',(118.559061607768,-3.75,49.8648852780125));
#201419=CARTESIAN_POINT('',(118.559061607768,-3.75,49.8648852780125));
#201420=CARTESIAN_POINT('',(118.616304581638,-3.75,49.5703971764828));
#201421=CARTESIAN_POINT('',(118.616304581638,-3.75,49.5703971764828));
#201422=CARTESIAN_POINT('',(118.616304581638,-3.75,49.5703971764828));
#201423=CARTESIAN_POINT('Origin',(119.107118084187,-3.75,49.6658021329321));
#201424=CARTESIAN_POINT('',(119.107118084187,-4.25,49.6658021329321));
#201425=CARTESIAN_POINT('',(119.049875110318,-4.25,49.9602902344618));
#201426=CARTESIAN_POINT('',(119.107118084187,-4.25,49.6658021329321));
#201427=CARTESIAN_POINT('',(119.049875110318,-3.75,49.9602902344618));
#201428=CARTESIAN_POINT('',(119.107118084187,-3.75,49.6658021329321));
#201429=CARTESIAN_POINT('Origin',(119.107118084187,-4.25,49.6658021329321));
#201430=CARTESIAN_POINT('',(118.616304581638,-4.25,49.5703971764828));
#201431=CARTESIAN_POINT('',(118.559061607768,-4.25,49.8648852780125));
#201432=CARTESIAN_POINT('',(118.616304581638,-4.25,49.5703971764828));
#201433=CARTESIAN_POINT('',(119.049875110318,-4.25,49.9602902344618));
#201434=CARTESIAN_POINT('',(119.107118084187,-4.25,49.6658021329321));
#201435=CARTESIAN_POINT('Origin',(118.616304581638,-4.25,49.5703971764828));
#201436=CARTESIAN_POINT('',(118.559061607768,-4.25,49.8648852780125));
#201437=CARTESIAN_POINT('',(118.616304581638,-4.25,49.5703971764828));
#201438=CARTESIAN_POINT('Origin',(119.401606185717,-3.75,49.7230451068016));
#201439=CARTESIAN_POINT('',(119.892419688267,-3.75,49.8184500632509));
#201440=CARTESIAN_POINT('',(119.835176714397,-3.75,50.1129381647806));
#201441=CARTESIAN_POINT('',(119.892419688267,-3.75,49.8184500632509));
#201442=CARTESIAN_POINT('',(119.344363211847,-3.75,50.0175332083313));
#201443=CARTESIAN_POINT('',(119.344363211847,-3.75,50.0175332083313));
#201444=CARTESIAN_POINT('',(119.401606185717,-3.75,49.7230451068016));
#201445=CARTESIAN_POINT('',(119.401606185717,-3.75,49.7230451068016));
#201446=CARTESIAN_POINT('',(119.401606185717,-3.75,49.7230451068016));
#201447=CARTESIAN_POINT('Origin',(119.892419688267,-3.75,49.8184500632509));
#201448=CARTESIAN_POINT('',(119.892419688267,-4.25,49.8184500632509));
#201449=CARTESIAN_POINT('',(119.835176714397,-4.25,50.1129381647806));
#201450=CARTESIAN_POINT('',(119.892419688267,-4.25,49.8184500632509));
#201451=CARTESIAN_POINT('',(119.835176714397,-3.75,50.1129381647806));
#201452=CARTESIAN_POINT('',(119.892419688267,-3.75,49.8184500632509));
#201453=CARTESIAN_POINT('Origin',(119.892419688267,-4.25,49.8184500632509));
#201454=CARTESIAN_POINT('',(119.401606185717,-4.25,49.7230451068016));
#201455=CARTESIAN_POINT('',(119.344363211847,-4.25,50.0175332083313));
#201456=CARTESIAN_POINT('',(119.401606185717,-4.25,49.7230451068016));
#201457=CARTESIAN_POINT('',(119.835176714397,-4.25,50.1129381647806));
#201458=CARTESIAN_POINT('',(119.892419688267,-4.25,49.8184500632509));
#201459=CARTESIAN_POINT('Origin',(119.401606185717,-4.25,49.7230451068016));
#201460=CARTESIAN_POINT('',(119.344363211847,-4.25,50.0175332083313));
#201461=CARTESIAN_POINT('',(119.401606185717,-4.25,49.7230451068016));
#201462=CARTESIAN_POINT('Origin',(120.186907789796,-3.75,49.8756930371204));
#201463=CARTESIAN_POINT('',(120.677721292346,-3.75,49.9710979935697));
#201464=CARTESIAN_POINT('',(120.620478318476,-3.75,50.2655860950994));
#201465=CARTESIAN_POINT('',(120.677721292346,-3.75,49.9710979935697));
#201466=CARTESIAN_POINT('',(120.129664815927,-3.75,50.1701811386501));
#201467=CARTESIAN_POINT('',(120.129664815927,-3.75,50.1701811386501));
#201468=CARTESIAN_POINT('',(120.186907789796,-3.75,49.8756930371204));
#201469=CARTESIAN_POINT('',(120.186907789796,-3.75,49.8756930371204));
#201470=CARTESIAN_POINT('',(120.186907789796,-3.75,49.8756930371204));
#201471=CARTESIAN_POINT('Origin',(120.677721292346,-3.75,49.9710979935697));
#201472=CARTESIAN_POINT('',(120.677721292346,-4.25,49.9710979935697));
#201473=CARTESIAN_POINT('',(120.620478318476,-4.25,50.2655860950994));
#201474=CARTESIAN_POINT('',(120.677721292346,-4.25,49.9710979935697));
#201475=CARTESIAN_POINT('',(120.620478318476,-3.75,50.2655860950994));
#201476=CARTESIAN_POINT('',(120.677721292346,-3.75,49.9710979935697));
#201477=CARTESIAN_POINT('Origin',(120.677721292346,-4.25,49.9710979935697));
#201478=CARTESIAN_POINT('',(120.186907789796,-4.25,49.8756930371204));
#201479=CARTESIAN_POINT('',(120.129664815927,-4.25,50.1701811386501));
#201480=CARTESIAN_POINT('',(120.186907789796,-4.25,49.8756930371204));
#201481=CARTESIAN_POINT('',(120.620478318476,-4.25,50.2655860950994));
#201482=CARTESIAN_POINT('',(120.677721292346,-4.25,49.9710979935697));
#201483=CARTESIAN_POINT('Origin',(120.186907789796,-4.25,49.8756930371204));
#201484=CARTESIAN_POINT('',(120.129664815927,-4.25,50.1701811386501));
#201485=CARTESIAN_POINT('',(120.186907789796,-4.25,49.8756930371204));
#201486=CARTESIAN_POINT('Origin',(120.972209393875,-3.75,50.0283409674392));
#201487=CARTESIAN_POINT('',(121.463022896425,-3.75,50.1237459238885));
#201488=CARTESIAN_POINT('',(121.405779922555,-3.75,50.4182340254182));
#201489=CARTESIAN_POINT('',(121.463022896425,-3.75,50.1237459238885));
#201490=CARTESIAN_POINT('',(120.914966420006,-3.75,50.3228290689689));
#201491=CARTESIAN_POINT('',(120.914966420006,-3.75,50.3228290689689));
#201492=CARTESIAN_POINT('',(120.972209393875,-3.75,50.0283409674392));
#201493=CARTESIAN_POINT('',(120.972209393875,-3.75,50.0283409674392));
#201494=CARTESIAN_POINT('',(120.972209393875,-3.75,50.0283409674392));
#201495=CARTESIAN_POINT('Origin',(121.463022896425,-3.75,50.1237459238885));
#201496=CARTESIAN_POINT('',(121.463022896425,-4.25,50.1237459238885));
#201497=CARTESIAN_POINT('',(121.405779922555,-4.25,50.4182340254182));
#201498=CARTESIAN_POINT('',(121.463022896425,-4.25,50.1237459238885));
#201499=CARTESIAN_POINT('',(121.405779922555,-3.75,50.4182340254182));
#201500=CARTESIAN_POINT('',(121.463022896425,-3.75,50.1237459238885));
#201501=CARTESIAN_POINT('Origin',(121.463022896425,-4.25,50.1237459238885));
#201502=CARTESIAN_POINT('',(120.972209393875,-4.25,50.0283409674392));
#201503=CARTESIAN_POINT('',(120.914966420006,-4.25,50.3228290689689));
#201504=CARTESIAN_POINT('',(120.972209393875,-4.25,50.0283409674392));
#201505=CARTESIAN_POINT('',(121.405779922555,-4.25,50.4182340254182));
#201506=CARTESIAN_POINT('',(121.463022896425,-4.25,50.1237459238885));
#201507=CARTESIAN_POINT('Origin',(120.972209393875,-4.25,50.0283409674392));
#201508=CARTESIAN_POINT('',(120.914966420006,-4.25,50.3228290689689));
#201509=CARTESIAN_POINT('',(120.972209393875,-4.25,50.0283409674392));
#201510=CARTESIAN_POINT('Origin',(120.972209393875,-2.95,50.0283409674392));
#201511=CARTESIAN_POINT('',(121.463022896425,-2.95,50.1237459238885));
#201512=CARTESIAN_POINT('',(121.405779922555,-2.95,50.4182340254182));
#201513=CARTESIAN_POINT('',(121.463022896425,-2.95,50.1237459238885));
#201514=CARTESIAN_POINT('',(120.914966420006,-2.95,50.3228290689689));
#201515=CARTESIAN_POINT('',(120.914966420006,-2.95,50.3228290689689));
#201516=CARTESIAN_POINT('',(120.972209393875,-2.95,50.0283409674392));
#201517=CARTESIAN_POINT('',(120.972209393875,-2.95,50.0283409674392));
#201518=CARTESIAN_POINT('',(120.972209393875,-2.95,50.0283409674392));
#201519=CARTESIAN_POINT('Origin',(121.463022896425,-2.95,50.1237459238885));
#201520=CARTESIAN_POINT('',(121.463022896425,-3.45,50.1237459238885));
#201521=CARTESIAN_POINT('',(121.405779922555,-3.45,50.4182340254182));
#201522=CARTESIAN_POINT('',(121.463022896425,-3.45,50.1237459238885));
#201523=CARTESIAN_POINT('',(121.405779922555,-2.95,50.4182340254182));
#201524=CARTESIAN_POINT('',(121.463022896425,-2.95,50.1237459238885));
#201525=CARTESIAN_POINT('Origin',(121.463022896425,-3.45,50.1237459238885));
#201526=CARTESIAN_POINT('',(120.972209393875,-3.45,50.0283409674392));
#201527=CARTESIAN_POINT('',(120.914966420006,-3.45,50.3228290689689));
#201528=CARTESIAN_POINT('',(120.972209393875,-3.45,50.0283409674392));
#201529=CARTESIAN_POINT('',(121.405779922555,-3.45,50.4182340254182));
#201530=CARTESIAN_POINT('',(121.463022896425,-3.45,50.1237459238885));
#201531=CARTESIAN_POINT('Origin',(120.972209393875,-3.45,50.0283409674392));
#201532=CARTESIAN_POINT('',(120.914966420006,-3.45,50.3228290689689));
#201533=CARTESIAN_POINT('',(120.972209393875,-3.45,50.0283409674392));
#201534=CARTESIAN_POINT('Origin',(120.972209393875,-2.15,50.0283409674392));
#201535=CARTESIAN_POINT('',(121.463022896425,-2.15,50.1237459238885));
#201536=CARTESIAN_POINT('',(121.405779922555,-2.15,50.4182340254182));
#201537=CARTESIAN_POINT('',(121.463022896425,-2.15,50.1237459238885));
#201538=CARTESIAN_POINT('',(120.914966420006,-2.15,50.3228290689689));
#201539=CARTESIAN_POINT('',(120.914966420006,-2.15,50.3228290689689));
#201540=CARTESIAN_POINT('',(120.972209393875,-2.15,50.0283409674392));
#201541=CARTESIAN_POINT('',(120.972209393875,-2.15,50.0283409674392));
#201542=CARTESIAN_POINT('',(120.972209393875,-2.15,50.0283409674392));
#201543=CARTESIAN_POINT('Origin',(121.463022896425,-2.15,50.1237459238885));
#201544=CARTESIAN_POINT('',(121.463022896425,-2.65,50.1237459238885));
#201545=CARTESIAN_POINT('',(121.405779922555,-2.65,50.4182340254182));
#201546=CARTESIAN_POINT('',(121.463022896425,-2.65,50.1237459238885));
#201547=CARTESIAN_POINT('',(121.405779922555,-2.15,50.4182340254182));
#201548=CARTESIAN_POINT('',(121.463022896425,-2.15,50.1237459238885));
#201549=CARTESIAN_POINT('Origin',(121.463022896425,-2.65,50.1237459238885));
#201550=CARTESIAN_POINT('',(120.972209393875,-2.65,50.0283409674392));
#201551=CARTESIAN_POINT('',(120.914966420006,-2.65,50.3228290689689));
#201552=CARTESIAN_POINT('',(120.972209393875,-2.65,50.0283409674392));
#201553=CARTESIAN_POINT('',(121.405779922555,-2.65,50.4182340254182));
#201554=CARTESIAN_POINT('',(121.463022896425,-2.65,50.1237459238885));
#201555=CARTESIAN_POINT('Origin',(120.972209393875,-2.65,50.0283409674392));
#201556=CARTESIAN_POINT('',(120.914966420006,-2.65,50.3228290689689));
#201557=CARTESIAN_POINT('',(120.972209393875,-2.65,50.0283409674392));
#201558=CARTESIAN_POINT('Origin',(120.972209393875,-1.35,50.0283409674392));
#201559=CARTESIAN_POINT('',(121.463022896425,-1.35,50.1237459238885));
#201560=CARTESIAN_POINT('',(121.405779922555,-1.35,50.4182340254182));
#201561=CARTESIAN_POINT('',(121.463022896425,-1.35,50.1237459238885));
#201562=CARTESIAN_POINT('',(120.914966420006,-1.35,50.3228290689689));
#201563=CARTESIAN_POINT('',(120.914966420006,-1.35,50.3228290689689));
#201564=CARTESIAN_POINT('',(120.972209393875,-1.35,50.0283409674392));
#201565=CARTESIAN_POINT('',(120.972209393875,-1.35,50.0283409674392));
#201566=CARTESIAN_POINT('',(120.972209393875,-1.35,50.0283409674392));
#201567=CARTESIAN_POINT('Origin',(121.463022896425,-1.35,50.1237459238885));
#201568=CARTESIAN_POINT('',(121.463022896425,-1.85,50.1237459238885));
#201569=CARTESIAN_POINT('',(121.405779922555,-1.85,50.4182340254182));
#201570=CARTESIAN_POINT('',(121.463022896425,-1.85,50.1237459238885));
#201571=CARTESIAN_POINT('',(121.405779922555,-1.35,50.4182340254182));
#201572=CARTESIAN_POINT('',(121.463022896425,-1.35,50.1237459238885));
#201573=CARTESIAN_POINT('Origin',(121.463022896425,-1.85,50.1237459238885));
#201574=CARTESIAN_POINT('',(120.972209393875,-1.85,50.0283409674392));
#201575=CARTESIAN_POINT('',(120.914966420006,-1.85,50.3228290689689));
#201576=CARTESIAN_POINT('',(120.972209393875,-1.85,50.0283409674392));
#201577=CARTESIAN_POINT('',(121.405779922555,-1.85,50.4182340254182));
#201578=CARTESIAN_POINT('',(121.463022896425,-1.85,50.1237459238885));
#201579=CARTESIAN_POINT('Origin',(120.972209393875,-1.85,50.0283409674392));
#201580=CARTESIAN_POINT('',(120.914966420006,-1.85,50.3228290689689));
#201581=CARTESIAN_POINT('',(120.972209393875,-1.85,50.0283409674392));
#201582=CARTESIAN_POINT('Origin',(120.972209393875,-0.549999999999986,50.0283409674392));
#201583=CARTESIAN_POINT('',(121.463022896425,-0.549999999999986,50.1237459238885));
#201584=CARTESIAN_POINT('',(121.405779922555,-0.549999999999986,50.4182340254182));
#201585=CARTESIAN_POINT('',(121.463022896425,-0.549999999999986,50.1237459238885));
#201586=CARTESIAN_POINT('',(120.914966420006,-0.549999999999986,50.3228290689689));
#201587=CARTESIAN_POINT('',(120.914966420006,-0.549999999999986,50.3228290689689));
#201588=CARTESIAN_POINT('',(120.972209393875,-0.549999999999986,50.0283409674392));
#201589=CARTESIAN_POINT('',(120.972209393875,-0.549999999999986,50.0283409674392));
#201590=CARTESIAN_POINT('',(120.972209393875,-0.549999999999986,50.0283409674392));
#201591=CARTESIAN_POINT('Origin',(121.463022896425,-0.549999999999986,50.1237459238885));
#201592=CARTESIAN_POINT('',(121.463022896425,-1.05,50.1237459238885));
#201593=CARTESIAN_POINT('',(121.405779922555,-1.05,50.4182340254182));
#201594=CARTESIAN_POINT('',(121.463022896425,-1.05,50.1237459238885));
#201595=CARTESIAN_POINT('',(121.405779922555,-0.549999999999986,50.4182340254182));
#201596=CARTESIAN_POINT('',(121.463022896425,-0.549999999999986,50.1237459238885));
#201597=CARTESIAN_POINT('Origin',(121.463022896425,-1.05,50.1237459238885));
#201598=CARTESIAN_POINT('',(120.972209393875,-1.05,50.0283409674392));
#201599=CARTESIAN_POINT('',(120.914966420006,-1.05,50.3228290689689));
#201600=CARTESIAN_POINT('',(120.972209393875,-1.05,50.0283409674392));
#201601=CARTESIAN_POINT('',(121.405779922555,-1.05,50.4182340254182));
#201602=CARTESIAN_POINT('',(121.463022896425,-1.05,50.1237459238885));
#201603=CARTESIAN_POINT('Origin',(120.972209393875,-1.05,50.0283409674392));
#201604=CARTESIAN_POINT('',(120.914966420006,-1.05,50.3228290689689));
#201605=CARTESIAN_POINT('',(120.972209393875,-1.05,50.0283409674392));
#201606=CARTESIAN_POINT('Origin',(120.972209393875,0.250000000000015,50.0283409674392));
#201607=CARTESIAN_POINT('',(121.463022896425,0.250000000000015,50.1237459238885));
#201608=CARTESIAN_POINT('',(121.405779922555,0.250000000000015,50.4182340254182));
#201609=CARTESIAN_POINT('',(121.463022896425,0.250000000000015,50.1237459238885));
#201610=CARTESIAN_POINT('',(120.914966420006,0.250000000000015,50.3228290689689));
#201611=CARTESIAN_POINT('',(120.914966420006,0.250000000000015,50.3228290689689));
#201612=CARTESIAN_POINT('',(120.972209393875,0.250000000000015,50.0283409674392));
#201613=CARTESIAN_POINT('',(120.972209393875,0.250000000000015,50.0283409674392));
#201614=CARTESIAN_POINT('',(120.972209393875,0.250000000000015,50.0283409674392));
#201615=CARTESIAN_POINT('Origin',(121.463022896425,0.250000000000015,50.1237459238885));
#201616=CARTESIAN_POINT('',(121.463022896425,-0.249999999999985,50.1237459238885));
#201617=CARTESIAN_POINT('',(121.405779922555,-0.249999999999985,50.4182340254182));
#201618=CARTESIAN_POINT('',(121.463022896425,-0.249999999999985,50.1237459238885));
#201619=CARTESIAN_POINT('',(121.405779922555,0.250000000000015,50.4182340254182));
#201620=CARTESIAN_POINT('',(121.463022896425,0.250000000000015,50.1237459238885));
#201621=CARTESIAN_POINT('Origin',(121.463022896425,-0.249999999999985,50.1237459238885));
#201622=CARTESIAN_POINT('',(120.972209393875,-0.249999999999985,50.0283409674392));
#201623=CARTESIAN_POINT('',(120.914966420006,-0.249999999999985,50.3228290689689));
#201624=CARTESIAN_POINT('',(120.972209393875,-0.249999999999985,50.0283409674392));
#201625=CARTESIAN_POINT('',(121.405779922555,-0.249999999999985,50.4182340254182));
#201626=CARTESIAN_POINT('',(121.463022896425,-0.249999999999985,50.1237459238885));
#201627=CARTESIAN_POINT('Origin',(120.972209393875,-0.249999999999985,50.0283409674392));
#201628=CARTESIAN_POINT('',(120.914966420006,-0.249999999999985,50.3228290689689));
#201629=CARTESIAN_POINT('',(120.972209393875,-0.249999999999985,50.0283409674392));
#201630=CARTESIAN_POINT('Origin',(120.972209393875,1.05,50.0283409674392));
#201631=CARTESIAN_POINT('',(121.463022896425,1.05,50.1237459238885));
#201632=CARTESIAN_POINT('',(121.405779922555,1.05,50.4182340254182));
#201633=CARTESIAN_POINT('',(121.463022896425,1.05,50.1237459238885));
#201634=CARTESIAN_POINT('',(120.914966420006,1.05,50.3228290689689));
#201635=CARTESIAN_POINT('',(120.914966420006,1.05,50.3228290689689));
#201636=CARTESIAN_POINT('',(120.972209393875,1.05,50.0283409674392));
#201637=CARTESIAN_POINT('',(120.972209393875,1.05,50.0283409674392));
#201638=CARTESIAN_POINT('',(120.972209393875,1.05,50.0283409674392));
#201639=CARTESIAN_POINT('Origin',(121.463022896425,1.05,50.1237459238885));
#201640=CARTESIAN_POINT('',(121.463022896425,0.550000000000015,50.1237459238885));
#201641=CARTESIAN_POINT('',(121.405779922555,0.550000000000015,50.4182340254182));
#201642=CARTESIAN_POINT('',(121.463022896425,0.550000000000015,50.1237459238885));
#201643=CARTESIAN_POINT('',(121.405779922555,1.05,50.4182340254182));
#201644=CARTESIAN_POINT('',(121.463022896425,1.05,50.1237459238885));
#201645=CARTESIAN_POINT('Origin',(121.463022896425,0.550000000000015,50.1237459238885));
#201646=CARTESIAN_POINT('',(120.972209393875,0.550000000000015,50.0283409674392));
#201647=CARTESIAN_POINT('',(120.914966420006,0.550000000000015,50.3228290689689));
#201648=CARTESIAN_POINT('',(120.972209393875,0.550000000000015,50.0283409674392));
#201649=CARTESIAN_POINT('',(121.405779922555,0.550000000000015,50.4182340254182));
#201650=CARTESIAN_POINT('',(121.463022896425,0.550000000000015,50.1237459238885));
#201651=CARTESIAN_POINT('Origin',(120.972209393875,0.550000000000015,50.0283409674392));
#201652=CARTESIAN_POINT('',(120.914966420006,0.550000000000015,50.3228290689689));
#201653=CARTESIAN_POINT('',(120.972209393875,0.550000000000015,50.0283409674392));
#201654=CARTESIAN_POINT('Origin',(120.972209393875,1.85,50.0283409674392));
#201655=CARTESIAN_POINT('',(121.463022896425,1.85,50.1237459238885));
#201656=CARTESIAN_POINT('',(121.405779922555,1.85,50.4182340254182));
#201657=CARTESIAN_POINT('',(121.463022896425,1.85,50.1237459238885));
#201658=CARTESIAN_POINT('',(120.914966420006,1.85,50.3228290689689));
#201659=CARTESIAN_POINT('',(120.914966420006,1.85,50.3228290689689));
#201660=CARTESIAN_POINT('',(120.972209393875,1.85,50.0283409674392));
#201661=CARTESIAN_POINT('',(120.972209393875,1.85,50.0283409674392));
#201662=CARTESIAN_POINT('',(120.972209393875,1.85,50.0283409674392));
#201663=CARTESIAN_POINT('Origin',(121.463022896425,1.85,50.1237459238885));
#201664=CARTESIAN_POINT('',(121.463022896425,1.35,50.1237459238885));
#201665=CARTESIAN_POINT('',(121.405779922555,1.35,50.4182340254182));
#201666=CARTESIAN_POINT('',(121.463022896425,1.35,50.1237459238885));
#201667=CARTESIAN_POINT('',(121.405779922555,1.85,50.4182340254182));
#201668=CARTESIAN_POINT('',(121.463022896425,1.85,50.1237459238885));
#201669=CARTESIAN_POINT('Origin',(121.463022896425,1.35,50.1237459238885));
#201670=CARTESIAN_POINT('',(120.972209393875,1.35,50.0283409674392));
#201671=CARTESIAN_POINT('',(120.914966420006,1.35,50.3228290689689));
#201672=CARTESIAN_POINT('',(120.972209393875,1.35,50.0283409674392));
#201673=CARTESIAN_POINT('',(121.405779922555,1.35,50.4182340254182));
#201674=CARTESIAN_POINT('',(121.463022896425,1.35,50.1237459238885));
#201675=CARTESIAN_POINT('Origin',(120.972209393875,1.35,50.0283409674392));
#201676=CARTESIAN_POINT('',(120.914966420006,1.35,50.3228290689689));
#201677=CARTESIAN_POINT('',(120.972209393875,1.35,50.0283409674392));
#201678=CARTESIAN_POINT('Origin',(120.972209393875,2.65,50.0283409674392));
#201679=CARTESIAN_POINT('',(121.463022896425,2.65,50.1237459238885));
#201680=CARTESIAN_POINT('',(121.405779922555,2.65,50.4182340254182));
#201681=CARTESIAN_POINT('',(121.463022896425,2.65,50.1237459238885));
#201682=CARTESIAN_POINT('',(120.914966420006,2.65,50.3228290689689));
#201683=CARTESIAN_POINT('',(120.914966420006,2.65,50.3228290689689));
#201684=CARTESIAN_POINT('',(120.972209393875,2.65,50.0283409674392));
#201685=CARTESIAN_POINT('',(120.972209393875,2.65,50.0283409674392));
#201686=CARTESIAN_POINT('',(120.972209393875,2.65,50.0283409674392));
#201687=CARTESIAN_POINT('Origin',(121.463022896425,2.65,50.1237459238885));
#201688=CARTESIAN_POINT('',(121.463022896425,2.15,50.1237459238885));
#201689=CARTESIAN_POINT('',(121.405779922555,2.15,50.4182340254182));
#201690=CARTESIAN_POINT('',(121.463022896425,2.15,50.1237459238885));
#201691=CARTESIAN_POINT('',(121.405779922555,2.65,50.4182340254182));
#201692=CARTESIAN_POINT('',(121.463022896425,2.65,50.1237459238885));
#201693=CARTESIAN_POINT('Origin',(121.463022896425,2.15,50.1237459238885));
#201694=CARTESIAN_POINT('',(120.972209393875,2.15,50.0283409674392));
#201695=CARTESIAN_POINT('',(120.914966420006,2.15,50.3228290689689));
#201696=CARTESIAN_POINT('',(120.972209393875,2.15,50.0283409674392));
#201697=CARTESIAN_POINT('',(121.405779922555,2.15,50.4182340254182));
#201698=CARTESIAN_POINT('',(121.463022896425,2.15,50.1237459238885));
#201699=CARTESIAN_POINT('Origin',(120.972209393875,2.15,50.0283409674392));
#201700=CARTESIAN_POINT('',(120.914966420006,2.15,50.3228290689689));
#201701=CARTESIAN_POINT('',(120.972209393875,2.15,50.0283409674392));
#201702=CARTESIAN_POINT('Origin',(120.972209393875,3.45,50.0283409674392));
#201703=CARTESIAN_POINT('',(121.463022896425,3.45,50.1237459238885));
#201704=CARTESIAN_POINT('',(121.405779922555,3.45,50.4182340254182));
#201705=CARTESIAN_POINT('',(121.463022896425,3.45,50.1237459238885));
#201706=CARTESIAN_POINT('',(120.914966420006,3.45,50.3228290689689));
#201707=CARTESIAN_POINT('',(120.914966420006,3.45,50.3228290689689));
#201708=CARTESIAN_POINT('',(120.972209393875,3.45,50.0283409674392));
#201709=CARTESIAN_POINT('',(120.972209393875,3.45,50.0283409674392));
#201710=CARTESIAN_POINT('',(120.972209393875,3.45,50.0283409674392));
#201711=CARTESIAN_POINT('Origin',(121.463022896425,3.45,50.1237459238885));
#201712=CARTESIAN_POINT('',(121.463022896425,2.95,50.1237459238885));
#201713=CARTESIAN_POINT('',(121.405779922555,2.95,50.4182340254182));
#201714=CARTESIAN_POINT('',(121.463022896425,2.95,50.1237459238885));
#201715=CARTESIAN_POINT('',(121.405779922555,3.45,50.4182340254182));
#201716=CARTESIAN_POINT('',(121.463022896425,3.45,50.1237459238885));
#201717=CARTESIAN_POINT('Origin',(121.463022896425,2.95,50.1237459238885));
#201718=CARTESIAN_POINT('',(120.972209393875,2.95,50.0283409674392));
#201719=CARTESIAN_POINT('',(120.914966420006,2.95,50.3228290689689));
#201720=CARTESIAN_POINT('',(120.972209393875,2.95,50.0283409674392));
#201721=CARTESIAN_POINT('',(121.405779922555,2.95,50.4182340254182));
#201722=CARTESIAN_POINT('',(121.463022896425,2.95,50.1237459238885));
#201723=CARTESIAN_POINT('Origin',(120.972209393875,2.95,50.0283409674392));
#201724=CARTESIAN_POINT('',(120.914966420006,2.95,50.3228290689689));
#201725=CARTESIAN_POINT('',(120.972209393875,2.95,50.0283409674392));
#201726=CARTESIAN_POINT('Origin',(120.972209393875,4.25,50.0283409674392));
#201727=CARTESIAN_POINT('',(121.463022896425,4.25,50.1237459238885));
#201728=CARTESIAN_POINT('',(121.405779922555,4.25,50.4182340254182));
#201729=CARTESIAN_POINT('',(121.463022896425,4.25,50.1237459238885));
#201730=CARTESIAN_POINT('',(120.914966420006,4.25,50.3228290689689));
#201731=CARTESIAN_POINT('',(120.914966420006,4.25,50.3228290689689));
#201732=CARTESIAN_POINT('',(120.972209393875,4.25,50.0283409674392));
#201733=CARTESIAN_POINT('',(120.972209393875,4.25,50.0283409674392));
#201734=CARTESIAN_POINT('',(120.972209393875,4.25,50.0283409674392));
#201735=CARTESIAN_POINT('Origin',(121.463022896425,4.25,50.1237459238885));
#201736=CARTESIAN_POINT('',(121.463022896425,3.75,50.1237459238885));
#201737=CARTESIAN_POINT('',(121.405779922555,3.75,50.4182340254182));
#201738=CARTESIAN_POINT('',(121.463022896425,3.75,50.1237459238885));
#201739=CARTESIAN_POINT('',(121.405779922555,4.25,50.4182340254182));
#201740=CARTESIAN_POINT('',(121.463022896425,4.25,50.1237459238885));
#201741=CARTESIAN_POINT('Origin',(121.463022896425,3.75,50.1237459238885));
#201742=CARTESIAN_POINT('',(120.972209393875,3.75,50.0283409674392));
#201743=CARTESIAN_POINT('',(120.914966420006,3.75,50.3228290689689));
#201744=CARTESIAN_POINT('',(120.972209393875,3.75,50.0283409674392));
#201745=CARTESIAN_POINT('',(121.405779922555,3.75,50.4182340254182));
#201746=CARTESIAN_POINT('',(121.463022896425,3.75,50.1237459238885));
#201747=CARTESIAN_POINT('Origin',(120.972209393875,3.75,50.0283409674392));
#201748=CARTESIAN_POINT('',(120.914966420006,3.75,50.3228290689689));
#201749=CARTESIAN_POINT('',(120.972209393875,3.75,50.0283409674392));
#201750=CARTESIAN_POINT('Origin',(120.186907789796,4.25,49.8756930371204));
#201751=CARTESIAN_POINT('',(120.677721292346,4.25,49.9710979935697));
#201752=CARTESIAN_POINT('',(120.620478318476,4.25,50.2655860950994));
#201753=CARTESIAN_POINT('',(120.677721292346,4.25,49.9710979935697));
#201754=CARTESIAN_POINT('',(120.129664815927,4.25,50.1701811386501));
#201755=CARTESIAN_POINT('',(120.129664815927,4.25,50.1701811386501));
#201756=CARTESIAN_POINT('',(120.186907789796,4.25,49.8756930371204));
#201757=CARTESIAN_POINT('',(120.186907789796,4.25,49.8756930371204));
#201758=CARTESIAN_POINT('',(120.186907789796,4.25,49.8756930371204));
#201759=CARTESIAN_POINT('Origin',(120.677721292346,4.25,49.9710979935697));
#201760=CARTESIAN_POINT('',(120.677721292346,3.75,49.9710979935697));
#201761=CARTESIAN_POINT('',(120.620478318476,3.75,50.2655860950994));
#201762=CARTESIAN_POINT('',(120.677721292346,3.75,49.9710979935697));
#201763=CARTESIAN_POINT('',(120.620478318476,4.25,50.2655860950994));
#201764=CARTESIAN_POINT('',(120.677721292346,4.25,49.9710979935697));
#201765=CARTESIAN_POINT('Origin',(120.677721292346,3.75,49.9710979935697));
#201766=CARTESIAN_POINT('',(120.186907789796,3.75,49.8756930371204));
#201767=CARTESIAN_POINT('',(120.129664815927,3.75,50.1701811386501));
#201768=CARTESIAN_POINT('',(120.186907789796,3.75,49.8756930371204));
#201769=CARTESIAN_POINT('',(120.620478318476,3.75,50.2655860950994));
#201770=CARTESIAN_POINT('',(120.677721292346,3.75,49.9710979935697));
#201771=CARTESIAN_POINT('Origin',(120.186907789796,3.75,49.8756930371204));
#201772=CARTESIAN_POINT('',(120.129664815927,3.75,50.1701811386501));
#201773=CARTESIAN_POINT('',(120.186907789796,3.75,49.8756930371204));
#201774=CARTESIAN_POINT('Origin',(119.401606185717,4.25,49.7230451068016));
#201775=CARTESIAN_POINT('',(119.892419688267,4.25,49.8184500632509));
#201776=CARTESIAN_POINT('',(119.835176714397,4.25,50.1129381647806));
#201777=CARTESIAN_POINT('',(119.892419688267,4.25,49.8184500632509));
#201778=CARTESIAN_POINT('',(119.344363211847,4.25,50.0175332083313));
#201779=CARTESIAN_POINT('',(119.344363211847,4.25,50.0175332083313));
#201780=CARTESIAN_POINT('',(119.401606185717,4.25,49.7230451068016));
#201781=CARTESIAN_POINT('',(119.401606185717,4.25,49.7230451068016));
#201782=CARTESIAN_POINT('',(119.401606185717,4.25,49.7230451068016));
#201783=CARTESIAN_POINT('Origin',(119.892419688267,4.25,49.8184500632509));
#201784=CARTESIAN_POINT('',(119.892419688267,3.75,49.8184500632509));
#201785=CARTESIAN_POINT('',(119.835176714397,3.75,50.1129381647806));
#201786=CARTESIAN_POINT('',(119.892419688267,3.75,49.8184500632509));
#201787=CARTESIAN_POINT('',(119.835176714397,4.25,50.1129381647806));
#201788=CARTESIAN_POINT('',(119.892419688267,4.25,49.8184500632509));
#201789=CARTESIAN_POINT('Origin',(119.892419688267,3.75,49.8184500632509));
#201790=CARTESIAN_POINT('',(119.401606185717,3.75,49.7230451068016));
#201791=CARTESIAN_POINT('',(119.344363211847,3.75,50.0175332083313));
#201792=CARTESIAN_POINT('',(119.401606185717,3.75,49.7230451068016));
#201793=CARTESIAN_POINT('',(119.835176714397,3.75,50.1129381647806));
#201794=CARTESIAN_POINT('',(119.892419688267,3.75,49.8184500632509));
#201795=CARTESIAN_POINT('Origin',(119.401606185717,3.75,49.7230451068016));
#201796=CARTESIAN_POINT('',(119.344363211847,3.75,50.0175332083313));
#201797=CARTESIAN_POINT('',(119.401606185717,3.75,49.7230451068016));
#201798=CARTESIAN_POINT('Origin',(118.616304581638,4.25,49.5703971764828));
#201799=CARTESIAN_POINT('',(119.107118084187,4.25,49.6658021329321));
#201800=CARTESIAN_POINT('',(119.049875110318,4.25,49.9602902344618));
#201801=CARTESIAN_POINT('',(119.107118084187,4.25,49.6658021329321));
#201802=CARTESIAN_POINT('',(118.559061607768,4.25,49.8648852780125));
#201803=CARTESIAN_POINT('',(118.559061607768,4.25,49.8648852780125));
#201804=CARTESIAN_POINT('',(118.616304581638,4.25,49.5703971764828));
#201805=CARTESIAN_POINT('',(118.616304581638,4.25,49.5703971764828));
#201806=CARTESIAN_POINT('',(118.616304581638,4.25,49.5703971764828));
#201807=CARTESIAN_POINT('Origin',(119.107118084187,4.25,49.6658021329321));
#201808=CARTESIAN_POINT('',(119.107118084187,3.75,49.6658021329321));
#201809=CARTESIAN_POINT('',(119.049875110318,3.75,49.9602902344618));
#201810=CARTESIAN_POINT('',(119.107118084187,3.75,49.6658021329321));
#201811=CARTESIAN_POINT('',(119.049875110318,4.25,49.9602902344618));
#201812=CARTESIAN_POINT('',(119.107118084187,4.25,49.6658021329321));
#201813=CARTESIAN_POINT('Origin',(119.107118084187,3.75,49.6658021329321));
#201814=CARTESIAN_POINT('',(118.616304581638,3.75,49.5703971764828));
#201815=CARTESIAN_POINT('',(118.559061607768,3.75,49.8648852780125));
#201816=CARTESIAN_POINT('',(118.616304581638,3.75,49.5703971764828));
#201817=CARTESIAN_POINT('',(119.049875110318,3.75,49.9602902344618));
#201818=CARTESIAN_POINT('',(119.107118084187,3.75,49.6658021329321));
#201819=CARTESIAN_POINT('Origin',(118.616304581638,3.75,49.5703971764828));
#201820=CARTESIAN_POINT('',(118.559061607768,3.75,49.8648852780125));
#201821=CARTESIAN_POINT('',(118.616304581638,3.75,49.5703971764828));
#201822=CARTESIAN_POINT('Origin',(117.831002977559,4.25,49.417749246164));
#201823=CARTESIAN_POINT('',(118.321816480108,4.25,49.5131542026133));
#201824=CARTESIAN_POINT('',(118.264573506239,4.25,49.807642304143));
#201825=CARTESIAN_POINT('',(118.321816480108,4.25,49.5131542026133));
#201826=CARTESIAN_POINT('',(117.773760003689,4.25,49.7122373476937));
#201827=CARTESIAN_POINT('',(117.773760003689,4.25,49.7122373476937));
#201828=CARTESIAN_POINT('',(117.831002977559,4.25,49.417749246164));
#201829=CARTESIAN_POINT('',(117.831002977559,4.25,49.417749246164));
#201830=CARTESIAN_POINT('',(117.831002977559,4.25,49.417749246164));
#201831=CARTESIAN_POINT('Origin',(118.321816480108,4.25,49.5131542026133));
#201832=CARTESIAN_POINT('',(118.321816480108,3.75,49.5131542026133));
#201833=CARTESIAN_POINT('',(118.264573506239,3.75,49.807642304143));
#201834=CARTESIAN_POINT('',(118.321816480108,3.75,49.5131542026133));
#201835=CARTESIAN_POINT('',(118.264573506239,4.25,49.807642304143));
#201836=CARTESIAN_POINT('',(118.321816480108,4.25,49.5131542026133));
#201837=CARTESIAN_POINT('Origin',(118.321816480108,3.75,49.5131542026133));
#201838=CARTESIAN_POINT('',(117.831002977559,3.75,49.417749246164));
#201839=CARTESIAN_POINT('',(117.773760003689,3.75,49.7122373476937));
#201840=CARTESIAN_POINT('',(117.831002977559,3.75,49.417749246164));
#201841=CARTESIAN_POINT('',(118.264573506239,3.75,49.807642304143));
#201842=CARTESIAN_POINT('',(118.321816480108,3.75,49.5131542026133));
#201843=CARTESIAN_POINT('Origin',(117.831002977559,3.75,49.417749246164));
#201844=CARTESIAN_POINT('',(117.773760003689,3.75,49.7122373476937));
#201845=CARTESIAN_POINT('',(117.831002977559,3.75,49.417749246164));
#201846=CARTESIAN_POINT('Origin',(117.045701373479,4.25,49.2651013158452));
#201847=CARTESIAN_POINT('',(117.536514876029,4.25,49.3605062722945));
#201848=CARTESIAN_POINT('',(117.479271902159,4.25,49.6549943738242));
#201849=CARTESIAN_POINT('',(117.536514876029,4.25,49.3605062722945));
#201850=CARTESIAN_POINT('',(116.98845839961,4.25,49.5595894173749));
#201851=CARTESIAN_POINT('',(116.98845839961,4.25,49.5595894173749));
#201852=CARTESIAN_POINT('',(117.045701373479,4.25,49.2651013158452));
#201853=CARTESIAN_POINT('',(117.045701373479,4.25,49.2651013158452));
#201854=CARTESIAN_POINT('',(117.045701373479,4.25,49.2651013158452));
#201855=CARTESIAN_POINT('Origin',(117.536514876029,4.25,49.3605062722945));
#201856=CARTESIAN_POINT('',(117.536514876029,3.75,49.3605062722945));
#201857=CARTESIAN_POINT('',(117.479271902159,3.75,49.6549943738242));
#201858=CARTESIAN_POINT('',(117.536514876029,3.75,49.3605062722945));
#201859=CARTESIAN_POINT('',(117.479271902159,4.25,49.6549943738242));
#201860=CARTESIAN_POINT('',(117.536514876029,4.25,49.3605062722945));
#201861=CARTESIAN_POINT('Origin',(117.536514876029,3.75,49.3605062722945));
#201862=CARTESIAN_POINT('',(117.045701373479,3.75,49.2651013158452));
#201863=CARTESIAN_POINT('',(116.98845839961,3.75,49.5595894173749));
#201864=CARTESIAN_POINT('',(117.045701373479,3.75,49.2651013158452));
#201865=CARTESIAN_POINT('',(117.479271902159,3.75,49.6549943738242));
#201866=CARTESIAN_POINT('',(117.536514876029,3.75,49.3605062722945));
#201867=CARTESIAN_POINT('Origin',(117.045701373479,3.75,49.2651013158452));
#201868=CARTESIAN_POINT('',(116.98845839961,3.75,49.5595894173749));
#201869=CARTESIAN_POINT('',(117.045701373479,3.75,49.2651013158452));
#201870=CARTESIAN_POINT('Origin',(116.2603997694,4.25,49.1124533855264));
#201871=CARTESIAN_POINT('',(116.75121327195,4.25,49.2078583419757));
#201872=CARTESIAN_POINT('',(116.69397029808,4.25,49.5023464435054));
#201873=CARTESIAN_POINT('',(116.75121327195,4.25,49.2078583419757));
#201874=CARTESIAN_POINT('',(116.203156795531,4.25,49.4069414870561));
#201875=CARTESIAN_POINT('',(116.203156795531,4.25,49.4069414870561));
#201876=CARTESIAN_POINT('',(116.2603997694,4.25,49.1124533855264));
#201877=CARTESIAN_POINT('',(116.2603997694,4.25,49.1124533855264));
#201878=CARTESIAN_POINT('',(116.2603997694,4.25,49.1124533855264));
#201879=CARTESIAN_POINT('Origin',(116.75121327195,4.25,49.2078583419757));
#201880=CARTESIAN_POINT('',(116.75121327195,3.75,49.2078583419757));
#201881=CARTESIAN_POINT('',(116.69397029808,3.75,49.5023464435054));
#201882=CARTESIAN_POINT('',(116.75121327195,3.75,49.2078583419757));
#201883=CARTESIAN_POINT('',(116.69397029808,4.25,49.5023464435054));
#201884=CARTESIAN_POINT('',(116.75121327195,4.25,49.2078583419757));
#201885=CARTESIAN_POINT('Origin',(116.75121327195,3.75,49.2078583419757));
#201886=CARTESIAN_POINT('',(116.2603997694,3.75,49.1124533855264));
#201887=CARTESIAN_POINT('',(116.203156795531,3.75,49.4069414870561));
#201888=CARTESIAN_POINT('',(116.2603997694,3.75,49.1124533855264));
#201889=CARTESIAN_POINT('',(116.69397029808,3.75,49.5023464435054));
#201890=CARTESIAN_POINT('',(116.75121327195,3.75,49.2078583419757));
#201891=CARTESIAN_POINT('Origin',(116.2603997694,3.75,49.1124533855264));
#201892=CARTESIAN_POINT('',(116.203156795531,3.75,49.4069414870561));
#201893=CARTESIAN_POINT('',(116.2603997694,3.75,49.1124533855264));
#201894=CARTESIAN_POINT('Origin',(115.475098165321,4.25,48.9598054552076));
#201895=CARTESIAN_POINT('',(115.96591166787,4.25,49.0552104116569));
#201896=CARTESIAN_POINT('',(115.908668694001,4.25,49.3496985131866));
#201897=CARTESIAN_POINT('',(115.96591166787,4.25,49.0552104116569));
#201898=CARTESIAN_POINT('',(115.417855191451,4.25,49.2542935567373));
#201899=CARTESIAN_POINT('',(115.417855191451,4.25,49.2542935567373));
#201900=CARTESIAN_POINT('',(115.475098165321,4.25,48.9598054552076));
#201901=CARTESIAN_POINT('',(115.475098165321,4.25,48.9598054552076));
#201902=CARTESIAN_POINT('',(115.475098165321,4.25,48.9598054552076));
#201903=CARTESIAN_POINT('Origin',(115.96591166787,4.25,49.0552104116569));
#201904=CARTESIAN_POINT('',(115.96591166787,3.75,49.0552104116569));
#201905=CARTESIAN_POINT('',(115.908668694001,3.75,49.3496985131866));
#201906=CARTESIAN_POINT('',(115.96591166787,3.75,49.0552104116569));
#201907=CARTESIAN_POINT('',(115.908668694001,4.25,49.3496985131866));
#201908=CARTESIAN_POINT('',(115.96591166787,4.25,49.0552104116569));
#201909=CARTESIAN_POINT('Origin',(115.96591166787,3.75,49.0552104116569));
#201910=CARTESIAN_POINT('',(115.475098165321,3.75,48.9598054552076));
#201911=CARTESIAN_POINT('',(115.417855191451,3.75,49.2542935567373));
#201912=CARTESIAN_POINT('',(115.475098165321,3.75,48.9598054552076));
#201913=CARTESIAN_POINT('',(115.908668694001,3.75,49.3496985131866));
#201914=CARTESIAN_POINT('',(115.96591166787,3.75,49.0552104116569));
#201915=CARTESIAN_POINT('Origin',(115.475098165321,3.75,48.9598054552076));
#201916=CARTESIAN_POINT('',(115.417855191451,3.75,49.2542935567373));
#201917=CARTESIAN_POINT('',(115.475098165321,3.75,48.9598054552076));
#201918=CARTESIAN_POINT('Origin',(114.689796561242,4.25,48.8071575248888));
#201919=CARTESIAN_POINT('',(115.180610063791,4.25,48.9025624813381));
#201920=CARTESIAN_POINT('',(115.123367089922,4.25,49.1970505828678));
#201921=CARTESIAN_POINT('',(115.180610063791,4.25,48.9025624813381));
#201922=CARTESIAN_POINT('',(114.632553587372,4.25,49.1016456264185));
#201923=CARTESIAN_POINT('',(114.632553587372,4.25,49.1016456264185));
#201924=CARTESIAN_POINT('',(114.689796561242,4.25,48.8071575248888));
#201925=CARTESIAN_POINT('',(114.689796561242,4.25,48.8071575248888));
#201926=CARTESIAN_POINT('',(114.689796561242,4.25,48.8071575248888));
#201927=CARTESIAN_POINT('Origin',(115.180610063791,4.25,48.9025624813381));
#201928=CARTESIAN_POINT('',(115.180610063791,3.75,48.9025624813381));
#201929=CARTESIAN_POINT('',(115.123367089922,3.75,49.1970505828678));
#201930=CARTESIAN_POINT('',(115.180610063791,3.75,48.9025624813381));
#201931=CARTESIAN_POINT('',(115.123367089922,4.25,49.1970505828678));
#201932=CARTESIAN_POINT('',(115.180610063791,4.25,48.9025624813381));
#201933=CARTESIAN_POINT('Origin',(115.180610063791,3.75,48.9025624813381));
#201934=CARTESIAN_POINT('',(114.689796561242,3.75,48.8071575248888));
#201935=CARTESIAN_POINT('',(114.632553587372,3.75,49.1016456264185));
#201936=CARTESIAN_POINT('',(114.689796561242,3.75,48.8071575248888));
#201937=CARTESIAN_POINT('',(115.123367089922,3.75,49.1970505828678));
#201938=CARTESIAN_POINT('',(115.180610063791,3.75,48.9025624813381));
#201939=CARTESIAN_POINT('Origin',(114.689796561242,3.75,48.8071575248888));
#201940=CARTESIAN_POINT('',(114.632553587372,3.75,49.1016456264185));
#201941=CARTESIAN_POINT('',(114.689796561242,3.75,48.8071575248888));
#201942=CARTESIAN_POINT('Origin',(113.904494957163,4.25,48.65450959457));
#201943=CARTESIAN_POINT('',(114.395308459712,4.25,48.7499145510193));
#201944=CARTESIAN_POINT('',(114.338065485842,4.25,49.044402652549));
#201945=CARTESIAN_POINT('',(114.395308459712,4.25,48.7499145510193));
#201946=CARTESIAN_POINT('',(113.847251983293,4.25,48.9489976960997));
#201947=CARTESIAN_POINT('',(113.847251983293,4.25,48.9489976960997));
#201948=CARTESIAN_POINT('',(113.904494957163,4.25,48.65450959457));
#201949=CARTESIAN_POINT('',(113.904494957163,4.25,48.65450959457));
#201950=CARTESIAN_POINT('',(113.904494957163,4.25,48.65450959457));
#201951=CARTESIAN_POINT('Origin',(114.395308459712,4.25,48.7499145510193));
#201952=CARTESIAN_POINT('',(114.395308459712,3.75,48.7499145510193));
#201953=CARTESIAN_POINT('',(114.338065485842,3.75,49.044402652549));
#201954=CARTESIAN_POINT('',(114.395308459712,3.75,48.7499145510193));
#201955=CARTESIAN_POINT('',(114.338065485842,4.25,49.044402652549));
#201956=CARTESIAN_POINT('',(114.395308459712,4.25,48.7499145510193));
#201957=CARTESIAN_POINT('Origin',(114.395308459712,3.75,48.7499145510193));
#201958=CARTESIAN_POINT('',(113.904494957163,3.75,48.65450959457));
#201959=CARTESIAN_POINT('',(113.847251983293,3.75,48.9489976960997));
#201960=CARTESIAN_POINT('',(113.904494957163,3.75,48.65450959457));
#201961=CARTESIAN_POINT('',(114.338065485842,3.75,49.044402652549));
#201962=CARTESIAN_POINT('',(114.395308459712,3.75,48.7499145510193));
#201963=CARTESIAN_POINT('Origin',(113.904494957163,3.75,48.65450959457));
#201964=CARTESIAN_POINT('',(113.847251983293,3.75,48.9489976960997));
#201965=CARTESIAN_POINT('',(113.904494957163,3.75,48.65450959457));
#201966=CARTESIAN_POINT('Origin',(113.904494957163,3.45,48.65450959457));
#201967=CARTESIAN_POINT('',(114.395308459712,3.45,48.7499145510193));
#201968=CARTESIAN_POINT('',(114.338065485842,3.45,49.044402652549));
#201969=CARTESIAN_POINT('',(114.395308459712,3.45,48.7499145510193));
#201970=CARTESIAN_POINT('',(113.847251983293,3.45,48.9489976960997));
#201971=CARTESIAN_POINT('',(113.847251983293,3.45,48.9489976960997));
#201972=CARTESIAN_POINT('',(113.904494957163,3.45,48.65450959457));
#201973=CARTESIAN_POINT('',(113.904494957163,3.45,48.65450959457));
#201974=CARTESIAN_POINT('',(113.904494957163,3.45,48.65450959457));
#201975=CARTESIAN_POINT('Origin',(114.395308459712,3.45,48.7499145510193));
#201976=CARTESIAN_POINT('',(114.395308459712,2.95,48.7499145510193));
#201977=CARTESIAN_POINT('',(114.338065485842,2.95,49.044402652549));
#201978=CARTESIAN_POINT('',(114.395308459712,2.95,48.7499145510193));
#201979=CARTESIAN_POINT('',(114.338065485842,3.45,49.044402652549));
#201980=CARTESIAN_POINT('',(114.395308459712,3.45,48.7499145510193));
#201981=CARTESIAN_POINT('Origin',(114.395308459712,2.95,48.7499145510193));
#201982=CARTESIAN_POINT('',(113.904494957163,2.95,48.65450959457));
#201983=CARTESIAN_POINT('',(113.847251983293,2.95,48.9489976960997));
#201984=CARTESIAN_POINT('',(113.904494957163,2.95,48.65450959457));
#201985=CARTESIAN_POINT('',(114.338065485842,2.95,49.044402652549));
#201986=CARTESIAN_POINT('',(114.395308459712,2.95,48.7499145510193));
#201987=CARTESIAN_POINT('Origin',(113.904494957163,2.95,48.65450959457));
#201988=CARTESIAN_POINT('',(113.847251983293,2.95,48.9489976960997));
#201989=CARTESIAN_POINT('',(113.904494957163,2.95,48.65450959457));
#201990=CARTESIAN_POINT('Origin',(113.904494957163,2.65,48.65450959457));
#201991=CARTESIAN_POINT('',(114.395308459712,2.65,48.7499145510193));
#201992=CARTESIAN_POINT('',(114.338065485842,2.65,49.044402652549));
#201993=CARTESIAN_POINT('',(114.395308459712,2.65,48.7499145510193));
#201994=CARTESIAN_POINT('',(113.847251983293,2.65,48.9489976960997));
#201995=CARTESIAN_POINT('',(113.847251983293,2.65,48.9489976960997));
#201996=CARTESIAN_POINT('',(113.904494957163,2.65,48.65450959457));
#201997=CARTESIAN_POINT('',(113.904494957163,2.65,48.65450959457));
#201998=CARTESIAN_POINT('',(113.904494957163,2.65,48.65450959457));
#201999=CARTESIAN_POINT('Origin',(114.395308459712,2.65,48.7499145510193));
#202000=CARTESIAN_POINT('',(114.395308459712,2.15,48.7499145510193));
#202001=CARTESIAN_POINT('',(114.338065485842,2.15,49.044402652549));
#202002=CARTESIAN_POINT('',(114.395308459712,2.15,48.7499145510193));
#202003=CARTESIAN_POINT('',(114.338065485842,2.65,49.044402652549));
#202004=CARTESIAN_POINT('',(114.395308459712,2.65,48.7499145510193));
#202005=CARTESIAN_POINT('Origin',(114.395308459712,2.15,48.7499145510193));
#202006=CARTESIAN_POINT('',(113.904494957163,2.15,48.65450959457));
#202007=CARTESIAN_POINT('',(113.847251983293,2.15,48.9489976960997));
#202008=CARTESIAN_POINT('',(113.904494957163,2.15,48.65450959457));
#202009=CARTESIAN_POINT('',(114.338065485842,2.15,49.044402652549));
#202010=CARTESIAN_POINT('',(114.395308459712,2.15,48.7499145510193));
#202011=CARTESIAN_POINT('Origin',(113.904494957163,2.15,48.65450959457));
#202012=CARTESIAN_POINT('',(113.847251983293,2.15,48.9489976960997));
#202013=CARTESIAN_POINT('',(113.904494957163,2.15,48.65450959457));
#202014=CARTESIAN_POINT('Origin',(113.904494957163,1.85,48.65450959457));
#202015=CARTESIAN_POINT('',(114.395308459712,1.85,48.7499145510193));
#202016=CARTESIAN_POINT('',(114.338065485842,1.85,49.044402652549));
#202017=CARTESIAN_POINT('',(114.395308459712,1.85,48.7499145510193));
#202018=CARTESIAN_POINT('',(113.847251983293,1.85,48.9489976960997));
#202019=CARTESIAN_POINT('',(113.847251983293,1.85,48.9489976960997));
#202020=CARTESIAN_POINT('',(113.904494957163,1.85,48.65450959457));
#202021=CARTESIAN_POINT('',(113.904494957163,1.85,48.65450959457));
#202022=CARTESIAN_POINT('',(113.904494957163,1.85,48.65450959457));
#202023=CARTESIAN_POINT('Origin',(114.395308459712,1.85,48.7499145510193));
#202024=CARTESIAN_POINT('',(114.395308459712,1.35,48.7499145510193));
#202025=CARTESIAN_POINT('',(114.338065485842,1.35,49.044402652549));
#202026=CARTESIAN_POINT('',(114.395308459712,1.35,48.7499145510193));
#202027=CARTESIAN_POINT('',(114.338065485842,1.85,49.044402652549));
#202028=CARTESIAN_POINT('',(114.395308459712,1.85,48.7499145510193));
#202029=CARTESIAN_POINT('Origin',(114.395308459712,1.35,48.7499145510193));
#202030=CARTESIAN_POINT('',(113.904494957163,1.35,48.65450959457));
#202031=CARTESIAN_POINT('',(113.847251983293,1.35,48.9489976960997));
#202032=CARTESIAN_POINT('',(113.904494957163,1.35,48.65450959457));
#202033=CARTESIAN_POINT('',(114.338065485842,1.35,49.044402652549));
#202034=CARTESIAN_POINT('',(114.395308459712,1.35,48.7499145510193));
#202035=CARTESIAN_POINT('Origin',(113.904494957163,1.35,48.65450959457));
#202036=CARTESIAN_POINT('',(113.847251983293,1.35,48.9489976960997));
#202037=CARTESIAN_POINT('',(113.904494957163,1.35,48.65450959457));
#202038=CARTESIAN_POINT('Origin',(113.904494957163,1.05,48.65450959457));
#202039=CARTESIAN_POINT('',(114.395308459712,1.05,48.7499145510193));
#202040=CARTESIAN_POINT('',(114.338065485842,1.05,49.044402652549));
#202041=CARTESIAN_POINT('',(114.395308459712,1.05,48.7499145510193));
#202042=CARTESIAN_POINT('',(113.847251983293,1.05,48.9489976960997));
#202043=CARTESIAN_POINT('',(113.847251983293,1.05,48.9489976960997));
#202044=CARTESIAN_POINT('',(113.904494957163,1.05,48.65450959457));
#202045=CARTESIAN_POINT('',(113.904494957163,1.05,48.65450959457));
#202046=CARTESIAN_POINT('',(113.904494957163,1.05,48.65450959457));
#202047=CARTESIAN_POINT('Origin',(114.395308459712,1.05,48.7499145510193));
#202048=CARTESIAN_POINT('',(114.395308459712,0.550000000000015,48.7499145510193));
#202049=CARTESIAN_POINT('',(114.338065485842,0.550000000000015,49.044402652549));
#202050=CARTESIAN_POINT('',(114.395308459712,0.550000000000015,48.7499145510193));
#202051=CARTESIAN_POINT('',(114.338065485842,1.05,49.044402652549));
#202052=CARTESIAN_POINT('',(114.395308459712,1.05,48.7499145510193));
#202053=CARTESIAN_POINT('Origin',(114.395308459712,0.550000000000015,48.7499145510193));
#202054=CARTESIAN_POINT('',(113.904494957163,0.550000000000015,48.65450959457));
#202055=CARTESIAN_POINT('',(113.847251983293,0.550000000000015,48.9489976960997));
#202056=CARTESIAN_POINT('',(113.904494957163,0.550000000000015,48.65450959457));
#202057=CARTESIAN_POINT('',(114.338065485842,0.550000000000015,49.044402652549));
#202058=CARTESIAN_POINT('',(114.395308459712,0.550000000000015,48.7499145510193));
#202059=CARTESIAN_POINT('Origin',(113.904494957163,0.550000000000015,48.65450959457));
#202060=CARTESIAN_POINT('',(113.847251983293,0.550000000000015,48.9489976960997));
#202061=CARTESIAN_POINT('',(113.904494957163,0.550000000000015,48.65450959457));
#202062=CARTESIAN_POINT('Origin',(113.904494957163,0.250000000000015,48.65450959457));
#202063=CARTESIAN_POINT('',(114.395308459712,0.250000000000015,48.7499145510193));
#202064=CARTESIAN_POINT('',(114.338065485842,0.250000000000015,49.044402652549));
#202065=CARTESIAN_POINT('',(114.395308459712,0.250000000000015,48.7499145510193));
#202066=CARTESIAN_POINT('',(113.847251983293,0.250000000000015,48.9489976960997));
#202067=CARTESIAN_POINT('',(113.847251983293,0.250000000000015,48.9489976960997));
#202068=CARTESIAN_POINT('',(113.904494957163,0.250000000000015,48.65450959457));
#202069=CARTESIAN_POINT('',(113.904494957163,0.250000000000015,48.65450959457));
#202070=CARTESIAN_POINT('',(113.904494957163,0.250000000000015,48.65450959457));
#202071=CARTESIAN_POINT('Origin',(114.395308459712,0.250000000000015,48.7499145510193));
#202072=CARTESIAN_POINT('',(114.395308459712,-0.249999999999985,48.7499145510193));
#202073=CARTESIAN_POINT('',(114.338065485842,-0.249999999999985,49.044402652549));
#202074=CARTESIAN_POINT('',(114.395308459712,-0.249999999999985,48.7499145510193));
#202075=CARTESIAN_POINT('',(114.338065485842,0.250000000000015,49.044402652549));
#202076=CARTESIAN_POINT('',(114.395308459712,0.250000000000015,48.7499145510193));
#202077=CARTESIAN_POINT('Origin',(114.395308459712,-0.249999999999985,48.7499145510193));
#202078=CARTESIAN_POINT('',(113.904494957163,-0.249999999999985,48.65450959457));
#202079=CARTESIAN_POINT('',(113.847251983293,-0.249999999999985,48.9489976960997));
#202080=CARTESIAN_POINT('',(113.904494957163,-0.249999999999985,48.65450959457));
#202081=CARTESIAN_POINT('',(114.338065485842,-0.249999999999985,49.044402652549));
#202082=CARTESIAN_POINT('',(114.395308459712,-0.249999999999985,48.7499145510193));
#202083=CARTESIAN_POINT('Origin',(113.904494957163,-0.249999999999985,48.65450959457));
#202084=CARTESIAN_POINT('',(113.847251983293,-0.249999999999985,48.9489976960997));
#202085=CARTESIAN_POINT('',(113.904494957163,-0.249999999999985,48.65450959457));
#202086=CARTESIAN_POINT('Origin',(113.904494957163,-0.549999999999986,48.65450959457));
#202087=CARTESIAN_POINT('',(114.395308459712,-0.549999999999986,48.7499145510193));
#202088=CARTESIAN_POINT('',(114.338065485842,-0.549999999999986,49.044402652549));
#202089=CARTESIAN_POINT('',(114.395308459712,-0.549999999999986,48.7499145510193));
#202090=CARTESIAN_POINT('',(113.847251983293,-0.549999999999986,48.9489976960997));
#202091=CARTESIAN_POINT('',(113.847251983293,-0.549999999999986,48.9489976960997));
#202092=CARTESIAN_POINT('',(113.904494957163,-0.549999999999986,48.65450959457));
#202093=CARTESIAN_POINT('',(113.904494957163,-0.549999999999986,48.65450959457));
#202094=CARTESIAN_POINT('',(113.904494957163,-0.549999999999986,48.65450959457));
#202095=CARTESIAN_POINT('Origin',(114.395308459712,-0.549999999999986,48.7499145510193));
#202096=CARTESIAN_POINT('',(114.395308459712,-1.05,48.7499145510193));
#202097=CARTESIAN_POINT('',(114.338065485842,-1.05,49.044402652549));
#202098=CARTESIAN_POINT('',(114.395308459712,-1.05,48.7499145510193));
#202099=CARTESIAN_POINT('',(114.338065485842,-0.549999999999986,49.044402652549));
#202100=CARTESIAN_POINT('',(114.395308459712,-0.549999999999986,48.7499145510193));
#202101=CARTESIAN_POINT('Origin',(114.395308459712,-1.05,48.7499145510193));
#202102=CARTESIAN_POINT('',(113.904494957163,-1.05,48.65450959457));
#202103=CARTESIAN_POINT('',(113.847251983293,-1.05,48.9489976960997));
#202104=CARTESIAN_POINT('',(113.904494957163,-1.05,48.65450959457));
#202105=CARTESIAN_POINT('',(114.338065485842,-1.05,49.044402652549));
#202106=CARTESIAN_POINT('',(114.395308459712,-1.05,48.7499145510193));
#202107=CARTESIAN_POINT('Origin',(113.904494957163,-1.05,48.65450959457));
#202108=CARTESIAN_POINT('',(113.847251983293,-1.05,48.9489976960997));
#202109=CARTESIAN_POINT('',(113.904494957163,-1.05,48.65450959457));
#202110=CARTESIAN_POINT('Origin',(113.904494957163,-1.35,48.65450959457));
#202111=CARTESIAN_POINT('',(114.395308459712,-1.35,48.7499145510193));
#202112=CARTESIAN_POINT('',(114.338065485842,-1.35,49.044402652549));
#202113=CARTESIAN_POINT('',(114.395308459712,-1.35,48.7499145510193));
#202114=CARTESIAN_POINT('',(113.847251983293,-1.35,48.9489976960997));
#202115=CARTESIAN_POINT('',(113.847251983293,-1.35,48.9489976960997));
#202116=CARTESIAN_POINT('',(113.904494957163,-1.35,48.65450959457));
#202117=CARTESIAN_POINT('',(113.904494957163,-1.35,48.65450959457));
#202118=CARTESIAN_POINT('',(113.904494957163,-1.35,48.65450959457));
#202119=CARTESIAN_POINT('Origin',(114.395308459712,-1.35,48.7499145510193));
#202120=CARTESIAN_POINT('',(114.395308459712,-1.85,48.7499145510193));
#202121=CARTESIAN_POINT('',(114.338065485842,-1.85,49.044402652549));
#202122=CARTESIAN_POINT('',(114.395308459712,-1.85,48.7499145510193));
#202123=CARTESIAN_POINT('',(114.338065485842,-1.35,49.044402652549));
#202124=CARTESIAN_POINT('',(114.395308459712,-1.35,48.7499145510193));
#202125=CARTESIAN_POINT('Origin',(114.395308459712,-1.85,48.7499145510193));
#202126=CARTESIAN_POINT('',(113.904494957163,-1.85,48.65450959457));
#202127=CARTESIAN_POINT('',(113.847251983293,-1.85,48.9489976960997));
#202128=CARTESIAN_POINT('',(113.904494957163,-1.85,48.65450959457));
#202129=CARTESIAN_POINT('',(114.338065485842,-1.85,49.044402652549));
#202130=CARTESIAN_POINT('',(114.395308459712,-1.85,48.7499145510193));
#202131=CARTESIAN_POINT('Origin',(113.904494957163,-1.85,48.65450959457));
#202132=CARTESIAN_POINT('',(113.847251983293,-1.85,48.9489976960997));
#202133=CARTESIAN_POINT('',(113.904494957163,-1.85,48.65450959457));
#202134=CARTESIAN_POINT('Origin',(113.904494957163,-2.15,48.65450959457));
#202135=CARTESIAN_POINT('',(114.395308459712,-2.15,48.7499145510193));
#202136=CARTESIAN_POINT('',(114.338065485842,-2.15,49.044402652549));
#202137=CARTESIAN_POINT('',(114.395308459712,-2.15,48.7499145510193));
#202138=CARTESIAN_POINT('',(113.847251983293,-2.15,48.9489976960997));
#202139=CARTESIAN_POINT('',(113.847251983293,-2.15,48.9489976960997));
#202140=CARTESIAN_POINT('',(113.904494957163,-2.15,48.65450959457));
#202141=CARTESIAN_POINT('',(113.904494957163,-2.15,48.65450959457));
#202142=CARTESIAN_POINT('',(113.904494957163,-2.15,48.65450959457));
#202143=CARTESIAN_POINT('Origin',(114.395308459712,-2.15,48.7499145510193));
#202144=CARTESIAN_POINT('',(114.395308459712,-2.65,48.7499145510193));
#202145=CARTESIAN_POINT('',(114.338065485842,-2.65,49.044402652549));
#202146=CARTESIAN_POINT('',(114.395308459712,-2.65,48.7499145510193));
#202147=CARTESIAN_POINT('',(114.338065485842,-2.15,49.044402652549));
#202148=CARTESIAN_POINT('',(114.395308459712,-2.15,48.7499145510193));
#202149=CARTESIAN_POINT('Origin',(114.395308459712,-2.65,48.7499145510193));
#202150=CARTESIAN_POINT('',(113.904494957163,-2.65,48.65450959457));
#202151=CARTESIAN_POINT('',(113.847251983293,-2.65,48.9489976960997));
#202152=CARTESIAN_POINT('',(113.904494957163,-2.65,48.65450959457));
#202153=CARTESIAN_POINT('',(114.338065485842,-2.65,49.044402652549));
#202154=CARTESIAN_POINT('',(114.395308459712,-2.65,48.7499145510193));
#202155=CARTESIAN_POINT('Origin',(113.904494957163,-2.65,48.65450959457));
#202156=CARTESIAN_POINT('',(113.847251983293,-2.65,48.9489976960997));
#202157=CARTESIAN_POINT('',(113.904494957163,-2.65,48.65450959457));
#202158=CARTESIAN_POINT('Origin',(113.904494957163,-2.95,48.65450959457));
#202159=CARTESIAN_POINT('',(114.395308459712,-2.95,48.7499145510193));
#202160=CARTESIAN_POINT('',(114.338065485842,-2.95,49.044402652549));
#202161=CARTESIAN_POINT('',(114.395308459712,-2.95,48.7499145510193));
#202162=CARTESIAN_POINT('',(113.847251983293,-2.95,48.9489976960997));
#202163=CARTESIAN_POINT('',(113.847251983293,-2.95,48.9489976960997));
#202164=CARTESIAN_POINT('',(113.904494957163,-2.95,48.65450959457));
#202165=CARTESIAN_POINT('',(113.904494957163,-2.95,48.65450959457));
#202166=CARTESIAN_POINT('',(113.904494957163,-2.95,48.65450959457));
#202167=CARTESIAN_POINT('Origin',(114.395308459712,-2.95,48.7499145510193));
#202168=CARTESIAN_POINT('',(114.395308459712,-3.45,48.7499145510193));
#202169=CARTESIAN_POINT('',(114.338065485842,-3.45,49.044402652549));
#202170=CARTESIAN_POINT('',(114.395308459712,-3.45,48.7499145510193));
#202171=CARTESIAN_POINT('',(114.338065485842,-2.95,49.044402652549));
#202172=CARTESIAN_POINT('',(114.395308459712,-2.95,48.7499145510193));
#202173=CARTESIAN_POINT('Origin',(114.395308459712,-3.45,48.7499145510193));
#202174=CARTESIAN_POINT('',(113.904494957163,-3.45,48.65450959457));
#202175=CARTESIAN_POINT('',(113.847251983293,-3.45,48.9489976960997));
#202176=CARTESIAN_POINT('',(113.904494957163,-3.45,48.65450959457));
#202177=CARTESIAN_POINT('',(114.338065485842,-3.45,49.044402652549));
#202178=CARTESIAN_POINT('',(114.395308459712,-3.45,48.7499145510193));
#202179=CARTESIAN_POINT('Origin',(113.904494957163,-3.45,48.65450959457));
#202180=CARTESIAN_POINT('',(113.847251983293,-3.45,48.9489976960997));
#202181=CARTESIAN_POINT('',(113.904494957163,-3.45,48.65450959457));
#202182=CARTESIAN_POINT('Origin',(114.689796561242,-2.95,48.8071575248888));
#202183=CARTESIAN_POINT('',(115.180610063791,-2.95,48.9025624813381));
#202184=CARTESIAN_POINT('',(115.123367089922,-2.95,49.1970505828678));
#202185=CARTESIAN_POINT('',(115.180610063791,-2.95,48.9025624813381));
#202186=CARTESIAN_POINT('',(114.632553587372,-2.95,49.1016456264185));
#202187=CARTESIAN_POINT('',(114.632553587372,-2.95,49.1016456264185));
#202188=CARTESIAN_POINT('',(114.689796561242,-2.95,48.8071575248888));
#202189=CARTESIAN_POINT('',(114.689796561242,-2.95,48.8071575248888));
#202190=CARTESIAN_POINT('',(114.689796561242,-2.95,48.8071575248888));
#202191=CARTESIAN_POINT('Origin',(115.180610063791,-2.95,48.9025624813381));
#202192=CARTESIAN_POINT('',(115.180610063791,-3.45,48.9025624813381));
#202193=CARTESIAN_POINT('',(115.123367089922,-3.45,49.1970505828678));
#202194=CARTESIAN_POINT('',(115.180610063791,-3.45,48.9025624813381));
#202195=CARTESIAN_POINT('',(115.123367089922,-2.95,49.1970505828678));
#202196=CARTESIAN_POINT('',(115.180610063791,-2.95,48.9025624813381));
#202197=CARTESIAN_POINT('Origin',(115.180610063791,-3.45,48.9025624813381));
#202198=CARTESIAN_POINT('',(114.689796561242,-3.45,48.8071575248888));
#202199=CARTESIAN_POINT('',(114.632553587372,-3.45,49.1016456264185));
#202200=CARTESIAN_POINT('',(114.689796561242,-3.45,48.8071575248888));
#202201=CARTESIAN_POINT('',(115.123367089922,-3.45,49.1970505828678));
#202202=CARTESIAN_POINT('',(115.180610063791,-3.45,48.9025624813381));
#202203=CARTESIAN_POINT('Origin',(114.689796561242,-3.45,48.8071575248888));
#202204=CARTESIAN_POINT('',(114.632553587372,-3.45,49.1016456264185));
#202205=CARTESIAN_POINT('',(114.689796561242,-3.45,48.8071575248888));
#202206=CARTESIAN_POINT('Origin',(115.475098165321,-2.95,48.9598054552076));
#202207=CARTESIAN_POINT('',(115.96591166787,-2.95,49.0552104116569));
#202208=CARTESIAN_POINT('',(115.908668694001,-2.95,49.3496985131866));
#202209=CARTESIAN_POINT('',(115.96591166787,-2.95,49.0552104116569));
#202210=CARTESIAN_POINT('',(115.417855191451,-2.95,49.2542935567373));
#202211=CARTESIAN_POINT('',(115.417855191451,-2.95,49.2542935567373));
#202212=CARTESIAN_POINT('',(115.475098165321,-2.95,48.9598054552076));
#202213=CARTESIAN_POINT('',(115.475098165321,-2.95,48.9598054552076));
#202214=CARTESIAN_POINT('',(115.475098165321,-2.95,48.9598054552076));
#202215=CARTESIAN_POINT('Origin',(115.96591166787,-2.95,49.0552104116569));
#202216=CARTESIAN_POINT('',(115.96591166787,-3.45,49.0552104116569));
#202217=CARTESIAN_POINT('',(115.908668694001,-3.45,49.3496985131866));
#202218=CARTESIAN_POINT('',(115.96591166787,-3.45,49.0552104116569));
#202219=CARTESIAN_POINT('',(115.908668694001,-2.95,49.3496985131866));
#202220=CARTESIAN_POINT('',(115.96591166787,-2.95,49.0552104116569));
#202221=CARTESIAN_POINT('Origin',(115.96591166787,-3.45,49.0552104116569));
#202222=CARTESIAN_POINT('',(115.475098165321,-3.45,48.9598054552076));
#202223=CARTESIAN_POINT('',(115.417855191451,-3.45,49.2542935567373));
#202224=CARTESIAN_POINT('',(115.475098165321,-3.45,48.9598054552076));
#202225=CARTESIAN_POINT('',(115.908668694001,-3.45,49.3496985131866));
#202226=CARTESIAN_POINT('',(115.96591166787,-3.45,49.0552104116569));
#202227=CARTESIAN_POINT('Origin',(115.475098165321,-3.45,48.9598054552076));
#202228=CARTESIAN_POINT('',(115.417855191451,-3.45,49.2542935567373));
#202229=CARTESIAN_POINT('',(115.475098165321,-3.45,48.9598054552076));
#202230=CARTESIAN_POINT('Origin',(116.2603997694,-2.95,49.1124533855264));
#202231=CARTESIAN_POINT('',(116.75121327195,-2.95,49.2078583419757));
#202232=CARTESIAN_POINT('',(116.69397029808,-2.95,49.5023464435054));
#202233=CARTESIAN_POINT('',(116.75121327195,-2.95,49.2078583419757));
#202234=CARTESIAN_POINT('',(116.203156795531,-2.95,49.4069414870561));
#202235=CARTESIAN_POINT('',(116.203156795531,-2.95,49.4069414870561));
#202236=CARTESIAN_POINT('',(116.2603997694,-2.95,49.1124533855264));
#202237=CARTESIAN_POINT('',(116.2603997694,-2.95,49.1124533855264));
#202238=CARTESIAN_POINT('',(116.2603997694,-2.95,49.1124533855264));
#202239=CARTESIAN_POINT('Origin',(116.75121327195,-2.95,49.2078583419757));
#202240=CARTESIAN_POINT('',(116.75121327195,-3.45,49.2078583419757));
#202241=CARTESIAN_POINT('',(116.69397029808,-3.45,49.5023464435054));
#202242=CARTESIAN_POINT('',(116.75121327195,-3.45,49.2078583419757));
#202243=CARTESIAN_POINT('',(116.69397029808,-2.95,49.5023464435054));
#202244=CARTESIAN_POINT('',(116.75121327195,-2.95,49.2078583419757));
#202245=CARTESIAN_POINT('Origin',(116.75121327195,-3.45,49.2078583419757));
#202246=CARTESIAN_POINT('',(116.2603997694,-3.45,49.1124533855264));
#202247=CARTESIAN_POINT('',(116.203156795531,-3.45,49.4069414870561));
#202248=CARTESIAN_POINT('',(116.2603997694,-3.45,49.1124533855264));
#202249=CARTESIAN_POINT('',(116.69397029808,-3.45,49.5023464435054));
#202250=CARTESIAN_POINT('',(116.75121327195,-3.45,49.2078583419757));
#202251=CARTESIAN_POINT('Origin',(116.2603997694,-3.45,49.1124533855264));
#202252=CARTESIAN_POINT('',(116.203156795531,-3.45,49.4069414870561));
#202253=CARTESIAN_POINT('',(116.2603997694,-3.45,49.1124533855264));
#202254=CARTESIAN_POINT('Origin',(117.045701373479,-2.95,49.2651013158452));
#202255=CARTESIAN_POINT('',(117.536514876029,-2.95,49.3605062722945));
#202256=CARTESIAN_POINT('',(117.479271902159,-2.95,49.6549943738242));
#202257=CARTESIAN_POINT('',(117.536514876029,-2.95,49.3605062722945));
#202258=CARTESIAN_POINT('',(116.98845839961,-2.95,49.5595894173749));
#202259=CARTESIAN_POINT('',(116.98845839961,-2.95,49.5595894173749));
#202260=CARTESIAN_POINT('',(117.045701373479,-2.95,49.2651013158452));
#202261=CARTESIAN_POINT('',(117.045701373479,-2.95,49.2651013158452));
#202262=CARTESIAN_POINT('',(117.045701373479,-2.95,49.2651013158452));
#202263=CARTESIAN_POINT('Origin',(117.536514876029,-2.95,49.3605062722945));
#202264=CARTESIAN_POINT('',(117.536514876029,-3.45,49.3605062722945));
#202265=CARTESIAN_POINT('',(117.479271902159,-3.45,49.6549943738242));
#202266=CARTESIAN_POINT('',(117.536514876029,-3.45,49.3605062722945));
#202267=CARTESIAN_POINT('',(117.479271902159,-2.95,49.6549943738242));
#202268=CARTESIAN_POINT('',(117.536514876029,-2.95,49.3605062722945));
#202269=CARTESIAN_POINT('Origin',(117.536514876029,-3.45,49.3605062722945));
#202270=CARTESIAN_POINT('',(117.045701373479,-3.45,49.2651013158452));
#202271=CARTESIAN_POINT('',(116.98845839961,-3.45,49.5595894173749));
#202272=CARTESIAN_POINT('',(117.045701373479,-3.45,49.2651013158452));
#202273=CARTESIAN_POINT('',(117.479271902159,-3.45,49.6549943738242));
#202274=CARTESIAN_POINT('',(117.536514876029,-3.45,49.3605062722945));
#202275=CARTESIAN_POINT('Origin',(117.045701373479,-3.45,49.2651013158452));
#202276=CARTESIAN_POINT('',(116.98845839961,-3.45,49.5595894173749));
#202277=CARTESIAN_POINT('',(117.045701373479,-3.45,49.2651013158452));
#202278=CARTESIAN_POINT('Origin',(117.831002977559,-2.95,49.417749246164));
#202279=CARTESIAN_POINT('',(118.321816480108,-2.95,49.5131542026133));
#202280=CARTESIAN_POINT('',(118.264573506239,-2.95,49.807642304143));
#202281=CARTESIAN_POINT('',(118.321816480108,-2.95,49.5131542026133));
#202282=CARTESIAN_POINT('',(117.773760003689,-2.95,49.7122373476937));
#202283=CARTESIAN_POINT('',(117.773760003689,-2.95,49.7122373476937));
#202284=CARTESIAN_POINT('',(117.831002977559,-2.95,49.417749246164));
#202285=CARTESIAN_POINT('',(117.831002977559,-2.95,49.417749246164));
#202286=CARTESIAN_POINT('',(117.831002977559,-2.95,49.417749246164));
#202287=CARTESIAN_POINT('Origin',(118.321816480108,-2.95,49.5131542026133));
#202288=CARTESIAN_POINT('',(118.321816480108,-3.45,49.5131542026133));
#202289=CARTESIAN_POINT('',(118.264573506239,-3.45,49.807642304143));
#202290=CARTESIAN_POINT('',(118.321816480108,-3.45,49.5131542026133));
#202291=CARTESIAN_POINT('',(118.264573506239,-2.95,49.807642304143));
#202292=CARTESIAN_POINT('',(118.321816480108,-2.95,49.5131542026133));
#202293=CARTESIAN_POINT('Origin',(118.321816480108,-3.45,49.5131542026133));
#202294=CARTESIAN_POINT('',(117.831002977559,-3.45,49.417749246164));
#202295=CARTESIAN_POINT('',(117.773760003689,-3.45,49.7122373476937));
#202296=CARTESIAN_POINT('',(117.831002977559,-3.45,49.417749246164));
#202297=CARTESIAN_POINT('',(118.264573506239,-3.45,49.807642304143));
#202298=CARTESIAN_POINT('',(118.321816480108,-3.45,49.5131542026133));
#202299=CARTESIAN_POINT('Origin',(117.831002977559,-3.45,49.417749246164));
#202300=CARTESIAN_POINT('',(117.773760003689,-3.45,49.7122373476937));
#202301=CARTESIAN_POINT('',(117.831002977559,-3.45,49.417749246164));
#202302=CARTESIAN_POINT('Origin',(118.616304581638,-2.95,49.5703971764828));
#202303=CARTESIAN_POINT('',(119.107118084187,-2.95,49.6658021329321));
#202304=CARTESIAN_POINT('',(119.049875110318,-2.95,49.9602902344618));
#202305=CARTESIAN_POINT('',(119.107118084187,-2.95,49.6658021329321));
#202306=CARTESIAN_POINT('',(118.559061607768,-2.95,49.8648852780125));
#202307=CARTESIAN_POINT('',(118.559061607768,-2.95,49.8648852780125));
#202308=CARTESIAN_POINT('',(118.616304581638,-2.95,49.5703971764828));
#202309=CARTESIAN_POINT('',(118.616304581638,-2.95,49.5703971764828));
#202310=CARTESIAN_POINT('',(118.616304581638,-2.95,49.5703971764828));
#202311=CARTESIAN_POINT('Origin',(119.107118084187,-2.95,49.6658021329321));
#202312=CARTESIAN_POINT('',(119.107118084187,-3.45,49.6658021329321));
#202313=CARTESIAN_POINT('',(119.049875110318,-3.45,49.9602902344618));
#202314=CARTESIAN_POINT('',(119.107118084187,-3.45,49.6658021329321));
#202315=CARTESIAN_POINT('',(119.049875110318,-2.95,49.9602902344618));
#202316=CARTESIAN_POINT('',(119.107118084187,-2.95,49.6658021329321));
#202317=CARTESIAN_POINT('Origin',(119.107118084187,-3.45,49.6658021329321));
#202318=CARTESIAN_POINT('',(118.616304581638,-3.45,49.5703971764828));
#202319=CARTESIAN_POINT('',(118.559061607768,-3.45,49.8648852780125));
#202320=CARTESIAN_POINT('',(118.616304581638,-3.45,49.5703971764828));
#202321=CARTESIAN_POINT('',(119.049875110318,-3.45,49.9602902344618));
#202322=CARTESIAN_POINT('',(119.107118084187,-3.45,49.6658021329321));
#202323=CARTESIAN_POINT('Origin',(118.616304581638,-3.45,49.5703971764828));
#202324=CARTESIAN_POINT('',(118.559061607768,-3.45,49.8648852780125));
#202325=CARTESIAN_POINT('',(118.616304581638,-3.45,49.5703971764828));
#202326=CARTESIAN_POINT('Origin',(119.401606185717,-2.95,49.7230451068016));
#202327=CARTESIAN_POINT('',(119.892419688267,-2.95,49.8184500632509));
#202328=CARTESIAN_POINT('',(119.835176714397,-2.95,50.1129381647806));
#202329=CARTESIAN_POINT('',(119.892419688267,-2.95,49.8184500632509));
#202330=CARTESIAN_POINT('',(119.344363211847,-2.95,50.0175332083313));
#202331=CARTESIAN_POINT('',(119.344363211847,-2.95,50.0175332083313));
#202332=CARTESIAN_POINT('',(119.401606185717,-2.95,49.7230451068016));
#202333=CARTESIAN_POINT('',(119.401606185717,-2.95,49.7230451068016));
#202334=CARTESIAN_POINT('',(119.401606185717,-2.95,49.7230451068016));
#202335=CARTESIAN_POINT('Origin',(119.892419688267,-2.95,49.8184500632509));
#202336=CARTESIAN_POINT('',(119.892419688267,-3.45,49.8184500632509));
#202337=CARTESIAN_POINT('',(119.835176714397,-3.45,50.1129381647806));
#202338=CARTESIAN_POINT('',(119.892419688267,-3.45,49.8184500632509));
#202339=CARTESIAN_POINT('',(119.835176714397,-2.95,50.1129381647806));
#202340=CARTESIAN_POINT('',(119.892419688267,-2.95,49.8184500632509));
#202341=CARTESIAN_POINT('Origin',(119.892419688267,-3.45,49.8184500632509));
#202342=CARTESIAN_POINT('',(119.401606185717,-3.45,49.7230451068016));
#202343=CARTESIAN_POINT('',(119.344363211847,-3.45,50.0175332083313));
#202344=CARTESIAN_POINT('',(119.401606185717,-3.45,49.7230451068016));
#202345=CARTESIAN_POINT('',(119.835176714397,-3.45,50.1129381647806));
#202346=CARTESIAN_POINT('',(119.892419688267,-3.45,49.8184500632509));
#202347=CARTESIAN_POINT('Origin',(119.401606185717,-3.45,49.7230451068016));
#202348=CARTESIAN_POINT('',(119.344363211847,-3.45,50.0175332083313));
#202349=CARTESIAN_POINT('',(119.401606185717,-3.45,49.7230451068016));
#202350=CARTESIAN_POINT('Origin',(120.186907789796,-2.95,49.8756930371204));
#202351=CARTESIAN_POINT('',(120.677721292346,-2.95,49.9710979935697));
#202352=CARTESIAN_POINT('',(120.620478318476,-2.95,50.2655860950994));
#202353=CARTESIAN_POINT('',(120.677721292346,-2.95,49.9710979935697));
#202354=CARTESIAN_POINT('',(120.129664815927,-2.95,50.1701811386501));
#202355=CARTESIAN_POINT('',(120.129664815927,-2.95,50.1701811386501));
#202356=CARTESIAN_POINT('',(120.186907789796,-2.95,49.8756930371204));
#202357=CARTESIAN_POINT('',(120.186907789796,-2.95,49.8756930371204));
#202358=CARTESIAN_POINT('',(120.186907789796,-2.95,49.8756930371204));
#202359=CARTESIAN_POINT('Origin',(120.677721292346,-2.95,49.9710979935697));
#202360=CARTESIAN_POINT('',(120.677721292346,-3.45,49.9710979935697));
#202361=CARTESIAN_POINT('',(120.620478318476,-3.45,50.2655860950994));
#202362=CARTESIAN_POINT('',(120.677721292346,-3.45,49.9710979935697));
#202363=CARTESIAN_POINT('',(120.620478318476,-2.95,50.2655860950994));
#202364=CARTESIAN_POINT('',(120.677721292346,-2.95,49.9710979935697));
#202365=CARTESIAN_POINT('Origin',(120.677721292346,-3.45,49.9710979935697));
#202366=CARTESIAN_POINT('',(120.186907789796,-3.45,49.8756930371204));
#202367=CARTESIAN_POINT('',(120.129664815927,-3.45,50.1701811386501));
#202368=CARTESIAN_POINT('',(120.186907789796,-3.45,49.8756930371204));
#202369=CARTESIAN_POINT('',(120.620478318476,-3.45,50.2655860950994));
#202370=CARTESIAN_POINT('',(120.677721292346,-3.45,49.9710979935697));
#202371=CARTESIAN_POINT('Origin',(120.186907789796,-3.45,49.8756930371204));
#202372=CARTESIAN_POINT('',(120.129664815927,-3.45,50.1701811386501));
#202373=CARTESIAN_POINT('',(120.186907789796,-3.45,49.8756930371204));
#202374=CARTESIAN_POINT('Origin',(120.186907789796,-2.15,49.8756930371204));
#202375=CARTESIAN_POINT('',(120.677721292346,-2.15,49.9710979935697));
#202376=CARTESIAN_POINT('',(120.620478318476,-2.15,50.2655860950994));
#202377=CARTESIAN_POINT('',(120.677721292346,-2.15,49.9710979935697));
#202378=CARTESIAN_POINT('',(120.129664815927,-2.15,50.1701811386501));
#202379=CARTESIAN_POINT('',(120.129664815927,-2.15,50.1701811386501));
#202380=CARTESIAN_POINT('',(120.186907789796,-2.15,49.8756930371204));
#202381=CARTESIAN_POINT('',(120.186907789796,-2.15,49.8756930371204));
#202382=CARTESIAN_POINT('',(120.186907789796,-2.15,49.8756930371204));
#202383=CARTESIAN_POINT('Origin',(120.677721292346,-2.15,49.9710979935697));
#202384=CARTESIAN_POINT('',(120.677721292346,-2.65,49.9710979935697));
#202385=CARTESIAN_POINT('',(120.620478318476,-2.65,50.2655860950994));
#202386=CARTESIAN_POINT('',(120.677721292346,-2.65,49.9710979935697));
#202387=CARTESIAN_POINT('',(120.620478318476,-2.15,50.2655860950994));
#202388=CARTESIAN_POINT('',(120.677721292346,-2.15,49.9710979935697));
#202389=CARTESIAN_POINT('Origin',(120.677721292346,-2.65,49.9710979935697));
#202390=CARTESIAN_POINT('',(120.186907789796,-2.65,49.8756930371204));
#202391=CARTESIAN_POINT('',(120.129664815927,-2.65,50.1701811386501));
#202392=CARTESIAN_POINT('',(120.186907789796,-2.65,49.8756930371204));
#202393=CARTESIAN_POINT('',(120.620478318476,-2.65,50.2655860950994));
#202394=CARTESIAN_POINT('',(120.677721292346,-2.65,49.9710979935697));
#202395=CARTESIAN_POINT('Origin',(120.186907789796,-2.65,49.8756930371204));
#202396=CARTESIAN_POINT('',(120.129664815927,-2.65,50.1701811386501));
#202397=CARTESIAN_POINT('',(120.186907789796,-2.65,49.8756930371204));
#202398=CARTESIAN_POINT('Origin',(120.186907789796,-1.35,49.8756930371204));
#202399=CARTESIAN_POINT('',(120.677721292346,-1.35,49.9710979935697));
#202400=CARTESIAN_POINT('',(120.620478318476,-1.35,50.2655860950994));
#202401=CARTESIAN_POINT('',(120.677721292346,-1.35,49.9710979935697));
#202402=CARTESIAN_POINT('',(120.129664815927,-1.35,50.1701811386501));
#202403=CARTESIAN_POINT('',(120.129664815927,-1.35,50.1701811386501));
#202404=CARTESIAN_POINT('',(120.186907789796,-1.35,49.8756930371204));
#202405=CARTESIAN_POINT('',(120.186907789796,-1.35,49.8756930371204));
#202406=CARTESIAN_POINT('',(120.186907789796,-1.35,49.8756930371204));
#202407=CARTESIAN_POINT('Origin',(120.677721292346,-1.35,49.9710979935697));
#202408=CARTESIAN_POINT('',(120.677721292346,-1.85,49.9710979935697));
#202409=CARTESIAN_POINT('',(120.620478318476,-1.85,50.2655860950994));
#202410=CARTESIAN_POINT('',(120.677721292346,-1.85,49.9710979935697));
#202411=CARTESIAN_POINT('',(120.620478318476,-1.35,50.2655860950994));
#202412=CARTESIAN_POINT('',(120.677721292346,-1.35,49.9710979935697));
#202413=CARTESIAN_POINT('Origin',(120.677721292346,-1.85,49.9710979935697));
#202414=CARTESIAN_POINT('',(120.186907789796,-1.85,49.8756930371204));
#202415=CARTESIAN_POINT('',(120.129664815927,-1.85,50.1701811386501));
#202416=CARTESIAN_POINT('',(120.186907789796,-1.85,49.8756930371204));
#202417=CARTESIAN_POINT('',(120.620478318476,-1.85,50.2655860950994));
#202418=CARTESIAN_POINT('',(120.677721292346,-1.85,49.9710979935697));
#202419=CARTESIAN_POINT('Origin',(120.186907789796,-1.85,49.8756930371204));
#202420=CARTESIAN_POINT('',(120.129664815927,-1.85,50.1701811386501));
#202421=CARTESIAN_POINT('',(120.186907789796,-1.85,49.8756930371204));
#202422=CARTESIAN_POINT('Origin',(120.186907789796,-0.549999999999986,49.8756930371204));
#202423=CARTESIAN_POINT('',(120.677721292346,-0.549999999999986,49.9710979935697));
#202424=CARTESIAN_POINT('',(120.620478318476,-0.549999999999986,50.2655860950994));
#202425=CARTESIAN_POINT('',(120.677721292346,-0.549999999999986,49.9710979935697));
#202426=CARTESIAN_POINT('',(120.129664815927,-0.549999999999986,50.1701811386501));
#202427=CARTESIAN_POINT('',(120.129664815927,-0.549999999999986,50.1701811386501));
#202428=CARTESIAN_POINT('',(120.186907789796,-0.549999999999986,49.8756930371204));
#202429=CARTESIAN_POINT('',(120.186907789796,-0.549999999999986,49.8756930371204));
#202430=CARTESIAN_POINT('',(120.186907789796,-0.549999999999986,49.8756930371204));
#202431=CARTESIAN_POINT('Origin',(120.677721292346,-0.549999999999986,49.9710979935697));
#202432=CARTESIAN_POINT('',(120.677721292346,-1.05,49.9710979935697));
#202433=CARTESIAN_POINT('',(120.620478318476,-1.05,50.2655860950994));
#202434=CARTESIAN_POINT('',(120.677721292346,-1.05,49.9710979935697));
#202435=CARTESIAN_POINT('',(120.620478318476,-0.549999999999986,50.2655860950994));
#202436=CARTESIAN_POINT('',(120.677721292346,-0.549999999999986,49.9710979935697));
#202437=CARTESIAN_POINT('Origin',(120.677721292346,-1.05,49.9710979935697));
#202438=CARTESIAN_POINT('',(120.186907789796,-1.05,49.8756930371204));
#202439=CARTESIAN_POINT('',(120.129664815927,-1.05,50.1701811386501));
#202440=CARTESIAN_POINT('',(120.186907789796,-1.05,49.8756930371204));
#202441=CARTESIAN_POINT('',(120.620478318476,-1.05,50.2655860950994));
#202442=CARTESIAN_POINT('',(120.677721292346,-1.05,49.9710979935697));
#202443=CARTESIAN_POINT('Origin',(120.186907789796,-1.05,49.8756930371204));
#202444=CARTESIAN_POINT('',(120.129664815927,-1.05,50.1701811386501));
#202445=CARTESIAN_POINT('',(120.186907789796,-1.05,49.8756930371204));
#202446=CARTESIAN_POINT('Origin',(120.186907789796,0.250000000000015,49.8756930371204));
#202447=CARTESIAN_POINT('',(120.677721292346,0.250000000000015,49.9710979935697));
#202448=CARTESIAN_POINT('',(120.620478318476,0.250000000000015,50.2655860950994));
#202449=CARTESIAN_POINT('',(120.677721292346,0.250000000000015,49.9710979935697));
#202450=CARTESIAN_POINT('',(120.129664815927,0.250000000000015,50.1701811386501));
#202451=CARTESIAN_POINT('',(120.129664815927,0.250000000000015,50.1701811386501));
#202452=CARTESIAN_POINT('',(120.186907789796,0.250000000000015,49.8756930371204));
#202453=CARTESIAN_POINT('',(120.186907789796,0.250000000000015,49.8756930371204));
#202454=CARTESIAN_POINT('',(120.186907789796,0.250000000000015,49.8756930371204));
#202455=CARTESIAN_POINT('Origin',(120.677721292346,0.250000000000015,49.9710979935697));
#202456=CARTESIAN_POINT('',(120.677721292346,-0.249999999999985,49.9710979935697));
#202457=CARTESIAN_POINT('',(120.620478318476,-0.249999999999985,50.2655860950994));
#202458=CARTESIAN_POINT('',(120.677721292346,-0.249999999999985,49.9710979935697));
#202459=CARTESIAN_POINT('',(120.620478318476,0.250000000000015,50.2655860950994));
#202460=CARTESIAN_POINT('',(120.677721292346,0.250000000000015,49.9710979935697));
#202461=CARTESIAN_POINT('Origin',(120.677721292346,-0.249999999999985,49.9710979935697));
#202462=CARTESIAN_POINT('',(120.186907789796,-0.249999999999985,49.8756930371204));
#202463=CARTESIAN_POINT('',(120.129664815927,-0.249999999999985,50.1701811386501));
#202464=CARTESIAN_POINT('',(120.186907789796,-0.249999999999985,49.8756930371204));
#202465=CARTESIAN_POINT('',(120.620478318476,-0.249999999999985,50.2655860950994));
#202466=CARTESIAN_POINT('',(120.677721292346,-0.249999999999985,49.9710979935697));
#202467=CARTESIAN_POINT('Origin',(120.186907789796,-0.249999999999985,49.8756930371204));
#202468=CARTESIAN_POINT('',(120.129664815927,-0.249999999999985,50.1701811386501));
#202469=CARTESIAN_POINT('',(120.186907789796,-0.249999999999985,49.8756930371204));
#202470=CARTESIAN_POINT('Origin',(120.186907789796,1.05,49.8756930371204));
#202471=CARTESIAN_POINT('',(120.677721292346,1.05,49.9710979935697));
#202472=CARTESIAN_POINT('',(120.620478318476,1.05,50.2655860950994));
#202473=CARTESIAN_POINT('',(120.677721292346,1.05,49.9710979935697));
#202474=CARTESIAN_POINT('',(120.129664815927,1.05,50.1701811386501));
#202475=CARTESIAN_POINT('',(120.129664815927,1.05,50.1701811386501));
#202476=CARTESIAN_POINT('',(120.186907789796,1.05,49.8756930371204));
#202477=CARTESIAN_POINT('',(120.186907789796,1.05,49.8756930371204));
#202478=CARTESIAN_POINT('',(120.186907789796,1.05,49.8756930371204));
#202479=CARTESIAN_POINT('Origin',(120.677721292346,1.05,49.9710979935697));
#202480=CARTESIAN_POINT('',(120.677721292346,0.550000000000015,49.9710979935697));
#202481=CARTESIAN_POINT('',(120.620478318476,0.550000000000015,50.2655860950994));
#202482=CARTESIAN_POINT('',(120.677721292346,0.550000000000015,49.9710979935697));
#202483=CARTESIAN_POINT('',(120.620478318476,1.05,50.2655860950994));
#202484=CARTESIAN_POINT('',(120.677721292346,1.05,49.9710979935697));
#202485=CARTESIAN_POINT('Origin',(120.677721292346,0.550000000000015,49.9710979935697));
#202486=CARTESIAN_POINT('',(120.186907789796,0.550000000000015,49.8756930371204));
#202487=CARTESIAN_POINT('',(120.129664815927,0.550000000000015,50.1701811386501));
#202488=CARTESIAN_POINT('',(120.186907789796,0.550000000000015,49.8756930371204));
#202489=CARTESIAN_POINT('',(120.620478318476,0.550000000000015,50.2655860950994));
#202490=CARTESIAN_POINT('',(120.677721292346,0.550000000000015,49.9710979935697));
#202491=CARTESIAN_POINT('Origin',(120.186907789796,0.550000000000015,49.8756930371204));
#202492=CARTESIAN_POINT('',(120.129664815927,0.550000000000015,50.1701811386501));
#202493=CARTESIAN_POINT('',(120.186907789796,0.550000000000015,49.8756930371204));
#202494=CARTESIAN_POINT('Origin',(120.186907789796,1.85,49.8756930371204));
#202495=CARTESIAN_POINT('',(120.677721292346,1.85,49.9710979935697));
#202496=CARTESIAN_POINT('',(120.620478318476,1.85,50.2655860950994));
#202497=CARTESIAN_POINT('',(120.677721292346,1.85,49.9710979935697));
#202498=CARTESIAN_POINT('',(120.129664815927,1.85,50.1701811386501));
#202499=CARTESIAN_POINT('',(120.129664815927,1.85,50.1701811386501));
#202500=CARTESIAN_POINT('',(120.186907789796,1.85,49.8756930371204));
#202501=CARTESIAN_POINT('',(120.186907789796,1.85,49.8756930371204));
#202502=CARTESIAN_POINT('',(120.186907789796,1.85,49.8756930371204));
#202503=CARTESIAN_POINT('Origin',(120.677721292346,1.85,49.9710979935697));
#202504=CARTESIAN_POINT('',(120.677721292346,1.35,49.9710979935697));
#202505=CARTESIAN_POINT('',(120.620478318476,1.35,50.2655860950994));
#202506=CARTESIAN_POINT('',(120.677721292346,1.35,49.9710979935697));
#202507=CARTESIAN_POINT('',(120.620478318476,1.85,50.2655860950994));
#202508=CARTESIAN_POINT('',(120.677721292346,1.85,49.9710979935697));
#202509=CARTESIAN_POINT('Origin',(120.677721292346,1.35,49.9710979935697));
#202510=CARTESIAN_POINT('',(120.186907789796,1.35,49.8756930371204));
#202511=CARTESIAN_POINT('',(120.129664815927,1.35,50.1701811386501));
#202512=CARTESIAN_POINT('',(120.186907789796,1.35,49.8756930371204));
#202513=CARTESIAN_POINT('',(120.620478318476,1.35,50.2655860950994));
#202514=CARTESIAN_POINT('',(120.677721292346,1.35,49.9710979935697));
#202515=CARTESIAN_POINT('Origin',(120.186907789796,1.35,49.8756930371204));
#202516=CARTESIAN_POINT('',(120.129664815927,1.35,50.1701811386501));
#202517=CARTESIAN_POINT('',(120.186907789796,1.35,49.8756930371204));
#202518=CARTESIAN_POINT('Origin',(120.186907789796,2.65,49.8756930371204));
#202519=CARTESIAN_POINT('',(120.677721292346,2.65,49.9710979935697));
#202520=CARTESIAN_POINT('',(120.620478318476,2.65,50.2655860950994));
#202521=CARTESIAN_POINT('',(120.677721292346,2.65,49.9710979935697));
#202522=CARTESIAN_POINT('',(120.129664815927,2.65,50.1701811386501));
#202523=CARTESIAN_POINT('',(120.129664815927,2.65,50.1701811386501));
#202524=CARTESIAN_POINT('',(120.186907789796,2.65,49.8756930371204));
#202525=CARTESIAN_POINT('',(120.186907789796,2.65,49.8756930371204));
#202526=CARTESIAN_POINT('',(120.186907789796,2.65,49.8756930371204));
#202527=CARTESIAN_POINT('Origin',(120.677721292346,2.65,49.9710979935697));
#202528=CARTESIAN_POINT('',(120.677721292346,2.15,49.9710979935697));
#202529=CARTESIAN_POINT('',(120.620478318476,2.15,50.2655860950994));
#202530=CARTESIAN_POINT('',(120.677721292346,2.15,49.9710979935697));
#202531=CARTESIAN_POINT('',(120.620478318476,2.65,50.2655860950994));
#202532=CARTESIAN_POINT('',(120.677721292346,2.65,49.9710979935697));
#202533=CARTESIAN_POINT('Origin',(120.677721292346,2.15,49.9710979935697));
#202534=CARTESIAN_POINT('',(120.186907789796,2.15,49.8756930371204));
#202535=CARTESIAN_POINT('',(120.129664815927,2.15,50.1701811386501));
#202536=CARTESIAN_POINT('',(120.186907789796,2.15,49.8756930371204));
#202537=CARTESIAN_POINT('',(120.620478318476,2.15,50.2655860950994));
#202538=CARTESIAN_POINT('',(120.677721292346,2.15,49.9710979935697));
#202539=CARTESIAN_POINT('Origin',(120.186907789796,2.15,49.8756930371204));
#202540=CARTESIAN_POINT('',(120.129664815927,2.15,50.1701811386501));
#202541=CARTESIAN_POINT('',(120.186907789796,2.15,49.8756930371204));
#202542=CARTESIAN_POINT('Origin',(120.186907789796,3.45,49.8756930371204));
#202543=CARTESIAN_POINT('',(120.677721292346,3.45,49.9710979935697));
#202544=CARTESIAN_POINT('',(120.620478318476,3.45,50.2655860950994));
#202545=CARTESIAN_POINT('',(120.677721292346,3.45,49.9710979935697));
#202546=CARTESIAN_POINT('',(120.129664815927,3.45,50.1701811386501));
#202547=CARTESIAN_POINT('',(120.129664815927,3.45,50.1701811386501));
#202548=CARTESIAN_POINT('',(120.186907789796,3.45,49.8756930371204));
#202549=CARTESIAN_POINT('',(120.186907789796,3.45,49.8756930371204));
#202550=CARTESIAN_POINT('',(120.186907789796,3.45,49.8756930371204));
#202551=CARTESIAN_POINT('Origin',(120.677721292346,3.45,49.9710979935697));
#202552=CARTESIAN_POINT('',(120.677721292346,2.95,49.9710979935697));
#202553=CARTESIAN_POINT('',(120.620478318476,2.95,50.2655860950994));
#202554=CARTESIAN_POINT('',(120.677721292346,2.95,49.9710979935697));
#202555=CARTESIAN_POINT('',(120.620478318476,3.45,50.2655860950994));
#202556=CARTESIAN_POINT('',(120.677721292346,3.45,49.9710979935697));
#202557=CARTESIAN_POINT('Origin',(120.677721292346,2.95,49.9710979935697));
#202558=CARTESIAN_POINT('',(120.186907789796,2.95,49.8756930371204));
#202559=CARTESIAN_POINT('',(120.129664815927,2.95,50.1701811386501));
#202560=CARTESIAN_POINT('',(120.186907789796,2.95,49.8756930371204));
#202561=CARTESIAN_POINT('',(120.620478318476,2.95,50.2655860950994));
#202562=CARTESIAN_POINT('',(120.677721292346,2.95,49.9710979935697));
#202563=CARTESIAN_POINT('Origin',(120.186907789796,2.95,49.8756930371204));
#202564=CARTESIAN_POINT('',(120.129664815927,2.95,50.1701811386501));
#202565=CARTESIAN_POINT('',(120.186907789796,2.95,49.8756930371204));
#202566=CARTESIAN_POINT('Origin',(119.401606185717,3.45,49.7230451068016));
#202567=CARTESIAN_POINT('',(119.892419688267,3.45,49.8184500632509));
#202568=CARTESIAN_POINT('',(119.835176714397,3.45,50.1129381647806));
#202569=CARTESIAN_POINT('',(119.892419688267,3.45,49.8184500632509));
#202570=CARTESIAN_POINT('',(119.344363211847,3.45,50.0175332083313));
#202571=CARTESIAN_POINT('',(119.344363211847,3.45,50.0175332083313));
#202572=CARTESIAN_POINT('',(119.401606185717,3.45,49.7230451068016));
#202573=CARTESIAN_POINT('',(119.401606185717,3.45,49.7230451068016));
#202574=CARTESIAN_POINT('',(119.401606185717,3.45,49.7230451068016));
#202575=CARTESIAN_POINT('Origin',(119.892419688267,3.45,49.8184500632509));
#202576=CARTESIAN_POINT('',(119.892419688267,2.95,49.8184500632509));
#202577=CARTESIAN_POINT('',(119.835176714397,2.95,50.1129381647806));
#202578=CARTESIAN_POINT('',(119.892419688267,2.95,49.8184500632509));
#202579=CARTESIAN_POINT('',(119.835176714397,3.45,50.1129381647806));
#202580=CARTESIAN_POINT('',(119.892419688267,3.45,49.8184500632509));
#202581=CARTESIAN_POINT('Origin',(119.892419688267,2.95,49.8184500632509));
#202582=CARTESIAN_POINT('',(119.401606185717,2.95,49.7230451068016));
#202583=CARTESIAN_POINT('',(119.344363211847,2.95,50.0175332083313));
#202584=CARTESIAN_POINT('',(119.401606185717,2.95,49.7230451068016));
#202585=CARTESIAN_POINT('',(119.835176714397,2.95,50.1129381647806));
#202586=CARTESIAN_POINT('',(119.892419688267,2.95,49.8184500632509));
#202587=CARTESIAN_POINT('Origin',(119.401606185717,2.95,49.7230451068016));
#202588=CARTESIAN_POINT('',(119.344363211847,2.95,50.0175332083313));
#202589=CARTESIAN_POINT('',(119.401606185717,2.95,49.7230451068016));
#202590=CARTESIAN_POINT('Origin',(118.616304581638,3.45,49.5703971764828));
#202591=CARTESIAN_POINT('',(119.107118084187,3.45,49.6658021329321));
#202592=CARTESIAN_POINT('',(119.049875110318,3.45,49.9602902344618));
#202593=CARTESIAN_POINT('',(119.107118084187,3.45,49.6658021329321));
#202594=CARTESIAN_POINT('',(118.559061607768,3.45,49.8648852780125));
#202595=CARTESIAN_POINT('',(118.559061607768,3.45,49.8648852780125));
#202596=CARTESIAN_POINT('',(118.616304581638,3.45,49.5703971764828));
#202597=CARTESIAN_POINT('',(118.616304581638,3.45,49.5703971764828));
#202598=CARTESIAN_POINT('',(118.616304581638,3.45,49.5703971764828));
#202599=CARTESIAN_POINT('Origin',(119.107118084187,3.45,49.6658021329321));
#202600=CARTESIAN_POINT('',(119.107118084187,2.95,49.6658021329321));
#202601=CARTESIAN_POINT('',(119.049875110318,2.95,49.9602902344618));
#202602=CARTESIAN_POINT('',(119.107118084187,2.95,49.6658021329321));
#202603=CARTESIAN_POINT('',(119.049875110318,3.45,49.9602902344618));
#202604=CARTESIAN_POINT('',(119.107118084187,3.45,49.6658021329321));
#202605=CARTESIAN_POINT('Origin',(119.107118084187,2.95,49.6658021329321));
#202606=CARTESIAN_POINT('',(118.616304581638,2.95,49.5703971764828));
#202607=CARTESIAN_POINT('',(118.559061607768,2.95,49.8648852780125));
#202608=CARTESIAN_POINT('',(118.616304581638,2.95,49.5703971764828));
#202609=CARTESIAN_POINT('',(119.049875110318,2.95,49.9602902344618));
#202610=CARTESIAN_POINT('',(119.107118084187,2.95,49.6658021329321));
#202611=CARTESIAN_POINT('Origin',(118.616304581638,2.95,49.5703971764828));
#202612=CARTESIAN_POINT('',(118.559061607768,2.95,49.8648852780125));
#202613=CARTESIAN_POINT('',(118.616304581638,2.95,49.5703971764828));
#202614=CARTESIAN_POINT('Origin',(117.831002977559,3.45,49.417749246164));
#202615=CARTESIAN_POINT('',(118.321816480108,3.45,49.5131542026133));
#202616=CARTESIAN_POINT('',(118.264573506239,3.45,49.807642304143));
#202617=CARTESIAN_POINT('',(118.321816480108,3.45,49.5131542026133));
#202618=CARTESIAN_POINT('',(117.773760003689,3.45,49.7122373476937));
#202619=CARTESIAN_POINT('',(117.773760003689,3.45,49.7122373476937));
#202620=CARTESIAN_POINT('',(117.831002977559,3.45,49.417749246164));
#202621=CARTESIAN_POINT('',(117.831002977559,3.45,49.417749246164));
#202622=CARTESIAN_POINT('',(117.831002977559,3.45,49.417749246164));
#202623=CARTESIAN_POINT('Origin',(118.321816480108,3.45,49.5131542026133));
#202624=CARTESIAN_POINT('',(118.321816480108,2.95,49.5131542026133));
#202625=CARTESIAN_POINT('',(118.264573506239,2.95,49.807642304143));
#202626=CARTESIAN_POINT('',(118.321816480108,2.95,49.5131542026133));
#202627=CARTESIAN_POINT('',(118.264573506239,3.45,49.807642304143));
#202628=CARTESIAN_POINT('',(118.321816480108,3.45,49.5131542026133));
#202629=CARTESIAN_POINT('Origin',(118.321816480108,2.95,49.5131542026133));
#202630=CARTESIAN_POINT('',(117.831002977559,2.95,49.417749246164));
#202631=CARTESIAN_POINT('',(117.773760003689,2.95,49.7122373476937));
#202632=CARTESIAN_POINT('',(117.831002977559,2.95,49.417749246164));
#202633=CARTESIAN_POINT('',(118.264573506239,2.95,49.807642304143));
#202634=CARTESIAN_POINT('',(118.321816480108,2.95,49.5131542026133));
#202635=CARTESIAN_POINT('Origin',(117.831002977559,2.95,49.417749246164));
#202636=CARTESIAN_POINT('',(117.773760003689,2.95,49.7122373476937));
#202637=CARTESIAN_POINT('',(117.831002977559,2.95,49.417749246164));
#202638=CARTESIAN_POINT('Origin',(117.045701373479,3.45,49.2651013158452));
#202639=CARTESIAN_POINT('',(117.536514876029,3.45,49.3605062722945));
#202640=CARTESIAN_POINT('',(117.479271902159,3.45,49.6549943738242));
#202641=CARTESIAN_POINT('',(117.536514876029,3.45,49.3605062722945));
#202642=CARTESIAN_POINT('',(116.98845839961,3.45,49.5595894173749));
#202643=CARTESIAN_POINT('',(116.98845839961,3.45,49.5595894173749));
#202644=CARTESIAN_POINT('',(117.045701373479,3.45,49.2651013158452));
#202645=CARTESIAN_POINT('',(117.045701373479,3.45,49.2651013158452));
#202646=CARTESIAN_POINT('',(117.045701373479,3.45,49.2651013158452));
#202647=CARTESIAN_POINT('Origin',(117.536514876029,3.45,49.3605062722945));
#202648=CARTESIAN_POINT('',(117.536514876029,2.95,49.3605062722945));
#202649=CARTESIAN_POINT('',(117.479271902159,2.95,49.6549943738242));
#202650=CARTESIAN_POINT('',(117.536514876029,2.95,49.3605062722945));
#202651=CARTESIAN_POINT('',(117.479271902159,3.45,49.6549943738242));
#202652=CARTESIAN_POINT('',(117.536514876029,3.45,49.3605062722945));
#202653=CARTESIAN_POINT('Origin',(117.536514876029,2.95,49.3605062722945));
#202654=CARTESIAN_POINT('',(117.045701373479,2.95,49.2651013158452));
#202655=CARTESIAN_POINT('',(116.98845839961,2.95,49.5595894173749));
#202656=CARTESIAN_POINT('',(117.045701373479,2.95,49.2651013158452));
#202657=CARTESIAN_POINT('',(117.479271902159,2.95,49.6549943738242));
#202658=CARTESIAN_POINT('',(117.536514876029,2.95,49.3605062722945));
#202659=CARTESIAN_POINT('Origin',(117.045701373479,2.95,49.2651013158452));
#202660=CARTESIAN_POINT('',(116.98845839961,2.95,49.5595894173749));
#202661=CARTESIAN_POINT('',(117.045701373479,2.95,49.2651013158452));
#202662=CARTESIAN_POINT('Origin',(116.2603997694,3.45,49.1124533855264));
#202663=CARTESIAN_POINT('',(116.75121327195,3.45,49.2078583419757));
#202664=CARTESIAN_POINT('',(116.69397029808,3.45,49.5023464435054));
#202665=CARTESIAN_POINT('',(116.75121327195,3.45,49.2078583419757));
#202666=CARTESIAN_POINT('',(116.203156795531,3.45,49.4069414870561));
#202667=CARTESIAN_POINT('',(116.203156795531,3.45,49.4069414870561));
#202668=CARTESIAN_POINT('',(116.2603997694,3.45,49.1124533855264));
#202669=CARTESIAN_POINT('',(116.2603997694,3.45,49.1124533855264));
#202670=CARTESIAN_POINT('',(116.2603997694,3.45,49.1124533855264));
#202671=CARTESIAN_POINT('Origin',(116.75121327195,3.45,49.2078583419757));
#202672=CARTESIAN_POINT('',(116.75121327195,2.95,49.2078583419757));
#202673=CARTESIAN_POINT('',(116.69397029808,2.95,49.5023464435054));
#202674=CARTESIAN_POINT('',(116.75121327195,2.95,49.2078583419757));
#202675=CARTESIAN_POINT('',(116.69397029808,3.45,49.5023464435054));
#202676=CARTESIAN_POINT('',(116.75121327195,3.45,49.2078583419757));
#202677=CARTESIAN_POINT('Origin',(116.75121327195,2.95,49.2078583419757));
#202678=CARTESIAN_POINT('',(116.2603997694,2.95,49.1124533855264));
#202679=CARTESIAN_POINT('',(116.203156795531,2.95,49.4069414870561));
#202680=CARTESIAN_POINT('',(116.2603997694,2.95,49.1124533855264));
#202681=CARTESIAN_POINT('',(116.69397029808,2.95,49.5023464435054));
#202682=CARTESIAN_POINT('',(116.75121327195,2.95,49.2078583419757));
#202683=CARTESIAN_POINT('Origin',(116.2603997694,2.95,49.1124533855264));
#202684=CARTESIAN_POINT('',(116.203156795531,2.95,49.4069414870561));
#202685=CARTESIAN_POINT('',(116.2603997694,2.95,49.1124533855264));
#202686=CARTESIAN_POINT('Origin',(115.475098165321,3.45,48.9598054552076));
#202687=CARTESIAN_POINT('',(115.96591166787,3.45,49.0552104116569));
#202688=CARTESIAN_POINT('',(115.908668694001,3.45,49.3496985131866));
#202689=CARTESIAN_POINT('',(115.96591166787,3.45,49.0552104116569));
#202690=CARTESIAN_POINT('',(115.417855191451,3.45,49.2542935567373));
#202691=CARTESIAN_POINT('',(115.417855191451,3.45,49.2542935567373));
#202692=CARTESIAN_POINT('',(115.475098165321,3.45,48.9598054552076));
#202693=CARTESIAN_POINT('',(115.475098165321,3.45,48.9598054552076));
#202694=CARTESIAN_POINT('',(115.475098165321,3.45,48.9598054552076));
#202695=CARTESIAN_POINT('Origin',(115.96591166787,3.45,49.0552104116569));
#202696=CARTESIAN_POINT('',(115.96591166787,2.95,49.0552104116569));
#202697=CARTESIAN_POINT('',(115.908668694001,2.95,49.3496985131866));
#202698=CARTESIAN_POINT('',(115.96591166787,2.95,49.0552104116569));
#202699=CARTESIAN_POINT('',(115.908668694001,3.45,49.3496985131866));
#202700=CARTESIAN_POINT('',(115.96591166787,3.45,49.0552104116569));
#202701=CARTESIAN_POINT('Origin',(115.96591166787,2.95,49.0552104116569));
#202702=CARTESIAN_POINT('',(115.475098165321,2.95,48.9598054552076));
#202703=CARTESIAN_POINT('',(115.417855191451,2.95,49.2542935567373));
#202704=CARTESIAN_POINT('',(115.475098165321,2.95,48.9598054552076));
#202705=CARTESIAN_POINT('',(115.908668694001,2.95,49.3496985131866));
#202706=CARTESIAN_POINT('',(115.96591166787,2.95,49.0552104116569));
#202707=CARTESIAN_POINT('Origin',(115.475098165321,2.95,48.9598054552076));
#202708=CARTESIAN_POINT('',(115.417855191451,2.95,49.2542935567373));
#202709=CARTESIAN_POINT('',(115.475098165321,2.95,48.9598054552076));
#202710=CARTESIAN_POINT('Origin',(114.689796561242,3.45,48.8071575248888));
#202711=CARTESIAN_POINT('',(115.180610063791,3.45,48.9025624813381));
#202712=CARTESIAN_POINT('',(115.123367089922,3.45,49.1970505828678));
#202713=CARTESIAN_POINT('',(115.180610063791,3.45,48.9025624813381));
#202714=CARTESIAN_POINT('',(114.632553587372,3.45,49.1016456264185));
#202715=CARTESIAN_POINT('',(114.632553587372,3.45,49.1016456264185));
#202716=CARTESIAN_POINT('',(114.689796561242,3.45,48.8071575248888));
#202717=CARTESIAN_POINT('',(114.689796561242,3.45,48.8071575248888));
#202718=CARTESIAN_POINT('',(114.689796561242,3.45,48.8071575248888));
#202719=CARTESIAN_POINT('Origin',(115.180610063791,3.45,48.9025624813381));
#202720=CARTESIAN_POINT('',(115.180610063791,2.95,48.9025624813381));
#202721=CARTESIAN_POINT('',(115.123367089922,2.95,49.1970505828678));
#202722=CARTESIAN_POINT('',(115.180610063791,2.95,48.9025624813381));
#202723=CARTESIAN_POINT('',(115.123367089922,3.45,49.1970505828678));
#202724=CARTESIAN_POINT('',(115.180610063791,3.45,48.9025624813381));
#202725=CARTESIAN_POINT('Origin',(115.180610063791,2.95,48.9025624813381));
#202726=CARTESIAN_POINT('',(114.689796561242,2.95,48.8071575248888));
#202727=CARTESIAN_POINT('',(114.632553587372,2.95,49.1016456264185));
#202728=CARTESIAN_POINT('',(114.689796561242,2.95,48.8071575248888));
#202729=CARTESIAN_POINT('',(115.123367089922,2.95,49.1970505828678));
#202730=CARTESIAN_POINT('',(115.180610063791,2.95,48.9025624813381));
#202731=CARTESIAN_POINT('Origin',(114.689796561242,2.95,48.8071575248888));
#202732=CARTESIAN_POINT('',(114.632553587372,2.95,49.1016456264185));
#202733=CARTESIAN_POINT('',(114.689796561242,2.95,48.8071575248888));
#202734=CARTESIAN_POINT('Origin',(114.689796561242,2.65,48.8071575248888));
#202735=CARTESIAN_POINT('',(115.180610063791,2.65,48.9025624813381));
#202736=CARTESIAN_POINT('',(115.123367089922,2.65,49.1970505828678));
#202737=CARTESIAN_POINT('',(115.180610063791,2.65,48.9025624813381));
#202738=CARTESIAN_POINT('',(114.632553587372,2.65,49.1016456264185));
#202739=CARTESIAN_POINT('',(114.632553587372,2.65,49.1016456264185));
#202740=CARTESIAN_POINT('',(114.689796561242,2.65,48.8071575248888));
#202741=CARTESIAN_POINT('',(114.689796561242,2.65,48.8071575248888));
#202742=CARTESIAN_POINT('',(114.689796561242,2.65,48.8071575248888));
#202743=CARTESIAN_POINT('Origin',(115.180610063791,2.65,48.9025624813381));
#202744=CARTESIAN_POINT('',(115.180610063791,2.15,48.9025624813381));
#202745=CARTESIAN_POINT('',(115.123367089922,2.15,49.1970505828678));
#202746=CARTESIAN_POINT('',(115.180610063791,2.15,48.9025624813381));
#202747=CARTESIAN_POINT('',(115.123367089922,2.65,49.1970505828678));
#202748=CARTESIAN_POINT('',(115.180610063791,2.65,48.9025624813381));
#202749=CARTESIAN_POINT('Origin',(115.180610063791,2.15,48.9025624813381));
#202750=CARTESIAN_POINT('',(114.689796561242,2.15,48.8071575248888));
#202751=CARTESIAN_POINT('',(114.632553587372,2.15,49.1016456264185));
#202752=CARTESIAN_POINT('',(114.689796561242,2.15,48.8071575248888));
#202753=CARTESIAN_POINT('',(115.123367089922,2.15,49.1970505828678));
#202754=CARTESIAN_POINT('',(115.180610063791,2.15,48.9025624813381));
#202755=CARTESIAN_POINT('Origin',(114.689796561242,2.15,48.8071575248888));
#202756=CARTESIAN_POINT('',(114.632553587372,2.15,49.1016456264185));
#202757=CARTESIAN_POINT('',(114.689796561242,2.15,48.8071575248888));
#202758=CARTESIAN_POINT('Origin',(114.689796561242,1.85,48.8071575248888));
#202759=CARTESIAN_POINT('',(115.180610063791,1.85,48.9025624813381));
#202760=CARTESIAN_POINT('',(115.123367089922,1.85,49.1970505828678));
#202761=CARTESIAN_POINT('',(115.180610063791,1.85,48.9025624813381));
#202762=CARTESIAN_POINT('',(114.632553587372,1.85,49.1016456264185));
#202763=CARTESIAN_POINT('',(114.632553587372,1.85,49.1016456264185));
#202764=CARTESIAN_POINT('',(114.689796561242,1.85,48.8071575248888));
#202765=CARTESIAN_POINT('',(114.689796561242,1.85,48.8071575248888));
#202766=CARTESIAN_POINT('',(114.689796561242,1.85,48.8071575248888));
#202767=CARTESIAN_POINT('Origin',(115.180610063791,1.85,48.9025624813381));
#202768=CARTESIAN_POINT('',(115.180610063791,1.35,48.9025624813381));
#202769=CARTESIAN_POINT('',(115.123367089922,1.35,49.1970505828678));
#202770=CARTESIAN_POINT('',(115.180610063791,1.35,48.9025624813381));
#202771=CARTESIAN_POINT('',(115.123367089922,1.85,49.1970505828678));
#202772=CARTESIAN_POINT('',(115.180610063791,1.85,48.9025624813381));
#202773=CARTESIAN_POINT('Origin',(115.180610063791,1.35,48.9025624813381));
#202774=CARTESIAN_POINT('',(114.689796561242,1.35,48.8071575248888));
#202775=CARTESIAN_POINT('',(114.632553587372,1.35,49.1016456264185));
#202776=CARTESIAN_POINT('',(114.689796561242,1.35,48.8071575248888));
#202777=CARTESIAN_POINT('',(115.123367089922,1.35,49.1970505828678));
#202778=CARTESIAN_POINT('',(115.180610063791,1.35,48.9025624813381));
#202779=CARTESIAN_POINT('Origin',(114.689796561242,1.35,48.8071575248888));
#202780=CARTESIAN_POINT('',(114.632553587372,1.35,49.1016456264185));
#202781=CARTESIAN_POINT('',(114.689796561242,1.35,48.8071575248888));
#202782=CARTESIAN_POINT('Origin',(114.689796561242,1.05,48.8071575248888));
#202783=CARTESIAN_POINT('',(115.180610063791,1.05,48.9025624813381));
#202784=CARTESIAN_POINT('',(115.123367089922,1.05,49.1970505828678));
#202785=CARTESIAN_POINT('',(115.180610063791,1.05,48.9025624813381));
#202786=CARTESIAN_POINT('',(114.632553587372,1.05,49.1016456264185));
#202787=CARTESIAN_POINT('',(114.632553587372,1.05,49.1016456264185));
#202788=CARTESIAN_POINT('',(114.689796561242,1.05,48.8071575248888));
#202789=CARTESIAN_POINT('',(114.689796561242,1.05,48.8071575248888));
#202790=CARTESIAN_POINT('',(114.689796561242,1.05,48.8071575248888));
#202791=CARTESIAN_POINT('Origin',(115.180610063791,1.05,48.9025624813381));
#202792=CARTESIAN_POINT('',(115.180610063791,0.550000000000015,48.9025624813381));
#202793=CARTESIAN_POINT('',(115.123367089922,0.550000000000015,49.1970505828678));
#202794=CARTESIAN_POINT('',(115.180610063791,0.550000000000015,48.9025624813381));
#202795=CARTESIAN_POINT('',(115.123367089922,1.05,49.1970505828678));
#202796=CARTESIAN_POINT('',(115.180610063791,1.05,48.9025624813381));
#202797=CARTESIAN_POINT('Origin',(115.180610063791,0.550000000000015,48.9025624813381));
#202798=CARTESIAN_POINT('',(114.689796561242,0.550000000000015,48.8071575248888));
#202799=CARTESIAN_POINT('',(114.632553587372,0.550000000000015,49.1016456264185));
#202800=CARTESIAN_POINT('',(114.689796561242,0.550000000000015,48.8071575248888));
#202801=CARTESIAN_POINT('',(115.123367089922,0.550000000000015,49.1970505828678));
#202802=CARTESIAN_POINT('',(115.180610063791,0.550000000000015,48.9025624813381));
#202803=CARTESIAN_POINT('Origin',(114.689796561242,0.550000000000015,48.8071575248888));
#202804=CARTESIAN_POINT('',(114.632553587372,0.550000000000015,49.1016456264185));
#202805=CARTESIAN_POINT('',(114.689796561242,0.550000000000015,48.8071575248888));
#202806=CARTESIAN_POINT('Origin',(114.689796561242,0.250000000000015,48.8071575248888));
#202807=CARTESIAN_POINT('',(115.180610063791,0.250000000000015,48.9025624813381));
#202808=CARTESIAN_POINT('',(115.123367089922,0.250000000000015,49.1970505828678));
#202809=CARTESIAN_POINT('',(115.180610063791,0.250000000000015,48.9025624813381));
#202810=CARTESIAN_POINT('',(114.632553587372,0.250000000000015,49.1016456264185));
#202811=CARTESIAN_POINT('',(114.632553587372,0.250000000000015,49.1016456264185));
#202812=CARTESIAN_POINT('',(114.689796561242,0.250000000000015,48.8071575248888));
#202813=CARTESIAN_POINT('',(114.689796561242,0.250000000000015,48.8071575248888));
#202814=CARTESIAN_POINT('',(114.689796561242,0.250000000000015,48.8071575248888));
#202815=CARTESIAN_POINT('Origin',(115.180610063791,0.250000000000015,48.9025624813381));
#202816=CARTESIAN_POINT('',(115.180610063791,-0.249999999999985,48.9025624813381));
#202817=CARTESIAN_POINT('',(115.123367089922,-0.249999999999985,49.1970505828678));
#202818=CARTESIAN_POINT('',(115.180610063791,-0.249999999999985,48.9025624813381));
#202819=CARTESIAN_POINT('',(115.123367089922,0.250000000000015,49.1970505828678));
#202820=CARTESIAN_POINT('',(115.180610063791,0.250000000000015,48.9025624813381));
#202821=CARTESIAN_POINT('Origin',(115.180610063791,-0.249999999999985,48.9025624813381));
#202822=CARTESIAN_POINT('',(114.689796561242,-0.249999999999985,48.8071575248888));
#202823=CARTESIAN_POINT('',(114.632553587372,-0.249999999999985,49.1016456264185));
#202824=CARTESIAN_POINT('',(114.689796561242,-0.249999999999985,48.8071575248888));
#202825=CARTESIAN_POINT('',(115.123367089922,-0.249999999999985,49.1970505828678));
#202826=CARTESIAN_POINT('',(115.180610063791,-0.249999999999985,48.9025624813381));
#202827=CARTESIAN_POINT('Origin',(114.689796561242,-0.249999999999985,48.8071575248888));
#202828=CARTESIAN_POINT('',(114.632553587372,-0.249999999999985,49.1016456264185));
#202829=CARTESIAN_POINT('',(114.689796561242,-0.249999999999985,48.8071575248888));
#202830=CARTESIAN_POINT('Origin',(114.689796561242,-0.549999999999986,48.8071575248888));
#202831=CARTESIAN_POINT('',(115.180610063791,-0.549999999999986,48.9025624813381));
#202832=CARTESIAN_POINT('',(115.123367089922,-0.549999999999986,49.1970505828678));
#202833=CARTESIAN_POINT('',(115.180610063791,-0.549999999999986,48.9025624813381));
#202834=CARTESIAN_POINT('',(114.632553587372,-0.549999999999986,49.1016456264185));
#202835=CARTESIAN_POINT('',(114.632553587372,-0.549999999999986,49.1016456264185));
#202836=CARTESIAN_POINT('',(114.689796561242,-0.549999999999986,48.8071575248888));
#202837=CARTESIAN_POINT('',(114.689796561242,-0.549999999999986,48.8071575248888));
#202838=CARTESIAN_POINT('',(114.689796561242,-0.549999999999986,48.8071575248888));
#202839=CARTESIAN_POINT('Origin',(115.180610063791,-0.549999999999986,48.9025624813381));
#202840=CARTESIAN_POINT('',(115.180610063791,-1.05,48.9025624813381));
#202841=CARTESIAN_POINT('',(115.123367089922,-1.05,49.1970505828678));
#202842=CARTESIAN_POINT('',(115.180610063791,-1.05,48.9025624813381));
#202843=CARTESIAN_POINT('',(115.123367089922,-0.549999999999986,49.1970505828678));
#202844=CARTESIAN_POINT('',(115.180610063791,-0.549999999999986,48.9025624813381));
#202845=CARTESIAN_POINT('Origin',(115.180610063791,-1.05,48.9025624813381));
#202846=CARTESIAN_POINT('',(114.689796561242,-1.05,48.8071575248888));
#202847=CARTESIAN_POINT('',(114.632553587372,-1.05,49.1016456264185));
#202848=CARTESIAN_POINT('',(114.689796561242,-1.05,48.8071575248888));
#202849=CARTESIAN_POINT('',(115.123367089922,-1.05,49.1970505828678));
#202850=CARTESIAN_POINT('',(115.180610063791,-1.05,48.9025624813381));
#202851=CARTESIAN_POINT('Origin',(114.689796561242,-1.05,48.8071575248888));
#202852=CARTESIAN_POINT('',(114.632553587372,-1.05,49.1016456264185));
#202853=CARTESIAN_POINT('',(114.689796561242,-1.05,48.8071575248888));
#202854=CARTESIAN_POINT('Origin',(114.689796561242,-1.35,48.8071575248888));
#202855=CARTESIAN_POINT('',(115.180610063791,-1.35,48.9025624813381));
#202856=CARTESIAN_POINT('',(115.123367089922,-1.35,49.1970505828678));
#202857=CARTESIAN_POINT('',(115.180610063791,-1.35,48.9025624813381));
#202858=CARTESIAN_POINT('',(114.632553587372,-1.35,49.1016456264185));
#202859=CARTESIAN_POINT('',(114.632553587372,-1.35,49.1016456264185));
#202860=CARTESIAN_POINT('',(114.689796561242,-1.35,48.8071575248888));
#202861=CARTESIAN_POINT('',(114.689796561242,-1.35,48.8071575248888));
#202862=CARTESIAN_POINT('',(114.689796561242,-1.35,48.8071575248888));
#202863=CARTESIAN_POINT('Origin',(115.180610063791,-1.35,48.9025624813381));
#202864=CARTESIAN_POINT('',(115.180610063791,-1.85,48.9025624813381));
#202865=CARTESIAN_POINT('',(115.123367089922,-1.85,49.1970505828678));
#202866=CARTESIAN_POINT('',(115.180610063791,-1.85,48.9025624813381));
#202867=CARTESIAN_POINT('',(115.123367089922,-1.35,49.1970505828678));
#202868=CARTESIAN_POINT('',(115.180610063791,-1.35,48.9025624813381));
#202869=CARTESIAN_POINT('Origin',(115.180610063791,-1.85,48.9025624813381));
#202870=CARTESIAN_POINT('',(114.689796561242,-1.85,48.8071575248888));
#202871=CARTESIAN_POINT('',(114.632553587372,-1.85,49.1016456264185));
#202872=CARTESIAN_POINT('',(114.689796561242,-1.85,48.8071575248888));
#202873=CARTESIAN_POINT('',(115.123367089922,-1.85,49.1970505828678));
#202874=CARTESIAN_POINT('',(115.180610063791,-1.85,48.9025624813381));
#202875=CARTESIAN_POINT('Origin',(114.689796561242,-1.85,48.8071575248888));
#202876=CARTESIAN_POINT('',(114.632553587372,-1.85,49.1016456264185));
#202877=CARTESIAN_POINT('',(114.689796561242,-1.85,48.8071575248888));
#202878=CARTESIAN_POINT('Origin',(114.689796561242,-2.15,48.8071575248888));
#202879=CARTESIAN_POINT('',(115.180610063791,-2.15,48.9025624813381));
#202880=CARTESIAN_POINT('',(115.123367089922,-2.15,49.1970505828678));
#202881=CARTESIAN_POINT('',(115.180610063791,-2.15,48.9025624813381));
#202882=CARTESIAN_POINT('',(114.632553587372,-2.15,49.1016456264185));
#202883=CARTESIAN_POINT('',(114.632553587372,-2.15,49.1016456264185));
#202884=CARTESIAN_POINT('',(114.689796561242,-2.15,48.8071575248888));
#202885=CARTESIAN_POINT('',(114.689796561242,-2.15,48.8071575248888));
#202886=CARTESIAN_POINT('',(114.689796561242,-2.15,48.8071575248888));
#202887=CARTESIAN_POINT('Origin',(115.180610063791,-2.15,48.9025624813381));
#202888=CARTESIAN_POINT('',(115.180610063791,-2.65,48.9025624813381));
#202889=CARTESIAN_POINT('',(115.123367089922,-2.65,49.1970505828678));
#202890=CARTESIAN_POINT('',(115.180610063791,-2.65,48.9025624813381));
#202891=CARTESIAN_POINT('',(115.123367089922,-2.15,49.1970505828678));
#202892=CARTESIAN_POINT('',(115.180610063791,-2.15,48.9025624813381));
#202893=CARTESIAN_POINT('Origin',(115.180610063791,-2.65,48.9025624813381));
#202894=CARTESIAN_POINT('',(114.689796561242,-2.65,48.8071575248888));
#202895=CARTESIAN_POINT('',(114.632553587372,-2.65,49.1016456264185));
#202896=CARTESIAN_POINT('',(114.689796561242,-2.65,48.8071575248888));
#202897=CARTESIAN_POINT('',(115.123367089922,-2.65,49.1970505828678));
#202898=CARTESIAN_POINT('',(115.180610063791,-2.65,48.9025624813381));
#202899=CARTESIAN_POINT('Origin',(114.689796561242,-2.65,48.8071575248888));
#202900=CARTESIAN_POINT('',(114.632553587372,-2.65,49.1016456264185));
#202901=CARTESIAN_POINT('',(114.689796561242,-2.65,48.8071575248888));
#202902=CARTESIAN_POINT('Origin',(115.475098165321,-2.15,48.9598054552076));
#202903=CARTESIAN_POINT('',(115.96591166787,-2.15,49.0552104116569));
#202904=CARTESIAN_POINT('',(115.908668694001,-2.15,49.3496985131866));
#202905=CARTESIAN_POINT('',(115.96591166787,-2.15,49.0552104116569));
#202906=CARTESIAN_POINT('',(115.417855191451,-2.15,49.2542935567373));
#202907=CARTESIAN_POINT('',(115.417855191451,-2.15,49.2542935567373));
#202908=CARTESIAN_POINT('',(115.475098165321,-2.15,48.9598054552076));
#202909=CARTESIAN_POINT('',(115.475098165321,-2.15,48.9598054552076));
#202910=CARTESIAN_POINT('',(115.475098165321,-2.15,48.9598054552076));
#202911=CARTESIAN_POINT('Origin',(115.96591166787,-2.15,49.0552104116569));
#202912=CARTESIAN_POINT('',(115.96591166787,-2.65,49.0552104116569));
#202913=CARTESIAN_POINT('',(115.908668694001,-2.65,49.3496985131866));
#202914=CARTESIAN_POINT('',(115.96591166787,-2.65,49.0552104116569));
#202915=CARTESIAN_POINT('',(115.908668694001,-2.15,49.3496985131866));
#202916=CARTESIAN_POINT('',(115.96591166787,-2.15,49.0552104116569));
#202917=CARTESIAN_POINT('Origin',(115.96591166787,-2.65,49.0552104116569));
#202918=CARTESIAN_POINT('',(115.475098165321,-2.65,48.9598054552076));
#202919=CARTESIAN_POINT('',(115.417855191451,-2.65,49.2542935567373));
#202920=CARTESIAN_POINT('',(115.475098165321,-2.65,48.9598054552076));
#202921=CARTESIAN_POINT('',(115.908668694001,-2.65,49.3496985131866));
#202922=CARTESIAN_POINT('',(115.96591166787,-2.65,49.0552104116569));
#202923=CARTESIAN_POINT('Origin',(115.475098165321,-2.65,48.9598054552076));
#202924=CARTESIAN_POINT('',(115.417855191451,-2.65,49.2542935567373));
#202925=CARTESIAN_POINT('',(115.475098165321,-2.65,48.9598054552076));
#202926=CARTESIAN_POINT('Origin',(116.2603997694,-2.15,49.1124533855264));
#202927=CARTESIAN_POINT('',(116.75121327195,-2.15,49.2078583419757));
#202928=CARTESIAN_POINT('',(116.69397029808,-2.15,49.5023464435054));
#202929=CARTESIAN_POINT('',(116.75121327195,-2.15,49.2078583419757));
#202930=CARTESIAN_POINT('',(116.203156795531,-2.15,49.4069414870561));
#202931=CARTESIAN_POINT('',(116.203156795531,-2.15,49.4069414870561));
#202932=CARTESIAN_POINT('',(116.2603997694,-2.15,49.1124533855264));
#202933=CARTESIAN_POINT('',(116.2603997694,-2.15,49.1124533855264));
#202934=CARTESIAN_POINT('',(116.2603997694,-2.15,49.1124533855264));
#202935=CARTESIAN_POINT('Origin',(116.75121327195,-2.15,49.2078583419757));
#202936=CARTESIAN_POINT('',(116.75121327195,-2.65,49.2078583419757));
#202937=CARTESIAN_POINT('',(116.69397029808,-2.65,49.5023464435054));
#202938=CARTESIAN_POINT('',(116.75121327195,-2.65,49.2078583419757));
#202939=CARTESIAN_POINT('',(116.69397029808,-2.15,49.5023464435054));
#202940=CARTESIAN_POINT('',(116.75121327195,-2.15,49.2078583419757));
#202941=CARTESIAN_POINT('Origin',(116.75121327195,-2.65,49.2078583419757));
#202942=CARTESIAN_POINT('',(116.2603997694,-2.65,49.1124533855264));
#202943=CARTESIAN_POINT('',(116.203156795531,-2.65,49.4069414870561));
#202944=CARTESIAN_POINT('',(116.2603997694,-2.65,49.1124533855264));
#202945=CARTESIAN_POINT('',(116.69397029808,-2.65,49.5023464435054));
#202946=CARTESIAN_POINT('',(116.75121327195,-2.65,49.2078583419757));
#202947=CARTESIAN_POINT('Origin',(116.2603997694,-2.65,49.1124533855264));
#202948=CARTESIAN_POINT('',(116.203156795531,-2.65,49.4069414870561));
#202949=CARTESIAN_POINT('',(116.2603997694,-2.65,49.1124533855264));
#202950=CARTESIAN_POINT('Origin',(117.045701373479,-2.15,49.2651013158452));
#202951=CARTESIAN_POINT('',(117.536514876029,-2.15,49.3605062722945));
#202952=CARTESIAN_POINT('',(117.479271902159,-2.15,49.6549943738242));
#202953=CARTESIAN_POINT('',(117.536514876029,-2.15,49.3605062722945));
#202954=CARTESIAN_POINT('',(116.98845839961,-2.15,49.5595894173749));
#202955=CARTESIAN_POINT('',(116.98845839961,-2.15,49.5595894173749));
#202956=CARTESIAN_POINT('',(117.045701373479,-2.15,49.2651013158452));
#202957=CARTESIAN_POINT('',(117.045701373479,-2.15,49.2651013158452));
#202958=CARTESIAN_POINT('',(117.045701373479,-2.15,49.2651013158452));
#202959=CARTESIAN_POINT('Origin',(117.536514876029,-2.15,49.3605062722945));
#202960=CARTESIAN_POINT('',(117.536514876029,-2.65,49.3605062722945));
#202961=CARTESIAN_POINT('',(117.479271902159,-2.65,49.6549943738242));
#202962=CARTESIAN_POINT('',(117.536514876029,-2.65,49.3605062722945));
#202963=CARTESIAN_POINT('',(117.479271902159,-2.15,49.6549943738242));
#202964=CARTESIAN_POINT('',(117.536514876029,-2.15,49.3605062722945));
#202965=CARTESIAN_POINT('Origin',(117.536514876029,-2.65,49.3605062722945));
#202966=CARTESIAN_POINT('',(117.045701373479,-2.65,49.2651013158452));
#202967=CARTESIAN_POINT('',(116.98845839961,-2.65,49.5595894173749));
#202968=CARTESIAN_POINT('',(117.045701373479,-2.65,49.2651013158452));
#202969=CARTESIAN_POINT('',(117.479271902159,-2.65,49.6549943738242));
#202970=CARTESIAN_POINT('',(117.536514876029,-2.65,49.3605062722945));
#202971=CARTESIAN_POINT('Origin',(117.045701373479,-2.65,49.2651013158452));
#202972=CARTESIAN_POINT('',(116.98845839961,-2.65,49.5595894173749));
#202973=CARTESIAN_POINT('',(117.045701373479,-2.65,49.2651013158452));
#202974=CARTESIAN_POINT('Origin',(117.831002977559,-2.15,49.417749246164));
#202975=CARTESIAN_POINT('',(118.321816480108,-2.15,49.5131542026133));
#202976=CARTESIAN_POINT('',(118.264573506239,-2.15,49.807642304143));
#202977=CARTESIAN_POINT('',(118.321816480108,-2.15,49.5131542026133));
#202978=CARTESIAN_POINT('',(117.773760003689,-2.15,49.7122373476937));
#202979=CARTESIAN_POINT('',(117.773760003689,-2.15,49.7122373476937));
#202980=CARTESIAN_POINT('',(117.831002977559,-2.15,49.417749246164));
#202981=CARTESIAN_POINT('',(117.831002977559,-2.15,49.417749246164));
#202982=CARTESIAN_POINT('',(117.831002977559,-2.15,49.417749246164));
#202983=CARTESIAN_POINT('Origin',(118.321816480108,-2.15,49.5131542026133));
#202984=CARTESIAN_POINT('',(118.321816480108,-2.65,49.5131542026133));
#202985=CARTESIAN_POINT('',(118.264573506239,-2.65,49.807642304143));
#202986=CARTESIAN_POINT('',(118.321816480108,-2.65,49.5131542026133));
#202987=CARTESIAN_POINT('',(118.264573506239,-2.15,49.807642304143));
#202988=CARTESIAN_POINT('',(118.321816480108,-2.15,49.5131542026133));
#202989=CARTESIAN_POINT('Origin',(118.321816480108,-2.65,49.5131542026133));
#202990=CARTESIAN_POINT('',(117.831002977559,-2.65,49.417749246164));
#202991=CARTESIAN_POINT('',(117.773760003689,-2.65,49.7122373476937));
#202992=CARTESIAN_POINT('',(117.831002977559,-2.65,49.417749246164));
#202993=CARTESIAN_POINT('',(118.264573506239,-2.65,49.807642304143));
#202994=CARTESIAN_POINT('',(118.321816480108,-2.65,49.5131542026133));
#202995=CARTESIAN_POINT('Origin',(117.831002977559,-2.65,49.417749246164));
#202996=CARTESIAN_POINT('',(117.773760003689,-2.65,49.7122373476937));
#202997=CARTESIAN_POINT('',(117.831002977559,-2.65,49.417749246164));
#202998=CARTESIAN_POINT('Origin',(118.616304581638,-2.15,49.5703971764828));
#202999=CARTESIAN_POINT('',(119.107118084187,-2.15,49.6658021329321));
#203000=CARTESIAN_POINT('',(119.049875110318,-2.15,49.9602902344618));
#203001=CARTESIAN_POINT('',(119.107118084187,-2.15,49.6658021329321));
#203002=CARTESIAN_POINT('',(118.559061607768,-2.15,49.8648852780125));
#203003=CARTESIAN_POINT('',(118.559061607768,-2.15,49.8648852780125));
#203004=CARTESIAN_POINT('',(118.616304581638,-2.15,49.5703971764828));
#203005=CARTESIAN_POINT('',(118.616304581638,-2.15,49.5703971764828));
#203006=CARTESIAN_POINT('',(118.616304581638,-2.15,49.5703971764828));
#203007=CARTESIAN_POINT('Origin',(119.107118084187,-2.15,49.6658021329321));
#203008=CARTESIAN_POINT('',(119.107118084187,-2.65,49.6658021329321));
#203009=CARTESIAN_POINT('',(119.049875110318,-2.65,49.9602902344618));
#203010=CARTESIAN_POINT('',(119.107118084187,-2.65,49.6658021329321));
#203011=CARTESIAN_POINT('',(119.049875110318,-2.15,49.9602902344618));
#203012=CARTESIAN_POINT('',(119.107118084187,-2.15,49.6658021329321));
#203013=CARTESIAN_POINT('Origin',(119.107118084187,-2.65,49.6658021329321));
#203014=CARTESIAN_POINT('',(118.616304581638,-2.65,49.5703971764828));
#203015=CARTESIAN_POINT('',(118.559061607768,-2.65,49.8648852780125));
#203016=CARTESIAN_POINT('',(118.616304581638,-2.65,49.5703971764828));
#203017=CARTESIAN_POINT('',(119.049875110318,-2.65,49.9602902344618));
#203018=CARTESIAN_POINT('',(119.107118084187,-2.65,49.6658021329321));
#203019=CARTESIAN_POINT('Origin',(118.616304581638,-2.65,49.5703971764828));
#203020=CARTESIAN_POINT('',(118.559061607768,-2.65,49.8648852780125));
#203021=CARTESIAN_POINT('',(118.616304581638,-2.65,49.5703971764828));
#203022=CARTESIAN_POINT('Origin',(119.401606185717,-2.15,49.7230451068016));
#203023=CARTESIAN_POINT('',(119.892419688267,-2.15,49.8184500632509));
#203024=CARTESIAN_POINT('',(119.835176714397,-2.15,50.1129381647806));
#203025=CARTESIAN_POINT('',(119.892419688267,-2.15,49.8184500632509));
#203026=CARTESIAN_POINT('',(119.344363211847,-2.15,50.0175332083313));
#203027=CARTESIAN_POINT('',(119.344363211847,-2.15,50.0175332083313));
#203028=CARTESIAN_POINT('',(119.401606185717,-2.15,49.7230451068016));
#203029=CARTESIAN_POINT('',(119.401606185717,-2.15,49.7230451068016));
#203030=CARTESIAN_POINT('',(119.401606185717,-2.15,49.7230451068016));
#203031=CARTESIAN_POINT('Origin',(119.892419688267,-2.15,49.8184500632509));
#203032=CARTESIAN_POINT('',(119.892419688267,-2.65,49.8184500632509));
#203033=CARTESIAN_POINT('',(119.835176714397,-2.65,50.1129381647806));
#203034=CARTESIAN_POINT('',(119.892419688267,-2.65,49.8184500632509));
#203035=CARTESIAN_POINT('',(119.835176714397,-2.15,50.1129381647806));
#203036=CARTESIAN_POINT('',(119.892419688267,-2.15,49.8184500632509));
#203037=CARTESIAN_POINT('Origin',(119.892419688267,-2.65,49.8184500632509));
#203038=CARTESIAN_POINT('',(119.401606185717,-2.65,49.7230451068016));
#203039=CARTESIAN_POINT('',(119.344363211847,-2.65,50.0175332083313));
#203040=CARTESIAN_POINT('',(119.401606185717,-2.65,49.7230451068016));
#203041=CARTESIAN_POINT('',(119.835176714397,-2.65,50.1129381647806));
#203042=CARTESIAN_POINT('',(119.892419688267,-2.65,49.8184500632509));
#203043=CARTESIAN_POINT('Origin',(119.401606185717,-2.65,49.7230451068016));
#203044=CARTESIAN_POINT('',(119.344363211847,-2.65,50.0175332083313));
#203045=CARTESIAN_POINT('',(119.401606185717,-2.65,49.7230451068016));
#203046=CARTESIAN_POINT('Origin',(119.401606185717,-1.35,49.7230451068016));
#203047=CARTESIAN_POINT('',(119.892419688267,-1.35,49.8184500632509));
#203048=CARTESIAN_POINT('',(119.835176714397,-1.35,50.1129381647806));
#203049=CARTESIAN_POINT('',(119.892419688267,-1.35,49.8184500632509));
#203050=CARTESIAN_POINT('',(119.344363211847,-1.35,50.0175332083313));
#203051=CARTESIAN_POINT('',(119.344363211847,-1.35,50.0175332083313));
#203052=CARTESIAN_POINT('',(119.401606185717,-1.35,49.7230451068016));
#203053=CARTESIAN_POINT('',(119.401606185717,-1.35,49.7230451068016));
#203054=CARTESIAN_POINT('',(119.401606185717,-1.35,49.7230451068016));
#203055=CARTESIAN_POINT('Origin',(119.892419688267,-1.35,49.8184500632509));
#203056=CARTESIAN_POINT('',(119.892419688267,-1.85,49.8184500632509));
#203057=CARTESIAN_POINT('',(119.835176714397,-1.85,50.1129381647806));
#203058=CARTESIAN_POINT('',(119.892419688267,-1.85,49.8184500632509));
#203059=CARTESIAN_POINT('',(119.835176714397,-1.35,50.1129381647806));
#203060=CARTESIAN_POINT('',(119.892419688267,-1.35,49.8184500632509));
#203061=CARTESIAN_POINT('Origin',(119.892419688267,-1.85,49.8184500632509));
#203062=CARTESIAN_POINT('',(119.401606185717,-1.85,49.7230451068016));
#203063=CARTESIAN_POINT('',(119.344363211847,-1.85,50.0175332083313));
#203064=CARTESIAN_POINT('',(119.401606185717,-1.85,49.7230451068016));
#203065=CARTESIAN_POINT('',(119.835176714397,-1.85,50.1129381647806));
#203066=CARTESIAN_POINT('',(119.892419688267,-1.85,49.8184500632509));
#203067=CARTESIAN_POINT('Origin',(119.401606185717,-1.85,49.7230451068016));
#203068=CARTESIAN_POINT('',(119.344363211847,-1.85,50.0175332083313));
#203069=CARTESIAN_POINT('',(119.401606185717,-1.85,49.7230451068016));
#203070=CARTESIAN_POINT('Origin',(119.401606185717,-0.549999999999986,49.7230451068016));
#203071=CARTESIAN_POINT('',(119.892419688267,-0.549999999999986,49.8184500632509));
#203072=CARTESIAN_POINT('',(119.835176714397,-0.549999999999986,50.1129381647806));
#203073=CARTESIAN_POINT('',(119.892419688267,-0.549999999999986,49.8184500632509));
#203074=CARTESIAN_POINT('',(119.344363211847,-0.549999999999986,50.0175332083313));
#203075=CARTESIAN_POINT('',(119.344363211847,-0.549999999999986,50.0175332083313));
#203076=CARTESIAN_POINT('',(119.401606185717,-0.549999999999986,49.7230451068016));
#203077=CARTESIAN_POINT('',(119.401606185717,-0.549999999999986,49.7230451068016));
#203078=CARTESIAN_POINT('',(119.401606185717,-0.549999999999986,49.7230451068016));
#203079=CARTESIAN_POINT('Origin',(119.892419688267,-0.549999999999986,49.8184500632509));
#203080=CARTESIAN_POINT('',(119.892419688267,-1.05,49.8184500632509));
#203081=CARTESIAN_POINT('',(119.835176714397,-1.05,50.1129381647806));
#203082=CARTESIAN_POINT('',(119.892419688267,-1.05,49.8184500632509));
#203083=CARTESIAN_POINT('',(119.835176714397,-0.549999999999986,50.1129381647806));
#203084=CARTESIAN_POINT('',(119.892419688267,-0.549999999999986,49.8184500632509));
#203085=CARTESIAN_POINT('Origin',(119.892419688267,-1.05,49.8184500632509));
#203086=CARTESIAN_POINT('',(119.401606185717,-1.05,49.7230451068016));
#203087=CARTESIAN_POINT('',(119.344363211847,-1.05,50.0175332083313));
#203088=CARTESIAN_POINT('',(119.401606185717,-1.05,49.7230451068016));
#203089=CARTESIAN_POINT('',(119.835176714397,-1.05,50.1129381647806));
#203090=CARTESIAN_POINT('',(119.892419688267,-1.05,49.8184500632509));
#203091=CARTESIAN_POINT('Origin',(119.401606185717,-1.05,49.7230451068016));
#203092=CARTESIAN_POINT('',(119.344363211847,-1.05,50.0175332083313));
#203093=CARTESIAN_POINT('',(119.401606185717,-1.05,49.7230451068016));
#203094=CARTESIAN_POINT('Origin',(119.401606185717,0.250000000000015,49.7230451068016));
#203095=CARTESIAN_POINT('',(119.892419688267,0.250000000000015,49.8184500632509));
#203096=CARTESIAN_POINT('',(119.835176714397,0.250000000000015,50.1129381647806));
#203097=CARTESIAN_POINT('',(119.892419688267,0.250000000000015,49.8184500632509));
#203098=CARTESIAN_POINT('',(119.344363211847,0.250000000000015,50.0175332083313));
#203099=CARTESIAN_POINT('',(119.344363211847,0.250000000000015,50.0175332083313));
#203100=CARTESIAN_POINT('',(119.401606185717,0.250000000000015,49.7230451068016));
#203101=CARTESIAN_POINT('',(119.401606185717,0.250000000000015,49.7230451068016));
#203102=CARTESIAN_POINT('',(119.401606185717,0.250000000000015,49.7230451068016));
#203103=CARTESIAN_POINT('Origin',(119.892419688267,0.250000000000015,49.8184500632509));
#203104=CARTESIAN_POINT('',(119.892419688267,-0.249999999999985,49.8184500632509));
#203105=CARTESIAN_POINT('',(119.835176714397,-0.249999999999985,50.1129381647806));
#203106=CARTESIAN_POINT('',(119.892419688267,-0.249999999999985,49.8184500632509));
#203107=CARTESIAN_POINT('',(119.835176714397,0.250000000000015,50.1129381647806));
#203108=CARTESIAN_POINT('',(119.892419688267,0.250000000000015,49.8184500632509));
#203109=CARTESIAN_POINT('Origin',(119.892419688267,-0.249999999999985,49.8184500632509));
#203110=CARTESIAN_POINT('',(119.401606185717,-0.249999999999985,49.7230451068016));
#203111=CARTESIAN_POINT('',(119.344363211847,-0.249999999999985,50.0175332083313));
#203112=CARTESIAN_POINT('',(119.401606185717,-0.249999999999985,49.7230451068016));
#203113=CARTESIAN_POINT('',(119.835176714397,-0.249999999999985,50.1129381647806));
#203114=CARTESIAN_POINT('',(119.892419688267,-0.249999999999985,49.8184500632509));
#203115=CARTESIAN_POINT('Origin',(119.401606185717,-0.249999999999985,49.7230451068016));
#203116=CARTESIAN_POINT('',(119.344363211847,-0.249999999999985,50.0175332083313));
#203117=CARTESIAN_POINT('',(119.401606185717,-0.249999999999985,49.7230451068016));
#203118=CARTESIAN_POINT('Origin',(119.401606185717,1.05,49.7230451068016));
#203119=CARTESIAN_POINT('',(119.892419688267,1.05,49.8184500632509));
#203120=CARTESIAN_POINT('',(119.835176714397,1.05,50.1129381647806));
#203121=CARTESIAN_POINT('',(119.892419688267,1.05,49.8184500632509));
#203122=CARTESIAN_POINT('',(119.344363211847,1.05,50.0175332083313));
#203123=CARTESIAN_POINT('',(119.344363211847,1.05,50.0175332083313));
#203124=CARTESIAN_POINT('',(119.401606185717,1.05,49.7230451068016));
#203125=CARTESIAN_POINT('',(119.401606185717,1.05,49.7230451068016));
#203126=CARTESIAN_POINT('',(119.401606185717,1.05,49.7230451068016));
#203127=CARTESIAN_POINT('Origin',(119.892419688267,1.05,49.8184500632509));
#203128=CARTESIAN_POINT('',(119.892419688267,0.550000000000015,49.8184500632509));
#203129=CARTESIAN_POINT('',(119.835176714397,0.550000000000015,50.1129381647806));
#203130=CARTESIAN_POINT('',(119.892419688267,0.550000000000015,49.8184500632509));
#203131=CARTESIAN_POINT('',(119.835176714397,1.05,50.1129381647806));
#203132=CARTESIAN_POINT('',(119.892419688267,1.05,49.8184500632509));
#203133=CARTESIAN_POINT('Origin',(119.892419688267,0.550000000000015,49.8184500632509));
#203134=CARTESIAN_POINT('',(119.401606185717,0.550000000000015,49.7230451068016));
#203135=CARTESIAN_POINT('',(119.344363211847,0.550000000000015,50.0175332083313));
#203136=CARTESIAN_POINT('',(119.401606185717,0.550000000000015,49.7230451068016));
#203137=CARTESIAN_POINT('',(119.835176714397,0.550000000000015,50.1129381647806));
#203138=CARTESIAN_POINT('',(119.892419688267,0.550000000000015,49.8184500632509));
#203139=CARTESIAN_POINT('Origin',(119.401606185717,0.550000000000015,49.7230451068016));
#203140=CARTESIAN_POINT('',(119.344363211847,0.550000000000015,50.0175332083313));
#203141=CARTESIAN_POINT('',(119.401606185717,0.550000000000015,49.7230451068016));
#203142=CARTESIAN_POINT('Origin',(119.401606185717,1.85,49.7230451068016));
#203143=CARTESIAN_POINT('',(119.892419688267,1.85,49.8184500632509));
#203144=CARTESIAN_POINT('',(119.835176714397,1.85,50.1129381647806));
#203145=CARTESIAN_POINT('',(119.892419688267,1.85,49.8184500632509));
#203146=CARTESIAN_POINT('',(119.344363211847,1.85,50.0175332083313));
#203147=CARTESIAN_POINT('',(119.344363211847,1.85,50.0175332083313));
#203148=CARTESIAN_POINT('',(119.401606185717,1.85,49.7230451068016));
#203149=CARTESIAN_POINT('',(119.401606185717,1.85,49.7230451068016));
#203150=CARTESIAN_POINT('',(119.401606185717,1.85,49.7230451068016));
#203151=CARTESIAN_POINT('Origin',(119.892419688267,1.85,49.8184500632509));
#203152=CARTESIAN_POINT('',(119.892419688267,1.35,49.8184500632509));
#203153=CARTESIAN_POINT('',(119.835176714397,1.35,50.1129381647806));
#203154=CARTESIAN_POINT('',(119.892419688267,1.35,49.8184500632509));
#203155=CARTESIAN_POINT('',(119.835176714397,1.85,50.1129381647806));
#203156=CARTESIAN_POINT('',(119.892419688267,1.85,49.8184500632509));
#203157=CARTESIAN_POINT('Origin',(119.892419688267,1.35,49.8184500632509));
#203158=CARTESIAN_POINT('',(119.401606185717,1.35,49.7230451068016));
#203159=CARTESIAN_POINT('',(119.344363211847,1.35,50.0175332083313));
#203160=CARTESIAN_POINT('',(119.401606185717,1.35,49.7230451068016));
#203161=CARTESIAN_POINT('',(119.835176714397,1.35,50.1129381647806));
#203162=CARTESIAN_POINT('',(119.892419688267,1.35,49.8184500632509));
#203163=CARTESIAN_POINT('Origin',(119.401606185717,1.35,49.7230451068016));
#203164=CARTESIAN_POINT('',(119.344363211847,1.35,50.0175332083313));
#203165=CARTESIAN_POINT('',(119.401606185717,1.35,49.7230451068016));
#203166=CARTESIAN_POINT('Origin',(119.401606185717,2.65,49.7230451068016));
#203167=CARTESIAN_POINT('',(119.892419688267,2.65,49.8184500632509));
#203168=CARTESIAN_POINT('',(119.835176714397,2.65,50.1129381647806));
#203169=CARTESIAN_POINT('',(119.892419688267,2.65,49.8184500632509));
#203170=CARTESIAN_POINT('',(119.344363211847,2.65,50.0175332083313));
#203171=CARTESIAN_POINT('',(119.344363211847,2.65,50.0175332083313));
#203172=CARTESIAN_POINT('',(119.401606185717,2.65,49.7230451068016));
#203173=CARTESIAN_POINT('',(119.401606185717,2.65,49.7230451068016));
#203174=CARTESIAN_POINT('',(119.401606185717,2.65,49.7230451068016));
#203175=CARTESIAN_POINT('Origin',(119.892419688267,2.65,49.8184500632509));
#203176=CARTESIAN_POINT('',(119.892419688267,2.15,49.8184500632509));
#203177=CARTESIAN_POINT('',(119.835176714397,2.15,50.1129381647806));
#203178=CARTESIAN_POINT('',(119.892419688267,2.15,49.8184500632509));
#203179=CARTESIAN_POINT('',(119.835176714397,2.65,50.1129381647806));
#203180=CARTESIAN_POINT('',(119.892419688267,2.65,49.8184500632509));
#203181=CARTESIAN_POINT('Origin',(119.892419688267,2.15,49.8184500632509));
#203182=CARTESIAN_POINT('',(119.401606185717,2.15,49.7230451068016));
#203183=CARTESIAN_POINT('',(119.344363211847,2.15,50.0175332083313));
#203184=CARTESIAN_POINT('',(119.401606185717,2.15,49.7230451068016));
#203185=CARTESIAN_POINT('',(119.835176714397,2.15,50.1129381647806));
#203186=CARTESIAN_POINT('',(119.892419688267,2.15,49.8184500632509));
#203187=CARTESIAN_POINT('Origin',(119.401606185717,2.15,49.7230451068016));
#203188=CARTESIAN_POINT('',(119.344363211847,2.15,50.0175332083313));
#203189=CARTESIAN_POINT('',(119.401606185717,2.15,49.7230451068016));
#203190=CARTESIAN_POINT('Origin',(118.616304581638,2.65,49.5703971764828));
#203191=CARTESIAN_POINT('',(119.107118084187,2.65,49.6658021329321));
#203192=CARTESIAN_POINT('',(119.049875110318,2.65,49.9602902344618));
#203193=CARTESIAN_POINT('',(119.107118084187,2.65,49.6658021329321));
#203194=CARTESIAN_POINT('',(118.559061607768,2.65,49.8648852780125));
#203195=CARTESIAN_POINT('',(118.559061607768,2.65,49.8648852780125));
#203196=CARTESIAN_POINT('',(118.616304581638,2.65,49.5703971764828));
#203197=CARTESIAN_POINT('',(118.616304581638,2.65,49.5703971764828));
#203198=CARTESIAN_POINT('',(118.616304581638,2.65,49.5703971764828));
#203199=CARTESIAN_POINT('Origin',(119.107118084187,2.65,49.6658021329321));
#203200=CARTESIAN_POINT('',(119.107118084187,2.15,49.6658021329321));
#203201=CARTESIAN_POINT('',(119.049875110318,2.15,49.9602902344618));
#203202=CARTESIAN_POINT('',(119.107118084187,2.15,49.6658021329321));
#203203=CARTESIAN_POINT('',(119.049875110318,2.65,49.9602902344618));
#203204=CARTESIAN_POINT('',(119.107118084187,2.65,49.6658021329321));
#203205=CARTESIAN_POINT('Origin',(119.107118084187,2.15,49.6658021329321));
#203206=CARTESIAN_POINT('',(118.616304581638,2.15,49.5703971764828));
#203207=CARTESIAN_POINT('',(118.559061607768,2.15,49.8648852780125));
#203208=CARTESIAN_POINT('',(118.616304581638,2.15,49.5703971764828));
#203209=CARTESIAN_POINT('',(119.049875110318,2.15,49.9602902344618));
#203210=CARTESIAN_POINT('',(119.107118084187,2.15,49.6658021329321));
#203211=CARTESIAN_POINT('Origin',(118.616304581638,2.15,49.5703971764828));
#203212=CARTESIAN_POINT('',(118.559061607768,2.15,49.8648852780125));
#203213=CARTESIAN_POINT('',(118.616304581638,2.15,49.5703971764828));
#203214=CARTESIAN_POINT('Origin',(117.831002977559,2.65,49.417749246164));
#203215=CARTESIAN_POINT('',(118.321816480108,2.65,49.5131542026133));
#203216=CARTESIAN_POINT('',(118.264573506239,2.65,49.807642304143));
#203217=CARTESIAN_POINT('',(118.321816480108,2.65,49.5131542026133));
#203218=CARTESIAN_POINT('',(117.773760003689,2.65,49.7122373476937));
#203219=CARTESIAN_POINT('',(117.773760003689,2.65,49.7122373476937));
#203220=CARTESIAN_POINT('',(117.831002977559,2.65,49.417749246164));
#203221=CARTESIAN_POINT('',(117.831002977559,2.65,49.417749246164));
#203222=CARTESIAN_POINT('',(117.831002977559,2.65,49.417749246164));
#203223=CARTESIAN_POINT('Origin',(118.321816480108,2.65,49.5131542026133));
#203224=CARTESIAN_POINT('',(118.321816480108,2.15,49.5131542026133));
#203225=CARTESIAN_POINT('',(118.264573506239,2.15,49.807642304143));
#203226=CARTESIAN_POINT('',(118.321816480108,2.15,49.5131542026133));
#203227=CARTESIAN_POINT('',(118.264573506239,2.65,49.807642304143));
#203228=CARTESIAN_POINT('',(118.321816480108,2.65,49.5131542026133));
#203229=CARTESIAN_POINT('Origin',(118.321816480108,2.15,49.5131542026133));
#203230=CARTESIAN_POINT('',(117.831002977559,2.15,49.417749246164));
#203231=CARTESIAN_POINT('',(117.773760003689,2.15,49.7122373476937));
#203232=CARTESIAN_POINT('',(117.831002977559,2.15,49.417749246164));
#203233=CARTESIAN_POINT('',(118.264573506239,2.15,49.807642304143));
#203234=CARTESIAN_POINT('',(118.321816480108,2.15,49.5131542026133));
#203235=CARTESIAN_POINT('Origin',(117.831002977559,2.15,49.417749246164));
#203236=CARTESIAN_POINT('',(117.773760003689,2.15,49.7122373476937));
#203237=CARTESIAN_POINT('',(117.831002977559,2.15,49.417749246164));
#203238=CARTESIAN_POINT('Origin',(117.045701373479,2.65,49.2651013158452));
#203239=CARTESIAN_POINT('',(117.536514876029,2.65,49.3605062722945));
#203240=CARTESIAN_POINT('',(117.479271902159,2.65,49.6549943738242));
#203241=CARTESIAN_POINT('',(117.536514876029,2.65,49.3605062722945));
#203242=CARTESIAN_POINT('',(116.98845839961,2.65,49.5595894173749));
#203243=CARTESIAN_POINT('',(116.98845839961,2.65,49.5595894173749));
#203244=CARTESIAN_POINT('',(117.045701373479,2.65,49.2651013158452));
#203245=CARTESIAN_POINT('',(117.045701373479,2.65,49.2651013158452));
#203246=CARTESIAN_POINT('',(117.045701373479,2.65,49.2651013158452));
#203247=CARTESIAN_POINT('Origin',(117.536514876029,2.65,49.3605062722945));
#203248=CARTESIAN_POINT('',(117.536514876029,2.15,49.3605062722945));
#203249=CARTESIAN_POINT('',(117.479271902159,2.15,49.6549943738242));
#203250=CARTESIAN_POINT('',(117.536514876029,2.15,49.3605062722945));
#203251=CARTESIAN_POINT('',(117.479271902159,2.65,49.6549943738242));
#203252=CARTESIAN_POINT('',(117.536514876029,2.65,49.3605062722945));
#203253=CARTESIAN_POINT('Origin',(117.536514876029,2.15,49.3605062722945));
#203254=CARTESIAN_POINT('',(117.045701373479,2.15,49.2651013158452));
#203255=CARTESIAN_POINT('',(116.98845839961,2.15,49.5595894173749));
#203256=CARTESIAN_POINT('',(117.045701373479,2.15,49.2651013158452));
#203257=CARTESIAN_POINT('',(117.479271902159,2.15,49.6549943738242));
#203258=CARTESIAN_POINT('',(117.536514876029,2.15,49.3605062722945));
#203259=CARTESIAN_POINT('Origin',(117.045701373479,2.15,49.2651013158452));
#203260=CARTESIAN_POINT('',(116.98845839961,2.15,49.5595894173749));
#203261=CARTESIAN_POINT('',(117.045701373479,2.15,49.2651013158452));
#203262=CARTESIAN_POINT('Origin',(116.2603997694,2.65,49.1124533855264));
#203263=CARTESIAN_POINT('',(116.75121327195,2.65,49.2078583419757));
#203264=CARTESIAN_POINT('',(116.69397029808,2.65,49.5023464435054));
#203265=CARTESIAN_POINT('',(116.75121327195,2.65,49.2078583419757));
#203266=CARTESIAN_POINT('',(116.203156795531,2.65,49.4069414870561));
#203267=CARTESIAN_POINT('',(116.203156795531,2.65,49.4069414870561));
#203268=CARTESIAN_POINT('',(116.2603997694,2.65,49.1124533855264));
#203269=CARTESIAN_POINT('',(116.2603997694,2.65,49.1124533855264));
#203270=CARTESIAN_POINT('',(116.2603997694,2.65,49.1124533855264));
#203271=CARTESIAN_POINT('Origin',(116.75121327195,2.65,49.2078583419757));
#203272=CARTESIAN_POINT('',(116.75121327195,2.15,49.2078583419757));
#203273=CARTESIAN_POINT('',(116.69397029808,2.15,49.5023464435054));
#203274=CARTESIAN_POINT('',(116.75121327195,2.15,49.2078583419757));
#203275=CARTESIAN_POINT('',(116.69397029808,2.65,49.5023464435054));
#203276=CARTESIAN_POINT('',(116.75121327195,2.65,49.2078583419757));
#203277=CARTESIAN_POINT('Origin',(116.75121327195,2.15,49.2078583419757));
#203278=CARTESIAN_POINT('',(116.2603997694,2.15,49.1124533855264));
#203279=CARTESIAN_POINT('',(116.203156795531,2.15,49.4069414870561));
#203280=CARTESIAN_POINT('',(116.2603997694,2.15,49.1124533855264));
#203281=CARTESIAN_POINT('',(116.69397029808,2.15,49.5023464435054));
#203282=CARTESIAN_POINT('',(116.75121327195,2.15,49.2078583419757));
#203283=CARTESIAN_POINT('Origin',(116.2603997694,2.15,49.1124533855264));
#203284=CARTESIAN_POINT('',(116.203156795531,2.15,49.4069414870561));
#203285=CARTESIAN_POINT('',(116.2603997694,2.15,49.1124533855264));
#203286=CARTESIAN_POINT('Origin',(115.475098165321,2.65,48.9598054552076));
#203287=CARTESIAN_POINT('',(115.96591166787,2.65,49.0552104116569));
#203288=CARTESIAN_POINT('',(115.908668694001,2.65,49.3496985131866));
#203289=CARTESIAN_POINT('',(115.96591166787,2.65,49.0552104116569));
#203290=CARTESIAN_POINT('',(115.417855191451,2.65,49.2542935567373));
#203291=CARTESIAN_POINT('',(115.417855191451,2.65,49.2542935567373));
#203292=CARTESIAN_POINT('',(115.475098165321,2.65,48.9598054552076));
#203293=CARTESIAN_POINT('',(115.475098165321,2.65,48.9598054552076));
#203294=CARTESIAN_POINT('',(115.475098165321,2.65,48.9598054552076));
#203295=CARTESIAN_POINT('Origin',(115.96591166787,2.65,49.0552104116569));
#203296=CARTESIAN_POINT('',(115.96591166787,2.15,49.0552104116569));
#203297=CARTESIAN_POINT('',(115.908668694001,2.15,49.3496985131866));
#203298=CARTESIAN_POINT('',(115.96591166787,2.15,49.0552104116569));
#203299=CARTESIAN_POINT('',(115.908668694001,2.65,49.3496985131866));
#203300=CARTESIAN_POINT('',(115.96591166787,2.65,49.0552104116569));
#203301=CARTESIAN_POINT('Origin',(115.96591166787,2.15,49.0552104116569));
#203302=CARTESIAN_POINT('',(115.475098165321,2.15,48.9598054552076));
#203303=CARTESIAN_POINT('',(115.417855191451,2.15,49.2542935567373));
#203304=CARTESIAN_POINT('',(115.475098165321,2.15,48.9598054552076));
#203305=CARTESIAN_POINT('',(115.908668694001,2.15,49.3496985131866));
#203306=CARTESIAN_POINT('',(115.96591166787,2.15,49.0552104116569));
#203307=CARTESIAN_POINT('Origin',(115.475098165321,2.15,48.9598054552076));
#203308=CARTESIAN_POINT('',(115.417855191451,2.15,49.2542935567373));
#203309=CARTESIAN_POINT('',(115.475098165321,2.15,48.9598054552076));
#203310=CARTESIAN_POINT('Origin',(115.475098165321,1.85,48.9598054552076));
#203311=CARTESIAN_POINT('',(115.96591166787,1.85,49.0552104116569));
#203312=CARTESIAN_POINT('',(115.908668694001,1.85,49.3496985131866));
#203313=CARTESIAN_POINT('',(115.96591166787,1.85,49.0552104116569));
#203314=CARTESIAN_POINT('',(115.417855191451,1.85,49.2542935567373));
#203315=CARTESIAN_POINT('',(115.417855191451,1.85,49.2542935567373));
#203316=CARTESIAN_POINT('',(115.475098165321,1.85,48.9598054552076));
#203317=CARTESIAN_POINT('',(115.475098165321,1.85,48.9598054552076));
#203318=CARTESIAN_POINT('',(115.475098165321,1.85,48.9598054552076));
#203319=CARTESIAN_POINT('Origin',(115.96591166787,1.85,49.0552104116569));
#203320=CARTESIAN_POINT('',(115.96591166787,1.35,49.0552104116569));
#203321=CARTESIAN_POINT('',(115.908668694001,1.35,49.3496985131866));
#203322=CARTESIAN_POINT('',(115.96591166787,1.35,49.0552104116569));
#203323=CARTESIAN_POINT('',(115.908668694001,1.85,49.3496985131866));
#203324=CARTESIAN_POINT('',(115.96591166787,1.85,49.0552104116569));
#203325=CARTESIAN_POINT('Origin',(115.96591166787,1.35,49.0552104116569));
#203326=CARTESIAN_POINT('',(115.475098165321,1.35,48.9598054552076));
#203327=CARTESIAN_POINT('',(115.417855191451,1.35,49.2542935567373));
#203328=CARTESIAN_POINT('',(115.475098165321,1.35,48.9598054552076));
#203329=CARTESIAN_POINT('',(115.908668694001,1.35,49.3496985131866));
#203330=CARTESIAN_POINT('',(115.96591166787,1.35,49.0552104116569));
#203331=CARTESIAN_POINT('Origin',(115.475098165321,1.35,48.9598054552076));
#203332=CARTESIAN_POINT('',(115.417855191451,1.35,49.2542935567373));
#203333=CARTESIAN_POINT('',(115.475098165321,1.35,48.9598054552076));
#203334=CARTESIAN_POINT('Origin',(115.475098165321,1.05,48.9598054552076));
#203335=CARTESIAN_POINT('',(115.96591166787,1.05,49.0552104116569));
#203336=CARTESIAN_POINT('',(115.908668694001,1.05,49.3496985131866));
#203337=CARTESIAN_POINT('',(115.96591166787,1.05,49.0552104116569));
#203338=CARTESIAN_POINT('',(115.417855191451,1.05,49.2542935567373));
#203339=CARTESIAN_POINT('',(115.417855191451,1.05,49.2542935567373));
#203340=CARTESIAN_POINT('',(115.475098165321,1.05,48.9598054552076));
#203341=CARTESIAN_POINT('',(115.475098165321,1.05,48.9598054552076));
#203342=CARTESIAN_POINT('',(115.475098165321,1.05,48.9598054552076));
#203343=CARTESIAN_POINT('Origin',(115.96591166787,1.05,49.0552104116569));
#203344=CARTESIAN_POINT('',(115.96591166787,0.550000000000015,49.0552104116569));
#203345=CARTESIAN_POINT('',(115.908668694001,0.550000000000015,49.3496985131866));
#203346=CARTESIAN_POINT('',(115.96591166787,0.550000000000015,49.0552104116569));
#203347=CARTESIAN_POINT('',(115.908668694001,1.05,49.3496985131866));
#203348=CARTESIAN_POINT('',(115.96591166787,1.05,49.0552104116569));
#203349=CARTESIAN_POINT('Origin',(115.96591166787,0.550000000000015,49.0552104116569));
#203350=CARTESIAN_POINT('',(115.475098165321,0.550000000000015,48.9598054552076));
#203351=CARTESIAN_POINT('',(115.417855191451,0.550000000000015,49.2542935567373));
#203352=CARTESIAN_POINT('',(115.475098165321,0.550000000000015,48.9598054552076));
#203353=CARTESIAN_POINT('',(115.908668694001,0.550000000000015,49.3496985131866));
#203354=CARTESIAN_POINT('',(115.96591166787,0.550000000000015,49.0552104116569));
#203355=CARTESIAN_POINT('Origin',(115.475098165321,0.550000000000015,48.9598054552076));
#203356=CARTESIAN_POINT('',(115.417855191451,0.550000000000015,49.2542935567373));
#203357=CARTESIAN_POINT('',(115.475098165321,0.550000000000015,48.9598054552076));
#203358=CARTESIAN_POINT('Origin',(115.475098165321,0.250000000000015,48.9598054552076));
#203359=CARTESIAN_POINT('',(115.96591166787,0.250000000000015,49.0552104116569));
#203360=CARTESIAN_POINT('',(115.908668694001,0.250000000000015,49.3496985131866));
#203361=CARTESIAN_POINT('',(115.96591166787,0.250000000000015,49.0552104116569));
#203362=CARTESIAN_POINT('',(115.417855191451,0.250000000000015,49.2542935567373));
#203363=CARTESIAN_POINT('',(115.417855191451,0.250000000000015,49.2542935567373));
#203364=CARTESIAN_POINT('',(115.475098165321,0.250000000000015,48.9598054552076));
#203365=CARTESIAN_POINT('',(115.475098165321,0.250000000000015,48.9598054552076));
#203366=CARTESIAN_POINT('',(115.475098165321,0.250000000000015,48.9598054552076));
#203367=CARTESIAN_POINT('Origin',(115.96591166787,0.250000000000015,49.0552104116569));
#203368=CARTESIAN_POINT('',(115.96591166787,-0.249999999999985,49.0552104116569));
#203369=CARTESIAN_POINT('',(115.908668694001,-0.249999999999985,49.3496985131866));
#203370=CARTESIAN_POINT('',(115.96591166787,-0.249999999999985,49.0552104116569));
#203371=CARTESIAN_POINT('',(115.908668694001,0.250000000000015,49.3496985131866));
#203372=CARTESIAN_POINT('',(115.96591166787,0.250000000000015,49.0552104116569));
#203373=CARTESIAN_POINT('Origin',(115.96591166787,-0.249999999999985,49.0552104116569));
#203374=CARTESIAN_POINT('',(115.475098165321,-0.249999999999985,48.9598054552076));
#203375=CARTESIAN_POINT('',(115.417855191451,-0.249999999999985,49.2542935567373));
#203376=CARTESIAN_POINT('',(115.475098165321,-0.249999999999985,48.9598054552076));
#203377=CARTESIAN_POINT('',(115.908668694001,-0.249999999999985,49.3496985131866));
#203378=CARTESIAN_POINT('',(115.96591166787,-0.249999999999985,49.0552104116569));
#203379=CARTESIAN_POINT('Origin',(115.475098165321,-0.249999999999985,48.9598054552076));
#203380=CARTESIAN_POINT('',(115.417855191451,-0.249999999999985,49.2542935567373));
#203381=CARTESIAN_POINT('',(115.475098165321,-0.249999999999985,48.9598054552076));
#203382=CARTESIAN_POINT('Origin',(115.475098165321,-0.549999999999986,48.9598054552076));
#203383=CARTESIAN_POINT('',(115.96591166787,-0.549999999999986,49.0552104116569));
#203384=CARTESIAN_POINT('',(115.908668694001,-0.549999999999986,49.3496985131866));
#203385=CARTESIAN_POINT('',(115.96591166787,-0.549999999999986,49.0552104116569));
#203386=CARTESIAN_POINT('',(115.417855191451,-0.549999999999986,49.2542935567373));
#203387=CARTESIAN_POINT('',(115.417855191451,-0.549999999999986,49.2542935567373));
#203388=CARTESIAN_POINT('',(115.475098165321,-0.549999999999986,48.9598054552076));
#203389=CARTESIAN_POINT('',(115.475098165321,-0.549999999999986,48.9598054552076));
#203390=CARTESIAN_POINT('',(115.475098165321,-0.549999999999986,48.9598054552076));
#203391=CARTESIAN_POINT('Origin',(115.96591166787,-0.549999999999986,49.0552104116569));
#203392=CARTESIAN_POINT('',(115.96591166787,-1.05,49.0552104116569));
#203393=CARTESIAN_POINT('',(115.908668694001,-1.05,49.3496985131866));
#203394=CARTESIAN_POINT('',(115.96591166787,-1.05,49.0552104116569));
#203395=CARTESIAN_POINT('',(115.908668694001,-0.549999999999986,49.3496985131866));
#203396=CARTESIAN_POINT('',(115.96591166787,-0.549999999999986,49.0552104116569));
#203397=CARTESIAN_POINT('Origin',(115.96591166787,-1.05,49.0552104116569));
#203398=CARTESIAN_POINT('',(115.475098165321,-1.05,48.9598054552076));
#203399=CARTESIAN_POINT('',(115.417855191451,-1.05,49.2542935567373));
#203400=CARTESIAN_POINT('',(115.475098165321,-1.05,48.9598054552076));
#203401=CARTESIAN_POINT('',(115.908668694001,-1.05,49.3496985131866));
#203402=CARTESIAN_POINT('',(115.96591166787,-1.05,49.0552104116569));
#203403=CARTESIAN_POINT('Origin',(115.475098165321,-1.05,48.9598054552076));
#203404=CARTESIAN_POINT('',(115.417855191451,-1.05,49.2542935567373));
#203405=CARTESIAN_POINT('',(115.475098165321,-1.05,48.9598054552076));
#203406=CARTESIAN_POINT('Origin',(115.475098165321,-1.35,48.9598054552076));
#203407=CARTESIAN_POINT('',(115.96591166787,-1.35,49.0552104116569));
#203408=CARTESIAN_POINT('',(115.908668694001,-1.35,49.3496985131866));
#203409=CARTESIAN_POINT('',(115.96591166787,-1.35,49.0552104116569));
#203410=CARTESIAN_POINT('',(115.417855191451,-1.35,49.2542935567373));
#203411=CARTESIAN_POINT('',(115.417855191451,-1.35,49.2542935567373));
#203412=CARTESIAN_POINT('',(115.475098165321,-1.35,48.9598054552076));
#203413=CARTESIAN_POINT('',(115.475098165321,-1.35,48.9598054552076));
#203414=CARTESIAN_POINT('',(115.475098165321,-1.35,48.9598054552076));
#203415=CARTESIAN_POINT('Origin',(115.96591166787,-1.35,49.0552104116569));
#203416=CARTESIAN_POINT('',(115.96591166787,-1.85,49.0552104116569));
#203417=CARTESIAN_POINT('',(115.908668694001,-1.85,49.3496985131866));
#203418=CARTESIAN_POINT('',(115.96591166787,-1.85,49.0552104116569));
#203419=CARTESIAN_POINT('',(115.908668694001,-1.35,49.3496985131866));
#203420=CARTESIAN_POINT('',(115.96591166787,-1.35,49.0552104116569));
#203421=CARTESIAN_POINT('Origin',(115.96591166787,-1.85,49.0552104116569));
#203422=CARTESIAN_POINT('',(115.475098165321,-1.85,48.9598054552076));
#203423=CARTESIAN_POINT('',(115.417855191451,-1.85,49.2542935567373));
#203424=CARTESIAN_POINT('',(115.475098165321,-1.85,48.9598054552076));
#203425=CARTESIAN_POINT('',(115.908668694001,-1.85,49.3496985131866));
#203426=CARTESIAN_POINT('',(115.96591166787,-1.85,49.0552104116569));
#203427=CARTESIAN_POINT('Origin',(115.475098165321,-1.85,48.9598054552076));
#203428=CARTESIAN_POINT('',(115.417855191451,-1.85,49.2542935567373));
#203429=CARTESIAN_POINT('',(115.475098165321,-1.85,48.9598054552076));
#203430=CARTESIAN_POINT('Origin',(116.2603997694,-1.35,49.1124533855264));
#203431=CARTESIAN_POINT('',(116.75121327195,-1.35,49.2078583419757));
#203432=CARTESIAN_POINT('',(116.69397029808,-1.35,49.5023464435054));
#203433=CARTESIAN_POINT('',(116.75121327195,-1.35,49.2078583419757));
#203434=CARTESIAN_POINT('',(116.203156795531,-1.35,49.4069414870561));
#203435=CARTESIAN_POINT('',(116.203156795531,-1.35,49.4069414870561));
#203436=CARTESIAN_POINT('',(116.2603997694,-1.35,49.1124533855264));
#203437=CARTESIAN_POINT('',(116.2603997694,-1.35,49.1124533855264));
#203438=CARTESIAN_POINT('',(116.2603997694,-1.35,49.1124533855264));
#203439=CARTESIAN_POINT('Origin',(116.75121327195,-1.35,49.2078583419757));
#203440=CARTESIAN_POINT('',(116.75121327195,-1.85,49.2078583419757));
#203441=CARTESIAN_POINT('',(116.69397029808,-1.85,49.5023464435054));
#203442=CARTESIAN_POINT('',(116.75121327195,-1.85,49.2078583419757));
#203443=CARTESIAN_POINT('',(116.69397029808,-1.35,49.5023464435054));
#203444=CARTESIAN_POINT('',(116.75121327195,-1.35,49.2078583419757));
#203445=CARTESIAN_POINT('Origin',(116.75121327195,-1.85,49.2078583419757));
#203446=CARTESIAN_POINT('',(116.2603997694,-1.85,49.1124533855264));
#203447=CARTESIAN_POINT('',(116.203156795531,-1.85,49.4069414870561));
#203448=CARTESIAN_POINT('',(116.2603997694,-1.85,49.1124533855264));
#203449=CARTESIAN_POINT('',(116.69397029808,-1.85,49.5023464435054));
#203450=CARTESIAN_POINT('',(116.75121327195,-1.85,49.2078583419757));
#203451=CARTESIAN_POINT('Origin',(116.2603997694,-1.85,49.1124533855264));
#203452=CARTESIAN_POINT('',(116.203156795531,-1.85,49.4069414870561));
#203453=CARTESIAN_POINT('',(116.2603997694,-1.85,49.1124533855264));
#203454=CARTESIAN_POINT('Origin',(117.045701373479,-1.35,49.2651013158452));
#203455=CARTESIAN_POINT('',(117.536514876029,-1.35,49.3605062722945));
#203456=CARTESIAN_POINT('',(117.479271902159,-1.35,49.6549943738242));
#203457=CARTESIAN_POINT('',(117.536514876029,-1.35,49.3605062722945));
#203458=CARTESIAN_POINT('',(116.98845839961,-1.35,49.5595894173749));
#203459=CARTESIAN_POINT('',(116.98845839961,-1.35,49.5595894173749));
#203460=CARTESIAN_POINT('',(117.045701373479,-1.35,49.2651013158452));
#203461=CARTESIAN_POINT('',(117.045701373479,-1.35,49.2651013158452));
#203462=CARTESIAN_POINT('',(117.045701373479,-1.35,49.2651013158452));
#203463=CARTESIAN_POINT('Origin',(117.536514876029,-1.35,49.3605062722945));
#203464=CARTESIAN_POINT('',(117.536514876029,-1.85,49.3605062722945));
#203465=CARTESIAN_POINT('',(117.479271902159,-1.85,49.6549943738242));
#203466=CARTESIAN_POINT('',(117.536514876029,-1.85,49.3605062722945));
#203467=CARTESIAN_POINT('',(117.479271902159,-1.35,49.6549943738242));
#203468=CARTESIAN_POINT('',(117.536514876029,-1.35,49.3605062722945));
#203469=CARTESIAN_POINT('Origin',(117.536514876029,-1.85,49.3605062722945));
#203470=CARTESIAN_POINT('',(117.045701373479,-1.85,49.2651013158452));
#203471=CARTESIAN_POINT('',(116.98845839961,-1.85,49.5595894173749));
#203472=CARTESIAN_POINT('',(117.045701373479,-1.85,49.2651013158452));
#203473=CARTESIAN_POINT('',(117.479271902159,-1.85,49.6549943738242));
#203474=CARTESIAN_POINT('',(117.536514876029,-1.85,49.3605062722945));
#203475=CARTESIAN_POINT('Origin',(117.045701373479,-1.85,49.2651013158452));
#203476=CARTESIAN_POINT('',(116.98845839961,-1.85,49.5595894173749));
#203477=CARTESIAN_POINT('',(117.045701373479,-1.85,49.2651013158452));
#203478=CARTESIAN_POINT('Origin',(117.831002977559,-1.35,49.417749246164));
#203479=CARTESIAN_POINT('',(118.321816480108,-1.35,49.5131542026133));
#203480=CARTESIAN_POINT('',(118.264573506239,-1.35,49.807642304143));
#203481=CARTESIAN_POINT('',(118.321816480108,-1.35,49.5131542026133));
#203482=CARTESIAN_POINT('',(117.773760003689,-1.35,49.7122373476937));
#203483=CARTESIAN_POINT('',(117.773760003689,-1.35,49.7122373476937));
#203484=CARTESIAN_POINT('',(117.831002977559,-1.35,49.417749246164));
#203485=CARTESIAN_POINT('',(117.831002977559,-1.35,49.417749246164));
#203486=CARTESIAN_POINT('',(117.831002977559,-1.35,49.417749246164));
#203487=CARTESIAN_POINT('Origin',(118.321816480108,-1.35,49.5131542026133));
#203488=CARTESIAN_POINT('',(118.321816480108,-1.85,49.5131542026133));
#203489=CARTESIAN_POINT('',(118.264573506239,-1.85,49.807642304143));
#203490=CARTESIAN_POINT('',(118.321816480108,-1.85,49.5131542026133));
#203491=CARTESIAN_POINT('',(118.264573506239,-1.35,49.807642304143));
#203492=CARTESIAN_POINT('',(118.321816480108,-1.35,49.5131542026133));
#203493=CARTESIAN_POINT('Origin',(118.321816480108,-1.85,49.5131542026133));
#203494=CARTESIAN_POINT('',(117.831002977559,-1.85,49.417749246164));
#203495=CARTESIAN_POINT('',(117.773760003689,-1.85,49.7122373476937));
#203496=CARTESIAN_POINT('',(117.831002977559,-1.85,49.417749246164));
#203497=CARTESIAN_POINT('',(118.264573506239,-1.85,49.807642304143));
#203498=CARTESIAN_POINT('',(118.321816480108,-1.85,49.5131542026133));
#203499=CARTESIAN_POINT('Origin',(117.831002977559,-1.85,49.417749246164));
#203500=CARTESIAN_POINT('',(117.773760003689,-1.85,49.7122373476937));
#203501=CARTESIAN_POINT('',(117.831002977559,-1.85,49.417749246164));
#203502=CARTESIAN_POINT('Origin',(118.616304581638,-1.35,49.5703971764828));
#203503=CARTESIAN_POINT('',(119.107118084187,-1.35,49.6658021329321));
#203504=CARTESIAN_POINT('',(119.049875110318,-1.35,49.9602902344618));
#203505=CARTESIAN_POINT('',(119.107118084187,-1.35,49.6658021329321));
#203506=CARTESIAN_POINT('',(118.559061607768,-1.35,49.8648852780125));
#203507=CARTESIAN_POINT('',(118.559061607768,-1.35,49.8648852780125));
#203508=CARTESIAN_POINT('',(118.616304581638,-1.35,49.5703971764828));
#203509=CARTESIAN_POINT('',(118.616304581638,-1.35,49.5703971764828));
#203510=CARTESIAN_POINT('',(118.616304581638,-1.35,49.5703971764828));
#203511=CARTESIAN_POINT('Origin',(119.107118084187,-1.35,49.6658021329321));
#203512=CARTESIAN_POINT('',(119.107118084187,-1.85,49.6658021329321));
#203513=CARTESIAN_POINT('',(119.049875110318,-1.85,49.9602902344618));
#203514=CARTESIAN_POINT('',(119.107118084187,-1.85,49.6658021329321));
#203515=CARTESIAN_POINT('',(119.049875110318,-1.35,49.9602902344618));
#203516=CARTESIAN_POINT('',(119.107118084187,-1.35,49.6658021329321));
#203517=CARTESIAN_POINT('Origin',(119.107118084187,-1.85,49.6658021329321));
#203518=CARTESIAN_POINT('',(118.616304581638,-1.85,49.5703971764828));
#203519=CARTESIAN_POINT('',(118.559061607768,-1.85,49.8648852780125));
#203520=CARTESIAN_POINT('',(118.616304581638,-1.85,49.5703971764828));
#203521=CARTESIAN_POINT('',(119.049875110318,-1.85,49.9602902344618));
#203522=CARTESIAN_POINT('',(119.107118084187,-1.85,49.6658021329321));
#203523=CARTESIAN_POINT('Origin',(118.616304581638,-1.85,49.5703971764828));
#203524=CARTESIAN_POINT('',(118.559061607768,-1.85,49.8648852780125));
#203525=CARTESIAN_POINT('',(118.616304581638,-1.85,49.5703971764828));
#203526=CARTESIAN_POINT('Origin',(118.616304581638,-0.549999999999986,49.5703971764828));
#203527=CARTESIAN_POINT('',(119.107118084187,-0.549999999999986,49.6658021329321));
#203528=CARTESIAN_POINT('',(119.049875110318,-0.549999999999986,49.9602902344618));
#203529=CARTESIAN_POINT('',(119.107118084187,-0.549999999999986,49.6658021329321));
#203530=CARTESIAN_POINT('',(118.559061607768,-0.549999999999986,49.8648852780125));
#203531=CARTESIAN_POINT('',(118.559061607768,-0.549999999999986,49.8648852780125));
#203532=CARTESIAN_POINT('',(118.616304581638,-0.549999999999986,49.5703971764828));
#203533=CARTESIAN_POINT('',(118.616304581638,-0.549999999999986,49.5703971764828));
#203534=CARTESIAN_POINT('',(118.616304581638,-0.549999999999986,49.5703971764828));
#203535=CARTESIAN_POINT('Origin',(119.107118084187,-0.549999999999986,49.6658021329321));
#203536=CARTESIAN_POINT('',(119.107118084187,-1.05,49.6658021329321));
#203537=CARTESIAN_POINT('',(119.049875110318,-1.05,49.9602902344618));
#203538=CARTESIAN_POINT('',(119.107118084187,-1.05,49.6658021329321));
#203539=CARTESIAN_POINT('',(119.049875110318,-0.549999999999986,49.9602902344618));
#203540=CARTESIAN_POINT('',(119.107118084187,-0.549999999999986,49.6658021329321));
#203541=CARTESIAN_POINT('Origin',(119.107118084187,-1.05,49.6658021329321));
#203542=CARTESIAN_POINT('',(118.616304581638,-1.05,49.5703971764828));
#203543=CARTESIAN_POINT('',(118.559061607768,-1.05,49.8648852780125));
#203544=CARTESIAN_POINT('',(118.616304581638,-1.05,49.5703971764828));
#203545=CARTESIAN_POINT('',(119.049875110318,-1.05,49.9602902344618));
#203546=CARTESIAN_POINT('',(119.107118084187,-1.05,49.6658021329321));
#203547=CARTESIAN_POINT('Origin',(118.616304581638,-1.05,49.5703971764828));
#203548=CARTESIAN_POINT('',(118.559061607768,-1.05,49.8648852780125));
#203549=CARTESIAN_POINT('',(118.616304581638,-1.05,49.5703971764828));
#203550=CARTESIAN_POINT('Origin',(118.616304581638,0.250000000000015,49.5703971764828));
#203551=CARTESIAN_POINT('',(119.107118084187,0.250000000000015,49.6658021329321));
#203552=CARTESIAN_POINT('',(119.049875110318,0.250000000000015,49.9602902344618));
#203553=CARTESIAN_POINT('',(119.107118084187,0.250000000000015,49.6658021329321));
#203554=CARTESIAN_POINT('',(118.559061607768,0.250000000000015,49.8648852780125));
#203555=CARTESIAN_POINT('',(118.559061607768,0.250000000000015,49.8648852780125));
#203556=CARTESIAN_POINT('',(118.616304581638,0.250000000000015,49.5703971764828));
#203557=CARTESIAN_POINT('',(118.616304581638,0.250000000000015,49.5703971764828));
#203558=CARTESIAN_POINT('',(118.616304581638,0.250000000000015,49.5703971764828));
#203559=CARTESIAN_POINT('Origin',(119.107118084187,0.250000000000015,49.6658021329321));
#203560=CARTESIAN_POINT('',(119.107118084187,-0.249999999999985,49.6658021329321));
#203561=CARTESIAN_POINT('',(119.049875110318,-0.249999999999985,49.9602902344618));
#203562=CARTESIAN_POINT('',(119.107118084187,-0.249999999999985,49.6658021329321));
#203563=CARTESIAN_POINT('',(119.049875110318,0.250000000000015,49.9602902344618));
#203564=CARTESIAN_POINT('',(119.107118084187,0.250000000000015,49.6658021329321));
#203565=CARTESIAN_POINT('Origin',(119.107118084187,-0.249999999999985,49.6658021329321));
#203566=CARTESIAN_POINT('',(118.616304581638,-0.249999999999985,49.5703971764828));
#203567=CARTESIAN_POINT('',(118.559061607768,-0.249999999999985,49.8648852780125));
#203568=CARTESIAN_POINT('',(118.616304581638,-0.249999999999985,49.5703971764828));
#203569=CARTESIAN_POINT('',(119.049875110318,-0.249999999999985,49.9602902344618));
#203570=CARTESIAN_POINT('',(119.107118084187,-0.249999999999985,49.6658021329321));
#203571=CARTESIAN_POINT('Origin',(118.616304581638,-0.249999999999985,49.5703971764828));
#203572=CARTESIAN_POINT('',(118.559061607768,-0.249999999999985,49.8648852780125));
#203573=CARTESIAN_POINT('',(118.616304581638,-0.249999999999985,49.5703971764828));
#203574=CARTESIAN_POINT('Origin',(118.616304581638,1.05,49.5703971764828));
#203575=CARTESIAN_POINT('',(119.107118084187,1.05,49.6658021329321));
#203576=CARTESIAN_POINT('',(119.049875110318,1.05,49.9602902344618));
#203577=CARTESIAN_POINT('',(119.107118084187,1.05,49.6658021329321));
#203578=CARTESIAN_POINT('',(118.559061607768,1.05,49.8648852780125));
#203579=CARTESIAN_POINT('',(118.559061607768,1.05,49.8648852780125));
#203580=CARTESIAN_POINT('',(118.616304581638,1.05,49.5703971764828));
#203581=CARTESIAN_POINT('',(118.616304581638,1.05,49.5703971764828));
#203582=CARTESIAN_POINT('',(118.616304581638,1.05,49.5703971764828));
#203583=CARTESIAN_POINT('Origin',(119.107118084187,1.05,49.6658021329321));
#203584=CARTESIAN_POINT('',(119.107118084187,0.550000000000015,49.6658021329321));
#203585=CARTESIAN_POINT('',(119.049875110318,0.550000000000015,49.9602902344618));
#203586=CARTESIAN_POINT('',(119.107118084187,0.550000000000015,49.6658021329321));
#203587=CARTESIAN_POINT('',(119.049875110318,1.05,49.9602902344618));
#203588=CARTESIAN_POINT('',(119.107118084187,1.05,49.6658021329321));
#203589=CARTESIAN_POINT('Origin',(119.107118084187,0.550000000000015,49.6658021329321));
#203590=CARTESIAN_POINT('',(118.616304581638,0.550000000000015,49.5703971764828));
#203591=CARTESIAN_POINT('',(118.559061607768,0.550000000000015,49.8648852780125));
#203592=CARTESIAN_POINT('',(118.616304581638,0.550000000000015,49.5703971764828));
#203593=CARTESIAN_POINT('',(119.049875110318,0.550000000000015,49.9602902344618));
#203594=CARTESIAN_POINT('',(119.107118084187,0.550000000000015,49.6658021329321));
#203595=CARTESIAN_POINT('Origin',(118.616304581638,0.550000000000015,49.5703971764828));
#203596=CARTESIAN_POINT('',(118.559061607768,0.550000000000015,49.8648852780125));
#203597=CARTESIAN_POINT('',(118.616304581638,0.550000000000015,49.5703971764828));
#203598=CARTESIAN_POINT('Origin',(118.616304581638,1.85,49.5703971764828));
#203599=CARTESIAN_POINT('',(119.107118084187,1.85,49.6658021329321));
#203600=CARTESIAN_POINT('',(119.049875110318,1.85,49.9602902344618));
#203601=CARTESIAN_POINT('',(119.107118084187,1.85,49.6658021329321));
#203602=CARTESIAN_POINT('',(118.559061607768,1.85,49.8648852780125));
#203603=CARTESIAN_POINT('',(118.559061607768,1.85,49.8648852780125));
#203604=CARTESIAN_POINT('',(118.616304581638,1.85,49.5703971764828));
#203605=CARTESIAN_POINT('',(118.616304581638,1.85,49.5703971764828));
#203606=CARTESIAN_POINT('',(118.616304581638,1.85,49.5703971764828));
#203607=CARTESIAN_POINT('Origin',(119.107118084187,1.85,49.6658021329321));
#203608=CARTESIAN_POINT('',(119.107118084187,1.35,49.6658021329321));
#203609=CARTESIAN_POINT('',(119.049875110318,1.35,49.9602902344618));
#203610=CARTESIAN_POINT('',(119.107118084187,1.35,49.6658021329321));
#203611=CARTESIAN_POINT('',(119.049875110318,1.85,49.9602902344618));
#203612=CARTESIAN_POINT('',(119.107118084187,1.85,49.6658021329321));
#203613=CARTESIAN_POINT('Origin',(119.107118084187,1.35,49.6658021329321));
#203614=CARTESIAN_POINT('',(118.616304581638,1.35,49.5703971764828));
#203615=CARTESIAN_POINT('',(118.559061607768,1.35,49.8648852780125));
#203616=CARTESIAN_POINT('',(118.616304581638,1.35,49.5703971764828));
#203617=CARTESIAN_POINT('',(119.049875110318,1.35,49.9602902344618));
#203618=CARTESIAN_POINT('',(119.107118084187,1.35,49.6658021329321));
#203619=CARTESIAN_POINT('Origin',(118.616304581638,1.35,49.5703971764828));
#203620=CARTESIAN_POINT('',(118.559061607768,1.35,49.8648852780125));
#203621=CARTESIAN_POINT('',(118.616304581638,1.35,49.5703971764828));
#203622=CARTESIAN_POINT('Origin',(117.831002977559,1.85,49.417749246164));
#203623=CARTESIAN_POINT('',(118.321816480108,1.85,49.5131542026133));
#203624=CARTESIAN_POINT('',(118.264573506239,1.85,49.807642304143));
#203625=CARTESIAN_POINT('',(118.321816480108,1.85,49.5131542026133));
#203626=CARTESIAN_POINT('',(117.773760003689,1.85,49.7122373476937));
#203627=CARTESIAN_POINT('',(117.773760003689,1.85,49.7122373476937));
#203628=CARTESIAN_POINT('',(117.831002977559,1.85,49.417749246164));
#203629=CARTESIAN_POINT('',(117.831002977559,1.85,49.417749246164));
#203630=CARTESIAN_POINT('',(117.831002977559,1.85,49.417749246164));
#203631=CARTESIAN_POINT('Origin',(118.321816480108,1.85,49.5131542026133));
#203632=CARTESIAN_POINT('',(118.321816480108,1.35,49.5131542026133));
#203633=CARTESIAN_POINT('',(118.264573506239,1.35,49.807642304143));
#203634=CARTESIAN_POINT('',(118.321816480108,1.35,49.5131542026133));
#203635=CARTESIAN_POINT('',(118.264573506239,1.85,49.807642304143));
#203636=CARTESIAN_POINT('',(118.321816480108,1.85,49.5131542026133));
#203637=CARTESIAN_POINT('Origin',(118.321816480108,1.35,49.5131542026133));
#203638=CARTESIAN_POINT('',(117.831002977559,1.35,49.417749246164));
#203639=CARTESIAN_POINT('',(117.773760003689,1.35,49.7122373476937));
#203640=CARTESIAN_POINT('',(117.831002977559,1.35,49.417749246164));
#203641=CARTESIAN_POINT('',(118.264573506239,1.35,49.807642304143));
#203642=CARTESIAN_POINT('',(118.321816480108,1.35,49.5131542026133));
#203643=CARTESIAN_POINT('Origin',(117.831002977559,1.35,49.417749246164));
#203644=CARTESIAN_POINT('',(117.773760003689,1.35,49.7122373476937));
#203645=CARTESIAN_POINT('',(117.831002977559,1.35,49.417749246164));
#203646=CARTESIAN_POINT('Origin',(117.045701373479,1.85,49.2651013158452));
#203647=CARTESIAN_POINT('',(117.536514876029,1.85,49.3605062722945));
#203648=CARTESIAN_POINT('',(117.479271902159,1.85,49.6549943738242));
#203649=CARTESIAN_POINT('',(117.536514876029,1.85,49.3605062722945));
#203650=CARTESIAN_POINT('',(116.98845839961,1.85,49.5595894173749));
#203651=CARTESIAN_POINT('',(116.98845839961,1.85,49.5595894173749));
#203652=CARTESIAN_POINT('',(117.045701373479,1.85,49.2651013158452));
#203653=CARTESIAN_POINT('',(117.045701373479,1.85,49.2651013158452));
#203654=CARTESIAN_POINT('',(117.045701373479,1.85,49.2651013158452));
#203655=CARTESIAN_POINT('Origin',(117.536514876029,1.85,49.3605062722945));
#203656=CARTESIAN_POINT('',(117.536514876029,1.35,49.3605062722945));
#203657=CARTESIAN_POINT('',(117.479271902159,1.35,49.6549943738242));
#203658=CARTESIAN_POINT('',(117.536514876029,1.35,49.3605062722945));
#203659=CARTESIAN_POINT('',(117.479271902159,1.85,49.6549943738242));
#203660=CARTESIAN_POINT('',(117.536514876029,1.85,49.3605062722945));
#203661=CARTESIAN_POINT('Origin',(117.536514876029,1.35,49.3605062722945));
#203662=CARTESIAN_POINT('',(117.045701373479,1.35,49.2651013158452));
#203663=CARTESIAN_POINT('',(116.98845839961,1.35,49.5595894173749));
#203664=CARTESIAN_POINT('',(117.045701373479,1.35,49.2651013158452));
#203665=CARTESIAN_POINT('',(117.479271902159,1.35,49.6549943738242));
#203666=CARTESIAN_POINT('',(117.536514876029,1.35,49.3605062722945));
#203667=CARTESIAN_POINT('Origin',(117.045701373479,1.35,49.2651013158452));
#203668=CARTESIAN_POINT('',(116.98845839961,1.35,49.5595894173749));
#203669=CARTESIAN_POINT('',(117.045701373479,1.35,49.2651013158452));
#203670=CARTESIAN_POINT('Origin',(116.2603997694,1.85,49.1124533855264));
#203671=CARTESIAN_POINT('',(116.75121327195,1.85,49.2078583419757));
#203672=CARTESIAN_POINT('',(116.69397029808,1.85,49.5023464435054));
#203673=CARTESIAN_POINT('',(116.75121327195,1.85,49.2078583419757));
#203674=CARTESIAN_POINT('',(116.203156795531,1.85,49.4069414870561));
#203675=CARTESIAN_POINT('',(116.203156795531,1.85,49.4069414870561));
#203676=CARTESIAN_POINT('',(116.2603997694,1.85,49.1124533855264));
#203677=CARTESIAN_POINT('',(116.2603997694,1.85,49.1124533855264));
#203678=CARTESIAN_POINT('',(116.2603997694,1.85,49.1124533855264));
#203679=CARTESIAN_POINT('Origin',(116.75121327195,1.85,49.2078583419757));
#203680=CARTESIAN_POINT('',(116.75121327195,1.35,49.2078583419757));
#203681=CARTESIAN_POINT('',(116.69397029808,1.35,49.5023464435054));
#203682=CARTESIAN_POINT('',(116.75121327195,1.35,49.2078583419757));
#203683=CARTESIAN_POINT('',(116.69397029808,1.85,49.5023464435054));
#203684=CARTESIAN_POINT('',(116.75121327195,1.85,49.2078583419757));
#203685=CARTESIAN_POINT('Origin',(116.75121327195,1.35,49.2078583419757));
#203686=CARTESIAN_POINT('',(116.2603997694,1.35,49.1124533855264));
#203687=CARTESIAN_POINT('',(116.203156795531,1.35,49.4069414870561));
#203688=CARTESIAN_POINT('',(116.2603997694,1.35,49.1124533855264));
#203689=CARTESIAN_POINT('',(116.69397029808,1.35,49.5023464435054));
#203690=CARTESIAN_POINT('',(116.75121327195,1.35,49.2078583419757));
#203691=CARTESIAN_POINT('Origin',(116.2603997694,1.35,49.1124533855264));
#203692=CARTESIAN_POINT('',(116.203156795531,1.35,49.4069414870561));
#203693=CARTESIAN_POINT('',(116.2603997694,1.35,49.1124533855264));
#203694=CARTESIAN_POINT('Origin',(116.2603997694,1.05,49.1124533855264));
#203695=CARTESIAN_POINT('',(116.75121327195,1.05,49.2078583419757));
#203696=CARTESIAN_POINT('',(116.69397029808,1.05,49.5023464435054));
#203697=CARTESIAN_POINT('',(116.75121327195,1.05,49.2078583419757));
#203698=CARTESIAN_POINT('',(116.203156795531,1.05,49.4069414870561));
#203699=CARTESIAN_POINT('',(116.203156795531,1.05,49.4069414870561));
#203700=CARTESIAN_POINT('',(116.2603997694,1.05,49.1124533855264));
#203701=CARTESIAN_POINT('',(116.2603997694,1.05,49.1124533855264));
#203702=CARTESIAN_POINT('',(116.2603997694,1.05,49.1124533855264));
#203703=CARTESIAN_POINT('Origin',(116.75121327195,1.05,49.2078583419757));
#203704=CARTESIAN_POINT('',(116.75121327195,0.550000000000015,49.2078583419757));
#203705=CARTESIAN_POINT('',(116.69397029808,0.550000000000015,49.5023464435054));
#203706=CARTESIAN_POINT('',(116.75121327195,0.550000000000015,49.2078583419757));
#203707=CARTESIAN_POINT('',(116.69397029808,1.05,49.5023464435054));
#203708=CARTESIAN_POINT('',(116.75121327195,1.05,49.2078583419757));
#203709=CARTESIAN_POINT('Origin',(116.75121327195,0.550000000000015,49.2078583419757));
#203710=CARTESIAN_POINT('',(116.2603997694,0.550000000000015,49.1124533855264));
#203711=CARTESIAN_POINT('',(116.203156795531,0.550000000000015,49.4069414870561));
#203712=CARTESIAN_POINT('',(116.2603997694,0.550000000000015,49.1124533855264));
#203713=CARTESIAN_POINT('',(116.69397029808,0.550000000000015,49.5023464435054));
#203714=CARTESIAN_POINT('',(116.75121327195,0.550000000000015,49.2078583419757));
#203715=CARTESIAN_POINT('Origin',(116.2603997694,0.550000000000015,49.1124533855264));
#203716=CARTESIAN_POINT('',(116.203156795531,0.550000000000015,49.4069414870561));
#203717=CARTESIAN_POINT('',(116.2603997694,0.550000000000015,49.1124533855264));
#203718=CARTESIAN_POINT('Origin',(116.2603997694,0.250000000000015,49.1124533855264));
#203719=CARTESIAN_POINT('',(116.75121327195,0.250000000000015,49.2078583419757));
#203720=CARTESIAN_POINT('',(116.69397029808,0.250000000000015,49.5023464435054));
#203721=CARTESIAN_POINT('',(116.75121327195,0.250000000000015,49.2078583419757));
#203722=CARTESIAN_POINT('',(116.203156795531,0.250000000000015,49.4069414870561));
#203723=CARTESIAN_POINT('',(116.203156795531,0.250000000000015,49.4069414870561));
#203724=CARTESIAN_POINT('',(116.2603997694,0.250000000000015,49.1124533855264));
#203725=CARTESIAN_POINT('',(116.2603997694,0.250000000000015,49.1124533855264));
#203726=CARTESIAN_POINT('',(116.2603997694,0.250000000000015,49.1124533855264));
#203727=CARTESIAN_POINT('Origin',(116.75121327195,0.250000000000015,49.2078583419757));
#203728=CARTESIAN_POINT('',(116.75121327195,-0.249999999999985,49.2078583419757));
#203729=CARTESIAN_POINT('',(116.69397029808,-0.249999999999985,49.5023464435054));
#203730=CARTESIAN_POINT('',(116.75121327195,-0.249999999999985,49.2078583419757));
#203731=CARTESIAN_POINT('',(116.69397029808,0.250000000000015,49.5023464435054));
#203732=CARTESIAN_POINT('',(116.75121327195,0.250000000000015,49.2078583419757));
#203733=CARTESIAN_POINT('Origin',(116.75121327195,-0.249999999999985,49.2078583419757));
#203734=CARTESIAN_POINT('',(116.2603997694,-0.249999999999985,49.1124533855264));
#203735=CARTESIAN_POINT('',(116.203156795531,-0.249999999999985,49.4069414870561));
#203736=CARTESIAN_POINT('',(116.2603997694,-0.249999999999985,49.1124533855264));
#203737=CARTESIAN_POINT('',(116.69397029808,-0.249999999999985,49.5023464435054));
#203738=CARTESIAN_POINT('',(116.75121327195,-0.249999999999985,49.2078583419757));
#203739=CARTESIAN_POINT('Origin',(116.2603997694,-0.249999999999985,49.1124533855264));
#203740=CARTESIAN_POINT('',(116.203156795531,-0.249999999999985,49.4069414870561));
#203741=CARTESIAN_POINT('',(116.2603997694,-0.249999999999985,49.1124533855264));
#203742=CARTESIAN_POINT('Origin',(116.2603997694,-0.549999999999986,49.1124533855264));
#203743=CARTESIAN_POINT('',(116.75121327195,-0.549999999999986,49.2078583419757));
#203744=CARTESIAN_POINT('',(116.69397029808,-0.549999999999986,49.5023464435054));
#203745=CARTESIAN_POINT('',(116.75121327195,-0.549999999999986,49.2078583419757));
#203746=CARTESIAN_POINT('',(116.203156795531,-0.549999999999986,49.4069414870561));
#203747=CARTESIAN_POINT('',(116.203156795531,-0.549999999999986,49.4069414870561));
#203748=CARTESIAN_POINT('',(116.2603997694,-0.549999999999986,49.1124533855264));
#203749=CARTESIAN_POINT('',(116.2603997694,-0.549999999999986,49.1124533855264));
#203750=CARTESIAN_POINT('',(116.2603997694,-0.549999999999986,49.1124533855264));
#203751=CARTESIAN_POINT('Origin',(116.75121327195,-0.549999999999986,49.2078583419757));
#203752=CARTESIAN_POINT('',(116.75121327195,-1.05,49.2078583419757));
#203753=CARTESIAN_POINT('',(116.69397029808,-1.05,49.5023464435054));
#203754=CARTESIAN_POINT('',(116.75121327195,-1.05,49.2078583419757));
#203755=CARTESIAN_POINT('',(116.69397029808,-0.549999999999986,49.5023464435054));
#203756=CARTESIAN_POINT('',(116.75121327195,-0.549999999999986,49.2078583419757));
#203757=CARTESIAN_POINT('Origin',(116.75121327195,-1.05,49.2078583419757));
#203758=CARTESIAN_POINT('',(116.2603997694,-1.05,49.1124533855264));
#203759=CARTESIAN_POINT('',(116.203156795531,-1.05,49.4069414870561));
#203760=CARTESIAN_POINT('',(116.2603997694,-1.05,49.1124533855264));
#203761=CARTESIAN_POINT('',(116.69397029808,-1.05,49.5023464435054));
#203762=CARTESIAN_POINT('',(116.75121327195,-1.05,49.2078583419757));
#203763=CARTESIAN_POINT('Origin',(116.2603997694,-1.05,49.1124533855264));
#203764=CARTESIAN_POINT('',(116.203156795531,-1.05,49.4069414870561));
#203765=CARTESIAN_POINT('',(116.2603997694,-1.05,49.1124533855264));
#203766=CARTESIAN_POINT('Origin',(117.045701373479,-0.549999999999986,49.2651013158452));
#203767=CARTESIAN_POINT('',(117.536514876029,-0.549999999999986,49.3605062722945));
#203768=CARTESIAN_POINT('',(117.479271902159,-0.549999999999986,49.6549943738242));
#203769=CARTESIAN_POINT('',(117.536514876029,-0.549999999999986,49.3605062722945));
#203770=CARTESIAN_POINT('',(116.98845839961,-0.549999999999986,49.5595894173749));
#203771=CARTESIAN_POINT('',(116.98845839961,-0.549999999999986,49.5595894173749));
#203772=CARTESIAN_POINT('',(117.045701373479,-0.549999999999986,49.2651013158452));
#203773=CARTESIAN_POINT('',(117.045701373479,-0.549999999999986,49.2651013158452));
#203774=CARTESIAN_POINT('',(117.045701373479,-0.549999999999986,49.2651013158452));
#203775=CARTESIAN_POINT('Origin',(117.536514876029,-0.549999999999986,49.3605062722945));
#203776=CARTESIAN_POINT('',(117.536514876029,-1.05,49.3605062722945));
#203777=CARTESIAN_POINT('',(117.479271902159,-1.05,49.6549943738242));
#203778=CARTESIAN_POINT('',(117.536514876029,-1.05,49.3605062722945));
#203779=CARTESIAN_POINT('',(117.479271902159,-0.549999999999986,49.6549943738242));
#203780=CARTESIAN_POINT('',(117.536514876029,-0.549999999999986,49.3605062722945));
#203781=CARTESIAN_POINT('Origin',(117.536514876029,-1.05,49.3605062722945));
#203782=CARTESIAN_POINT('',(117.045701373479,-1.05,49.2651013158452));
#203783=CARTESIAN_POINT('',(116.98845839961,-1.05,49.5595894173749));
#203784=CARTESIAN_POINT('',(117.045701373479,-1.05,49.2651013158452));
#203785=CARTESIAN_POINT('',(117.479271902159,-1.05,49.6549943738242));
#203786=CARTESIAN_POINT('',(117.536514876029,-1.05,49.3605062722945));
#203787=CARTESIAN_POINT('Origin',(117.045701373479,-1.05,49.2651013158452));
#203788=CARTESIAN_POINT('',(116.98845839961,-1.05,49.5595894173749));
#203789=CARTESIAN_POINT('',(117.045701373479,-1.05,49.2651013158452));
#203790=CARTESIAN_POINT('Origin',(117.831002977559,-0.549999999999986,49.417749246164));
#203791=CARTESIAN_POINT('',(118.321816480108,-0.549999999999986,49.5131542026133));
#203792=CARTESIAN_POINT('',(118.264573506239,-0.549999999999986,49.807642304143));
#203793=CARTESIAN_POINT('',(118.321816480108,-0.549999999999986,49.5131542026133));
#203794=CARTESIAN_POINT('',(117.773760003689,-0.549999999999986,49.7122373476937));
#203795=CARTESIAN_POINT('',(117.773760003689,-0.549999999999986,49.7122373476937));
#203796=CARTESIAN_POINT('',(117.831002977559,-0.549999999999986,49.417749246164));
#203797=CARTESIAN_POINT('',(117.831002977559,-0.549999999999986,49.417749246164));
#203798=CARTESIAN_POINT('',(117.831002977559,-0.549999999999986,49.417749246164));
#203799=CARTESIAN_POINT('Origin',(118.321816480108,-0.549999999999986,49.5131542026133));
#203800=CARTESIAN_POINT('',(118.321816480108,-1.05,49.5131542026133));
#203801=CARTESIAN_POINT('',(118.264573506239,-1.05,49.807642304143));
#203802=CARTESIAN_POINT('',(118.321816480108,-1.05,49.5131542026133));
#203803=CARTESIAN_POINT('',(118.264573506239,-0.549999999999986,49.807642304143));
#203804=CARTESIAN_POINT('',(118.321816480108,-0.549999999999986,49.5131542026133));
#203805=CARTESIAN_POINT('Origin',(118.321816480108,-1.05,49.5131542026133));
#203806=CARTESIAN_POINT('',(117.831002977559,-1.05,49.417749246164));
#203807=CARTESIAN_POINT('',(117.773760003689,-1.05,49.7122373476937));
#203808=CARTESIAN_POINT('',(117.831002977559,-1.05,49.417749246164));
#203809=CARTESIAN_POINT('',(118.264573506239,-1.05,49.807642304143));
#203810=CARTESIAN_POINT('',(118.321816480108,-1.05,49.5131542026133));
#203811=CARTESIAN_POINT('Origin',(117.831002977559,-1.05,49.417749246164));
#203812=CARTESIAN_POINT('',(117.773760003689,-1.05,49.7122373476937));
#203813=CARTESIAN_POINT('',(117.831002977559,-1.05,49.417749246164));
#203814=CARTESIAN_POINT('Origin',(117.831002977559,0.250000000000015,49.417749246164));
#203815=CARTESIAN_POINT('',(118.321816480108,0.250000000000015,49.5131542026133));
#203816=CARTESIAN_POINT('',(118.264573506239,0.250000000000015,49.807642304143));
#203817=CARTESIAN_POINT('',(118.321816480108,0.250000000000015,49.5131542026133));
#203818=CARTESIAN_POINT('',(117.773760003689,0.250000000000015,49.7122373476937));
#203819=CARTESIAN_POINT('',(117.773760003689,0.250000000000015,49.7122373476937));
#203820=CARTESIAN_POINT('',(117.831002977559,0.250000000000015,49.417749246164));
#203821=CARTESIAN_POINT('',(117.831002977559,0.250000000000015,49.417749246164));
#203822=CARTESIAN_POINT('',(117.831002977559,0.250000000000015,49.417749246164));
#203823=CARTESIAN_POINT('Origin',(118.321816480108,0.250000000000015,49.5131542026133));
#203824=CARTESIAN_POINT('',(118.321816480108,-0.249999999999985,49.5131542026133));
#203825=CARTESIAN_POINT('',(118.264573506239,-0.249999999999985,49.807642304143));
#203826=CARTESIAN_POINT('',(118.321816480108,-0.249999999999985,49.5131542026133));
#203827=CARTESIAN_POINT('',(118.264573506239,0.250000000000015,49.807642304143));
#203828=CARTESIAN_POINT('',(118.321816480108,0.250000000000015,49.5131542026133));
#203829=CARTESIAN_POINT('Origin',(118.321816480108,-0.249999999999985,49.5131542026133));
#203830=CARTESIAN_POINT('',(117.831002977559,-0.249999999999985,49.417749246164));
#203831=CARTESIAN_POINT('',(117.773760003689,-0.249999999999985,49.7122373476937));
#203832=CARTESIAN_POINT('',(117.831002977559,-0.249999999999985,49.417749246164));
#203833=CARTESIAN_POINT('',(118.264573506239,-0.249999999999985,49.807642304143));
#203834=CARTESIAN_POINT('',(118.321816480108,-0.249999999999985,49.5131542026133));
#203835=CARTESIAN_POINT('Origin',(117.831002977559,-0.249999999999985,49.417749246164));
#203836=CARTESIAN_POINT('',(117.773760003689,-0.249999999999985,49.7122373476937));
#203837=CARTESIAN_POINT('',(117.831002977559,-0.249999999999985,49.417749246164));
#203838=CARTESIAN_POINT('Origin',(117.831002977559,1.05,49.417749246164));
#203839=CARTESIAN_POINT('',(118.321816480108,1.05,49.5131542026133));
#203840=CARTESIAN_POINT('',(118.264573506239,1.05,49.807642304143));
#203841=CARTESIAN_POINT('',(118.321816480108,1.05,49.5131542026133));
#203842=CARTESIAN_POINT('',(117.773760003689,1.05,49.7122373476937));
#203843=CARTESIAN_POINT('',(117.773760003689,1.05,49.7122373476937));
#203844=CARTESIAN_POINT('',(117.831002977559,1.05,49.417749246164));
#203845=CARTESIAN_POINT('',(117.831002977559,1.05,49.417749246164));
#203846=CARTESIAN_POINT('',(117.831002977559,1.05,49.417749246164));
#203847=CARTESIAN_POINT('Origin',(118.321816480108,1.05,49.5131542026133));
#203848=CARTESIAN_POINT('',(118.321816480108,0.550000000000015,49.5131542026133));
#203849=CARTESIAN_POINT('',(118.264573506239,0.550000000000015,49.807642304143));
#203850=CARTESIAN_POINT('',(118.321816480108,0.550000000000015,49.5131542026133));
#203851=CARTESIAN_POINT('',(118.264573506239,1.05,49.807642304143));
#203852=CARTESIAN_POINT('',(118.321816480108,1.05,49.5131542026133));
#203853=CARTESIAN_POINT('Origin',(118.321816480108,0.550000000000015,49.5131542026133));
#203854=CARTESIAN_POINT('',(117.831002977559,0.550000000000015,49.417749246164));
#203855=CARTESIAN_POINT('',(117.773760003689,0.550000000000015,49.7122373476937));
#203856=CARTESIAN_POINT('',(117.831002977559,0.550000000000015,49.417749246164));
#203857=CARTESIAN_POINT('',(118.264573506239,0.550000000000015,49.807642304143));
#203858=CARTESIAN_POINT('',(118.321816480108,0.550000000000015,49.5131542026133));
#203859=CARTESIAN_POINT('Origin',(117.831002977559,0.550000000000015,49.417749246164));
#203860=CARTESIAN_POINT('',(117.773760003689,0.550000000000015,49.7122373476937));
#203861=CARTESIAN_POINT('',(117.831002977559,0.550000000000015,49.417749246164));
#203862=CARTESIAN_POINT('Origin',(117.045701373479,1.05,49.2651013158452));
#203863=CARTESIAN_POINT('',(117.536514876029,1.05,49.3605062722945));
#203864=CARTESIAN_POINT('',(117.479271902159,1.05,49.6549943738242));
#203865=CARTESIAN_POINT('',(117.536514876029,1.05,49.3605062722945));
#203866=CARTESIAN_POINT('',(116.98845839961,1.05,49.5595894173749));
#203867=CARTESIAN_POINT('',(116.98845839961,1.05,49.5595894173749));
#203868=CARTESIAN_POINT('',(117.045701373479,1.05,49.2651013158452));
#203869=CARTESIAN_POINT('',(117.045701373479,1.05,49.2651013158452));
#203870=CARTESIAN_POINT('',(117.045701373479,1.05,49.2651013158452));
#203871=CARTESIAN_POINT('Origin',(117.536514876029,1.05,49.3605062722945));
#203872=CARTESIAN_POINT('',(117.536514876029,0.550000000000015,49.3605062722945));
#203873=CARTESIAN_POINT('',(117.479271902159,0.550000000000015,49.6549943738242));
#203874=CARTESIAN_POINT('',(117.536514876029,0.550000000000015,49.3605062722945));
#203875=CARTESIAN_POINT('',(117.479271902159,1.05,49.6549943738242));
#203876=CARTESIAN_POINT('',(117.536514876029,1.05,49.3605062722945));
#203877=CARTESIAN_POINT('Origin',(117.536514876029,0.550000000000015,49.3605062722945));
#203878=CARTESIAN_POINT('',(117.045701373479,0.550000000000015,49.2651013158452));
#203879=CARTESIAN_POINT('',(116.98845839961,0.550000000000015,49.5595894173749));
#203880=CARTESIAN_POINT('',(117.045701373479,0.550000000000015,49.2651013158452));
#203881=CARTESIAN_POINT('',(117.479271902159,0.550000000000015,49.6549943738242));
#203882=CARTESIAN_POINT('',(117.536514876029,0.550000000000015,49.3605062722945));
#203883=CARTESIAN_POINT('Origin',(117.045701373479,0.550000000000015,49.2651013158452));
#203884=CARTESIAN_POINT('',(116.98845839961,0.550000000000015,49.5595894173749));
#203885=CARTESIAN_POINT('',(117.045701373479,0.550000000000015,49.2651013158452));
#203886=CARTESIAN_POINT('Origin',(117.329270107334,1.45439216225896E-14,
49.11647839305));
#203887=CARTESIAN_POINT('Origin',(117.233865150885,1.45439216225896E-14,
49.6072918955995));
#203888=CARTESIAN_POINT('',(116.98845839961,0.250000000000015,49.5595894173749));
#203889=CARTESIAN_POINT('',(117.479271902159,0.250000000000015,49.6549943738242));
#203890=CARTESIAN_POINT('',(116.98845839961,0.250000000000015,49.5595894173749));
#203891=CARTESIAN_POINT('',(117.479271902159,-0.249999999999985,49.6549943738242));
#203892=CARTESIAN_POINT('',(117.479271902159,0.250000000000015,49.6549943738242));
#203893=CARTESIAN_POINT('',(116.98845839961,-0.249999999999985,49.5595894173749));
#203894=CARTESIAN_POINT('',(117.479271902159,-0.249999999999985,49.6549943738242));
#203895=CARTESIAN_POINT('',(116.98845839961,-0.249999999999985,49.5595894173749));
#203896=CARTESIAN_POINT('Origin',(117.045701373479,0.250000000000015,49.2651013158452));
#203897=CARTESIAN_POINT('',(117.536514876029,0.250000000000015,49.3605062722945));
#203898=CARTESIAN_POINT('',(117.536514876029,0.250000000000015,49.3605062722945));
#203899=CARTESIAN_POINT('',(117.045701373479,0.250000000000015,49.2651013158452));
#203900=CARTESIAN_POINT('',(117.045701373479,0.250000000000015,49.2651013158452));
#203901=CARTESIAN_POINT('',(117.045701373479,0.250000000000015,49.2651013158452));
#203902=CARTESIAN_POINT('Origin',(117.536514876029,0.250000000000015,49.3605062722945));
#203903=CARTESIAN_POINT('',(117.536514876029,-0.249999999999985,49.3605062722945));
#203904=CARTESIAN_POINT('',(117.536514876029,-0.249999999999985,49.3605062722945));
#203905=CARTESIAN_POINT('',(117.536514876029,0.250000000000015,49.3605062722945));
#203906=CARTESIAN_POINT('Origin',(117.536514876029,-0.249999999999985,49.3605062722945));
#203907=CARTESIAN_POINT('',(117.045701373479,-0.249999999999985,49.2651013158452));
#203908=CARTESIAN_POINT('',(117.045701373479,-0.249999999999985,49.2651013158452));
#203909=CARTESIAN_POINT('',(117.536514876029,-0.249999999999985,49.3605062722945));
#203910=CARTESIAN_POINT('Origin',(117.045701373479,-0.249999999999985,49.2651013158452));
#203911=CARTESIAN_POINT('',(117.045701373479,-0.249999999999985,49.2651013158452));
#203912=CARTESIAN_POINT('Origin',(117.291108124754,1.45439216225896E-14,
49.3128037940698));
#203913=CARTESIAN_POINT('Origin',(117.386513081203,1.45439216225896E-14,
48.8219902915203));
#203914=CARTESIAN_POINT('Origin',(130.840764973451,4.75,59.7907234006794));
#203915=CARTESIAN_POINT('',(106.028205189486,4.75,54.9676262909074));
#203916=CARTESIAN_POINT('Origin',(130.840764973451,4.75,59.7907234006794));
#203917=CARTESIAN_POINT('',(125.940727510725,4.75,58.8382478507959));
#203918=CARTESIAN_POINT('Origin',(130.554550104103,-4.75,61.2631639083279));
#203919=CARTESIAN_POINT('',(105.741990320138,4.75,56.4400667985559));
#203920=CARTESIAN_POINT('Origin',(130.554550104103,-4.75,61.2631639083279));
#203921=CARTESIAN_POINT('',(125.654512641377,4.75,60.3106883584444));
#203922=CARTESIAN_POINT('Origin',(130.697657538777,4.75,60.5269436545036));
#203923=CARTESIAN_POINT('Origin',(130.697657538777,4.75,60.5269436545036));
#203924=CARTESIAN_POINT('Origin',(120.198385200308,15.3,59.2501193272487));
#203925=CARTESIAN_POINT('',(110.872928651868,10.30824912388,57.4374251547129));
#203926=CARTESIAN_POINT('Origin',(120.198385200308,15.3,59.2501193272487));
#203927=CARTESIAN_POINT('',(110.872928651868,-9.97697348898999,57.4374251547129));
#203928=CARTESIAN_POINT('Origin',(111.159143521215,15.3,55.9649846470644));
#203929=CARTESIAN_POINT('',(111.159143521215,10.30824912388,55.9649846470644));
#203930=CARTESIAN_POINT('Origin',(111.159143521215,15.3,55.9649846470644));
#203931=CARTESIAN_POINT('',(111.159143521215,-9.97697348898999,55.9649846470644));
#203932=CARTESIAN_POINT('Origin',(111.016036086541,15.3,56.7012049008886));
#203933=CARTESIAN_POINT('Origin',(111.016036086541,15.3,56.7012049008886));
#203934=CARTESIAN_POINT('Origin',(114.581607361595,1.45439216225896E-14,
63.2519072664759));
#203935=CARTESIAN_POINT('',(123.565639834831,1.45439216225896E-14,64.998234990541));
#203936=CARTESIAN_POINT('Origin',(114.581607361595,1.45439216225896E-14,
63.2519072664759));
#203937=CARTESIAN_POINT('Origin',(116.959178380441,1.45439216225896E-14,
51.0204257716897));
#203938=CARTESIAN_POINT('',(114.699588927787,0.200000000000015,66.3135202594736));
#203939=CARTESIAN_POINT('',(114.205996738637,0.200000000000015,66.2324103349957));
#203940=CARTESIAN_POINT('Origin',(116.959178380441,0.200000000000015,51.0204257716897));
#203941=CARTESIAN_POINT('',(114.702370237086,0.700000000000015,66.2992117349507));
#203942=CARTESIAN_POINT('Origin',(117.64631728401,1.45439216225896E-14,
51.1539927107186));
#203943=CARTESIAN_POINT('',(114.208775425237,0.700000000000015,66.2181153030243));
#203944=CARTESIAN_POINT('Origin',(116.959178380441,0.700000000000015,51.0204257716897));
#203945=CARTESIAN_POINT('Origin',(117.155503781461,1.45439216225896E-14,
51.0585877542694));
#203946=CARTESIAN_POINT('Origin',(114.720689788746,0.200000000000015,63.5845573505853));
#203947=CARTESIAN_POINT('',(114.642283596451,0.200000000000015,66.6083291607529));
#203948=CARTESIAN_POINT('',(114.699588927787,0.200000000000015,66.3135202594736));
#203949=CARTESIAN_POINT('',(114.148744365364,0.200000000000015,66.5269467920214));
#203950=CARTESIAN_POINT('',(114.205996738637,0.200000000000015,66.2324103349957));
#203951=CARTESIAN_POINT('Origin',(116.959178380441,0.200000000000015,51.0204257716897));
#203952=CARTESIAN_POINT('Origin',(115.211503291295,0.200000000000015,63.6799623070345));
#203953=CARTESIAN_POINT('',(114.64501180044,0.700000000000015,66.5942938380051));
#203954=CARTESIAN_POINT('',(114.702370237086,0.700000000000015,66.2992117349507));
#203955=CARTESIAN_POINT('Origin',(117.64631728401,1.45439216225896E-14,
51.1539927107186));
#203956=CARTESIAN_POINT('Origin',(115.211503291295,0.700000000000015,63.6799623070345));
#203957=CARTESIAN_POINT('',(114.151470093902,0.700000000000015,66.5129242043036));
#203958=CARTESIAN_POINT('',(114.208775425237,0.700000000000015,66.2181153030243));
#203959=CARTESIAN_POINT('Origin',(116.959178380441,0.700000000000015,51.0204257716897));
#203960=CARTESIAN_POINT('Origin',(114.720689788746,0.700000000000015,63.5845573505853));
#203961=CARTESIAN_POINT('Origin',(117.155503781461,1.45439216225896E-14,
51.0585877542694));
#203962=CARTESIAN_POINT('Origin',(116.959178380441,1.45439216225896E-14,
51.0204257716897));
#203963=CARTESIAN_POINT('',(123.604414184892,1.45439216225896E-14,65.3113870623167));
#203964=CARTESIAN_POINT('Origin',(114.524364387726,1.45439216225896E-14,
63.5463953680056));
#203965=CARTESIAN_POINT('Origin',(114.524364387726,1.45439216225896E-14,
63.5463953680056));
#221644=UNCERTAINTY_MEASURE_WITH_UNIT(LENGTH_MEASURE(0.01),#221663,
'DISTANCE_ACCURACY_VALUE',
'Maximum model space distance between geometric entities at asserted c
onnectivities');
#221647=UNCERTAINTY_MEASURE_WITH_UNIT(LENGTH_MEASURE(0.01),#221663,
'DISTANCE_ACCURACY_VALUE',
'Maximum model space distance between geometric entities at asserted c
onnectivities');
#221659=(
GEOMETRIC_REPRESENTATION_CONTEXT(3)
GLOBAL_UNCERTAINTY_ASSIGNED_CONTEXT((#221644))
GLOBAL_UNIT_ASSIGNED_CONTEXT((#221663,#221665,#221666))
REPRESENTATION_CONTEXT('','3D')
);
#221662=(
GEOMETRIC_REPRESENTATION_CONTEXT(3)
GLOBAL_UNCERTAINTY_ASSIGNED_CONTEXT((#221647))
GLOBAL_UNIT_ASSIGNED_CONTEXT((#221663,#221665,#221666))
REPRESENTATION_CONTEXT('','3D')
);
#221663=(
LENGTH_UNIT()
NAMED_UNIT(*)
SI_UNIT(.MILLI.,.METRE.)
);
#221665=(
NAMED_UNIT(*)
PLANE_ANGLE_UNIT()
SI_UNIT($,.RADIAN.)
);
#221666=(
NAMED_UNIT(*)
SI_UNIT($,.STERADIAN.)
SOLID_ANGLE_UNIT()
);
#221678=SHAPE_DEFINITION_REPRESENTATION(#221692,#221719);
#221692=PRODUCT_DEFINITION_SHAPE('',$,#221734);
#221719=SHAPE_REPRESENTATION('',(#80981),#221659);
#221722=PRODUCT_DEFINITION_CONTEXT('part definition',#221766,'design');
#221734=PRODUCT_DEFINITION('2026-10-05-23-02-46-115','Aerator',#221748,
#221722);
#221748=PRODUCT_DEFINITION_FORMATION('',$,#221779);
#221766=APPLICATION_CONTEXT(
'Core Data for Automotive Mechanical Design Process');
#221767=PRODUCT_CONTEXT('part definition',#221766,'mechanical');
#221779=PRODUCT('2026-10-05-23-02-46-115','Aerator',$,(#221767));
#221783=PRESENTATION_STYLE_ASSIGNMENT((#221785));
#221785=SURFACE_STYLE_USAGE(.BOTH.,#221787);
#221787=SURFACE_SIDE_STYLE('',(#221789));
#221789=SURFACE_STYLE_FILL_AREA(#221791);
#221791=FILL_AREA_STYLE('Opaque(202,209,238)',(#221793));
#221793=FILL_AREA_STYLE_COLOUR('Opaque(202,209,238)',#221795);
#221795=COLOUR_RGB('Opaque(202,209,238)', 0.09019608, 0.27058824, 0.51372549);
ENDSEC;
END-ISO-10303-21;
